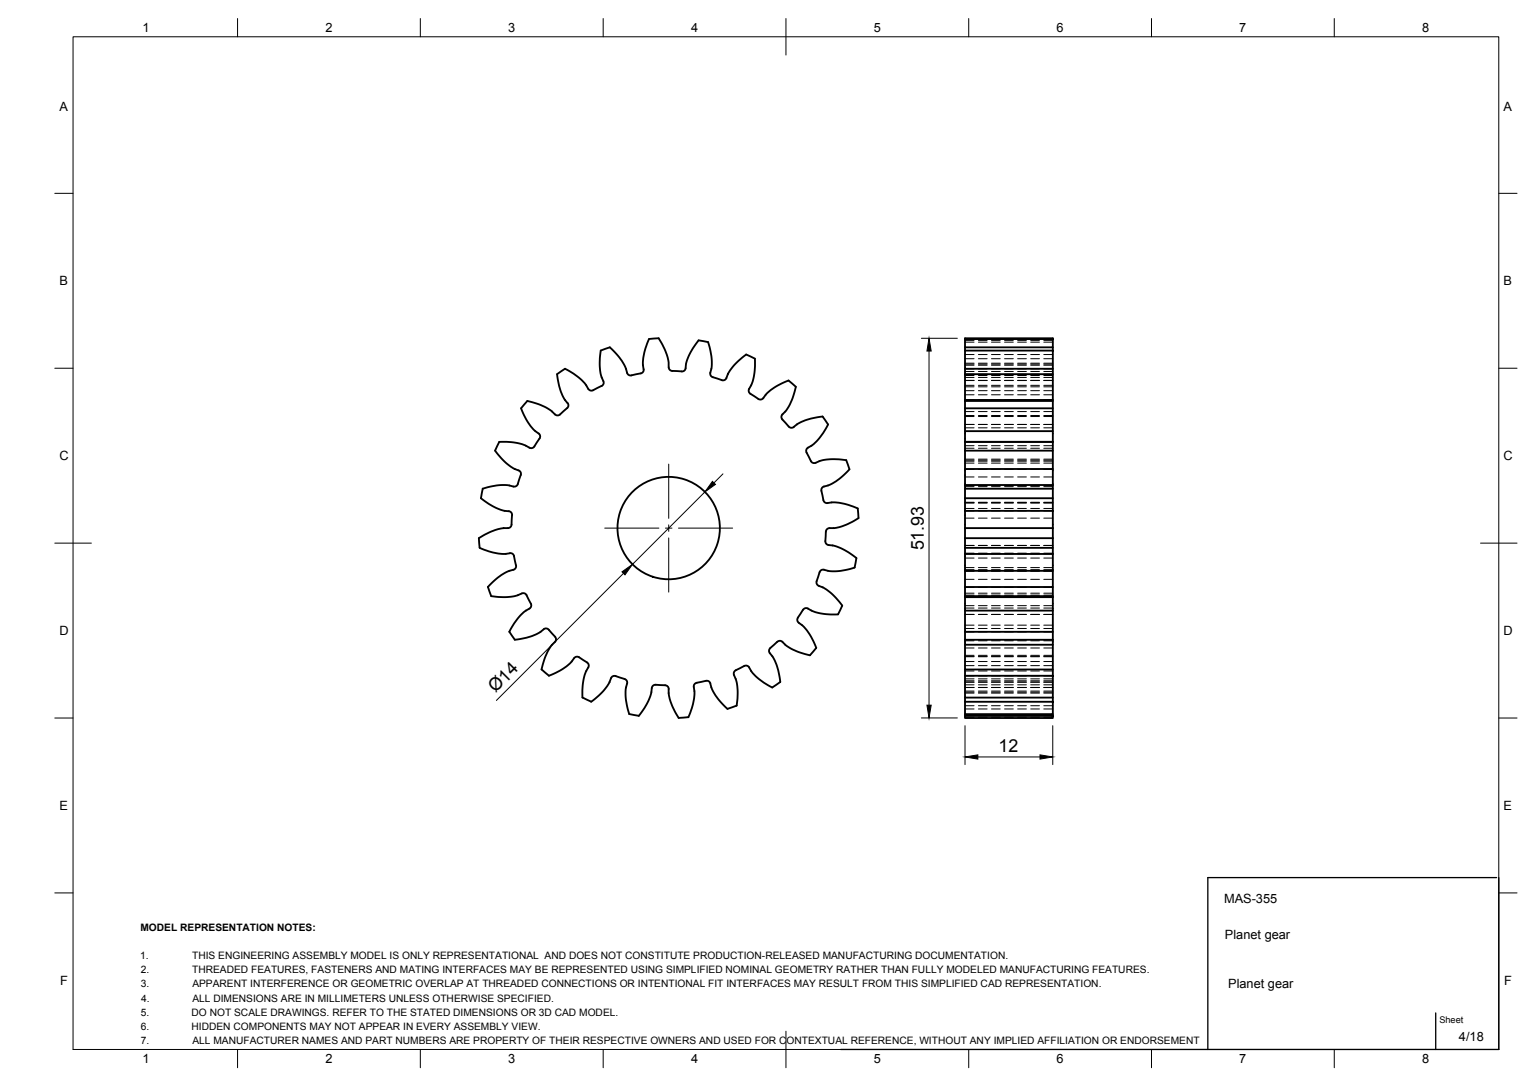
ISO-10303-21;
HEADER;
/* Generated by software containing ST-Developer
 * from STEP Tools, Inc. (www.steptools.com) 
 */

FILE_DESCRIPTION(
/* description */ ('Independent two-stage fixed-ring planetary gearbox,24/24/72 teeth,mod
ule2,20deg involutes,three planets per stage,4:1 x4:1=16:1. Native cut
-space/fillet/pattern tooth profiles derived from reusable gear blanks
; shared sun/planet/ring/carrier parts across both stages. Captured br
onze-journal input/carriers, headed retained planet pins, keyed inters
tage drive and modular keyed output interface. Native ideal gear links
; no torque, precision grade, production backlash/fits, lubrication, s
peed or life rating.'),
/* implementation_level */ '2;1');

FILE_NAME(
/* name */ 'Planet gear.step',
/* time_stamp */ '2026-11-08T19:10:00-08:00',
/* author */ (''),
/* organization */ (''),
/* preprocessor_version */ 'ST-DEVELOPER v20.2',
/* originating_system */ 'Autodesk Translation Framework v15.17.0.0',
/* authorisation */ '');

FILE_SCHEMA (('AUTOMOTIVE_DESIGN { 1 0 10303 214 3 1 1 }'));
ENDSEC;

DATA;
#10=MECHANICAL_DESIGN_GEOMETRIC_PRESENTATION_REPRESENTATION('',(#1169),#259224);
#787=(
BOUNDED_CURVE()
B_SPLINE_CURVE(5,(#216419,#216420,#216421,#216422,#216423,#216424,#216425,
#216426,#216427,#216428,#216429,#216430,#216431,#216432,#216433,#216434,
#216435,#216436,#216437,#216438,#216439,#216440,#216441,#216442,#216443,
#216444,#216445,#216446,#216447,#216448,#216449,#216450,#216451,#216452,
#216453,#216454,#216455,#216456,#216457,#216458,#216459,#216460,#216461,
#216462,#216463,#216464,#216465,#216466,#216467,#216468,#216469,#216470,
#216471,#216472,#216473,#216474,#216475,#216476,#216477,#216478,#216479,
#216480,#216481,#216482,#216483,#216484,#216485,#216486,#216487,#216488,
#216489,#216490,#216491,#216492,#216493,#216494,#216495,#216496,#216497,
#216498,#216499,#216500,#216501,#216502,#216503,#216504,#216505,#216506,
#216507,#216508,#216509,#216510,#216511,#216512,#216513,#216514,#216515,
#216516,#216517,#216518,#216519,#216520,#216521,#216522,#216523,#216524,
#216525,#216526,#216527,#216528,#216529,#216530,#216531,#216532,#216533,
#216534,#216535,#216536,#216537,#216538,#216539,#216540,#216541,#216542,
#216543,#216544,#216545,#216546,#216547,#216548,#216549,#216550,#216551,
#216552,#216553,#216554,#216555,#216556,#216557,#216558,#216559,#216560,
#216561,#216562,#216563,#216564,#216565,#216566,#216567,#216568,#216569,
#216570,#216571,#216572,#216573,#216574,#216575,#216576,#216577,#216578,
#216579,#216580,#216581,#216582,#216583,#216584,#216585,#216586,#216587,
#216588,#216589,#216590,#216591,#216592,#216593,#216594,#216595,#216596,
#216597,#216598,#216599,#216600,#216601,#216602,#216603,#216604,#216605,
#216606,#216607,#216608,#216609,#216610,#216611,#216612,#216613,#216614,
#216615,#216616,#216617,#216618,#216619,#216620,#216621,#216622,#216623),
 .UNSPECIFIED.,.F.,.F.)
B_SPLINE_CURVE_WITH_KNOTS((6,1,1,1,1,1,1,1,1,1,1,1,1,1,1,1,1,1,1,1,1,1,
1,1,1,1,1,1,1,1,1,1,1,1,1,1,1,1,1,1,1,1,1,1,1,1,1,1,1,1,1,1,1,1,1,1,1,1,
1,1,1,1,1,1,1,1,1,1,1,1,1,1,1,1,1,1,1,1,1,1,1,1,1,1,1,1,1,1,1,1,1,1,1,1,
1,1,1,1,1,1,1,1,1,1,1,1,1,1,1,1,1,1,1,1,1,1,1,1,1,1,1,1,1,1,1,1,1,1,1,1,
1,1,1,1,1,1,1,1,1,1,1,1,1,1,1,1,1,1,1,1,1,1,1,1,1,1,1,1,1,1,1,1,1,1,1,1,
1,1,1,1,1,1,1,1,1,1,1,1,1,1,1,1,1,1,1,1,1,1,1,1,1,1,1,1,1,1,1,1,1,1,6),
(-1.,-0.995000000000001,-0.990000000000001,-0.985000000000001,-0.980000000000001,
-0.975000000000001,-0.970000000000001,-0.965000000000001,-0.960000000000001,
-0.955000000000001,-0.950000000000001,-0.945000000000001,-0.940000000000001,
-0.935000000000001,-0.930000000000001,-0.925000000000001,-0.920000000000001,
-0.915000000000001,-0.910000000000001,-0.905000000000001,-0.900000000000001,
-0.895000000000001,-0.890000000000001,-0.885000000000001,-0.880000000000001,
-0.875000000000001,-0.870000000000001,-0.865000000000001,-0.860000000000001,
-0.855000000000001,-0.850000000000001,-0.845000000000001,-0.840000000000001,
-0.835000000000001,-0.830000000000001,-0.825000000000001,-0.820000000000001,
-0.815000000000001,-0.810000000000001,-0.805000000000001,-0.800000000000001,
-0.795000000000001,-0.790000000000001,-0.785000000000001,-0.780000000000001,
-0.775000000000001,-0.770000000000001,-0.765000000000001,-0.760000000000001,
-0.755000000000001,-0.750000000000001,-0.745000000000001,-0.740000000000001,
-0.735000000000001,-0.730000000000001,-0.725000000000001,-0.720000000000001,
-0.715000000000001,-0.710000000000001,-0.705000000000001,-0.700000000000001,
-0.695000000000001,-0.690000000000001,-0.685,-0.68,-0.675,-0.67,-0.665,
-0.66,-0.655,-0.65,-0.645,-0.64,-0.635,-0.63,-0.625,-0.62,-0.615,-0.61,
-0.605,-0.6,-0.595,-0.59,-0.585,-0.58,-0.575,-0.57,-0.565,-0.56,-0.555,
-0.55,-0.545,-0.54,-0.535,-0.53,-0.525,-0.52,-0.515,-0.51,-0.505,-0.5,-0.495,
-0.49,-0.485,-0.48,-0.475,-0.47,-0.465,-0.46,-0.455,-0.45,-0.445,-0.44,
-0.435,-0.43,-0.425,-0.42,-0.415,-0.41,-0.405,-0.4,-0.395,-0.39,-0.385,
-0.38,-0.375,-0.37,-0.365,-0.36,-0.355,-0.35,-0.345,-0.34,-0.335,-0.33,
-0.325,-0.32,-0.315,-0.31,-0.305,-0.3,-0.295,-0.29,-0.285,-0.28,-0.275,
-0.27,-0.265,-0.26,-0.255,-0.25,-0.245,-0.24,-0.235,-0.23,-0.225,-0.22,
-0.215,-0.21,-0.205,-0.2,-0.195,-0.19,-0.185,-0.18,-0.175,-0.17,-0.165,
-0.16,-0.155,-0.15,-0.145,-0.14,-0.135,-0.13,-0.125,-0.12,-0.115,-0.11,
-0.105,-0.1,-0.095,-0.09,-0.085,-0.08,-0.075,-0.07,-0.065,-0.06,-0.055,
-0.05,-0.045,-0.04,-0.035,-0.03,-0.025,-0.02,-0.015,-0.01,-0.005,0.),
 .UNSPECIFIED.)
CURVE()
GEOMETRIC_REPRESENTATION_ITEM()
RATIONAL_B_SPLINE_CURVE((1.,1.,1.,1.,1.,1.,1.,1.,1.,1.,1.,1.,1.,1.,1.,1.,
1.,1.,1.,1.,1.,1.,1.,1.,1.,1.,1.,1.,1.,1.,1.,1.,1.,1.,1.,1.,1.,1.,1.,1.,
1.,1.,1.,1.,1.,1.,1.,1.,1.,1.,1.,1.,1.,1.,1.,1.,1.,1.,1.,1.,1.,1.,1.,1.,
1.,1.,1.,1.,1.,1.,1.,1.,1.,1.,1.,1.,1.,1.,1.,1.,1.,1.,1.,1.,1.,1.,1.,1.,
1.,1.,1.,1.,1.,1.,1.,1.,1.,1.,1.,1.,1.,1.,1.,1.,1.,1.,1.,1.,1.,1.,1.,1.,
1.,1.,1.,1.,1.,1.,1.,1.,1.,1.,1.,1.,1.,1.,1.,1.,1.,1.,1.,1.,1.,1.,1.,1.,
1.,1.,1.,1.,1.,1.,1.,1.,1.,1.,1.,1.,1.,1.,1.,1.,1.,1.,1.,1.,1.,1.,1.,1.,
1.,1.,1.,1.,1.,1.,1.,1.,1.,1.,1.,1.,1.,1.,1.,1.,1.,1.,1.,1.,1.,1.,1.,1.,
1.,1.,1.,1.,1.,1.,1.,1.,1.,1.,1.,1.,1.,1.,1.,1.,1.,1.,1.,1.,1.))
REPRESENTATION_ITEM('')
);
#788=(
BOUNDED_CURVE()
B_SPLINE_CURVE(5,(#216626,#216627,#216628,#216629,#216630,#216631,#216632,
#216633,#216634,#216635,#216636,#216637,#216638,#216639,#216640,#216641,
#216642,#216643,#216644,#216645,#216646,#216647,#216648,#216649,#216650,
#216651,#216652,#216653,#216654,#216655,#216656,#216657,#216658,#216659,
#216660,#216661,#216662,#216663,#216664,#216665,#216666,#216667,#216668,
#216669,#216670,#216671,#216672,#216673,#216674,#216675,#216676,#216677,
#216678,#216679,#216680,#216681,#216682,#216683,#216684,#216685,#216686,
#216687,#216688,#216689,#216690,#216691,#216692,#216693,#216694,#216695,
#216696,#216697,#216698,#216699,#216700,#216701,#216702,#216703,#216704,
#216705,#216706,#216707,#216708,#216709,#216710,#216711,#216712,#216713,
#216714,#216715,#216716,#216717,#216718,#216719,#216720,#216721,#216722,
#216723,#216724,#216725,#216726,#216727,#216728,#216729,#216730,#216731,
#216732,#216733,#216734,#216735,#216736,#216737,#216738,#216739,#216740,
#216741,#216742,#216743,#216744,#216745,#216746,#216747,#216748,#216749,
#216750,#216751,#216752,#216753,#216754,#216755,#216756,#216757,#216758,
#216759,#216760,#216761,#216762,#216763,#216764,#216765,#216766,#216767,
#216768,#216769,#216770,#216771,#216772,#216773,#216774,#216775,#216776,
#216777,#216778,#216779,#216780,#216781,#216782,#216783,#216784,#216785,
#216786,#216787,#216788,#216789,#216790,#216791,#216792,#216793,#216794,
#216795,#216796,#216797,#216798,#216799,#216800,#216801,#216802,#216803,
#216804,#216805,#216806,#216807,#216808,#216809,#216810,#216811,#216812,
#216813,#216814,#216815,#216816,#216817,#216818,#216819,#216820,#216821,
#216822,#216823,#216824,#216825,#216826,#216827,#216828,#216829,#216830),
 .UNSPECIFIED.,.F.,.F.)
B_SPLINE_CURVE_WITH_KNOTS((6,1,1,1,1,1,1,1,1,1,1,1,1,1,1,1,1,1,1,1,1,1,
1,1,1,1,1,1,1,1,1,1,1,1,1,1,1,1,1,1,1,1,1,1,1,1,1,1,1,1,1,1,1,1,1,1,1,1,
1,1,1,1,1,1,1,1,1,1,1,1,1,1,1,1,1,1,1,1,1,1,1,1,1,1,1,1,1,1,1,1,1,1,1,1,
1,1,1,1,1,1,1,1,1,1,1,1,1,1,1,1,1,1,1,1,1,1,1,1,1,1,1,1,1,1,1,1,1,1,1,1,
1,1,1,1,1,1,1,1,1,1,1,1,1,1,1,1,1,1,1,1,1,1,1,1,1,1,1,1,1,1,1,1,1,1,1,1,
1,1,1,1,1,1,1,1,1,1,1,1,1,1,1,1,1,1,1,1,1,1,1,1,1,1,1,1,1,1,1,1,1,1,6),
(0.,0.005,0.01,0.015,0.02,0.025,0.03,0.035,0.04,0.045,0.05,0.055,0.06,0.065,
0.07,0.075,0.08,0.085,0.09,0.095,0.1,0.105,0.11,0.115,0.12,0.125,0.13,0.135,
0.14,0.145,0.15,0.155,0.16,0.165,0.17,0.175,0.18,0.185,0.19,0.195,0.2,0.205,
0.21,0.215,0.22,0.225,0.23,0.235,0.24,0.245,0.25,0.255,0.26,0.265,0.27,
0.275,0.28,0.285,0.29,0.295,0.3,0.305,0.31,0.315,0.32,0.325,0.33,0.335,
0.34,0.345,0.35,0.355,0.36,0.365,0.37,0.375,0.38,0.385,0.39,0.395,0.4,0.405,
0.41,0.415,0.42,0.425,0.43,0.435,0.44,0.445,0.45,0.455,0.46,0.465,0.47,
0.475,0.48,0.485,0.49,0.495,0.5,0.505,0.51,0.515,0.52,0.525,0.53,0.535,
0.54,0.545,0.55,0.555,0.56,0.565,0.57,0.575,0.58,0.585,0.59,0.595,0.6,0.605,
0.61,0.615,0.62,0.625,0.63,0.635,0.64,0.645,0.65,0.655,0.66,0.665,0.67,
0.675,0.68,0.685,0.690000000000001,0.695000000000001,0.700000000000001,
0.705000000000001,0.710000000000001,0.715000000000001,0.720000000000001,
0.725000000000001,0.730000000000001,0.735000000000001,0.740000000000001,
0.745000000000001,0.750000000000001,0.755000000000001,0.760000000000001,
0.765000000000001,0.770000000000001,0.775000000000001,0.780000000000001,
0.785000000000001,0.790000000000001,0.795000000000001,0.800000000000001,
0.805000000000001,0.810000000000001,0.815000000000001,0.820000000000001,
0.825000000000001,0.830000000000001,0.835000000000001,0.840000000000001,
0.845000000000001,0.850000000000001,0.855000000000001,0.860000000000001,
0.865000000000001,0.870000000000001,0.875000000000001,0.880000000000001,
0.885000000000001,0.890000000000001,0.895000000000001,0.900000000000001,
0.905000000000001,0.910000000000001,0.915000000000001,0.920000000000001,
0.925000000000001,0.930000000000001,0.935000000000001,0.940000000000001,
0.945000000000001,0.950000000000001,0.955000000000001,0.960000000000001,
0.965000000000001,0.970000000000001,0.975000000000001,0.980000000000001,
0.985000000000001,0.990000000000001,0.995000000000001,1.),.UNSPECIFIED.)
CURVE()
GEOMETRIC_REPRESENTATION_ITEM()
RATIONAL_B_SPLINE_CURVE((1.,1.,1.,1.,1.,1.,1.,1.,1.,1.,1.,1.,1.,1.,1.,1.,
1.,1.,1.,1.,1.,1.,1.,1.,1.,1.,1.,1.,1.,1.,1.,1.,1.,1.,1.,1.,1.,1.,1.,1.,
1.,1.,1.,1.,1.,1.,1.,1.,1.,1.,1.,1.,1.,1.,1.,1.,1.,1.,1.,1.,1.,1.,1.,1.,
1.,1.,1.,1.,1.,1.,1.,1.,1.,1.,1.,1.,1.,1.,1.,1.,1.,1.,1.,1.,1.,1.,1.,1.,
1.,1.,1.,1.,1.,1.,1.,1.,1.,1.,1.,1.,1.,1.,1.,1.,1.,1.,1.,1.,1.,1.,1.,1.,
1.,1.,1.,1.,1.,1.,1.,1.,1.,1.,1.,1.,1.,1.,1.,1.,1.,1.,1.,1.,1.,1.,1.,1.,
1.,1.,1.,1.,1.,1.,1.,1.,1.,1.,1.,1.,1.,1.,1.,1.,1.,1.,1.,1.,1.,1.,1.,1.,
1.,1.,1.,1.,1.,1.,1.,1.,1.,1.,1.,1.,1.,1.,1.,1.,1.,1.,1.,1.,1.,1.,1.,1.,
1.,1.,1.,1.,1.,1.,1.,1.,1.,1.,1.,1.,1.,1.,1.,1.,1.,1.,1.,1.,1.))
REPRESENTATION_ITEM('')
);
#789=(
BOUNDED_CURVE()
B_SPLINE_CURVE(5,(#217242,#217243,#217244,#217245,#217246,#217247,#217248,
#217249,#217250,#217251,#217252,#217253,#217254,#217255,#217256,#217257,
#217258,#217259,#217260,#217261,#217262,#217263,#217264,#217265,#217266,
#217267,#217268,#217269,#217270,#217271,#217272,#217273,#217274,#217275,
#217276,#217277,#217278,#217279,#217280,#217281,#217282,#217283,#217284,
#217285,#217286,#217287,#217288,#217289,#217290,#217291,#217292,#217293,
#217294,#217295,#217296,#217297,#217298,#217299,#217300,#217301,#217302,
#217303,#217304,#217305,#217306,#217307,#217308,#217309,#217310,#217311,
#217312,#217313,#217314,#217315,#217316,#217317,#217318,#217319,#217320,
#217321,#217322,#217323,#217324,#217325,#217326,#217327,#217328,#217329,
#217330,#217331,#217332,#217333,#217334,#217335,#217336,#217337,#217338,
#217339,#217340,#217341,#217342,#217343,#217344,#217345,#217346,#217347,
#217348,#217349,#217350,#217351,#217352,#217353,#217354,#217355,#217356,
#217357,#217358,#217359,#217360,#217361,#217362,#217363,#217364,#217365,
#217366,#217367,#217368,#217369,#217370,#217371,#217372,#217373,#217374,
#217375,#217376,#217377,#217378,#217379,#217380,#217381,#217382,#217383,
#217384,#217385,#217386,#217387,#217388,#217389,#217390,#217391,#217392,
#217393,#217394,#217395,#217396,#217397,#217398,#217399,#217400,#217401,
#217402,#217403,#217404,#217405,#217406,#217407,#217408,#217409,#217410,
#217411,#217412,#217413,#217414,#217415,#217416,#217417,#217418,#217419,
#217420,#217421,#217422,#217423,#217424,#217425,#217426,#217427,#217428,
#217429,#217430,#217431,#217432,#217433,#217434,#217435,#217436,#217437,
#217438,#217439,#217440,#217441,#217442,#217443,#217444,#217445,#217446),
 .UNSPECIFIED.,.F.,.F.)
B_SPLINE_CURVE_WITH_KNOTS((6,1,1,1,1,1,1,1,1,1,1,1,1,1,1,1,1,1,1,1,1,1,
1,1,1,1,1,1,1,1,1,1,1,1,1,1,1,1,1,1,1,1,1,1,1,1,1,1,1,1,1,1,1,1,1,1,1,1,
1,1,1,1,1,1,1,1,1,1,1,1,1,1,1,1,1,1,1,1,1,1,1,1,1,1,1,1,1,1,1,1,1,1,1,1,
1,1,1,1,1,1,1,1,1,1,1,1,1,1,1,1,1,1,1,1,1,1,1,1,1,1,1,1,1,1,1,1,1,1,1,1,
1,1,1,1,1,1,1,1,1,1,1,1,1,1,1,1,1,1,1,1,1,1,1,1,1,1,1,1,1,1,1,1,1,1,1,1,
1,1,1,1,1,1,1,1,1,1,1,1,1,1,1,1,1,1,1,1,1,1,1,1,1,1,1,1,1,1,1,1,1,1,6),
(0.,0.005,0.01,0.015,0.02,0.025,0.03,0.035,0.04,0.045,0.05,0.055,0.06,0.065,
0.07,0.075,0.08,0.085,0.09,0.095,0.1,0.105,0.11,0.115,0.12,0.125,0.13,0.135,
0.14,0.145,0.15,0.155,0.16,0.165,0.17,0.175,0.18,0.185,0.19,0.195,0.2,0.205,
0.21,0.215,0.22,0.225,0.23,0.235,0.24,0.245,0.25,0.255,0.26,0.265,0.27,
0.275,0.28,0.285,0.29,0.295,0.3,0.305,0.31,0.315,0.32,0.325,0.33,0.335,
0.34,0.345,0.35,0.355,0.36,0.365,0.37,0.375,0.38,0.385,0.39,0.395,0.4,0.405,
0.41,0.415,0.42,0.425,0.43,0.435,0.44,0.445,0.45,0.455,0.46,0.465,0.47,
0.475,0.48,0.485,0.49,0.495,0.5,0.505,0.51,0.515,0.52,0.525,0.53,0.535,
0.54,0.545,0.55,0.555,0.56,0.565,0.57,0.575,0.58,0.585,0.59,0.595,0.6,0.605,
0.61,0.615,0.62,0.625,0.63,0.635,0.64,0.645,0.65,0.655,0.66,0.665,0.67,
0.675,0.68,0.685,0.690000000000001,0.695000000000001,0.700000000000001,
0.705000000000001,0.710000000000001,0.715000000000001,0.720000000000001,
0.725000000000001,0.730000000000001,0.735000000000001,0.740000000000001,
0.745000000000001,0.750000000000001,0.755000000000001,0.760000000000001,
0.765000000000001,0.770000000000001,0.775000000000001,0.780000000000001,
0.785000000000001,0.790000000000001,0.795000000000001,0.800000000000001,
0.805000000000001,0.810000000000001,0.815000000000001,0.820000000000001,
0.825000000000001,0.830000000000001,0.835000000000001,0.840000000000001,
0.845000000000001,0.850000000000001,0.855000000000001,0.860000000000001,
0.865000000000001,0.870000000000001,0.875000000000001,0.880000000000001,
0.885000000000001,0.890000000000001,0.895000000000001,0.900000000000001,
0.905000000000001,0.910000000000001,0.915000000000001,0.920000000000001,
0.925000000000001,0.930000000000001,0.935000000000001,0.940000000000001,
0.945000000000001,0.950000000000001,0.955000000000001,0.960000000000001,
0.965000000000001,0.970000000000001,0.975000000000001,0.980000000000001,
0.985000000000001,0.990000000000001,0.995000000000001,1.),.UNSPECIFIED.)
CURVE()
GEOMETRIC_REPRESENTATION_ITEM()
RATIONAL_B_SPLINE_CURVE((1.,1.,1.,1.,1.,1.,1.,1.,1.,1.,1.,1.,1.,1.,1.,1.,
1.,1.,1.,1.,1.,1.,1.,1.,1.,1.,1.,1.,1.,1.,1.,1.,1.,1.,1.,1.,1.,1.,1.,1.,
1.,1.,1.,1.,1.,1.,1.,1.,1.,1.,1.,1.,1.,1.,1.,1.,1.,1.,1.,1.,1.,1.,1.,1.,
1.,1.,1.,1.,1.,1.,1.,1.,1.,1.,1.,1.,1.,1.,1.,1.,1.,1.,1.,1.,1.,1.,1.,1.,
1.,1.,1.,1.,1.,1.,1.,1.,1.,1.,1.,1.,1.,1.,1.,1.,1.,1.,1.,1.,1.,1.,1.,1.,
1.,1.,1.,1.,1.,1.,1.,1.,1.,1.,1.,1.,1.,1.,1.,1.,1.,1.,1.,1.,1.,1.,1.,1.,
1.,1.,1.,1.,1.,1.,1.,1.,1.,1.,1.,1.,1.,1.,1.,1.,1.,1.,1.,1.,1.,1.,1.,1.,
1.,1.,1.,1.,1.,1.,1.,1.,1.,1.,1.,1.,1.,1.,1.,1.,1.,1.,1.,1.,1.,1.,1.,1.,
1.,1.,1.,1.,1.,1.,1.,1.,1.,1.,1.,1.,1.,1.,1.,1.,1.,1.,1.,1.,1.))
REPRESENTATION_ITEM('')
);
#790=(
BOUNDED_CURVE()
B_SPLINE_CURVE(5,(#217448,#217449,#217450,#217451,#217452,#217453,#217454,
#217455,#217456,#217457,#217458,#217459,#217460,#217461,#217462,#217463,
#217464,#217465,#217466,#217467,#217468,#217469,#217470,#217471,#217472,
#217473,#217474,#217475,#217476,#217477,#217478,#217479,#217480,#217481,
#217482,#217483,#217484,#217485,#217486,#217487,#217488,#217489,#217490,
#217491,#217492,#217493,#217494,#217495,#217496,#217497,#217498,#217499,
#217500,#217501,#217502,#217503,#217504,#217505,#217506,#217507,#217508,
#217509,#217510,#217511,#217512,#217513,#217514,#217515,#217516,#217517,
#217518,#217519,#217520,#217521,#217522,#217523,#217524,#217525,#217526,
#217527,#217528,#217529,#217530,#217531,#217532,#217533,#217534,#217535,
#217536,#217537,#217538,#217539,#217540,#217541,#217542,#217543,#217544,
#217545,#217546,#217547,#217548,#217549,#217550,#217551,#217552,#217553,
#217554,#217555,#217556,#217557,#217558,#217559,#217560,#217561,#217562,
#217563,#217564,#217565,#217566,#217567,#217568,#217569,#217570,#217571,
#217572,#217573,#217574,#217575,#217576,#217577,#217578,#217579,#217580,
#217581,#217582,#217583,#217584,#217585,#217586,#217587,#217588,#217589,
#217590,#217591,#217592,#217593,#217594,#217595,#217596,#217597,#217598,
#217599,#217600,#217601,#217602,#217603,#217604,#217605,#217606,#217607,
#217608,#217609,#217610,#217611,#217612,#217613,#217614,#217615,#217616,
#217617,#217618,#217619,#217620,#217621,#217622,#217623,#217624,#217625,
#217626,#217627,#217628,#217629,#217630,#217631,#217632,#217633,#217634,
#217635,#217636,#217637,#217638,#217639,#217640,#217641,#217642,#217643,
#217644,#217645,#217646,#217647,#217648,#217649,#217650,#217651,#217652),
 .UNSPECIFIED.,.F.,.F.)
B_SPLINE_CURVE_WITH_KNOTS((6,1,1,1,1,1,1,1,1,1,1,1,1,1,1,1,1,1,1,1,1,1,
1,1,1,1,1,1,1,1,1,1,1,1,1,1,1,1,1,1,1,1,1,1,1,1,1,1,1,1,1,1,1,1,1,1,1,1,
1,1,1,1,1,1,1,1,1,1,1,1,1,1,1,1,1,1,1,1,1,1,1,1,1,1,1,1,1,1,1,1,1,1,1,1,
1,1,1,1,1,1,1,1,1,1,1,1,1,1,1,1,1,1,1,1,1,1,1,1,1,1,1,1,1,1,1,1,1,1,1,1,
1,1,1,1,1,1,1,1,1,1,1,1,1,1,1,1,1,1,1,1,1,1,1,1,1,1,1,1,1,1,1,1,1,1,1,1,
1,1,1,1,1,1,1,1,1,1,1,1,1,1,1,1,1,1,1,1,1,1,1,1,1,1,1,1,1,1,1,1,1,1,6),
(-1.,-0.995000000000001,-0.990000000000001,-0.985000000000001,-0.980000000000001,
-0.975000000000001,-0.970000000000001,-0.965000000000001,-0.960000000000001,
-0.955000000000001,-0.950000000000001,-0.945000000000001,-0.940000000000001,
-0.935000000000001,-0.930000000000001,-0.925000000000001,-0.920000000000001,
-0.915000000000001,-0.910000000000001,-0.905000000000001,-0.900000000000001,
-0.895000000000001,-0.890000000000001,-0.885000000000001,-0.880000000000001,
-0.875000000000001,-0.870000000000001,-0.865000000000001,-0.860000000000001,
-0.855000000000001,-0.850000000000001,-0.845000000000001,-0.840000000000001,
-0.835000000000001,-0.830000000000001,-0.825000000000001,-0.820000000000001,
-0.815000000000001,-0.810000000000001,-0.805000000000001,-0.800000000000001,
-0.795000000000001,-0.790000000000001,-0.785000000000001,-0.780000000000001,
-0.775000000000001,-0.770000000000001,-0.765000000000001,-0.760000000000001,
-0.755000000000001,-0.750000000000001,-0.745000000000001,-0.740000000000001,
-0.735000000000001,-0.730000000000001,-0.725000000000001,-0.720000000000001,
-0.715000000000001,-0.710000000000001,-0.705000000000001,-0.700000000000001,
-0.695000000000001,-0.690000000000001,-0.685,-0.68,-0.675,-0.67,-0.665,
-0.66,-0.655,-0.65,-0.645,-0.64,-0.635,-0.63,-0.625,-0.62,-0.615,-0.61,
-0.605,-0.6,-0.595,-0.59,-0.585,-0.58,-0.575,-0.57,-0.565,-0.56,-0.555,
-0.55,-0.545,-0.54,-0.535,-0.53,-0.525,-0.52,-0.515,-0.51,-0.505,-0.5,-0.495,
-0.49,-0.485,-0.48,-0.475,-0.47,-0.465,-0.46,-0.455,-0.45,-0.445,-0.44,
-0.435,-0.43,-0.425,-0.42,-0.415,-0.41,-0.405,-0.4,-0.395,-0.39,-0.385,
-0.38,-0.375,-0.37,-0.365,-0.36,-0.355,-0.35,-0.345,-0.34,-0.335,-0.33,
-0.325,-0.32,-0.315,-0.31,-0.305,-0.3,-0.295,-0.29,-0.285,-0.28,-0.275,
-0.27,-0.265,-0.26,-0.255,-0.25,-0.245,-0.24,-0.235,-0.23,-0.225,-0.22,
-0.215,-0.21,-0.205,-0.2,-0.195,-0.19,-0.185,-0.18,-0.175,-0.17,-0.165,
-0.16,-0.155,-0.15,-0.145,-0.14,-0.135,-0.13,-0.125,-0.12,-0.115,-0.11,
-0.105,-0.1,-0.095,-0.09,-0.085,-0.08,-0.075,-0.07,-0.065,-0.06,-0.055,
-0.05,-0.045,-0.04,-0.035,-0.03,-0.025,-0.02,-0.015,-0.01,-0.005,0.),
 .UNSPECIFIED.)
CURVE()
GEOMETRIC_REPRESENTATION_ITEM()
RATIONAL_B_SPLINE_CURVE((1.,1.,1.,1.,1.,1.,1.,1.,1.,1.,1.,1.,1.,1.,1.,1.,
1.,1.,1.,1.,1.,1.,1.,1.,1.,1.,1.,1.,1.,1.,1.,1.,1.,1.,1.,1.,1.,1.,1.,1.,
1.,1.,1.,1.,1.,1.,1.,1.,1.,1.,1.,1.,1.,1.,1.,1.,1.,1.,1.,1.,1.,1.,1.,1.,
1.,1.,1.,1.,1.,1.,1.,1.,1.,1.,1.,1.,1.,1.,1.,1.,1.,1.,1.,1.,1.,1.,1.,1.,
1.,1.,1.,1.,1.,1.,1.,1.,1.,1.,1.,1.,1.,1.,1.,1.,1.,1.,1.,1.,1.,1.,1.,1.,
1.,1.,1.,1.,1.,1.,1.,1.,1.,1.,1.,1.,1.,1.,1.,1.,1.,1.,1.,1.,1.,1.,1.,1.,
1.,1.,1.,1.,1.,1.,1.,1.,1.,1.,1.,1.,1.,1.,1.,1.,1.,1.,1.,1.,1.,1.,1.,1.,
1.,1.,1.,1.,1.,1.,1.,1.,1.,1.,1.,1.,1.,1.,1.,1.,1.,1.,1.,1.,1.,1.,1.,1.,
1.,1.,1.,1.,1.,1.,1.,1.,1.,1.,1.,1.,1.,1.,1.,1.,1.,1.,1.,1.,1.))
REPRESENTATION_ITEM('')
);
#791=(
BOUNDED_CURVE()
B_SPLINE_CURVE(5,(#218071,#218072,#218073,#218074,#218075,#218076,#218077,
#218078,#218079,#218080,#218081,#218082,#218083,#218084,#218085,#218086,
#218087,#218088,#218089,#218090,#218091,#218092,#218093,#218094,#218095,
#218096,#218097,#218098,#218099,#218100,#218101,#218102,#218103,#218104,
#218105,#218106,#218107,#218108,#218109,#218110,#218111,#218112,#218113,
#218114,#218115,#218116,#218117,#218118,#218119,#218120,#218121,#218122,
#218123,#218124,#218125,#218126,#218127,#218128,#218129,#218130,#218131,
#218132,#218133,#218134,#218135,#218136,#218137,#218138,#218139,#218140,
#218141,#218142,#218143,#218144,#218145,#218146,#218147,#218148,#218149,
#218150,#218151,#218152,#218153,#218154,#218155,#218156,#218157,#218158,
#218159,#218160,#218161,#218162,#218163,#218164,#218165,#218166,#218167,
#218168,#218169,#218170,#218171,#218172,#218173,#218174,#218175,#218176,
#218177,#218178,#218179,#218180,#218181,#218182,#218183,#218184,#218185,
#218186,#218187,#218188,#218189,#218190,#218191,#218192,#218193,#218194,
#218195,#218196,#218197,#218198,#218199,#218200,#218201,#218202,#218203,
#218204,#218205,#218206,#218207,#218208,#218209,#218210,#218211,#218212,
#218213,#218214,#218215,#218216,#218217,#218218,#218219,#218220,#218221,
#218222,#218223,#218224,#218225,#218226,#218227,#218228,#218229,#218230,
#218231,#218232,#218233,#218234,#218235,#218236,#218237,#218238,#218239,
#218240,#218241,#218242,#218243,#218244,#218245,#218246,#218247,#218248,
#218249,#218250,#218251,#218252,#218253,#218254,#218255,#218256,#218257,
#218258,#218259,#218260,#218261,#218262,#218263,#218264,#218265,#218266,
#218267,#218268,#218269,#218270,#218271,#218272,#218273,#218274,#218275),
 .UNSPECIFIED.,.F.,.F.)
B_SPLINE_CURVE_WITH_KNOTS((6,1,1,1,1,1,1,1,1,1,1,1,1,1,1,1,1,1,1,1,1,1,
1,1,1,1,1,1,1,1,1,1,1,1,1,1,1,1,1,1,1,1,1,1,1,1,1,1,1,1,1,1,1,1,1,1,1,1,
1,1,1,1,1,1,1,1,1,1,1,1,1,1,1,1,1,1,1,1,1,1,1,1,1,1,1,1,1,1,1,1,1,1,1,1,
1,1,1,1,1,1,1,1,1,1,1,1,1,1,1,1,1,1,1,1,1,1,1,1,1,1,1,1,1,1,1,1,1,1,1,1,
1,1,1,1,1,1,1,1,1,1,1,1,1,1,1,1,1,1,1,1,1,1,1,1,1,1,1,1,1,1,1,1,1,1,1,1,
1,1,1,1,1,1,1,1,1,1,1,1,1,1,1,1,1,1,1,1,1,1,1,1,1,1,1,1,1,1,1,1,1,1,6),
(-1.,-0.995000000000001,-0.990000000000001,-0.985000000000001,-0.980000000000001,
-0.975000000000001,-0.970000000000001,-0.965000000000001,-0.960000000000001,
-0.955000000000001,-0.950000000000001,-0.945000000000001,-0.940000000000001,
-0.935000000000001,-0.930000000000001,-0.925000000000001,-0.920000000000001,
-0.915000000000001,-0.910000000000001,-0.905000000000001,-0.900000000000001,
-0.895000000000001,-0.890000000000001,-0.885000000000001,-0.880000000000001,
-0.875000000000001,-0.870000000000001,-0.865000000000001,-0.860000000000001,
-0.855000000000001,-0.850000000000001,-0.845000000000001,-0.840000000000001,
-0.835000000000001,-0.830000000000001,-0.825000000000001,-0.820000000000001,
-0.815000000000001,-0.810000000000001,-0.805000000000001,-0.800000000000001,
-0.795000000000001,-0.790000000000001,-0.785000000000001,-0.780000000000001,
-0.775000000000001,-0.770000000000001,-0.765000000000001,-0.760000000000001,
-0.755000000000001,-0.750000000000001,-0.745000000000001,-0.740000000000001,
-0.735000000000001,-0.730000000000001,-0.725000000000001,-0.720000000000001,
-0.715000000000001,-0.710000000000001,-0.705000000000001,-0.700000000000001,
-0.695000000000001,-0.690000000000001,-0.685,-0.68,-0.675,-0.67,-0.665,
-0.66,-0.655,-0.65,-0.645,-0.64,-0.635,-0.63,-0.625,-0.62,-0.615,-0.61,
-0.605,-0.6,-0.595,-0.59,-0.585,-0.58,-0.575,-0.57,-0.565,-0.56,-0.555,
-0.55,-0.545,-0.54,-0.535,-0.53,-0.525,-0.52,-0.515,-0.51,-0.505,-0.5,-0.495,
-0.49,-0.485,-0.48,-0.475,-0.47,-0.465,-0.46,-0.455,-0.45,-0.445,-0.44,
-0.435,-0.43,-0.425,-0.42,-0.415,-0.41,-0.405,-0.4,-0.395,-0.39,-0.385,
-0.38,-0.375,-0.37,-0.365,-0.36,-0.355,-0.35,-0.345,-0.34,-0.335,-0.33,
-0.325,-0.32,-0.315,-0.31,-0.305,-0.3,-0.295,-0.29,-0.285,-0.28,-0.275,
-0.27,-0.265,-0.26,-0.255,-0.25,-0.245,-0.24,-0.235,-0.23,-0.225,-0.22,
-0.215,-0.21,-0.205,-0.2,-0.195,-0.19,-0.185,-0.18,-0.175,-0.17,-0.165,
-0.16,-0.155,-0.15,-0.145,-0.14,-0.135,-0.13,-0.125,-0.12,-0.115,-0.11,
-0.105,-0.1,-0.095,-0.09,-0.085,-0.08,-0.075,-0.07,-0.065,-0.06,-0.055,
-0.05,-0.045,-0.04,-0.035,-0.03,-0.025,-0.02,-0.015,-0.01,-0.005,0.),
 .UNSPECIFIED.)
CURVE()
GEOMETRIC_REPRESENTATION_ITEM()
RATIONAL_B_SPLINE_CURVE((1.,1.,1.,1.,1.,1.,1.,1.,1.,1.,1.,1.,1.,1.,1.,1.,
1.,1.,1.,1.,1.,1.,1.,1.,1.,1.,1.,1.,1.,1.,1.,1.,1.,1.,1.,1.,1.,1.,1.,1.,
1.,1.,1.,1.,1.,1.,1.,1.,1.,1.,1.,1.,1.,1.,1.,1.,1.,1.,1.,1.,1.,1.,1.,1.,
1.,1.,1.,1.,1.,1.,1.,1.,1.,1.,1.,1.,1.,1.,1.,1.,1.,1.,1.,1.,1.,1.,1.,1.,
1.,1.,1.,1.,1.,1.,1.,1.,1.,1.,1.,1.,1.,1.,1.,1.,1.,1.,1.,1.,1.,1.,1.,1.,
1.,1.,1.,1.,1.,1.,1.,1.,1.,1.,1.,1.,1.,1.,1.,1.,1.,1.,1.,1.,1.,1.,1.,1.,
1.,1.,1.,1.,1.,1.,1.,1.,1.,1.,1.,1.,1.,1.,1.,1.,1.,1.,1.,1.,1.,1.,1.,1.,
1.,1.,1.,1.,1.,1.,1.,1.,1.,1.,1.,1.,1.,1.,1.,1.,1.,1.,1.,1.,1.,1.,1.,1.,
1.,1.,1.,1.,1.,1.,1.,1.,1.,1.,1.,1.,1.,1.,1.,1.,1.,1.,1.,1.,1.))
REPRESENTATION_ITEM('')
);
#792=(
BOUNDED_CURVE()
B_SPLINE_CURVE(5,(#218278,#218279,#218280,#218281,#218282,#218283,#218284,
#218285,#218286,#218287,#218288,#218289,#218290,#218291,#218292,#218293,
#218294,#218295,#218296,#218297,#218298,#218299,#218300,#218301,#218302,
#218303,#218304,#218305,#218306,#218307,#218308,#218309,#218310,#218311,
#218312,#218313,#218314,#218315,#218316,#218317,#218318,#218319,#218320,
#218321,#218322,#218323,#218324,#218325,#218326,#218327,#218328,#218329,
#218330,#218331,#218332,#218333,#218334,#218335,#218336,#218337,#218338,
#218339,#218340,#218341,#218342,#218343,#218344,#218345,#218346,#218347,
#218348,#218349,#218350,#218351,#218352,#218353,#218354,#218355,#218356,
#218357,#218358,#218359,#218360,#218361,#218362,#218363,#218364,#218365,
#218366,#218367,#218368,#218369,#218370,#218371,#218372,#218373,#218374,
#218375,#218376,#218377,#218378,#218379,#218380,#218381,#218382,#218383,
#218384,#218385,#218386,#218387,#218388,#218389,#218390,#218391,#218392,
#218393,#218394,#218395,#218396,#218397,#218398,#218399,#218400,#218401,
#218402,#218403,#218404,#218405,#218406,#218407,#218408,#218409,#218410,
#218411,#218412,#218413,#218414,#218415,#218416,#218417,#218418,#218419,
#218420,#218421,#218422,#218423,#218424,#218425,#218426,#218427,#218428,
#218429,#218430,#218431,#218432,#218433,#218434,#218435,#218436,#218437,
#218438,#218439,#218440,#218441,#218442,#218443,#218444,#218445,#218446,
#218447,#218448,#218449,#218450,#218451,#218452,#218453,#218454,#218455,
#218456,#218457,#218458,#218459,#218460,#218461,#218462,#218463,#218464,
#218465,#218466,#218467,#218468,#218469,#218470,#218471,#218472,#218473,
#218474,#218475,#218476,#218477,#218478,#218479,#218480,#218481,#218482),
 .UNSPECIFIED.,.F.,.F.)
B_SPLINE_CURVE_WITH_KNOTS((6,1,1,1,1,1,1,1,1,1,1,1,1,1,1,1,1,1,1,1,1,1,
1,1,1,1,1,1,1,1,1,1,1,1,1,1,1,1,1,1,1,1,1,1,1,1,1,1,1,1,1,1,1,1,1,1,1,1,
1,1,1,1,1,1,1,1,1,1,1,1,1,1,1,1,1,1,1,1,1,1,1,1,1,1,1,1,1,1,1,1,1,1,1,1,
1,1,1,1,1,1,1,1,1,1,1,1,1,1,1,1,1,1,1,1,1,1,1,1,1,1,1,1,1,1,1,1,1,1,1,1,
1,1,1,1,1,1,1,1,1,1,1,1,1,1,1,1,1,1,1,1,1,1,1,1,1,1,1,1,1,1,1,1,1,1,1,1,
1,1,1,1,1,1,1,1,1,1,1,1,1,1,1,1,1,1,1,1,1,1,1,1,1,1,1,1,1,1,1,1,1,1,6),
(0.,0.005,0.01,0.015,0.02,0.025,0.03,0.035,0.04,0.045,0.05,0.055,0.06,0.065,
0.07,0.075,0.08,0.085,0.09,0.095,0.1,0.105,0.11,0.115,0.12,0.125,0.13,0.135,
0.14,0.145,0.15,0.155,0.16,0.165,0.17,0.175,0.18,0.185,0.19,0.195,0.2,0.205,
0.21,0.215,0.22,0.225,0.23,0.235,0.24,0.245,0.25,0.255,0.26,0.265,0.27,
0.275,0.28,0.285,0.29,0.295,0.3,0.305,0.31,0.315,0.32,0.325,0.33,0.335,
0.34,0.345,0.35,0.355,0.36,0.365,0.37,0.375,0.38,0.385,0.39,0.395,0.4,0.405,
0.41,0.415,0.42,0.425,0.43,0.435,0.44,0.445,0.45,0.455,0.46,0.465,0.47,
0.475,0.48,0.485,0.49,0.495,0.5,0.505,0.51,0.515,0.52,0.525,0.53,0.535,
0.54,0.545,0.55,0.555,0.56,0.565,0.57,0.575,0.58,0.585,0.59,0.595,0.6,0.605,
0.61,0.615,0.62,0.625,0.63,0.635,0.64,0.645,0.65,0.655,0.66,0.665,0.67,
0.675,0.68,0.685,0.690000000000001,0.695000000000001,0.700000000000001,
0.705000000000001,0.710000000000001,0.715000000000001,0.720000000000001,
0.725000000000001,0.730000000000001,0.735000000000001,0.740000000000001,
0.745000000000001,0.750000000000001,0.755000000000001,0.760000000000001,
0.765000000000001,0.770000000000001,0.775000000000001,0.780000000000001,
0.785000000000001,0.790000000000001,0.795000000000001,0.800000000000001,
0.805000000000001,0.810000000000001,0.815000000000001,0.820000000000001,
0.825000000000001,0.830000000000001,0.835000000000001,0.840000000000001,
0.845000000000001,0.850000000000001,0.855000000000001,0.860000000000001,
0.865000000000001,0.870000000000001,0.875000000000001,0.880000000000001,
0.885000000000001,0.890000000000001,0.895000000000001,0.900000000000001,
0.905000000000001,0.910000000000001,0.915000000000001,0.920000000000001,
0.925000000000001,0.930000000000001,0.935000000000001,0.940000000000001,
0.945000000000001,0.950000000000001,0.955000000000001,0.960000000000001,
0.965000000000001,0.970000000000001,0.975000000000001,0.980000000000001,
0.985000000000001,0.990000000000001,0.995000000000001,1.),.UNSPECIFIED.)
CURVE()
GEOMETRIC_REPRESENTATION_ITEM()
RATIONAL_B_SPLINE_CURVE((1.,1.,1.,1.,1.,1.,1.,1.,1.,1.,1.,1.,1.,1.,1.,1.,
1.,1.,1.,1.,1.,1.,1.,1.,1.,1.,1.,1.,1.,1.,1.,1.,1.,1.,1.,1.,1.,1.,1.,1.,
1.,1.,1.,1.,1.,1.,1.,1.,1.,1.,1.,1.,1.,1.,1.,1.,1.,1.,1.,1.,1.,1.,1.,1.,
1.,1.,1.,1.,1.,1.,1.,1.,1.,1.,1.,1.,1.,1.,1.,1.,1.,1.,1.,1.,1.,1.,1.,1.,
1.,1.,1.,1.,1.,1.,1.,1.,1.,1.,1.,1.,1.,1.,1.,1.,1.,1.,1.,1.,1.,1.,1.,1.,
1.,1.,1.,1.,1.,1.,1.,1.,1.,1.,1.,1.,1.,1.,1.,1.,1.,1.,1.,1.,1.,1.,1.,1.,
1.,1.,1.,1.,1.,1.,1.,1.,1.,1.,1.,1.,1.,1.,1.,1.,1.,1.,1.,1.,1.,1.,1.,1.,
1.,1.,1.,1.,1.,1.,1.,1.,1.,1.,1.,1.,1.,1.,1.,1.,1.,1.,1.,1.,1.,1.,1.,1.,
1.,1.,1.,1.,1.,1.,1.,1.,1.,1.,1.,1.,1.,1.,1.,1.,1.,1.,1.,1.,1.))
REPRESENTATION_ITEM('')
);
#793=(
BOUNDED_CURVE()
B_SPLINE_CURVE(5,(#218894,#218895,#218896,#218897,#218898,#218899,#218900,
#218901,#218902,#218903,#218904,#218905,#218906,#218907,#218908,#218909,
#218910,#218911,#218912,#218913,#218914,#218915,#218916,#218917,#218918,
#218919,#218920,#218921,#218922,#218923,#218924,#218925,#218926,#218927,
#218928,#218929,#218930,#218931,#218932,#218933,#218934,#218935,#218936,
#218937,#218938,#218939,#218940,#218941,#218942,#218943,#218944,#218945,
#218946,#218947,#218948,#218949,#218950,#218951,#218952,#218953,#218954,
#218955,#218956,#218957,#218958,#218959,#218960,#218961,#218962,#218963,
#218964,#218965,#218966,#218967,#218968,#218969,#218970,#218971,#218972,
#218973,#218974,#218975,#218976,#218977,#218978,#218979,#218980,#218981,
#218982,#218983,#218984,#218985,#218986,#218987,#218988,#218989,#218990,
#218991,#218992,#218993,#218994,#218995,#218996,#218997,#218998,#218999,
#219000,#219001,#219002,#219003,#219004,#219005,#219006,#219007,#219008,
#219009,#219010,#219011,#219012,#219013,#219014,#219015,#219016,#219017,
#219018,#219019,#219020,#219021,#219022,#219023,#219024,#219025,#219026,
#219027,#219028,#219029,#219030,#219031,#219032,#219033,#219034,#219035,
#219036,#219037,#219038,#219039,#219040,#219041,#219042,#219043,#219044,
#219045,#219046,#219047,#219048,#219049,#219050,#219051,#219052,#219053,
#219054,#219055,#219056,#219057,#219058,#219059,#219060,#219061,#219062,
#219063,#219064,#219065,#219066,#219067,#219068,#219069,#219070,#219071,
#219072,#219073,#219074,#219075,#219076,#219077,#219078,#219079,#219080,
#219081,#219082,#219083,#219084,#219085,#219086,#219087,#219088,#219089,
#219090,#219091,#219092,#219093,#219094,#219095,#219096,#219097,#219098),
 .UNSPECIFIED.,.F.,.F.)
B_SPLINE_CURVE_WITH_KNOTS((6,1,1,1,1,1,1,1,1,1,1,1,1,1,1,1,1,1,1,1,1,1,
1,1,1,1,1,1,1,1,1,1,1,1,1,1,1,1,1,1,1,1,1,1,1,1,1,1,1,1,1,1,1,1,1,1,1,1,
1,1,1,1,1,1,1,1,1,1,1,1,1,1,1,1,1,1,1,1,1,1,1,1,1,1,1,1,1,1,1,1,1,1,1,1,
1,1,1,1,1,1,1,1,1,1,1,1,1,1,1,1,1,1,1,1,1,1,1,1,1,1,1,1,1,1,1,1,1,1,1,1,
1,1,1,1,1,1,1,1,1,1,1,1,1,1,1,1,1,1,1,1,1,1,1,1,1,1,1,1,1,1,1,1,1,1,1,1,
1,1,1,1,1,1,1,1,1,1,1,1,1,1,1,1,1,1,1,1,1,1,1,1,1,1,1,1,1,1,1,1,1,1,6),
(0.,0.005,0.01,0.015,0.02,0.025,0.03,0.035,0.04,0.045,0.05,0.055,0.06,0.065,
0.07,0.075,0.08,0.085,0.09,0.095,0.1,0.105,0.11,0.115,0.12,0.125,0.13,0.135,
0.14,0.145,0.15,0.155,0.16,0.165,0.17,0.175,0.18,0.185,0.19,0.195,0.2,0.205,
0.21,0.215,0.22,0.225,0.23,0.235,0.24,0.245,0.25,0.255,0.26,0.265,0.27,
0.275,0.28,0.285,0.29,0.295,0.3,0.305,0.31,0.315,0.32,0.325,0.33,0.335,
0.34,0.345,0.35,0.355,0.36,0.365,0.37,0.375,0.38,0.385,0.39,0.395,0.4,0.405,
0.41,0.415,0.42,0.425,0.43,0.435,0.44,0.445,0.45,0.455,0.46,0.465,0.47,
0.475,0.48,0.485,0.49,0.495,0.5,0.505,0.51,0.515,0.52,0.525,0.53,0.535,
0.54,0.545,0.55,0.555,0.56,0.565,0.57,0.575,0.58,0.585,0.59,0.595,0.6,0.605,
0.61,0.615,0.62,0.625,0.63,0.635,0.64,0.645,0.65,0.655,0.66,0.665,0.67,
0.675,0.68,0.685,0.690000000000001,0.695000000000001,0.700000000000001,
0.705000000000001,0.710000000000001,0.715000000000001,0.720000000000001,
0.725000000000001,0.730000000000001,0.735000000000001,0.740000000000001,
0.745000000000001,0.750000000000001,0.755000000000001,0.760000000000001,
0.765000000000001,0.770000000000001,0.775000000000001,0.780000000000001,
0.785000000000001,0.790000000000001,0.795000000000001,0.800000000000001,
0.805000000000001,0.810000000000001,0.815000000000001,0.820000000000001,
0.825000000000001,0.830000000000001,0.835000000000001,0.840000000000001,
0.845000000000001,0.850000000000001,0.855000000000001,0.860000000000001,
0.865000000000001,0.870000000000001,0.875000000000001,0.880000000000001,
0.885000000000001,0.890000000000001,0.895000000000001,0.900000000000001,
0.905000000000001,0.910000000000001,0.915000000000001,0.920000000000001,
0.925000000000001,0.930000000000001,0.935000000000001,0.940000000000001,
0.945000000000001,0.950000000000001,0.955000000000001,0.960000000000001,
0.965000000000001,0.970000000000001,0.975000000000001,0.980000000000001,
0.985000000000001,0.990000000000001,0.995000000000001,1.),.UNSPECIFIED.)
CURVE()
GEOMETRIC_REPRESENTATION_ITEM()
RATIONAL_B_SPLINE_CURVE((1.,1.,1.,1.,1.,1.,1.,1.,1.,1.,1.,1.,1.,1.,1.,1.,
1.,1.,1.,1.,1.,1.,1.,1.,1.,1.,1.,1.,1.,1.,1.,1.,1.,1.,1.,1.,1.,1.,1.,1.,
1.,1.,1.,1.,1.,1.,1.,1.,1.,1.,1.,1.,1.,1.,1.,1.,1.,1.,1.,1.,1.,1.,1.,1.,
1.,1.,1.,1.,1.,1.,1.,1.,1.,1.,1.,1.,1.,1.,1.,1.,1.,1.,1.,1.,1.,1.,1.,1.,
1.,1.,1.,1.,1.,1.,1.,1.,1.,1.,1.,1.,1.,1.,1.,1.,1.,1.,1.,1.,1.,1.,1.,1.,
1.,1.,1.,1.,1.,1.,1.,1.,1.,1.,1.,1.,1.,1.,1.,1.,1.,1.,1.,1.,1.,1.,1.,1.,
1.,1.,1.,1.,1.,1.,1.,1.,1.,1.,1.,1.,1.,1.,1.,1.,1.,1.,1.,1.,1.,1.,1.,1.,
1.,1.,1.,1.,1.,1.,1.,1.,1.,1.,1.,1.,1.,1.,1.,1.,1.,1.,1.,1.,1.,1.,1.,1.,
1.,1.,1.,1.,1.,1.,1.,1.,1.,1.,1.,1.,1.,1.,1.,1.,1.,1.,1.,1.,1.))
REPRESENTATION_ITEM('')
);
#794=(
BOUNDED_CURVE()
B_SPLINE_CURVE(5,(#219100,#219101,#219102,#219103,#219104,#219105,#219106,
#219107,#219108,#219109,#219110,#219111,#219112,#219113,#219114,#219115,
#219116,#219117,#219118,#219119,#219120,#219121,#219122,#219123,#219124,
#219125,#219126,#219127,#219128,#219129,#219130,#219131,#219132,#219133,
#219134,#219135,#219136,#219137,#219138,#219139,#219140,#219141,#219142,
#219143,#219144,#219145,#219146,#219147,#219148,#219149,#219150,#219151,
#219152,#219153,#219154,#219155,#219156,#219157,#219158,#219159,#219160,
#219161,#219162,#219163,#219164,#219165,#219166,#219167,#219168,#219169,
#219170,#219171,#219172,#219173,#219174,#219175,#219176,#219177,#219178,
#219179,#219180,#219181,#219182,#219183,#219184,#219185,#219186,#219187,
#219188,#219189,#219190,#219191,#219192,#219193,#219194,#219195,#219196,
#219197,#219198,#219199,#219200,#219201,#219202,#219203,#219204,#219205,
#219206,#219207,#219208,#219209,#219210,#219211,#219212,#219213,#219214,
#219215,#219216,#219217,#219218,#219219,#219220,#219221,#219222,#219223,
#219224,#219225,#219226,#219227,#219228,#219229,#219230,#219231,#219232,
#219233,#219234,#219235,#219236,#219237,#219238,#219239,#219240,#219241,
#219242,#219243,#219244,#219245,#219246,#219247,#219248,#219249,#219250,
#219251,#219252,#219253,#219254,#219255,#219256,#219257,#219258,#219259,
#219260,#219261,#219262,#219263,#219264,#219265,#219266,#219267,#219268,
#219269,#219270,#219271,#219272,#219273,#219274,#219275,#219276,#219277,
#219278,#219279,#219280,#219281,#219282,#219283,#219284,#219285,#219286,
#219287,#219288,#219289,#219290,#219291,#219292,#219293,#219294,#219295,
#219296,#219297,#219298,#219299,#219300,#219301,#219302,#219303,#219304),
 .UNSPECIFIED.,.F.,.F.)
B_SPLINE_CURVE_WITH_KNOTS((6,1,1,1,1,1,1,1,1,1,1,1,1,1,1,1,1,1,1,1,1,1,
1,1,1,1,1,1,1,1,1,1,1,1,1,1,1,1,1,1,1,1,1,1,1,1,1,1,1,1,1,1,1,1,1,1,1,1,
1,1,1,1,1,1,1,1,1,1,1,1,1,1,1,1,1,1,1,1,1,1,1,1,1,1,1,1,1,1,1,1,1,1,1,1,
1,1,1,1,1,1,1,1,1,1,1,1,1,1,1,1,1,1,1,1,1,1,1,1,1,1,1,1,1,1,1,1,1,1,1,1,
1,1,1,1,1,1,1,1,1,1,1,1,1,1,1,1,1,1,1,1,1,1,1,1,1,1,1,1,1,1,1,1,1,1,1,1,
1,1,1,1,1,1,1,1,1,1,1,1,1,1,1,1,1,1,1,1,1,1,1,1,1,1,1,1,1,1,1,1,1,1,6),
(-1.,-0.995000000000001,-0.990000000000001,-0.985000000000001,-0.980000000000001,
-0.975000000000001,-0.970000000000001,-0.965000000000001,-0.960000000000001,
-0.955000000000001,-0.950000000000001,-0.945000000000001,-0.940000000000001,
-0.935000000000001,-0.930000000000001,-0.925000000000001,-0.920000000000001,
-0.915000000000001,-0.910000000000001,-0.905000000000001,-0.900000000000001,
-0.895000000000001,-0.890000000000001,-0.885000000000001,-0.880000000000001,
-0.875000000000001,-0.870000000000001,-0.865000000000001,-0.860000000000001,
-0.855000000000001,-0.850000000000001,-0.845000000000001,-0.840000000000001,
-0.835000000000001,-0.830000000000001,-0.825000000000001,-0.820000000000001,
-0.815000000000001,-0.810000000000001,-0.805000000000001,-0.800000000000001,
-0.795000000000001,-0.790000000000001,-0.785000000000001,-0.780000000000001,
-0.775000000000001,-0.770000000000001,-0.765000000000001,-0.760000000000001,
-0.755000000000001,-0.750000000000001,-0.745000000000001,-0.740000000000001,
-0.735000000000001,-0.730000000000001,-0.725000000000001,-0.720000000000001,
-0.715000000000001,-0.710000000000001,-0.705000000000001,-0.700000000000001,
-0.695000000000001,-0.690000000000001,-0.685,-0.68,-0.675,-0.67,-0.665,
-0.66,-0.655,-0.65,-0.645,-0.64,-0.635,-0.63,-0.625,-0.62,-0.615,-0.61,
-0.605,-0.6,-0.595,-0.59,-0.585,-0.58,-0.575,-0.57,-0.565,-0.56,-0.555,
-0.55,-0.545,-0.54,-0.535,-0.53,-0.525,-0.52,-0.515,-0.51,-0.505,-0.5,-0.495,
-0.49,-0.485,-0.48,-0.475,-0.47,-0.465,-0.46,-0.455,-0.45,-0.445,-0.44,
-0.435,-0.43,-0.425,-0.42,-0.415,-0.41,-0.405,-0.4,-0.395,-0.39,-0.385,
-0.38,-0.375,-0.37,-0.365,-0.36,-0.355,-0.35,-0.345,-0.34,-0.335,-0.33,
-0.325,-0.32,-0.315,-0.31,-0.305,-0.3,-0.295,-0.29,-0.285,-0.28,-0.275,
-0.27,-0.265,-0.26,-0.255,-0.25,-0.245,-0.24,-0.235,-0.23,-0.225,-0.22,
-0.215,-0.21,-0.205,-0.2,-0.195,-0.19,-0.185,-0.18,-0.175,-0.17,-0.165,
-0.16,-0.155,-0.15,-0.145,-0.14,-0.135,-0.13,-0.125,-0.12,-0.115,-0.11,
-0.105,-0.1,-0.095,-0.09,-0.085,-0.08,-0.075,-0.07,-0.065,-0.06,-0.055,
-0.05,-0.045,-0.04,-0.035,-0.03,-0.025,-0.02,-0.015,-0.01,-0.005,0.),
 .UNSPECIFIED.)
CURVE()
GEOMETRIC_REPRESENTATION_ITEM()
RATIONAL_B_SPLINE_CURVE((1.,1.,1.,1.,1.,1.,1.,1.,1.,1.,1.,1.,1.,1.,1.,1.,
1.,1.,1.,1.,1.,1.,1.,1.,1.,1.,1.,1.,1.,1.,1.,1.,1.,1.,1.,1.,1.,1.,1.,1.,
1.,1.,1.,1.,1.,1.,1.,1.,1.,1.,1.,1.,1.,1.,1.,1.,1.,1.,1.,1.,1.,1.,1.,1.,
1.,1.,1.,1.,1.,1.,1.,1.,1.,1.,1.,1.,1.,1.,1.,1.,1.,1.,1.,1.,1.,1.,1.,1.,
1.,1.,1.,1.,1.,1.,1.,1.,1.,1.,1.,1.,1.,1.,1.,1.,1.,1.,1.,1.,1.,1.,1.,1.,
1.,1.,1.,1.,1.,1.,1.,1.,1.,1.,1.,1.,1.,1.,1.,1.,1.,1.,1.,1.,1.,1.,1.,1.,
1.,1.,1.,1.,1.,1.,1.,1.,1.,1.,1.,1.,1.,1.,1.,1.,1.,1.,1.,1.,1.,1.,1.,1.,
1.,1.,1.,1.,1.,1.,1.,1.,1.,1.,1.,1.,1.,1.,1.,1.,1.,1.,1.,1.,1.,1.,1.,1.,
1.,1.,1.,1.,1.,1.,1.,1.,1.,1.,1.,1.,1.,1.,1.,1.,1.,1.,1.,1.,1.))
REPRESENTATION_ITEM('')
);
#795=(
BOUNDED_CURVE()
B_SPLINE_CURVE(5,(#219723,#219724,#219725,#219726,#219727,#219728,#219729,
#219730,#219731,#219732,#219733,#219734,#219735,#219736,#219737,#219738,
#219739,#219740,#219741,#219742,#219743,#219744,#219745,#219746,#219747,
#219748,#219749,#219750,#219751,#219752,#219753,#219754,#219755,#219756,
#219757,#219758,#219759,#219760,#219761,#219762,#219763,#219764,#219765,
#219766,#219767,#219768,#219769,#219770,#219771,#219772,#219773,#219774,
#219775,#219776,#219777,#219778,#219779,#219780,#219781,#219782,#219783,
#219784,#219785,#219786,#219787,#219788,#219789,#219790,#219791,#219792,
#219793,#219794,#219795,#219796,#219797,#219798,#219799,#219800,#219801,
#219802,#219803,#219804,#219805,#219806,#219807,#219808,#219809,#219810,
#219811,#219812,#219813,#219814,#219815,#219816,#219817,#219818,#219819,
#219820,#219821,#219822,#219823,#219824,#219825,#219826,#219827,#219828,
#219829,#219830,#219831,#219832,#219833,#219834,#219835,#219836,#219837,
#219838,#219839,#219840,#219841,#219842,#219843,#219844,#219845,#219846,
#219847,#219848,#219849,#219850,#219851,#219852,#219853,#219854,#219855,
#219856,#219857,#219858,#219859,#219860,#219861,#219862,#219863,#219864,
#219865,#219866,#219867,#219868,#219869,#219870,#219871,#219872,#219873,
#219874,#219875,#219876,#219877,#219878,#219879,#219880,#219881,#219882,
#219883,#219884,#219885,#219886,#219887,#219888,#219889,#219890,#219891,
#219892,#219893,#219894,#219895,#219896,#219897,#219898,#219899,#219900,
#219901,#219902,#219903,#219904,#219905,#219906,#219907,#219908,#219909,
#219910,#219911,#219912,#219913,#219914,#219915,#219916,#219917,#219918,
#219919,#219920,#219921,#219922,#219923,#219924,#219925,#219926,#219927),
 .UNSPECIFIED.,.F.,.F.)
B_SPLINE_CURVE_WITH_KNOTS((6,1,1,1,1,1,1,1,1,1,1,1,1,1,1,1,1,1,1,1,1,1,
1,1,1,1,1,1,1,1,1,1,1,1,1,1,1,1,1,1,1,1,1,1,1,1,1,1,1,1,1,1,1,1,1,1,1,1,
1,1,1,1,1,1,1,1,1,1,1,1,1,1,1,1,1,1,1,1,1,1,1,1,1,1,1,1,1,1,1,1,1,1,1,1,
1,1,1,1,1,1,1,1,1,1,1,1,1,1,1,1,1,1,1,1,1,1,1,1,1,1,1,1,1,1,1,1,1,1,1,1,
1,1,1,1,1,1,1,1,1,1,1,1,1,1,1,1,1,1,1,1,1,1,1,1,1,1,1,1,1,1,1,1,1,1,1,1,
1,1,1,1,1,1,1,1,1,1,1,1,1,1,1,1,1,1,1,1,1,1,1,1,1,1,1,1,1,1,1,1,1,1,6),
(-1.,-0.995000000000001,-0.990000000000001,-0.985000000000001,-0.980000000000001,
-0.975000000000001,-0.970000000000001,-0.965000000000001,-0.960000000000001,
-0.955000000000001,-0.950000000000001,-0.945000000000001,-0.940000000000001,
-0.935000000000001,-0.930000000000001,-0.925000000000001,-0.920000000000001,
-0.915000000000001,-0.910000000000001,-0.905000000000001,-0.900000000000001,
-0.895000000000001,-0.890000000000001,-0.885000000000001,-0.880000000000001,
-0.875000000000001,-0.870000000000001,-0.865000000000001,-0.860000000000001,
-0.855000000000001,-0.850000000000001,-0.845000000000001,-0.840000000000001,
-0.835000000000001,-0.830000000000001,-0.825000000000001,-0.820000000000001,
-0.815000000000001,-0.810000000000001,-0.805000000000001,-0.800000000000001,
-0.795000000000001,-0.790000000000001,-0.785000000000001,-0.780000000000001,
-0.775000000000001,-0.770000000000001,-0.765000000000001,-0.760000000000001,
-0.755000000000001,-0.750000000000001,-0.745000000000001,-0.740000000000001,
-0.735000000000001,-0.730000000000001,-0.725000000000001,-0.720000000000001,
-0.715000000000001,-0.710000000000001,-0.705000000000001,-0.700000000000001,
-0.695000000000001,-0.690000000000001,-0.685,-0.68,-0.675,-0.67,-0.665,
-0.66,-0.655,-0.65,-0.645,-0.64,-0.635,-0.63,-0.625,-0.62,-0.615,-0.61,
-0.605,-0.6,-0.595,-0.59,-0.585,-0.58,-0.575,-0.57,-0.565,-0.56,-0.555,
-0.55,-0.545,-0.54,-0.535,-0.53,-0.525,-0.52,-0.515,-0.51,-0.505,-0.5,-0.495,
-0.49,-0.485,-0.48,-0.475,-0.47,-0.465,-0.46,-0.455,-0.45,-0.445,-0.44,
-0.435,-0.43,-0.425,-0.42,-0.415,-0.41,-0.405,-0.4,-0.395,-0.39,-0.385,
-0.38,-0.375,-0.37,-0.365,-0.36,-0.355,-0.35,-0.345,-0.34,-0.335,-0.33,
-0.325,-0.32,-0.315,-0.31,-0.305,-0.3,-0.295,-0.29,-0.285,-0.28,-0.275,
-0.27,-0.265,-0.26,-0.255,-0.25,-0.245,-0.24,-0.235,-0.23,-0.225,-0.22,
-0.215,-0.21,-0.205,-0.2,-0.195,-0.19,-0.185,-0.18,-0.175,-0.17,-0.165,
-0.16,-0.155,-0.15,-0.145,-0.14,-0.135,-0.13,-0.125,-0.12,-0.115,-0.11,
-0.105,-0.1,-0.095,-0.09,-0.085,-0.08,-0.075,-0.07,-0.065,-0.06,-0.055,
-0.05,-0.045,-0.04,-0.035,-0.03,-0.025,-0.02,-0.015,-0.01,-0.005,0.),
 .UNSPECIFIED.)
CURVE()
GEOMETRIC_REPRESENTATION_ITEM()
RATIONAL_B_SPLINE_CURVE((1.,1.,1.,1.,1.,1.,1.,1.,1.,1.,1.,1.,1.,1.,1.,1.,
1.,1.,1.,1.,1.,1.,1.,1.,1.,1.,1.,1.,1.,1.,1.,1.,1.,1.,1.,1.,1.,1.,1.,1.,
1.,1.,1.,1.,1.,1.,1.,1.,1.,1.,1.,1.,1.,1.,1.,1.,1.,1.,1.,1.,1.,1.,1.,1.,
1.,1.,1.,1.,1.,1.,1.,1.,1.,1.,1.,1.,1.,1.,1.,1.,1.,1.,1.,1.,1.,1.,1.,1.,
1.,1.,1.,1.,1.,1.,1.,1.,1.,1.,1.,1.,1.,1.,1.,1.,1.,1.,1.,1.,1.,1.,1.,1.,
1.,1.,1.,1.,1.,1.,1.,1.,1.,1.,1.,1.,1.,1.,1.,1.,1.,1.,1.,1.,1.,1.,1.,1.,
1.,1.,1.,1.,1.,1.,1.,1.,1.,1.,1.,1.,1.,1.,1.,1.,1.,1.,1.,1.,1.,1.,1.,1.,
1.,1.,1.,1.,1.,1.,1.,1.,1.,1.,1.,1.,1.,1.,1.,1.,1.,1.,1.,1.,1.,1.,1.,1.,
1.,1.,1.,1.,1.,1.,1.,1.,1.,1.,1.,1.,1.,1.,1.,1.,1.,1.,1.,1.,1.))
REPRESENTATION_ITEM('')
);
#796=(
BOUNDED_CURVE()
B_SPLINE_CURVE(5,(#219930,#219931,#219932,#219933,#219934,#219935,#219936,
#219937,#219938,#219939,#219940,#219941,#219942,#219943,#219944,#219945,
#219946,#219947,#219948,#219949,#219950,#219951,#219952,#219953,#219954,
#219955,#219956,#219957,#219958,#219959,#219960,#219961,#219962,#219963,
#219964,#219965,#219966,#219967,#219968,#219969,#219970,#219971,#219972,
#219973,#219974,#219975,#219976,#219977,#219978,#219979,#219980,#219981,
#219982,#219983,#219984,#219985,#219986,#219987,#219988,#219989,#219990,
#219991,#219992,#219993,#219994,#219995,#219996,#219997,#219998,#219999,
#220000,#220001,#220002,#220003,#220004,#220005,#220006,#220007,#220008,
#220009,#220010,#220011,#220012,#220013,#220014,#220015,#220016,#220017,
#220018,#220019,#220020,#220021,#220022,#220023,#220024,#220025,#220026,
#220027,#220028,#220029,#220030,#220031,#220032,#220033,#220034,#220035,
#220036,#220037,#220038,#220039,#220040,#220041,#220042,#220043,#220044,
#220045,#220046,#220047,#220048,#220049,#220050,#220051,#220052,#220053,
#220054,#220055,#220056,#220057,#220058,#220059,#220060,#220061,#220062,
#220063,#220064,#220065,#220066,#220067,#220068,#220069,#220070,#220071,
#220072,#220073,#220074,#220075,#220076,#220077,#220078,#220079,#220080,
#220081,#220082,#220083,#220084,#220085,#220086,#220087,#220088,#220089,
#220090,#220091,#220092,#220093,#220094,#220095,#220096,#220097,#220098,
#220099,#220100,#220101,#220102,#220103,#220104,#220105,#220106,#220107,
#220108,#220109,#220110,#220111,#220112,#220113,#220114,#220115,#220116,
#220117,#220118,#220119,#220120,#220121,#220122,#220123,#220124,#220125,
#220126,#220127,#220128,#220129,#220130,#220131,#220132,#220133,#220134),
 .UNSPECIFIED.,.F.,.F.)
B_SPLINE_CURVE_WITH_KNOTS((6,1,1,1,1,1,1,1,1,1,1,1,1,1,1,1,1,1,1,1,1,1,
1,1,1,1,1,1,1,1,1,1,1,1,1,1,1,1,1,1,1,1,1,1,1,1,1,1,1,1,1,1,1,1,1,1,1,1,
1,1,1,1,1,1,1,1,1,1,1,1,1,1,1,1,1,1,1,1,1,1,1,1,1,1,1,1,1,1,1,1,1,1,1,1,
1,1,1,1,1,1,1,1,1,1,1,1,1,1,1,1,1,1,1,1,1,1,1,1,1,1,1,1,1,1,1,1,1,1,1,1,
1,1,1,1,1,1,1,1,1,1,1,1,1,1,1,1,1,1,1,1,1,1,1,1,1,1,1,1,1,1,1,1,1,1,1,1,
1,1,1,1,1,1,1,1,1,1,1,1,1,1,1,1,1,1,1,1,1,1,1,1,1,1,1,1,1,1,1,1,1,1,6),
(0.,0.005,0.01,0.015,0.02,0.025,0.03,0.035,0.04,0.045,0.05,0.055,0.06,0.065,
0.07,0.075,0.08,0.085,0.09,0.095,0.1,0.105,0.11,0.115,0.12,0.125,0.13,0.135,
0.14,0.145,0.15,0.155,0.16,0.165,0.17,0.175,0.18,0.185,0.19,0.195,0.2,0.205,
0.21,0.215,0.22,0.225,0.23,0.235,0.24,0.245,0.25,0.255,0.26,0.265,0.27,
0.275,0.28,0.285,0.29,0.295,0.3,0.305,0.31,0.315,0.32,0.325,0.33,0.335,
0.34,0.345,0.35,0.355,0.36,0.365,0.37,0.375,0.38,0.385,0.39,0.395,0.4,0.405,
0.41,0.415,0.42,0.425,0.43,0.435,0.44,0.445,0.45,0.455,0.46,0.465,0.47,
0.475,0.48,0.485,0.49,0.495,0.5,0.505,0.51,0.515,0.52,0.525,0.53,0.535,
0.54,0.545,0.55,0.555,0.56,0.565,0.57,0.575,0.58,0.585,0.59,0.595,0.6,0.605,
0.61,0.615,0.62,0.625,0.63,0.635,0.64,0.645,0.65,0.655,0.66,0.665,0.67,
0.675,0.68,0.685,0.690000000000001,0.695000000000001,0.700000000000001,
0.705000000000001,0.710000000000001,0.715000000000001,0.720000000000001,
0.725000000000001,0.730000000000001,0.735000000000001,0.740000000000001,
0.745000000000001,0.750000000000001,0.755000000000001,0.760000000000001,
0.765000000000001,0.770000000000001,0.775000000000001,0.780000000000001,
0.785000000000001,0.790000000000001,0.795000000000001,0.800000000000001,
0.805000000000001,0.810000000000001,0.815000000000001,0.820000000000001,
0.825000000000001,0.830000000000001,0.835000000000001,0.840000000000001,
0.845000000000001,0.850000000000001,0.855000000000001,0.860000000000001,
0.865000000000001,0.870000000000001,0.875000000000001,0.880000000000001,
0.885000000000001,0.890000000000001,0.895000000000001,0.900000000000001,
0.905000000000001,0.910000000000001,0.915000000000001,0.920000000000001,
0.925000000000001,0.930000000000001,0.935000000000001,0.940000000000001,
0.945000000000001,0.950000000000001,0.955000000000001,0.960000000000001,
0.965000000000001,0.970000000000001,0.975000000000001,0.980000000000001,
0.985000000000001,0.990000000000001,0.995000000000001,1.),.UNSPECIFIED.)
CURVE()
GEOMETRIC_REPRESENTATION_ITEM()
RATIONAL_B_SPLINE_CURVE((1.,1.,1.,1.,1.,1.,1.,1.,1.,1.,1.,1.,1.,1.,1.,1.,
1.,1.,1.,1.,1.,1.,1.,1.,1.,1.,1.,1.,1.,1.,1.,1.,1.,1.,1.,1.,1.,1.,1.,1.,
1.,1.,1.,1.,1.,1.,1.,1.,1.,1.,1.,1.,1.,1.,1.,1.,1.,1.,1.,1.,1.,1.,1.,1.,
1.,1.,1.,1.,1.,1.,1.,1.,1.,1.,1.,1.,1.,1.,1.,1.,1.,1.,1.,1.,1.,1.,1.,1.,
1.,1.,1.,1.,1.,1.,1.,1.,1.,1.,1.,1.,1.,1.,1.,1.,1.,1.,1.,1.,1.,1.,1.,1.,
1.,1.,1.,1.,1.,1.,1.,1.,1.,1.,1.,1.,1.,1.,1.,1.,1.,1.,1.,1.,1.,1.,1.,1.,
1.,1.,1.,1.,1.,1.,1.,1.,1.,1.,1.,1.,1.,1.,1.,1.,1.,1.,1.,1.,1.,1.,1.,1.,
1.,1.,1.,1.,1.,1.,1.,1.,1.,1.,1.,1.,1.,1.,1.,1.,1.,1.,1.,1.,1.,1.,1.,1.,
1.,1.,1.,1.,1.,1.,1.,1.,1.,1.,1.,1.,1.,1.,1.,1.,1.,1.,1.,1.,1.))
REPRESENTATION_ITEM('')
);
#797=(
BOUNDED_CURVE()
B_SPLINE_CURVE(5,(#220546,#220547,#220548,#220549,#220550,#220551,#220552,
#220553,#220554,#220555,#220556,#220557,#220558,#220559,#220560,#220561,
#220562,#220563,#220564,#220565,#220566,#220567,#220568,#220569,#220570,
#220571,#220572,#220573,#220574,#220575,#220576,#220577,#220578,#220579,
#220580,#220581,#220582,#220583,#220584,#220585,#220586,#220587,#220588,
#220589,#220590,#220591,#220592,#220593,#220594,#220595,#220596,#220597,
#220598,#220599,#220600,#220601,#220602,#220603,#220604,#220605,#220606,
#220607,#220608,#220609,#220610,#220611,#220612,#220613,#220614,#220615,
#220616,#220617,#220618,#220619,#220620,#220621,#220622,#220623,#220624,
#220625,#220626,#220627,#220628,#220629,#220630,#220631,#220632,#220633,
#220634,#220635,#220636,#220637,#220638,#220639,#220640,#220641,#220642,
#220643,#220644,#220645,#220646,#220647,#220648,#220649,#220650,#220651,
#220652,#220653,#220654,#220655,#220656,#220657,#220658,#220659,#220660,
#220661,#220662,#220663,#220664,#220665,#220666,#220667,#220668,#220669,
#220670,#220671,#220672,#220673,#220674,#220675,#220676,#220677,#220678,
#220679,#220680,#220681,#220682,#220683,#220684,#220685,#220686,#220687,
#220688,#220689,#220690,#220691,#220692,#220693,#220694,#220695,#220696,
#220697,#220698,#220699,#220700,#220701,#220702,#220703,#220704,#220705,
#220706,#220707,#220708,#220709,#220710,#220711,#220712,#220713,#220714,
#220715,#220716,#220717,#220718,#220719,#220720,#220721,#220722,#220723,
#220724,#220725,#220726,#220727,#220728,#220729,#220730,#220731,#220732,
#220733,#220734,#220735,#220736,#220737,#220738,#220739,#220740,#220741,
#220742,#220743,#220744,#220745,#220746,#220747,#220748,#220749,#220750),
 .UNSPECIFIED.,.F.,.F.)
B_SPLINE_CURVE_WITH_KNOTS((6,1,1,1,1,1,1,1,1,1,1,1,1,1,1,1,1,1,1,1,1,1,
1,1,1,1,1,1,1,1,1,1,1,1,1,1,1,1,1,1,1,1,1,1,1,1,1,1,1,1,1,1,1,1,1,1,1,1,
1,1,1,1,1,1,1,1,1,1,1,1,1,1,1,1,1,1,1,1,1,1,1,1,1,1,1,1,1,1,1,1,1,1,1,1,
1,1,1,1,1,1,1,1,1,1,1,1,1,1,1,1,1,1,1,1,1,1,1,1,1,1,1,1,1,1,1,1,1,1,1,1,
1,1,1,1,1,1,1,1,1,1,1,1,1,1,1,1,1,1,1,1,1,1,1,1,1,1,1,1,1,1,1,1,1,1,1,1,
1,1,1,1,1,1,1,1,1,1,1,1,1,1,1,1,1,1,1,1,1,1,1,1,1,1,1,1,1,1,1,1,1,1,6),
(0.,0.005,0.01,0.015,0.02,0.025,0.03,0.035,0.04,0.045,0.05,0.055,0.06,0.065,
0.07,0.075,0.08,0.085,0.09,0.095,0.1,0.105,0.11,0.115,0.12,0.125,0.13,0.135,
0.14,0.145,0.15,0.155,0.16,0.165,0.17,0.175,0.18,0.185,0.19,0.195,0.2,0.205,
0.21,0.215,0.22,0.225,0.23,0.235,0.24,0.245,0.25,0.255,0.26,0.265,0.27,
0.275,0.28,0.285,0.29,0.295,0.3,0.305,0.31,0.315,0.32,0.325,0.33,0.335,
0.34,0.345,0.35,0.355,0.36,0.365,0.37,0.375,0.38,0.385,0.39,0.395,0.4,0.405,
0.41,0.415,0.42,0.425,0.43,0.435,0.44,0.445,0.45,0.455,0.46,0.465,0.47,
0.475,0.48,0.485,0.49,0.495,0.5,0.505,0.51,0.515,0.52,0.525,0.53,0.535,
0.54,0.545,0.55,0.555,0.56,0.565,0.57,0.575,0.58,0.585,0.59,0.595,0.6,0.605,
0.61,0.615,0.62,0.625,0.63,0.635,0.64,0.645,0.65,0.655,0.66,0.665,0.67,
0.675,0.68,0.685,0.690000000000001,0.695000000000001,0.700000000000001,
0.705000000000001,0.710000000000001,0.715000000000001,0.720000000000001,
0.725000000000001,0.730000000000001,0.735000000000001,0.740000000000001,
0.745000000000001,0.750000000000001,0.755000000000001,0.760000000000001,
0.765000000000001,0.770000000000001,0.775000000000001,0.780000000000001,
0.785000000000001,0.790000000000001,0.795000000000001,0.800000000000001,
0.805000000000001,0.810000000000001,0.815000000000001,0.820000000000001,
0.825000000000001,0.830000000000001,0.835000000000001,0.840000000000001,
0.845000000000001,0.850000000000001,0.855000000000001,0.860000000000001,
0.865000000000001,0.870000000000001,0.875000000000001,0.880000000000001,
0.885000000000001,0.890000000000001,0.895000000000001,0.900000000000001,
0.905000000000001,0.910000000000001,0.915000000000001,0.920000000000001,
0.925000000000001,0.930000000000001,0.935000000000001,0.940000000000001,
0.945000000000001,0.950000000000001,0.955000000000001,0.960000000000001,
0.965000000000001,0.970000000000001,0.975000000000001,0.980000000000001,
0.985000000000001,0.990000000000001,0.995000000000001,1.),.UNSPECIFIED.)
CURVE()
GEOMETRIC_REPRESENTATION_ITEM()
RATIONAL_B_SPLINE_CURVE((1.,1.,1.,1.,1.,1.,1.,1.,1.,1.,1.,1.,1.,1.,1.,1.,
1.,1.,1.,1.,1.,1.,1.,1.,1.,1.,1.,1.,1.,1.,1.,1.,1.,1.,1.,1.,1.,1.,1.,1.,
1.,1.,1.,1.,1.,1.,1.,1.,1.,1.,1.,1.,1.,1.,1.,1.,1.,1.,1.,1.,1.,1.,1.,1.,
1.,1.,1.,1.,1.,1.,1.,1.,1.,1.,1.,1.,1.,1.,1.,1.,1.,1.,1.,1.,1.,1.,1.,1.,
1.,1.,1.,1.,1.,1.,1.,1.,1.,1.,1.,1.,1.,1.,1.,1.,1.,1.,1.,1.,1.,1.,1.,1.,
1.,1.,1.,1.,1.,1.,1.,1.,1.,1.,1.,1.,1.,1.,1.,1.,1.,1.,1.,1.,1.,1.,1.,1.,
1.,1.,1.,1.,1.,1.,1.,1.,1.,1.,1.,1.,1.,1.,1.,1.,1.,1.,1.,1.,1.,1.,1.,1.,
1.,1.,1.,1.,1.,1.,1.,1.,1.,1.,1.,1.,1.,1.,1.,1.,1.,1.,1.,1.,1.,1.,1.,1.,
1.,1.,1.,1.,1.,1.,1.,1.,1.,1.,1.,1.,1.,1.,1.,1.,1.,1.,1.,1.,1.))
REPRESENTATION_ITEM('')
);
#798=(
BOUNDED_CURVE()
B_SPLINE_CURVE(5,(#220752,#220753,#220754,#220755,#220756,#220757,#220758,
#220759,#220760,#220761,#220762,#220763,#220764,#220765,#220766,#220767,
#220768,#220769,#220770,#220771,#220772,#220773,#220774,#220775,#220776,
#220777,#220778,#220779,#220780,#220781,#220782,#220783,#220784,#220785,
#220786,#220787,#220788,#220789,#220790,#220791,#220792,#220793,#220794,
#220795,#220796,#220797,#220798,#220799,#220800,#220801,#220802,#220803,
#220804,#220805,#220806,#220807,#220808,#220809,#220810,#220811,#220812,
#220813,#220814,#220815,#220816,#220817,#220818,#220819,#220820,#220821,
#220822,#220823,#220824,#220825,#220826,#220827,#220828,#220829,#220830,
#220831,#220832,#220833,#220834,#220835,#220836,#220837,#220838,#220839,
#220840,#220841,#220842,#220843,#220844,#220845,#220846,#220847,#220848,
#220849,#220850,#220851,#220852,#220853,#220854,#220855,#220856,#220857,
#220858,#220859,#220860,#220861,#220862,#220863,#220864,#220865,#220866,
#220867,#220868,#220869,#220870,#220871,#220872,#220873,#220874,#220875,
#220876,#220877,#220878,#220879,#220880,#220881,#220882,#220883,#220884,
#220885,#220886,#220887,#220888,#220889,#220890,#220891,#220892,#220893,
#220894,#220895,#220896,#220897,#220898,#220899,#220900,#220901,#220902,
#220903,#220904,#220905,#220906,#220907,#220908,#220909,#220910,#220911,
#220912,#220913,#220914,#220915,#220916,#220917,#220918,#220919,#220920,
#220921,#220922,#220923,#220924,#220925,#220926,#220927,#220928,#220929,
#220930,#220931,#220932,#220933,#220934,#220935,#220936,#220937,#220938,
#220939,#220940,#220941,#220942,#220943,#220944,#220945,#220946,#220947,
#220948,#220949,#220950,#220951,#220952,#220953,#220954,#220955,#220956),
 .UNSPECIFIED.,.F.,.F.)
B_SPLINE_CURVE_WITH_KNOTS((6,1,1,1,1,1,1,1,1,1,1,1,1,1,1,1,1,1,1,1,1,1,
1,1,1,1,1,1,1,1,1,1,1,1,1,1,1,1,1,1,1,1,1,1,1,1,1,1,1,1,1,1,1,1,1,1,1,1,
1,1,1,1,1,1,1,1,1,1,1,1,1,1,1,1,1,1,1,1,1,1,1,1,1,1,1,1,1,1,1,1,1,1,1,1,
1,1,1,1,1,1,1,1,1,1,1,1,1,1,1,1,1,1,1,1,1,1,1,1,1,1,1,1,1,1,1,1,1,1,1,1,
1,1,1,1,1,1,1,1,1,1,1,1,1,1,1,1,1,1,1,1,1,1,1,1,1,1,1,1,1,1,1,1,1,1,1,1,
1,1,1,1,1,1,1,1,1,1,1,1,1,1,1,1,1,1,1,1,1,1,1,1,1,1,1,1,1,1,1,1,1,1,6),
(-1.,-0.995000000000001,-0.990000000000001,-0.985000000000001,-0.980000000000001,
-0.975000000000001,-0.970000000000001,-0.965000000000001,-0.960000000000001,
-0.955000000000001,-0.950000000000001,-0.945000000000001,-0.940000000000001,
-0.935000000000001,-0.930000000000001,-0.925000000000001,-0.920000000000001,
-0.915000000000001,-0.910000000000001,-0.905000000000001,-0.900000000000001,
-0.895000000000001,-0.890000000000001,-0.885000000000001,-0.880000000000001,
-0.875000000000001,-0.870000000000001,-0.865000000000001,-0.860000000000001,
-0.855000000000001,-0.850000000000001,-0.845000000000001,-0.840000000000001,
-0.835000000000001,-0.830000000000001,-0.825000000000001,-0.820000000000001,
-0.815000000000001,-0.810000000000001,-0.805000000000001,-0.800000000000001,
-0.795000000000001,-0.790000000000001,-0.785000000000001,-0.780000000000001,
-0.775000000000001,-0.770000000000001,-0.765000000000001,-0.760000000000001,
-0.755000000000001,-0.750000000000001,-0.745000000000001,-0.740000000000001,
-0.735000000000001,-0.730000000000001,-0.725000000000001,-0.720000000000001,
-0.715000000000001,-0.710000000000001,-0.705000000000001,-0.700000000000001,
-0.695000000000001,-0.690000000000001,-0.685,-0.68,-0.675,-0.67,-0.665,
-0.66,-0.655,-0.65,-0.645,-0.64,-0.635,-0.63,-0.625,-0.62,-0.615,-0.61,
-0.605,-0.6,-0.595,-0.59,-0.585,-0.58,-0.575,-0.57,-0.565,-0.56,-0.555,
-0.55,-0.545,-0.54,-0.535,-0.53,-0.525,-0.52,-0.515,-0.51,-0.505,-0.5,-0.495,
-0.49,-0.485,-0.48,-0.475,-0.47,-0.465,-0.46,-0.455,-0.45,-0.445,-0.44,
-0.435,-0.43,-0.425,-0.42,-0.415,-0.41,-0.405,-0.4,-0.395,-0.39,-0.385,
-0.38,-0.375,-0.37,-0.365,-0.36,-0.355,-0.35,-0.345,-0.34,-0.335,-0.33,
-0.325,-0.32,-0.315,-0.31,-0.305,-0.3,-0.295,-0.29,-0.285,-0.28,-0.275,
-0.27,-0.265,-0.26,-0.255,-0.25,-0.245,-0.24,-0.235,-0.23,-0.225,-0.22,
-0.215,-0.21,-0.205,-0.2,-0.195,-0.19,-0.185,-0.18,-0.175,-0.17,-0.165,
-0.16,-0.155,-0.15,-0.145,-0.14,-0.135,-0.13,-0.125,-0.12,-0.115,-0.11,
-0.105,-0.1,-0.095,-0.09,-0.085,-0.08,-0.075,-0.07,-0.065,-0.06,-0.055,
-0.05,-0.045,-0.04,-0.035,-0.03,-0.025,-0.02,-0.015,-0.01,-0.005,0.),
 .UNSPECIFIED.)
CURVE()
GEOMETRIC_REPRESENTATION_ITEM()
RATIONAL_B_SPLINE_CURVE((1.,1.,1.,1.,1.,1.,1.,1.,1.,1.,1.,1.,1.,1.,1.,1.,
1.,1.,1.,1.,1.,1.,1.,1.,1.,1.,1.,1.,1.,1.,1.,1.,1.,1.,1.,1.,1.,1.,1.,1.,
1.,1.,1.,1.,1.,1.,1.,1.,1.,1.,1.,1.,1.,1.,1.,1.,1.,1.,1.,1.,1.,1.,1.,1.,
1.,1.,1.,1.,1.,1.,1.,1.,1.,1.,1.,1.,1.,1.,1.,1.,1.,1.,1.,1.,1.,1.,1.,1.,
1.,1.,1.,1.,1.,1.,1.,1.,1.,1.,1.,1.,1.,1.,1.,1.,1.,1.,1.,1.,1.,1.,1.,1.,
1.,1.,1.,1.,1.,1.,1.,1.,1.,1.,1.,1.,1.,1.,1.,1.,1.,1.,1.,1.,1.,1.,1.,1.,
1.,1.,1.,1.,1.,1.,1.,1.,1.,1.,1.,1.,1.,1.,1.,1.,1.,1.,1.,1.,1.,1.,1.,1.,
1.,1.,1.,1.,1.,1.,1.,1.,1.,1.,1.,1.,1.,1.,1.,1.,1.,1.,1.,1.,1.,1.,1.,1.,
1.,1.,1.,1.,1.,1.,1.,1.,1.,1.,1.,1.,1.,1.,1.,1.,1.,1.,1.,1.,1.))
REPRESENTATION_ITEM('')
);
#799=(
BOUNDED_CURVE()
B_SPLINE_CURVE(5,(#221375,#221376,#221377,#221378,#221379,#221380,#221381,
#221382,#221383,#221384,#221385,#221386,#221387,#221388,#221389,#221390,
#221391,#221392,#221393,#221394,#221395,#221396,#221397,#221398,#221399,
#221400,#221401,#221402,#221403,#221404,#221405,#221406,#221407,#221408,
#221409,#221410,#221411,#221412,#221413,#221414,#221415,#221416,#221417,
#221418,#221419,#221420,#221421,#221422,#221423,#221424,#221425,#221426,
#221427,#221428,#221429,#221430,#221431,#221432,#221433,#221434,#221435,
#221436,#221437,#221438,#221439,#221440,#221441,#221442,#221443,#221444,
#221445,#221446,#221447,#221448,#221449,#221450,#221451,#221452,#221453,
#221454,#221455,#221456,#221457,#221458,#221459,#221460,#221461,#221462,
#221463,#221464,#221465,#221466,#221467,#221468,#221469,#221470,#221471,
#221472,#221473,#221474,#221475,#221476,#221477,#221478,#221479,#221480,
#221481,#221482,#221483,#221484,#221485,#221486,#221487,#221488,#221489,
#221490,#221491,#221492,#221493,#221494,#221495,#221496,#221497,#221498,
#221499,#221500,#221501,#221502,#221503,#221504,#221505,#221506,#221507,
#221508,#221509,#221510,#221511,#221512,#221513,#221514,#221515,#221516,
#221517,#221518,#221519,#221520,#221521,#221522,#221523,#221524,#221525,
#221526,#221527,#221528,#221529,#221530,#221531,#221532,#221533,#221534,
#221535,#221536,#221537,#221538,#221539,#221540,#221541,#221542,#221543,
#221544,#221545,#221546,#221547,#221548,#221549,#221550,#221551,#221552,
#221553,#221554,#221555,#221556,#221557,#221558,#221559,#221560,#221561,
#221562,#221563,#221564,#221565,#221566,#221567,#221568,#221569,#221570,
#221571,#221572,#221573,#221574,#221575,#221576,#221577,#221578,#221579),
 .UNSPECIFIED.,.F.,.F.)
B_SPLINE_CURVE_WITH_KNOTS((6,1,1,1,1,1,1,1,1,1,1,1,1,1,1,1,1,1,1,1,1,1,
1,1,1,1,1,1,1,1,1,1,1,1,1,1,1,1,1,1,1,1,1,1,1,1,1,1,1,1,1,1,1,1,1,1,1,1,
1,1,1,1,1,1,1,1,1,1,1,1,1,1,1,1,1,1,1,1,1,1,1,1,1,1,1,1,1,1,1,1,1,1,1,1,
1,1,1,1,1,1,1,1,1,1,1,1,1,1,1,1,1,1,1,1,1,1,1,1,1,1,1,1,1,1,1,1,1,1,1,1,
1,1,1,1,1,1,1,1,1,1,1,1,1,1,1,1,1,1,1,1,1,1,1,1,1,1,1,1,1,1,1,1,1,1,1,1,
1,1,1,1,1,1,1,1,1,1,1,1,1,1,1,1,1,1,1,1,1,1,1,1,1,1,1,1,1,1,1,1,1,1,6),
(-1.,-0.995000000000001,-0.990000000000001,-0.985000000000001,-0.980000000000001,
-0.975000000000001,-0.970000000000001,-0.965000000000001,-0.960000000000001,
-0.955000000000001,-0.950000000000001,-0.945000000000001,-0.940000000000001,
-0.935000000000001,-0.930000000000001,-0.925000000000001,-0.920000000000001,
-0.915000000000001,-0.910000000000001,-0.905000000000001,-0.900000000000001,
-0.895000000000001,-0.890000000000001,-0.885000000000001,-0.880000000000001,
-0.875000000000001,-0.870000000000001,-0.865000000000001,-0.860000000000001,
-0.855000000000001,-0.850000000000001,-0.845000000000001,-0.840000000000001,
-0.835000000000001,-0.830000000000001,-0.825000000000001,-0.820000000000001,
-0.815000000000001,-0.810000000000001,-0.805000000000001,-0.800000000000001,
-0.795000000000001,-0.790000000000001,-0.785000000000001,-0.780000000000001,
-0.775000000000001,-0.770000000000001,-0.765000000000001,-0.760000000000001,
-0.755000000000001,-0.750000000000001,-0.745000000000001,-0.740000000000001,
-0.735000000000001,-0.730000000000001,-0.725000000000001,-0.720000000000001,
-0.715000000000001,-0.710000000000001,-0.705000000000001,-0.700000000000001,
-0.695000000000001,-0.690000000000001,-0.685,-0.68,-0.675,-0.67,-0.665,
-0.66,-0.655,-0.65,-0.645,-0.64,-0.635,-0.63,-0.625,-0.62,-0.615,-0.61,
-0.605,-0.6,-0.595,-0.59,-0.585,-0.58,-0.575,-0.57,-0.565,-0.56,-0.555,
-0.55,-0.545,-0.54,-0.535,-0.53,-0.525,-0.52,-0.515,-0.51,-0.505,-0.5,-0.495,
-0.49,-0.485,-0.48,-0.475,-0.47,-0.465,-0.46,-0.455,-0.45,-0.445,-0.44,
-0.435,-0.43,-0.425,-0.42,-0.415,-0.41,-0.405,-0.4,-0.395,-0.39,-0.385,
-0.38,-0.375,-0.37,-0.365,-0.36,-0.355,-0.35,-0.345,-0.34,-0.335,-0.33,
-0.325,-0.32,-0.315,-0.31,-0.305,-0.3,-0.295,-0.29,-0.285,-0.28,-0.275,
-0.27,-0.265,-0.26,-0.255,-0.25,-0.245,-0.24,-0.235,-0.23,-0.225,-0.22,
-0.215,-0.21,-0.205,-0.2,-0.195,-0.19,-0.185,-0.18,-0.175,-0.17,-0.165,
-0.16,-0.155,-0.15,-0.145,-0.14,-0.135,-0.13,-0.125,-0.12,-0.115,-0.11,
-0.105,-0.1,-0.095,-0.09,-0.085,-0.08,-0.075,-0.07,-0.065,-0.06,-0.055,
-0.05,-0.045,-0.04,-0.035,-0.03,-0.025,-0.02,-0.015,-0.01,-0.005,0.),
 .UNSPECIFIED.)
CURVE()
GEOMETRIC_REPRESENTATION_ITEM()
RATIONAL_B_SPLINE_CURVE((1.,1.,1.,1.,1.,1.,1.,1.,1.,1.,1.,1.,1.,1.,1.,1.,
1.,1.,1.,1.,1.,1.,1.,1.,1.,1.,1.,1.,1.,1.,1.,1.,1.,1.,1.,1.,1.,1.,1.,1.,
1.,1.,1.,1.,1.,1.,1.,1.,1.,1.,1.,1.,1.,1.,1.,1.,1.,1.,1.,1.,1.,1.,1.,1.,
1.,1.,1.,1.,1.,1.,1.,1.,1.,1.,1.,1.,1.,1.,1.,1.,1.,1.,1.,1.,1.,1.,1.,1.,
1.,1.,1.,1.,1.,1.,1.,1.,1.,1.,1.,1.,1.,1.,1.,1.,1.,1.,1.,1.,1.,1.,1.,1.,
1.,1.,1.,1.,1.,1.,1.,1.,1.,1.,1.,1.,1.,1.,1.,1.,1.,1.,1.,1.,1.,1.,1.,1.,
1.,1.,1.,1.,1.,1.,1.,1.,1.,1.,1.,1.,1.,1.,1.,1.,1.,1.,1.,1.,1.,1.,1.,1.,
1.,1.,1.,1.,1.,1.,1.,1.,1.,1.,1.,1.,1.,1.,1.,1.,1.,1.,1.,1.,1.,1.,1.,1.,
1.,1.,1.,1.,1.,1.,1.,1.,1.,1.,1.,1.,1.,1.,1.,1.,1.,1.,1.,1.,1.))
REPRESENTATION_ITEM('')
);
#800=(
BOUNDED_CURVE()
B_SPLINE_CURVE(5,(#221582,#221583,#221584,#221585,#221586,#221587,#221588,
#221589,#221590,#221591,#221592,#221593,#221594,#221595,#221596,#221597,
#221598,#221599,#221600,#221601,#221602,#221603,#221604,#221605,#221606,
#221607,#221608,#221609,#221610,#221611,#221612,#221613,#221614,#221615,
#221616,#221617,#221618,#221619,#221620,#221621,#221622,#221623,#221624,
#221625,#221626,#221627,#221628,#221629,#221630,#221631,#221632,#221633,
#221634,#221635,#221636,#221637,#221638,#221639,#221640,#221641,#221642,
#221643,#221644,#221645,#221646,#221647,#221648,#221649,#221650,#221651,
#221652,#221653,#221654,#221655,#221656,#221657,#221658,#221659,#221660,
#221661,#221662,#221663,#221664,#221665,#221666,#221667,#221668,#221669,
#221670,#221671,#221672,#221673,#221674,#221675,#221676,#221677,#221678,
#221679,#221680,#221681,#221682,#221683,#221684,#221685,#221686,#221687,
#221688,#221689,#221690,#221691,#221692,#221693,#221694,#221695,#221696,
#221697,#221698,#221699,#221700,#221701,#221702,#221703,#221704,#221705,
#221706,#221707,#221708,#221709,#221710,#221711,#221712,#221713,#221714,
#221715,#221716,#221717,#221718,#221719,#221720,#221721,#221722,#221723,
#221724,#221725,#221726,#221727,#221728,#221729,#221730,#221731,#221732,
#221733,#221734,#221735,#221736,#221737,#221738,#221739,#221740,#221741,
#221742,#221743,#221744,#221745,#221746,#221747,#221748,#221749,#221750,
#221751,#221752,#221753,#221754,#221755,#221756,#221757,#221758,#221759,
#221760,#221761,#221762,#221763,#221764,#221765,#221766,#221767,#221768,
#221769,#221770,#221771,#221772,#221773,#221774,#221775,#221776,#221777,
#221778,#221779,#221780,#221781,#221782,#221783,#221784,#221785,#221786),
 .UNSPECIFIED.,.F.,.F.)
B_SPLINE_CURVE_WITH_KNOTS((6,1,1,1,1,1,1,1,1,1,1,1,1,1,1,1,1,1,1,1,1,1,
1,1,1,1,1,1,1,1,1,1,1,1,1,1,1,1,1,1,1,1,1,1,1,1,1,1,1,1,1,1,1,1,1,1,1,1,
1,1,1,1,1,1,1,1,1,1,1,1,1,1,1,1,1,1,1,1,1,1,1,1,1,1,1,1,1,1,1,1,1,1,1,1,
1,1,1,1,1,1,1,1,1,1,1,1,1,1,1,1,1,1,1,1,1,1,1,1,1,1,1,1,1,1,1,1,1,1,1,1,
1,1,1,1,1,1,1,1,1,1,1,1,1,1,1,1,1,1,1,1,1,1,1,1,1,1,1,1,1,1,1,1,1,1,1,1,
1,1,1,1,1,1,1,1,1,1,1,1,1,1,1,1,1,1,1,1,1,1,1,1,1,1,1,1,1,1,1,1,1,1,6),
(0.,0.005,0.01,0.015,0.02,0.025,0.03,0.035,0.04,0.045,0.05,0.055,0.06,0.065,
0.07,0.075,0.08,0.085,0.09,0.095,0.1,0.105,0.11,0.115,0.12,0.125,0.13,0.135,
0.14,0.145,0.15,0.155,0.16,0.165,0.17,0.175,0.18,0.185,0.19,0.195,0.2,0.205,
0.21,0.215,0.22,0.225,0.23,0.235,0.24,0.245,0.25,0.255,0.26,0.265,0.27,
0.275,0.28,0.285,0.29,0.295,0.3,0.305,0.31,0.315,0.32,0.325,0.33,0.335,
0.34,0.345,0.35,0.355,0.36,0.365,0.37,0.375,0.38,0.385,0.39,0.395,0.4,0.405,
0.41,0.415,0.42,0.425,0.43,0.435,0.44,0.445,0.45,0.455,0.46,0.465,0.47,
0.475,0.48,0.485,0.49,0.495,0.5,0.505,0.51,0.515,0.52,0.525,0.53,0.535,
0.54,0.545,0.55,0.555,0.56,0.565,0.57,0.575,0.58,0.585,0.59,0.595,0.6,0.605,
0.61,0.615,0.62,0.625,0.63,0.635,0.64,0.645,0.65,0.655,0.66,0.665,0.67,
0.675,0.68,0.685,0.690000000000001,0.695000000000001,0.700000000000001,
0.705000000000001,0.710000000000001,0.715000000000001,0.720000000000001,
0.725000000000001,0.730000000000001,0.735000000000001,0.740000000000001,
0.745000000000001,0.750000000000001,0.755000000000001,0.760000000000001,
0.765000000000001,0.770000000000001,0.775000000000001,0.780000000000001,
0.785000000000001,0.790000000000001,0.795000000000001,0.800000000000001,
0.805000000000001,0.810000000000001,0.815000000000001,0.820000000000001,
0.825000000000001,0.830000000000001,0.835000000000001,0.840000000000001,
0.845000000000001,0.850000000000001,0.855000000000001,0.860000000000001,
0.865000000000001,0.870000000000001,0.875000000000001,0.880000000000001,
0.885000000000001,0.890000000000001,0.895000000000001,0.900000000000001,
0.905000000000001,0.910000000000001,0.915000000000001,0.920000000000001,
0.925000000000001,0.930000000000001,0.935000000000001,0.940000000000001,
0.945000000000001,0.950000000000001,0.955000000000001,0.960000000000001,
0.965000000000001,0.970000000000001,0.975000000000001,0.980000000000001,
0.985000000000001,0.990000000000001,0.995000000000001,1.),.UNSPECIFIED.)
CURVE()
GEOMETRIC_REPRESENTATION_ITEM()
RATIONAL_B_SPLINE_CURVE((1.,1.,1.,1.,1.,1.,1.,1.,1.,1.,1.,1.,1.,1.,1.,1.,
1.,1.,1.,1.,1.,1.,1.,1.,1.,1.,1.,1.,1.,1.,1.,1.,1.,1.,1.,1.,1.,1.,1.,1.,
1.,1.,1.,1.,1.,1.,1.,1.,1.,1.,1.,1.,1.,1.,1.,1.,1.,1.,1.,1.,1.,1.,1.,1.,
1.,1.,1.,1.,1.,1.,1.,1.,1.,1.,1.,1.,1.,1.,1.,1.,1.,1.,1.,1.,1.,1.,1.,1.,
1.,1.,1.,1.,1.,1.,1.,1.,1.,1.,1.,1.,1.,1.,1.,1.,1.,1.,1.,1.,1.,1.,1.,1.,
1.,1.,1.,1.,1.,1.,1.,1.,1.,1.,1.,1.,1.,1.,1.,1.,1.,1.,1.,1.,1.,1.,1.,1.,
1.,1.,1.,1.,1.,1.,1.,1.,1.,1.,1.,1.,1.,1.,1.,1.,1.,1.,1.,1.,1.,1.,1.,1.,
1.,1.,1.,1.,1.,1.,1.,1.,1.,1.,1.,1.,1.,1.,1.,1.,1.,1.,1.,1.,1.,1.,1.,1.,
1.,1.,1.,1.,1.,1.,1.,1.,1.,1.,1.,1.,1.,1.,1.,1.,1.,1.,1.,1.,1.))
REPRESENTATION_ITEM('')
);
#801=(
BOUNDED_CURVE()
B_SPLINE_CURVE(5,(#222198,#222199,#222200,#222201,#222202,#222203,#222204,
#222205,#222206,#222207,#222208,#222209,#222210,#222211,#222212,#222213,
#222214,#222215,#222216,#222217,#222218,#222219,#222220,#222221,#222222,
#222223,#222224,#222225,#222226,#222227,#222228,#222229,#222230,#222231,
#222232,#222233,#222234,#222235,#222236,#222237,#222238,#222239,#222240,
#222241,#222242,#222243,#222244,#222245,#222246,#222247,#222248,#222249,
#222250,#222251,#222252,#222253,#222254,#222255,#222256,#222257,#222258,
#222259,#222260,#222261,#222262,#222263,#222264,#222265,#222266,#222267,
#222268,#222269,#222270,#222271,#222272,#222273,#222274,#222275,#222276,
#222277,#222278,#222279,#222280,#222281,#222282,#222283,#222284,#222285,
#222286,#222287,#222288,#222289,#222290,#222291,#222292,#222293,#222294,
#222295,#222296,#222297,#222298,#222299,#222300,#222301,#222302,#222303,
#222304,#222305,#222306,#222307,#222308,#222309,#222310,#222311,#222312,
#222313,#222314,#222315,#222316,#222317,#222318,#222319,#222320,#222321,
#222322,#222323,#222324,#222325,#222326,#222327,#222328,#222329,#222330,
#222331,#222332,#222333,#222334,#222335,#222336,#222337,#222338,#222339,
#222340,#222341,#222342,#222343,#222344,#222345,#222346,#222347,#222348,
#222349,#222350,#222351,#222352,#222353,#222354,#222355,#222356,#222357,
#222358,#222359,#222360,#222361,#222362,#222363,#222364,#222365,#222366,
#222367,#222368,#222369,#222370,#222371,#222372,#222373,#222374,#222375,
#222376,#222377,#222378,#222379,#222380,#222381,#222382,#222383,#222384,
#222385,#222386,#222387,#222388,#222389,#222390,#222391,#222392,#222393,
#222394,#222395,#222396,#222397,#222398,#222399,#222400,#222401,#222402),
 .UNSPECIFIED.,.F.,.F.)
B_SPLINE_CURVE_WITH_KNOTS((6,1,1,1,1,1,1,1,1,1,1,1,1,1,1,1,1,1,1,1,1,1,
1,1,1,1,1,1,1,1,1,1,1,1,1,1,1,1,1,1,1,1,1,1,1,1,1,1,1,1,1,1,1,1,1,1,1,1,
1,1,1,1,1,1,1,1,1,1,1,1,1,1,1,1,1,1,1,1,1,1,1,1,1,1,1,1,1,1,1,1,1,1,1,1,
1,1,1,1,1,1,1,1,1,1,1,1,1,1,1,1,1,1,1,1,1,1,1,1,1,1,1,1,1,1,1,1,1,1,1,1,
1,1,1,1,1,1,1,1,1,1,1,1,1,1,1,1,1,1,1,1,1,1,1,1,1,1,1,1,1,1,1,1,1,1,1,1,
1,1,1,1,1,1,1,1,1,1,1,1,1,1,1,1,1,1,1,1,1,1,1,1,1,1,1,1,1,1,1,1,1,1,6),
(0.,0.005,0.01,0.015,0.02,0.025,0.03,0.035,0.04,0.045,0.05,0.055,0.06,0.065,
0.07,0.075,0.08,0.085,0.09,0.095,0.1,0.105,0.11,0.115,0.12,0.125,0.13,0.135,
0.14,0.145,0.15,0.155,0.16,0.165,0.17,0.175,0.18,0.185,0.19,0.195,0.2,0.205,
0.21,0.215,0.22,0.225,0.23,0.235,0.24,0.245,0.25,0.255,0.26,0.265,0.27,
0.275,0.28,0.285,0.29,0.295,0.3,0.305,0.31,0.315,0.32,0.325,0.33,0.335,
0.34,0.345,0.35,0.355,0.36,0.365,0.37,0.375,0.38,0.385,0.39,0.395,0.4,0.405,
0.41,0.415,0.42,0.425,0.43,0.435,0.44,0.445,0.45,0.455,0.46,0.465,0.47,
0.475,0.48,0.485,0.49,0.495,0.5,0.505,0.51,0.515,0.52,0.525,0.53,0.535,
0.54,0.545,0.55,0.555,0.56,0.565,0.57,0.575,0.58,0.585,0.59,0.595,0.6,0.605,
0.61,0.615,0.62,0.625,0.63,0.635,0.64,0.645,0.65,0.655,0.66,0.665,0.67,
0.675,0.68,0.685,0.690000000000001,0.695000000000001,0.700000000000001,
0.705000000000001,0.710000000000001,0.715000000000001,0.720000000000001,
0.725000000000001,0.730000000000001,0.735000000000001,0.740000000000001,
0.745000000000001,0.750000000000001,0.755000000000001,0.760000000000001,
0.765000000000001,0.770000000000001,0.775000000000001,0.780000000000001,
0.785000000000001,0.790000000000001,0.795000000000001,0.800000000000001,
0.805000000000001,0.810000000000001,0.815000000000001,0.820000000000001,
0.825000000000001,0.830000000000001,0.835000000000001,0.840000000000001,
0.845000000000001,0.850000000000001,0.855000000000001,0.860000000000001,
0.865000000000001,0.870000000000001,0.875000000000001,0.880000000000001,
0.885000000000001,0.890000000000001,0.895000000000001,0.900000000000001,
0.905000000000001,0.910000000000001,0.915000000000001,0.920000000000001,
0.925000000000001,0.930000000000001,0.935000000000001,0.940000000000001,
0.945000000000001,0.950000000000001,0.955000000000001,0.960000000000001,
0.965000000000001,0.970000000000001,0.975000000000001,0.980000000000001,
0.985000000000001,0.990000000000001,0.995000000000001,1.),.UNSPECIFIED.)
CURVE()
GEOMETRIC_REPRESENTATION_ITEM()
RATIONAL_B_SPLINE_CURVE((1.,1.,1.,1.,1.,1.,1.,1.,1.,1.,1.,1.,1.,1.,1.,1.,
1.,1.,1.,1.,1.,1.,1.,1.,1.,1.,1.,1.,1.,1.,1.,1.,1.,1.,1.,1.,1.,1.,1.,1.,
1.,1.,1.,1.,1.,1.,1.,1.,1.,1.,1.,1.,1.,1.,1.,1.,1.,1.,1.,1.,1.,1.,1.,1.,
1.,1.,1.,1.,1.,1.,1.,1.,1.,1.,1.,1.,1.,1.,1.,1.,1.,1.,1.,1.,1.,1.,1.,1.,
1.,1.,1.,1.,1.,1.,1.,1.,1.,1.,1.,1.,1.,1.,1.,1.,1.,1.,1.,1.,1.,1.,1.,1.,
1.,1.,1.,1.,1.,1.,1.,1.,1.,1.,1.,1.,1.,1.,1.,1.,1.,1.,1.,1.,1.,1.,1.,1.,
1.,1.,1.,1.,1.,1.,1.,1.,1.,1.,1.,1.,1.,1.,1.,1.,1.,1.,1.,1.,1.,1.,1.,1.,
1.,1.,1.,1.,1.,1.,1.,1.,1.,1.,1.,1.,1.,1.,1.,1.,1.,1.,1.,1.,1.,1.,1.,1.,
1.,1.,1.,1.,1.,1.,1.,1.,1.,1.,1.,1.,1.,1.,1.,1.,1.,1.,1.,1.,1.))
REPRESENTATION_ITEM('')
);
#802=(
BOUNDED_CURVE()
B_SPLINE_CURVE(5,(#222404,#222405,#222406,#222407,#222408,#222409,#222410,
#222411,#222412,#222413,#222414,#222415,#222416,#222417,#222418,#222419,
#222420,#222421,#222422,#222423,#222424,#222425,#222426,#222427,#222428,
#222429,#222430,#222431,#222432,#222433,#222434,#222435,#222436,#222437,
#222438,#222439,#222440,#222441,#222442,#222443,#222444,#222445,#222446,
#222447,#222448,#222449,#222450,#222451,#222452,#222453,#222454,#222455,
#222456,#222457,#222458,#222459,#222460,#222461,#222462,#222463,#222464,
#222465,#222466,#222467,#222468,#222469,#222470,#222471,#222472,#222473,
#222474,#222475,#222476,#222477,#222478,#222479,#222480,#222481,#222482,
#222483,#222484,#222485,#222486,#222487,#222488,#222489,#222490,#222491,
#222492,#222493,#222494,#222495,#222496,#222497,#222498,#222499,#222500,
#222501,#222502,#222503,#222504,#222505,#222506,#222507,#222508,#222509,
#222510,#222511,#222512,#222513,#222514,#222515,#222516,#222517,#222518,
#222519,#222520,#222521,#222522,#222523,#222524,#222525,#222526,#222527,
#222528,#222529,#222530,#222531,#222532,#222533,#222534,#222535,#222536,
#222537,#222538,#222539,#222540,#222541,#222542,#222543,#222544,#222545,
#222546,#222547,#222548,#222549,#222550,#222551,#222552,#222553,#222554,
#222555,#222556,#222557,#222558,#222559,#222560,#222561,#222562,#222563,
#222564,#222565,#222566,#222567,#222568,#222569,#222570,#222571,#222572,
#222573,#222574,#222575,#222576,#222577,#222578,#222579,#222580,#222581,
#222582,#222583,#222584,#222585,#222586,#222587,#222588,#222589,#222590,
#222591,#222592,#222593,#222594,#222595,#222596,#222597,#222598,#222599,
#222600,#222601,#222602,#222603,#222604,#222605,#222606,#222607,#222608),
 .UNSPECIFIED.,.F.,.F.)
B_SPLINE_CURVE_WITH_KNOTS((6,1,1,1,1,1,1,1,1,1,1,1,1,1,1,1,1,1,1,1,1,1,
1,1,1,1,1,1,1,1,1,1,1,1,1,1,1,1,1,1,1,1,1,1,1,1,1,1,1,1,1,1,1,1,1,1,1,1,
1,1,1,1,1,1,1,1,1,1,1,1,1,1,1,1,1,1,1,1,1,1,1,1,1,1,1,1,1,1,1,1,1,1,1,1,
1,1,1,1,1,1,1,1,1,1,1,1,1,1,1,1,1,1,1,1,1,1,1,1,1,1,1,1,1,1,1,1,1,1,1,1,
1,1,1,1,1,1,1,1,1,1,1,1,1,1,1,1,1,1,1,1,1,1,1,1,1,1,1,1,1,1,1,1,1,1,1,1,
1,1,1,1,1,1,1,1,1,1,1,1,1,1,1,1,1,1,1,1,1,1,1,1,1,1,1,1,1,1,1,1,1,1,6),
(-1.,-0.995000000000001,-0.990000000000001,-0.985000000000001,-0.980000000000001,
-0.975000000000001,-0.970000000000001,-0.965000000000001,-0.960000000000001,
-0.955000000000001,-0.950000000000001,-0.945000000000001,-0.940000000000001,
-0.935000000000001,-0.930000000000001,-0.925000000000001,-0.920000000000001,
-0.915000000000001,-0.910000000000001,-0.905000000000001,-0.900000000000001,
-0.895000000000001,-0.890000000000001,-0.885000000000001,-0.880000000000001,
-0.875000000000001,-0.870000000000001,-0.865000000000001,-0.860000000000001,
-0.855000000000001,-0.850000000000001,-0.845000000000001,-0.840000000000001,
-0.835000000000001,-0.830000000000001,-0.825000000000001,-0.820000000000001,
-0.815000000000001,-0.810000000000001,-0.805000000000001,-0.800000000000001,
-0.795000000000001,-0.790000000000001,-0.785000000000001,-0.780000000000001,
-0.775000000000001,-0.770000000000001,-0.765000000000001,-0.760000000000001,
-0.755000000000001,-0.750000000000001,-0.745000000000001,-0.740000000000001,
-0.735000000000001,-0.730000000000001,-0.725000000000001,-0.720000000000001,
-0.715000000000001,-0.710000000000001,-0.705000000000001,-0.700000000000001,
-0.695000000000001,-0.690000000000001,-0.685,-0.68,-0.675,-0.67,-0.665,
-0.66,-0.655,-0.65,-0.645,-0.64,-0.635,-0.63,-0.625,-0.62,-0.615,-0.61,
-0.605,-0.6,-0.595,-0.59,-0.585,-0.58,-0.575,-0.57,-0.565,-0.56,-0.555,
-0.55,-0.545,-0.54,-0.535,-0.53,-0.525,-0.52,-0.515,-0.51,-0.505,-0.5,-0.495,
-0.49,-0.485,-0.48,-0.475,-0.47,-0.465,-0.46,-0.455,-0.45,-0.445,-0.44,
-0.435,-0.43,-0.425,-0.42,-0.415,-0.41,-0.405,-0.4,-0.395,-0.39,-0.385,
-0.38,-0.375,-0.37,-0.365,-0.36,-0.355,-0.35,-0.345,-0.34,-0.335,-0.33,
-0.325,-0.32,-0.315,-0.31,-0.305,-0.3,-0.295,-0.29,-0.285,-0.28,-0.275,
-0.27,-0.265,-0.26,-0.255,-0.25,-0.245,-0.24,-0.235,-0.23,-0.225,-0.22,
-0.215,-0.21,-0.205,-0.2,-0.195,-0.19,-0.185,-0.18,-0.175,-0.17,-0.165,
-0.16,-0.155,-0.15,-0.145,-0.14,-0.135,-0.13,-0.125,-0.12,-0.115,-0.11,
-0.105,-0.1,-0.095,-0.09,-0.085,-0.08,-0.075,-0.07,-0.065,-0.06,-0.055,
-0.05,-0.045,-0.04,-0.035,-0.03,-0.025,-0.02,-0.015,-0.01,-0.005,0.),
 .UNSPECIFIED.)
CURVE()
GEOMETRIC_REPRESENTATION_ITEM()
RATIONAL_B_SPLINE_CURVE((1.,1.,1.,1.,1.,1.,1.,1.,1.,1.,1.,1.,1.,1.,1.,1.,
1.,1.,1.,1.,1.,1.,1.,1.,1.,1.,1.,1.,1.,1.,1.,1.,1.,1.,1.,1.,1.,1.,1.,1.,
1.,1.,1.,1.,1.,1.,1.,1.,1.,1.,1.,1.,1.,1.,1.,1.,1.,1.,1.,1.,1.,1.,1.,1.,
1.,1.,1.,1.,1.,1.,1.,1.,1.,1.,1.,1.,1.,1.,1.,1.,1.,1.,1.,1.,1.,1.,1.,1.,
1.,1.,1.,1.,1.,1.,1.,1.,1.,1.,1.,1.,1.,1.,1.,1.,1.,1.,1.,1.,1.,1.,1.,1.,
1.,1.,1.,1.,1.,1.,1.,1.,1.,1.,1.,1.,1.,1.,1.,1.,1.,1.,1.,1.,1.,1.,1.,1.,
1.,1.,1.,1.,1.,1.,1.,1.,1.,1.,1.,1.,1.,1.,1.,1.,1.,1.,1.,1.,1.,1.,1.,1.,
1.,1.,1.,1.,1.,1.,1.,1.,1.,1.,1.,1.,1.,1.,1.,1.,1.,1.,1.,1.,1.,1.,1.,1.,
1.,1.,1.,1.,1.,1.,1.,1.,1.,1.,1.,1.,1.,1.,1.,1.,1.,1.,1.,1.,1.))
REPRESENTATION_ITEM('')
);
#803=(
BOUNDED_CURVE()
B_SPLINE_CURVE(5,(#223027,#223028,#223029,#223030,#223031,#223032,#223033,
#223034,#223035,#223036,#223037,#223038,#223039,#223040,#223041,#223042,
#223043,#223044,#223045,#223046,#223047,#223048,#223049,#223050,#223051,
#223052,#223053,#223054,#223055,#223056,#223057,#223058,#223059,#223060,
#223061,#223062,#223063,#223064,#223065,#223066,#223067,#223068,#223069,
#223070,#223071,#223072,#223073,#223074,#223075,#223076,#223077,#223078,
#223079,#223080,#223081,#223082,#223083,#223084,#223085,#223086,#223087,
#223088,#223089,#223090,#223091,#223092,#223093,#223094,#223095,#223096,
#223097,#223098,#223099,#223100,#223101,#223102,#223103,#223104,#223105,
#223106,#223107,#223108,#223109,#223110,#223111,#223112,#223113,#223114,
#223115,#223116,#223117,#223118,#223119,#223120,#223121,#223122,#223123,
#223124,#223125,#223126,#223127,#223128,#223129,#223130,#223131,#223132,
#223133,#223134,#223135,#223136,#223137,#223138,#223139,#223140,#223141,
#223142,#223143,#223144,#223145,#223146,#223147,#223148,#223149,#223150,
#223151,#223152,#223153,#223154,#223155,#223156,#223157,#223158,#223159,
#223160,#223161,#223162,#223163,#223164,#223165,#223166,#223167,#223168,
#223169,#223170,#223171,#223172,#223173,#223174,#223175,#223176,#223177,
#223178,#223179,#223180,#223181,#223182,#223183,#223184,#223185,#223186,
#223187,#223188,#223189,#223190,#223191,#223192,#223193,#223194,#223195,
#223196,#223197,#223198,#223199,#223200,#223201,#223202,#223203,#223204,
#223205,#223206,#223207,#223208,#223209,#223210,#223211,#223212,#223213,
#223214,#223215,#223216,#223217,#223218,#223219,#223220,#223221,#223222,
#223223,#223224,#223225,#223226,#223227,#223228,#223229,#223230,#223231),
 .UNSPECIFIED.,.F.,.F.)
B_SPLINE_CURVE_WITH_KNOTS((6,1,1,1,1,1,1,1,1,1,1,1,1,1,1,1,1,1,1,1,1,1,
1,1,1,1,1,1,1,1,1,1,1,1,1,1,1,1,1,1,1,1,1,1,1,1,1,1,1,1,1,1,1,1,1,1,1,1,
1,1,1,1,1,1,1,1,1,1,1,1,1,1,1,1,1,1,1,1,1,1,1,1,1,1,1,1,1,1,1,1,1,1,1,1,
1,1,1,1,1,1,1,1,1,1,1,1,1,1,1,1,1,1,1,1,1,1,1,1,1,1,1,1,1,1,1,1,1,1,1,1,
1,1,1,1,1,1,1,1,1,1,1,1,1,1,1,1,1,1,1,1,1,1,1,1,1,1,1,1,1,1,1,1,1,1,1,1,
1,1,1,1,1,1,1,1,1,1,1,1,1,1,1,1,1,1,1,1,1,1,1,1,1,1,1,1,1,1,1,1,1,1,6),
(-1.,-0.995000000000001,-0.990000000000001,-0.985000000000001,-0.980000000000001,
-0.975000000000001,-0.970000000000001,-0.965000000000001,-0.960000000000001,
-0.955000000000001,-0.950000000000001,-0.945000000000001,-0.940000000000001,
-0.935000000000001,-0.930000000000001,-0.925000000000001,-0.920000000000001,
-0.915000000000001,-0.910000000000001,-0.905000000000001,-0.900000000000001,
-0.895000000000001,-0.890000000000001,-0.885000000000001,-0.880000000000001,
-0.875000000000001,-0.870000000000001,-0.865000000000001,-0.860000000000001,
-0.855000000000001,-0.850000000000001,-0.845000000000001,-0.840000000000001,
-0.835000000000001,-0.830000000000001,-0.825000000000001,-0.820000000000001,
-0.815000000000001,-0.810000000000001,-0.805000000000001,-0.800000000000001,
-0.795000000000001,-0.790000000000001,-0.785000000000001,-0.780000000000001,
-0.775000000000001,-0.770000000000001,-0.765000000000001,-0.760000000000001,
-0.755000000000001,-0.750000000000001,-0.745000000000001,-0.740000000000001,
-0.735000000000001,-0.730000000000001,-0.725000000000001,-0.720000000000001,
-0.715000000000001,-0.710000000000001,-0.705000000000001,-0.700000000000001,
-0.695000000000001,-0.690000000000001,-0.685,-0.68,-0.675,-0.67,-0.665,
-0.66,-0.655,-0.65,-0.645,-0.64,-0.635,-0.63,-0.625,-0.62,-0.615,-0.61,
-0.605,-0.6,-0.595,-0.59,-0.585,-0.58,-0.575,-0.57,-0.565,-0.56,-0.555,
-0.55,-0.545,-0.54,-0.535,-0.53,-0.525,-0.52,-0.515,-0.51,-0.505,-0.5,-0.495,
-0.49,-0.485,-0.48,-0.475,-0.47,-0.465,-0.46,-0.455,-0.45,-0.445,-0.44,
-0.435,-0.43,-0.425,-0.42,-0.415,-0.41,-0.405,-0.4,-0.395,-0.39,-0.385,
-0.38,-0.375,-0.37,-0.365,-0.36,-0.355,-0.35,-0.345,-0.34,-0.335,-0.33,
-0.325,-0.32,-0.315,-0.31,-0.305,-0.3,-0.295,-0.29,-0.285,-0.28,-0.275,
-0.27,-0.265,-0.26,-0.255,-0.25,-0.245,-0.24,-0.235,-0.23,-0.225,-0.22,
-0.215,-0.21,-0.205,-0.2,-0.195,-0.19,-0.185,-0.18,-0.175,-0.17,-0.165,
-0.16,-0.155,-0.15,-0.145,-0.14,-0.135,-0.13,-0.125,-0.12,-0.115,-0.11,
-0.105,-0.1,-0.095,-0.09,-0.085,-0.08,-0.075,-0.07,-0.065,-0.06,-0.055,
-0.05,-0.045,-0.04,-0.035,-0.03,-0.025,-0.02,-0.015,-0.01,-0.005,0.),
 .UNSPECIFIED.)
CURVE()
GEOMETRIC_REPRESENTATION_ITEM()
RATIONAL_B_SPLINE_CURVE((1.,1.,1.,1.,1.,1.,1.,1.,1.,1.,1.,1.,1.,1.,1.,1.,
1.,1.,1.,1.,1.,1.,1.,1.,1.,1.,1.,1.,1.,1.,1.,1.,1.,1.,1.,1.,1.,1.,1.,1.,
1.,1.,1.,1.,1.,1.,1.,1.,1.,1.,1.,1.,1.,1.,1.,1.,1.,1.,1.,1.,1.,1.,1.,1.,
1.,1.,1.,1.,1.,1.,1.,1.,1.,1.,1.,1.,1.,1.,1.,1.,1.,1.,1.,1.,1.,1.,1.,1.,
1.,1.,1.,1.,1.,1.,1.,1.,1.,1.,1.,1.,1.,1.,1.,1.,1.,1.,1.,1.,1.,1.,1.,1.,
1.,1.,1.,1.,1.,1.,1.,1.,1.,1.,1.,1.,1.,1.,1.,1.,1.,1.,1.,1.,1.,1.,1.,1.,
1.,1.,1.,1.,1.,1.,1.,1.,1.,1.,1.,1.,1.,1.,1.,1.,1.,1.,1.,1.,1.,1.,1.,1.,
1.,1.,1.,1.,1.,1.,1.,1.,1.,1.,1.,1.,1.,1.,1.,1.,1.,1.,1.,1.,1.,1.,1.,1.,
1.,1.,1.,1.,1.,1.,1.,1.,1.,1.,1.,1.,1.,1.,1.,1.,1.,1.,1.,1.,1.))
REPRESENTATION_ITEM('')
);
#804=(
BOUNDED_CURVE()
B_SPLINE_CURVE(5,(#223234,#223235,#223236,#223237,#223238,#223239,#223240,
#223241,#223242,#223243,#223244,#223245,#223246,#223247,#223248,#223249,
#223250,#223251,#223252,#223253,#223254,#223255,#223256,#223257,#223258,
#223259,#223260,#223261,#223262,#223263,#223264,#223265,#223266,#223267,
#223268,#223269,#223270,#223271,#223272,#223273,#223274,#223275,#223276,
#223277,#223278,#223279,#223280,#223281,#223282,#223283,#223284,#223285,
#223286,#223287,#223288,#223289,#223290,#223291,#223292,#223293,#223294,
#223295,#223296,#223297,#223298,#223299,#223300,#223301,#223302,#223303,
#223304,#223305,#223306,#223307,#223308,#223309,#223310,#223311,#223312,
#223313,#223314,#223315,#223316,#223317,#223318,#223319,#223320,#223321,
#223322,#223323,#223324,#223325,#223326,#223327,#223328,#223329,#223330,
#223331,#223332,#223333,#223334,#223335,#223336,#223337,#223338,#223339,
#223340,#223341,#223342,#223343,#223344,#223345,#223346,#223347,#223348,
#223349,#223350,#223351,#223352,#223353,#223354,#223355,#223356,#223357,
#223358,#223359,#223360,#223361,#223362,#223363,#223364,#223365,#223366,
#223367,#223368,#223369,#223370,#223371,#223372,#223373,#223374,#223375,
#223376,#223377,#223378,#223379,#223380,#223381,#223382,#223383,#223384,
#223385,#223386,#223387,#223388,#223389,#223390,#223391,#223392,#223393,
#223394,#223395,#223396,#223397,#223398,#223399,#223400,#223401,#223402,
#223403,#223404,#223405,#223406,#223407,#223408,#223409,#223410,#223411,
#223412,#223413,#223414,#223415,#223416,#223417,#223418,#223419,#223420,
#223421,#223422,#223423,#223424,#223425,#223426,#223427,#223428,#223429,
#223430,#223431,#223432,#223433,#223434,#223435,#223436,#223437,#223438),
 .UNSPECIFIED.,.F.,.F.)
B_SPLINE_CURVE_WITH_KNOTS((6,1,1,1,1,1,1,1,1,1,1,1,1,1,1,1,1,1,1,1,1,1,
1,1,1,1,1,1,1,1,1,1,1,1,1,1,1,1,1,1,1,1,1,1,1,1,1,1,1,1,1,1,1,1,1,1,1,1,
1,1,1,1,1,1,1,1,1,1,1,1,1,1,1,1,1,1,1,1,1,1,1,1,1,1,1,1,1,1,1,1,1,1,1,1,
1,1,1,1,1,1,1,1,1,1,1,1,1,1,1,1,1,1,1,1,1,1,1,1,1,1,1,1,1,1,1,1,1,1,1,1,
1,1,1,1,1,1,1,1,1,1,1,1,1,1,1,1,1,1,1,1,1,1,1,1,1,1,1,1,1,1,1,1,1,1,1,1,
1,1,1,1,1,1,1,1,1,1,1,1,1,1,1,1,1,1,1,1,1,1,1,1,1,1,1,1,1,1,1,1,1,1,6),
(0.,0.005,0.01,0.015,0.02,0.025,0.03,0.035,0.04,0.045,0.05,0.055,0.06,0.065,
0.07,0.075,0.08,0.085,0.09,0.095,0.1,0.105,0.11,0.115,0.12,0.125,0.13,0.135,
0.14,0.145,0.15,0.155,0.16,0.165,0.17,0.175,0.18,0.185,0.19,0.195,0.2,0.205,
0.21,0.215,0.22,0.225,0.23,0.235,0.24,0.245,0.25,0.255,0.26,0.265,0.27,
0.275,0.28,0.285,0.29,0.295,0.3,0.305,0.31,0.315,0.32,0.325,0.33,0.335,
0.34,0.345,0.35,0.355,0.36,0.365,0.37,0.375,0.38,0.385,0.39,0.395,0.4,0.405,
0.41,0.415,0.42,0.425,0.43,0.435,0.44,0.445,0.45,0.455,0.46,0.465,0.47,
0.475,0.48,0.485,0.49,0.495,0.5,0.505,0.51,0.515,0.52,0.525,0.53,0.535,
0.54,0.545,0.55,0.555,0.56,0.565,0.57,0.575,0.58,0.585,0.59,0.595,0.6,0.605,
0.61,0.615,0.62,0.625,0.63,0.635,0.64,0.645,0.65,0.655,0.66,0.665,0.67,
0.675,0.68,0.685,0.690000000000001,0.695000000000001,0.700000000000001,
0.705000000000001,0.710000000000001,0.715000000000001,0.720000000000001,
0.725000000000001,0.730000000000001,0.735000000000001,0.740000000000001,
0.745000000000001,0.750000000000001,0.755000000000001,0.760000000000001,
0.765000000000001,0.770000000000001,0.775000000000001,0.780000000000001,
0.785000000000001,0.790000000000001,0.795000000000001,0.800000000000001,
0.805000000000001,0.810000000000001,0.815000000000001,0.820000000000001,
0.825000000000001,0.830000000000001,0.835000000000001,0.840000000000001,
0.845000000000001,0.850000000000001,0.855000000000001,0.860000000000001,
0.865000000000001,0.870000000000001,0.875000000000001,0.880000000000001,
0.885000000000001,0.890000000000001,0.895000000000001,0.900000000000001,
0.905000000000001,0.910000000000001,0.915000000000001,0.920000000000001,
0.925000000000001,0.930000000000001,0.935000000000001,0.940000000000001,
0.945000000000001,0.950000000000001,0.955000000000001,0.960000000000001,
0.965000000000001,0.970000000000001,0.975000000000001,0.980000000000001,
0.985000000000001,0.990000000000001,0.995000000000001,1.),.UNSPECIFIED.)
CURVE()
GEOMETRIC_REPRESENTATION_ITEM()
RATIONAL_B_SPLINE_CURVE((1.,1.,1.,1.,1.,1.,1.,1.,1.,1.,1.,1.,1.,1.,1.,1.,
1.,1.,1.,1.,1.,1.,1.,1.,1.,1.,1.,1.,1.,1.,1.,1.,1.,1.,1.,1.,1.,1.,1.,1.,
1.,1.,1.,1.,1.,1.,1.,1.,1.,1.,1.,1.,1.,1.,1.,1.,1.,1.,1.,1.,1.,1.,1.,1.,
1.,1.,1.,1.,1.,1.,1.,1.,1.,1.,1.,1.,1.,1.,1.,1.,1.,1.,1.,1.,1.,1.,1.,1.,
1.,1.,1.,1.,1.,1.,1.,1.,1.,1.,1.,1.,1.,1.,1.,1.,1.,1.,1.,1.,1.,1.,1.,1.,
1.,1.,1.,1.,1.,1.,1.,1.,1.,1.,1.,1.,1.,1.,1.,1.,1.,1.,1.,1.,1.,1.,1.,1.,
1.,1.,1.,1.,1.,1.,1.,1.,1.,1.,1.,1.,1.,1.,1.,1.,1.,1.,1.,1.,1.,1.,1.,1.,
1.,1.,1.,1.,1.,1.,1.,1.,1.,1.,1.,1.,1.,1.,1.,1.,1.,1.,1.,1.,1.,1.,1.,1.,
1.,1.,1.,1.,1.,1.,1.,1.,1.,1.,1.,1.,1.,1.,1.,1.,1.,1.,1.,1.,1.))
REPRESENTATION_ITEM('')
);
#805=(
BOUNDED_CURVE()
B_SPLINE_CURVE(5,(#223850,#223851,#223852,#223853,#223854,#223855,#223856,
#223857,#223858,#223859,#223860,#223861,#223862,#223863,#223864,#223865,
#223866,#223867,#223868,#223869,#223870,#223871,#223872,#223873,#223874,
#223875,#223876,#223877,#223878,#223879,#223880,#223881,#223882,#223883,
#223884,#223885,#223886,#223887,#223888,#223889,#223890,#223891,#223892,
#223893,#223894,#223895,#223896,#223897,#223898,#223899,#223900,#223901,
#223902,#223903,#223904,#223905,#223906,#223907,#223908,#223909,#223910,
#223911,#223912,#223913,#223914,#223915,#223916,#223917,#223918,#223919,
#223920,#223921,#223922,#223923,#223924,#223925,#223926,#223927,#223928,
#223929,#223930,#223931,#223932,#223933,#223934,#223935,#223936,#223937,
#223938,#223939,#223940,#223941,#223942,#223943,#223944,#223945,#223946,
#223947,#223948,#223949,#223950,#223951,#223952,#223953,#223954,#223955,
#223956,#223957,#223958,#223959,#223960,#223961,#223962,#223963,#223964,
#223965,#223966,#223967,#223968,#223969,#223970,#223971,#223972,#223973,
#223974,#223975,#223976,#223977,#223978,#223979,#223980,#223981,#223982,
#223983,#223984,#223985,#223986,#223987,#223988,#223989,#223990,#223991,
#223992,#223993,#223994,#223995,#223996,#223997,#223998,#223999,#224000,
#224001,#224002,#224003,#224004,#224005,#224006,#224007,#224008,#224009,
#224010,#224011,#224012,#224013,#224014,#224015,#224016,#224017,#224018,
#224019,#224020,#224021,#224022,#224023,#224024,#224025,#224026,#224027,
#224028,#224029,#224030,#224031,#224032,#224033,#224034,#224035,#224036,
#224037,#224038,#224039,#224040,#224041,#224042,#224043,#224044,#224045,
#224046,#224047,#224048,#224049,#224050,#224051,#224052,#224053,#224054),
 .UNSPECIFIED.,.F.,.F.)
B_SPLINE_CURVE_WITH_KNOTS((6,1,1,1,1,1,1,1,1,1,1,1,1,1,1,1,1,1,1,1,1,1,
1,1,1,1,1,1,1,1,1,1,1,1,1,1,1,1,1,1,1,1,1,1,1,1,1,1,1,1,1,1,1,1,1,1,1,1,
1,1,1,1,1,1,1,1,1,1,1,1,1,1,1,1,1,1,1,1,1,1,1,1,1,1,1,1,1,1,1,1,1,1,1,1,
1,1,1,1,1,1,1,1,1,1,1,1,1,1,1,1,1,1,1,1,1,1,1,1,1,1,1,1,1,1,1,1,1,1,1,1,
1,1,1,1,1,1,1,1,1,1,1,1,1,1,1,1,1,1,1,1,1,1,1,1,1,1,1,1,1,1,1,1,1,1,1,1,
1,1,1,1,1,1,1,1,1,1,1,1,1,1,1,1,1,1,1,1,1,1,1,1,1,1,1,1,1,1,1,1,1,1,6),
(0.,0.005,0.01,0.015,0.02,0.025,0.03,0.035,0.04,0.045,0.05,0.055,0.06,0.065,
0.07,0.075,0.08,0.085,0.09,0.095,0.1,0.105,0.11,0.115,0.12,0.125,0.13,0.135,
0.14,0.145,0.15,0.155,0.16,0.165,0.17,0.175,0.18,0.185,0.19,0.195,0.2,0.205,
0.21,0.215,0.22,0.225,0.23,0.235,0.24,0.245,0.25,0.255,0.26,0.265,0.27,
0.275,0.28,0.285,0.29,0.295,0.3,0.305,0.31,0.315,0.32,0.325,0.33,0.335,
0.34,0.345,0.35,0.355,0.36,0.365,0.37,0.375,0.38,0.385,0.39,0.395,0.4,0.405,
0.41,0.415,0.42,0.425,0.43,0.435,0.44,0.445,0.45,0.455,0.46,0.465,0.47,
0.475,0.48,0.485,0.49,0.495,0.5,0.505,0.51,0.515,0.52,0.525,0.53,0.535,
0.54,0.545,0.55,0.555,0.56,0.565,0.57,0.575,0.58,0.585,0.59,0.595,0.6,0.605,
0.61,0.615,0.62,0.625,0.63,0.635,0.64,0.645,0.65,0.655,0.66,0.665,0.67,
0.675,0.68,0.685,0.690000000000001,0.695000000000001,0.700000000000001,
0.705000000000001,0.710000000000001,0.715000000000001,0.720000000000001,
0.725000000000001,0.730000000000001,0.735000000000001,0.740000000000001,
0.745000000000001,0.750000000000001,0.755000000000001,0.760000000000001,
0.765000000000001,0.770000000000001,0.775000000000001,0.780000000000001,
0.785000000000001,0.790000000000001,0.795000000000001,0.800000000000001,
0.805000000000001,0.810000000000001,0.815000000000001,0.820000000000001,
0.825000000000001,0.830000000000001,0.835000000000001,0.840000000000001,
0.845000000000001,0.850000000000001,0.855000000000001,0.860000000000001,
0.865000000000001,0.870000000000001,0.875000000000001,0.880000000000001,
0.885000000000001,0.890000000000001,0.895000000000001,0.900000000000001,
0.905000000000001,0.910000000000001,0.915000000000001,0.920000000000001,
0.925000000000001,0.930000000000001,0.935000000000001,0.940000000000001,
0.945000000000001,0.950000000000001,0.955000000000001,0.960000000000001,
0.965000000000001,0.970000000000001,0.975000000000001,0.980000000000001,
0.985000000000001,0.990000000000001,0.995000000000001,1.),.UNSPECIFIED.)
CURVE()
GEOMETRIC_REPRESENTATION_ITEM()
RATIONAL_B_SPLINE_CURVE((1.,1.,1.,1.,1.,1.,1.,1.,1.,1.,1.,1.,1.,1.,1.,1.,
1.,1.,1.,1.,1.,1.,1.,1.,1.,1.,1.,1.,1.,1.,1.,1.,1.,1.,1.,1.,1.,1.,1.,1.,
1.,1.,1.,1.,1.,1.,1.,1.,1.,1.,1.,1.,1.,1.,1.,1.,1.,1.,1.,1.,1.,1.,1.,1.,
1.,1.,1.,1.,1.,1.,1.,1.,1.,1.,1.,1.,1.,1.,1.,1.,1.,1.,1.,1.,1.,1.,1.,1.,
1.,1.,1.,1.,1.,1.,1.,1.,1.,1.,1.,1.,1.,1.,1.,1.,1.,1.,1.,1.,1.,1.,1.,1.,
1.,1.,1.,1.,1.,1.,1.,1.,1.,1.,1.,1.,1.,1.,1.,1.,1.,1.,1.,1.,1.,1.,1.,1.,
1.,1.,1.,1.,1.,1.,1.,1.,1.,1.,1.,1.,1.,1.,1.,1.,1.,1.,1.,1.,1.,1.,1.,1.,
1.,1.,1.,1.,1.,1.,1.,1.,1.,1.,1.,1.,1.,1.,1.,1.,1.,1.,1.,1.,1.,1.,1.,1.,
1.,1.,1.,1.,1.,1.,1.,1.,1.,1.,1.,1.,1.,1.,1.,1.,1.,1.,1.,1.,1.))
REPRESENTATION_ITEM('')
);
#806=(
BOUNDED_CURVE()
B_SPLINE_CURVE(5,(#224056,#224057,#224058,#224059,#224060,#224061,#224062,
#224063,#224064,#224065,#224066,#224067,#224068,#224069,#224070,#224071,
#224072,#224073,#224074,#224075,#224076,#224077,#224078,#224079,#224080,
#224081,#224082,#224083,#224084,#224085,#224086,#224087,#224088,#224089,
#224090,#224091,#224092,#224093,#224094,#224095,#224096,#224097,#224098,
#224099,#224100,#224101,#224102,#224103,#224104,#224105,#224106,#224107,
#224108,#224109,#224110,#224111,#224112,#224113,#224114,#224115,#224116,
#224117,#224118,#224119,#224120,#224121,#224122,#224123,#224124,#224125,
#224126,#224127,#224128,#224129,#224130,#224131,#224132,#224133,#224134,
#224135,#224136,#224137,#224138,#224139,#224140,#224141,#224142,#224143,
#224144,#224145,#224146,#224147,#224148,#224149,#224150,#224151,#224152,
#224153,#224154,#224155,#224156,#224157,#224158,#224159,#224160,#224161,
#224162,#224163,#224164,#224165,#224166,#224167,#224168,#224169,#224170,
#224171,#224172,#224173,#224174,#224175,#224176,#224177,#224178,#224179,
#224180,#224181,#224182,#224183,#224184,#224185,#224186,#224187,#224188,
#224189,#224190,#224191,#224192,#224193,#224194,#224195,#224196,#224197,
#224198,#224199,#224200,#224201,#224202,#224203,#224204,#224205,#224206,
#224207,#224208,#224209,#224210,#224211,#224212,#224213,#224214,#224215,
#224216,#224217,#224218,#224219,#224220,#224221,#224222,#224223,#224224,
#224225,#224226,#224227,#224228,#224229,#224230,#224231,#224232,#224233,
#224234,#224235,#224236,#224237,#224238,#224239,#224240,#224241,#224242,
#224243,#224244,#224245,#224246,#224247,#224248,#224249,#224250,#224251,
#224252,#224253,#224254,#224255,#224256,#224257,#224258,#224259,#224260),
 .UNSPECIFIED.,.F.,.F.)
B_SPLINE_CURVE_WITH_KNOTS((6,1,1,1,1,1,1,1,1,1,1,1,1,1,1,1,1,1,1,1,1,1,
1,1,1,1,1,1,1,1,1,1,1,1,1,1,1,1,1,1,1,1,1,1,1,1,1,1,1,1,1,1,1,1,1,1,1,1,
1,1,1,1,1,1,1,1,1,1,1,1,1,1,1,1,1,1,1,1,1,1,1,1,1,1,1,1,1,1,1,1,1,1,1,1,
1,1,1,1,1,1,1,1,1,1,1,1,1,1,1,1,1,1,1,1,1,1,1,1,1,1,1,1,1,1,1,1,1,1,1,1,
1,1,1,1,1,1,1,1,1,1,1,1,1,1,1,1,1,1,1,1,1,1,1,1,1,1,1,1,1,1,1,1,1,1,1,1,
1,1,1,1,1,1,1,1,1,1,1,1,1,1,1,1,1,1,1,1,1,1,1,1,1,1,1,1,1,1,1,1,1,1,6),
(-1.,-0.995000000000001,-0.990000000000001,-0.985000000000001,-0.980000000000001,
-0.975000000000001,-0.970000000000001,-0.965000000000001,-0.960000000000001,
-0.955000000000001,-0.950000000000001,-0.945000000000001,-0.940000000000001,
-0.935000000000001,-0.930000000000001,-0.925000000000001,-0.920000000000001,
-0.915000000000001,-0.910000000000001,-0.905000000000001,-0.900000000000001,
-0.895000000000001,-0.890000000000001,-0.885000000000001,-0.880000000000001,
-0.875000000000001,-0.870000000000001,-0.865000000000001,-0.860000000000001,
-0.855000000000001,-0.850000000000001,-0.845000000000001,-0.840000000000001,
-0.835000000000001,-0.830000000000001,-0.825000000000001,-0.820000000000001,
-0.815000000000001,-0.810000000000001,-0.805000000000001,-0.800000000000001,
-0.795000000000001,-0.790000000000001,-0.785000000000001,-0.780000000000001,
-0.775000000000001,-0.770000000000001,-0.765000000000001,-0.760000000000001,
-0.755000000000001,-0.750000000000001,-0.745000000000001,-0.740000000000001,
-0.735000000000001,-0.730000000000001,-0.725000000000001,-0.720000000000001,
-0.715000000000001,-0.710000000000001,-0.705000000000001,-0.700000000000001,
-0.695000000000001,-0.690000000000001,-0.685,-0.68,-0.675,-0.67,-0.665,
-0.66,-0.655,-0.65,-0.645,-0.64,-0.635,-0.63,-0.625,-0.62,-0.615,-0.61,
-0.605,-0.6,-0.595,-0.59,-0.585,-0.58,-0.575,-0.57,-0.565,-0.56,-0.555,
-0.55,-0.545,-0.54,-0.535,-0.53,-0.525,-0.52,-0.515,-0.51,-0.505,-0.5,-0.495,
-0.49,-0.485,-0.48,-0.475,-0.47,-0.465,-0.46,-0.455,-0.45,-0.445,-0.44,
-0.435,-0.43,-0.425,-0.42,-0.415,-0.41,-0.405,-0.4,-0.395,-0.39,-0.385,
-0.38,-0.375,-0.37,-0.365,-0.36,-0.355,-0.35,-0.345,-0.34,-0.335,-0.33,
-0.325,-0.32,-0.315,-0.31,-0.305,-0.3,-0.295,-0.29,-0.285,-0.28,-0.275,
-0.27,-0.265,-0.26,-0.255,-0.25,-0.245,-0.24,-0.235,-0.23,-0.225,-0.22,
-0.215,-0.21,-0.205,-0.2,-0.195,-0.19,-0.185,-0.18,-0.175,-0.17,-0.165,
-0.16,-0.155,-0.15,-0.145,-0.14,-0.135,-0.13,-0.125,-0.12,-0.115,-0.11,
-0.105,-0.1,-0.095,-0.09,-0.085,-0.08,-0.075,-0.07,-0.065,-0.06,-0.055,
-0.05,-0.045,-0.04,-0.035,-0.03,-0.025,-0.02,-0.015,-0.01,-0.005,0.),
 .UNSPECIFIED.)
CURVE()
GEOMETRIC_REPRESENTATION_ITEM()
RATIONAL_B_SPLINE_CURVE((1.,1.,1.,1.,1.,1.,1.,1.,1.,1.,1.,1.,1.,1.,1.,1.,
1.,1.,1.,1.,1.,1.,1.,1.,1.,1.,1.,1.,1.,1.,1.,1.,1.,1.,1.,1.,1.,1.,1.,1.,
1.,1.,1.,1.,1.,1.,1.,1.,1.,1.,1.,1.,1.,1.,1.,1.,1.,1.,1.,1.,1.,1.,1.,1.,
1.,1.,1.,1.,1.,1.,1.,1.,1.,1.,1.,1.,1.,1.,1.,1.,1.,1.,1.,1.,1.,1.,1.,1.,
1.,1.,1.,1.,1.,1.,1.,1.,1.,1.,1.,1.,1.,1.,1.,1.,1.,1.,1.,1.,1.,1.,1.,1.,
1.,1.,1.,1.,1.,1.,1.,1.,1.,1.,1.,1.,1.,1.,1.,1.,1.,1.,1.,1.,1.,1.,1.,1.,
1.,1.,1.,1.,1.,1.,1.,1.,1.,1.,1.,1.,1.,1.,1.,1.,1.,1.,1.,1.,1.,1.,1.,1.,
1.,1.,1.,1.,1.,1.,1.,1.,1.,1.,1.,1.,1.,1.,1.,1.,1.,1.,1.,1.,1.,1.,1.,1.,
1.,1.,1.,1.,1.,1.,1.,1.,1.,1.,1.,1.,1.,1.,1.,1.,1.,1.,1.,1.,1.))
REPRESENTATION_ITEM('')
);
#807=(
BOUNDED_CURVE()
B_SPLINE_CURVE(5,(#224679,#224680,#224681,#224682,#224683,#224684,#224685,
#224686,#224687,#224688,#224689,#224690,#224691,#224692,#224693,#224694,
#224695,#224696,#224697,#224698,#224699,#224700,#224701,#224702,#224703,
#224704,#224705,#224706,#224707,#224708,#224709,#224710,#224711,#224712,
#224713,#224714,#224715,#224716,#224717,#224718,#224719,#224720,#224721,
#224722,#224723,#224724,#224725,#224726,#224727,#224728,#224729,#224730,
#224731,#224732,#224733,#224734,#224735,#224736,#224737,#224738,#224739,
#224740,#224741,#224742,#224743,#224744,#224745,#224746,#224747,#224748,
#224749,#224750,#224751,#224752,#224753,#224754,#224755,#224756,#224757,
#224758,#224759,#224760,#224761,#224762,#224763,#224764,#224765,#224766,
#224767,#224768,#224769,#224770,#224771,#224772,#224773,#224774,#224775,
#224776,#224777,#224778,#224779,#224780,#224781,#224782,#224783,#224784,
#224785,#224786,#224787,#224788,#224789,#224790,#224791,#224792,#224793,
#224794,#224795,#224796,#224797,#224798,#224799,#224800,#224801,#224802,
#224803,#224804,#224805,#224806,#224807,#224808,#224809,#224810,#224811,
#224812,#224813,#224814,#224815,#224816,#224817,#224818,#224819,#224820,
#224821,#224822,#224823,#224824,#224825,#224826,#224827,#224828,#224829,
#224830,#224831,#224832,#224833,#224834,#224835,#224836,#224837,#224838,
#224839,#224840,#224841,#224842,#224843,#224844,#224845,#224846,#224847,
#224848,#224849,#224850,#224851,#224852,#224853,#224854,#224855,#224856,
#224857,#224858,#224859,#224860,#224861,#224862,#224863,#224864,#224865,
#224866,#224867,#224868,#224869,#224870,#224871,#224872,#224873,#224874,
#224875,#224876,#224877,#224878,#224879,#224880,#224881,#224882,#224883),
 .UNSPECIFIED.,.F.,.F.)
B_SPLINE_CURVE_WITH_KNOTS((6,1,1,1,1,1,1,1,1,1,1,1,1,1,1,1,1,1,1,1,1,1,
1,1,1,1,1,1,1,1,1,1,1,1,1,1,1,1,1,1,1,1,1,1,1,1,1,1,1,1,1,1,1,1,1,1,1,1,
1,1,1,1,1,1,1,1,1,1,1,1,1,1,1,1,1,1,1,1,1,1,1,1,1,1,1,1,1,1,1,1,1,1,1,1,
1,1,1,1,1,1,1,1,1,1,1,1,1,1,1,1,1,1,1,1,1,1,1,1,1,1,1,1,1,1,1,1,1,1,1,1,
1,1,1,1,1,1,1,1,1,1,1,1,1,1,1,1,1,1,1,1,1,1,1,1,1,1,1,1,1,1,1,1,1,1,1,1,
1,1,1,1,1,1,1,1,1,1,1,1,1,1,1,1,1,1,1,1,1,1,1,1,1,1,1,1,1,1,1,1,1,1,6),
(-1.,-0.995000000000001,-0.990000000000001,-0.985000000000001,-0.980000000000001,
-0.975000000000001,-0.970000000000001,-0.965000000000001,-0.960000000000001,
-0.955000000000001,-0.950000000000001,-0.945000000000001,-0.940000000000001,
-0.935000000000001,-0.930000000000001,-0.925000000000001,-0.920000000000001,
-0.915000000000001,-0.910000000000001,-0.905000000000001,-0.900000000000001,
-0.895000000000001,-0.890000000000001,-0.885000000000001,-0.880000000000001,
-0.875000000000001,-0.870000000000001,-0.865000000000001,-0.860000000000001,
-0.855000000000001,-0.850000000000001,-0.845000000000001,-0.840000000000001,
-0.835000000000001,-0.830000000000001,-0.825000000000001,-0.820000000000001,
-0.815000000000001,-0.810000000000001,-0.805000000000001,-0.800000000000001,
-0.795000000000001,-0.790000000000001,-0.785000000000001,-0.780000000000001,
-0.775000000000001,-0.770000000000001,-0.765000000000001,-0.760000000000001,
-0.755000000000001,-0.750000000000001,-0.745000000000001,-0.740000000000001,
-0.735000000000001,-0.730000000000001,-0.725000000000001,-0.720000000000001,
-0.715000000000001,-0.710000000000001,-0.705000000000001,-0.700000000000001,
-0.695000000000001,-0.690000000000001,-0.685,-0.68,-0.675,-0.67,-0.665,
-0.66,-0.655,-0.65,-0.645,-0.64,-0.635,-0.63,-0.625,-0.62,-0.615,-0.61,
-0.605,-0.6,-0.595,-0.59,-0.585,-0.58,-0.575,-0.57,-0.565,-0.56,-0.555,
-0.55,-0.545,-0.54,-0.535,-0.53,-0.525,-0.52,-0.515,-0.51,-0.505,-0.5,-0.495,
-0.49,-0.485,-0.48,-0.475,-0.47,-0.465,-0.46,-0.455,-0.45,-0.445,-0.44,
-0.435,-0.43,-0.425,-0.42,-0.415,-0.41,-0.405,-0.4,-0.395,-0.39,-0.385,
-0.38,-0.375,-0.37,-0.365,-0.36,-0.355,-0.35,-0.345,-0.34,-0.335,-0.33,
-0.325,-0.32,-0.315,-0.31,-0.305,-0.3,-0.295,-0.29,-0.285,-0.28,-0.275,
-0.27,-0.265,-0.26,-0.255,-0.25,-0.245,-0.24,-0.235,-0.23,-0.225,-0.22,
-0.215,-0.21,-0.205,-0.2,-0.195,-0.19,-0.185,-0.18,-0.175,-0.17,-0.165,
-0.16,-0.155,-0.15,-0.145,-0.14,-0.135,-0.13,-0.125,-0.12,-0.115,-0.11,
-0.105,-0.1,-0.095,-0.09,-0.085,-0.08,-0.075,-0.07,-0.065,-0.06,-0.055,
-0.05,-0.045,-0.04,-0.035,-0.03,-0.025,-0.02,-0.015,-0.01,-0.005,0.),
 .UNSPECIFIED.)
CURVE()
GEOMETRIC_REPRESENTATION_ITEM()
RATIONAL_B_SPLINE_CURVE((1.,1.,1.,1.,1.,1.,1.,1.,1.,1.,1.,1.,1.,1.,1.,1.,
1.,1.,1.,1.,1.,1.,1.,1.,1.,1.,1.,1.,1.,1.,1.,1.,1.,1.,1.,1.,1.,1.,1.,1.,
1.,1.,1.,1.,1.,1.,1.,1.,1.,1.,1.,1.,1.,1.,1.,1.,1.,1.,1.,1.,1.,1.,1.,1.,
1.,1.,1.,1.,1.,1.,1.,1.,1.,1.,1.,1.,1.,1.,1.,1.,1.,1.,1.,1.,1.,1.,1.,1.,
1.,1.,1.,1.,1.,1.,1.,1.,1.,1.,1.,1.,1.,1.,1.,1.,1.,1.,1.,1.,1.,1.,1.,1.,
1.,1.,1.,1.,1.,1.,1.,1.,1.,1.,1.,1.,1.,1.,1.,1.,1.,1.,1.,1.,1.,1.,1.,1.,
1.,1.,1.,1.,1.,1.,1.,1.,1.,1.,1.,1.,1.,1.,1.,1.,1.,1.,1.,1.,1.,1.,1.,1.,
1.,1.,1.,1.,1.,1.,1.,1.,1.,1.,1.,1.,1.,1.,1.,1.,1.,1.,1.,1.,1.,1.,1.,1.,
1.,1.,1.,1.,1.,1.,1.,1.,1.,1.,1.,1.,1.,1.,1.,1.,1.,1.,1.,1.,1.))
REPRESENTATION_ITEM('')
);
#808=(
BOUNDED_CURVE()
B_SPLINE_CURVE(5,(#224886,#224887,#224888,#224889,#224890,#224891,#224892,
#224893,#224894,#224895,#224896,#224897,#224898,#224899,#224900,#224901,
#224902,#224903,#224904,#224905,#224906,#224907,#224908,#224909,#224910,
#224911,#224912,#224913,#224914,#224915,#224916,#224917,#224918,#224919,
#224920,#224921,#224922,#224923,#224924,#224925,#224926,#224927,#224928,
#224929,#224930,#224931,#224932,#224933,#224934,#224935,#224936,#224937,
#224938,#224939,#224940,#224941,#224942,#224943,#224944,#224945,#224946,
#224947,#224948,#224949,#224950,#224951,#224952,#224953,#224954,#224955,
#224956,#224957,#224958,#224959,#224960,#224961,#224962,#224963,#224964,
#224965,#224966,#224967,#224968,#224969,#224970,#224971,#224972,#224973,
#224974,#224975,#224976,#224977,#224978,#224979,#224980,#224981,#224982,
#224983,#224984,#224985,#224986,#224987,#224988,#224989,#224990,#224991,
#224992,#224993,#224994,#224995,#224996,#224997,#224998,#224999,#225000,
#225001,#225002,#225003,#225004,#225005,#225006,#225007,#225008,#225009,
#225010,#225011,#225012,#225013,#225014,#225015,#225016,#225017,#225018,
#225019,#225020,#225021,#225022,#225023,#225024,#225025,#225026,#225027,
#225028,#225029,#225030,#225031,#225032,#225033,#225034,#225035,#225036,
#225037,#225038,#225039,#225040,#225041,#225042,#225043,#225044,#225045,
#225046,#225047,#225048,#225049,#225050,#225051,#225052,#225053,#225054,
#225055,#225056,#225057,#225058,#225059,#225060,#225061,#225062,#225063,
#225064,#225065,#225066,#225067,#225068,#225069,#225070,#225071,#225072,
#225073,#225074,#225075,#225076,#225077,#225078,#225079,#225080,#225081,
#225082,#225083,#225084,#225085,#225086,#225087,#225088,#225089,#225090),
 .UNSPECIFIED.,.F.,.F.)
B_SPLINE_CURVE_WITH_KNOTS((6,1,1,1,1,1,1,1,1,1,1,1,1,1,1,1,1,1,1,1,1,1,
1,1,1,1,1,1,1,1,1,1,1,1,1,1,1,1,1,1,1,1,1,1,1,1,1,1,1,1,1,1,1,1,1,1,1,1,
1,1,1,1,1,1,1,1,1,1,1,1,1,1,1,1,1,1,1,1,1,1,1,1,1,1,1,1,1,1,1,1,1,1,1,1,
1,1,1,1,1,1,1,1,1,1,1,1,1,1,1,1,1,1,1,1,1,1,1,1,1,1,1,1,1,1,1,1,1,1,1,1,
1,1,1,1,1,1,1,1,1,1,1,1,1,1,1,1,1,1,1,1,1,1,1,1,1,1,1,1,1,1,1,1,1,1,1,1,
1,1,1,1,1,1,1,1,1,1,1,1,1,1,1,1,1,1,1,1,1,1,1,1,1,1,1,1,1,1,1,1,1,1,6),
(0.,0.005,0.01,0.015,0.02,0.025,0.03,0.035,0.04,0.045,0.05,0.055,0.06,0.065,
0.07,0.075,0.08,0.085,0.09,0.095,0.1,0.105,0.11,0.115,0.12,0.125,0.13,0.135,
0.14,0.145,0.15,0.155,0.16,0.165,0.17,0.175,0.18,0.185,0.19,0.195,0.2,0.205,
0.21,0.215,0.22,0.225,0.23,0.235,0.24,0.245,0.25,0.255,0.26,0.265,0.27,
0.275,0.28,0.285,0.29,0.295,0.3,0.305,0.31,0.315,0.32,0.325,0.33,0.335,
0.34,0.345,0.35,0.355,0.36,0.365,0.37,0.375,0.38,0.385,0.39,0.395,0.4,0.405,
0.41,0.415,0.42,0.425,0.43,0.435,0.44,0.445,0.45,0.455,0.46,0.465,0.47,
0.475,0.48,0.485,0.49,0.495,0.5,0.505,0.51,0.515,0.52,0.525,0.53,0.535,
0.54,0.545,0.55,0.555,0.56,0.565,0.57,0.575,0.58,0.585,0.59,0.595,0.6,0.605,
0.61,0.615,0.62,0.625,0.63,0.635,0.64,0.645,0.65,0.655,0.66,0.665,0.67,
0.675,0.68,0.685,0.690000000000001,0.695000000000001,0.700000000000001,
0.705000000000001,0.710000000000001,0.715000000000001,0.720000000000001,
0.725000000000001,0.730000000000001,0.735000000000001,0.740000000000001,
0.745000000000001,0.750000000000001,0.755000000000001,0.760000000000001,
0.765000000000001,0.770000000000001,0.775000000000001,0.780000000000001,
0.785000000000001,0.790000000000001,0.795000000000001,0.800000000000001,
0.805000000000001,0.810000000000001,0.815000000000001,0.820000000000001,
0.825000000000001,0.830000000000001,0.835000000000001,0.840000000000001,
0.845000000000001,0.850000000000001,0.855000000000001,0.860000000000001,
0.865000000000001,0.870000000000001,0.875000000000001,0.880000000000001,
0.885000000000001,0.890000000000001,0.895000000000001,0.900000000000001,
0.905000000000001,0.910000000000001,0.915000000000001,0.920000000000001,
0.925000000000001,0.930000000000001,0.935000000000001,0.940000000000001,
0.945000000000001,0.950000000000001,0.955000000000001,0.960000000000001,
0.965000000000001,0.970000000000001,0.975000000000001,0.980000000000001,
0.985000000000001,0.990000000000001,0.995000000000001,1.),.UNSPECIFIED.)
CURVE()
GEOMETRIC_REPRESENTATION_ITEM()
RATIONAL_B_SPLINE_CURVE((1.,1.,1.,1.,1.,1.,1.,1.,1.,1.,1.,1.,1.,1.,1.,1.,
1.,1.,1.,1.,1.,1.,1.,1.,1.,1.,1.,1.,1.,1.,1.,1.,1.,1.,1.,1.,1.,1.,1.,1.,
1.,1.,1.,1.,1.,1.,1.,1.,1.,1.,1.,1.,1.,1.,1.,1.,1.,1.,1.,1.,1.,1.,1.,1.,
1.,1.,1.,1.,1.,1.,1.,1.,1.,1.,1.,1.,1.,1.,1.,1.,1.,1.,1.,1.,1.,1.,1.,1.,
1.,1.,1.,1.,1.,1.,1.,1.,1.,1.,1.,1.,1.,1.,1.,1.,1.,1.,1.,1.,1.,1.,1.,1.,
1.,1.,1.,1.,1.,1.,1.,1.,1.,1.,1.,1.,1.,1.,1.,1.,1.,1.,1.,1.,1.,1.,1.,1.,
1.,1.,1.,1.,1.,1.,1.,1.,1.,1.,1.,1.,1.,1.,1.,1.,1.,1.,1.,1.,1.,1.,1.,1.,
1.,1.,1.,1.,1.,1.,1.,1.,1.,1.,1.,1.,1.,1.,1.,1.,1.,1.,1.,1.,1.,1.,1.,1.,
1.,1.,1.,1.,1.,1.,1.,1.,1.,1.,1.,1.,1.,1.,1.,1.,1.,1.,1.,1.,1.))
REPRESENTATION_ITEM('')
);
#809=(
BOUNDED_CURVE()
B_SPLINE_CURVE(5,(#225502,#225503,#225504,#225505,#225506,#225507,#225508,
#225509,#225510,#225511,#225512,#225513,#225514,#225515,#225516,#225517,
#225518,#225519,#225520,#225521,#225522,#225523,#225524,#225525,#225526,
#225527,#225528,#225529,#225530,#225531,#225532,#225533,#225534,#225535,
#225536,#225537,#225538,#225539,#225540,#225541,#225542,#225543,#225544,
#225545,#225546,#225547,#225548,#225549,#225550,#225551,#225552,#225553,
#225554,#225555,#225556,#225557,#225558,#225559,#225560,#225561,#225562,
#225563,#225564,#225565,#225566,#225567,#225568,#225569,#225570,#225571,
#225572,#225573,#225574,#225575,#225576,#225577,#225578,#225579,#225580,
#225581,#225582,#225583,#225584,#225585,#225586,#225587,#225588,#225589,
#225590,#225591,#225592,#225593,#225594,#225595,#225596,#225597,#225598,
#225599,#225600,#225601,#225602,#225603,#225604,#225605,#225606,#225607,
#225608,#225609,#225610,#225611,#225612,#225613,#225614,#225615,#225616,
#225617,#225618,#225619,#225620,#225621,#225622,#225623,#225624,#225625,
#225626,#225627,#225628,#225629,#225630,#225631,#225632,#225633,#225634,
#225635,#225636,#225637,#225638,#225639,#225640,#225641,#225642,#225643,
#225644,#225645,#225646,#225647,#225648,#225649,#225650,#225651,#225652,
#225653,#225654,#225655,#225656,#225657,#225658,#225659,#225660,#225661,
#225662,#225663,#225664,#225665,#225666,#225667,#225668,#225669,#225670,
#225671,#225672,#225673,#225674,#225675,#225676,#225677,#225678,#225679,
#225680,#225681,#225682,#225683,#225684,#225685,#225686,#225687,#225688,
#225689,#225690,#225691,#225692,#225693,#225694,#225695,#225696,#225697,
#225698,#225699,#225700,#225701,#225702,#225703,#225704,#225705,#225706),
 .UNSPECIFIED.,.F.,.F.)
B_SPLINE_CURVE_WITH_KNOTS((6,1,1,1,1,1,1,1,1,1,1,1,1,1,1,1,1,1,1,1,1,1,
1,1,1,1,1,1,1,1,1,1,1,1,1,1,1,1,1,1,1,1,1,1,1,1,1,1,1,1,1,1,1,1,1,1,1,1,
1,1,1,1,1,1,1,1,1,1,1,1,1,1,1,1,1,1,1,1,1,1,1,1,1,1,1,1,1,1,1,1,1,1,1,1,
1,1,1,1,1,1,1,1,1,1,1,1,1,1,1,1,1,1,1,1,1,1,1,1,1,1,1,1,1,1,1,1,1,1,1,1,
1,1,1,1,1,1,1,1,1,1,1,1,1,1,1,1,1,1,1,1,1,1,1,1,1,1,1,1,1,1,1,1,1,1,1,1,
1,1,1,1,1,1,1,1,1,1,1,1,1,1,1,1,1,1,1,1,1,1,1,1,1,1,1,1,1,1,1,1,1,1,6),
(0.,0.005,0.01,0.015,0.02,0.025,0.03,0.035,0.04,0.045,0.05,0.055,0.06,0.065,
0.07,0.075,0.08,0.085,0.09,0.095,0.1,0.105,0.11,0.115,0.12,0.125,0.13,0.135,
0.14,0.145,0.15,0.155,0.16,0.165,0.17,0.175,0.18,0.185,0.19,0.195,0.2,0.205,
0.21,0.215,0.22,0.225,0.23,0.235,0.24,0.245,0.25,0.255,0.26,0.265,0.27,
0.275,0.28,0.285,0.29,0.295,0.3,0.305,0.31,0.315,0.32,0.325,0.33,0.335,
0.34,0.345,0.35,0.355,0.36,0.365,0.37,0.375,0.38,0.385,0.39,0.395,0.4,0.405,
0.41,0.415,0.42,0.425,0.43,0.435,0.44,0.445,0.45,0.455,0.46,0.465,0.47,
0.475,0.48,0.485,0.49,0.495,0.5,0.505,0.51,0.515,0.52,0.525,0.53,0.535,
0.54,0.545,0.55,0.555,0.56,0.565,0.57,0.575,0.58,0.585,0.59,0.595,0.6,0.605,
0.61,0.615,0.62,0.625,0.63,0.635,0.64,0.645,0.65,0.655,0.66,0.665,0.67,
0.675,0.68,0.685,0.690000000000001,0.695000000000001,0.700000000000001,
0.705000000000001,0.710000000000001,0.715000000000001,0.720000000000001,
0.725000000000001,0.730000000000001,0.735000000000001,0.740000000000001,
0.745000000000001,0.750000000000001,0.755000000000001,0.760000000000001,
0.765000000000001,0.770000000000001,0.775000000000001,0.780000000000001,
0.785000000000001,0.790000000000001,0.795000000000001,0.800000000000001,
0.805000000000001,0.810000000000001,0.815000000000001,0.820000000000001,
0.825000000000001,0.830000000000001,0.835000000000001,0.840000000000001,
0.845000000000001,0.850000000000001,0.855000000000001,0.860000000000001,
0.865000000000001,0.870000000000001,0.875000000000001,0.880000000000001,
0.885000000000001,0.890000000000001,0.895000000000001,0.900000000000001,
0.905000000000001,0.910000000000001,0.915000000000001,0.920000000000001,
0.925000000000001,0.930000000000001,0.935000000000001,0.940000000000001,
0.945000000000001,0.950000000000001,0.955000000000001,0.960000000000001,
0.965000000000001,0.970000000000001,0.975000000000001,0.980000000000001,
0.985000000000001,0.990000000000001,0.995000000000001,1.),.UNSPECIFIED.)
CURVE()
GEOMETRIC_REPRESENTATION_ITEM()
RATIONAL_B_SPLINE_CURVE((1.,1.,1.,1.,1.,1.,1.,1.,1.,1.,1.,1.,1.,1.,1.,1.,
1.,1.,1.,1.,1.,1.,1.,1.,1.,1.,1.,1.,1.,1.,1.,1.,1.,1.,1.,1.,1.,1.,1.,1.,
1.,1.,1.,1.,1.,1.,1.,1.,1.,1.,1.,1.,1.,1.,1.,1.,1.,1.,1.,1.,1.,1.,1.,1.,
1.,1.,1.,1.,1.,1.,1.,1.,1.,1.,1.,1.,1.,1.,1.,1.,1.,1.,1.,1.,1.,1.,1.,1.,
1.,1.,1.,1.,1.,1.,1.,1.,1.,1.,1.,1.,1.,1.,1.,1.,1.,1.,1.,1.,1.,1.,1.,1.,
1.,1.,1.,1.,1.,1.,1.,1.,1.,1.,1.,1.,1.,1.,1.,1.,1.,1.,1.,1.,1.,1.,1.,1.,
1.,1.,1.,1.,1.,1.,1.,1.,1.,1.,1.,1.,1.,1.,1.,1.,1.,1.,1.,1.,1.,1.,1.,1.,
1.,1.,1.,1.,1.,1.,1.,1.,1.,1.,1.,1.,1.,1.,1.,1.,1.,1.,1.,1.,1.,1.,1.,1.,
1.,1.,1.,1.,1.,1.,1.,1.,1.,1.,1.,1.,1.,1.,1.,1.,1.,1.,1.,1.,1.))
REPRESENTATION_ITEM('')
);
#810=(
BOUNDED_CURVE()
B_SPLINE_CURVE(5,(#225708,#225709,#225710,#225711,#225712,#225713,#225714,
#225715,#225716,#225717,#225718,#225719,#225720,#225721,#225722,#225723,
#225724,#225725,#225726,#225727,#225728,#225729,#225730,#225731,#225732,
#225733,#225734,#225735,#225736,#225737,#225738,#225739,#225740,#225741,
#225742,#225743,#225744,#225745,#225746,#225747,#225748,#225749,#225750,
#225751,#225752,#225753,#225754,#225755,#225756,#225757,#225758,#225759,
#225760,#225761,#225762,#225763,#225764,#225765,#225766,#225767,#225768,
#225769,#225770,#225771,#225772,#225773,#225774,#225775,#225776,#225777,
#225778,#225779,#225780,#225781,#225782,#225783,#225784,#225785,#225786,
#225787,#225788,#225789,#225790,#225791,#225792,#225793,#225794,#225795,
#225796,#225797,#225798,#225799,#225800,#225801,#225802,#225803,#225804,
#225805,#225806,#225807,#225808,#225809,#225810,#225811,#225812,#225813,
#225814,#225815,#225816,#225817,#225818,#225819,#225820,#225821,#225822,
#225823,#225824,#225825,#225826,#225827,#225828,#225829,#225830,#225831,
#225832,#225833,#225834,#225835,#225836,#225837,#225838,#225839,#225840,
#225841,#225842,#225843,#225844,#225845,#225846,#225847,#225848,#225849,
#225850,#225851,#225852,#225853,#225854,#225855,#225856,#225857,#225858,
#225859,#225860,#225861,#225862,#225863,#225864,#225865,#225866,#225867,
#225868,#225869,#225870,#225871,#225872,#225873,#225874,#225875,#225876,
#225877,#225878,#225879,#225880,#225881,#225882,#225883,#225884,#225885,
#225886,#225887,#225888,#225889,#225890,#225891,#225892,#225893,#225894,
#225895,#225896,#225897,#225898,#225899,#225900,#225901,#225902,#225903,
#225904,#225905,#225906,#225907,#225908,#225909,#225910,#225911,#225912),
 .UNSPECIFIED.,.F.,.F.)
B_SPLINE_CURVE_WITH_KNOTS((6,1,1,1,1,1,1,1,1,1,1,1,1,1,1,1,1,1,1,1,1,1,
1,1,1,1,1,1,1,1,1,1,1,1,1,1,1,1,1,1,1,1,1,1,1,1,1,1,1,1,1,1,1,1,1,1,1,1,
1,1,1,1,1,1,1,1,1,1,1,1,1,1,1,1,1,1,1,1,1,1,1,1,1,1,1,1,1,1,1,1,1,1,1,1,
1,1,1,1,1,1,1,1,1,1,1,1,1,1,1,1,1,1,1,1,1,1,1,1,1,1,1,1,1,1,1,1,1,1,1,1,
1,1,1,1,1,1,1,1,1,1,1,1,1,1,1,1,1,1,1,1,1,1,1,1,1,1,1,1,1,1,1,1,1,1,1,1,
1,1,1,1,1,1,1,1,1,1,1,1,1,1,1,1,1,1,1,1,1,1,1,1,1,1,1,1,1,1,1,1,1,1,6),
(-1.,-0.995000000000001,-0.990000000000001,-0.985000000000001,-0.980000000000001,
-0.975000000000001,-0.970000000000001,-0.965000000000001,-0.960000000000001,
-0.955000000000001,-0.950000000000001,-0.945000000000001,-0.940000000000001,
-0.935000000000001,-0.930000000000001,-0.925000000000001,-0.920000000000001,
-0.915000000000001,-0.910000000000001,-0.905000000000001,-0.900000000000001,
-0.895000000000001,-0.890000000000001,-0.885000000000001,-0.880000000000001,
-0.875000000000001,-0.870000000000001,-0.865000000000001,-0.860000000000001,
-0.855000000000001,-0.850000000000001,-0.845000000000001,-0.840000000000001,
-0.835000000000001,-0.830000000000001,-0.825000000000001,-0.820000000000001,
-0.815000000000001,-0.810000000000001,-0.805000000000001,-0.800000000000001,
-0.795000000000001,-0.790000000000001,-0.785000000000001,-0.780000000000001,
-0.775000000000001,-0.770000000000001,-0.765000000000001,-0.760000000000001,
-0.755000000000001,-0.750000000000001,-0.745000000000001,-0.740000000000001,
-0.735000000000001,-0.730000000000001,-0.725000000000001,-0.720000000000001,
-0.715000000000001,-0.710000000000001,-0.705000000000001,-0.700000000000001,
-0.695000000000001,-0.690000000000001,-0.685,-0.68,-0.675,-0.67,-0.665,
-0.66,-0.655,-0.65,-0.645,-0.64,-0.635,-0.63,-0.625,-0.62,-0.615,-0.61,
-0.605,-0.6,-0.595,-0.59,-0.585,-0.58,-0.575,-0.57,-0.565,-0.56,-0.555,
-0.55,-0.545,-0.54,-0.535,-0.53,-0.525,-0.52,-0.515,-0.51,-0.505,-0.5,-0.495,
-0.49,-0.485,-0.48,-0.475,-0.47,-0.465,-0.46,-0.455,-0.45,-0.445,-0.44,
-0.435,-0.43,-0.425,-0.42,-0.415,-0.41,-0.405,-0.4,-0.395,-0.39,-0.385,
-0.38,-0.375,-0.37,-0.365,-0.36,-0.355,-0.35,-0.345,-0.34,-0.335,-0.33,
-0.325,-0.32,-0.315,-0.31,-0.305,-0.3,-0.295,-0.29,-0.285,-0.28,-0.275,
-0.27,-0.265,-0.26,-0.255,-0.25,-0.245,-0.24,-0.235,-0.23,-0.225,-0.22,
-0.215,-0.21,-0.205,-0.2,-0.195,-0.19,-0.185,-0.18,-0.175,-0.17,-0.165,
-0.16,-0.155,-0.15,-0.145,-0.14,-0.135,-0.13,-0.125,-0.12,-0.115,-0.11,
-0.105,-0.1,-0.095,-0.09,-0.085,-0.08,-0.075,-0.07,-0.065,-0.06,-0.055,
-0.05,-0.045,-0.04,-0.035,-0.03,-0.025,-0.02,-0.015,-0.01,-0.005,0.),
 .UNSPECIFIED.)
CURVE()
GEOMETRIC_REPRESENTATION_ITEM()
RATIONAL_B_SPLINE_CURVE((1.,1.,1.,1.,1.,1.,1.,1.,1.,1.,1.,1.,1.,1.,1.,1.,
1.,1.,1.,1.,1.,1.,1.,1.,1.,1.,1.,1.,1.,1.,1.,1.,1.,1.,1.,1.,1.,1.,1.,1.,
1.,1.,1.,1.,1.,1.,1.,1.,1.,1.,1.,1.,1.,1.,1.,1.,1.,1.,1.,1.,1.,1.,1.,1.,
1.,1.,1.,1.,1.,1.,1.,1.,1.,1.,1.,1.,1.,1.,1.,1.,1.,1.,1.,1.,1.,1.,1.,1.,
1.,1.,1.,1.,1.,1.,1.,1.,1.,1.,1.,1.,1.,1.,1.,1.,1.,1.,1.,1.,1.,1.,1.,1.,
1.,1.,1.,1.,1.,1.,1.,1.,1.,1.,1.,1.,1.,1.,1.,1.,1.,1.,1.,1.,1.,1.,1.,1.,
1.,1.,1.,1.,1.,1.,1.,1.,1.,1.,1.,1.,1.,1.,1.,1.,1.,1.,1.,1.,1.,1.,1.,1.,
1.,1.,1.,1.,1.,1.,1.,1.,1.,1.,1.,1.,1.,1.,1.,1.,1.,1.,1.,1.,1.,1.,1.,1.,
1.,1.,1.,1.,1.,1.,1.,1.,1.,1.,1.,1.,1.,1.,1.,1.,1.,1.,1.,1.,1.))
REPRESENTATION_ITEM('')
);
#811=(
BOUNDED_CURVE()
B_SPLINE_CURVE(5,(#226331,#226332,#226333,#226334,#226335,#226336,#226337,
#226338,#226339,#226340,#226341,#226342,#226343,#226344,#226345,#226346,
#226347,#226348,#226349,#226350,#226351,#226352,#226353,#226354,#226355,
#226356,#226357,#226358,#226359,#226360,#226361,#226362,#226363,#226364,
#226365,#226366,#226367,#226368,#226369,#226370,#226371,#226372,#226373,
#226374,#226375,#226376,#226377,#226378,#226379,#226380,#226381,#226382,
#226383,#226384,#226385,#226386,#226387,#226388,#226389,#226390,#226391,
#226392,#226393,#226394,#226395,#226396,#226397,#226398,#226399,#226400,
#226401,#226402,#226403,#226404,#226405,#226406,#226407,#226408,#226409,
#226410,#226411,#226412,#226413,#226414,#226415,#226416,#226417,#226418,
#226419,#226420,#226421,#226422,#226423,#226424,#226425,#226426,#226427,
#226428,#226429,#226430,#226431,#226432,#226433,#226434,#226435,#226436,
#226437,#226438,#226439,#226440,#226441,#226442,#226443,#226444,#226445,
#226446,#226447,#226448,#226449,#226450,#226451,#226452,#226453,#226454,
#226455,#226456,#226457,#226458,#226459,#226460,#226461,#226462,#226463,
#226464,#226465,#226466,#226467,#226468,#226469,#226470,#226471,#226472,
#226473,#226474,#226475,#226476,#226477,#226478,#226479,#226480,#226481,
#226482,#226483,#226484,#226485,#226486,#226487,#226488,#226489,#226490,
#226491,#226492,#226493,#226494,#226495,#226496,#226497,#226498,#226499,
#226500,#226501,#226502,#226503,#226504,#226505,#226506,#226507,#226508,
#226509,#226510,#226511,#226512,#226513,#226514,#226515,#226516,#226517,
#226518,#226519,#226520,#226521,#226522,#226523,#226524,#226525,#226526,
#226527,#226528,#226529,#226530,#226531,#226532,#226533,#226534,#226535),
 .UNSPECIFIED.,.F.,.F.)
B_SPLINE_CURVE_WITH_KNOTS((6,1,1,1,1,1,1,1,1,1,1,1,1,1,1,1,1,1,1,1,1,1,
1,1,1,1,1,1,1,1,1,1,1,1,1,1,1,1,1,1,1,1,1,1,1,1,1,1,1,1,1,1,1,1,1,1,1,1,
1,1,1,1,1,1,1,1,1,1,1,1,1,1,1,1,1,1,1,1,1,1,1,1,1,1,1,1,1,1,1,1,1,1,1,1,
1,1,1,1,1,1,1,1,1,1,1,1,1,1,1,1,1,1,1,1,1,1,1,1,1,1,1,1,1,1,1,1,1,1,1,1,
1,1,1,1,1,1,1,1,1,1,1,1,1,1,1,1,1,1,1,1,1,1,1,1,1,1,1,1,1,1,1,1,1,1,1,1,
1,1,1,1,1,1,1,1,1,1,1,1,1,1,1,1,1,1,1,1,1,1,1,1,1,1,1,1,1,1,1,1,1,1,6),
(-1.,-0.995000000000001,-0.990000000000001,-0.985000000000001,-0.980000000000001,
-0.975000000000001,-0.970000000000001,-0.965000000000001,-0.960000000000001,
-0.955000000000001,-0.950000000000001,-0.945000000000001,-0.940000000000001,
-0.935000000000001,-0.930000000000001,-0.925000000000001,-0.920000000000001,
-0.915000000000001,-0.910000000000001,-0.905000000000001,-0.900000000000001,
-0.895000000000001,-0.890000000000001,-0.885000000000001,-0.880000000000001,
-0.875000000000001,-0.870000000000001,-0.865000000000001,-0.860000000000001,
-0.855000000000001,-0.850000000000001,-0.845000000000001,-0.840000000000001,
-0.835000000000001,-0.830000000000001,-0.825000000000001,-0.820000000000001,
-0.815000000000001,-0.810000000000001,-0.805000000000001,-0.800000000000001,
-0.795000000000001,-0.790000000000001,-0.785000000000001,-0.780000000000001,
-0.775000000000001,-0.770000000000001,-0.765000000000001,-0.760000000000001,
-0.755000000000001,-0.750000000000001,-0.745000000000001,-0.740000000000001,
-0.735000000000001,-0.730000000000001,-0.725000000000001,-0.720000000000001,
-0.715000000000001,-0.710000000000001,-0.705000000000001,-0.700000000000001,
-0.695000000000001,-0.690000000000001,-0.685,-0.68,-0.675,-0.67,-0.665,
-0.66,-0.655,-0.65,-0.645,-0.64,-0.635,-0.63,-0.625,-0.62,-0.615,-0.61,
-0.605,-0.6,-0.595,-0.59,-0.585,-0.58,-0.575,-0.57,-0.565,-0.56,-0.555,
-0.55,-0.545,-0.54,-0.535,-0.53,-0.525,-0.52,-0.515,-0.51,-0.505,-0.5,-0.495,
-0.49,-0.485,-0.48,-0.475,-0.47,-0.465,-0.46,-0.455,-0.45,-0.445,-0.44,
-0.435,-0.43,-0.425,-0.42,-0.415,-0.41,-0.405,-0.4,-0.395,-0.39,-0.385,
-0.38,-0.375,-0.37,-0.365,-0.36,-0.355,-0.35,-0.345,-0.34,-0.335,-0.33,
-0.325,-0.32,-0.315,-0.31,-0.305,-0.3,-0.295,-0.29,-0.285,-0.28,-0.275,
-0.27,-0.265,-0.26,-0.255,-0.25,-0.245,-0.24,-0.235,-0.23,-0.225,-0.22,
-0.215,-0.21,-0.205,-0.2,-0.195,-0.19,-0.185,-0.18,-0.175,-0.17,-0.165,
-0.16,-0.155,-0.15,-0.145,-0.14,-0.135,-0.13,-0.125,-0.12,-0.115,-0.11,
-0.105,-0.1,-0.095,-0.09,-0.085,-0.08,-0.075,-0.07,-0.065,-0.06,-0.055,
-0.05,-0.045,-0.04,-0.035,-0.03,-0.025,-0.02,-0.015,-0.01,-0.005,0.),
 .UNSPECIFIED.)
CURVE()
GEOMETRIC_REPRESENTATION_ITEM()
RATIONAL_B_SPLINE_CURVE((1.,1.,1.,1.,1.,1.,1.,1.,1.,1.,1.,1.,1.,1.,1.,1.,
1.,1.,1.,1.,1.,1.,1.,1.,1.,1.,1.,1.,1.,1.,1.,1.,1.,1.,1.,1.,1.,1.,1.,1.,
1.,1.,1.,1.,1.,1.,1.,1.,1.,1.,1.,1.,1.,1.,1.,1.,1.,1.,1.,1.,1.,1.,1.,1.,
1.,1.,1.,1.,1.,1.,1.,1.,1.,1.,1.,1.,1.,1.,1.,1.,1.,1.,1.,1.,1.,1.,1.,1.,
1.,1.,1.,1.,1.,1.,1.,1.,1.,1.,1.,1.,1.,1.,1.,1.,1.,1.,1.,1.,1.,1.,1.,1.,
1.,1.,1.,1.,1.,1.,1.,1.,1.,1.,1.,1.,1.,1.,1.,1.,1.,1.,1.,1.,1.,1.,1.,1.,
1.,1.,1.,1.,1.,1.,1.,1.,1.,1.,1.,1.,1.,1.,1.,1.,1.,1.,1.,1.,1.,1.,1.,1.,
1.,1.,1.,1.,1.,1.,1.,1.,1.,1.,1.,1.,1.,1.,1.,1.,1.,1.,1.,1.,1.,1.,1.,1.,
1.,1.,1.,1.,1.,1.,1.,1.,1.,1.,1.,1.,1.,1.,1.,1.,1.,1.,1.,1.,1.))
REPRESENTATION_ITEM('')
);
#812=(
BOUNDED_CURVE()
B_SPLINE_CURVE(5,(#226538,#226539,#226540,#226541,#226542,#226543,#226544,
#226545,#226546,#226547,#226548,#226549,#226550,#226551,#226552,#226553,
#226554,#226555,#226556,#226557,#226558,#226559,#226560,#226561,#226562,
#226563,#226564,#226565,#226566,#226567,#226568,#226569,#226570,#226571,
#226572,#226573,#226574,#226575,#226576,#226577,#226578,#226579,#226580,
#226581,#226582,#226583,#226584,#226585,#226586,#226587,#226588,#226589,
#226590,#226591,#226592,#226593,#226594,#226595,#226596,#226597,#226598,
#226599,#226600,#226601,#226602,#226603,#226604,#226605,#226606,#226607,
#226608,#226609,#226610,#226611,#226612,#226613,#226614,#226615,#226616,
#226617,#226618,#226619,#226620,#226621,#226622,#226623,#226624,#226625,
#226626,#226627,#226628,#226629,#226630,#226631,#226632,#226633,#226634,
#226635,#226636,#226637,#226638,#226639,#226640,#226641,#226642,#226643,
#226644,#226645,#226646,#226647,#226648,#226649,#226650,#226651,#226652,
#226653,#226654,#226655,#226656,#226657,#226658,#226659,#226660,#226661,
#226662,#226663,#226664,#226665,#226666,#226667,#226668,#226669,#226670,
#226671,#226672,#226673,#226674,#226675,#226676,#226677,#226678,#226679,
#226680,#226681,#226682,#226683,#226684,#226685,#226686,#226687,#226688,
#226689,#226690,#226691,#226692,#226693,#226694,#226695,#226696,#226697,
#226698,#226699,#226700,#226701,#226702,#226703,#226704,#226705,#226706,
#226707,#226708,#226709,#226710,#226711,#226712,#226713,#226714,#226715,
#226716,#226717,#226718,#226719,#226720,#226721,#226722,#226723,#226724,
#226725,#226726,#226727,#226728,#226729,#226730,#226731,#226732,#226733,
#226734,#226735,#226736,#226737,#226738,#226739,#226740,#226741,#226742),
 .UNSPECIFIED.,.F.,.F.)
B_SPLINE_CURVE_WITH_KNOTS((6,1,1,1,1,1,1,1,1,1,1,1,1,1,1,1,1,1,1,1,1,1,
1,1,1,1,1,1,1,1,1,1,1,1,1,1,1,1,1,1,1,1,1,1,1,1,1,1,1,1,1,1,1,1,1,1,1,1,
1,1,1,1,1,1,1,1,1,1,1,1,1,1,1,1,1,1,1,1,1,1,1,1,1,1,1,1,1,1,1,1,1,1,1,1,
1,1,1,1,1,1,1,1,1,1,1,1,1,1,1,1,1,1,1,1,1,1,1,1,1,1,1,1,1,1,1,1,1,1,1,1,
1,1,1,1,1,1,1,1,1,1,1,1,1,1,1,1,1,1,1,1,1,1,1,1,1,1,1,1,1,1,1,1,1,1,1,1,
1,1,1,1,1,1,1,1,1,1,1,1,1,1,1,1,1,1,1,1,1,1,1,1,1,1,1,1,1,1,1,1,1,1,6),
(0.,0.005,0.01,0.015,0.02,0.025,0.03,0.035,0.04,0.045,0.05,0.055,0.06,0.065,
0.07,0.075,0.08,0.085,0.09,0.095,0.1,0.105,0.11,0.115,0.12,0.125,0.13,0.135,
0.14,0.145,0.15,0.155,0.16,0.165,0.17,0.175,0.18,0.185,0.19,0.195,0.2,0.205,
0.21,0.215,0.22,0.225,0.23,0.235,0.24,0.245,0.25,0.255,0.26,0.265,0.27,
0.275,0.28,0.285,0.29,0.295,0.3,0.305,0.31,0.315,0.32,0.325,0.33,0.335,
0.34,0.345,0.35,0.355,0.36,0.365,0.37,0.375,0.38,0.385,0.39,0.395,0.4,0.405,
0.41,0.415,0.42,0.425,0.43,0.435,0.44,0.445,0.45,0.455,0.46,0.465,0.47,
0.475,0.48,0.485,0.49,0.495,0.5,0.505,0.51,0.515,0.52,0.525,0.53,0.535,
0.54,0.545,0.55,0.555,0.56,0.565,0.57,0.575,0.58,0.585,0.59,0.595,0.6,0.605,
0.61,0.615,0.62,0.625,0.63,0.635,0.64,0.645,0.65,0.655,0.66,0.665,0.67,
0.675,0.68,0.685,0.690000000000001,0.695000000000001,0.700000000000001,
0.705000000000001,0.710000000000001,0.715000000000001,0.720000000000001,
0.725000000000001,0.730000000000001,0.735000000000001,0.740000000000001,
0.745000000000001,0.750000000000001,0.755000000000001,0.760000000000001,
0.765000000000001,0.770000000000001,0.775000000000001,0.780000000000001,
0.785000000000001,0.790000000000001,0.795000000000001,0.800000000000001,
0.805000000000001,0.810000000000001,0.815000000000001,0.820000000000001,
0.825000000000001,0.830000000000001,0.835000000000001,0.840000000000001,
0.845000000000001,0.850000000000001,0.855000000000001,0.860000000000001,
0.865000000000001,0.870000000000001,0.875000000000001,0.880000000000001,
0.885000000000001,0.890000000000001,0.895000000000001,0.900000000000001,
0.905000000000001,0.910000000000001,0.915000000000001,0.920000000000001,
0.925000000000001,0.930000000000001,0.935000000000001,0.940000000000001,
0.945000000000001,0.950000000000001,0.955000000000001,0.960000000000001,
0.965000000000001,0.970000000000001,0.975000000000001,0.980000000000001,
0.985000000000001,0.990000000000001,0.995000000000001,1.),.UNSPECIFIED.)
CURVE()
GEOMETRIC_REPRESENTATION_ITEM()
RATIONAL_B_SPLINE_CURVE((1.,1.,1.,1.,1.,1.,1.,1.,1.,1.,1.,1.,1.,1.,1.,1.,
1.,1.,1.,1.,1.,1.,1.,1.,1.,1.,1.,1.,1.,1.,1.,1.,1.,1.,1.,1.,1.,1.,1.,1.,
1.,1.,1.,1.,1.,1.,1.,1.,1.,1.,1.,1.,1.,1.,1.,1.,1.,1.,1.,1.,1.,1.,1.,1.,
1.,1.,1.,1.,1.,1.,1.,1.,1.,1.,1.,1.,1.,1.,1.,1.,1.,1.,1.,1.,1.,1.,1.,1.,
1.,1.,1.,1.,1.,1.,1.,1.,1.,1.,1.,1.,1.,1.,1.,1.,1.,1.,1.,1.,1.,1.,1.,1.,
1.,1.,1.,1.,1.,1.,1.,1.,1.,1.,1.,1.,1.,1.,1.,1.,1.,1.,1.,1.,1.,1.,1.,1.,
1.,1.,1.,1.,1.,1.,1.,1.,1.,1.,1.,1.,1.,1.,1.,1.,1.,1.,1.,1.,1.,1.,1.,1.,
1.,1.,1.,1.,1.,1.,1.,1.,1.,1.,1.,1.,1.,1.,1.,1.,1.,1.,1.,1.,1.,1.,1.,1.,
1.,1.,1.,1.,1.,1.,1.,1.,1.,1.,1.,1.,1.,1.,1.,1.,1.,1.,1.,1.,1.))
REPRESENTATION_ITEM('')
);
#813=(
BOUNDED_CURVE()
B_SPLINE_CURVE(5,(#227154,#227155,#227156,#227157,#227158,#227159,#227160,
#227161,#227162,#227163,#227164,#227165,#227166,#227167,#227168,#227169,
#227170,#227171,#227172,#227173,#227174,#227175,#227176,#227177,#227178,
#227179,#227180,#227181,#227182,#227183,#227184,#227185,#227186,#227187,
#227188,#227189,#227190,#227191,#227192,#227193,#227194,#227195,#227196,
#227197,#227198,#227199,#227200,#227201,#227202,#227203,#227204,#227205,
#227206,#227207,#227208,#227209,#227210,#227211,#227212,#227213,#227214,
#227215,#227216,#227217,#227218,#227219,#227220,#227221,#227222,#227223,
#227224,#227225,#227226,#227227,#227228,#227229,#227230,#227231,#227232,
#227233,#227234,#227235,#227236,#227237,#227238,#227239,#227240,#227241,
#227242,#227243,#227244,#227245,#227246,#227247,#227248,#227249,#227250,
#227251,#227252,#227253,#227254,#227255,#227256,#227257,#227258,#227259,
#227260,#227261,#227262,#227263,#227264,#227265,#227266,#227267,#227268,
#227269,#227270,#227271,#227272,#227273,#227274,#227275,#227276,#227277,
#227278,#227279,#227280,#227281,#227282,#227283,#227284,#227285,#227286,
#227287,#227288,#227289,#227290,#227291,#227292,#227293,#227294,#227295,
#227296,#227297,#227298,#227299,#227300,#227301,#227302,#227303,#227304,
#227305,#227306,#227307,#227308,#227309,#227310,#227311,#227312,#227313,
#227314,#227315,#227316,#227317,#227318,#227319,#227320,#227321,#227322,
#227323,#227324,#227325,#227326,#227327,#227328,#227329,#227330,#227331,
#227332,#227333,#227334,#227335,#227336,#227337,#227338,#227339,#227340,
#227341,#227342,#227343,#227344,#227345,#227346,#227347,#227348,#227349,
#227350,#227351,#227352,#227353,#227354,#227355,#227356,#227357,#227358),
 .UNSPECIFIED.,.F.,.F.)
B_SPLINE_CURVE_WITH_KNOTS((6,1,1,1,1,1,1,1,1,1,1,1,1,1,1,1,1,1,1,1,1,1,
1,1,1,1,1,1,1,1,1,1,1,1,1,1,1,1,1,1,1,1,1,1,1,1,1,1,1,1,1,1,1,1,1,1,1,1,
1,1,1,1,1,1,1,1,1,1,1,1,1,1,1,1,1,1,1,1,1,1,1,1,1,1,1,1,1,1,1,1,1,1,1,1,
1,1,1,1,1,1,1,1,1,1,1,1,1,1,1,1,1,1,1,1,1,1,1,1,1,1,1,1,1,1,1,1,1,1,1,1,
1,1,1,1,1,1,1,1,1,1,1,1,1,1,1,1,1,1,1,1,1,1,1,1,1,1,1,1,1,1,1,1,1,1,1,1,
1,1,1,1,1,1,1,1,1,1,1,1,1,1,1,1,1,1,1,1,1,1,1,1,1,1,1,1,1,1,1,1,1,1,6),
(0.,0.005,0.01,0.015,0.02,0.025,0.03,0.035,0.04,0.045,0.05,0.055,0.06,0.065,
0.07,0.075,0.08,0.085,0.09,0.095,0.1,0.105,0.11,0.115,0.12,0.125,0.13,0.135,
0.14,0.145,0.15,0.155,0.16,0.165,0.17,0.175,0.18,0.185,0.19,0.195,0.2,0.205,
0.21,0.215,0.22,0.225,0.23,0.235,0.24,0.245,0.25,0.255,0.26,0.265,0.27,
0.275,0.28,0.285,0.29,0.295,0.3,0.305,0.31,0.315,0.32,0.325,0.33,0.335,
0.34,0.345,0.35,0.355,0.36,0.365,0.37,0.375,0.38,0.385,0.39,0.395,0.4,0.405,
0.41,0.415,0.42,0.425,0.43,0.435,0.44,0.445,0.45,0.455,0.46,0.465,0.47,
0.475,0.48,0.485,0.49,0.495,0.5,0.505,0.51,0.515,0.52,0.525,0.53,0.535,
0.54,0.545,0.55,0.555,0.56,0.565,0.57,0.575,0.58,0.585,0.59,0.595,0.6,0.605,
0.61,0.615,0.62,0.625,0.63,0.635,0.64,0.645,0.65,0.655,0.66,0.665,0.67,
0.675,0.68,0.685,0.690000000000001,0.695000000000001,0.700000000000001,
0.705000000000001,0.710000000000001,0.715000000000001,0.720000000000001,
0.725000000000001,0.730000000000001,0.735000000000001,0.740000000000001,
0.745000000000001,0.750000000000001,0.755000000000001,0.760000000000001,
0.765000000000001,0.770000000000001,0.775000000000001,0.780000000000001,
0.785000000000001,0.790000000000001,0.795000000000001,0.800000000000001,
0.805000000000001,0.810000000000001,0.815000000000001,0.820000000000001,
0.825000000000001,0.830000000000001,0.835000000000001,0.840000000000001,
0.845000000000001,0.850000000000001,0.855000000000001,0.860000000000001,
0.865000000000001,0.870000000000001,0.875000000000001,0.880000000000001,
0.885000000000001,0.890000000000001,0.895000000000001,0.900000000000001,
0.905000000000001,0.910000000000001,0.915000000000001,0.920000000000001,
0.925000000000001,0.930000000000001,0.935000000000001,0.940000000000001,
0.945000000000001,0.950000000000001,0.955000000000001,0.960000000000001,
0.965000000000001,0.970000000000001,0.975000000000001,0.980000000000001,
0.985000000000001,0.990000000000001,0.995000000000001,1.),.UNSPECIFIED.)
CURVE()
GEOMETRIC_REPRESENTATION_ITEM()
RATIONAL_B_SPLINE_CURVE((1.,1.,1.,1.,1.,1.,1.,1.,1.,1.,1.,1.,1.,1.,1.,1.,
1.,1.,1.,1.,1.,1.,1.,1.,1.,1.,1.,1.,1.,1.,1.,1.,1.,1.,1.,1.,1.,1.,1.,1.,
1.,1.,1.,1.,1.,1.,1.,1.,1.,1.,1.,1.,1.,1.,1.,1.,1.,1.,1.,1.,1.,1.,1.,1.,
1.,1.,1.,1.,1.,1.,1.,1.,1.,1.,1.,1.,1.,1.,1.,1.,1.,1.,1.,1.,1.,1.,1.,1.,
1.,1.,1.,1.,1.,1.,1.,1.,1.,1.,1.,1.,1.,1.,1.,1.,1.,1.,1.,1.,1.,1.,1.,1.,
1.,1.,1.,1.,1.,1.,1.,1.,1.,1.,1.,1.,1.,1.,1.,1.,1.,1.,1.,1.,1.,1.,1.,1.,
1.,1.,1.,1.,1.,1.,1.,1.,1.,1.,1.,1.,1.,1.,1.,1.,1.,1.,1.,1.,1.,1.,1.,1.,
1.,1.,1.,1.,1.,1.,1.,1.,1.,1.,1.,1.,1.,1.,1.,1.,1.,1.,1.,1.,1.,1.,1.,1.,
1.,1.,1.,1.,1.,1.,1.,1.,1.,1.,1.,1.,1.,1.,1.,1.,1.,1.,1.,1.,1.))
REPRESENTATION_ITEM('')
);
#814=(
BOUNDED_CURVE()
B_SPLINE_CURVE(5,(#227360,#227361,#227362,#227363,#227364,#227365,#227366,
#227367,#227368,#227369,#227370,#227371,#227372,#227373,#227374,#227375,
#227376,#227377,#227378,#227379,#227380,#227381,#227382,#227383,#227384,
#227385,#227386,#227387,#227388,#227389,#227390,#227391,#227392,#227393,
#227394,#227395,#227396,#227397,#227398,#227399,#227400,#227401,#227402,
#227403,#227404,#227405,#227406,#227407,#227408,#227409,#227410,#227411,
#227412,#227413,#227414,#227415,#227416,#227417,#227418,#227419,#227420,
#227421,#227422,#227423,#227424,#227425,#227426,#227427,#227428,#227429,
#227430,#227431,#227432,#227433,#227434,#227435,#227436,#227437,#227438,
#227439,#227440,#227441,#227442,#227443,#227444,#227445,#227446,#227447,
#227448,#227449,#227450,#227451,#227452,#227453,#227454,#227455,#227456,
#227457,#227458,#227459,#227460,#227461,#227462,#227463,#227464,#227465,
#227466,#227467,#227468,#227469,#227470,#227471,#227472,#227473,#227474,
#227475,#227476,#227477,#227478,#227479,#227480,#227481,#227482,#227483,
#227484,#227485,#227486,#227487,#227488,#227489,#227490,#227491,#227492,
#227493,#227494,#227495,#227496,#227497,#227498,#227499,#227500,#227501,
#227502,#227503,#227504,#227505,#227506,#227507,#227508,#227509,#227510,
#227511,#227512,#227513,#227514,#227515,#227516,#227517,#227518,#227519,
#227520,#227521,#227522,#227523,#227524,#227525,#227526,#227527,#227528,
#227529,#227530,#227531,#227532,#227533,#227534,#227535,#227536,#227537,
#227538,#227539,#227540,#227541,#227542,#227543,#227544,#227545,#227546,
#227547,#227548,#227549,#227550,#227551,#227552,#227553,#227554,#227555,
#227556,#227557,#227558,#227559,#227560,#227561,#227562,#227563,#227564),
 .UNSPECIFIED.,.F.,.F.)
B_SPLINE_CURVE_WITH_KNOTS((6,1,1,1,1,1,1,1,1,1,1,1,1,1,1,1,1,1,1,1,1,1,
1,1,1,1,1,1,1,1,1,1,1,1,1,1,1,1,1,1,1,1,1,1,1,1,1,1,1,1,1,1,1,1,1,1,1,1,
1,1,1,1,1,1,1,1,1,1,1,1,1,1,1,1,1,1,1,1,1,1,1,1,1,1,1,1,1,1,1,1,1,1,1,1,
1,1,1,1,1,1,1,1,1,1,1,1,1,1,1,1,1,1,1,1,1,1,1,1,1,1,1,1,1,1,1,1,1,1,1,1,
1,1,1,1,1,1,1,1,1,1,1,1,1,1,1,1,1,1,1,1,1,1,1,1,1,1,1,1,1,1,1,1,1,1,1,1,
1,1,1,1,1,1,1,1,1,1,1,1,1,1,1,1,1,1,1,1,1,1,1,1,1,1,1,1,1,1,1,1,1,1,6),
(-1.,-0.995000000000001,-0.990000000000001,-0.985000000000001,-0.980000000000001,
-0.975000000000001,-0.970000000000001,-0.965000000000001,-0.960000000000001,
-0.955000000000001,-0.950000000000001,-0.945000000000001,-0.940000000000001,
-0.935000000000001,-0.930000000000001,-0.925000000000001,-0.920000000000001,
-0.915000000000001,-0.910000000000001,-0.905000000000001,-0.900000000000001,
-0.895000000000001,-0.890000000000001,-0.885000000000001,-0.880000000000001,
-0.875000000000001,-0.870000000000001,-0.865000000000001,-0.860000000000001,
-0.855000000000001,-0.850000000000001,-0.845000000000001,-0.840000000000001,
-0.835000000000001,-0.830000000000001,-0.825000000000001,-0.820000000000001,
-0.815000000000001,-0.810000000000001,-0.805000000000001,-0.800000000000001,
-0.795000000000001,-0.790000000000001,-0.785000000000001,-0.780000000000001,
-0.775000000000001,-0.770000000000001,-0.765000000000001,-0.760000000000001,
-0.755000000000001,-0.750000000000001,-0.745000000000001,-0.740000000000001,
-0.735000000000001,-0.730000000000001,-0.725000000000001,-0.720000000000001,
-0.715000000000001,-0.710000000000001,-0.705000000000001,-0.700000000000001,
-0.695000000000001,-0.690000000000001,-0.685,-0.68,-0.675,-0.67,-0.665,
-0.66,-0.655,-0.65,-0.645,-0.64,-0.635,-0.63,-0.625,-0.62,-0.615,-0.61,
-0.605,-0.6,-0.595,-0.59,-0.585,-0.58,-0.575,-0.57,-0.565,-0.56,-0.555,
-0.55,-0.545,-0.54,-0.535,-0.53,-0.525,-0.52,-0.515,-0.51,-0.505,-0.5,-0.495,
-0.49,-0.485,-0.48,-0.475,-0.47,-0.465,-0.46,-0.455,-0.45,-0.445,-0.44,
-0.435,-0.43,-0.425,-0.42,-0.415,-0.41,-0.405,-0.4,-0.395,-0.39,-0.385,
-0.38,-0.375,-0.37,-0.365,-0.36,-0.355,-0.35,-0.345,-0.34,-0.335,-0.33,
-0.325,-0.32,-0.315,-0.31,-0.305,-0.3,-0.295,-0.29,-0.285,-0.28,-0.275,
-0.27,-0.265,-0.26,-0.255,-0.25,-0.245,-0.24,-0.235,-0.23,-0.225,-0.22,
-0.215,-0.21,-0.205,-0.2,-0.195,-0.19,-0.185,-0.18,-0.175,-0.17,-0.165,
-0.16,-0.155,-0.15,-0.145,-0.14,-0.135,-0.13,-0.125,-0.12,-0.115,-0.11,
-0.105,-0.1,-0.095,-0.09,-0.085,-0.08,-0.075,-0.07,-0.065,-0.06,-0.055,
-0.05,-0.045,-0.04,-0.035,-0.03,-0.025,-0.02,-0.015,-0.01,-0.005,0.),
 .UNSPECIFIED.)
CURVE()
GEOMETRIC_REPRESENTATION_ITEM()
RATIONAL_B_SPLINE_CURVE((1.,1.,1.,1.,1.,1.,1.,1.,1.,1.,1.,1.,1.,1.,1.,1.,
1.,1.,1.,1.,1.,1.,1.,1.,1.,1.,1.,1.,1.,1.,1.,1.,1.,1.,1.,1.,1.,1.,1.,1.,
1.,1.,1.,1.,1.,1.,1.,1.,1.,1.,1.,1.,1.,1.,1.,1.,1.,1.,1.,1.,1.,1.,1.,1.,
1.,1.,1.,1.,1.,1.,1.,1.,1.,1.,1.,1.,1.,1.,1.,1.,1.,1.,1.,1.,1.,1.,1.,1.,
1.,1.,1.,1.,1.,1.,1.,1.,1.,1.,1.,1.,1.,1.,1.,1.,1.,1.,1.,1.,1.,1.,1.,1.,
1.,1.,1.,1.,1.,1.,1.,1.,1.,1.,1.,1.,1.,1.,1.,1.,1.,1.,1.,1.,1.,1.,1.,1.,
1.,1.,1.,1.,1.,1.,1.,1.,1.,1.,1.,1.,1.,1.,1.,1.,1.,1.,1.,1.,1.,1.,1.,1.,
1.,1.,1.,1.,1.,1.,1.,1.,1.,1.,1.,1.,1.,1.,1.,1.,1.,1.,1.,1.,1.,1.,1.,1.,
1.,1.,1.,1.,1.,1.,1.,1.,1.,1.,1.,1.,1.,1.,1.,1.,1.,1.,1.,1.,1.))
REPRESENTATION_ITEM('')
);
#815=(
BOUNDED_CURVE()
B_SPLINE_CURVE(5,(#227983,#227984,#227985,#227986,#227987,#227988,#227989,
#227990,#227991,#227992,#227993,#227994,#227995,#227996,#227997,#227998,
#227999,#228000,#228001,#228002,#228003,#228004,#228005,#228006,#228007,
#228008,#228009,#228010,#228011,#228012,#228013,#228014,#228015,#228016,
#228017,#228018,#228019,#228020,#228021,#228022,#228023,#228024,#228025,
#228026,#228027,#228028,#228029,#228030,#228031,#228032,#228033,#228034,
#228035,#228036,#228037,#228038,#228039,#228040,#228041,#228042,#228043,
#228044,#228045,#228046,#228047,#228048,#228049,#228050,#228051,#228052,
#228053,#228054,#228055,#228056,#228057,#228058,#228059,#228060,#228061,
#228062,#228063,#228064,#228065,#228066,#228067,#228068,#228069,#228070,
#228071,#228072,#228073,#228074,#228075,#228076,#228077,#228078,#228079,
#228080,#228081,#228082,#228083,#228084,#228085,#228086,#228087,#228088,
#228089,#228090,#228091,#228092,#228093,#228094,#228095,#228096,#228097,
#228098,#228099,#228100,#228101,#228102,#228103,#228104,#228105,#228106,
#228107,#228108,#228109,#228110,#228111,#228112,#228113,#228114,#228115,
#228116,#228117,#228118,#228119,#228120,#228121,#228122,#228123,#228124,
#228125,#228126,#228127,#228128,#228129,#228130,#228131,#228132,#228133,
#228134,#228135,#228136,#228137,#228138,#228139,#228140,#228141,#228142,
#228143,#228144,#228145,#228146,#228147,#228148,#228149,#228150,#228151,
#228152,#228153,#228154,#228155,#228156,#228157,#228158,#228159,#228160,
#228161,#228162,#228163,#228164,#228165,#228166,#228167,#228168,#228169,
#228170,#228171,#228172,#228173,#228174,#228175,#228176,#228177,#228178,
#228179,#228180,#228181,#228182,#228183,#228184,#228185,#228186,#228187),
 .UNSPECIFIED.,.F.,.F.)
B_SPLINE_CURVE_WITH_KNOTS((6,1,1,1,1,1,1,1,1,1,1,1,1,1,1,1,1,1,1,1,1,1,
1,1,1,1,1,1,1,1,1,1,1,1,1,1,1,1,1,1,1,1,1,1,1,1,1,1,1,1,1,1,1,1,1,1,1,1,
1,1,1,1,1,1,1,1,1,1,1,1,1,1,1,1,1,1,1,1,1,1,1,1,1,1,1,1,1,1,1,1,1,1,1,1,
1,1,1,1,1,1,1,1,1,1,1,1,1,1,1,1,1,1,1,1,1,1,1,1,1,1,1,1,1,1,1,1,1,1,1,1,
1,1,1,1,1,1,1,1,1,1,1,1,1,1,1,1,1,1,1,1,1,1,1,1,1,1,1,1,1,1,1,1,1,1,1,1,
1,1,1,1,1,1,1,1,1,1,1,1,1,1,1,1,1,1,1,1,1,1,1,1,1,1,1,1,1,1,1,1,1,1,6),
(-1.,-0.995000000000001,-0.990000000000001,-0.985000000000001,-0.980000000000001,
-0.975000000000001,-0.970000000000001,-0.965000000000001,-0.960000000000001,
-0.955000000000001,-0.950000000000001,-0.945000000000001,-0.940000000000001,
-0.935000000000001,-0.930000000000001,-0.925000000000001,-0.920000000000001,
-0.915000000000001,-0.910000000000001,-0.905000000000001,-0.900000000000001,
-0.895000000000001,-0.890000000000001,-0.885000000000001,-0.880000000000001,
-0.875000000000001,-0.870000000000001,-0.865000000000001,-0.860000000000001,
-0.855000000000001,-0.850000000000001,-0.845000000000001,-0.840000000000001,
-0.835000000000001,-0.830000000000001,-0.825000000000001,-0.820000000000001,
-0.815000000000001,-0.810000000000001,-0.805000000000001,-0.800000000000001,
-0.795000000000001,-0.790000000000001,-0.785000000000001,-0.780000000000001,
-0.775000000000001,-0.770000000000001,-0.765000000000001,-0.760000000000001,
-0.755000000000001,-0.750000000000001,-0.745000000000001,-0.740000000000001,
-0.735000000000001,-0.730000000000001,-0.725000000000001,-0.720000000000001,
-0.715000000000001,-0.710000000000001,-0.705000000000001,-0.700000000000001,
-0.695000000000001,-0.690000000000001,-0.685,-0.68,-0.675,-0.67,-0.665,
-0.66,-0.655,-0.65,-0.645,-0.64,-0.635,-0.63,-0.625,-0.62,-0.615,-0.61,
-0.605,-0.6,-0.595,-0.59,-0.585,-0.58,-0.575,-0.57,-0.565,-0.56,-0.555,
-0.55,-0.545,-0.54,-0.535,-0.53,-0.525,-0.52,-0.515,-0.51,-0.505,-0.5,-0.495,
-0.49,-0.485,-0.48,-0.475,-0.47,-0.465,-0.46,-0.455,-0.45,-0.445,-0.44,
-0.435,-0.43,-0.425,-0.42,-0.415,-0.41,-0.405,-0.4,-0.395,-0.39,-0.385,
-0.38,-0.375,-0.37,-0.365,-0.36,-0.355,-0.35,-0.345,-0.34,-0.335,-0.33,
-0.325,-0.32,-0.315,-0.31,-0.305,-0.3,-0.295,-0.29,-0.285,-0.28,-0.275,
-0.27,-0.265,-0.26,-0.255,-0.25,-0.245,-0.24,-0.235,-0.23,-0.225,-0.22,
-0.215,-0.21,-0.205,-0.2,-0.195,-0.19,-0.185,-0.18,-0.175,-0.17,-0.165,
-0.16,-0.155,-0.15,-0.145,-0.14,-0.135,-0.13,-0.125,-0.12,-0.115,-0.11,
-0.105,-0.1,-0.095,-0.09,-0.085,-0.08,-0.075,-0.07,-0.065,-0.06,-0.055,
-0.05,-0.045,-0.04,-0.035,-0.03,-0.025,-0.02,-0.015,-0.01,-0.005,0.),
 .UNSPECIFIED.)
CURVE()
GEOMETRIC_REPRESENTATION_ITEM()
RATIONAL_B_SPLINE_CURVE((1.,1.,1.,1.,1.,1.,1.,1.,1.,1.,1.,1.,1.,1.,1.,1.,
1.,1.,1.,1.,1.,1.,1.,1.,1.,1.,1.,1.,1.,1.,1.,1.,1.,1.,1.,1.,1.,1.,1.,1.,
1.,1.,1.,1.,1.,1.,1.,1.,1.,1.,1.,1.,1.,1.,1.,1.,1.,1.,1.,1.,1.,1.,1.,1.,
1.,1.,1.,1.,1.,1.,1.,1.,1.,1.,1.,1.,1.,1.,1.,1.,1.,1.,1.,1.,1.,1.,1.,1.,
1.,1.,1.,1.,1.,1.,1.,1.,1.,1.,1.,1.,1.,1.,1.,1.,1.,1.,1.,1.,1.,1.,1.,1.,
1.,1.,1.,1.,1.,1.,1.,1.,1.,1.,1.,1.,1.,1.,1.,1.,1.,1.,1.,1.,1.,1.,1.,1.,
1.,1.,1.,1.,1.,1.,1.,1.,1.,1.,1.,1.,1.,1.,1.,1.,1.,1.,1.,1.,1.,1.,1.,1.,
1.,1.,1.,1.,1.,1.,1.,1.,1.,1.,1.,1.,1.,1.,1.,1.,1.,1.,1.,1.,1.,1.,1.,1.,
1.,1.,1.,1.,1.,1.,1.,1.,1.,1.,1.,1.,1.,1.,1.,1.,1.,1.,1.,1.,1.))
REPRESENTATION_ITEM('')
);
#816=(
BOUNDED_CURVE()
B_SPLINE_CURVE(5,(#228190,#228191,#228192,#228193,#228194,#228195,#228196,
#228197,#228198,#228199,#228200,#228201,#228202,#228203,#228204,#228205,
#228206,#228207,#228208,#228209,#228210,#228211,#228212,#228213,#228214,
#228215,#228216,#228217,#228218,#228219,#228220,#228221,#228222,#228223,
#228224,#228225,#228226,#228227,#228228,#228229,#228230,#228231,#228232,
#228233,#228234,#228235,#228236,#228237,#228238,#228239,#228240,#228241,
#228242,#228243,#228244,#228245,#228246,#228247,#228248,#228249,#228250,
#228251,#228252,#228253,#228254,#228255,#228256,#228257,#228258,#228259,
#228260,#228261,#228262,#228263,#228264,#228265,#228266,#228267,#228268,
#228269,#228270,#228271,#228272,#228273,#228274,#228275,#228276,#228277,
#228278,#228279,#228280,#228281,#228282,#228283,#228284,#228285,#228286,
#228287,#228288,#228289,#228290,#228291,#228292,#228293,#228294,#228295,
#228296,#228297,#228298,#228299,#228300,#228301,#228302,#228303,#228304,
#228305,#228306,#228307,#228308,#228309,#228310,#228311,#228312,#228313,
#228314,#228315,#228316,#228317,#228318,#228319,#228320,#228321,#228322,
#228323,#228324,#228325,#228326,#228327,#228328,#228329,#228330,#228331,
#228332,#228333,#228334,#228335,#228336,#228337,#228338,#228339,#228340,
#228341,#228342,#228343,#228344,#228345,#228346,#228347,#228348,#228349,
#228350,#228351,#228352,#228353,#228354,#228355,#228356,#228357,#228358,
#228359,#228360,#228361,#228362,#228363,#228364,#228365,#228366,#228367,
#228368,#228369,#228370,#228371,#228372,#228373,#228374,#228375,#228376,
#228377,#228378,#228379,#228380,#228381,#228382,#228383,#228384,#228385,
#228386,#228387,#228388,#228389,#228390,#228391,#228392,#228393,#228394),
 .UNSPECIFIED.,.F.,.F.)
B_SPLINE_CURVE_WITH_KNOTS((6,1,1,1,1,1,1,1,1,1,1,1,1,1,1,1,1,1,1,1,1,1,
1,1,1,1,1,1,1,1,1,1,1,1,1,1,1,1,1,1,1,1,1,1,1,1,1,1,1,1,1,1,1,1,1,1,1,1,
1,1,1,1,1,1,1,1,1,1,1,1,1,1,1,1,1,1,1,1,1,1,1,1,1,1,1,1,1,1,1,1,1,1,1,1,
1,1,1,1,1,1,1,1,1,1,1,1,1,1,1,1,1,1,1,1,1,1,1,1,1,1,1,1,1,1,1,1,1,1,1,1,
1,1,1,1,1,1,1,1,1,1,1,1,1,1,1,1,1,1,1,1,1,1,1,1,1,1,1,1,1,1,1,1,1,1,1,1,
1,1,1,1,1,1,1,1,1,1,1,1,1,1,1,1,1,1,1,1,1,1,1,1,1,1,1,1,1,1,1,1,1,1,6),
(0.,0.005,0.01,0.015,0.02,0.025,0.03,0.035,0.04,0.045,0.05,0.055,0.06,0.065,
0.07,0.075,0.08,0.085,0.09,0.095,0.1,0.105,0.11,0.115,0.12,0.125,0.13,0.135,
0.14,0.145,0.15,0.155,0.16,0.165,0.17,0.175,0.18,0.185,0.19,0.195,0.2,0.205,
0.21,0.215,0.22,0.225,0.23,0.235,0.24,0.245,0.25,0.255,0.26,0.265,0.27,
0.275,0.28,0.285,0.29,0.295,0.3,0.305,0.31,0.315,0.32,0.325,0.33,0.335,
0.34,0.345,0.35,0.355,0.36,0.365,0.37,0.375,0.38,0.385,0.39,0.395,0.4,0.405,
0.41,0.415,0.42,0.425,0.43,0.435,0.44,0.445,0.45,0.455,0.46,0.465,0.47,
0.475,0.48,0.485,0.49,0.495,0.5,0.505,0.51,0.515,0.52,0.525,0.53,0.535,
0.54,0.545,0.55,0.555,0.56,0.565,0.57,0.575,0.58,0.585,0.59,0.595,0.6,0.605,
0.61,0.615,0.62,0.625,0.63,0.635,0.64,0.645,0.65,0.655,0.66,0.665,0.67,
0.675,0.68,0.685,0.690000000000001,0.695000000000001,0.700000000000001,
0.705000000000001,0.710000000000001,0.715000000000001,0.720000000000001,
0.725000000000001,0.730000000000001,0.735000000000001,0.740000000000001,
0.745000000000001,0.750000000000001,0.755000000000001,0.760000000000001,
0.765000000000001,0.770000000000001,0.775000000000001,0.780000000000001,
0.785000000000001,0.790000000000001,0.795000000000001,0.800000000000001,
0.805000000000001,0.810000000000001,0.815000000000001,0.820000000000001,
0.825000000000001,0.830000000000001,0.835000000000001,0.840000000000001,
0.845000000000001,0.850000000000001,0.855000000000001,0.860000000000001,
0.865000000000001,0.870000000000001,0.875000000000001,0.880000000000001,
0.885000000000001,0.890000000000001,0.895000000000001,0.900000000000001,
0.905000000000001,0.910000000000001,0.915000000000001,0.920000000000001,
0.925000000000001,0.930000000000001,0.935000000000001,0.940000000000001,
0.945000000000001,0.950000000000001,0.955000000000001,0.960000000000001,
0.965000000000001,0.970000000000001,0.975000000000001,0.980000000000001,
0.985000000000001,0.990000000000001,0.995000000000001,1.),.UNSPECIFIED.)
CURVE()
GEOMETRIC_REPRESENTATION_ITEM()
RATIONAL_B_SPLINE_CURVE((1.,1.,1.,1.,1.,1.,1.,1.,1.,1.,1.,1.,1.,1.,1.,1.,
1.,1.,1.,1.,1.,1.,1.,1.,1.,1.,1.,1.,1.,1.,1.,1.,1.,1.,1.,1.,1.,1.,1.,1.,
1.,1.,1.,1.,1.,1.,1.,1.,1.,1.,1.,1.,1.,1.,1.,1.,1.,1.,1.,1.,1.,1.,1.,1.,
1.,1.,1.,1.,1.,1.,1.,1.,1.,1.,1.,1.,1.,1.,1.,1.,1.,1.,1.,1.,1.,1.,1.,1.,
1.,1.,1.,1.,1.,1.,1.,1.,1.,1.,1.,1.,1.,1.,1.,1.,1.,1.,1.,1.,1.,1.,1.,1.,
1.,1.,1.,1.,1.,1.,1.,1.,1.,1.,1.,1.,1.,1.,1.,1.,1.,1.,1.,1.,1.,1.,1.,1.,
1.,1.,1.,1.,1.,1.,1.,1.,1.,1.,1.,1.,1.,1.,1.,1.,1.,1.,1.,1.,1.,1.,1.,1.,
1.,1.,1.,1.,1.,1.,1.,1.,1.,1.,1.,1.,1.,1.,1.,1.,1.,1.,1.,1.,1.,1.,1.,1.,
1.,1.,1.,1.,1.,1.,1.,1.,1.,1.,1.,1.,1.,1.,1.,1.,1.,1.,1.,1.,1.))
REPRESENTATION_ITEM('')
);
#817=(
BOUNDED_CURVE()
B_SPLINE_CURVE(5,(#228806,#228807,#228808,#228809,#228810,#228811,#228812,
#228813,#228814,#228815,#228816,#228817,#228818,#228819,#228820,#228821,
#228822,#228823,#228824,#228825,#228826,#228827,#228828,#228829,#228830,
#228831,#228832,#228833,#228834,#228835,#228836,#228837,#228838,#228839,
#228840,#228841,#228842,#228843,#228844,#228845,#228846,#228847,#228848,
#228849,#228850,#228851,#228852,#228853,#228854,#228855,#228856,#228857,
#228858,#228859,#228860,#228861,#228862,#228863,#228864,#228865,#228866,
#228867,#228868,#228869,#228870,#228871,#228872,#228873,#228874,#228875,
#228876,#228877,#228878,#228879,#228880,#228881,#228882,#228883,#228884,
#228885,#228886,#228887,#228888,#228889,#228890,#228891,#228892,#228893,
#228894,#228895,#228896,#228897,#228898,#228899,#228900,#228901,#228902,
#228903,#228904,#228905,#228906,#228907,#228908,#228909,#228910,#228911,
#228912,#228913,#228914,#228915,#228916,#228917,#228918,#228919,#228920,
#228921,#228922,#228923,#228924,#228925,#228926,#228927,#228928,#228929,
#228930,#228931,#228932,#228933,#228934,#228935,#228936,#228937,#228938,
#228939,#228940,#228941,#228942,#228943,#228944,#228945,#228946,#228947,
#228948,#228949,#228950,#228951,#228952,#228953,#228954,#228955,#228956,
#228957,#228958,#228959,#228960,#228961,#228962,#228963,#228964,#228965,
#228966,#228967,#228968,#228969,#228970,#228971,#228972,#228973,#228974,
#228975,#228976,#228977,#228978,#228979,#228980,#228981,#228982,#228983,
#228984,#228985,#228986,#228987,#228988,#228989,#228990,#228991,#228992,
#228993,#228994,#228995,#228996,#228997,#228998,#228999,#229000,#229001,
#229002,#229003,#229004,#229005,#229006,#229007,#229008,#229009,#229010),
 .UNSPECIFIED.,.F.,.F.)
B_SPLINE_CURVE_WITH_KNOTS((6,1,1,1,1,1,1,1,1,1,1,1,1,1,1,1,1,1,1,1,1,1,
1,1,1,1,1,1,1,1,1,1,1,1,1,1,1,1,1,1,1,1,1,1,1,1,1,1,1,1,1,1,1,1,1,1,1,1,
1,1,1,1,1,1,1,1,1,1,1,1,1,1,1,1,1,1,1,1,1,1,1,1,1,1,1,1,1,1,1,1,1,1,1,1,
1,1,1,1,1,1,1,1,1,1,1,1,1,1,1,1,1,1,1,1,1,1,1,1,1,1,1,1,1,1,1,1,1,1,1,1,
1,1,1,1,1,1,1,1,1,1,1,1,1,1,1,1,1,1,1,1,1,1,1,1,1,1,1,1,1,1,1,1,1,1,1,1,
1,1,1,1,1,1,1,1,1,1,1,1,1,1,1,1,1,1,1,1,1,1,1,1,1,1,1,1,1,1,1,1,1,1,6),
(0.,0.005,0.01,0.015,0.02,0.025,0.03,0.035,0.04,0.045,0.05,0.055,0.06,0.065,
0.07,0.075,0.08,0.085,0.09,0.095,0.1,0.105,0.11,0.115,0.12,0.125,0.13,0.135,
0.14,0.145,0.15,0.155,0.16,0.165,0.17,0.175,0.18,0.185,0.19,0.195,0.2,0.205,
0.21,0.215,0.22,0.225,0.23,0.235,0.24,0.245,0.25,0.255,0.26,0.265,0.27,
0.275,0.28,0.285,0.29,0.295,0.3,0.305,0.31,0.315,0.32,0.325,0.33,0.335,
0.34,0.345,0.35,0.355,0.36,0.365,0.37,0.375,0.38,0.385,0.39,0.395,0.4,0.405,
0.41,0.415,0.42,0.425,0.43,0.435,0.44,0.445,0.45,0.455,0.46,0.465,0.47,
0.475,0.48,0.485,0.49,0.495,0.5,0.505,0.51,0.515,0.52,0.525,0.53,0.535,
0.54,0.545,0.55,0.555,0.56,0.565,0.57,0.575,0.58,0.585,0.59,0.595,0.6,0.605,
0.61,0.615,0.62,0.625,0.63,0.635,0.64,0.645,0.65,0.655,0.66,0.665,0.67,
0.675,0.68,0.685,0.690000000000001,0.695000000000001,0.700000000000001,
0.705000000000001,0.710000000000001,0.715000000000001,0.720000000000001,
0.725000000000001,0.730000000000001,0.735000000000001,0.740000000000001,
0.745000000000001,0.750000000000001,0.755000000000001,0.760000000000001,
0.765000000000001,0.770000000000001,0.775000000000001,0.780000000000001,
0.785000000000001,0.790000000000001,0.795000000000001,0.800000000000001,
0.805000000000001,0.810000000000001,0.815000000000001,0.820000000000001,
0.825000000000001,0.830000000000001,0.835000000000001,0.840000000000001,
0.845000000000001,0.850000000000001,0.855000000000001,0.860000000000001,
0.865000000000001,0.870000000000001,0.875000000000001,0.880000000000001,
0.885000000000001,0.890000000000001,0.895000000000001,0.900000000000001,
0.905000000000001,0.910000000000001,0.915000000000001,0.920000000000001,
0.925000000000001,0.930000000000001,0.935000000000001,0.940000000000001,
0.945000000000001,0.950000000000001,0.955000000000001,0.960000000000001,
0.965000000000001,0.970000000000001,0.975000000000001,0.980000000000001,
0.985000000000001,0.990000000000001,0.995000000000001,1.),.UNSPECIFIED.)
CURVE()
GEOMETRIC_REPRESENTATION_ITEM()
RATIONAL_B_SPLINE_CURVE((1.,1.,1.,1.,1.,1.,1.,1.,1.,1.,1.,1.,1.,1.,1.,1.,
1.,1.,1.,1.,1.,1.,1.,1.,1.,1.,1.,1.,1.,1.,1.,1.,1.,1.,1.,1.,1.,1.,1.,1.,
1.,1.,1.,1.,1.,1.,1.,1.,1.,1.,1.,1.,1.,1.,1.,1.,1.,1.,1.,1.,1.,1.,1.,1.,
1.,1.,1.,1.,1.,1.,1.,1.,1.,1.,1.,1.,1.,1.,1.,1.,1.,1.,1.,1.,1.,1.,1.,1.,
1.,1.,1.,1.,1.,1.,1.,1.,1.,1.,1.,1.,1.,1.,1.,1.,1.,1.,1.,1.,1.,1.,1.,1.,
1.,1.,1.,1.,1.,1.,1.,1.,1.,1.,1.,1.,1.,1.,1.,1.,1.,1.,1.,1.,1.,1.,1.,1.,
1.,1.,1.,1.,1.,1.,1.,1.,1.,1.,1.,1.,1.,1.,1.,1.,1.,1.,1.,1.,1.,1.,1.,1.,
1.,1.,1.,1.,1.,1.,1.,1.,1.,1.,1.,1.,1.,1.,1.,1.,1.,1.,1.,1.,1.,1.,1.,1.,
1.,1.,1.,1.,1.,1.,1.,1.,1.,1.,1.,1.,1.,1.,1.,1.,1.,1.,1.,1.,1.))
REPRESENTATION_ITEM('')
);
#818=(
BOUNDED_CURVE()
B_SPLINE_CURVE(5,(#229012,#229013,#229014,#229015,#229016,#229017,#229018,
#229019,#229020,#229021,#229022,#229023,#229024,#229025,#229026,#229027,
#229028,#229029,#229030,#229031,#229032,#229033,#229034,#229035,#229036,
#229037,#229038,#229039,#229040,#229041,#229042,#229043,#229044,#229045,
#229046,#229047,#229048,#229049,#229050,#229051,#229052,#229053,#229054,
#229055,#229056,#229057,#229058,#229059,#229060,#229061,#229062,#229063,
#229064,#229065,#229066,#229067,#229068,#229069,#229070,#229071,#229072,
#229073,#229074,#229075,#229076,#229077,#229078,#229079,#229080,#229081,
#229082,#229083,#229084,#229085,#229086,#229087,#229088,#229089,#229090,
#229091,#229092,#229093,#229094,#229095,#229096,#229097,#229098,#229099,
#229100,#229101,#229102,#229103,#229104,#229105,#229106,#229107,#229108,
#229109,#229110,#229111,#229112,#229113,#229114,#229115,#229116,#229117,
#229118,#229119,#229120,#229121,#229122,#229123,#229124,#229125,#229126,
#229127,#229128,#229129,#229130,#229131,#229132,#229133,#229134,#229135,
#229136,#229137,#229138,#229139,#229140,#229141,#229142,#229143,#229144,
#229145,#229146,#229147,#229148,#229149,#229150,#229151,#229152,#229153,
#229154,#229155,#229156,#229157,#229158,#229159,#229160,#229161,#229162,
#229163,#229164,#229165,#229166,#229167,#229168,#229169,#229170,#229171,
#229172,#229173,#229174,#229175,#229176,#229177,#229178,#229179,#229180,
#229181,#229182,#229183,#229184,#229185,#229186,#229187,#229188,#229189,
#229190,#229191,#229192,#229193,#229194,#229195,#229196,#229197,#229198,
#229199,#229200,#229201,#229202,#229203,#229204,#229205,#229206,#229207,
#229208,#229209,#229210,#229211,#229212,#229213,#229214,#229215,#229216),
 .UNSPECIFIED.,.F.,.F.)
B_SPLINE_CURVE_WITH_KNOTS((6,1,1,1,1,1,1,1,1,1,1,1,1,1,1,1,1,1,1,1,1,1,
1,1,1,1,1,1,1,1,1,1,1,1,1,1,1,1,1,1,1,1,1,1,1,1,1,1,1,1,1,1,1,1,1,1,1,1,
1,1,1,1,1,1,1,1,1,1,1,1,1,1,1,1,1,1,1,1,1,1,1,1,1,1,1,1,1,1,1,1,1,1,1,1,
1,1,1,1,1,1,1,1,1,1,1,1,1,1,1,1,1,1,1,1,1,1,1,1,1,1,1,1,1,1,1,1,1,1,1,1,
1,1,1,1,1,1,1,1,1,1,1,1,1,1,1,1,1,1,1,1,1,1,1,1,1,1,1,1,1,1,1,1,1,1,1,1,
1,1,1,1,1,1,1,1,1,1,1,1,1,1,1,1,1,1,1,1,1,1,1,1,1,1,1,1,1,1,1,1,1,1,6),
(-1.,-0.995000000000001,-0.990000000000001,-0.985000000000001,-0.980000000000001,
-0.975000000000001,-0.970000000000001,-0.965000000000001,-0.960000000000001,
-0.955000000000001,-0.950000000000001,-0.945000000000001,-0.940000000000001,
-0.935000000000001,-0.930000000000001,-0.925000000000001,-0.920000000000001,
-0.915000000000001,-0.910000000000001,-0.905000000000001,-0.900000000000001,
-0.895000000000001,-0.890000000000001,-0.885000000000001,-0.880000000000001,
-0.875000000000001,-0.870000000000001,-0.865000000000001,-0.860000000000001,
-0.855000000000001,-0.850000000000001,-0.845000000000001,-0.840000000000001,
-0.835000000000001,-0.830000000000001,-0.825000000000001,-0.820000000000001,
-0.815000000000001,-0.810000000000001,-0.805000000000001,-0.800000000000001,
-0.795000000000001,-0.790000000000001,-0.785000000000001,-0.780000000000001,
-0.775000000000001,-0.770000000000001,-0.765000000000001,-0.760000000000001,
-0.755000000000001,-0.750000000000001,-0.745000000000001,-0.740000000000001,
-0.735000000000001,-0.730000000000001,-0.725000000000001,-0.720000000000001,
-0.715000000000001,-0.710000000000001,-0.705000000000001,-0.700000000000001,
-0.695000000000001,-0.690000000000001,-0.685,-0.68,-0.675,-0.67,-0.665,
-0.66,-0.655,-0.65,-0.645,-0.64,-0.635,-0.63,-0.625,-0.62,-0.615,-0.61,
-0.605,-0.6,-0.595,-0.59,-0.585,-0.58,-0.575,-0.57,-0.565,-0.56,-0.555,
-0.55,-0.545,-0.54,-0.535,-0.53,-0.525,-0.52,-0.515,-0.51,-0.505,-0.5,-0.495,
-0.49,-0.485,-0.48,-0.475,-0.47,-0.465,-0.46,-0.455,-0.45,-0.445,-0.44,
-0.435,-0.43,-0.425,-0.42,-0.415,-0.41,-0.405,-0.4,-0.395,-0.39,-0.385,
-0.38,-0.375,-0.37,-0.365,-0.36,-0.355,-0.35,-0.345,-0.34,-0.335,-0.33,
-0.325,-0.32,-0.315,-0.31,-0.305,-0.3,-0.295,-0.29,-0.285,-0.28,-0.275,
-0.27,-0.265,-0.26,-0.255,-0.25,-0.245,-0.24,-0.235,-0.23,-0.225,-0.22,
-0.215,-0.21,-0.205,-0.2,-0.195,-0.19,-0.185,-0.18,-0.175,-0.17,-0.165,
-0.16,-0.155,-0.15,-0.145,-0.14,-0.135,-0.13,-0.125,-0.12,-0.115,-0.11,
-0.105,-0.1,-0.095,-0.09,-0.085,-0.08,-0.075,-0.07,-0.065,-0.06,-0.055,
-0.05,-0.045,-0.04,-0.035,-0.03,-0.025,-0.02,-0.015,-0.01,-0.005,0.),
 .UNSPECIFIED.)
CURVE()
GEOMETRIC_REPRESENTATION_ITEM()
RATIONAL_B_SPLINE_CURVE((1.,1.,1.,1.,1.,1.,1.,1.,1.,1.,1.,1.,1.,1.,1.,1.,
1.,1.,1.,1.,1.,1.,1.,1.,1.,1.,1.,1.,1.,1.,1.,1.,1.,1.,1.,1.,1.,1.,1.,1.,
1.,1.,1.,1.,1.,1.,1.,1.,1.,1.,1.,1.,1.,1.,1.,1.,1.,1.,1.,1.,1.,1.,1.,1.,
1.,1.,1.,1.,1.,1.,1.,1.,1.,1.,1.,1.,1.,1.,1.,1.,1.,1.,1.,1.,1.,1.,1.,1.,
1.,1.,1.,1.,1.,1.,1.,1.,1.,1.,1.,1.,1.,1.,1.,1.,1.,1.,1.,1.,1.,1.,1.,1.,
1.,1.,1.,1.,1.,1.,1.,1.,1.,1.,1.,1.,1.,1.,1.,1.,1.,1.,1.,1.,1.,1.,1.,1.,
1.,1.,1.,1.,1.,1.,1.,1.,1.,1.,1.,1.,1.,1.,1.,1.,1.,1.,1.,1.,1.,1.,1.,1.,
1.,1.,1.,1.,1.,1.,1.,1.,1.,1.,1.,1.,1.,1.,1.,1.,1.,1.,1.,1.,1.,1.,1.,1.,
1.,1.,1.,1.,1.,1.,1.,1.,1.,1.,1.,1.,1.,1.,1.,1.,1.,1.,1.,1.,1.))
REPRESENTATION_ITEM('')
);
#819=(
BOUNDED_CURVE()
B_SPLINE_CURVE(5,(#229635,#229636,#229637,#229638,#229639,#229640,#229641,
#229642,#229643,#229644,#229645,#229646,#229647,#229648,#229649,#229650,
#229651,#229652,#229653,#229654,#229655,#229656,#229657,#229658,#229659,
#229660,#229661,#229662,#229663,#229664,#229665,#229666,#229667,#229668,
#229669,#229670,#229671,#229672,#229673,#229674,#229675,#229676,#229677,
#229678,#229679,#229680,#229681,#229682,#229683,#229684,#229685,#229686,
#229687,#229688,#229689,#229690,#229691,#229692,#229693,#229694,#229695,
#229696,#229697,#229698,#229699,#229700,#229701,#229702,#229703,#229704,
#229705,#229706,#229707,#229708,#229709,#229710,#229711,#229712,#229713,
#229714,#229715,#229716,#229717,#229718,#229719,#229720,#229721,#229722,
#229723,#229724,#229725,#229726,#229727,#229728,#229729,#229730,#229731,
#229732,#229733,#229734,#229735,#229736,#229737,#229738,#229739,#229740,
#229741,#229742,#229743,#229744,#229745,#229746,#229747,#229748,#229749,
#229750,#229751,#229752,#229753,#229754,#229755,#229756,#229757,#229758,
#229759,#229760,#229761,#229762,#229763,#229764,#229765,#229766,#229767,
#229768,#229769,#229770,#229771,#229772,#229773,#229774,#229775,#229776,
#229777,#229778,#229779,#229780,#229781,#229782,#229783,#229784,#229785,
#229786,#229787,#229788,#229789,#229790,#229791,#229792,#229793,#229794,
#229795,#229796,#229797,#229798,#229799,#229800,#229801,#229802,#229803,
#229804,#229805,#229806,#229807,#229808,#229809,#229810,#229811,#229812,
#229813,#229814,#229815,#229816,#229817,#229818,#229819,#229820,#229821,
#229822,#229823,#229824,#229825,#229826,#229827,#229828,#229829,#229830,
#229831,#229832,#229833,#229834,#229835,#229836,#229837,#229838,#229839),
 .UNSPECIFIED.,.F.,.F.)
B_SPLINE_CURVE_WITH_KNOTS((6,1,1,1,1,1,1,1,1,1,1,1,1,1,1,1,1,1,1,1,1,1,
1,1,1,1,1,1,1,1,1,1,1,1,1,1,1,1,1,1,1,1,1,1,1,1,1,1,1,1,1,1,1,1,1,1,1,1,
1,1,1,1,1,1,1,1,1,1,1,1,1,1,1,1,1,1,1,1,1,1,1,1,1,1,1,1,1,1,1,1,1,1,1,1,
1,1,1,1,1,1,1,1,1,1,1,1,1,1,1,1,1,1,1,1,1,1,1,1,1,1,1,1,1,1,1,1,1,1,1,1,
1,1,1,1,1,1,1,1,1,1,1,1,1,1,1,1,1,1,1,1,1,1,1,1,1,1,1,1,1,1,1,1,1,1,1,1,
1,1,1,1,1,1,1,1,1,1,1,1,1,1,1,1,1,1,1,1,1,1,1,1,1,1,1,1,1,1,1,1,1,1,6),
(-1.,-0.995000000000001,-0.990000000000001,-0.985000000000001,-0.980000000000001,
-0.975000000000001,-0.970000000000001,-0.965000000000001,-0.960000000000001,
-0.955000000000001,-0.950000000000001,-0.945000000000001,-0.940000000000001,
-0.935000000000001,-0.930000000000001,-0.925000000000001,-0.920000000000001,
-0.915000000000001,-0.910000000000001,-0.905000000000001,-0.900000000000001,
-0.895000000000001,-0.890000000000001,-0.885000000000001,-0.880000000000001,
-0.875000000000001,-0.870000000000001,-0.865000000000001,-0.860000000000001,
-0.855000000000001,-0.850000000000001,-0.845000000000001,-0.840000000000001,
-0.835000000000001,-0.830000000000001,-0.825000000000001,-0.820000000000001,
-0.815000000000001,-0.810000000000001,-0.805000000000001,-0.800000000000001,
-0.795000000000001,-0.790000000000001,-0.785000000000001,-0.780000000000001,
-0.775000000000001,-0.770000000000001,-0.765000000000001,-0.760000000000001,
-0.755000000000001,-0.750000000000001,-0.745000000000001,-0.740000000000001,
-0.735000000000001,-0.730000000000001,-0.725000000000001,-0.720000000000001,
-0.715000000000001,-0.710000000000001,-0.705000000000001,-0.700000000000001,
-0.695000000000001,-0.690000000000001,-0.685,-0.68,-0.675,-0.67,-0.665,
-0.66,-0.655,-0.65,-0.645,-0.64,-0.635,-0.63,-0.625,-0.62,-0.615,-0.61,
-0.605,-0.6,-0.595,-0.59,-0.585,-0.58,-0.575,-0.57,-0.565,-0.56,-0.555,
-0.55,-0.545,-0.54,-0.535,-0.53,-0.525,-0.52,-0.515,-0.51,-0.505,-0.5,-0.495,
-0.49,-0.485,-0.48,-0.475,-0.47,-0.465,-0.46,-0.455,-0.45,-0.445,-0.44,
-0.435,-0.43,-0.425,-0.42,-0.415,-0.41,-0.405,-0.4,-0.395,-0.39,-0.385,
-0.38,-0.375,-0.37,-0.365,-0.36,-0.355,-0.35,-0.345,-0.34,-0.335,-0.33,
-0.325,-0.32,-0.315,-0.31,-0.305,-0.3,-0.295,-0.29,-0.285,-0.28,-0.275,
-0.27,-0.265,-0.26,-0.255,-0.25,-0.245,-0.24,-0.235,-0.23,-0.225,-0.22,
-0.215,-0.21,-0.205,-0.2,-0.195,-0.19,-0.185,-0.18,-0.175,-0.17,-0.165,
-0.16,-0.155,-0.15,-0.145,-0.14,-0.135,-0.13,-0.125,-0.12,-0.115,-0.11,
-0.105,-0.1,-0.095,-0.09,-0.085,-0.08,-0.075,-0.07,-0.065,-0.06,-0.055,
-0.05,-0.045,-0.04,-0.035,-0.03,-0.025,-0.02,-0.015,-0.01,-0.005,0.),
 .UNSPECIFIED.)
CURVE()
GEOMETRIC_REPRESENTATION_ITEM()
RATIONAL_B_SPLINE_CURVE((1.,1.,1.,1.,1.,1.,1.,1.,1.,1.,1.,1.,1.,1.,1.,1.,
1.,1.,1.,1.,1.,1.,1.,1.,1.,1.,1.,1.,1.,1.,1.,1.,1.,1.,1.,1.,1.,1.,1.,1.,
1.,1.,1.,1.,1.,1.,1.,1.,1.,1.,1.,1.,1.,1.,1.,1.,1.,1.,1.,1.,1.,1.,1.,1.,
1.,1.,1.,1.,1.,1.,1.,1.,1.,1.,1.,1.,1.,1.,1.,1.,1.,1.,1.,1.,1.,1.,1.,1.,
1.,1.,1.,1.,1.,1.,1.,1.,1.,1.,1.,1.,1.,1.,1.,1.,1.,1.,1.,1.,1.,1.,1.,1.,
1.,1.,1.,1.,1.,1.,1.,1.,1.,1.,1.,1.,1.,1.,1.,1.,1.,1.,1.,1.,1.,1.,1.,1.,
1.,1.,1.,1.,1.,1.,1.,1.,1.,1.,1.,1.,1.,1.,1.,1.,1.,1.,1.,1.,1.,1.,1.,1.,
1.,1.,1.,1.,1.,1.,1.,1.,1.,1.,1.,1.,1.,1.,1.,1.,1.,1.,1.,1.,1.,1.,1.,1.,
1.,1.,1.,1.,1.,1.,1.,1.,1.,1.,1.,1.,1.,1.,1.,1.,1.,1.,1.,1.,1.))
REPRESENTATION_ITEM('')
);
#820=(
BOUNDED_CURVE()
B_SPLINE_CURVE(5,(#229842,#229843,#229844,#229845,#229846,#229847,#229848,
#229849,#229850,#229851,#229852,#229853,#229854,#229855,#229856,#229857,
#229858,#229859,#229860,#229861,#229862,#229863,#229864,#229865,#229866,
#229867,#229868,#229869,#229870,#229871,#229872,#229873,#229874,#229875,
#229876,#229877,#229878,#229879,#229880,#229881,#229882,#229883,#229884,
#229885,#229886,#229887,#229888,#229889,#229890,#229891,#229892,#229893,
#229894,#229895,#229896,#229897,#229898,#229899,#229900,#229901,#229902,
#229903,#229904,#229905,#229906,#229907,#229908,#229909,#229910,#229911,
#229912,#229913,#229914,#229915,#229916,#229917,#229918,#229919,#229920,
#229921,#229922,#229923,#229924,#229925,#229926,#229927,#229928,#229929,
#229930,#229931,#229932,#229933,#229934,#229935,#229936,#229937,#229938,
#229939,#229940,#229941,#229942,#229943,#229944,#229945,#229946,#229947,
#229948,#229949,#229950,#229951,#229952,#229953,#229954,#229955,#229956,
#229957,#229958,#229959,#229960,#229961,#229962,#229963,#229964,#229965,
#229966,#229967,#229968,#229969,#229970,#229971,#229972,#229973,#229974,
#229975,#229976,#229977,#229978,#229979,#229980,#229981,#229982,#229983,
#229984,#229985,#229986,#229987,#229988,#229989,#229990,#229991,#229992,
#229993,#229994,#229995,#229996,#229997,#229998,#229999,#230000,#230001,
#230002,#230003,#230004,#230005,#230006,#230007,#230008,#230009,#230010,
#230011,#230012,#230013,#230014,#230015,#230016,#230017,#230018,#230019,
#230020,#230021,#230022,#230023,#230024,#230025,#230026,#230027,#230028,
#230029,#230030,#230031,#230032,#230033,#230034,#230035,#230036,#230037,
#230038,#230039,#230040,#230041,#230042,#230043,#230044,#230045,#230046),
 .UNSPECIFIED.,.F.,.F.)
B_SPLINE_CURVE_WITH_KNOTS((6,1,1,1,1,1,1,1,1,1,1,1,1,1,1,1,1,1,1,1,1,1,
1,1,1,1,1,1,1,1,1,1,1,1,1,1,1,1,1,1,1,1,1,1,1,1,1,1,1,1,1,1,1,1,1,1,1,1,
1,1,1,1,1,1,1,1,1,1,1,1,1,1,1,1,1,1,1,1,1,1,1,1,1,1,1,1,1,1,1,1,1,1,1,1,
1,1,1,1,1,1,1,1,1,1,1,1,1,1,1,1,1,1,1,1,1,1,1,1,1,1,1,1,1,1,1,1,1,1,1,1,
1,1,1,1,1,1,1,1,1,1,1,1,1,1,1,1,1,1,1,1,1,1,1,1,1,1,1,1,1,1,1,1,1,1,1,1,
1,1,1,1,1,1,1,1,1,1,1,1,1,1,1,1,1,1,1,1,1,1,1,1,1,1,1,1,1,1,1,1,1,1,6),
(0.,0.005,0.01,0.015,0.02,0.025,0.03,0.035,0.04,0.045,0.05,0.055,0.06,0.065,
0.07,0.075,0.08,0.085,0.09,0.095,0.1,0.105,0.11,0.115,0.12,0.125,0.13,0.135,
0.14,0.145,0.15,0.155,0.16,0.165,0.17,0.175,0.18,0.185,0.19,0.195,0.2,0.205,
0.21,0.215,0.22,0.225,0.23,0.235,0.24,0.245,0.25,0.255,0.26,0.265,0.27,
0.275,0.28,0.285,0.29,0.295,0.3,0.305,0.31,0.315,0.32,0.325,0.33,0.335,
0.34,0.345,0.35,0.355,0.36,0.365,0.37,0.375,0.38,0.385,0.39,0.395,0.4,0.405,
0.41,0.415,0.42,0.425,0.43,0.435,0.44,0.445,0.45,0.455,0.46,0.465,0.47,
0.475,0.48,0.485,0.49,0.495,0.5,0.505,0.51,0.515,0.52,0.525,0.53,0.535,
0.54,0.545,0.55,0.555,0.56,0.565,0.57,0.575,0.58,0.585,0.59,0.595,0.6,0.605,
0.61,0.615,0.62,0.625,0.63,0.635,0.64,0.645,0.65,0.655,0.66,0.665,0.67,
0.675,0.68,0.685,0.690000000000001,0.695000000000001,0.700000000000001,
0.705000000000001,0.710000000000001,0.715000000000001,0.720000000000001,
0.725000000000001,0.730000000000001,0.735000000000001,0.740000000000001,
0.745000000000001,0.750000000000001,0.755000000000001,0.760000000000001,
0.765000000000001,0.770000000000001,0.775000000000001,0.780000000000001,
0.785000000000001,0.790000000000001,0.795000000000001,0.800000000000001,
0.805000000000001,0.810000000000001,0.815000000000001,0.820000000000001,
0.825000000000001,0.830000000000001,0.835000000000001,0.840000000000001,
0.845000000000001,0.850000000000001,0.855000000000001,0.860000000000001,
0.865000000000001,0.870000000000001,0.875000000000001,0.880000000000001,
0.885000000000001,0.890000000000001,0.895000000000001,0.900000000000001,
0.905000000000001,0.910000000000001,0.915000000000001,0.920000000000001,
0.925000000000001,0.930000000000001,0.935000000000001,0.940000000000001,
0.945000000000001,0.950000000000001,0.955000000000001,0.960000000000001,
0.965000000000001,0.970000000000001,0.975000000000001,0.980000000000001,
0.985000000000001,0.990000000000001,0.995000000000001,1.),.UNSPECIFIED.)
CURVE()
GEOMETRIC_REPRESENTATION_ITEM()
RATIONAL_B_SPLINE_CURVE((1.,1.,1.,1.,1.,1.,1.,1.,1.,1.,1.,1.,1.,1.,1.,1.,
1.,1.,1.,1.,1.,1.,1.,1.,1.,1.,1.,1.,1.,1.,1.,1.,1.,1.,1.,1.,1.,1.,1.,1.,
1.,1.,1.,1.,1.,1.,1.,1.,1.,1.,1.,1.,1.,1.,1.,1.,1.,1.,1.,1.,1.,1.,1.,1.,
1.,1.,1.,1.,1.,1.,1.,1.,1.,1.,1.,1.,1.,1.,1.,1.,1.,1.,1.,1.,1.,1.,1.,1.,
1.,1.,1.,1.,1.,1.,1.,1.,1.,1.,1.,1.,1.,1.,1.,1.,1.,1.,1.,1.,1.,1.,1.,1.,
1.,1.,1.,1.,1.,1.,1.,1.,1.,1.,1.,1.,1.,1.,1.,1.,1.,1.,1.,1.,1.,1.,1.,1.,
1.,1.,1.,1.,1.,1.,1.,1.,1.,1.,1.,1.,1.,1.,1.,1.,1.,1.,1.,1.,1.,1.,1.,1.,
1.,1.,1.,1.,1.,1.,1.,1.,1.,1.,1.,1.,1.,1.,1.,1.,1.,1.,1.,1.,1.,1.,1.,1.,
1.,1.,1.,1.,1.,1.,1.,1.,1.,1.,1.,1.,1.,1.,1.,1.,1.,1.,1.,1.,1.))
REPRESENTATION_ITEM('')
);
#821=(
BOUNDED_CURVE()
B_SPLINE_CURVE(5,(#230458,#230459,#230460,#230461,#230462,#230463,#230464,
#230465,#230466,#230467,#230468,#230469,#230470,#230471,#230472,#230473,
#230474,#230475,#230476,#230477,#230478,#230479,#230480,#230481,#230482,
#230483,#230484,#230485,#230486,#230487,#230488,#230489,#230490,#230491,
#230492,#230493,#230494,#230495,#230496,#230497,#230498,#230499,#230500,
#230501,#230502,#230503,#230504,#230505,#230506,#230507,#230508,#230509,
#230510,#230511,#230512,#230513,#230514,#230515,#230516,#230517,#230518,
#230519,#230520,#230521,#230522,#230523,#230524,#230525,#230526,#230527,
#230528,#230529,#230530,#230531,#230532,#230533,#230534,#230535,#230536,
#230537,#230538,#230539,#230540,#230541,#230542,#230543,#230544,#230545,
#230546,#230547,#230548,#230549,#230550,#230551,#230552,#230553,#230554,
#230555,#230556,#230557,#230558,#230559,#230560,#230561,#230562,#230563,
#230564,#230565,#230566,#230567,#230568,#230569,#230570,#230571,#230572,
#230573,#230574,#230575,#230576,#230577,#230578,#230579,#230580,#230581,
#230582,#230583,#230584,#230585,#230586,#230587,#230588,#230589,#230590,
#230591,#230592,#230593,#230594,#230595,#230596,#230597,#230598,#230599,
#230600,#230601,#230602,#230603,#230604,#230605,#230606,#230607,#230608,
#230609,#230610,#230611,#230612,#230613,#230614,#230615,#230616,#230617,
#230618,#230619,#230620,#230621,#230622,#230623,#230624,#230625,#230626,
#230627,#230628,#230629,#230630,#230631,#230632,#230633,#230634,#230635,
#230636,#230637,#230638,#230639,#230640,#230641,#230642,#230643,#230644,
#230645,#230646,#230647,#230648,#230649,#230650,#230651,#230652,#230653,
#230654,#230655,#230656,#230657,#230658,#230659,#230660,#230661,#230662),
 .UNSPECIFIED.,.F.,.F.)
B_SPLINE_CURVE_WITH_KNOTS((6,1,1,1,1,1,1,1,1,1,1,1,1,1,1,1,1,1,1,1,1,1,
1,1,1,1,1,1,1,1,1,1,1,1,1,1,1,1,1,1,1,1,1,1,1,1,1,1,1,1,1,1,1,1,1,1,1,1,
1,1,1,1,1,1,1,1,1,1,1,1,1,1,1,1,1,1,1,1,1,1,1,1,1,1,1,1,1,1,1,1,1,1,1,1,
1,1,1,1,1,1,1,1,1,1,1,1,1,1,1,1,1,1,1,1,1,1,1,1,1,1,1,1,1,1,1,1,1,1,1,1,
1,1,1,1,1,1,1,1,1,1,1,1,1,1,1,1,1,1,1,1,1,1,1,1,1,1,1,1,1,1,1,1,1,1,1,1,
1,1,1,1,1,1,1,1,1,1,1,1,1,1,1,1,1,1,1,1,1,1,1,1,1,1,1,1,1,1,1,1,1,1,6),
(0.,0.005,0.01,0.015,0.02,0.025,0.03,0.035,0.04,0.045,0.05,0.055,0.06,0.065,
0.07,0.075,0.08,0.085,0.09,0.095,0.1,0.105,0.11,0.115,0.12,0.125,0.13,0.135,
0.14,0.145,0.15,0.155,0.16,0.165,0.17,0.175,0.18,0.185,0.19,0.195,0.2,0.205,
0.21,0.215,0.22,0.225,0.23,0.235,0.24,0.245,0.25,0.255,0.26,0.265,0.27,
0.275,0.28,0.285,0.29,0.295,0.3,0.305,0.31,0.315,0.32,0.325,0.33,0.335,
0.34,0.345,0.35,0.355,0.36,0.365,0.37,0.375,0.38,0.385,0.39,0.395,0.4,0.405,
0.41,0.415,0.42,0.425,0.43,0.435,0.44,0.445,0.45,0.455,0.46,0.465,0.47,
0.475,0.48,0.485,0.49,0.495,0.5,0.505,0.51,0.515,0.52,0.525,0.53,0.535,
0.54,0.545,0.55,0.555,0.56,0.565,0.57,0.575,0.58,0.585,0.59,0.595,0.6,0.605,
0.61,0.615,0.62,0.625,0.63,0.635,0.64,0.645,0.65,0.655,0.66,0.665,0.67,
0.675,0.68,0.685,0.690000000000001,0.695000000000001,0.700000000000001,
0.705000000000001,0.710000000000001,0.715000000000001,0.720000000000001,
0.725000000000001,0.730000000000001,0.735000000000001,0.740000000000001,
0.745000000000001,0.750000000000001,0.755000000000001,0.760000000000001,
0.765000000000001,0.770000000000001,0.775000000000001,0.780000000000001,
0.785000000000001,0.790000000000001,0.795000000000001,0.800000000000001,
0.805000000000001,0.810000000000001,0.815000000000001,0.820000000000001,
0.825000000000001,0.830000000000001,0.835000000000001,0.840000000000001,
0.845000000000001,0.850000000000001,0.855000000000001,0.860000000000001,
0.865000000000001,0.870000000000001,0.875000000000001,0.880000000000001,
0.885000000000001,0.890000000000001,0.895000000000001,0.900000000000001,
0.905000000000001,0.910000000000001,0.915000000000001,0.920000000000001,
0.925000000000001,0.930000000000001,0.935000000000001,0.940000000000001,
0.945000000000001,0.950000000000001,0.955000000000001,0.960000000000001,
0.965000000000001,0.970000000000001,0.975000000000001,0.980000000000001,
0.985000000000001,0.990000000000001,0.995000000000001,1.),.UNSPECIFIED.)
CURVE()
GEOMETRIC_REPRESENTATION_ITEM()
RATIONAL_B_SPLINE_CURVE((1.,1.,1.,1.,1.,1.,1.,1.,1.,1.,1.,1.,1.,1.,1.,1.,
1.,1.,1.,1.,1.,1.,1.,1.,1.,1.,1.,1.,1.,1.,1.,1.,1.,1.,1.,1.,1.,1.,1.,1.,
1.,1.,1.,1.,1.,1.,1.,1.,1.,1.,1.,1.,1.,1.,1.,1.,1.,1.,1.,1.,1.,1.,1.,1.,
1.,1.,1.,1.,1.,1.,1.,1.,1.,1.,1.,1.,1.,1.,1.,1.,1.,1.,1.,1.,1.,1.,1.,1.,
1.,1.,1.,1.,1.,1.,1.,1.,1.,1.,1.,1.,1.,1.,1.,1.,1.,1.,1.,1.,1.,1.,1.,1.,
1.,1.,1.,1.,1.,1.,1.,1.,1.,1.,1.,1.,1.,1.,1.,1.,1.,1.,1.,1.,1.,1.,1.,1.,
1.,1.,1.,1.,1.,1.,1.,1.,1.,1.,1.,1.,1.,1.,1.,1.,1.,1.,1.,1.,1.,1.,1.,1.,
1.,1.,1.,1.,1.,1.,1.,1.,1.,1.,1.,1.,1.,1.,1.,1.,1.,1.,1.,1.,1.,1.,1.,1.,
1.,1.,1.,1.,1.,1.,1.,1.,1.,1.,1.,1.,1.,1.,1.,1.,1.,1.,1.,1.,1.))
REPRESENTATION_ITEM('')
);
#822=(
BOUNDED_CURVE()
B_SPLINE_CURVE(5,(#230664,#230665,#230666,#230667,#230668,#230669,#230670,
#230671,#230672,#230673,#230674,#230675,#230676,#230677,#230678,#230679,
#230680,#230681,#230682,#230683,#230684,#230685,#230686,#230687,#230688,
#230689,#230690,#230691,#230692,#230693,#230694,#230695,#230696,#230697,
#230698,#230699,#230700,#230701,#230702,#230703,#230704,#230705,#230706,
#230707,#230708,#230709,#230710,#230711,#230712,#230713,#230714,#230715,
#230716,#230717,#230718,#230719,#230720,#230721,#230722,#230723,#230724,
#230725,#230726,#230727,#230728,#230729,#230730,#230731,#230732,#230733,
#230734,#230735,#230736,#230737,#230738,#230739,#230740,#230741,#230742,
#230743,#230744,#230745,#230746,#230747,#230748,#230749,#230750,#230751,
#230752,#230753,#230754,#230755,#230756,#230757,#230758,#230759,#230760,
#230761,#230762,#230763,#230764,#230765,#230766,#230767,#230768,#230769,
#230770,#230771,#230772,#230773,#230774,#230775,#230776,#230777,#230778,
#230779,#230780,#230781,#230782,#230783,#230784,#230785,#230786,#230787,
#230788,#230789,#230790,#230791,#230792,#230793,#230794,#230795,#230796,
#230797,#230798,#230799,#230800,#230801,#230802,#230803,#230804,#230805,
#230806,#230807,#230808,#230809,#230810,#230811,#230812,#230813,#230814,
#230815,#230816,#230817,#230818,#230819,#230820,#230821,#230822,#230823,
#230824,#230825,#230826,#230827,#230828,#230829,#230830,#230831,#230832,
#230833,#230834,#230835,#230836,#230837,#230838,#230839,#230840,#230841,
#230842,#230843,#230844,#230845,#230846,#230847,#230848,#230849,#230850,
#230851,#230852,#230853,#230854,#230855,#230856,#230857,#230858,#230859,
#230860,#230861,#230862,#230863,#230864,#230865,#230866,#230867,#230868),
 .UNSPECIFIED.,.F.,.F.)
B_SPLINE_CURVE_WITH_KNOTS((6,1,1,1,1,1,1,1,1,1,1,1,1,1,1,1,1,1,1,1,1,1,
1,1,1,1,1,1,1,1,1,1,1,1,1,1,1,1,1,1,1,1,1,1,1,1,1,1,1,1,1,1,1,1,1,1,1,1,
1,1,1,1,1,1,1,1,1,1,1,1,1,1,1,1,1,1,1,1,1,1,1,1,1,1,1,1,1,1,1,1,1,1,1,1,
1,1,1,1,1,1,1,1,1,1,1,1,1,1,1,1,1,1,1,1,1,1,1,1,1,1,1,1,1,1,1,1,1,1,1,1,
1,1,1,1,1,1,1,1,1,1,1,1,1,1,1,1,1,1,1,1,1,1,1,1,1,1,1,1,1,1,1,1,1,1,1,1,
1,1,1,1,1,1,1,1,1,1,1,1,1,1,1,1,1,1,1,1,1,1,1,1,1,1,1,1,1,1,1,1,1,1,6),
(-1.,-0.995000000000001,-0.990000000000001,-0.985000000000001,-0.980000000000001,
-0.975000000000001,-0.970000000000001,-0.965000000000001,-0.960000000000001,
-0.955000000000001,-0.950000000000001,-0.945000000000001,-0.940000000000001,
-0.935000000000001,-0.930000000000001,-0.925000000000001,-0.920000000000001,
-0.915000000000001,-0.910000000000001,-0.905000000000001,-0.900000000000001,
-0.895000000000001,-0.890000000000001,-0.885000000000001,-0.880000000000001,
-0.875000000000001,-0.870000000000001,-0.865000000000001,-0.860000000000001,
-0.855000000000001,-0.850000000000001,-0.845000000000001,-0.840000000000001,
-0.835000000000001,-0.830000000000001,-0.825000000000001,-0.820000000000001,
-0.815000000000001,-0.810000000000001,-0.805000000000001,-0.800000000000001,
-0.795000000000001,-0.790000000000001,-0.785000000000001,-0.780000000000001,
-0.775000000000001,-0.770000000000001,-0.765000000000001,-0.760000000000001,
-0.755000000000001,-0.750000000000001,-0.745000000000001,-0.740000000000001,
-0.735000000000001,-0.730000000000001,-0.725000000000001,-0.720000000000001,
-0.715000000000001,-0.710000000000001,-0.705000000000001,-0.700000000000001,
-0.695000000000001,-0.690000000000001,-0.685,-0.68,-0.675,-0.67,-0.665,
-0.66,-0.655,-0.65,-0.645,-0.64,-0.635,-0.63,-0.625,-0.62,-0.615,-0.61,
-0.605,-0.6,-0.595,-0.59,-0.585,-0.58,-0.575,-0.57,-0.565,-0.56,-0.555,
-0.55,-0.545,-0.54,-0.535,-0.53,-0.525,-0.52,-0.515,-0.51,-0.505,-0.5,-0.495,
-0.49,-0.485,-0.48,-0.475,-0.47,-0.465,-0.46,-0.455,-0.45,-0.445,-0.44,
-0.435,-0.43,-0.425,-0.42,-0.415,-0.41,-0.405,-0.4,-0.395,-0.39,-0.385,
-0.38,-0.375,-0.37,-0.365,-0.36,-0.355,-0.35,-0.345,-0.34,-0.335,-0.33,
-0.325,-0.32,-0.315,-0.31,-0.305,-0.3,-0.295,-0.29,-0.285,-0.28,-0.275,
-0.27,-0.265,-0.26,-0.255,-0.25,-0.245,-0.24,-0.235,-0.23,-0.225,-0.22,
-0.215,-0.21,-0.205,-0.2,-0.195,-0.19,-0.185,-0.18,-0.175,-0.17,-0.165,
-0.16,-0.155,-0.15,-0.145,-0.14,-0.135,-0.13,-0.125,-0.12,-0.115,-0.11,
-0.105,-0.1,-0.095,-0.09,-0.085,-0.08,-0.075,-0.07,-0.065,-0.06,-0.055,
-0.05,-0.045,-0.04,-0.035,-0.03,-0.025,-0.02,-0.015,-0.01,-0.005,0.),
 .UNSPECIFIED.)
CURVE()
GEOMETRIC_REPRESENTATION_ITEM()
RATIONAL_B_SPLINE_CURVE((1.,1.,1.,1.,1.,1.,1.,1.,1.,1.,1.,1.,1.,1.,1.,1.,
1.,1.,1.,1.,1.,1.,1.,1.,1.,1.,1.,1.,1.,1.,1.,1.,1.,1.,1.,1.,1.,1.,1.,1.,
1.,1.,1.,1.,1.,1.,1.,1.,1.,1.,1.,1.,1.,1.,1.,1.,1.,1.,1.,1.,1.,1.,1.,1.,
1.,1.,1.,1.,1.,1.,1.,1.,1.,1.,1.,1.,1.,1.,1.,1.,1.,1.,1.,1.,1.,1.,1.,1.,
1.,1.,1.,1.,1.,1.,1.,1.,1.,1.,1.,1.,1.,1.,1.,1.,1.,1.,1.,1.,1.,1.,1.,1.,
1.,1.,1.,1.,1.,1.,1.,1.,1.,1.,1.,1.,1.,1.,1.,1.,1.,1.,1.,1.,1.,1.,1.,1.,
1.,1.,1.,1.,1.,1.,1.,1.,1.,1.,1.,1.,1.,1.,1.,1.,1.,1.,1.,1.,1.,1.,1.,1.,
1.,1.,1.,1.,1.,1.,1.,1.,1.,1.,1.,1.,1.,1.,1.,1.,1.,1.,1.,1.,1.,1.,1.,1.,
1.,1.,1.,1.,1.,1.,1.,1.,1.,1.,1.,1.,1.,1.,1.,1.,1.,1.,1.,1.,1.))
REPRESENTATION_ITEM('')
);
#823=(
BOUNDED_CURVE()
B_SPLINE_CURVE(5,(#231287,#231288,#231289,#231290,#231291,#231292,#231293,
#231294,#231295,#231296,#231297,#231298,#231299,#231300,#231301,#231302,
#231303,#231304,#231305,#231306,#231307,#231308,#231309,#231310,#231311,
#231312,#231313,#231314,#231315,#231316,#231317,#231318,#231319,#231320,
#231321,#231322,#231323,#231324,#231325,#231326,#231327,#231328,#231329,
#231330,#231331,#231332,#231333,#231334,#231335,#231336,#231337,#231338,
#231339,#231340,#231341,#231342,#231343,#231344,#231345,#231346,#231347,
#231348,#231349,#231350,#231351,#231352,#231353,#231354,#231355,#231356,
#231357,#231358,#231359,#231360,#231361,#231362,#231363,#231364,#231365,
#231366,#231367,#231368,#231369,#231370,#231371,#231372,#231373,#231374,
#231375,#231376,#231377,#231378,#231379,#231380,#231381,#231382,#231383,
#231384,#231385,#231386,#231387,#231388,#231389,#231390,#231391,#231392,
#231393,#231394,#231395,#231396,#231397,#231398,#231399,#231400,#231401,
#231402,#231403,#231404,#231405,#231406,#231407,#231408,#231409,#231410,
#231411,#231412,#231413,#231414,#231415,#231416,#231417,#231418,#231419,
#231420,#231421,#231422,#231423,#231424,#231425,#231426,#231427,#231428,
#231429,#231430,#231431,#231432,#231433,#231434,#231435,#231436,#231437,
#231438,#231439,#231440,#231441,#231442,#231443,#231444,#231445,#231446,
#231447,#231448,#231449,#231450,#231451,#231452,#231453,#231454,#231455,
#231456,#231457,#231458,#231459,#231460,#231461,#231462,#231463,#231464,
#231465,#231466,#231467,#231468,#231469,#231470,#231471,#231472,#231473,
#231474,#231475,#231476,#231477,#231478,#231479,#231480,#231481,#231482,
#231483,#231484,#231485,#231486,#231487,#231488,#231489,#231490,#231491),
 .UNSPECIFIED.,.F.,.F.)
B_SPLINE_CURVE_WITH_KNOTS((6,1,1,1,1,1,1,1,1,1,1,1,1,1,1,1,1,1,1,1,1,1,
1,1,1,1,1,1,1,1,1,1,1,1,1,1,1,1,1,1,1,1,1,1,1,1,1,1,1,1,1,1,1,1,1,1,1,1,
1,1,1,1,1,1,1,1,1,1,1,1,1,1,1,1,1,1,1,1,1,1,1,1,1,1,1,1,1,1,1,1,1,1,1,1,
1,1,1,1,1,1,1,1,1,1,1,1,1,1,1,1,1,1,1,1,1,1,1,1,1,1,1,1,1,1,1,1,1,1,1,1,
1,1,1,1,1,1,1,1,1,1,1,1,1,1,1,1,1,1,1,1,1,1,1,1,1,1,1,1,1,1,1,1,1,1,1,1,
1,1,1,1,1,1,1,1,1,1,1,1,1,1,1,1,1,1,1,1,1,1,1,1,1,1,1,1,1,1,1,1,1,1,6),
(-1.,-0.995000000000001,-0.990000000000001,-0.985000000000001,-0.980000000000001,
-0.975000000000001,-0.970000000000001,-0.965000000000001,-0.960000000000001,
-0.955000000000001,-0.950000000000001,-0.945000000000001,-0.940000000000001,
-0.935000000000001,-0.930000000000001,-0.925000000000001,-0.920000000000001,
-0.915000000000001,-0.910000000000001,-0.905000000000001,-0.900000000000001,
-0.895000000000001,-0.890000000000001,-0.885000000000001,-0.880000000000001,
-0.875000000000001,-0.870000000000001,-0.865000000000001,-0.860000000000001,
-0.855000000000001,-0.850000000000001,-0.845000000000001,-0.840000000000001,
-0.835000000000001,-0.830000000000001,-0.825000000000001,-0.820000000000001,
-0.815000000000001,-0.810000000000001,-0.805000000000001,-0.800000000000001,
-0.795000000000001,-0.790000000000001,-0.785000000000001,-0.780000000000001,
-0.775000000000001,-0.770000000000001,-0.765000000000001,-0.760000000000001,
-0.755000000000001,-0.750000000000001,-0.745000000000001,-0.740000000000001,
-0.735000000000001,-0.730000000000001,-0.725000000000001,-0.720000000000001,
-0.715000000000001,-0.710000000000001,-0.705000000000001,-0.700000000000001,
-0.695000000000001,-0.690000000000001,-0.685,-0.68,-0.675,-0.67,-0.665,
-0.66,-0.655,-0.65,-0.645,-0.64,-0.635,-0.63,-0.625,-0.62,-0.615,-0.61,
-0.605,-0.6,-0.595,-0.59,-0.585,-0.58,-0.575,-0.57,-0.565,-0.56,-0.555,
-0.55,-0.545,-0.54,-0.535,-0.53,-0.525,-0.52,-0.515,-0.51,-0.505,-0.5,-0.495,
-0.49,-0.485,-0.48,-0.475,-0.47,-0.465,-0.46,-0.455,-0.45,-0.445,-0.44,
-0.435,-0.43,-0.425,-0.42,-0.415,-0.41,-0.405,-0.4,-0.395,-0.39,-0.385,
-0.38,-0.375,-0.37,-0.365,-0.36,-0.355,-0.35,-0.345,-0.34,-0.335,-0.33,
-0.325,-0.32,-0.315,-0.31,-0.305,-0.3,-0.295,-0.29,-0.285,-0.28,-0.275,
-0.27,-0.265,-0.26,-0.255,-0.25,-0.245,-0.24,-0.235,-0.23,-0.225,-0.22,
-0.215,-0.21,-0.205,-0.2,-0.195,-0.19,-0.185,-0.18,-0.175,-0.17,-0.165,
-0.16,-0.155,-0.15,-0.145,-0.14,-0.135,-0.13,-0.125,-0.12,-0.115,-0.11,
-0.105,-0.1,-0.095,-0.09,-0.085,-0.08,-0.075,-0.07,-0.065,-0.06,-0.055,
-0.05,-0.045,-0.04,-0.035,-0.03,-0.025,-0.02,-0.015,-0.01,-0.005,0.),
 .UNSPECIFIED.)
CURVE()
GEOMETRIC_REPRESENTATION_ITEM()
RATIONAL_B_SPLINE_CURVE((1.,1.,1.,1.,1.,1.,1.,1.,1.,1.,1.,1.,1.,1.,1.,1.,
1.,1.,1.,1.,1.,1.,1.,1.,1.,1.,1.,1.,1.,1.,1.,1.,1.,1.,1.,1.,1.,1.,1.,1.,
1.,1.,1.,1.,1.,1.,1.,1.,1.,1.,1.,1.,1.,1.,1.,1.,1.,1.,1.,1.,1.,1.,1.,1.,
1.,1.,1.,1.,1.,1.,1.,1.,1.,1.,1.,1.,1.,1.,1.,1.,1.,1.,1.,1.,1.,1.,1.,1.,
1.,1.,1.,1.,1.,1.,1.,1.,1.,1.,1.,1.,1.,1.,1.,1.,1.,1.,1.,1.,1.,1.,1.,1.,
1.,1.,1.,1.,1.,1.,1.,1.,1.,1.,1.,1.,1.,1.,1.,1.,1.,1.,1.,1.,1.,1.,1.,1.,
1.,1.,1.,1.,1.,1.,1.,1.,1.,1.,1.,1.,1.,1.,1.,1.,1.,1.,1.,1.,1.,1.,1.,1.,
1.,1.,1.,1.,1.,1.,1.,1.,1.,1.,1.,1.,1.,1.,1.,1.,1.,1.,1.,1.,1.,1.,1.,1.,
1.,1.,1.,1.,1.,1.,1.,1.,1.,1.,1.,1.,1.,1.,1.,1.,1.,1.,1.,1.,1.))
REPRESENTATION_ITEM('')
);
#824=(
BOUNDED_CURVE()
B_SPLINE_CURVE(5,(#231494,#231495,#231496,#231497,#231498,#231499,#231500,
#231501,#231502,#231503,#231504,#231505,#231506,#231507,#231508,#231509,
#231510,#231511,#231512,#231513,#231514,#231515,#231516,#231517,#231518,
#231519,#231520,#231521,#231522,#231523,#231524,#231525,#231526,#231527,
#231528,#231529,#231530,#231531,#231532,#231533,#231534,#231535,#231536,
#231537,#231538,#231539,#231540,#231541,#231542,#231543,#231544,#231545,
#231546,#231547,#231548,#231549,#231550,#231551,#231552,#231553,#231554,
#231555,#231556,#231557,#231558,#231559,#231560,#231561,#231562,#231563,
#231564,#231565,#231566,#231567,#231568,#231569,#231570,#231571,#231572,
#231573,#231574,#231575,#231576,#231577,#231578,#231579,#231580,#231581,
#231582,#231583,#231584,#231585,#231586,#231587,#231588,#231589,#231590,
#231591,#231592,#231593,#231594,#231595,#231596,#231597,#231598,#231599,
#231600,#231601,#231602,#231603,#231604,#231605,#231606,#231607,#231608,
#231609,#231610,#231611,#231612,#231613,#231614,#231615,#231616,#231617,
#231618,#231619,#231620,#231621,#231622,#231623,#231624,#231625,#231626,
#231627,#231628,#231629,#231630,#231631,#231632,#231633,#231634,#231635,
#231636,#231637,#231638,#231639,#231640,#231641,#231642,#231643,#231644,
#231645,#231646,#231647,#231648,#231649,#231650,#231651,#231652,#231653,
#231654,#231655,#231656,#231657,#231658,#231659,#231660,#231661,#231662,
#231663,#231664,#231665,#231666,#231667,#231668,#231669,#231670,#231671,
#231672,#231673,#231674,#231675,#231676,#231677,#231678,#231679,#231680,
#231681,#231682,#231683,#231684,#231685,#231686,#231687,#231688,#231689,
#231690,#231691,#231692,#231693,#231694,#231695,#231696,#231697,#231698),
 .UNSPECIFIED.,.F.,.F.)
B_SPLINE_CURVE_WITH_KNOTS((6,1,1,1,1,1,1,1,1,1,1,1,1,1,1,1,1,1,1,1,1,1,
1,1,1,1,1,1,1,1,1,1,1,1,1,1,1,1,1,1,1,1,1,1,1,1,1,1,1,1,1,1,1,1,1,1,1,1,
1,1,1,1,1,1,1,1,1,1,1,1,1,1,1,1,1,1,1,1,1,1,1,1,1,1,1,1,1,1,1,1,1,1,1,1,
1,1,1,1,1,1,1,1,1,1,1,1,1,1,1,1,1,1,1,1,1,1,1,1,1,1,1,1,1,1,1,1,1,1,1,1,
1,1,1,1,1,1,1,1,1,1,1,1,1,1,1,1,1,1,1,1,1,1,1,1,1,1,1,1,1,1,1,1,1,1,1,1,
1,1,1,1,1,1,1,1,1,1,1,1,1,1,1,1,1,1,1,1,1,1,1,1,1,1,1,1,1,1,1,1,1,1,6),
(0.,0.005,0.01,0.015,0.02,0.025,0.03,0.035,0.04,0.045,0.05,0.055,0.06,0.065,
0.07,0.075,0.08,0.085,0.09,0.095,0.1,0.105,0.11,0.115,0.12,0.125,0.13,0.135,
0.14,0.145,0.15,0.155,0.16,0.165,0.17,0.175,0.18,0.185,0.19,0.195,0.2,0.205,
0.21,0.215,0.22,0.225,0.23,0.235,0.24,0.245,0.25,0.255,0.26,0.265,0.27,
0.275,0.28,0.285,0.29,0.295,0.3,0.305,0.31,0.315,0.32,0.325,0.33,0.335,
0.34,0.345,0.35,0.355,0.36,0.365,0.37,0.375,0.38,0.385,0.39,0.395,0.4,0.405,
0.41,0.415,0.42,0.425,0.43,0.435,0.44,0.445,0.45,0.455,0.46,0.465,0.47,
0.475,0.48,0.485,0.49,0.495,0.5,0.505,0.51,0.515,0.52,0.525,0.53,0.535,
0.54,0.545,0.55,0.555,0.56,0.565,0.57,0.575,0.58,0.585,0.59,0.595,0.6,0.605,
0.61,0.615,0.62,0.625,0.63,0.635,0.64,0.645,0.65,0.655,0.66,0.665,0.67,
0.675,0.68,0.685,0.690000000000001,0.695000000000001,0.700000000000001,
0.705000000000001,0.710000000000001,0.715000000000001,0.720000000000001,
0.725000000000001,0.730000000000001,0.735000000000001,0.740000000000001,
0.745000000000001,0.750000000000001,0.755000000000001,0.760000000000001,
0.765000000000001,0.770000000000001,0.775000000000001,0.780000000000001,
0.785000000000001,0.790000000000001,0.795000000000001,0.800000000000001,
0.805000000000001,0.810000000000001,0.815000000000001,0.820000000000001,
0.825000000000001,0.830000000000001,0.835000000000001,0.840000000000001,
0.845000000000001,0.850000000000001,0.855000000000001,0.860000000000001,
0.865000000000001,0.870000000000001,0.875000000000001,0.880000000000001,
0.885000000000001,0.890000000000001,0.895000000000001,0.900000000000001,
0.905000000000001,0.910000000000001,0.915000000000001,0.920000000000001,
0.925000000000001,0.930000000000001,0.935000000000001,0.940000000000001,
0.945000000000001,0.950000000000001,0.955000000000001,0.960000000000001,
0.965000000000001,0.970000000000001,0.975000000000001,0.980000000000001,
0.985000000000001,0.990000000000001,0.995000000000001,1.),.UNSPECIFIED.)
CURVE()
GEOMETRIC_REPRESENTATION_ITEM()
RATIONAL_B_SPLINE_CURVE((1.,1.,1.,1.,1.,1.,1.,1.,1.,1.,1.,1.,1.,1.,1.,1.,
1.,1.,1.,1.,1.,1.,1.,1.,1.,1.,1.,1.,1.,1.,1.,1.,1.,1.,1.,1.,1.,1.,1.,1.,
1.,1.,1.,1.,1.,1.,1.,1.,1.,1.,1.,1.,1.,1.,1.,1.,1.,1.,1.,1.,1.,1.,1.,1.,
1.,1.,1.,1.,1.,1.,1.,1.,1.,1.,1.,1.,1.,1.,1.,1.,1.,1.,1.,1.,1.,1.,1.,1.,
1.,1.,1.,1.,1.,1.,1.,1.,1.,1.,1.,1.,1.,1.,1.,1.,1.,1.,1.,1.,1.,1.,1.,1.,
1.,1.,1.,1.,1.,1.,1.,1.,1.,1.,1.,1.,1.,1.,1.,1.,1.,1.,1.,1.,1.,1.,1.,1.,
1.,1.,1.,1.,1.,1.,1.,1.,1.,1.,1.,1.,1.,1.,1.,1.,1.,1.,1.,1.,1.,1.,1.,1.,
1.,1.,1.,1.,1.,1.,1.,1.,1.,1.,1.,1.,1.,1.,1.,1.,1.,1.,1.,1.,1.,1.,1.,1.,
1.,1.,1.,1.,1.,1.,1.,1.,1.,1.,1.,1.,1.,1.,1.,1.,1.,1.,1.,1.,1.))
REPRESENTATION_ITEM('')
);
#825=(
BOUNDED_CURVE()
B_SPLINE_CURVE(5,(#232110,#232111,#232112,#232113,#232114,#232115,#232116,
#232117,#232118,#232119,#232120,#232121,#232122,#232123,#232124,#232125,
#232126,#232127,#232128,#232129,#232130,#232131,#232132,#232133,#232134,
#232135,#232136,#232137,#232138,#232139,#232140,#232141,#232142,#232143,
#232144,#232145,#232146,#232147,#232148,#232149,#232150,#232151,#232152,
#232153,#232154,#232155,#232156,#232157,#232158,#232159,#232160,#232161,
#232162,#232163,#232164,#232165,#232166,#232167,#232168,#232169,#232170,
#232171,#232172,#232173,#232174,#232175,#232176,#232177,#232178,#232179,
#232180,#232181,#232182,#232183,#232184,#232185,#232186,#232187,#232188,
#232189,#232190,#232191,#232192,#232193,#232194,#232195,#232196,#232197,
#232198,#232199,#232200,#232201,#232202,#232203,#232204,#232205,#232206,
#232207,#232208,#232209,#232210,#232211,#232212,#232213,#232214,#232215,
#232216,#232217,#232218,#232219,#232220,#232221,#232222,#232223,#232224,
#232225,#232226,#232227,#232228,#232229,#232230,#232231,#232232,#232233,
#232234,#232235,#232236,#232237,#232238,#232239,#232240,#232241,#232242,
#232243,#232244,#232245,#232246,#232247,#232248,#232249,#232250,#232251,
#232252,#232253,#232254,#232255,#232256,#232257,#232258,#232259,#232260,
#232261,#232262,#232263,#232264,#232265,#232266,#232267,#232268,#232269,
#232270,#232271,#232272,#232273,#232274,#232275,#232276,#232277,#232278,
#232279,#232280,#232281,#232282,#232283,#232284,#232285,#232286,#232287,
#232288,#232289,#232290,#232291,#232292,#232293,#232294,#232295,#232296,
#232297,#232298,#232299,#232300,#232301,#232302,#232303,#232304,#232305,
#232306,#232307,#232308,#232309,#232310,#232311,#232312,#232313,#232314),
 .UNSPECIFIED.,.F.,.F.)
B_SPLINE_CURVE_WITH_KNOTS((6,1,1,1,1,1,1,1,1,1,1,1,1,1,1,1,1,1,1,1,1,1,
1,1,1,1,1,1,1,1,1,1,1,1,1,1,1,1,1,1,1,1,1,1,1,1,1,1,1,1,1,1,1,1,1,1,1,1,
1,1,1,1,1,1,1,1,1,1,1,1,1,1,1,1,1,1,1,1,1,1,1,1,1,1,1,1,1,1,1,1,1,1,1,1,
1,1,1,1,1,1,1,1,1,1,1,1,1,1,1,1,1,1,1,1,1,1,1,1,1,1,1,1,1,1,1,1,1,1,1,1,
1,1,1,1,1,1,1,1,1,1,1,1,1,1,1,1,1,1,1,1,1,1,1,1,1,1,1,1,1,1,1,1,1,1,1,1,
1,1,1,1,1,1,1,1,1,1,1,1,1,1,1,1,1,1,1,1,1,1,1,1,1,1,1,1,1,1,1,1,1,1,6),
(0.,0.005,0.01,0.015,0.02,0.025,0.03,0.035,0.04,0.045,0.05,0.055,0.06,0.065,
0.07,0.075,0.08,0.085,0.09,0.095,0.1,0.105,0.11,0.115,0.12,0.125,0.13,0.135,
0.14,0.145,0.15,0.155,0.16,0.165,0.17,0.175,0.18,0.185,0.19,0.195,0.2,0.205,
0.21,0.215,0.22,0.225,0.23,0.235,0.24,0.245,0.25,0.255,0.26,0.265,0.27,
0.275,0.28,0.285,0.29,0.295,0.3,0.305,0.31,0.315,0.32,0.325,0.33,0.335,
0.34,0.345,0.35,0.355,0.36,0.365,0.37,0.375,0.38,0.385,0.39,0.395,0.4,0.405,
0.41,0.415,0.42,0.425,0.43,0.435,0.44,0.445,0.45,0.455,0.46,0.465,0.47,
0.475,0.48,0.485,0.49,0.495,0.5,0.505,0.51,0.515,0.52,0.525,0.53,0.535,
0.54,0.545,0.55,0.555,0.56,0.565,0.57,0.575,0.58,0.585,0.59,0.595,0.6,0.605,
0.61,0.615,0.62,0.625,0.63,0.635,0.64,0.645,0.65,0.655,0.66,0.665,0.67,
0.675,0.68,0.685,0.690000000000001,0.695000000000001,0.700000000000001,
0.705000000000001,0.710000000000001,0.715000000000001,0.720000000000001,
0.725000000000001,0.730000000000001,0.735000000000001,0.740000000000001,
0.745000000000001,0.750000000000001,0.755000000000001,0.760000000000001,
0.765000000000001,0.770000000000001,0.775000000000001,0.780000000000001,
0.785000000000001,0.790000000000001,0.795000000000001,0.800000000000001,
0.805000000000001,0.810000000000001,0.815000000000001,0.820000000000001,
0.825000000000001,0.830000000000001,0.835000000000001,0.840000000000001,
0.845000000000001,0.850000000000001,0.855000000000001,0.860000000000001,
0.865000000000001,0.870000000000001,0.875000000000001,0.880000000000001,
0.885000000000001,0.890000000000001,0.895000000000001,0.900000000000001,
0.905000000000001,0.910000000000001,0.915000000000001,0.920000000000001,
0.925000000000001,0.930000000000001,0.935000000000001,0.940000000000001,
0.945000000000001,0.950000000000001,0.955000000000001,0.960000000000001,
0.965000000000001,0.970000000000001,0.975000000000001,0.980000000000001,
0.985000000000001,0.990000000000001,0.995000000000001,1.),.UNSPECIFIED.)
CURVE()
GEOMETRIC_REPRESENTATION_ITEM()
RATIONAL_B_SPLINE_CURVE((1.,1.,1.,1.,1.,1.,1.,1.,1.,1.,1.,1.,1.,1.,1.,1.,
1.,1.,1.,1.,1.,1.,1.,1.,1.,1.,1.,1.,1.,1.,1.,1.,1.,1.,1.,1.,1.,1.,1.,1.,
1.,1.,1.,1.,1.,1.,1.,1.,1.,1.,1.,1.,1.,1.,1.,1.,1.,1.,1.,1.,1.,1.,1.,1.,
1.,1.,1.,1.,1.,1.,1.,1.,1.,1.,1.,1.,1.,1.,1.,1.,1.,1.,1.,1.,1.,1.,1.,1.,
1.,1.,1.,1.,1.,1.,1.,1.,1.,1.,1.,1.,1.,1.,1.,1.,1.,1.,1.,1.,1.,1.,1.,1.,
1.,1.,1.,1.,1.,1.,1.,1.,1.,1.,1.,1.,1.,1.,1.,1.,1.,1.,1.,1.,1.,1.,1.,1.,
1.,1.,1.,1.,1.,1.,1.,1.,1.,1.,1.,1.,1.,1.,1.,1.,1.,1.,1.,1.,1.,1.,1.,1.,
1.,1.,1.,1.,1.,1.,1.,1.,1.,1.,1.,1.,1.,1.,1.,1.,1.,1.,1.,1.,1.,1.,1.,1.,
1.,1.,1.,1.,1.,1.,1.,1.,1.,1.,1.,1.,1.,1.,1.,1.,1.,1.,1.,1.,1.))
REPRESENTATION_ITEM('')
);
#826=(
BOUNDED_CURVE()
B_SPLINE_CURVE(5,(#232316,#232317,#232318,#232319,#232320,#232321,#232322,
#232323,#232324,#232325,#232326,#232327,#232328,#232329,#232330,#232331,
#232332,#232333,#232334,#232335,#232336,#232337,#232338,#232339,#232340,
#232341,#232342,#232343,#232344,#232345,#232346,#232347,#232348,#232349,
#232350,#232351,#232352,#232353,#232354,#232355,#232356,#232357,#232358,
#232359,#232360,#232361,#232362,#232363,#232364,#232365,#232366,#232367,
#232368,#232369,#232370,#232371,#232372,#232373,#232374,#232375,#232376,
#232377,#232378,#232379,#232380,#232381,#232382,#232383,#232384,#232385,
#232386,#232387,#232388,#232389,#232390,#232391,#232392,#232393,#232394,
#232395,#232396,#232397,#232398,#232399,#232400,#232401,#232402,#232403,
#232404,#232405,#232406,#232407,#232408,#232409,#232410,#232411,#232412,
#232413,#232414,#232415,#232416,#232417,#232418,#232419,#232420,#232421,
#232422,#232423,#232424,#232425,#232426,#232427,#232428,#232429,#232430,
#232431,#232432,#232433,#232434,#232435,#232436,#232437,#232438,#232439,
#232440,#232441,#232442,#232443,#232444,#232445,#232446,#232447,#232448,
#232449,#232450,#232451,#232452,#232453,#232454,#232455,#232456,#232457,
#232458,#232459,#232460,#232461,#232462,#232463,#232464,#232465,#232466,
#232467,#232468,#232469,#232470,#232471,#232472,#232473,#232474,#232475,
#232476,#232477,#232478,#232479,#232480,#232481,#232482,#232483,#232484,
#232485,#232486,#232487,#232488,#232489,#232490,#232491,#232492,#232493,
#232494,#232495,#232496,#232497,#232498,#232499,#232500,#232501,#232502,
#232503,#232504,#232505,#232506,#232507,#232508,#232509,#232510,#232511,
#232512,#232513,#232514,#232515,#232516,#232517,#232518,#232519,#232520),
 .UNSPECIFIED.,.F.,.F.)
B_SPLINE_CURVE_WITH_KNOTS((6,1,1,1,1,1,1,1,1,1,1,1,1,1,1,1,1,1,1,1,1,1,
1,1,1,1,1,1,1,1,1,1,1,1,1,1,1,1,1,1,1,1,1,1,1,1,1,1,1,1,1,1,1,1,1,1,1,1,
1,1,1,1,1,1,1,1,1,1,1,1,1,1,1,1,1,1,1,1,1,1,1,1,1,1,1,1,1,1,1,1,1,1,1,1,
1,1,1,1,1,1,1,1,1,1,1,1,1,1,1,1,1,1,1,1,1,1,1,1,1,1,1,1,1,1,1,1,1,1,1,1,
1,1,1,1,1,1,1,1,1,1,1,1,1,1,1,1,1,1,1,1,1,1,1,1,1,1,1,1,1,1,1,1,1,1,1,1,
1,1,1,1,1,1,1,1,1,1,1,1,1,1,1,1,1,1,1,1,1,1,1,1,1,1,1,1,1,1,1,1,1,1,6),
(-1.,-0.995000000000001,-0.990000000000001,-0.985000000000001,-0.980000000000001,
-0.975000000000001,-0.970000000000001,-0.965000000000001,-0.960000000000001,
-0.955000000000001,-0.950000000000001,-0.945000000000001,-0.940000000000001,
-0.935000000000001,-0.930000000000001,-0.925000000000001,-0.920000000000001,
-0.915000000000001,-0.910000000000001,-0.905000000000001,-0.900000000000001,
-0.895000000000001,-0.890000000000001,-0.885000000000001,-0.880000000000001,
-0.875000000000001,-0.870000000000001,-0.865000000000001,-0.860000000000001,
-0.855000000000001,-0.850000000000001,-0.845000000000001,-0.840000000000001,
-0.835000000000001,-0.830000000000001,-0.825000000000001,-0.820000000000001,
-0.815000000000001,-0.810000000000001,-0.805000000000001,-0.800000000000001,
-0.795000000000001,-0.790000000000001,-0.785000000000001,-0.780000000000001,
-0.775000000000001,-0.770000000000001,-0.765000000000001,-0.760000000000001,
-0.755000000000001,-0.750000000000001,-0.745000000000001,-0.740000000000001,
-0.735000000000001,-0.730000000000001,-0.725000000000001,-0.720000000000001,
-0.715000000000001,-0.710000000000001,-0.705000000000001,-0.700000000000001,
-0.695000000000001,-0.690000000000001,-0.685,-0.68,-0.675,-0.67,-0.665,
-0.66,-0.655,-0.65,-0.645,-0.64,-0.635,-0.63,-0.625,-0.62,-0.615,-0.61,
-0.605,-0.6,-0.595,-0.59,-0.585,-0.58,-0.575,-0.57,-0.565,-0.56,-0.555,
-0.55,-0.545,-0.54,-0.535,-0.53,-0.525,-0.52,-0.515,-0.51,-0.505,-0.5,-0.495,
-0.49,-0.485,-0.48,-0.475,-0.47,-0.465,-0.46,-0.455,-0.45,-0.445,-0.44,
-0.435,-0.43,-0.425,-0.42,-0.415,-0.41,-0.405,-0.4,-0.395,-0.39,-0.385,
-0.38,-0.375,-0.37,-0.365,-0.36,-0.355,-0.35,-0.345,-0.34,-0.335,-0.33,
-0.325,-0.32,-0.315,-0.31,-0.305,-0.3,-0.295,-0.29,-0.285,-0.28,-0.275,
-0.27,-0.265,-0.26,-0.255,-0.25,-0.245,-0.24,-0.235,-0.23,-0.225,-0.22,
-0.215,-0.21,-0.205,-0.2,-0.195,-0.19,-0.185,-0.18,-0.175,-0.17,-0.165,
-0.16,-0.155,-0.15,-0.145,-0.14,-0.135,-0.13,-0.125,-0.12,-0.115,-0.11,
-0.105,-0.1,-0.095,-0.09,-0.085,-0.08,-0.075,-0.07,-0.065,-0.06,-0.055,
-0.05,-0.045,-0.04,-0.035,-0.03,-0.025,-0.02,-0.015,-0.01,-0.005,0.),
 .UNSPECIFIED.)
CURVE()
GEOMETRIC_REPRESENTATION_ITEM()
RATIONAL_B_SPLINE_CURVE((1.,1.,1.,1.,1.,1.,1.,1.,1.,1.,1.,1.,1.,1.,1.,1.,
1.,1.,1.,1.,1.,1.,1.,1.,1.,1.,1.,1.,1.,1.,1.,1.,1.,1.,1.,1.,1.,1.,1.,1.,
1.,1.,1.,1.,1.,1.,1.,1.,1.,1.,1.,1.,1.,1.,1.,1.,1.,1.,1.,1.,1.,1.,1.,1.,
1.,1.,1.,1.,1.,1.,1.,1.,1.,1.,1.,1.,1.,1.,1.,1.,1.,1.,1.,1.,1.,1.,1.,1.,
1.,1.,1.,1.,1.,1.,1.,1.,1.,1.,1.,1.,1.,1.,1.,1.,1.,1.,1.,1.,1.,1.,1.,1.,
1.,1.,1.,1.,1.,1.,1.,1.,1.,1.,1.,1.,1.,1.,1.,1.,1.,1.,1.,1.,1.,1.,1.,1.,
1.,1.,1.,1.,1.,1.,1.,1.,1.,1.,1.,1.,1.,1.,1.,1.,1.,1.,1.,1.,1.,1.,1.,1.,
1.,1.,1.,1.,1.,1.,1.,1.,1.,1.,1.,1.,1.,1.,1.,1.,1.,1.,1.,1.,1.,1.,1.,1.,
1.,1.,1.,1.,1.,1.,1.,1.,1.,1.,1.,1.,1.,1.,1.,1.,1.,1.,1.,1.,1.))
REPRESENTATION_ITEM('')
);
#827=(
BOUNDED_CURVE()
B_SPLINE_CURVE(5,(#232939,#232940,#232941,#232942,#232943,#232944,#232945,
#232946,#232947,#232948,#232949,#232950,#232951,#232952,#232953,#232954,
#232955,#232956,#232957,#232958,#232959,#232960,#232961,#232962,#232963,
#232964,#232965,#232966,#232967,#232968,#232969,#232970,#232971,#232972,
#232973,#232974,#232975,#232976,#232977,#232978,#232979,#232980,#232981,
#232982,#232983,#232984,#232985,#232986,#232987,#232988,#232989,#232990,
#232991,#232992,#232993,#232994,#232995,#232996,#232997,#232998,#232999,
#233000,#233001,#233002,#233003,#233004,#233005,#233006,#233007,#233008,
#233009,#233010,#233011,#233012,#233013,#233014,#233015,#233016,#233017,
#233018,#233019,#233020,#233021,#233022,#233023,#233024,#233025,#233026,
#233027,#233028,#233029,#233030,#233031,#233032,#233033,#233034,#233035,
#233036,#233037,#233038,#233039,#233040,#233041,#233042,#233043,#233044,
#233045,#233046,#233047,#233048,#233049,#233050,#233051,#233052,#233053,
#233054,#233055,#233056,#233057,#233058,#233059,#233060,#233061,#233062,
#233063,#233064,#233065,#233066,#233067,#233068,#233069,#233070,#233071,
#233072,#233073,#233074,#233075,#233076,#233077,#233078,#233079,#233080,
#233081,#233082,#233083,#233084,#233085,#233086,#233087,#233088,#233089,
#233090,#233091,#233092,#233093,#233094,#233095,#233096,#233097,#233098,
#233099,#233100,#233101,#233102,#233103,#233104,#233105,#233106,#233107,
#233108,#233109,#233110,#233111,#233112,#233113,#233114,#233115,#233116,
#233117,#233118,#233119,#233120,#233121,#233122,#233123,#233124,#233125,
#233126,#233127,#233128,#233129,#233130,#233131,#233132,#233133,#233134,
#233135,#233136,#233137,#233138,#233139,#233140,#233141,#233142,#233143),
 .UNSPECIFIED.,.F.,.F.)
B_SPLINE_CURVE_WITH_KNOTS((6,1,1,1,1,1,1,1,1,1,1,1,1,1,1,1,1,1,1,1,1,1,
1,1,1,1,1,1,1,1,1,1,1,1,1,1,1,1,1,1,1,1,1,1,1,1,1,1,1,1,1,1,1,1,1,1,1,1,
1,1,1,1,1,1,1,1,1,1,1,1,1,1,1,1,1,1,1,1,1,1,1,1,1,1,1,1,1,1,1,1,1,1,1,1,
1,1,1,1,1,1,1,1,1,1,1,1,1,1,1,1,1,1,1,1,1,1,1,1,1,1,1,1,1,1,1,1,1,1,1,1,
1,1,1,1,1,1,1,1,1,1,1,1,1,1,1,1,1,1,1,1,1,1,1,1,1,1,1,1,1,1,1,1,1,1,1,1,
1,1,1,1,1,1,1,1,1,1,1,1,1,1,1,1,1,1,1,1,1,1,1,1,1,1,1,1,1,1,1,1,1,1,6),
(-1.,-0.995000000000001,-0.990000000000001,-0.985000000000001,-0.980000000000001,
-0.975000000000001,-0.970000000000001,-0.965000000000001,-0.960000000000001,
-0.955000000000001,-0.950000000000001,-0.945000000000001,-0.940000000000001,
-0.935000000000001,-0.930000000000001,-0.925000000000001,-0.920000000000001,
-0.915000000000001,-0.910000000000001,-0.905000000000001,-0.900000000000001,
-0.895000000000001,-0.890000000000001,-0.885000000000001,-0.880000000000001,
-0.875000000000001,-0.870000000000001,-0.865000000000001,-0.860000000000001,
-0.855000000000001,-0.850000000000001,-0.845000000000001,-0.840000000000001,
-0.835000000000001,-0.830000000000001,-0.825000000000001,-0.820000000000001,
-0.815000000000001,-0.810000000000001,-0.805000000000001,-0.800000000000001,
-0.795000000000001,-0.790000000000001,-0.785000000000001,-0.780000000000001,
-0.775000000000001,-0.770000000000001,-0.765000000000001,-0.760000000000001,
-0.755000000000001,-0.750000000000001,-0.745000000000001,-0.740000000000001,
-0.735000000000001,-0.730000000000001,-0.725000000000001,-0.720000000000001,
-0.715000000000001,-0.710000000000001,-0.705000000000001,-0.700000000000001,
-0.695000000000001,-0.690000000000001,-0.685,-0.68,-0.675,-0.67,-0.665,
-0.66,-0.655,-0.65,-0.645,-0.64,-0.635,-0.63,-0.625,-0.62,-0.615,-0.61,
-0.605,-0.6,-0.595,-0.59,-0.585,-0.58,-0.575,-0.57,-0.565,-0.56,-0.555,
-0.55,-0.545,-0.54,-0.535,-0.53,-0.525,-0.52,-0.515,-0.51,-0.505,-0.5,-0.495,
-0.49,-0.485,-0.48,-0.475,-0.47,-0.465,-0.46,-0.455,-0.45,-0.445,-0.44,
-0.435,-0.43,-0.425,-0.42,-0.415,-0.41,-0.405,-0.4,-0.395,-0.39,-0.385,
-0.38,-0.375,-0.37,-0.365,-0.36,-0.355,-0.35,-0.345,-0.34,-0.335,-0.33,
-0.325,-0.32,-0.315,-0.31,-0.305,-0.3,-0.295,-0.29,-0.285,-0.28,-0.275,
-0.27,-0.265,-0.26,-0.255,-0.25,-0.245,-0.24,-0.235,-0.23,-0.225,-0.22,
-0.215,-0.21,-0.205,-0.2,-0.195,-0.19,-0.185,-0.18,-0.175,-0.17,-0.165,
-0.16,-0.155,-0.15,-0.145,-0.14,-0.135,-0.13,-0.125,-0.12,-0.115,-0.11,
-0.105,-0.1,-0.095,-0.09,-0.085,-0.08,-0.075,-0.07,-0.065,-0.06,-0.055,
-0.05,-0.045,-0.04,-0.035,-0.03,-0.025,-0.02,-0.015,-0.01,-0.005,0.),
 .UNSPECIFIED.)
CURVE()
GEOMETRIC_REPRESENTATION_ITEM()
RATIONAL_B_SPLINE_CURVE((1.,1.,1.,1.,1.,1.,1.,1.,1.,1.,1.,1.,1.,1.,1.,1.,
1.,1.,1.,1.,1.,1.,1.,1.,1.,1.,1.,1.,1.,1.,1.,1.,1.,1.,1.,1.,1.,1.,1.,1.,
1.,1.,1.,1.,1.,1.,1.,1.,1.,1.,1.,1.,1.,1.,1.,1.,1.,1.,1.,1.,1.,1.,1.,1.,
1.,1.,1.,1.,1.,1.,1.,1.,1.,1.,1.,1.,1.,1.,1.,1.,1.,1.,1.,1.,1.,1.,1.,1.,
1.,1.,1.,1.,1.,1.,1.,1.,1.,1.,1.,1.,1.,1.,1.,1.,1.,1.,1.,1.,1.,1.,1.,1.,
1.,1.,1.,1.,1.,1.,1.,1.,1.,1.,1.,1.,1.,1.,1.,1.,1.,1.,1.,1.,1.,1.,1.,1.,
1.,1.,1.,1.,1.,1.,1.,1.,1.,1.,1.,1.,1.,1.,1.,1.,1.,1.,1.,1.,1.,1.,1.,1.,
1.,1.,1.,1.,1.,1.,1.,1.,1.,1.,1.,1.,1.,1.,1.,1.,1.,1.,1.,1.,1.,1.,1.,1.,
1.,1.,1.,1.,1.,1.,1.,1.,1.,1.,1.,1.,1.,1.,1.,1.,1.,1.,1.,1.,1.))
REPRESENTATION_ITEM('')
);
#828=(
BOUNDED_CURVE()
B_SPLINE_CURVE(5,(#233146,#233147,#233148,#233149,#233150,#233151,#233152,
#233153,#233154,#233155,#233156,#233157,#233158,#233159,#233160,#233161,
#233162,#233163,#233164,#233165,#233166,#233167,#233168,#233169,#233170,
#233171,#233172,#233173,#233174,#233175,#233176,#233177,#233178,#233179,
#233180,#233181,#233182,#233183,#233184,#233185,#233186,#233187,#233188,
#233189,#233190,#233191,#233192,#233193,#233194,#233195,#233196,#233197,
#233198,#233199,#233200,#233201,#233202,#233203,#233204,#233205,#233206,
#233207,#233208,#233209,#233210,#233211,#233212,#233213,#233214,#233215,
#233216,#233217,#233218,#233219,#233220,#233221,#233222,#233223,#233224,
#233225,#233226,#233227,#233228,#233229,#233230,#233231,#233232,#233233,
#233234,#233235,#233236,#233237,#233238,#233239,#233240,#233241,#233242,
#233243,#233244,#233245,#233246,#233247,#233248,#233249,#233250,#233251,
#233252,#233253,#233254,#233255,#233256,#233257,#233258,#233259,#233260,
#233261,#233262,#233263,#233264,#233265,#233266,#233267,#233268,#233269,
#233270,#233271,#233272,#233273,#233274,#233275,#233276,#233277,#233278,
#233279,#233280,#233281,#233282,#233283,#233284,#233285,#233286,#233287,
#233288,#233289,#233290,#233291,#233292,#233293,#233294,#233295,#233296,
#233297,#233298,#233299,#233300,#233301,#233302,#233303,#233304,#233305,
#233306,#233307,#233308,#233309,#233310,#233311,#233312,#233313,#233314,
#233315,#233316,#233317,#233318,#233319,#233320,#233321,#233322,#233323,
#233324,#233325,#233326,#233327,#233328,#233329,#233330,#233331,#233332,
#233333,#233334,#233335,#233336,#233337,#233338,#233339,#233340,#233341,
#233342,#233343,#233344,#233345,#233346,#233347,#233348,#233349,#233350),
 .UNSPECIFIED.,.F.,.F.)
B_SPLINE_CURVE_WITH_KNOTS((6,1,1,1,1,1,1,1,1,1,1,1,1,1,1,1,1,1,1,1,1,1,
1,1,1,1,1,1,1,1,1,1,1,1,1,1,1,1,1,1,1,1,1,1,1,1,1,1,1,1,1,1,1,1,1,1,1,1,
1,1,1,1,1,1,1,1,1,1,1,1,1,1,1,1,1,1,1,1,1,1,1,1,1,1,1,1,1,1,1,1,1,1,1,1,
1,1,1,1,1,1,1,1,1,1,1,1,1,1,1,1,1,1,1,1,1,1,1,1,1,1,1,1,1,1,1,1,1,1,1,1,
1,1,1,1,1,1,1,1,1,1,1,1,1,1,1,1,1,1,1,1,1,1,1,1,1,1,1,1,1,1,1,1,1,1,1,1,
1,1,1,1,1,1,1,1,1,1,1,1,1,1,1,1,1,1,1,1,1,1,1,1,1,1,1,1,1,1,1,1,1,1,6),
(0.,0.005,0.01,0.015,0.02,0.025,0.03,0.035,0.04,0.045,0.05,0.055,0.06,0.065,
0.07,0.075,0.08,0.085,0.09,0.095,0.1,0.105,0.11,0.115,0.12,0.125,0.13,0.135,
0.14,0.145,0.15,0.155,0.16,0.165,0.17,0.175,0.18,0.185,0.19,0.195,0.2,0.205,
0.21,0.215,0.22,0.225,0.23,0.235,0.24,0.245,0.25,0.255,0.26,0.265,0.27,
0.275,0.28,0.285,0.29,0.295,0.3,0.305,0.31,0.315,0.32,0.325,0.33,0.335,
0.34,0.345,0.35,0.355,0.36,0.365,0.37,0.375,0.38,0.385,0.39,0.395,0.4,0.405,
0.41,0.415,0.42,0.425,0.43,0.435,0.44,0.445,0.45,0.455,0.46,0.465,0.47,
0.475,0.48,0.485,0.49,0.495,0.5,0.505,0.51,0.515,0.52,0.525,0.53,0.535,
0.54,0.545,0.55,0.555,0.56,0.565,0.57,0.575,0.58,0.585,0.59,0.595,0.6,0.605,
0.61,0.615,0.62,0.625,0.63,0.635,0.64,0.645,0.65,0.655,0.66,0.665,0.67,
0.675,0.68,0.685,0.690000000000001,0.695000000000001,0.700000000000001,
0.705000000000001,0.710000000000001,0.715000000000001,0.720000000000001,
0.725000000000001,0.730000000000001,0.735000000000001,0.740000000000001,
0.745000000000001,0.750000000000001,0.755000000000001,0.760000000000001,
0.765000000000001,0.770000000000001,0.775000000000001,0.780000000000001,
0.785000000000001,0.790000000000001,0.795000000000001,0.800000000000001,
0.805000000000001,0.810000000000001,0.815000000000001,0.820000000000001,
0.825000000000001,0.830000000000001,0.835000000000001,0.840000000000001,
0.845000000000001,0.850000000000001,0.855000000000001,0.860000000000001,
0.865000000000001,0.870000000000001,0.875000000000001,0.880000000000001,
0.885000000000001,0.890000000000001,0.895000000000001,0.900000000000001,
0.905000000000001,0.910000000000001,0.915000000000001,0.920000000000001,
0.925000000000001,0.930000000000001,0.935000000000001,0.940000000000001,
0.945000000000001,0.950000000000001,0.955000000000001,0.960000000000001,
0.965000000000001,0.970000000000001,0.975000000000001,0.980000000000001,
0.985000000000001,0.990000000000001,0.995000000000001,1.),.UNSPECIFIED.)
CURVE()
GEOMETRIC_REPRESENTATION_ITEM()
RATIONAL_B_SPLINE_CURVE((1.,1.,1.,1.,1.,1.,1.,1.,1.,1.,1.,1.,1.,1.,1.,1.,
1.,1.,1.,1.,1.,1.,1.,1.,1.,1.,1.,1.,1.,1.,1.,1.,1.,1.,1.,1.,1.,1.,1.,1.,
1.,1.,1.,1.,1.,1.,1.,1.,1.,1.,1.,1.,1.,1.,1.,1.,1.,1.,1.,1.,1.,1.,1.,1.,
1.,1.,1.,1.,1.,1.,1.,1.,1.,1.,1.,1.,1.,1.,1.,1.,1.,1.,1.,1.,1.,1.,1.,1.,
1.,1.,1.,1.,1.,1.,1.,1.,1.,1.,1.,1.,1.,1.,1.,1.,1.,1.,1.,1.,1.,1.,1.,1.,
1.,1.,1.,1.,1.,1.,1.,1.,1.,1.,1.,1.,1.,1.,1.,1.,1.,1.,1.,1.,1.,1.,1.,1.,
1.,1.,1.,1.,1.,1.,1.,1.,1.,1.,1.,1.,1.,1.,1.,1.,1.,1.,1.,1.,1.,1.,1.,1.,
1.,1.,1.,1.,1.,1.,1.,1.,1.,1.,1.,1.,1.,1.,1.,1.,1.,1.,1.,1.,1.,1.,1.,1.,
1.,1.,1.,1.,1.,1.,1.,1.,1.,1.,1.,1.,1.,1.,1.,1.,1.,1.,1.,1.,1.))
REPRESENTATION_ITEM('')
);
#829=(
BOUNDED_CURVE()
B_SPLINE_CURVE(5,(#233762,#233763,#233764,#233765,#233766,#233767,#233768,
#233769,#233770,#233771,#233772,#233773,#233774,#233775,#233776,#233777,
#233778,#233779,#233780,#233781,#233782,#233783,#233784,#233785,#233786,
#233787,#233788,#233789,#233790,#233791,#233792,#233793,#233794,#233795,
#233796,#233797,#233798,#233799,#233800,#233801,#233802,#233803,#233804,
#233805,#233806,#233807,#233808,#233809,#233810,#233811,#233812,#233813,
#233814,#233815,#233816,#233817,#233818,#233819,#233820,#233821,#233822,
#233823,#233824,#233825,#233826,#233827,#233828,#233829,#233830,#233831,
#233832,#233833,#233834,#233835,#233836,#233837,#233838,#233839,#233840,
#233841,#233842,#233843,#233844,#233845,#233846,#233847,#233848,#233849,
#233850,#233851,#233852,#233853,#233854,#233855,#233856,#233857,#233858,
#233859,#233860,#233861,#233862,#233863,#233864,#233865,#233866,#233867,
#233868,#233869,#233870,#233871,#233872,#233873,#233874,#233875,#233876,
#233877,#233878,#233879,#233880,#233881,#233882,#233883,#233884,#233885,
#233886,#233887,#233888,#233889,#233890,#233891,#233892,#233893,#233894,
#233895,#233896,#233897,#233898,#233899,#233900,#233901,#233902,#233903,
#233904,#233905,#233906,#233907,#233908,#233909,#233910,#233911,#233912,
#233913,#233914,#233915,#233916,#233917,#233918,#233919,#233920,#233921,
#233922,#233923,#233924,#233925,#233926,#233927,#233928,#233929,#233930,
#233931,#233932,#233933,#233934,#233935,#233936,#233937,#233938,#233939,
#233940,#233941,#233942,#233943,#233944,#233945,#233946,#233947,#233948,
#233949,#233950,#233951,#233952,#233953,#233954,#233955,#233956,#233957,
#233958,#233959,#233960,#233961,#233962,#233963,#233964,#233965,#233966),
 .UNSPECIFIED.,.F.,.F.)
B_SPLINE_CURVE_WITH_KNOTS((6,1,1,1,1,1,1,1,1,1,1,1,1,1,1,1,1,1,1,1,1,1,
1,1,1,1,1,1,1,1,1,1,1,1,1,1,1,1,1,1,1,1,1,1,1,1,1,1,1,1,1,1,1,1,1,1,1,1,
1,1,1,1,1,1,1,1,1,1,1,1,1,1,1,1,1,1,1,1,1,1,1,1,1,1,1,1,1,1,1,1,1,1,1,1,
1,1,1,1,1,1,1,1,1,1,1,1,1,1,1,1,1,1,1,1,1,1,1,1,1,1,1,1,1,1,1,1,1,1,1,1,
1,1,1,1,1,1,1,1,1,1,1,1,1,1,1,1,1,1,1,1,1,1,1,1,1,1,1,1,1,1,1,1,1,1,1,1,
1,1,1,1,1,1,1,1,1,1,1,1,1,1,1,1,1,1,1,1,1,1,1,1,1,1,1,1,1,1,1,1,1,1,6),
(0.,0.005,0.01,0.015,0.02,0.025,0.03,0.035,0.04,0.045,0.05,0.055,0.06,0.065,
0.07,0.075,0.08,0.085,0.09,0.095,0.1,0.105,0.11,0.115,0.12,0.125,0.13,0.135,
0.14,0.145,0.15,0.155,0.16,0.165,0.17,0.175,0.18,0.185,0.19,0.195,0.2,0.205,
0.21,0.215,0.22,0.225,0.23,0.235,0.24,0.245,0.25,0.255,0.26,0.265,0.27,
0.275,0.28,0.285,0.29,0.295,0.3,0.305,0.31,0.315,0.32,0.325,0.33,0.335,
0.34,0.345,0.35,0.355,0.36,0.365,0.37,0.375,0.38,0.385,0.39,0.395,0.4,0.405,
0.41,0.415,0.42,0.425,0.43,0.435,0.44,0.445,0.45,0.455,0.46,0.465,0.47,
0.475,0.48,0.485,0.49,0.495,0.5,0.505,0.51,0.515,0.52,0.525,0.53,0.535,
0.54,0.545,0.55,0.555,0.56,0.565,0.57,0.575,0.58,0.585,0.59,0.595,0.6,0.605,
0.61,0.615,0.62,0.625,0.63,0.635,0.64,0.645,0.65,0.655,0.66,0.665,0.67,
0.675,0.68,0.685,0.690000000000001,0.695000000000001,0.700000000000001,
0.705000000000001,0.710000000000001,0.715000000000001,0.720000000000001,
0.725000000000001,0.730000000000001,0.735000000000001,0.740000000000001,
0.745000000000001,0.750000000000001,0.755000000000001,0.760000000000001,
0.765000000000001,0.770000000000001,0.775000000000001,0.780000000000001,
0.785000000000001,0.790000000000001,0.795000000000001,0.800000000000001,
0.805000000000001,0.810000000000001,0.815000000000001,0.820000000000001,
0.825000000000001,0.830000000000001,0.835000000000001,0.840000000000001,
0.845000000000001,0.850000000000001,0.855000000000001,0.860000000000001,
0.865000000000001,0.870000000000001,0.875000000000001,0.880000000000001,
0.885000000000001,0.890000000000001,0.895000000000001,0.900000000000001,
0.905000000000001,0.910000000000001,0.915000000000001,0.920000000000001,
0.925000000000001,0.930000000000001,0.935000000000001,0.940000000000001,
0.945000000000001,0.950000000000001,0.955000000000001,0.960000000000001,
0.965000000000001,0.970000000000001,0.975000000000001,0.980000000000001,
0.985000000000001,0.990000000000001,0.995000000000001,1.),.UNSPECIFIED.)
CURVE()
GEOMETRIC_REPRESENTATION_ITEM()
RATIONAL_B_SPLINE_CURVE((1.,1.,1.,1.,1.,1.,1.,1.,1.,1.,1.,1.,1.,1.,1.,1.,
1.,1.,1.,1.,1.,1.,1.,1.,1.,1.,1.,1.,1.,1.,1.,1.,1.,1.,1.,1.,1.,1.,1.,1.,
1.,1.,1.,1.,1.,1.,1.,1.,1.,1.,1.,1.,1.,1.,1.,1.,1.,1.,1.,1.,1.,1.,1.,1.,
1.,1.,1.,1.,1.,1.,1.,1.,1.,1.,1.,1.,1.,1.,1.,1.,1.,1.,1.,1.,1.,1.,1.,1.,
1.,1.,1.,1.,1.,1.,1.,1.,1.,1.,1.,1.,1.,1.,1.,1.,1.,1.,1.,1.,1.,1.,1.,1.,
1.,1.,1.,1.,1.,1.,1.,1.,1.,1.,1.,1.,1.,1.,1.,1.,1.,1.,1.,1.,1.,1.,1.,1.,
1.,1.,1.,1.,1.,1.,1.,1.,1.,1.,1.,1.,1.,1.,1.,1.,1.,1.,1.,1.,1.,1.,1.,1.,
1.,1.,1.,1.,1.,1.,1.,1.,1.,1.,1.,1.,1.,1.,1.,1.,1.,1.,1.,1.,1.,1.,1.,1.,
1.,1.,1.,1.,1.,1.,1.,1.,1.,1.,1.,1.,1.,1.,1.,1.,1.,1.,1.,1.,1.))
REPRESENTATION_ITEM('')
);
#830=(
BOUNDED_CURVE()
B_SPLINE_CURVE(5,(#233968,#233969,#233970,#233971,#233972,#233973,#233974,
#233975,#233976,#233977,#233978,#233979,#233980,#233981,#233982,#233983,
#233984,#233985,#233986,#233987,#233988,#233989,#233990,#233991,#233992,
#233993,#233994,#233995,#233996,#233997,#233998,#233999,#234000,#234001,
#234002,#234003,#234004,#234005,#234006,#234007,#234008,#234009,#234010,
#234011,#234012,#234013,#234014,#234015,#234016,#234017,#234018,#234019,
#234020,#234021,#234022,#234023,#234024,#234025,#234026,#234027,#234028,
#234029,#234030,#234031,#234032,#234033,#234034,#234035,#234036,#234037,
#234038,#234039,#234040,#234041,#234042,#234043,#234044,#234045,#234046,
#234047,#234048,#234049,#234050,#234051,#234052,#234053,#234054,#234055,
#234056,#234057,#234058,#234059,#234060,#234061,#234062,#234063,#234064,
#234065,#234066,#234067,#234068,#234069,#234070,#234071,#234072,#234073,
#234074,#234075,#234076,#234077,#234078,#234079,#234080,#234081,#234082,
#234083,#234084,#234085,#234086,#234087,#234088,#234089,#234090,#234091,
#234092,#234093,#234094,#234095,#234096,#234097,#234098,#234099,#234100,
#234101,#234102,#234103,#234104,#234105,#234106,#234107,#234108,#234109,
#234110,#234111,#234112,#234113,#234114,#234115,#234116,#234117,#234118,
#234119,#234120,#234121,#234122,#234123,#234124,#234125,#234126,#234127,
#234128,#234129,#234130,#234131,#234132,#234133,#234134,#234135,#234136,
#234137,#234138,#234139,#234140,#234141,#234142,#234143,#234144,#234145,
#234146,#234147,#234148,#234149,#234150,#234151,#234152,#234153,#234154,
#234155,#234156,#234157,#234158,#234159,#234160,#234161,#234162,#234163,
#234164,#234165,#234166,#234167,#234168,#234169,#234170,#234171,#234172),
 .UNSPECIFIED.,.F.,.F.)
B_SPLINE_CURVE_WITH_KNOTS((6,1,1,1,1,1,1,1,1,1,1,1,1,1,1,1,1,1,1,1,1,1,
1,1,1,1,1,1,1,1,1,1,1,1,1,1,1,1,1,1,1,1,1,1,1,1,1,1,1,1,1,1,1,1,1,1,1,1,
1,1,1,1,1,1,1,1,1,1,1,1,1,1,1,1,1,1,1,1,1,1,1,1,1,1,1,1,1,1,1,1,1,1,1,1,
1,1,1,1,1,1,1,1,1,1,1,1,1,1,1,1,1,1,1,1,1,1,1,1,1,1,1,1,1,1,1,1,1,1,1,1,
1,1,1,1,1,1,1,1,1,1,1,1,1,1,1,1,1,1,1,1,1,1,1,1,1,1,1,1,1,1,1,1,1,1,1,1,
1,1,1,1,1,1,1,1,1,1,1,1,1,1,1,1,1,1,1,1,1,1,1,1,1,1,1,1,1,1,1,1,1,1,6),
(-1.,-0.995000000000001,-0.990000000000001,-0.985000000000001,-0.980000000000001,
-0.975000000000001,-0.970000000000001,-0.965000000000001,-0.960000000000001,
-0.955000000000001,-0.950000000000001,-0.945000000000001,-0.940000000000001,
-0.935000000000001,-0.930000000000001,-0.925000000000001,-0.920000000000001,
-0.915000000000001,-0.910000000000001,-0.905000000000001,-0.900000000000001,
-0.895000000000001,-0.890000000000001,-0.885000000000001,-0.880000000000001,
-0.875000000000001,-0.870000000000001,-0.865000000000001,-0.860000000000001,
-0.855000000000001,-0.850000000000001,-0.845000000000001,-0.840000000000001,
-0.835000000000001,-0.830000000000001,-0.825000000000001,-0.820000000000001,
-0.815000000000001,-0.810000000000001,-0.805000000000001,-0.800000000000001,
-0.795000000000001,-0.790000000000001,-0.785000000000001,-0.780000000000001,
-0.775000000000001,-0.770000000000001,-0.765000000000001,-0.760000000000001,
-0.755000000000001,-0.750000000000001,-0.745000000000001,-0.740000000000001,
-0.735000000000001,-0.730000000000001,-0.725000000000001,-0.720000000000001,
-0.715000000000001,-0.710000000000001,-0.705000000000001,-0.700000000000001,
-0.695000000000001,-0.690000000000001,-0.685,-0.68,-0.675,-0.67,-0.665,
-0.66,-0.655,-0.65,-0.645,-0.64,-0.635,-0.63,-0.625,-0.62,-0.615,-0.61,
-0.605,-0.6,-0.595,-0.59,-0.585,-0.58,-0.575,-0.57,-0.565,-0.56,-0.555,
-0.55,-0.545,-0.54,-0.535,-0.53,-0.525,-0.52,-0.515,-0.51,-0.505,-0.5,-0.495,
-0.49,-0.485,-0.48,-0.475,-0.47,-0.465,-0.46,-0.455,-0.45,-0.445,-0.44,
-0.435,-0.43,-0.425,-0.42,-0.415,-0.41,-0.405,-0.4,-0.395,-0.39,-0.385,
-0.38,-0.375,-0.37,-0.365,-0.36,-0.355,-0.35,-0.345,-0.34,-0.335,-0.33,
-0.325,-0.32,-0.315,-0.31,-0.305,-0.3,-0.295,-0.29,-0.285,-0.28,-0.275,
-0.27,-0.265,-0.26,-0.255,-0.25,-0.245,-0.24,-0.235,-0.23,-0.225,-0.22,
-0.215,-0.21,-0.205,-0.2,-0.195,-0.19,-0.185,-0.18,-0.175,-0.17,-0.165,
-0.16,-0.155,-0.15,-0.145,-0.14,-0.135,-0.13,-0.125,-0.12,-0.115,-0.11,
-0.105,-0.1,-0.095,-0.09,-0.085,-0.08,-0.075,-0.07,-0.065,-0.06,-0.055,
-0.05,-0.045,-0.04,-0.035,-0.03,-0.025,-0.02,-0.015,-0.01,-0.005,0.),
 .UNSPECIFIED.)
CURVE()
GEOMETRIC_REPRESENTATION_ITEM()
RATIONAL_B_SPLINE_CURVE((1.,1.,1.,1.,1.,1.,1.,1.,1.,1.,1.,1.,1.,1.,1.,1.,
1.,1.,1.,1.,1.,1.,1.,1.,1.,1.,1.,1.,1.,1.,1.,1.,1.,1.,1.,1.,1.,1.,1.,1.,
1.,1.,1.,1.,1.,1.,1.,1.,1.,1.,1.,1.,1.,1.,1.,1.,1.,1.,1.,1.,1.,1.,1.,1.,
1.,1.,1.,1.,1.,1.,1.,1.,1.,1.,1.,1.,1.,1.,1.,1.,1.,1.,1.,1.,1.,1.,1.,1.,
1.,1.,1.,1.,1.,1.,1.,1.,1.,1.,1.,1.,1.,1.,1.,1.,1.,1.,1.,1.,1.,1.,1.,1.,
1.,1.,1.,1.,1.,1.,1.,1.,1.,1.,1.,1.,1.,1.,1.,1.,1.,1.,1.,1.,1.,1.,1.,1.,
1.,1.,1.,1.,1.,1.,1.,1.,1.,1.,1.,1.,1.,1.,1.,1.,1.,1.,1.,1.,1.,1.,1.,1.,
1.,1.,1.,1.,1.,1.,1.,1.,1.,1.,1.,1.,1.,1.,1.,1.,1.,1.,1.,1.,1.,1.,1.,1.,
1.,1.,1.,1.,1.,1.,1.,1.,1.,1.,1.,1.,1.,1.,1.,1.,1.,1.,1.,1.,1.))
REPRESENTATION_ITEM('')
);
#831=(
BOUNDED_CURVE()
B_SPLINE_CURVE(5,(#234591,#234592,#234593,#234594,#234595,#234596,#234597,
#234598,#234599,#234600,#234601,#234602,#234603,#234604,#234605,#234606,
#234607,#234608,#234609,#234610,#234611,#234612,#234613,#234614,#234615,
#234616,#234617,#234618,#234619,#234620,#234621,#234622,#234623,#234624,
#234625,#234626,#234627,#234628,#234629,#234630,#234631,#234632,#234633,
#234634,#234635,#234636,#234637,#234638,#234639,#234640,#234641,#234642,
#234643,#234644,#234645,#234646,#234647,#234648,#234649,#234650,#234651,
#234652,#234653,#234654,#234655,#234656,#234657,#234658,#234659,#234660,
#234661,#234662,#234663,#234664,#234665,#234666,#234667,#234668,#234669,
#234670,#234671,#234672,#234673,#234674,#234675,#234676,#234677,#234678,
#234679,#234680,#234681,#234682,#234683,#234684,#234685,#234686,#234687,
#234688,#234689,#234690,#234691,#234692,#234693,#234694,#234695,#234696,
#234697,#234698,#234699,#234700,#234701,#234702,#234703,#234704,#234705,
#234706,#234707,#234708,#234709,#234710,#234711,#234712,#234713,#234714,
#234715,#234716,#234717,#234718,#234719,#234720,#234721,#234722,#234723,
#234724,#234725,#234726,#234727,#234728,#234729,#234730,#234731,#234732,
#234733,#234734,#234735,#234736,#234737,#234738,#234739,#234740,#234741,
#234742,#234743,#234744,#234745,#234746,#234747,#234748,#234749,#234750,
#234751,#234752,#234753,#234754,#234755,#234756,#234757,#234758,#234759,
#234760,#234761,#234762,#234763,#234764,#234765,#234766,#234767,#234768,
#234769,#234770,#234771,#234772,#234773,#234774,#234775,#234776,#234777,
#234778,#234779,#234780,#234781,#234782,#234783,#234784,#234785,#234786,
#234787,#234788,#234789,#234790,#234791,#234792,#234793,#234794,#234795),
 .UNSPECIFIED.,.F.,.F.)
B_SPLINE_CURVE_WITH_KNOTS((6,1,1,1,1,1,1,1,1,1,1,1,1,1,1,1,1,1,1,1,1,1,
1,1,1,1,1,1,1,1,1,1,1,1,1,1,1,1,1,1,1,1,1,1,1,1,1,1,1,1,1,1,1,1,1,1,1,1,
1,1,1,1,1,1,1,1,1,1,1,1,1,1,1,1,1,1,1,1,1,1,1,1,1,1,1,1,1,1,1,1,1,1,1,1,
1,1,1,1,1,1,1,1,1,1,1,1,1,1,1,1,1,1,1,1,1,1,1,1,1,1,1,1,1,1,1,1,1,1,1,1,
1,1,1,1,1,1,1,1,1,1,1,1,1,1,1,1,1,1,1,1,1,1,1,1,1,1,1,1,1,1,1,1,1,1,1,1,
1,1,1,1,1,1,1,1,1,1,1,1,1,1,1,1,1,1,1,1,1,1,1,1,1,1,1,1,1,1,1,1,1,1,6),
(-1.,-0.995000000000001,-0.990000000000001,-0.985000000000001,-0.980000000000001,
-0.975000000000001,-0.970000000000001,-0.965000000000001,-0.960000000000001,
-0.955000000000001,-0.950000000000001,-0.945000000000001,-0.940000000000001,
-0.935000000000001,-0.930000000000001,-0.925000000000001,-0.920000000000001,
-0.915000000000001,-0.910000000000001,-0.905000000000001,-0.900000000000001,
-0.895000000000001,-0.890000000000001,-0.885000000000001,-0.880000000000001,
-0.875000000000001,-0.870000000000001,-0.865000000000001,-0.860000000000001,
-0.855000000000001,-0.850000000000001,-0.845000000000001,-0.840000000000001,
-0.835000000000001,-0.830000000000001,-0.825000000000001,-0.820000000000001,
-0.815000000000001,-0.810000000000001,-0.805000000000001,-0.800000000000001,
-0.795000000000001,-0.790000000000001,-0.785000000000001,-0.780000000000001,
-0.775000000000001,-0.770000000000001,-0.765000000000001,-0.760000000000001,
-0.755000000000001,-0.750000000000001,-0.745000000000001,-0.740000000000001,
-0.735000000000001,-0.730000000000001,-0.725000000000001,-0.720000000000001,
-0.715000000000001,-0.710000000000001,-0.705000000000001,-0.700000000000001,
-0.695000000000001,-0.690000000000001,-0.685,-0.68,-0.675,-0.67,-0.665,
-0.66,-0.655,-0.65,-0.645,-0.64,-0.635,-0.63,-0.625,-0.62,-0.615,-0.61,
-0.605,-0.6,-0.595,-0.59,-0.585,-0.58,-0.575,-0.57,-0.565,-0.56,-0.555,
-0.55,-0.545,-0.54,-0.535,-0.53,-0.525,-0.52,-0.515,-0.51,-0.505,-0.5,-0.495,
-0.49,-0.485,-0.48,-0.475,-0.47,-0.465,-0.46,-0.455,-0.45,-0.445,-0.44,
-0.435,-0.43,-0.425,-0.42,-0.415,-0.41,-0.405,-0.4,-0.395,-0.39,-0.385,
-0.38,-0.375,-0.37,-0.365,-0.36,-0.355,-0.35,-0.345,-0.34,-0.335,-0.33,
-0.325,-0.32,-0.315,-0.31,-0.305,-0.3,-0.295,-0.29,-0.285,-0.28,-0.275,
-0.27,-0.265,-0.26,-0.255,-0.25,-0.245,-0.24,-0.235,-0.23,-0.225,-0.22,
-0.215,-0.21,-0.205,-0.2,-0.195,-0.19,-0.185,-0.18,-0.175,-0.17,-0.165,
-0.16,-0.155,-0.15,-0.145,-0.14,-0.135,-0.13,-0.125,-0.12,-0.115,-0.11,
-0.105,-0.1,-0.095,-0.09,-0.085,-0.08,-0.075,-0.07,-0.065,-0.06,-0.055,
-0.05,-0.045,-0.04,-0.035,-0.03,-0.025,-0.02,-0.015,-0.01,-0.005,0.),
 .UNSPECIFIED.)
CURVE()
GEOMETRIC_REPRESENTATION_ITEM()
RATIONAL_B_SPLINE_CURVE((1.,1.,1.,1.,1.,1.,1.,1.,1.,1.,1.,1.,1.,1.,1.,1.,
1.,1.,1.,1.,1.,1.,1.,1.,1.,1.,1.,1.,1.,1.,1.,1.,1.,1.,1.,1.,1.,1.,1.,1.,
1.,1.,1.,1.,1.,1.,1.,1.,1.,1.,1.,1.,1.,1.,1.,1.,1.,1.,1.,1.,1.,1.,1.,1.,
1.,1.,1.,1.,1.,1.,1.,1.,1.,1.,1.,1.,1.,1.,1.,1.,1.,1.,1.,1.,1.,1.,1.,1.,
1.,1.,1.,1.,1.,1.,1.,1.,1.,1.,1.,1.,1.,1.,1.,1.,1.,1.,1.,1.,1.,1.,1.,1.,
1.,1.,1.,1.,1.,1.,1.,1.,1.,1.,1.,1.,1.,1.,1.,1.,1.,1.,1.,1.,1.,1.,1.,1.,
1.,1.,1.,1.,1.,1.,1.,1.,1.,1.,1.,1.,1.,1.,1.,1.,1.,1.,1.,1.,1.,1.,1.,1.,
1.,1.,1.,1.,1.,1.,1.,1.,1.,1.,1.,1.,1.,1.,1.,1.,1.,1.,1.,1.,1.,1.,1.,1.,
1.,1.,1.,1.,1.,1.,1.,1.,1.,1.,1.,1.,1.,1.,1.,1.,1.,1.,1.,1.,1.))
REPRESENTATION_ITEM('')
);
#832=(
BOUNDED_CURVE()
B_SPLINE_CURVE(5,(#234798,#234799,#234800,#234801,#234802,#234803,#234804,
#234805,#234806,#234807,#234808,#234809,#234810,#234811,#234812,#234813,
#234814,#234815,#234816,#234817,#234818,#234819,#234820,#234821,#234822,
#234823,#234824,#234825,#234826,#234827,#234828,#234829,#234830,#234831,
#234832,#234833,#234834,#234835,#234836,#234837,#234838,#234839,#234840,
#234841,#234842,#234843,#234844,#234845,#234846,#234847,#234848,#234849,
#234850,#234851,#234852,#234853,#234854,#234855,#234856,#234857,#234858,
#234859,#234860,#234861,#234862,#234863,#234864,#234865,#234866,#234867,
#234868,#234869,#234870,#234871,#234872,#234873,#234874,#234875,#234876,
#234877,#234878,#234879,#234880,#234881,#234882,#234883,#234884,#234885,
#234886,#234887,#234888,#234889,#234890,#234891,#234892,#234893,#234894,
#234895,#234896,#234897,#234898,#234899,#234900,#234901,#234902,#234903,
#234904,#234905,#234906,#234907,#234908,#234909,#234910,#234911,#234912,
#234913,#234914,#234915,#234916,#234917,#234918,#234919,#234920,#234921,
#234922,#234923,#234924,#234925,#234926,#234927,#234928,#234929,#234930,
#234931,#234932,#234933,#234934,#234935,#234936,#234937,#234938,#234939,
#234940,#234941,#234942,#234943,#234944,#234945,#234946,#234947,#234948,
#234949,#234950,#234951,#234952,#234953,#234954,#234955,#234956,#234957,
#234958,#234959,#234960,#234961,#234962,#234963,#234964,#234965,#234966,
#234967,#234968,#234969,#234970,#234971,#234972,#234973,#234974,#234975,
#234976,#234977,#234978,#234979,#234980,#234981,#234982,#234983,#234984,
#234985,#234986,#234987,#234988,#234989,#234990,#234991,#234992,#234993,
#234994,#234995,#234996,#234997,#234998,#234999,#235000,#235001,#235002),
 .UNSPECIFIED.,.F.,.F.)
B_SPLINE_CURVE_WITH_KNOTS((6,1,1,1,1,1,1,1,1,1,1,1,1,1,1,1,1,1,1,1,1,1,
1,1,1,1,1,1,1,1,1,1,1,1,1,1,1,1,1,1,1,1,1,1,1,1,1,1,1,1,1,1,1,1,1,1,1,1,
1,1,1,1,1,1,1,1,1,1,1,1,1,1,1,1,1,1,1,1,1,1,1,1,1,1,1,1,1,1,1,1,1,1,1,1,
1,1,1,1,1,1,1,1,1,1,1,1,1,1,1,1,1,1,1,1,1,1,1,1,1,1,1,1,1,1,1,1,1,1,1,1,
1,1,1,1,1,1,1,1,1,1,1,1,1,1,1,1,1,1,1,1,1,1,1,1,1,1,1,1,1,1,1,1,1,1,1,1,
1,1,1,1,1,1,1,1,1,1,1,1,1,1,1,1,1,1,1,1,1,1,1,1,1,1,1,1,1,1,1,1,1,1,6),
(0.,0.005,0.01,0.015,0.02,0.025,0.03,0.035,0.04,0.045,0.05,0.055,0.06,0.065,
0.07,0.075,0.08,0.085,0.09,0.095,0.1,0.105,0.11,0.115,0.12,0.125,0.13,0.135,
0.14,0.145,0.15,0.155,0.16,0.165,0.17,0.175,0.18,0.185,0.19,0.195,0.2,0.205,
0.21,0.215,0.22,0.225,0.23,0.235,0.24,0.245,0.25,0.255,0.26,0.265,0.27,
0.275,0.28,0.285,0.29,0.295,0.3,0.305,0.31,0.315,0.32,0.325,0.33,0.335,
0.34,0.345,0.35,0.355,0.36,0.365,0.37,0.375,0.38,0.385,0.39,0.395,0.4,0.405,
0.41,0.415,0.42,0.425,0.43,0.435,0.44,0.445,0.45,0.455,0.46,0.465,0.47,
0.475,0.48,0.485,0.49,0.495,0.5,0.505,0.51,0.515,0.52,0.525,0.53,0.535,
0.54,0.545,0.55,0.555,0.56,0.565,0.57,0.575,0.58,0.585,0.59,0.595,0.6,0.605,
0.61,0.615,0.62,0.625,0.63,0.635,0.64,0.645,0.65,0.655,0.66,0.665,0.67,
0.675,0.68,0.685,0.690000000000001,0.695000000000001,0.700000000000001,
0.705000000000001,0.710000000000001,0.715000000000001,0.720000000000001,
0.725000000000001,0.730000000000001,0.735000000000001,0.740000000000001,
0.745000000000001,0.750000000000001,0.755000000000001,0.760000000000001,
0.765000000000001,0.770000000000001,0.775000000000001,0.780000000000001,
0.785000000000001,0.790000000000001,0.795000000000001,0.800000000000001,
0.805000000000001,0.810000000000001,0.815000000000001,0.820000000000001,
0.825000000000001,0.830000000000001,0.835000000000001,0.840000000000001,
0.845000000000001,0.850000000000001,0.855000000000001,0.860000000000001,
0.865000000000001,0.870000000000001,0.875000000000001,0.880000000000001,
0.885000000000001,0.890000000000001,0.895000000000001,0.900000000000001,
0.905000000000001,0.910000000000001,0.915000000000001,0.920000000000001,
0.925000000000001,0.930000000000001,0.935000000000001,0.940000000000001,
0.945000000000001,0.950000000000001,0.955000000000001,0.960000000000001,
0.965000000000001,0.970000000000001,0.975000000000001,0.980000000000001,
0.985000000000001,0.990000000000001,0.995000000000001,1.),.UNSPECIFIED.)
CURVE()
GEOMETRIC_REPRESENTATION_ITEM()
RATIONAL_B_SPLINE_CURVE((1.,1.,1.,1.,1.,1.,1.,1.,1.,1.,1.,1.,1.,1.,1.,1.,
1.,1.,1.,1.,1.,1.,1.,1.,1.,1.,1.,1.,1.,1.,1.,1.,1.,1.,1.,1.,1.,1.,1.,1.,
1.,1.,1.,1.,1.,1.,1.,1.,1.,1.,1.,1.,1.,1.,1.,1.,1.,1.,1.,1.,1.,1.,1.,1.,
1.,1.,1.,1.,1.,1.,1.,1.,1.,1.,1.,1.,1.,1.,1.,1.,1.,1.,1.,1.,1.,1.,1.,1.,
1.,1.,1.,1.,1.,1.,1.,1.,1.,1.,1.,1.,1.,1.,1.,1.,1.,1.,1.,1.,1.,1.,1.,1.,
1.,1.,1.,1.,1.,1.,1.,1.,1.,1.,1.,1.,1.,1.,1.,1.,1.,1.,1.,1.,1.,1.,1.,1.,
1.,1.,1.,1.,1.,1.,1.,1.,1.,1.,1.,1.,1.,1.,1.,1.,1.,1.,1.,1.,1.,1.,1.,1.,
1.,1.,1.,1.,1.,1.,1.,1.,1.,1.,1.,1.,1.,1.,1.,1.,1.,1.,1.,1.,1.,1.,1.,1.,
1.,1.,1.,1.,1.,1.,1.,1.,1.,1.,1.,1.,1.,1.,1.,1.,1.,1.,1.,1.,1.))
REPRESENTATION_ITEM('')
);
#833=(
BOUNDED_CURVE()
B_SPLINE_CURVE(5,(#235414,#235415,#235416,#235417,#235418,#235419,#235420,
#235421,#235422,#235423,#235424,#235425,#235426,#235427,#235428,#235429,
#235430,#235431,#235432,#235433,#235434,#235435,#235436,#235437,#235438,
#235439,#235440,#235441,#235442,#235443,#235444,#235445,#235446,#235447,
#235448,#235449,#235450,#235451,#235452,#235453,#235454,#235455,#235456,
#235457,#235458,#235459,#235460,#235461,#235462,#235463,#235464,#235465,
#235466,#235467,#235468,#235469,#235470,#235471,#235472,#235473,#235474,
#235475,#235476,#235477,#235478,#235479,#235480,#235481,#235482,#235483,
#235484,#235485,#235486,#235487,#235488,#235489,#235490,#235491,#235492,
#235493,#235494,#235495,#235496,#235497,#235498,#235499,#235500,#235501,
#235502,#235503,#235504,#235505,#235506,#235507,#235508,#235509,#235510,
#235511,#235512,#235513,#235514,#235515,#235516,#235517,#235518,#235519,
#235520,#235521,#235522,#235523,#235524,#235525,#235526,#235527,#235528,
#235529,#235530,#235531,#235532,#235533,#235534,#235535,#235536,#235537,
#235538,#235539,#235540,#235541,#235542,#235543,#235544,#235545,#235546,
#235547,#235548,#235549,#235550,#235551,#235552,#235553,#235554,#235555,
#235556,#235557,#235558,#235559,#235560,#235561,#235562,#235563,#235564,
#235565,#235566,#235567,#235568,#235569,#235570,#235571,#235572,#235573,
#235574,#235575,#235576,#235577,#235578,#235579,#235580,#235581,#235582,
#235583,#235584,#235585,#235586,#235587,#235588,#235589,#235590,#235591,
#235592,#235593,#235594,#235595,#235596,#235597,#235598,#235599,#235600,
#235601,#235602,#235603,#235604,#235605,#235606,#235607,#235608,#235609,
#235610,#235611,#235612,#235613,#235614,#235615,#235616,#235617,#235618),
 .UNSPECIFIED.,.F.,.F.)
B_SPLINE_CURVE_WITH_KNOTS((6,1,1,1,1,1,1,1,1,1,1,1,1,1,1,1,1,1,1,1,1,1,
1,1,1,1,1,1,1,1,1,1,1,1,1,1,1,1,1,1,1,1,1,1,1,1,1,1,1,1,1,1,1,1,1,1,1,1,
1,1,1,1,1,1,1,1,1,1,1,1,1,1,1,1,1,1,1,1,1,1,1,1,1,1,1,1,1,1,1,1,1,1,1,1,
1,1,1,1,1,1,1,1,1,1,1,1,1,1,1,1,1,1,1,1,1,1,1,1,1,1,1,1,1,1,1,1,1,1,1,1,
1,1,1,1,1,1,1,1,1,1,1,1,1,1,1,1,1,1,1,1,1,1,1,1,1,1,1,1,1,1,1,1,1,1,1,1,
1,1,1,1,1,1,1,1,1,1,1,1,1,1,1,1,1,1,1,1,1,1,1,1,1,1,1,1,1,1,1,1,1,1,6),
(0.,0.005,0.01,0.015,0.02,0.025,0.03,0.035,0.04,0.045,0.05,0.055,0.06,0.065,
0.07,0.075,0.08,0.085,0.09,0.095,0.1,0.105,0.11,0.115,0.12,0.125,0.13,0.135,
0.14,0.145,0.15,0.155,0.16,0.165,0.17,0.175,0.18,0.185,0.19,0.195,0.2,0.205,
0.21,0.215,0.22,0.225,0.23,0.235,0.24,0.245,0.25,0.255,0.26,0.265,0.27,
0.275,0.28,0.285,0.29,0.295,0.3,0.305,0.31,0.315,0.32,0.325,0.33,0.335,
0.34,0.345,0.35,0.355,0.36,0.365,0.37,0.375,0.38,0.385,0.39,0.395,0.4,0.405,
0.41,0.415,0.42,0.425,0.43,0.435,0.44,0.445,0.45,0.455,0.46,0.465,0.47,
0.475,0.48,0.485,0.49,0.495,0.5,0.505,0.51,0.515,0.52,0.525,0.53,0.535,
0.54,0.545,0.55,0.555,0.56,0.565,0.57,0.575,0.58,0.585,0.59,0.595,0.6,0.605,
0.61,0.615,0.62,0.625,0.63,0.635,0.64,0.645,0.65,0.655,0.66,0.665,0.67,
0.675,0.68,0.685,0.690000000000001,0.695000000000001,0.700000000000001,
0.705000000000001,0.710000000000001,0.715000000000001,0.720000000000001,
0.725000000000001,0.730000000000001,0.735000000000001,0.740000000000001,
0.745000000000001,0.750000000000001,0.755000000000001,0.760000000000001,
0.765000000000001,0.770000000000001,0.775000000000001,0.780000000000001,
0.785000000000001,0.790000000000001,0.795000000000001,0.800000000000001,
0.805000000000001,0.810000000000001,0.815000000000001,0.820000000000001,
0.825000000000001,0.830000000000001,0.835000000000001,0.840000000000001,
0.845000000000001,0.850000000000001,0.855000000000001,0.860000000000001,
0.865000000000001,0.870000000000001,0.875000000000001,0.880000000000001,
0.885000000000001,0.890000000000001,0.895000000000001,0.900000000000001,
0.905000000000001,0.910000000000001,0.915000000000001,0.920000000000001,
0.925000000000001,0.930000000000001,0.935000000000001,0.940000000000001,
0.945000000000001,0.950000000000001,0.955000000000001,0.960000000000001,
0.965000000000001,0.970000000000001,0.975000000000001,0.980000000000001,
0.985000000000001,0.990000000000001,0.995000000000001,1.),.UNSPECIFIED.)
CURVE()
GEOMETRIC_REPRESENTATION_ITEM()
RATIONAL_B_SPLINE_CURVE((1.,1.,1.,1.,1.,1.,1.,1.,1.,1.,1.,1.,1.,1.,1.,1.,
1.,1.,1.,1.,1.,1.,1.,1.,1.,1.,1.,1.,1.,1.,1.,1.,1.,1.,1.,1.,1.,1.,1.,1.,
1.,1.,1.,1.,1.,1.,1.,1.,1.,1.,1.,1.,1.,1.,1.,1.,1.,1.,1.,1.,1.,1.,1.,1.,
1.,1.,1.,1.,1.,1.,1.,1.,1.,1.,1.,1.,1.,1.,1.,1.,1.,1.,1.,1.,1.,1.,1.,1.,
1.,1.,1.,1.,1.,1.,1.,1.,1.,1.,1.,1.,1.,1.,1.,1.,1.,1.,1.,1.,1.,1.,1.,1.,
1.,1.,1.,1.,1.,1.,1.,1.,1.,1.,1.,1.,1.,1.,1.,1.,1.,1.,1.,1.,1.,1.,1.,1.,
1.,1.,1.,1.,1.,1.,1.,1.,1.,1.,1.,1.,1.,1.,1.,1.,1.,1.,1.,1.,1.,1.,1.,1.,
1.,1.,1.,1.,1.,1.,1.,1.,1.,1.,1.,1.,1.,1.,1.,1.,1.,1.,1.,1.,1.,1.,1.,1.,
1.,1.,1.,1.,1.,1.,1.,1.,1.,1.,1.,1.,1.,1.,1.,1.,1.,1.,1.,1.,1.))
REPRESENTATION_ITEM('')
);
#834=(
BOUNDED_CURVE()
B_SPLINE_CURVE(5,(#235620,#235621,#235622,#235623,#235624,#235625,#235626,
#235627,#235628,#235629,#235630,#235631,#235632,#235633,#235634,#235635,
#235636,#235637,#235638,#235639,#235640,#235641,#235642,#235643,#235644,
#235645,#235646,#235647,#235648,#235649,#235650,#235651,#235652,#235653,
#235654,#235655,#235656,#235657,#235658,#235659,#235660,#235661,#235662,
#235663,#235664,#235665,#235666,#235667,#235668,#235669,#235670,#235671,
#235672,#235673,#235674,#235675,#235676,#235677,#235678,#235679,#235680,
#235681,#235682,#235683,#235684,#235685,#235686,#235687,#235688,#235689,
#235690,#235691,#235692,#235693,#235694,#235695,#235696,#235697,#235698,
#235699,#235700,#235701,#235702,#235703,#235704,#235705,#235706,#235707,
#235708,#235709,#235710,#235711,#235712,#235713,#235714,#235715,#235716,
#235717,#235718,#235719,#235720,#235721,#235722,#235723,#235724,#235725,
#235726,#235727,#235728,#235729,#235730,#235731,#235732,#235733,#235734,
#235735,#235736,#235737,#235738,#235739,#235740,#235741,#235742,#235743,
#235744,#235745,#235746,#235747,#235748,#235749,#235750,#235751,#235752,
#235753,#235754,#235755,#235756,#235757,#235758,#235759,#235760,#235761,
#235762,#235763,#235764,#235765,#235766,#235767,#235768,#235769,#235770,
#235771,#235772,#235773,#235774,#235775,#235776,#235777,#235778,#235779,
#235780,#235781,#235782,#235783,#235784,#235785,#235786,#235787,#235788,
#235789,#235790,#235791,#235792,#235793,#235794,#235795,#235796,#235797,
#235798,#235799,#235800,#235801,#235802,#235803,#235804,#235805,#235806,
#235807,#235808,#235809,#235810,#235811,#235812,#235813,#235814,#235815,
#235816,#235817,#235818,#235819,#235820,#235821,#235822,#235823,#235824),
 .UNSPECIFIED.,.F.,.F.)
B_SPLINE_CURVE_WITH_KNOTS((6,1,1,1,1,1,1,1,1,1,1,1,1,1,1,1,1,1,1,1,1,1,
1,1,1,1,1,1,1,1,1,1,1,1,1,1,1,1,1,1,1,1,1,1,1,1,1,1,1,1,1,1,1,1,1,1,1,1,
1,1,1,1,1,1,1,1,1,1,1,1,1,1,1,1,1,1,1,1,1,1,1,1,1,1,1,1,1,1,1,1,1,1,1,1,
1,1,1,1,1,1,1,1,1,1,1,1,1,1,1,1,1,1,1,1,1,1,1,1,1,1,1,1,1,1,1,1,1,1,1,1,
1,1,1,1,1,1,1,1,1,1,1,1,1,1,1,1,1,1,1,1,1,1,1,1,1,1,1,1,1,1,1,1,1,1,1,1,
1,1,1,1,1,1,1,1,1,1,1,1,1,1,1,1,1,1,1,1,1,1,1,1,1,1,1,1,1,1,1,1,1,1,6),
(-1.,-0.995000000000001,-0.990000000000001,-0.985000000000001,-0.980000000000001,
-0.975000000000001,-0.970000000000001,-0.965000000000001,-0.960000000000001,
-0.955000000000001,-0.950000000000001,-0.945000000000001,-0.940000000000001,
-0.935000000000001,-0.930000000000001,-0.925000000000001,-0.920000000000001,
-0.915000000000001,-0.910000000000001,-0.905000000000001,-0.900000000000001,
-0.895000000000001,-0.890000000000001,-0.885000000000001,-0.880000000000001,
-0.875000000000001,-0.870000000000001,-0.865000000000001,-0.860000000000001,
-0.855000000000001,-0.850000000000001,-0.845000000000001,-0.840000000000001,
-0.835000000000001,-0.830000000000001,-0.825000000000001,-0.820000000000001,
-0.815000000000001,-0.810000000000001,-0.805000000000001,-0.800000000000001,
-0.795000000000001,-0.790000000000001,-0.785000000000001,-0.780000000000001,
-0.775000000000001,-0.770000000000001,-0.765000000000001,-0.760000000000001,
-0.755000000000001,-0.750000000000001,-0.745000000000001,-0.740000000000001,
-0.735000000000001,-0.730000000000001,-0.725000000000001,-0.720000000000001,
-0.715000000000001,-0.710000000000001,-0.705000000000001,-0.700000000000001,
-0.695000000000001,-0.690000000000001,-0.685,-0.68,-0.675,-0.67,-0.665,
-0.66,-0.655,-0.65,-0.645,-0.64,-0.635,-0.63,-0.625,-0.62,-0.615,-0.61,
-0.605,-0.6,-0.595,-0.59,-0.585,-0.58,-0.575,-0.57,-0.565,-0.56,-0.555,
-0.55,-0.545,-0.54,-0.535,-0.53,-0.525,-0.52,-0.515,-0.51,-0.505,-0.5,-0.495,
-0.49,-0.485,-0.48,-0.475,-0.47,-0.465,-0.46,-0.455,-0.45,-0.445,-0.44,
-0.435,-0.43,-0.425,-0.42,-0.415,-0.41,-0.405,-0.4,-0.395,-0.39,-0.385,
-0.38,-0.375,-0.37,-0.365,-0.36,-0.355,-0.35,-0.345,-0.34,-0.335,-0.33,
-0.325,-0.32,-0.315,-0.31,-0.305,-0.3,-0.295,-0.29,-0.285,-0.28,-0.275,
-0.27,-0.265,-0.26,-0.255,-0.25,-0.245,-0.24,-0.235,-0.23,-0.225,-0.22,
-0.215,-0.21,-0.205,-0.2,-0.195,-0.19,-0.185,-0.18,-0.175,-0.17,-0.165,
-0.16,-0.155,-0.15,-0.145,-0.14,-0.135,-0.13,-0.125,-0.12,-0.115,-0.11,
-0.105,-0.1,-0.095,-0.09,-0.085,-0.08,-0.075,-0.07,-0.065,-0.06,-0.055,
-0.05,-0.045,-0.04,-0.035,-0.03,-0.025,-0.02,-0.015,-0.01,-0.005,0.),
 .UNSPECIFIED.)
CURVE()
GEOMETRIC_REPRESENTATION_ITEM()
RATIONAL_B_SPLINE_CURVE((1.,1.,1.,1.,1.,1.,1.,1.,1.,1.,1.,1.,1.,1.,1.,1.,
1.,1.,1.,1.,1.,1.,1.,1.,1.,1.,1.,1.,1.,1.,1.,1.,1.,1.,1.,1.,1.,1.,1.,1.,
1.,1.,1.,1.,1.,1.,1.,1.,1.,1.,1.,1.,1.,1.,1.,1.,1.,1.,1.,1.,1.,1.,1.,1.,
1.,1.,1.,1.,1.,1.,1.,1.,1.,1.,1.,1.,1.,1.,1.,1.,1.,1.,1.,1.,1.,1.,1.,1.,
1.,1.,1.,1.,1.,1.,1.,1.,1.,1.,1.,1.,1.,1.,1.,1.,1.,1.,1.,1.,1.,1.,1.,1.,
1.,1.,1.,1.,1.,1.,1.,1.,1.,1.,1.,1.,1.,1.,1.,1.,1.,1.,1.,1.,1.,1.,1.,1.,
1.,1.,1.,1.,1.,1.,1.,1.,1.,1.,1.,1.,1.,1.,1.,1.,1.,1.,1.,1.,1.,1.,1.,1.,
1.,1.,1.,1.,1.,1.,1.,1.,1.,1.,1.,1.,1.,1.,1.,1.,1.,1.,1.,1.,1.,1.,1.,1.,
1.,1.,1.,1.,1.,1.,1.,1.,1.,1.,1.,1.,1.,1.,1.,1.,1.,1.,1.,1.,1.))
REPRESENTATION_ITEM('')
);
#835=(
BOUNDED_CURVE()
B_SPLINE_CURVE(5,(#236243,#236244,#236245,#236246,#236247,#236248,#236249,
#236250,#236251,#236252,#236253,#236254,#236255,#236256,#236257,#236258,
#236259,#236260,#236261,#236262,#236263,#236264,#236265,#236266,#236267,
#236268,#236269,#236270,#236271,#236272,#236273,#236274,#236275,#236276,
#236277,#236278,#236279,#236280,#236281,#236282,#236283,#236284,#236285,
#236286,#236287,#236288,#236289,#236290,#236291,#236292,#236293,#236294,
#236295,#236296,#236297,#236298,#236299,#236300,#236301,#236302,#236303,
#236304,#236305,#236306,#236307,#236308,#236309,#236310,#236311,#236312,
#236313,#236314,#236315,#236316,#236317,#236318,#236319,#236320,#236321,
#236322,#236323,#236324,#236325,#236326,#236327,#236328,#236329,#236330,
#236331,#236332,#236333,#236334,#236335,#236336,#236337,#236338,#236339,
#236340,#236341,#236342,#236343,#236344,#236345,#236346,#236347,#236348,
#236349,#236350,#236351,#236352,#236353,#236354,#236355,#236356,#236357,
#236358,#236359,#236360,#236361,#236362,#236363,#236364,#236365,#236366,
#236367,#236368,#236369,#236370,#236371,#236372,#236373,#236374,#236375,
#236376,#236377,#236378,#236379,#236380,#236381,#236382,#236383,#236384,
#236385,#236386,#236387,#236388,#236389,#236390,#236391,#236392,#236393,
#236394,#236395,#236396,#236397,#236398,#236399,#236400,#236401,#236402,
#236403,#236404,#236405,#236406,#236407,#236408,#236409,#236410,#236411,
#236412,#236413,#236414,#236415,#236416,#236417,#236418,#236419,#236420,
#236421,#236422,#236423,#236424,#236425,#236426,#236427,#236428,#236429,
#236430,#236431,#236432,#236433,#236434,#236435,#236436,#236437,#236438,
#236439,#236440,#236441,#236442,#236443,#236444,#236445,#236446,#236447),
 .UNSPECIFIED.,.F.,.F.)
B_SPLINE_CURVE_WITH_KNOTS((6,1,1,1,1,1,1,1,1,1,1,1,1,1,1,1,1,1,1,1,1,1,
1,1,1,1,1,1,1,1,1,1,1,1,1,1,1,1,1,1,1,1,1,1,1,1,1,1,1,1,1,1,1,1,1,1,1,1,
1,1,1,1,1,1,1,1,1,1,1,1,1,1,1,1,1,1,1,1,1,1,1,1,1,1,1,1,1,1,1,1,1,1,1,1,
1,1,1,1,1,1,1,1,1,1,1,1,1,1,1,1,1,1,1,1,1,1,1,1,1,1,1,1,1,1,1,1,1,1,1,1,
1,1,1,1,1,1,1,1,1,1,1,1,1,1,1,1,1,1,1,1,1,1,1,1,1,1,1,1,1,1,1,1,1,1,1,1,
1,1,1,1,1,1,1,1,1,1,1,1,1,1,1,1,1,1,1,1,1,1,1,1,1,1,1,1,1,1,1,1,1,1,6),
(-1.,-0.995000000000001,-0.990000000000001,-0.985000000000001,-0.980000000000001,
-0.975000000000001,-0.970000000000001,-0.965000000000001,-0.960000000000001,
-0.955000000000001,-0.950000000000001,-0.945000000000001,-0.940000000000001,
-0.935000000000001,-0.930000000000001,-0.925000000000001,-0.920000000000001,
-0.915000000000001,-0.910000000000001,-0.905000000000001,-0.900000000000001,
-0.895000000000001,-0.890000000000001,-0.885000000000001,-0.880000000000001,
-0.875000000000001,-0.870000000000001,-0.865000000000001,-0.860000000000001,
-0.855000000000001,-0.850000000000001,-0.845000000000001,-0.840000000000001,
-0.835000000000001,-0.830000000000001,-0.825000000000001,-0.820000000000001,
-0.815000000000001,-0.810000000000001,-0.805000000000001,-0.800000000000001,
-0.795000000000001,-0.790000000000001,-0.785000000000001,-0.780000000000001,
-0.775000000000001,-0.770000000000001,-0.765000000000001,-0.760000000000001,
-0.755000000000001,-0.750000000000001,-0.745000000000001,-0.740000000000001,
-0.735000000000001,-0.730000000000001,-0.725000000000001,-0.720000000000001,
-0.715000000000001,-0.710000000000001,-0.705000000000001,-0.700000000000001,
-0.695000000000001,-0.690000000000001,-0.685,-0.68,-0.675,-0.67,-0.665,
-0.66,-0.655,-0.65,-0.645,-0.64,-0.635,-0.63,-0.625,-0.62,-0.615,-0.61,
-0.605,-0.6,-0.595,-0.59,-0.585,-0.58,-0.575,-0.57,-0.565,-0.56,-0.555,
-0.55,-0.545,-0.54,-0.535,-0.53,-0.525,-0.52,-0.515,-0.51,-0.505,-0.5,-0.495,
-0.49,-0.485,-0.48,-0.475,-0.47,-0.465,-0.46,-0.455,-0.45,-0.445,-0.44,
-0.435,-0.43,-0.425,-0.42,-0.415,-0.41,-0.405,-0.4,-0.395,-0.39,-0.385,
-0.38,-0.375,-0.37,-0.365,-0.36,-0.355,-0.35,-0.345,-0.34,-0.335,-0.33,
-0.325,-0.32,-0.315,-0.31,-0.305,-0.3,-0.295,-0.29,-0.285,-0.28,-0.275,
-0.27,-0.265,-0.26,-0.255,-0.25,-0.245,-0.24,-0.235,-0.23,-0.225,-0.22,
-0.215,-0.21,-0.205,-0.2,-0.195,-0.19,-0.185,-0.18,-0.175,-0.17,-0.165,
-0.16,-0.155,-0.15,-0.145,-0.14,-0.135,-0.13,-0.125,-0.12,-0.115,-0.11,
-0.105,-0.1,-0.095,-0.09,-0.085,-0.08,-0.075,-0.07,-0.065,-0.06,-0.055,
-0.05,-0.045,-0.04,-0.035,-0.03,-0.025,-0.02,-0.015,-0.01,-0.005,0.),
 .UNSPECIFIED.)
CURVE()
GEOMETRIC_REPRESENTATION_ITEM()
RATIONAL_B_SPLINE_CURVE((1.,1.,1.,1.,1.,1.,1.,1.,1.,1.,1.,1.,1.,1.,1.,1.,
1.,1.,1.,1.,1.,1.,1.,1.,1.,1.,1.,1.,1.,1.,1.,1.,1.,1.,1.,1.,1.,1.,1.,1.,
1.,1.,1.,1.,1.,1.,1.,1.,1.,1.,1.,1.,1.,1.,1.,1.,1.,1.,1.,1.,1.,1.,1.,1.,
1.,1.,1.,1.,1.,1.,1.,1.,1.,1.,1.,1.,1.,1.,1.,1.,1.,1.,1.,1.,1.,1.,1.,1.,
1.,1.,1.,1.,1.,1.,1.,1.,1.,1.,1.,1.,1.,1.,1.,1.,1.,1.,1.,1.,1.,1.,1.,1.,
1.,1.,1.,1.,1.,1.,1.,1.,1.,1.,1.,1.,1.,1.,1.,1.,1.,1.,1.,1.,1.,1.,1.,1.,
1.,1.,1.,1.,1.,1.,1.,1.,1.,1.,1.,1.,1.,1.,1.,1.,1.,1.,1.,1.,1.,1.,1.,1.,
1.,1.,1.,1.,1.,1.,1.,1.,1.,1.,1.,1.,1.,1.,1.,1.,1.,1.,1.,1.,1.,1.,1.,1.,
1.,1.,1.,1.,1.,1.,1.,1.,1.,1.,1.,1.,1.,1.,1.,1.,1.,1.,1.,1.,1.))
REPRESENTATION_ITEM('')
);
#836=(
BOUNDED_CURVE()
B_SPLINE_CURVE(5,(#236450,#236451,#236452,#236453,#236454,#236455,#236456,
#236457,#236458,#236459,#236460,#236461,#236462,#236463,#236464,#236465,
#236466,#236467,#236468,#236469,#236470,#236471,#236472,#236473,#236474,
#236475,#236476,#236477,#236478,#236479,#236480,#236481,#236482,#236483,
#236484,#236485,#236486,#236487,#236488,#236489,#236490,#236491,#236492,
#236493,#236494,#236495,#236496,#236497,#236498,#236499,#236500,#236501,
#236502,#236503,#236504,#236505,#236506,#236507,#236508,#236509,#236510,
#236511,#236512,#236513,#236514,#236515,#236516,#236517,#236518,#236519,
#236520,#236521,#236522,#236523,#236524,#236525,#236526,#236527,#236528,
#236529,#236530,#236531,#236532,#236533,#236534,#236535,#236536,#236537,
#236538,#236539,#236540,#236541,#236542,#236543,#236544,#236545,#236546,
#236547,#236548,#236549,#236550,#236551,#236552,#236553,#236554,#236555,
#236556,#236557,#236558,#236559,#236560,#236561,#236562,#236563,#236564,
#236565,#236566,#236567,#236568,#236569,#236570,#236571,#236572,#236573,
#236574,#236575,#236576,#236577,#236578,#236579,#236580,#236581,#236582,
#236583,#236584,#236585,#236586,#236587,#236588,#236589,#236590,#236591,
#236592,#236593,#236594,#236595,#236596,#236597,#236598,#236599,#236600,
#236601,#236602,#236603,#236604,#236605,#236606,#236607,#236608,#236609,
#236610,#236611,#236612,#236613,#236614,#236615,#236616,#236617,#236618,
#236619,#236620,#236621,#236622,#236623,#236624,#236625,#236626,#236627,
#236628,#236629,#236630,#236631,#236632,#236633,#236634,#236635,#236636,
#236637,#236638,#236639,#236640,#236641,#236642,#236643,#236644,#236645,
#236646,#236647,#236648,#236649,#236650,#236651,#236652,#236653,#236654),
 .UNSPECIFIED.,.F.,.F.)
B_SPLINE_CURVE_WITH_KNOTS((6,1,1,1,1,1,1,1,1,1,1,1,1,1,1,1,1,1,1,1,1,1,
1,1,1,1,1,1,1,1,1,1,1,1,1,1,1,1,1,1,1,1,1,1,1,1,1,1,1,1,1,1,1,1,1,1,1,1,
1,1,1,1,1,1,1,1,1,1,1,1,1,1,1,1,1,1,1,1,1,1,1,1,1,1,1,1,1,1,1,1,1,1,1,1,
1,1,1,1,1,1,1,1,1,1,1,1,1,1,1,1,1,1,1,1,1,1,1,1,1,1,1,1,1,1,1,1,1,1,1,1,
1,1,1,1,1,1,1,1,1,1,1,1,1,1,1,1,1,1,1,1,1,1,1,1,1,1,1,1,1,1,1,1,1,1,1,1,
1,1,1,1,1,1,1,1,1,1,1,1,1,1,1,1,1,1,1,1,1,1,1,1,1,1,1,1,1,1,1,1,1,1,6),
(0.,0.005,0.01,0.015,0.02,0.025,0.03,0.035,0.04,0.045,0.05,0.055,0.06,0.065,
0.07,0.075,0.08,0.085,0.09,0.095,0.1,0.105,0.11,0.115,0.12,0.125,0.13,0.135,
0.14,0.145,0.15,0.155,0.16,0.165,0.17,0.175,0.18,0.185,0.19,0.195,0.2,0.205,
0.21,0.215,0.22,0.225,0.23,0.235,0.24,0.245,0.25,0.255,0.26,0.265,0.27,
0.275,0.28,0.285,0.29,0.295,0.3,0.305,0.31,0.315,0.32,0.325,0.33,0.335,
0.34,0.345,0.35,0.355,0.36,0.365,0.37,0.375,0.38,0.385,0.39,0.395,0.4,0.405,
0.41,0.415,0.42,0.425,0.43,0.435,0.44,0.445,0.45,0.455,0.46,0.465,0.47,
0.475,0.48,0.485,0.49,0.495,0.5,0.505,0.51,0.515,0.52,0.525,0.53,0.535,
0.54,0.545,0.55,0.555,0.56,0.565,0.57,0.575,0.58,0.585,0.59,0.595,0.6,0.605,
0.61,0.615,0.62,0.625,0.63,0.635,0.64,0.645,0.65,0.655,0.66,0.665,0.67,
0.675,0.68,0.685,0.690000000000001,0.695000000000001,0.700000000000001,
0.705000000000001,0.710000000000001,0.715000000000001,0.720000000000001,
0.725000000000001,0.730000000000001,0.735000000000001,0.740000000000001,
0.745000000000001,0.750000000000001,0.755000000000001,0.760000000000001,
0.765000000000001,0.770000000000001,0.775000000000001,0.780000000000001,
0.785000000000001,0.790000000000001,0.795000000000001,0.800000000000001,
0.805000000000001,0.810000000000001,0.815000000000001,0.820000000000001,
0.825000000000001,0.830000000000001,0.835000000000001,0.840000000000001,
0.845000000000001,0.850000000000001,0.855000000000001,0.860000000000001,
0.865000000000001,0.870000000000001,0.875000000000001,0.880000000000001,
0.885000000000001,0.890000000000001,0.895000000000001,0.900000000000001,
0.905000000000001,0.910000000000001,0.915000000000001,0.920000000000001,
0.925000000000001,0.930000000000001,0.935000000000001,0.940000000000001,
0.945000000000001,0.950000000000001,0.955000000000001,0.960000000000001,
0.965000000000001,0.970000000000001,0.975000000000001,0.980000000000001,
0.985000000000001,0.990000000000001,0.995000000000001,1.),.UNSPECIFIED.)
CURVE()
GEOMETRIC_REPRESENTATION_ITEM()
RATIONAL_B_SPLINE_CURVE((1.,1.,1.,1.,1.,1.,1.,1.,1.,1.,1.,1.,1.,1.,1.,1.,
1.,1.,1.,1.,1.,1.,1.,1.,1.,1.,1.,1.,1.,1.,1.,1.,1.,1.,1.,1.,1.,1.,1.,1.,
1.,1.,1.,1.,1.,1.,1.,1.,1.,1.,1.,1.,1.,1.,1.,1.,1.,1.,1.,1.,1.,1.,1.,1.,
1.,1.,1.,1.,1.,1.,1.,1.,1.,1.,1.,1.,1.,1.,1.,1.,1.,1.,1.,1.,1.,1.,1.,1.,
1.,1.,1.,1.,1.,1.,1.,1.,1.,1.,1.,1.,1.,1.,1.,1.,1.,1.,1.,1.,1.,1.,1.,1.,
1.,1.,1.,1.,1.,1.,1.,1.,1.,1.,1.,1.,1.,1.,1.,1.,1.,1.,1.,1.,1.,1.,1.,1.,
1.,1.,1.,1.,1.,1.,1.,1.,1.,1.,1.,1.,1.,1.,1.,1.,1.,1.,1.,1.,1.,1.,1.,1.,
1.,1.,1.,1.,1.,1.,1.,1.,1.,1.,1.,1.,1.,1.,1.,1.,1.,1.,1.,1.,1.,1.,1.,1.,
1.,1.,1.,1.,1.,1.,1.,1.,1.,1.,1.,1.,1.,1.,1.,1.,1.,1.,1.,1.,1.))
REPRESENTATION_ITEM('')
);
#837=(
BOUNDED_CURVE()
B_SPLINE_CURVE(5,(#237066,#237067,#237068,#237069,#237070,#237071,#237072,
#237073,#237074,#237075,#237076,#237077,#237078,#237079,#237080,#237081,
#237082,#237083,#237084,#237085,#237086,#237087,#237088,#237089,#237090,
#237091,#237092,#237093,#237094,#237095,#237096,#237097,#237098,#237099,
#237100,#237101,#237102,#237103,#237104,#237105,#237106,#237107,#237108,
#237109,#237110,#237111,#237112,#237113,#237114,#237115,#237116,#237117,
#237118,#237119,#237120,#237121,#237122,#237123,#237124,#237125,#237126,
#237127,#237128,#237129,#237130,#237131,#237132,#237133,#237134,#237135,
#237136,#237137,#237138,#237139,#237140,#237141,#237142,#237143,#237144,
#237145,#237146,#237147,#237148,#237149,#237150,#237151,#237152,#237153,
#237154,#237155,#237156,#237157,#237158,#237159,#237160,#237161,#237162,
#237163,#237164,#237165,#237166,#237167,#237168,#237169,#237170,#237171,
#237172,#237173,#237174,#237175,#237176,#237177,#237178,#237179,#237180,
#237181,#237182,#237183,#237184,#237185,#237186,#237187,#237188,#237189,
#237190,#237191,#237192,#237193,#237194,#237195,#237196,#237197,#237198,
#237199,#237200,#237201,#237202,#237203,#237204,#237205,#237206,#237207,
#237208,#237209,#237210,#237211,#237212,#237213,#237214,#237215,#237216,
#237217,#237218,#237219,#237220,#237221,#237222,#237223,#237224,#237225,
#237226,#237227,#237228,#237229,#237230,#237231,#237232,#237233,#237234,
#237235,#237236,#237237,#237238,#237239,#237240,#237241,#237242,#237243,
#237244,#237245,#237246,#237247,#237248,#237249,#237250,#237251,#237252,
#237253,#237254,#237255,#237256,#237257,#237258,#237259,#237260,#237261,
#237262,#237263,#237264,#237265,#237266,#237267,#237268,#237269,#237270),
 .UNSPECIFIED.,.F.,.F.)
B_SPLINE_CURVE_WITH_KNOTS((6,1,1,1,1,1,1,1,1,1,1,1,1,1,1,1,1,1,1,1,1,1,
1,1,1,1,1,1,1,1,1,1,1,1,1,1,1,1,1,1,1,1,1,1,1,1,1,1,1,1,1,1,1,1,1,1,1,1,
1,1,1,1,1,1,1,1,1,1,1,1,1,1,1,1,1,1,1,1,1,1,1,1,1,1,1,1,1,1,1,1,1,1,1,1,
1,1,1,1,1,1,1,1,1,1,1,1,1,1,1,1,1,1,1,1,1,1,1,1,1,1,1,1,1,1,1,1,1,1,1,1,
1,1,1,1,1,1,1,1,1,1,1,1,1,1,1,1,1,1,1,1,1,1,1,1,1,1,1,1,1,1,1,1,1,1,1,1,
1,1,1,1,1,1,1,1,1,1,1,1,1,1,1,1,1,1,1,1,1,1,1,1,1,1,1,1,1,1,1,1,1,1,6),
(0.,0.005,0.01,0.015,0.02,0.025,0.03,0.035,0.04,0.045,0.05,0.055,0.06,0.065,
0.07,0.075,0.08,0.085,0.09,0.095,0.1,0.105,0.11,0.115,0.12,0.125,0.13,0.135,
0.14,0.145,0.15,0.155,0.16,0.165,0.17,0.175,0.18,0.185,0.19,0.195,0.2,0.205,
0.21,0.215,0.22,0.225,0.23,0.235,0.24,0.245,0.25,0.255,0.26,0.265,0.27,
0.275,0.28,0.285,0.29,0.295,0.3,0.305,0.31,0.315,0.32,0.325,0.33,0.335,
0.34,0.345,0.35,0.355,0.36,0.365,0.37,0.375,0.38,0.385,0.39,0.395,0.4,0.405,
0.41,0.415,0.42,0.425,0.43,0.435,0.44,0.445,0.45,0.455,0.46,0.465,0.47,
0.475,0.48,0.485,0.49,0.495,0.5,0.505,0.51,0.515,0.52,0.525,0.53,0.535,
0.54,0.545,0.55,0.555,0.56,0.565,0.57,0.575,0.58,0.585,0.59,0.595,0.6,0.605,
0.61,0.615,0.62,0.625,0.63,0.635,0.64,0.645,0.65,0.655,0.66,0.665,0.67,
0.675,0.68,0.685,0.690000000000001,0.695000000000001,0.700000000000001,
0.705000000000001,0.710000000000001,0.715000000000001,0.720000000000001,
0.725000000000001,0.730000000000001,0.735000000000001,0.740000000000001,
0.745000000000001,0.750000000000001,0.755000000000001,0.760000000000001,
0.765000000000001,0.770000000000001,0.775000000000001,0.780000000000001,
0.785000000000001,0.790000000000001,0.795000000000001,0.800000000000001,
0.805000000000001,0.810000000000001,0.815000000000001,0.820000000000001,
0.825000000000001,0.830000000000001,0.835000000000001,0.840000000000001,
0.845000000000001,0.850000000000001,0.855000000000001,0.860000000000001,
0.865000000000001,0.870000000000001,0.875000000000001,0.880000000000001,
0.885000000000001,0.890000000000001,0.895000000000001,0.900000000000001,
0.905000000000001,0.910000000000001,0.915000000000001,0.920000000000001,
0.925000000000001,0.930000000000001,0.935000000000001,0.940000000000001,
0.945000000000001,0.950000000000001,0.955000000000001,0.960000000000001,
0.965000000000001,0.970000000000001,0.975000000000001,0.980000000000001,
0.985000000000001,0.990000000000001,0.995000000000001,1.),.UNSPECIFIED.)
CURVE()
GEOMETRIC_REPRESENTATION_ITEM()
RATIONAL_B_SPLINE_CURVE((1.,1.,1.,1.,1.,1.,1.,1.,1.,1.,1.,1.,1.,1.,1.,1.,
1.,1.,1.,1.,1.,1.,1.,1.,1.,1.,1.,1.,1.,1.,1.,1.,1.,1.,1.,1.,1.,1.,1.,1.,
1.,1.,1.,1.,1.,1.,1.,1.,1.,1.,1.,1.,1.,1.,1.,1.,1.,1.,1.,1.,1.,1.,1.,1.,
1.,1.,1.,1.,1.,1.,1.,1.,1.,1.,1.,1.,1.,1.,1.,1.,1.,1.,1.,1.,1.,1.,1.,1.,
1.,1.,1.,1.,1.,1.,1.,1.,1.,1.,1.,1.,1.,1.,1.,1.,1.,1.,1.,1.,1.,1.,1.,1.,
1.,1.,1.,1.,1.,1.,1.,1.,1.,1.,1.,1.,1.,1.,1.,1.,1.,1.,1.,1.,1.,1.,1.,1.,
1.,1.,1.,1.,1.,1.,1.,1.,1.,1.,1.,1.,1.,1.,1.,1.,1.,1.,1.,1.,1.,1.,1.,1.,
1.,1.,1.,1.,1.,1.,1.,1.,1.,1.,1.,1.,1.,1.,1.,1.,1.,1.,1.,1.,1.,1.,1.,1.,
1.,1.,1.,1.,1.,1.,1.,1.,1.,1.,1.,1.,1.,1.,1.,1.,1.,1.,1.,1.,1.))
REPRESENTATION_ITEM('')
);
#838=(
BOUNDED_CURVE()
B_SPLINE_CURVE(5,(#237272,#237273,#237274,#237275,#237276,#237277,#237278,
#237279,#237280,#237281,#237282,#237283,#237284,#237285,#237286,#237287,
#237288,#237289,#237290,#237291,#237292,#237293,#237294,#237295,#237296,
#237297,#237298,#237299,#237300,#237301,#237302,#237303,#237304,#237305,
#237306,#237307,#237308,#237309,#237310,#237311,#237312,#237313,#237314,
#237315,#237316,#237317,#237318,#237319,#237320,#237321,#237322,#237323,
#237324,#237325,#237326,#237327,#237328,#237329,#237330,#237331,#237332,
#237333,#237334,#237335,#237336,#237337,#237338,#237339,#237340,#237341,
#237342,#237343,#237344,#237345,#237346,#237347,#237348,#237349,#237350,
#237351,#237352,#237353,#237354,#237355,#237356,#237357,#237358,#237359,
#237360,#237361,#237362,#237363,#237364,#237365,#237366,#237367,#237368,
#237369,#237370,#237371,#237372,#237373,#237374,#237375,#237376,#237377,
#237378,#237379,#237380,#237381,#237382,#237383,#237384,#237385,#237386,
#237387,#237388,#237389,#237390,#237391,#237392,#237393,#237394,#237395,
#237396,#237397,#237398,#237399,#237400,#237401,#237402,#237403,#237404,
#237405,#237406,#237407,#237408,#237409,#237410,#237411,#237412,#237413,
#237414,#237415,#237416,#237417,#237418,#237419,#237420,#237421,#237422,
#237423,#237424,#237425,#237426,#237427,#237428,#237429,#237430,#237431,
#237432,#237433,#237434,#237435,#237436,#237437,#237438,#237439,#237440,
#237441,#237442,#237443,#237444,#237445,#237446,#237447,#237448,#237449,
#237450,#237451,#237452,#237453,#237454,#237455,#237456,#237457,#237458,
#237459,#237460,#237461,#237462,#237463,#237464,#237465,#237466,#237467,
#237468,#237469,#237470,#237471,#237472,#237473,#237474,#237475,#237476),
 .UNSPECIFIED.,.F.,.F.)
B_SPLINE_CURVE_WITH_KNOTS((6,1,1,1,1,1,1,1,1,1,1,1,1,1,1,1,1,1,1,1,1,1,
1,1,1,1,1,1,1,1,1,1,1,1,1,1,1,1,1,1,1,1,1,1,1,1,1,1,1,1,1,1,1,1,1,1,1,1,
1,1,1,1,1,1,1,1,1,1,1,1,1,1,1,1,1,1,1,1,1,1,1,1,1,1,1,1,1,1,1,1,1,1,1,1,
1,1,1,1,1,1,1,1,1,1,1,1,1,1,1,1,1,1,1,1,1,1,1,1,1,1,1,1,1,1,1,1,1,1,1,1,
1,1,1,1,1,1,1,1,1,1,1,1,1,1,1,1,1,1,1,1,1,1,1,1,1,1,1,1,1,1,1,1,1,1,1,1,
1,1,1,1,1,1,1,1,1,1,1,1,1,1,1,1,1,1,1,1,1,1,1,1,1,1,1,1,1,1,1,1,1,1,6),
(-1.,-0.995000000000001,-0.990000000000001,-0.985000000000001,-0.980000000000001,
-0.975000000000001,-0.970000000000001,-0.965000000000001,-0.960000000000001,
-0.955000000000001,-0.950000000000001,-0.945000000000001,-0.940000000000001,
-0.935000000000001,-0.930000000000001,-0.925000000000001,-0.920000000000001,
-0.915000000000001,-0.910000000000001,-0.905000000000001,-0.900000000000001,
-0.895000000000001,-0.890000000000001,-0.885000000000001,-0.880000000000001,
-0.875000000000001,-0.870000000000001,-0.865000000000001,-0.860000000000001,
-0.855000000000001,-0.850000000000001,-0.845000000000001,-0.840000000000001,
-0.835000000000001,-0.830000000000001,-0.825000000000001,-0.820000000000001,
-0.815000000000001,-0.810000000000001,-0.805000000000001,-0.800000000000001,
-0.795000000000001,-0.790000000000001,-0.785000000000001,-0.780000000000001,
-0.775000000000001,-0.770000000000001,-0.765000000000001,-0.760000000000001,
-0.755000000000001,-0.750000000000001,-0.745000000000001,-0.740000000000001,
-0.735000000000001,-0.730000000000001,-0.725000000000001,-0.720000000000001,
-0.715000000000001,-0.710000000000001,-0.705000000000001,-0.700000000000001,
-0.695000000000001,-0.690000000000001,-0.685,-0.68,-0.675,-0.67,-0.665,
-0.66,-0.655,-0.65,-0.645,-0.64,-0.635,-0.63,-0.625,-0.62,-0.615,-0.61,
-0.605,-0.6,-0.595,-0.59,-0.585,-0.58,-0.575,-0.57,-0.565,-0.56,-0.555,
-0.55,-0.545,-0.54,-0.535,-0.53,-0.525,-0.52,-0.515,-0.51,-0.505,-0.5,-0.495,
-0.49,-0.485,-0.48,-0.475,-0.47,-0.465,-0.46,-0.455,-0.45,-0.445,-0.44,
-0.435,-0.43,-0.425,-0.42,-0.415,-0.41,-0.405,-0.4,-0.395,-0.39,-0.385,
-0.38,-0.375,-0.37,-0.365,-0.36,-0.355,-0.35,-0.345,-0.34,-0.335,-0.33,
-0.325,-0.32,-0.315,-0.31,-0.305,-0.3,-0.295,-0.29,-0.285,-0.28,-0.275,
-0.27,-0.265,-0.26,-0.255,-0.25,-0.245,-0.24,-0.235,-0.23,-0.225,-0.22,
-0.215,-0.21,-0.205,-0.2,-0.195,-0.19,-0.185,-0.18,-0.175,-0.17,-0.165,
-0.16,-0.155,-0.15,-0.145,-0.14,-0.135,-0.13,-0.125,-0.12,-0.115,-0.11,
-0.105,-0.1,-0.095,-0.09,-0.085,-0.08,-0.075,-0.07,-0.065,-0.06,-0.055,
-0.05,-0.045,-0.04,-0.035,-0.03,-0.025,-0.02,-0.015,-0.01,-0.005,0.),
 .UNSPECIFIED.)
CURVE()
GEOMETRIC_REPRESENTATION_ITEM()
RATIONAL_B_SPLINE_CURVE((1.,1.,1.,1.,1.,1.,1.,1.,1.,1.,1.,1.,1.,1.,1.,1.,
1.,1.,1.,1.,1.,1.,1.,1.,1.,1.,1.,1.,1.,1.,1.,1.,1.,1.,1.,1.,1.,1.,1.,1.,
1.,1.,1.,1.,1.,1.,1.,1.,1.,1.,1.,1.,1.,1.,1.,1.,1.,1.,1.,1.,1.,1.,1.,1.,
1.,1.,1.,1.,1.,1.,1.,1.,1.,1.,1.,1.,1.,1.,1.,1.,1.,1.,1.,1.,1.,1.,1.,1.,
1.,1.,1.,1.,1.,1.,1.,1.,1.,1.,1.,1.,1.,1.,1.,1.,1.,1.,1.,1.,1.,1.,1.,1.,
1.,1.,1.,1.,1.,1.,1.,1.,1.,1.,1.,1.,1.,1.,1.,1.,1.,1.,1.,1.,1.,1.,1.,1.,
1.,1.,1.,1.,1.,1.,1.,1.,1.,1.,1.,1.,1.,1.,1.,1.,1.,1.,1.,1.,1.,1.,1.,1.,
1.,1.,1.,1.,1.,1.,1.,1.,1.,1.,1.,1.,1.,1.,1.,1.,1.,1.,1.,1.,1.,1.,1.,1.,
1.,1.,1.,1.,1.,1.,1.,1.,1.,1.,1.,1.,1.,1.,1.,1.,1.,1.,1.,1.,1.))
REPRESENTATION_ITEM('')
);
#839=(
BOUNDED_CURVE()
B_SPLINE_CURVE(5,(#237895,#237896,#237897,#237898,#237899,#237900,#237901,
#237902,#237903,#237904,#237905,#237906,#237907,#237908,#237909,#237910,
#237911,#237912,#237913,#237914,#237915,#237916,#237917,#237918,#237919,
#237920,#237921,#237922,#237923,#237924,#237925,#237926,#237927,#237928,
#237929,#237930,#237931,#237932,#237933,#237934,#237935,#237936,#237937,
#237938,#237939,#237940,#237941,#237942,#237943,#237944,#237945,#237946,
#237947,#237948,#237949,#237950,#237951,#237952,#237953,#237954,#237955,
#237956,#237957,#237958,#237959,#237960,#237961,#237962,#237963,#237964,
#237965,#237966,#237967,#237968,#237969,#237970,#237971,#237972,#237973,
#237974,#237975,#237976,#237977,#237978,#237979,#237980,#237981,#237982,
#237983,#237984,#237985,#237986,#237987,#237988,#237989,#237990,#237991,
#237992,#237993,#237994,#237995,#237996,#237997,#237998,#237999,#238000,
#238001,#238002,#238003,#238004,#238005,#238006,#238007,#238008,#238009,
#238010,#238011,#238012,#238013,#238014,#238015,#238016,#238017,#238018,
#238019,#238020,#238021,#238022,#238023,#238024,#238025,#238026,#238027,
#238028,#238029,#238030,#238031,#238032,#238033,#238034,#238035,#238036,
#238037,#238038,#238039,#238040,#238041,#238042,#238043,#238044,#238045,
#238046,#238047,#238048,#238049,#238050,#238051,#238052,#238053,#238054,
#238055,#238056,#238057,#238058,#238059,#238060,#238061,#238062,#238063,
#238064,#238065,#238066,#238067,#238068,#238069,#238070,#238071,#238072,
#238073,#238074,#238075,#238076,#238077,#238078,#238079,#238080,#238081,
#238082,#238083,#238084,#238085,#238086,#238087,#238088,#238089,#238090,
#238091,#238092,#238093,#238094,#238095,#238096,#238097,#238098,#238099),
 .UNSPECIFIED.,.F.,.F.)
B_SPLINE_CURVE_WITH_KNOTS((6,1,1,1,1,1,1,1,1,1,1,1,1,1,1,1,1,1,1,1,1,1,
1,1,1,1,1,1,1,1,1,1,1,1,1,1,1,1,1,1,1,1,1,1,1,1,1,1,1,1,1,1,1,1,1,1,1,1,
1,1,1,1,1,1,1,1,1,1,1,1,1,1,1,1,1,1,1,1,1,1,1,1,1,1,1,1,1,1,1,1,1,1,1,1,
1,1,1,1,1,1,1,1,1,1,1,1,1,1,1,1,1,1,1,1,1,1,1,1,1,1,1,1,1,1,1,1,1,1,1,1,
1,1,1,1,1,1,1,1,1,1,1,1,1,1,1,1,1,1,1,1,1,1,1,1,1,1,1,1,1,1,1,1,1,1,1,1,
1,1,1,1,1,1,1,1,1,1,1,1,1,1,1,1,1,1,1,1,1,1,1,1,1,1,1,1,1,1,1,1,1,1,6),
(-1.,-0.995000000000001,-0.990000000000001,-0.985000000000001,-0.980000000000001,
-0.975000000000001,-0.970000000000001,-0.965000000000001,-0.960000000000001,
-0.955000000000001,-0.950000000000001,-0.945000000000001,-0.940000000000001,
-0.935000000000001,-0.930000000000001,-0.925000000000001,-0.920000000000001,
-0.915000000000001,-0.910000000000001,-0.905000000000001,-0.900000000000001,
-0.895000000000001,-0.890000000000001,-0.885000000000001,-0.880000000000001,
-0.875000000000001,-0.870000000000001,-0.865000000000001,-0.860000000000001,
-0.855000000000001,-0.850000000000001,-0.845000000000001,-0.840000000000001,
-0.835000000000001,-0.830000000000001,-0.825000000000001,-0.820000000000001,
-0.815000000000001,-0.810000000000001,-0.805000000000001,-0.800000000000001,
-0.795000000000001,-0.790000000000001,-0.785000000000001,-0.780000000000001,
-0.775000000000001,-0.770000000000001,-0.765000000000001,-0.760000000000001,
-0.755000000000001,-0.750000000000001,-0.745000000000001,-0.740000000000001,
-0.735000000000001,-0.730000000000001,-0.725000000000001,-0.720000000000001,
-0.715000000000001,-0.710000000000001,-0.705000000000001,-0.700000000000001,
-0.695000000000001,-0.690000000000001,-0.685,-0.68,-0.675,-0.67,-0.665,
-0.66,-0.655,-0.65,-0.645,-0.64,-0.635,-0.63,-0.625,-0.62,-0.615,-0.61,
-0.605,-0.6,-0.595,-0.59,-0.585,-0.58,-0.575,-0.57,-0.565,-0.56,-0.555,
-0.55,-0.545,-0.54,-0.535,-0.53,-0.525,-0.52,-0.515,-0.51,-0.505,-0.5,-0.495,
-0.49,-0.485,-0.48,-0.475,-0.47,-0.465,-0.46,-0.455,-0.45,-0.445,-0.44,
-0.435,-0.43,-0.425,-0.42,-0.415,-0.41,-0.405,-0.4,-0.395,-0.39,-0.385,
-0.38,-0.375,-0.37,-0.365,-0.36,-0.355,-0.35,-0.345,-0.34,-0.335,-0.33,
-0.325,-0.32,-0.315,-0.31,-0.305,-0.3,-0.295,-0.29,-0.285,-0.28,-0.275,
-0.27,-0.265,-0.26,-0.255,-0.25,-0.245,-0.24,-0.235,-0.23,-0.225,-0.22,
-0.215,-0.21,-0.205,-0.2,-0.195,-0.19,-0.185,-0.18,-0.175,-0.17,-0.165,
-0.16,-0.155,-0.15,-0.145,-0.14,-0.135,-0.13,-0.125,-0.12,-0.115,-0.11,
-0.105,-0.1,-0.095,-0.09,-0.085,-0.08,-0.075,-0.07,-0.065,-0.06,-0.055,
-0.05,-0.045,-0.04,-0.035,-0.03,-0.025,-0.02,-0.015,-0.01,-0.005,0.),
 .UNSPECIFIED.)
CURVE()
GEOMETRIC_REPRESENTATION_ITEM()
RATIONAL_B_SPLINE_CURVE((1.,1.,1.,1.,1.,1.,1.,1.,1.,1.,1.,1.,1.,1.,1.,1.,
1.,1.,1.,1.,1.,1.,1.,1.,1.,1.,1.,1.,1.,1.,1.,1.,1.,1.,1.,1.,1.,1.,1.,1.,
1.,1.,1.,1.,1.,1.,1.,1.,1.,1.,1.,1.,1.,1.,1.,1.,1.,1.,1.,1.,1.,1.,1.,1.,
1.,1.,1.,1.,1.,1.,1.,1.,1.,1.,1.,1.,1.,1.,1.,1.,1.,1.,1.,1.,1.,1.,1.,1.,
1.,1.,1.,1.,1.,1.,1.,1.,1.,1.,1.,1.,1.,1.,1.,1.,1.,1.,1.,1.,1.,1.,1.,1.,
1.,1.,1.,1.,1.,1.,1.,1.,1.,1.,1.,1.,1.,1.,1.,1.,1.,1.,1.,1.,1.,1.,1.,1.,
1.,1.,1.,1.,1.,1.,1.,1.,1.,1.,1.,1.,1.,1.,1.,1.,1.,1.,1.,1.,1.,1.,1.,1.,
1.,1.,1.,1.,1.,1.,1.,1.,1.,1.,1.,1.,1.,1.,1.,1.,1.,1.,1.,1.,1.,1.,1.,1.,
1.,1.,1.,1.,1.,1.,1.,1.,1.,1.,1.,1.,1.,1.,1.,1.,1.,1.,1.,1.,1.))
REPRESENTATION_ITEM('')
);
#840=(
BOUNDED_CURVE()
B_SPLINE_CURVE(5,(#238102,#238103,#238104,#238105,#238106,#238107,#238108,
#238109,#238110,#238111,#238112,#238113,#238114,#238115,#238116,#238117,
#238118,#238119,#238120,#238121,#238122,#238123,#238124,#238125,#238126,
#238127,#238128,#238129,#238130,#238131,#238132,#238133,#238134,#238135,
#238136,#238137,#238138,#238139,#238140,#238141,#238142,#238143,#238144,
#238145,#238146,#238147,#238148,#238149,#238150,#238151,#238152,#238153,
#238154,#238155,#238156,#238157,#238158,#238159,#238160,#238161,#238162,
#238163,#238164,#238165,#238166,#238167,#238168,#238169,#238170,#238171,
#238172,#238173,#238174,#238175,#238176,#238177,#238178,#238179,#238180,
#238181,#238182,#238183,#238184,#238185,#238186,#238187,#238188,#238189,
#238190,#238191,#238192,#238193,#238194,#238195,#238196,#238197,#238198,
#238199,#238200,#238201,#238202,#238203,#238204,#238205,#238206,#238207,
#238208,#238209,#238210,#238211,#238212,#238213,#238214,#238215,#238216,
#238217,#238218,#238219,#238220,#238221,#238222,#238223,#238224,#238225,
#238226,#238227,#238228,#238229,#238230,#238231,#238232,#238233,#238234,
#238235,#238236,#238237,#238238,#238239,#238240,#238241,#238242,#238243,
#238244,#238245,#238246,#238247,#238248,#238249,#238250,#238251,#238252,
#238253,#238254,#238255,#238256,#238257,#238258,#238259,#238260,#238261,
#238262,#238263,#238264,#238265,#238266,#238267,#238268,#238269,#238270,
#238271,#238272,#238273,#238274,#238275,#238276,#238277,#238278,#238279,
#238280,#238281,#238282,#238283,#238284,#238285,#238286,#238287,#238288,
#238289,#238290,#238291,#238292,#238293,#238294,#238295,#238296,#238297,
#238298,#238299,#238300,#238301,#238302,#238303,#238304,#238305,#238306),
 .UNSPECIFIED.,.F.,.F.)
B_SPLINE_CURVE_WITH_KNOTS((6,1,1,1,1,1,1,1,1,1,1,1,1,1,1,1,1,1,1,1,1,1,
1,1,1,1,1,1,1,1,1,1,1,1,1,1,1,1,1,1,1,1,1,1,1,1,1,1,1,1,1,1,1,1,1,1,1,1,
1,1,1,1,1,1,1,1,1,1,1,1,1,1,1,1,1,1,1,1,1,1,1,1,1,1,1,1,1,1,1,1,1,1,1,1,
1,1,1,1,1,1,1,1,1,1,1,1,1,1,1,1,1,1,1,1,1,1,1,1,1,1,1,1,1,1,1,1,1,1,1,1,
1,1,1,1,1,1,1,1,1,1,1,1,1,1,1,1,1,1,1,1,1,1,1,1,1,1,1,1,1,1,1,1,1,1,1,1,
1,1,1,1,1,1,1,1,1,1,1,1,1,1,1,1,1,1,1,1,1,1,1,1,1,1,1,1,1,1,1,1,1,1,6),
(0.,0.005,0.01,0.015,0.02,0.025,0.03,0.035,0.04,0.045,0.05,0.055,0.06,0.065,
0.07,0.075,0.08,0.085,0.09,0.095,0.1,0.105,0.11,0.115,0.12,0.125,0.13,0.135,
0.14,0.145,0.15,0.155,0.16,0.165,0.17,0.175,0.18,0.185,0.19,0.195,0.2,0.205,
0.21,0.215,0.22,0.225,0.23,0.235,0.24,0.245,0.25,0.255,0.26,0.265,0.27,
0.275,0.28,0.285,0.29,0.295,0.3,0.305,0.31,0.315,0.32,0.325,0.33,0.335,
0.34,0.345,0.35,0.355,0.36,0.365,0.37,0.375,0.38,0.385,0.39,0.395,0.4,0.405,
0.41,0.415,0.42,0.425,0.43,0.435,0.44,0.445,0.45,0.455,0.46,0.465,0.47,
0.475,0.48,0.485,0.49,0.495,0.5,0.505,0.51,0.515,0.52,0.525,0.53,0.535,
0.54,0.545,0.55,0.555,0.56,0.565,0.57,0.575,0.58,0.585,0.59,0.595,0.6,0.605,
0.61,0.615,0.62,0.625,0.63,0.635,0.64,0.645,0.65,0.655,0.66,0.665,0.67,
0.675,0.68,0.685,0.690000000000001,0.695000000000001,0.700000000000001,
0.705000000000001,0.710000000000001,0.715000000000001,0.720000000000001,
0.725000000000001,0.730000000000001,0.735000000000001,0.740000000000001,
0.745000000000001,0.750000000000001,0.755000000000001,0.760000000000001,
0.765000000000001,0.770000000000001,0.775000000000001,0.780000000000001,
0.785000000000001,0.790000000000001,0.795000000000001,0.800000000000001,
0.805000000000001,0.810000000000001,0.815000000000001,0.820000000000001,
0.825000000000001,0.830000000000001,0.835000000000001,0.840000000000001,
0.845000000000001,0.850000000000001,0.855000000000001,0.860000000000001,
0.865000000000001,0.870000000000001,0.875000000000001,0.880000000000001,
0.885000000000001,0.890000000000001,0.895000000000001,0.900000000000001,
0.905000000000001,0.910000000000001,0.915000000000001,0.920000000000001,
0.925000000000001,0.930000000000001,0.935000000000001,0.940000000000001,
0.945000000000001,0.950000000000001,0.955000000000001,0.960000000000001,
0.965000000000001,0.970000000000001,0.975000000000001,0.980000000000001,
0.985000000000001,0.990000000000001,0.995000000000001,1.),.UNSPECIFIED.)
CURVE()
GEOMETRIC_REPRESENTATION_ITEM()
RATIONAL_B_SPLINE_CURVE((1.,1.,1.,1.,1.,1.,1.,1.,1.,1.,1.,1.,1.,1.,1.,1.,
1.,1.,1.,1.,1.,1.,1.,1.,1.,1.,1.,1.,1.,1.,1.,1.,1.,1.,1.,1.,1.,1.,1.,1.,
1.,1.,1.,1.,1.,1.,1.,1.,1.,1.,1.,1.,1.,1.,1.,1.,1.,1.,1.,1.,1.,1.,1.,1.,
1.,1.,1.,1.,1.,1.,1.,1.,1.,1.,1.,1.,1.,1.,1.,1.,1.,1.,1.,1.,1.,1.,1.,1.,
1.,1.,1.,1.,1.,1.,1.,1.,1.,1.,1.,1.,1.,1.,1.,1.,1.,1.,1.,1.,1.,1.,1.,1.,
1.,1.,1.,1.,1.,1.,1.,1.,1.,1.,1.,1.,1.,1.,1.,1.,1.,1.,1.,1.,1.,1.,1.,1.,
1.,1.,1.,1.,1.,1.,1.,1.,1.,1.,1.,1.,1.,1.,1.,1.,1.,1.,1.,1.,1.,1.,1.,1.,
1.,1.,1.,1.,1.,1.,1.,1.,1.,1.,1.,1.,1.,1.,1.,1.,1.,1.,1.,1.,1.,1.,1.,1.,
1.,1.,1.,1.,1.,1.,1.,1.,1.,1.,1.,1.,1.,1.,1.,1.,1.,1.,1.,1.,1.))
REPRESENTATION_ITEM('')
);
#841=(
BOUNDED_CURVE()
B_SPLINE_CURVE(5,(#238718,#238719,#238720,#238721,#238722,#238723,#238724,
#238725,#238726,#238727,#238728,#238729,#238730,#238731,#238732,#238733,
#238734,#238735,#238736,#238737,#238738,#238739,#238740,#238741,#238742,
#238743,#238744,#238745,#238746,#238747,#238748,#238749,#238750,#238751,
#238752,#238753,#238754,#238755,#238756,#238757,#238758,#238759,#238760,
#238761,#238762,#238763,#238764,#238765,#238766,#238767,#238768,#238769,
#238770,#238771,#238772,#238773,#238774,#238775,#238776,#238777,#238778,
#238779,#238780,#238781,#238782,#238783,#238784,#238785,#238786,#238787,
#238788,#238789,#238790,#238791,#238792,#238793,#238794,#238795,#238796,
#238797,#238798,#238799,#238800,#238801,#238802,#238803,#238804,#238805,
#238806,#238807,#238808,#238809,#238810,#238811,#238812,#238813,#238814,
#238815,#238816,#238817,#238818,#238819,#238820,#238821,#238822,#238823,
#238824,#238825,#238826,#238827,#238828,#238829,#238830,#238831,#238832,
#238833,#238834,#238835,#238836,#238837,#238838,#238839,#238840,#238841,
#238842,#238843,#238844,#238845,#238846,#238847,#238848,#238849,#238850,
#238851,#238852,#238853,#238854,#238855,#238856,#238857,#238858,#238859,
#238860,#238861,#238862,#238863,#238864,#238865,#238866,#238867,#238868,
#238869,#238870,#238871,#238872,#238873,#238874,#238875,#238876,#238877,
#238878,#238879,#238880,#238881,#238882,#238883,#238884,#238885,#238886,
#238887,#238888,#238889,#238890,#238891,#238892,#238893,#238894,#238895,
#238896,#238897,#238898,#238899,#238900,#238901,#238902,#238903,#238904,
#238905,#238906,#238907,#238908,#238909,#238910,#238911,#238912,#238913,
#238914,#238915,#238916,#238917,#238918,#238919,#238920,#238921,#238922),
 .UNSPECIFIED.,.F.,.F.)
B_SPLINE_CURVE_WITH_KNOTS((6,1,1,1,1,1,1,1,1,1,1,1,1,1,1,1,1,1,1,1,1,1,
1,1,1,1,1,1,1,1,1,1,1,1,1,1,1,1,1,1,1,1,1,1,1,1,1,1,1,1,1,1,1,1,1,1,1,1,
1,1,1,1,1,1,1,1,1,1,1,1,1,1,1,1,1,1,1,1,1,1,1,1,1,1,1,1,1,1,1,1,1,1,1,1,
1,1,1,1,1,1,1,1,1,1,1,1,1,1,1,1,1,1,1,1,1,1,1,1,1,1,1,1,1,1,1,1,1,1,1,1,
1,1,1,1,1,1,1,1,1,1,1,1,1,1,1,1,1,1,1,1,1,1,1,1,1,1,1,1,1,1,1,1,1,1,1,1,
1,1,1,1,1,1,1,1,1,1,1,1,1,1,1,1,1,1,1,1,1,1,1,1,1,1,1,1,1,1,1,1,1,1,6),
(0.,0.005,0.01,0.015,0.02,0.025,0.03,0.035,0.04,0.045,0.05,0.055,0.06,0.065,
0.07,0.075,0.08,0.085,0.09,0.095,0.1,0.105,0.11,0.115,0.12,0.125,0.13,0.135,
0.14,0.145,0.15,0.155,0.16,0.165,0.17,0.175,0.18,0.185,0.19,0.195,0.2,0.205,
0.21,0.215,0.22,0.225,0.23,0.235,0.24,0.245,0.25,0.255,0.26,0.265,0.27,
0.275,0.28,0.285,0.29,0.295,0.3,0.305,0.31,0.315,0.32,0.325,0.33,0.335,
0.34,0.345,0.35,0.355,0.36,0.365,0.37,0.375,0.38,0.385,0.39,0.395,0.4,0.405,
0.41,0.415,0.42,0.425,0.43,0.435,0.44,0.445,0.45,0.455,0.46,0.465,0.47,
0.475,0.48,0.485,0.49,0.495,0.5,0.505,0.51,0.515,0.52,0.525,0.53,0.535,
0.54,0.545,0.55,0.555,0.56,0.565,0.57,0.575,0.58,0.585,0.59,0.595,0.6,0.605,
0.61,0.615,0.62,0.625,0.63,0.635,0.64,0.645,0.65,0.655,0.66,0.665,0.67,
0.675,0.68,0.685,0.690000000000001,0.695000000000001,0.700000000000001,
0.705000000000001,0.710000000000001,0.715000000000001,0.720000000000001,
0.725000000000001,0.730000000000001,0.735000000000001,0.740000000000001,
0.745000000000001,0.750000000000001,0.755000000000001,0.760000000000001,
0.765000000000001,0.770000000000001,0.775000000000001,0.780000000000001,
0.785000000000001,0.790000000000001,0.795000000000001,0.800000000000001,
0.805000000000001,0.810000000000001,0.815000000000001,0.820000000000001,
0.825000000000001,0.830000000000001,0.835000000000001,0.840000000000001,
0.845000000000001,0.850000000000001,0.855000000000001,0.860000000000001,
0.865000000000001,0.870000000000001,0.875000000000001,0.880000000000001,
0.885000000000001,0.890000000000001,0.895000000000001,0.900000000000001,
0.905000000000001,0.910000000000001,0.915000000000001,0.920000000000001,
0.925000000000001,0.930000000000001,0.935000000000001,0.940000000000001,
0.945000000000001,0.950000000000001,0.955000000000001,0.960000000000001,
0.965000000000001,0.970000000000001,0.975000000000001,0.980000000000001,
0.985000000000001,0.990000000000001,0.995000000000001,1.),.UNSPECIFIED.)
CURVE()
GEOMETRIC_REPRESENTATION_ITEM()
RATIONAL_B_SPLINE_CURVE((1.,1.,1.,1.,1.,1.,1.,1.,1.,1.,1.,1.,1.,1.,1.,1.,
1.,1.,1.,1.,1.,1.,1.,1.,1.,1.,1.,1.,1.,1.,1.,1.,1.,1.,1.,1.,1.,1.,1.,1.,
1.,1.,1.,1.,1.,1.,1.,1.,1.,1.,1.,1.,1.,1.,1.,1.,1.,1.,1.,1.,1.,1.,1.,1.,
1.,1.,1.,1.,1.,1.,1.,1.,1.,1.,1.,1.,1.,1.,1.,1.,1.,1.,1.,1.,1.,1.,1.,1.,
1.,1.,1.,1.,1.,1.,1.,1.,1.,1.,1.,1.,1.,1.,1.,1.,1.,1.,1.,1.,1.,1.,1.,1.,
1.,1.,1.,1.,1.,1.,1.,1.,1.,1.,1.,1.,1.,1.,1.,1.,1.,1.,1.,1.,1.,1.,1.,1.,
1.,1.,1.,1.,1.,1.,1.,1.,1.,1.,1.,1.,1.,1.,1.,1.,1.,1.,1.,1.,1.,1.,1.,1.,
1.,1.,1.,1.,1.,1.,1.,1.,1.,1.,1.,1.,1.,1.,1.,1.,1.,1.,1.,1.,1.,1.,1.,1.,
1.,1.,1.,1.,1.,1.,1.,1.,1.,1.,1.,1.,1.,1.,1.,1.,1.,1.,1.,1.,1.))
REPRESENTATION_ITEM('')
);
#842=(
BOUNDED_CURVE()
B_SPLINE_CURVE(5,(#238924,#238925,#238926,#238927,#238928,#238929,#238930,
#238931,#238932,#238933,#238934,#238935,#238936,#238937,#238938,#238939,
#238940,#238941,#238942,#238943,#238944,#238945,#238946,#238947,#238948,
#238949,#238950,#238951,#238952,#238953,#238954,#238955,#238956,#238957,
#238958,#238959,#238960,#238961,#238962,#238963,#238964,#238965,#238966,
#238967,#238968,#238969,#238970,#238971,#238972,#238973,#238974,#238975,
#238976,#238977,#238978,#238979,#238980,#238981,#238982,#238983,#238984,
#238985,#238986,#238987,#238988,#238989,#238990,#238991,#238992,#238993,
#238994,#238995,#238996,#238997,#238998,#238999,#239000,#239001,#239002,
#239003,#239004,#239005,#239006,#239007,#239008,#239009,#239010,#239011,
#239012,#239013,#239014,#239015,#239016,#239017,#239018,#239019,#239020,
#239021,#239022,#239023,#239024,#239025,#239026,#239027,#239028,#239029,
#239030,#239031,#239032,#239033,#239034,#239035,#239036,#239037,#239038,
#239039,#239040,#239041,#239042,#239043,#239044,#239045,#239046,#239047,
#239048,#239049,#239050,#239051,#239052,#239053,#239054,#239055,#239056,
#239057,#239058,#239059,#239060,#239061,#239062,#239063,#239064,#239065,
#239066,#239067,#239068,#239069,#239070,#239071,#239072,#239073,#239074,
#239075,#239076,#239077,#239078,#239079,#239080,#239081,#239082,#239083,
#239084,#239085,#239086,#239087,#239088,#239089,#239090,#239091,#239092,
#239093,#239094,#239095,#239096,#239097,#239098,#239099,#239100,#239101,
#239102,#239103,#239104,#239105,#239106,#239107,#239108,#239109,#239110,
#239111,#239112,#239113,#239114,#239115,#239116,#239117,#239118,#239119,
#239120,#239121,#239122,#239123,#239124,#239125,#239126,#239127,#239128),
 .UNSPECIFIED.,.F.,.F.)
B_SPLINE_CURVE_WITH_KNOTS((6,1,1,1,1,1,1,1,1,1,1,1,1,1,1,1,1,1,1,1,1,1,
1,1,1,1,1,1,1,1,1,1,1,1,1,1,1,1,1,1,1,1,1,1,1,1,1,1,1,1,1,1,1,1,1,1,1,1,
1,1,1,1,1,1,1,1,1,1,1,1,1,1,1,1,1,1,1,1,1,1,1,1,1,1,1,1,1,1,1,1,1,1,1,1,
1,1,1,1,1,1,1,1,1,1,1,1,1,1,1,1,1,1,1,1,1,1,1,1,1,1,1,1,1,1,1,1,1,1,1,1,
1,1,1,1,1,1,1,1,1,1,1,1,1,1,1,1,1,1,1,1,1,1,1,1,1,1,1,1,1,1,1,1,1,1,1,1,
1,1,1,1,1,1,1,1,1,1,1,1,1,1,1,1,1,1,1,1,1,1,1,1,1,1,1,1,1,1,1,1,1,1,6),
(-1.,-0.995000000000001,-0.990000000000001,-0.985000000000001,-0.980000000000001,
-0.975000000000001,-0.970000000000001,-0.965000000000001,-0.960000000000001,
-0.955000000000001,-0.950000000000001,-0.945000000000001,-0.940000000000001,
-0.935000000000001,-0.930000000000001,-0.925000000000001,-0.920000000000001,
-0.915000000000001,-0.910000000000001,-0.905000000000001,-0.900000000000001,
-0.895000000000001,-0.890000000000001,-0.885000000000001,-0.880000000000001,
-0.875000000000001,-0.870000000000001,-0.865000000000001,-0.860000000000001,
-0.855000000000001,-0.850000000000001,-0.845000000000001,-0.840000000000001,
-0.835000000000001,-0.830000000000001,-0.825000000000001,-0.820000000000001,
-0.815000000000001,-0.810000000000001,-0.805000000000001,-0.800000000000001,
-0.795000000000001,-0.790000000000001,-0.785000000000001,-0.780000000000001,
-0.775000000000001,-0.770000000000001,-0.765000000000001,-0.760000000000001,
-0.755000000000001,-0.750000000000001,-0.745000000000001,-0.740000000000001,
-0.735000000000001,-0.730000000000001,-0.725000000000001,-0.720000000000001,
-0.715000000000001,-0.710000000000001,-0.705000000000001,-0.700000000000001,
-0.695000000000001,-0.690000000000001,-0.685,-0.68,-0.675,-0.67,-0.665,
-0.66,-0.655,-0.65,-0.645,-0.64,-0.635,-0.63,-0.625,-0.62,-0.615,-0.61,
-0.605,-0.6,-0.595,-0.59,-0.585,-0.58,-0.575,-0.57,-0.565,-0.56,-0.555,
-0.55,-0.545,-0.54,-0.535,-0.53,-0.525,-0.52,-0.515,-0.51,-0.505,-0.5,-0.495,
-0.49,-0.485,-0.48,-0.475,-0.47,-0.465,-0.46,-0.455,-0.45,-0.445,-0.44,
-0.435,-0.43,-0.425,-0.42,-0.415,-0.41,-0.405,-0.4,-0.395,-0.39,-0.385,
-0.38,-0.375,-0.37,-0.365,-0.36,-0.355,-0.35,-0.345,-0.34,-0.335,-0.33,
-0.325,-0.32,-0.315,-0.31,-0.305,-0.3,-0.295,-0.29,-0.285,-0.28,-0.275,
-0.27,-0.265,-0.26,-0.255,-0.25,-0.245,-0.24,-0.235,-0.23,-0.225,-0.22,
-0.215,-0.21,-0.205,-0.2,-0.195,-0.19,-0.185,-0.18,-0.175,-0.17,-0.165,
-0.16,-0.155,-0.15,-0.145,-0.14,-0.135,-0.13,-0.125,-0.12,-0.115,-0.11,
-0.105,-0.1,-0.095,-0.09,-0.085,-0.08,-0.075,-0.07,-0.065,-0.06,-0.055,
-0.05,-0.045,-0.04,-0.035,-0.03,-0.025,-0.02,-0.015,-0.01,-0.005,0.),
 .UNSPECIFIED.)
CURVE()
GEOMETRIC_REPRESENTATION_ITEM()
RATIONAL_B_SPLINE_CURVE((1.,1.,1.,1.,1.,1.,1.,1.,1.,1.,1.,1.,1.,1.,1.,1.,
1.,1.,1.,1.,1.,1.,1.,1.,1.,1.,1.,1.,1.,1.,1.,1.,1.,1.,1.,1.,1.,1.,1.,1.,
1.,1.,1.,1.,1.,1.,1.,1.,1.,1.,1.,1.,1.,1.,1.,1.,1.,1.,1.,1.,1.,1.,1.,1.,
1.,1.,1.,1.,1.,1.,1.,1.,1.,1.,1.,1.,1.,1.,1.,1.,1.,1.,1.,1.,1.,1.,1.,1.,
1.,1.,1.,1.,1.,1.,1.,1.,1.,1.,1.,1.,1.,1.,1.,1.,1.,1.,1.,1.,1.,1.,1.,1.,
1.,1.,1.,1.,1.,1.,1.,1.,1.,1.,1.,1.,1.,1.,1.,1.,1.,1.,1.,1.,1.,1.,1.,1.,
1.,1.,1.,1.,1.,1.,1.,1.,1.,1.,1.,1.,1.,1.,1.,1.,1.,1.,1.,1.,1.,1.,1.,1.,
1.,1.,1.,1.,1.,1.,1.,1.,1.,1.,1.,1.,1.,1.,1.,1.,1.,1.,1.,1.,1.,1.,1.,1.,
1.,1.,1.,1.,1.,1.,1.,1.,1.,1.,1.,1.,1.,1.,1.,1.,1.,1.,1.,1.,1.))
REPRESENTATION_ITEM('')
);
#843=(
BOUNDED_CURVE()
B_SPLINE_CURVE(5,(#239547,#239548,#239549,#239550,#239551,#239552,#239553,
#239554,#239555,#239556,#239557,#239558,#239559,#239560,#239561,#239562,
#239563,#239564,#239565,#239566,#239567,#239568,#239569,#239570,#239571,
#239572,#239573,#239574,#239575,#239576,#239577,#239578,#239579,#239580,
#239581,#239582,#239583,#239584,#239585,#239586,#239587,#239588,#239589,
#239590,#239591,#239592,#239593,#239594,#239595,#239596,#239597,#239598,
#239599,#239600,#239601,#239602,#239603,#239604,#239605,#239606,#239607,
#239608,#239609,#239610,#239611,#239612,#239613,#239614,#239615,#239616,
#239617,#239618,#239619,#239620,#239621,#239622,#239623,#239624,#239625,
#239626,#239627,#239628,#239629,#239630,#239631,#239632,#239633,#239634,
#239635,#239636,#239637,#239638,#239639,#239640,#239641,#239642,#239643,
#239644,#239645,#239646,#239647,#239648,#239649,#239650,#239651,#239652,
#239653,#239654,#239655,#239656,#239657,#239658,#239659,#239660,#239661,
#239662,#239663,#239664,#239665,#239666,#239667,#239668,#239669,#239670,
#239671,#239672,#239673,#239674,#239675,#239676,#239677,#239678,#239679,
#239680,#239681,#239682,#239683,#239684,#239685,#239686,#239687,#239688,
#239689,#239690,#239691,#239692,#239693,#239694,#239695,#239696,#239697,
#239698,#239699,#239700,#239701,#239702,#239703,#239704,#239705,#239706,
#239707,#239708,#239709,#239710,#239711,#239712,#239713,#239714,#239715,
#239716,#239717,#239718,#239719,#239720,#239721,#239722,#239723,#239724,
#239725,#239726,#239727,#239728,#239729,#239730,#239731,#239732,#239733,
#239734,#239735,#239736,#239737,#239738,#239739,#239740,#239741,#239742,
#239743,#239744,#239745,#239746,#239747,#239748,#239749,#239750,#239751),
 .UNSPECIFIED.,.F.,.F.)
B_SPLINE_CURVE_WITH_KNOTS((6,1,1,1,1,1,1,1,1,1,1,1,1,1,1,1,1,1,1,1,1,1,
1,1,1,1,1,1,1,1,1,1,1,1,1,1,1,1,1,1,1,1,1,1,1,1,1,1,1,1,1,1,1,1,1,1,1,1,
1,1,1,1,1,1,1,1,1,1,1,1,1,1,1,1,1,1,1,1,1,1,1,1,1,1,1,1,1,1,1,1,1,1,1,1,
1,1,1,1,1,1,1,1,1,1,1,1,1,1,1,1,1,1,1,1,1,1,1,1,1,1,1,1,1,1,1,1,1,1,1,1,
1,1,1,1,1,1,1,1,1,1,1,1,1,1,1,1,1,1,1,1,1,1,1,1,1,1,1,1,1,1,1,1,1,1,1,1,
1,1,1,1,1,1,1,1,1,1,1,1,1,1,1,1,1,1,1,1,1,1,1,1,1,1,1,1,1,1,1,1,1,1,6),
(-1.,-0.995000000000001,-0.990000000000001,-0.985000000000001,-0.980000000000001,
-0.975000000000001,-0.970000000000001,-0.965000000000001,-0.960000000000001,
-0.955000000000001,-0.950000000000001,-0.945000000000001,-0.940000000000001,
-0.935000000000001,-0.930000000000001,-0.925000000000001,-0.920000000000001,
-0.915000000000001,-0.910000000000001,-0.905000000000001,-0.900000000000001,
-0.895000000000001,-0.890000000000001,-0.885000000000001,-0.880000000000001,
-0.875000000000001,-0.870000000000001,-0.865000000000001,-0.860000000000001,
-0.855000000000001,-0.850000000000001,-0.845000000000001,-0.840000000000001,
-0.835000000000001,-0.830000000000001,-0.825000000000001,-0.820000000000001,
-0.815000000000001,-0.810000000000001,-0.805000000000001,-0.800000000000001,
-0.795000000000001,-0.790000000000001,-0.785000000000001,-0.780000000000001,
-0.775000000000001,-0.770000000000001,-0.765000000000001,-0.760000000000001,
-0.755000000000001,-0.750000000000001,-0.745000000000001,-0.740000000000001,
-0.735000000000001,-0.730000000000001,-0.725000000000001,-0.720000000000001,
-0.715000000000001,-0.710000000000001,-0.705000000000001,-0.700000000000001,
-0.695000000000001,-0.690000000000001,-0.685,-0.68,-0.675,-0.67,-0.665,
-0.66,-0.655,-0.65,-0.645,-0.64,-0.635,-0.63,-0.625,-0.62,-0.615,-0.61,
-0.605,-0.6,-0.595,-0.59,-0.585,-0.58,-0.575,-0.57,-0.565,-0.56,-0.555,
-0.55,-0.545,-0.54,-0.535,-0.53,-0.525,-0.52,-0.515,-0.51,-0.505,-0.5,-0.495,
-0.49,-0.485,-0.48,-0.475,-0.47,-0.465,-0.46,-0.455,-0.45,-0.445,-0.44,
-0.435,-0.43,-0.425,-0.42,-0.415,-0.41,-0.405,-0.4,-0.395,-0.39,-0.385,
-0.38,-0.375,-0.37,-0.365,-0.36,-0.355,-0.35,-0.345,-0.34,-0.335,-0.33,
-0.325,-0.32,-0.315,-0.31,-0.305,-0.3,-0.295,-0.29,-0.285,-0.28,-0.275,
-0.27,-0.265,-0.26,-0.255,-0.25,-0.245,-0.24,-0.235,-0.23,-0.225,-0.22,
-0.215,-0.21,-0.205,-0.2,-0.195,-0.19,-0.185,-0.18,-0.175,-0.17,-0.165,
-0.16,-0.155,-0.15,-0.145,-0.14,-0.135,-0.13,-0.125,-0.12,-0.115,-0.11,
-0.105,-0.1,-0.095,-0.09,-0.085,-0.08,-0.075,-0.07,-0.065,-0.06,-0.055,
-0.05,-0.045,-0.04,-0.035,-0.03,-0.025,-0.02,-0.015,-0.01,-0.005,0.),
 .UNSPECIFIED.)
CURVE()
GEOMETRIC_REPRESENTATION_ITEM()
RATIONAL_B_SPLINE_CURVE((1.,1.,1.,1.,1.,1.,1.,1.,1.,1.,1.,1.,1.,1.,1.,1.,
1.,1.,1.,1.,1.,1.,1.,1.,1.,1.,1.,1.,1.,1.,1.,1.,1.,1.,1.,1.,1.,1.,1.,1.,
1.,1.,1.,1.,1.,1.,1.,1.,1.,1.,1.,1.,1.,1.,1.,1.,1.,1.,1.,1.,1.,1.,1.,1.,
1.,1.,1.,1.,1.,1.,1.,1.,1.,1.,1.,1.,1.,1.,1.,1.,1.,1.,1.,1.,1.,1.,1.,1.,
1.,1.,1.,1.,1.,1.,1.,1.,1.,1.,1.,1.,1.,1.,1.,1.,1.,1.,1.,1.,1.,1.,1.,1.,
1.,1.,1.,1.,1.,1.,1.,1.,1.,1.,1.,1.,1.,1.,1.,1.,1.,1.,1.,1.,1.,1.,1.,1.,
1.,1.,1.,1.,1.,1.,1.,1.,1.,1.,1.,1.,1.,1.,1.,1.,1.,1.,1.,1.,1.,1.,1.,1.,
1.,1.,1.,1.,1.,1.,1.,1.,1.,1.,1.,1.,1.,1.,1.,1.,1.,1.,1.,1.,1.,1.,1.,1.,
1.,1.,1.,1.,1.,1.,1.,1.,1.,1.,1.,1.,1.,1.,1.,1.,1.,1.,1.,1.,1.))
REPRESENTATION_ITEM('')
);
#844=(
BOUNDED_CURVE()
B_SPLINE_CURVE(5,(#239754,#239755,#239756,#239757,#239758,#239759,#239760,
#239761,#239762,#239763,#239764,#239765,#239766,#239767,#239768,#239769,
#239770,#239771,#239772,#239773,#239774,#239775,#239776,#239777,#239778,
#239779,#239780,#239781,#239782,#239783,#239784,#239785,#239786,#239787,
#239788,#239789,#239790,#239791,#239792,#239793,#239794,#239795,#239796,
#239797,#239798,#239799,#239800,#239801,#239802,#239803,#239804,#239805,
#239806,#239807,#239808,#239809,#239810,#239811,#239812,#239813,#239814,
#239815,#239816,#239817,#239818,#239819,#239820,#239821,#239822,#239823,
#239824,#239825,#239826,#239827,#239828,#239829,#239830,#239831,#239832,
#239833,#239834,#239835,#239836,#239837,#239838,#239839,#239840,#239841,
#239842,#239843,#239844,#239845,#239846,#239847,#239848,#239849,#239850,
#239851,#239852,#239853,#239854,#239855,#239856,#239857,#239858,#239859,
#239860,#239861,#239862,#239863,#239864,#239865,#239866,#239867,#239868,
#239869,#239870,#239871,#239872,#239873,#239874,#239875,#239876,#239877,
#239878,#239879,#239880,#239881,#239882,#239883,#239884,#239885,#239886,
#239887,#239888,#239889,#239890,#239891,#239892,#239893,#239894,#239895,
#239896,#239897,#239898,#239899,#239900,#239901,#239902,#239903,#239904,
#239905,#239906,#239907,#239908,#239909,#239910,#239911,#239912,#239913,
#239914,#239915,#239916,#239917,#239918,#239919,#239920,#239921,#239922,
#239923,#239924,#239925,#239926,#239927,#239928,#239929,#239930,#239931,
#239932,#239933,#239934,#239935,#239936,#239937,#239938,#239939,#239940,
#239941,#239942,#239943,#239944,#239945,#239946,#239947,#239948,#239949,
#239950,#239951,#239952,#239953,#239954,#239955,#239956,#239957,#239958),
 .UNSPECIFIED.,.F.,.F.)
B_SPLINE_CURVE_WITH_KNOTS((6,1,1,1,1,1,1,1,1,1,1,1,1,1,1,1,1,1,1,1,1,1,
1,1,1,1,1,1,1,1,1,1,1,1,1,1,1,1,1,1,1,1,1,1,1,1,1,1,1,1,1,1,1,1,1,1,1,1,
1,1,1,1,1,1,1,1,1,1,1,1,1,1,1,1,1,1,1,1,1,1,1,1,1,1,1,1,1,1,1,1,1,1,1,1,
1,1,1,1,1,1,1,1,1,1,1,1,1,1,1,1,1,1,1,1,1,1,1,1,1,1,1,1,1,1,1,1,1,1,1,1,
1,1,1,1,1,1,1,1,1,1,1,1,1,1,1,1,1,1,1,1,1,1,1,1,1,1,1,1,1,1,1,1,1,1,1,1,
1,1,1,1,1,1,1,1,1,1,1,1,1,1,1,1,1,1,1,1,1,1,1,1,1,1,1,1,1,1,1,1,1,1,6),
(0.,0.005,0.01,0.015,0.02,0.025,0.03,0.035,0.04,0.045,0.05,0.055,0.06,0.065,
0.07,0.075,0.08,0.085,0.09,0.095,0.1,0.105,0.11,0.115,0.12,0.125,0.13,0.135,
0.14,0.145,0.15,0.155,0.16,0.165,0.17,0.175,0.18,0.185,0.19,0.195,0.2,0.205,
0.21,0.215,0.22,0.225,0.23,0.235,0.24,0.245,0.25,0.255,0.26,0.265,0.27,
0.275,0.28,0.285,0.29,0.295,0.3,0.305,0.31,0.315,0.32,0.325,0.33,0.335,
0.34,0.345,0.35,0.355,0.36,0.365,0.37,0.375,0.38,0.385,0.39,0.395,0.4,0.405,
0.41,0.415,0.42,0.425,0.43,0.435,0.44,0.445,0.45,0.455,0.46,0.465,0.47,
0.475,0.48,0.485,0.49,0.495,0.5,0.505,0.51,0.515,0.52,0.525,0.53,0.535,
0.54,0.545,0.55,0.555,0.56,0.565,0.57,0.575,0.58,0.585,0.59,0.595,0.6,0.605,
0.61,0.615,0.62,0.625,0.63,0.635,0.64,0.645,0.65,0.655,0.66,0.665,0.67,
0.675,0.68,0.685,0.690000000000001,0.695000000000001,0.700000000000001,
0.705000000000001,0.710000000000001,0.715000000000001,0.720000000000001,
0.725000000000001,0.730000000000001,0.735000000000001,0.740000000000001,
0.745000000000001,0.750000000000001,0.755000000000001,0.760000000000001,
0.765000000000001,0.770000000000001,0.775000000000001,0.780000000000001,
0.785000000000001,0.790000000000001,0.795000000000001,0.800000000000001,
0.805000000000001,0.810000000000001,0.815000000000001,0.820000000000001,
0.825000000000001,0.830000000000001,0.835000000000001,0.840000000000001,
0.845000000000001,0.850000000000001,0.855000000000001,0.860000000000001,
0.865000000000001,0.870000000000001,0.875000000000001,0.880000000000001,
0.885000000000001,0.890000000000001,0.895000000000001,0.900000000000001,
0.905000000000001,0.910000000000001,0.915000000000001,0.920000000000001,
0.925000000000001,0.930000000000001,0.935000000000001,0.940000000000001,
0.945000000000001,0.950000000000001,0.955000000000001,0.960000000000001,
0.965000000000001,0.970000000000001,0.975000000000001,0.980000000000001,
0.985000000000001,0.990000000000001,0.995000000000001,1.),.UNSPECIFIED.)
CURVE()
GEOMETRIC_REPRESENTATION_ITEM()
RATIONAL_B_SPLINE_CURVE((1.,1.,1.,1.,1.,1.,1.,1.,1.,1.,1.,1.,1.,1.,1.,1.,
1.,1.,1.,1.,1.,1.,1.,1.,1.,1.,1.,1.,1.,1.,1.,1.,1.,1.,1.,1.,1.,1.,1.,1.,
1.,1.,1.,1.,1.,1.,1.,1.,1.,1.,1.,1.,1.,1.,1.,1.,1.,1.,1.,1.,1.,1.,1.,1.,
1.,1.,1.,1.,1.,1.,1.,1.,1.,1.,1.,1.,1.,1.,1.,1.,1.,1.,1.,1.,1.,1.,1.,1.,
1.,1.,1.,1.,1.,1.,1.,1.,1.,1.,1.,1.,1.,1.,1.,1.,1.,1.,1.,1.,1.,1.,1.,1.,
1.,1.,1.,1.,1.,1.,1.,1.,1.,1.,1.,1.,1.,1.,1.,1.,1.,1.,1.,1.,1.,1.,1.,1.,
1.,1.,1.,1.,1.,1.,1.,1.,1.,1.,1.,1.,1.,1.,1.,1.,1.,1.,1.,1.,1.,1.,1.,1.,
1.,1.,1.,1.,1.,1.,1.,1.,1.,1.,1.,1.,1.,1.,1.,1.,1.,1.,1.,1.,1.,1.,1.,1.,
1.,1.,1.,1.,1.,1.,1.,1.,1.,1.,1.,1.,1.,1.,1.,1.,1.,1.,1.,1.,1.))
REPRESENTATION_ITEM('')
);
#845=(
BOUNDED_CURVE()
B_SPLINE_CURVE(5,(#240370,#240371,#240372,#240373,#240374,#240375,#240376,
#240377,#240378,#240379,#240380,#240381,#240382,#240383,#240384,#240385,
#240386,#240387,#240388,#240389,#240390,#240391,#240392,#240393,#240394,
#240395,#240396,#240397,#240398,#240399,#240400,#240401,#240402,#240403,
#240404,#240405,#240406,#240407,#240408,#240409,#240410,#240411,#240412,
#240413,#240414,#240415,#240416,#240417,#240418,#240419,#240420,#240421,
#240422,#240423,#240424,#240425,#240426,#240427,#240428,#240429,#240430,
#240431,#240432,#240433,#240434,#240435,#240436,#240437,#240438,#240439,
#240440,#240441,#240442,#240443,#240444,#240445,#240446,#240447,#240448,
#240449,#240450,#240451,#240452,#240453,#240454,#240455,#240456,#240457,
#240458,#240459,#240460,#240461,#240462,#240463,#240464,#240465,#240466,
#240467,#240468,#240469,#240470,#240471,#240472,#240473,#240474,#240475,
#240476,#240477,#240478,#240479,#240480,#240481,#240482,#240483,#240484,
#240485,#240486,#240487,#240488,#240489,#240490,#240491,#240492,#240493,
#240494,#240495,#240496,#240497,#240498,#240499,#240500,#240501,#240502,
#240503,#240504,#240505,#240506,#240507,#240508,#240509,#240510,#240511,
#240512,#240513,#240514,#240515,#240516,#240517,#240518,#240519,#240520,
#240521,#240522,#240523,#240524,#240525,#240526,#240527,#240528,#240529,
#240530,#240531,#240532,#240533,#240534,#240535,#240536,#240537,#240538,
#240539,#240540,#240541,#240542,#240543,#240544,#240545,#240546,#240547,
#240548,#240549,#240550,#240551,#240552,#240553,#240554,#240555,#240556,
#240557,#240558,#240559,#240560,#240561,#240562,#240563,#240564,#240565,
#240566,#240567,#240568,#240569,#240570,#240571,#240572,#240573,#240574),
 .UNSPECIFIED.,.F.,.F.)
B_SPLINE_CURVE_WITH_KNOTS((6,1,1,1,1,1,1,1,1,1,1,1,1,1,1,1,1,1,1,1,1,1,
1,1,1,1,1,1,1,1,1,1,1,1,1,1,1,1,1,1,1,1,1,1,1,1,1,1,1,1,1,1,1,1,1,1,1,1,
1,1,1,1,1,1,1,1,1,1,1,1,1,1,1,1,1,1,1,1,1,1,1,1,1,1,1,1,1,1,1,1,1,1,1,1,
1,1,1,1,1,1,1,1,1,1,1,1,1,1,1,1,1,1,1,1,1,1,1,1,1,1,1,1,1,1,1,1,1,1,1,1,
1,1,1,1,1,1,1,1,1,1,1,1,1,1,1,1,1,1,1,1,1,1,1,1,1,1,1,1,1,1,1,1,1,1,1,1,
1,1,1,1,1,1,1,1,1,1,1,1,1,1,1,1,1,1,1,1,1,1,1,1,1,1,1,1,1,1,1,1,1,1,6),
(0.,0.005,0.01,0.015,0.02,0.025,0.03,0.035,0.04,0.045,0.05,0.055,0.06,0.065,
0.07,0.075,0.08,0.085,0.09,0.095,0.1,0.105,0.11,0.115,0.12,0.125,0.13,0.135,
0.14,0.145,0.15,0.155,0.16,0.165,0.17,0.175,0.18,0.185,0.19,0.195,0.2,0.205,
0.21,0.215,0.22,0.225,0.23,0.235,0.24,0.245,0.25,0.255,0.26,0.265,0.27,
0.275,0.28,0.285,0.29,0.295,0.3,0.305,0.31,0.315,0.32,0.325,0.33,0.335,
0.34,0.345,0.35,0.355,0.36,0.365,0.37,0.375,0.38,0.385,0.39,0.395,0.4,0.405,
0.41,0.415,0.42,0.425,0.43,0.435,0.44,0.445,0.45,0.455,0.46,0.465,0.47,
0.475,0.48,0.485,0.49,0.495,0.5,0.505,0.51,0.515,0.52,0.525,0.53,0.535,
0.54,0.545,0.55,0.555,0.56,0.565,0.57,0.575,0.58,0.585,0.59,0.595,0.6,0.605,
0.61,0.615,0.62,0.625,0.63,0.635,0.64,0.645,0.65,0.655,0.66,0.665,0.67,
0.675,0.68,0.685,0.690000000000001,0.695000000000001,0.700000000000001,
0.705000000000001,0.710000000000001,0.715000000000001,0.720000000000001,
0.725000000000001,0.730000000000001,0.735000000000001,0.740000000000001,
0.745000000000001,0.750000000000001,0.755000000000001,0.760000000000001,
0.765000000000001,0.770000000000001,0.775000000000001,0.780000000000001,
0.785000000000001,0.790000000000001,0.795000000000001,0.800000000000001,
0.805000000000001,0.810000000000001,0.815000000000001,0.820000000000001,
0.825000000000001,0.830000000000001,0.835000000000001,0.840000000000001,
0.845000000000001,0.850000000000001,0.855000000000001,0.860000000000001,
0.865000000000001,0.870000000000001,0.875000000000001,0.880000000000001,
0.885000000000001,0.890000000000001,0.895000000000001,0.900000000000001,
0.905000000000001,0.910000000000001,0.915000000000001,0.920000000000001,
0.925000000000001,0.930000000000001,0.935000000000001,0.940000000000001,
0.945000000000001,0.950000000000001,0.955000000000001,0.960000000000001,
0.965000000000001,0.970000000000001,0.975000000000001,0.980000000000001,
0.985000000000001,0.990000000000001,0.995000000000001,1.),.UNSPECIFIED.)
CURVE()
GEOMETRIC_REPRESENTATION_ITEM()
RATIONAL_B_SPLINE_CURVE((1.,1.,1.,1.,1.,1.,1.,1.,1.,1.,1.,1.,1.,1.,1.,1.,
1.,1.,1.,1.,1.,1.,1.,1.,1.,1.,1.,1.,1.,1.,1.,1.,1.,1.,1.,1.,1.,1.,1.,1.,
1.,1.,1.,1.,1.,1.,1.,1.,1.,1.,1.,1.,1.,1.,1.,1.,1.,1.,1.,1.,1.,1.,1.,1.,
1.,1.,1.,1.,1.,1.,1.,1.,1.,1.,1.,1.,1.,1.,1.,1.,1.,1.,1.,1.,1.,1.,1.,1.,
1.,1.,1.,1.,1.,1.,1.,1.,1.,1.,1.,1.,1.,1.,1.,1.,1.,1.,1.,1.,1.,1.,1.,1.,
1.,1.,1.,1.,1.,1.,1.,1.,1.,1.,1.,1.,1.,1.,1.,1.,1.,1.,1.,1.,1.,1.,1.,1.,
1.,1.,1.,1.,1.,1.,1.,1.,1.,1.,1.,1.,1.,1.,1.,1.,1.,1.,1.,1.,1.,1.,1.,1.,
1.,1.,1.,1.,1.,1.,1.,1.,1.,1.,1.,1.,1.,1.,1.,1.,1.,1.,1.,1.,1.,1.,1.,1.,
1.,1.,1.,1.,1.,1.,1.,1.,1.,1.,1.,1.,1.,1.,1.,1.,1.,1.,1.,1.,1.))
REPRESENTATION_ITEM('')
);
#846=(
BOUNDED_CURVE()
B_SPLINE_CURVE(5,(#240576,#240577,#240578,#240579,#240580,#240581,#240582,
#240583,#240584,#240585,#240586,#240587,#240588,#240589,#240590,#240591,
#240592,#240593,#240594,#240595,#240596,#240597,#240598,#240599,#240600,
#240601,#240602,#240603,#240604,#240605,#240606,#240607,#240608,#240609,
#240610,#240611,#240612,#240613,#240614,#240615,#240616,#240617,#240618,
#240619,#240620,#240621,#240622,#240623,#240624,#240625,#240626,#240627,
#240628,#240629,#240630,#240631,#240632,#240633,#240634,#240635,#240636,
#240637,#240638,#240639,#240640,#240641,#240642,#240643,#240644,#240645,
#240646,#240647,#240648,#240649,#240650,#240651,#240652,#240653,#240654,
#240655,#240656,#240657,#240658,#240659,#240660,#240661,#240662,#240663,
#240664,#240665,#240666,#240667,#240668,#240669,#240670,#240671,#240672,
#240673,#240674,#240675,#240676,#240677,#240678,#240679,#240680,#240681,
#240682,#240683,#240684,#240685,#240686,#240687,#240688,#240689,#240690,
#240691,#240692,#240693,#240694,#240695,#240696,#240697,#240698,#240699,
#240700,#240701,#240702,#240703,#240704,#240705,#240706,#240707,#240708,
#240709,#240710,#240711,#240712,#240713,#240714,#240715,#240716,#240717,
#240718,#240719,#240720,#240721,#240722,#240723,#240724,#240725,#240726,
#240727,#240728,#240729,#240730,#240731,#240732,#240733,#240734,#240735,
#240736,#240737,#240738,#240739,#240740,#240741,#240742,#240743,#240744,
#240745,#240746,#240747,#240748,#240749,#240750,#240751,#240752,#240753,
#240754,#240755,#240756,#240757,#240758,#240759,#240760,#240761,#240762,
#240763,#240764,#240765,#240766,#240767,#240768,#240769,#240770,#240771,
#240772,#240773,#240774,#240775,#240776,#240777,#240778,#240779,#240780),
 .UNSPECIFIED.,.F.,.F.)
B_SPLINE_CURVE_WITH_KNOTS((6,1,1,1,1,1,1,1,1,1,1,1,1,1,1,1,1,1,1,1,1,1,
1,1,1,1,1,1,1,1,1,1,1,1,1,1,1,1,1,1,1,1,1,1,1,1,1,1,1,1,1,1,1,1,1,1,1,1,
1,1,1,1,1,1,1,1,1,1,1,1,1,1,1,1,1,1,1,1,1,1,1,1,1,1,1,1,1,1,1,1,1,1,1,1,
1,1,1,1,1,1,1,1,1,1,1,1,1,1,1,1,1,1,1,1,1,1,1,1,1,1,1,1,1,1,1,1,1,1,1,1,
1,1,1,1,1,1,1,1,1,1,1,1,1,1,1,1,1,1,1,1,1,1,1,1,1,1,1,1,1,1,1,1,1,1,1,1,
1,1,1,1,1,1,1,1,1,1,1,1,1,1,1,1,1,1,1,1,1,1,1,1,1,1,1,1,1,1,1,1,1,1,6),
(-1.,-0.995000000000001,-0.990000000000001,-0.985000000000001,-0.980000000000001,
-0.975000000000001,-0.970000000000001,-0.965000000000001,-0.960000000000001,
-0.955000000000001,-0.950000000000001,-0.945000000000001,-0.940000000000001,
-0.935000000000001,-0.930000000000001,-0.925000000000001,-0.920000000000001,
-0.915000000000001,-0.910000000000001,-0.905000000000001,-0.900000000000001,
-0.895000000000001,-0.890000000000001,-0.885000000000001,-0.880000000000001,
-0.875000000000001,-0.870000000000001,-0.865000000000001,-0.860000000000001,
-0.855000000000001,-0.850000000000001,-0.845000000000001,-0.840000000000001,
-0.835000000000001,-0.830000000000001,-0.825000000000001,-0.820000000000001,
-0.815000000000001,-0.810000000000001,-0.805000000000001,-0.800000000000001,
-0.795000000000001,-0.790000000000001,-0.785000000000001,-0.780000000000001,
-0.775000000000001,-0.770000000000001,-0.765000000000001,-0.760000000000001,
-0.755000000000001,-0.750000000000001,-0.745000000000001,-0.740000000000001,
-0.735000000000001,-0.730000000000001,-0.725000000000001,-0.720000000000001,
-0.715000000000001,-0.710000000000001,-0.705000000000001,-0.700000000000001,
-0.695000000000001,-0.690000000000001,-0.685,-0.68,-0.675,-0.67,-0.665,
-0.66,-0.655,-0.65,-0.645,-0.64,-0.635,-0.63,-0.625,-0.62,-0.615,-0.61,
-0.605,-0.6,-0.595,-0.59,-0.585,-0.58,-0.575,-0.57,-0.565,-0.56,-0.555,
-0.55,-0.545,-0.54,-0.535,-0.53,-0.525,-0.52,-0.515,-0.51,-0.505,-0.5,-0.495,
-0.49,-0.485,-0.48,-0.475,-0.47,-0.465,-0.46,-0.455,-0.45,-0.445,-0.44,
-0.435,-0.43,-0.425,-0.42,-0.415,-0.41,-0.405,-0.4,-0.395,-0.39,-0.385,
-0.38,-0.375,-0.37,-0.365,-0.36,-0.355,-0.35,-0.345,-0.34,-0.335,-0.33,
-0.325,-0.32,-0.315,-0.31,-0.305,-0.3,-0.295,-0.29,-0.285,-0.28,-0.275,
-0.27,-0.265,-0.26,-0.255,-0.25,-0.245,-0.24,-0.235,-0.23,-0.225,-0.22,
-0.215,-0.21,-0.205,-0.2,-0.195,-0.19,-0.185,-0.18,-0.175,-0.17,-0.165,
-0.16,-0.155,-0.15,-0.145,-0.14,-0.135,-0.13,-0.125,-0.12,-0.115,-0.11,
-0.105,-0.1,-0.095,-0.09,-0.085,-0.08,-0.075,-0.07,-0.065,-0.06,-0.055,
-0.05,-0.045,-0.04,-0.035,-0.03,-0.025,-0.02,-0.015,-0.01,-0.005,0.),
 .UNSPECIFIED.)
CURVE()
GEOMETRIC_REPRESENTATION_ITEM()
RATIONAL_B_SPLINE_CURVE((1.,1.,1.,1.,1.,1.,1.,1.,1.,1.,1.,1.,1.,1.,1.,1.,
1.,1.,1.,1.,1.,1.,1.,1.,1.,1.,1.,1.,1.,1.,1.,1.,1.,1.,1.,1.,1.,1.,1.,1.,
1.,1.,1.,1.,1.,1.,1.,1.,1.,1.,1.,1.,1.,1.,1.,1.,1.,1.,1.,1.,1.,1.,1.,1.,
1.,1.,1.,1.,1.,1.,1.,1.,1.,1.,1.,1.,1.,1.,1.,1.,1.,1.,1.,1.,1.,1.,1.,1.,
1.,1.,1.,1.,1.,1.,1.,1.,1.,1.,1.,1.,1.,1.,1.,1.,1.,1.,1.,1.,1.,1.,1.,1.,
1.,1.,1.,1.,1.,1.,1.,1.,1.,1.,1.,1.,1.,1.,1.,1.,1.,1.,1.,1.,1.,1.,1.,1.,
1.,1.,1.,1.,1.,1.,1.,1.,1.,1.,1.,1.,1.,1.,1.,1.,1.,1.,1.,1.,1.,1.,1.,1.,
1.,1.,1.,1.,1.,1.,1.,1.,1.,1.,1.,1.,1.,1.,1.,1.,1.,1.,1.,1.,1.,1.,1.,1.,
1.,1.,1.,1.,1.,1.,1.,1.,1.,1.,1.,1.,1.,1.,1.,1.,1.,1.,1.,1.,1.))
REPRESENTATION_ITEM('')
);
#847=(
BOUNDED_CURVE()
B_SPLINE_CURVE(5,(#241199,#241200,#241201,#241202,#241203,#241204,#241205,
#241206,#241207,#241208,#241209,#241210,#241211,#241212,#241213,#241214,
#241215,#241216,#241217,#241218,#241219,#241220,#241221,#241222,#241223,
#241224,#241225,#241226,#241227,#241228,#241229,#241230,#241231,#241232,
#241233,#241234,#241235,#241236,#241237,#241238,#241239,#241240,#241241,
#241242,#241243,#241244,#241245,#241246,#241247,#241248,#241249,#241250,
#241251,#241252,#241253,#241254,#241255,#241256,#241257,#241258,#241259,
#241260,#241261,#241262,#241263,#241264,#241265,#241266,#241267,#241268,
#241269,#241270,#241271,#241272,#241273,#241274,#241275,#241276,#241277,
#241278,#241279,#241280,#241281,#241282,#241283,#241284,#241285,#241286,
#241287,#241288,#241289,#241290,#241291,#241292,#241293,#241294,#241295,
#241296,#241297,#241298,#241299,#241300,#241301,#241302,#241303,#241304,
#241305,#241306,#241307,#241308,#241309,#241310,#241311,#241312,#241313,
#241314,#241315,#241316,#241317,#241318,#241319,#241320,#241321,#241322,
#241323,#241324,#241325,#241326,#241327,#241328,#241329,#241330,#241331,
#241332,#241333,#241334,#241335,#241336,#241337,#241338,#241339,#241340,
#241341,#241342,#241343,#241344,#241345,#241346,#241347,#241348,#241349,
#241350,#241351,#241352,#241353,#241354,#241355,#241356,#241357,#241358,
#241359,#241360,#241361,#241362,#241363,#241364,#241365,#241366,#241367,
#241368,#241369,#241370,#241371,#241372,#241373,#241374,#241375,#241376,
#241377,#241378,#241379,#241380,#241381,#241382,#241383,#241384,#241385,
#241386,#241387,#241388,#241389,#241390,#241391,#241392,#241393,#241394,
#241395,#241396,#241397,#241398,#241399,#241400,#241401,#241402,#241403),
 .UNSPECIFIED.,.F.,.F.)
B_SPLINE_CURVE_WITH_KNOTS((6,1,1,1,1,1,1,1,1,1,1,1,1,1,1,1,1,1,1,1,1,1,
1,1,1,1,1,1,1,1,1,1,1,1,1,1,1,1,1,1,1,1,1,1,1,1,1,1,1,1,1,1,1,1,1,1,1,1,
1,1,1,1,1,1,1,1,1,1,1,1,1,1,1,1,1,1,1,1,1,1,1,1,1,1,1,1,1,1,1,1,1,1,1,1,
1,1,1,1,1,1,1,1,1,1,1,1,1,1,1,1,1,1,1,1,1,1,1,1,1,1,1,1,1,1,1,1,1,1,1,1,
1,1,1,1,1,1,1,1,1,1,1,1,1,1,1,1,1,1,1,1,1,1,1,1,1,1,1,1,1,1,1,1,1,1,1,1,
1,1,1,1,1,1,1,1,1,1,1,1,1,1,1,1,1,1,1,1,1,1,1,1,1,1,1,1,1,1,1,1,1,1,6),
(-1.,-0.995000000000001,-0.990000000000001,-0.985000000000001,-0.980000000000001,
-0.975000000000001,-0.970000000000001,-0.965000000000001,-0.960000000000001,
-0.955000000000001,-0.950000000000001,-0.945000000000001,-0.940000000000001,
-0.935000000000001,-0.930000000000001,-0.925000000000001,-0.920000000000001,
-0.915000000000001,-0.910000000000001,-0.905000000000001,-0.900000000000001,
-0.895000000000001,-0.890000000000001,-0.885000000000001,-0.880000000000001,
-0.875000000000001,-0.870000000000001,-0.865000000000001,-0.860000000000001,
-0.855000000000001,-0.850000000000001,-0.845000000000001,-0.840000000000001,
-0.835000000000001,-0.830000000000001,-0.825000000000001,-0.820000000000001,
-0.815000000000001,-0.810000000000001,-0.805000000000001,-0.800000000000001,
-0.795000000000001,-0.790000000000001,-0.785000000000001,-0.780000000000001,
-0.775000000000001,-0.770000000000001,-0.765000000000001,-0.760000000000001,
-0.755000000000001,-0.750000000000001,-0.745000000000001,-0.740000000000001,
-0.735000000000001,-0.730000000000001,-0.725000000000001,-0.720000000000001,
-0.715000000000001,-0.710000000000001,-0.705000000000001,-0.700000000000001,
-0.695000000000001,-0.690000000000001,-0.685,-0.68,-0.675,-0.67,-0.665,
-0.66,-0.655,-0.65,-0.645,-0.64,-0.635,-0.63,-0.625,-0.62,-0.615,-0.61,
-0.605,-0.6,-0.595,-0.59,-0.585,-0.58,-0.575,-0.57,-0.565,-0.56,-0.555,
-0.55,-0.545,-0.54,-0.535,-0.53,-0.525,-0.52,-0.515,-0.51,-0.505,-0.5,-0.495,
-0.49,-0.485,-0.48,-0.475,-0.47,-0.465,-0.46,-0.455,-0.45,-0.445,-0.44,
-0.435,-0.43,-0.425,-0.42,-0.415,-0.41,-0.405,-0.4,-0.395,-0.39,-0.385,
-0.38,-0.375,-0.37,-0.365,-0.36,-0.355,-0.35,-0.345,-0.34,-0.335,-0.33,
-0.325,-0.32,-0.315,-0.31,-0.305,-0.3,-0.295,-0.29,-0.285,-0.28,-0.275,
-0.27,-0.265,-0.26,-0.255,-0.25,-0.245,-0.24,-0.235,-0.23,-0.225,-0.22,
-0.215,-0.21,-0.205,-0.2,-0.195,-0.19,-0.185,-0.18,-0.175,-0.17,-0.165,
-0.16,-0.155,-0.15,-0.145,-0.14,-0.135,-0.13,-0.125,-0.12,-0.115,-0.11,
-0.105,-0.1,-0.095,-0.09,-0.085,-0.08,-0.075,-0.07,-0.065,-0.06,-0.055,
-0.05,-0.045,-0.04,-0.035,-0.03,-0.025,-0.02,-0.015,-0.01,-0.005,0.),
 .UNSPECIFIED.)
CURVE()
GEOMETRIC_REPRESENTATION_ITEM()
RATIONAL_B_SPLINE_CURVE((1.,1.,1.,1.,1.,1.,1.,1.,1.,1.,1.,1.,1.,1.,1.,1.,
1.,1.,1.,1.,1.,1.,1.,1.,1.,1.,1.,1.,1.,1.,1.,1.,1.,1.,1.,1.,1.,1.,1.,1.,
1.,1.,1.,1.,1.,1.,1.,1.,1.,1.,1.,1.,1.,1.,1.,1.,1.,1.,1.,1.,1.,1.,1.,1.,
1.,1.,1.,1.,1.,1.,1.,1.,1.,1.,1.,1.,1.,1.,1.,1.,1.,1.,1.,1.,1.,1.,1.,1.,
1.,1.,1.,1.,1.,1.,1.,1.,1.,1.,1.,1.,1.,1.,1.,1.,1.,1.,1.,1.,1.,1.,1.,1.,
1.,1.,1.,1.,1.,1.,1.,1.,1.,1.,1.,1.,1.,1.,1.,1.,1.,1.,1.,1.,1.,1.,1.,1.,
1.,1.,1.,1.,1.,1.,1.,1.,1.,1.,1.,1.,1.,1.,1.,1.,1.,1.,1.,1.,1.,1.,1.,1.,
1.,1.,1.,1.,1.,1.,1.,1.,1.,1.,1.,1.,1.,1.,1.,1.,1.,1.,1.,1.,1.,1.,1.,1.,
1.,1.,1.,1.,1.,1.,1.,1.,1.,1.,1.,1.,1.,1.,1.,1.,1.,1.,1.,1.,1.))
REPRESENTATION_ITEM('')
);
#848=(
BOUNDED_CURVE()
B_SPLINE_CURVE(5,(#241406,#241407,#241408,#241409,#241410,#241411,#241412,
#241413,#241414,#241415,#241416,#241417,#241418,#241419,#241420,#241421,
#241422,#241423,#241424,#241425,#241426,#241427,#241428,#241429,#241430,
#241431,#241432,#241433,#241434,#241435,#241436,#241437,#241438,#241439,
#241440,#241441,#241442,#241443,#241444,#241445,#241446,#241447,#241448,
#241449,#241450,#241451,#241452,#241453,#241454,#241455,#241456,#241457,
#241458,#241459,#241460,#241461,#241462,#241463,#241464,#241465,#241466,
#241467,#241468,#241469,#241470,#241471,#241472,#241473,#241474,#241475,
#241476,#241477,#241478,#241479,#241480,#241481,#241482,#241483,#241484,
#241485,#241486,#241487,#241488,#241489,#241490,#241491,#241492,#241493,
#241494,#241495,#241496,#241497,#241498,#241499,#241500,#241501,#241502,
#241503,#241504,#241505,#241506,#241507,#241508,#241509,#241510,#241511,
#241512,#241513,#241514,#241515,#241516,#241517,#241518,#241519,#241520,
#241521,#241522,#241523,#241524,#241525,#241526,#241527,#241528,#241529,
#241530,#241531,#241532,#241533,#241534,#241535,#241536,#241537,#241538,
#241539,#241540,#241541,#241542,#241543,#241544,#241545,#241546,#241547,
#241548,#241549,#241550,#241551,#241552,#241553,#241554,#241555,#241556,
#241557,#241558,#241559,#241560,#241561,#241562,#241563,#241564,#241565,
#241566,#241567,#241568,#241569,#241570,#241571,#241572,#241573,#241574,
#241575,#241576,#241577,#241578,#241579,#241580,#241581,#241582,#241583,
#241584,#241585,#241586,#241587,#241588,#241589,#241590,#241591,#241592,
#241593,#241594,#241595,#241596,#241597,#241598,#241599,#241600,#241601,
#241602,#241603,#241604,#241605,#241606,#241607,#241608,#241609,#241610),
 .UNSPECIFIED.,.F.,.F.)
B_SPLINE_CURVE_WITH_KNOTS((6,1,1,1,1,1,1,1,1,1,1,1,1,1,1,1,1,1,1,1,1,1,
1,1,1,1,1,1,1,1,1,1,1,1,1,1,1,1,1,1,1,1,1,1,1,1,1,1,1,1,1,1,1,1,1,1,1,1,
1,1,1,1,1,1,1,1,1,1,1,1,1,1,1,1,1,1,1,1,1,1,1,1,1,1,1,1,1,1,1,1,1,1,1,1,
1,1,1,1,1,1,1,1,1,1,1,1,1,1,1,1,1,1,1,1,1,1,1,1,1,1,1,1,1,1,1,1,1,1,1,1,
1,1,1,1,1,1,1,1,1,1,1,1,1,1,1,1,1,1,1,1,1,1,1,1,1,1,1,1,1,1,1,1,1,1,1,1,
1,1,1,1,1,1,1,1,1,1,1,1,1,1,1,1,1,1,1,1,1,1,1,1,1,1,1,1,1,1,1,1,1,1,6),
(0.,0.005,0.01,0.015,0.02,0.025,0.03,0.035,0.04,0.045,0.05,0.055,0.06,0.065,
0.07,0.075,0.08,0.085,0.09,0.095,0.1,0.105,0.11,0.115,0.12,0.125,0.13,0.135,
0.14,0.145,0.15,0.155,0.16,0.165,0.17,0.175,0.18,0.185,0.19,0.195,0.2,0.205,
0.21,0.215,0.22,0.225,0.23,0.235,0.24,0.245,0.25,0.255,0.26,0.265,0.27,
0.275,0.28,0.285,0.29,0.295,0.3,0.305,0.31,0.315,0.32,0.325,0.33,0.335,
0.34,0.345,0.35,0.355,0.36,0.365,0.37,0.375,0.38,0.385,0.39,0.395,0.4,0.405,
0.41,0.415,0.42,0.425,0.43,0.435,0.44,0.445,0.45,0.455,0.46,0.465,0.47,
0.475,0.48,0.485,0.49,0.495,0.5,0.505,0.51,0.515,0.52,0.525,0.53,0.535,
0.54,0.545,0.55,0.555,0.56,0.565,0.57,0.575,0.58,0.585,0.59,0.595,0.6,0.605,
0.61,0.615,0.62,0.625,0.63,0.635,0.64,0.645,0.65,0.655,0.66,0.665,0.67,
0.675,0.68,0.685,0.690000000000001,0.695000000000001,0.700000000000001,
0.705000000000001,0.710000000000001,0.715000000000001,0.720000000000001,
0.725000000000001,0.730000000000001,0.735000000000001,0.740000000000001,
0.745000000000001,0.750000000000001,0.755000000000001,0.760000000000001,
0.765000000000001,0.770000000000001,0.775000000000001,0.780000000000001,
0.785000000000001,0.790000000000001,0.795000000000001,0.800000000000001,
0.805000000000001,0.810000000000001,0.815000000000001,0.820000000000001,
0.825000000000001,0.830000000000001,0.835000000000001,0.840000000000001,
0.845000000000001,0.850000000000001,0.855000000000001,0.860000000000001,
0.865000000000001,0.870000000000001,0.875000000000001,0.880000000000001,
0.885000000000001,0.890000000000001,0.895000000000001,0.900000000000001,
0.905000000000001,0.910000000000001,0.915000000000001,0.920000000000001,
0.925000000000001,0.930000000000001,0.935000000000001,0.940000000000001,
0.945000000000001,0.950000000000001,0.955000000000001,0.960000000000001,
0.965000000000001,0.970000000000001,0.975000000000001,0.980000000000001,
0.985000000000001,0.990000000000001,0.995000000000001,1.),.UNSPECIFIED.)
CURVE()
GEOMETRIC_REPRESENTATION_ITEM()
RATIONAL_B_SPLINE_CURVE((1.,1.,1.,1.,1.,1.,1.,1.,1.,1.,1.,1.,1.,1.,1.,1.,
1.,1.,1.,1.,1.,1.,1.,1.,1.,1.,1.,1.,1.,1.,1.,1.,1.,1.,1.,1.,1.,1.,1.,1.,
1.,1.,1.,1.,1.,1.,1.,1.,1.,1.,1.,1.,1.,1.,1.,1.,1.,1.,1.,1.,1.,1.,1.,1.,
1.,1.,1.,1.,1.,1.,1.,1.,1.,1.,1.,1.,1.,1.,1.,1.,1.,1.,1.,1.,1.,1.,1.,1.,
1.,1.,1.,1.,1.,1.,1.,1.,1.,1.,1.,1.,1.,1.,1.,1.,1.,1.,1.,1.,1.,1.,1.,1.,
1.,1.,1.,1.,1.,1.,1.,1.,1.,1.,1.,1.,1.,1.,1.,1.,1.,1.,1.,1.,1.,1.,1.,1.,
1.,1.,1.,1.,1.,1.,1.,1.,1.,1.,1.,1.,1.,1.,1.,1.,1.,1.,1.,1.,1.,1.,1.,1.,
1.,1.,1.,1.,1.,1.,1.,1.,1.,1.,1.,1.,1.,1.,1.,1.,1.,1.,1.,1.,1.,1.,1.,1.,
1.,1.,1.,1.,1.,1.,1.,1.,1.,1.,1.,1.,1.,1.,1.,1.,1.,1.,1.,1.,1.))
REPRESENTATION_ITEM('')
);
#849=(
BOUNDED_CURVE()
B_SPLINE_CURVE(5,(#242022,#242023,#242024,#242025,#242026,#242027,#242028,
#242029,#242030,#242031,#242032,#242033,#242034,#242035,#242036,#242037,
#242038,#242039,#242040,#242041,#242042,#242043,#242044,#242045,#242046,
#242047,#242048,#242049,#242050,#242051,#242052,#242053,#242054,#242055,
#242056,#242057,#242058,#242059,#242060,#242061,#242062,#242063,#242064,
#242065,#242066,#242067,#242068,#242069,#242070,#242071,#242072,#242073,
#242074,#242075,#242076,#242077,#242078,#242079,#242080,#242081,#242082,
#242083,#242084,#242085,#242086,#242087,#242088,#242089,#242090,#242091,
#242092,#242093,#242094,#242095,#242096,#242097,#242098,#242099,#242100,
#242101,#242102,#242103,#242104,#242105,#242106,#242107,#242108,#242109,
#242110,#242111,#242112,#242113,#242114,#242115,#242116,#242117,#242118,
#242119,#242120,#242121,#242122,#242123,#242124,#242125,#242126,#242127,
#242128,#242129,#242130,#242131,#242132,#242133,#242134,#242135,#242136,
#242137,#242138,#242139,#242140,#242141,#242142,#242143,#242144,#242145,
#242146,#242147,#242148,#242149,#242150,#242151,#242152,#242153,#242154,
#242155,#242156,#242157,#242158,#242159,#242160,#242161,#242162,#242163,
#242164,#242165,#242166,#242167,#242168,#242169,#242170,#242171,#242172,
#242173,#242174,#242175,#242176,#242177,#242178,#242179,#242180,#242181,
#242182,#242183,#242184,#242185,#242186,#242187,#242188,#242189,#242190,
#242191,#242192,#242193,#242194,#242195,#242196,#242197,#242198,#242199,
#242200,#242201,#242202,#242203,#242204,#242205,#242206,#242207,#242208,
#242209,#242210,#242211,#242212,#242213,#242214,#242215,#242216,#242217,
#242218,#242219,#242220,#242221,#242222,#242223,#242224,#242225,#242226),
 .UNSPECIFIED.,.F.,.F.)
B_SPLINE_CURVE_WITH_KNOTS((6,1,1,1,1,1,1,1,1,1,1,1,1,1,1,1,1,1,1,1,1,1,
1,1,1,1,1,1,1,1,1,1,1,1,1,1,1,1,1,1,1,1,1,1,1,1,1,1,1,1,1,1,1,1,1,1,1,1,
1,1,1,1,1,1,1,1,1,1,1,1,1,1,1,1,1,1,1,1,1,1,1,1,1,1,1,1,1,1,1,1,1,1,1,1,
1,1,1,1,1,1,1,1,1,1,1,1,1,1,1,1,1,1,1,1,1,1,1,1,1,1,1,1,1,1,1,1,1,1,1,1,
1,1,1,1,1,1,1,1,1,1,1,1,1,1,1,1,1,1,1,1,1,1,1,1,1,1,1,1,1,1,1,1,1,1,1,1,
1,1,1,1,1,1,1,1,1,1,1,1,1,1,1,1,1,1,1,1,1,1,1,1,1,1,1,1,1,1,1,1,1,1,6),
(0.,0.005,0.01,0.015,0.02,0.025,0.03,0.035,0.04,0.045,0.05,0.055,0.06,0.065,
0.07,0.075,0.08,0.085,0.09,0.095,0.1,0.105,0.11,0.115,0.12,0.125,0.13,0.135,
0.14,0.145,0.15,0.155,0.16,0.165,0.17,0.175,0.18,0.185,0.19,0.195,0.2,0.205,
0.21,0.215,0.22,0.225,0.23,0.235,0.24,0.245,0.25,0.255,0.26,0.265,0.27,
0.275,0.28,0.285,0.29,0.295,0.3,0.305,0.31,0.315,0.32,0.325,0.33,0.335,
0.34,0.345,0.35,0.355,0.36,0.365,0.37,0.375,0.38,0.385,0.39,0.395,0.4,0.405,
0.41,0.415,0.42,0.425,0.43,0.435,0.44,0.445,0.45,0.455,0.46,0.465,0.47,
0.475,0.48,0.485,0.49,0.495,0.5,0.505,0.51,0.515,0.52,0.525,0.53,0.535,
0.54,0.545,0.55,0.555,0.56,0.565,0.57,0.575,0.58,0.585,0.59,0.595,0.6,0.605,
0.61,0.615,0.62,0.625,0.63,0.635,0.64,0.645,0.65,0.655,0.66,0.665,0.67,
0.675,0.68,0.685,0.690000000000001,0.695000000000001,0.700000000000001,
0.705000000000001,0.710000000000001,0.715000000000001,0.720000000000001,
0.725000000000001,0.730000000000001,0.735000000000001,0.740000000000001,
0.745000000000001,0.750000000000001,0.755000000000001,0.760000000000001,
0.765000000000001,0.770000000000001,0.775000000000001,0.780000000000001,
0.785000000000001,0.790000000000001,0.795000000000001,0.800000000000001,
0.805000000000001,0.810000000000001,0.815000000000001,0.820000000000001,
0.825000000000001,0.830000000000001,0.835000000000001,0.840000000000001,
0.845000000000001,0.850000000000001,0.855000000000001,0.860000000000001,
0.865000000000001,0.870000000000001,0.875000000000001,0.880000000000001,
0.885000000000001,0.890000000000001,0.895000000000001,0.900000000000001,
0.905000000000001,0.910000000000001,0.915000000000001,0.920000000000001,
0.925000000000001,0.930000000000001,0.935000000000001,0.940000000000001,
0.945000000000001,0.950000000000001,0.955000000000001,0.960000000000001,
0.965000000000001,0.970000000000001,0.975000000000001,0.980000000000001,
0.985000000000001,0.990000000000001,0.995000000000001,1.),.UNSPECIFIED.)
CURVE()
GEOMETRIC_REPRESENTATION_ITEM()
RATIONAL_B_SPLINE_CURVE((1.,1.,1.,1.,1.,1.,1.,1.,1.,1.,1.,1.,1.,1.,1.,1.,
1.,1.,1.,1.,1.,1.,1.,1.,1.,1.,1.,1.,1.,1.,1.,1.,1.,1.,1.,1.,1.,1.,1.,1.,
1.,1.,1.,1.,1.,1.,1.,1.,1.,1.,1.,1.,1.,1.,1.,1.,1.,1.,1.,1.,1.,1.,1.,1.,
1.,1.,1.,1.,1.,1.,1.,1.,1.,1.,1.,1.,1.,1.,1.,1.,1.,1.,1.,1.,1.,1.,1.,1.,
1.,1.,1.,1.,1.,1.,1.,1.,1.,1.,1.,1.,1.,1.,1.,1.,1.,1.,1.,1.,1.,1.,1.,1.,
1.,1.,1.,1.,1.,1.,1.,1.,1.,1.,1.,1.,1.,1.,1.,1.,1.,1.,1.,1.,1.,1.,1.,1.,
1.,1.,1.,1.,1.,1.,1.,1.,1.,1.,1.,1.,1.,1.,1.,1.,1.,1.,1.,1.,1.,1.,1.,1.,
1.,1.,1.,1.,1.,1.,1.,1.,1.,1.,1.,1.,1.,1.,1.,1.,1.,1.,1.,1.,1.,1.,1.,1.,
1.,1.,1.,1.,1.,1.,1.,1.,1.,1.,1.,1.,1.,1.,1.,1.,1.,1.,1.,1.,1.))
REPRESENTATION_ITEM('')
);
#850=(
BOUNDED_CURVE()
B_SPLINE_CURVE(5,(#242228,#242229,#242230,#242231,#242232,#242233,#242234,
#242235,#242236,#242237,#242238,#242239,#242240,#242241,#242242,#242243,
#242244,#242245,#242246,#242247,#242248,#242249,#242250,#242251,#242252,
#242253,#242254,#242255,#242256,#242257,#242258,#242259,#242260,#242261,
#242262,#242263,#242264,#242265,#242266,#242267,#242268,#242269,#242270,
#242271,#242272,#242273,#242274,#242275,#242276,#242277,#242278,#242279,
#242280,#242281,#242282,#242283,#242284,#242285,#242286,#242287,#242288,
#242289,#242290,#242291,#242292,#242293,#242294,#242295,#242296,#242297,
#242298,#242299,#242300,#242301,#242302,#242303,#242304,#242305,#242306,
#242307,#242308,#242309,#242310,#242311,#242312,#242313,#242314,#242315,
#242316,#242317,#242318,#242319,#242320,#242321,#242322,#242323,#242324,
#242325,#242326,#242327,#242328,#242329,#242330,#242331,#242332,#242333,
#242334,#242335,#242336,#242337,#242338,#242339,#242340,#242341,#242342,
#242343,#242344,#242345,#242346,#242347,#242348,#242349,#242350,#242351,
#242352,#242353,#242354,#242355,#242356,#242357,#242358,#242359,#242360,
#242361,#242362,#242363,#242364,#242365,#242366,#242367,#242368,#242369,
#242370,#242371,#242372,#242373,#242374,#242375,#242376,#242377,#242378,
#242379,#242380,#242381,#242382,#242383,#242384,#242385,#242386,#242387,
#242388,#242389,#242390,#242391,#242392,#242393,#242394,#242395,#242396,
#242397,#242398,#242399,#242400,#242401,#242402,#242403,#242404,#242405,
#242406,#242407,#242408,#242409,#242410,#242411,#242412,#242413,#242414,
#242415,#242416,#242417,#242418,#242419,#242420,#242421,#242422,#242423,
#242424,#242425,#242426,#242427,#242428,#242429,#242430,#242431,#242432),
 .UNSPECIFIED.,.F.,.F.)
B_SPLINE_CURVE_WITH_KNOTS((6,1,1,1,1,1,1,1,1,1,1,1,1,1,1,1,1,1,1,1,1,1,
1,1,1,1,1,1,1,1,1,1,1,1,1,1,1,1,1,1,1,1,1,1,1,1,1,1,1,1,1,1,1,1,1,1,1,1,
1,1,1,1,1,1,1,1,1,1,1,1,1,1,1,1,1,1,1,1,1,1,1,1,1,1,1,1,1,1,1,1,1,1,1,1,
1,1,1,1,1,1,1,1,1,1,1,1,1,1,1,1,1,1,1,1,1,1,1,1,1,1,1,1,1,1,1,1,1,1,1,1,
1,1,1,1,1,1,1,1,1,1,1,1,1,1,1,1,1,1,1,1,1,1,1,1,1,1,1,1,1,1,1,1,1,1,1,1,
1,1,1,1,1,1,1,1,1,1,1,1,1,1,1,1,1,1,1,1,1,1,1,1,1,1,1,1,1,1,1,1,1,1,6),
(-1.,-0.995000000000001,-0.990000000000001,-0.985000000000001,-0.980000000000001,
-0.975000000000001,-0.970000000000001,-0.965000000000001,-0.960000000000001,
-0.955000000000001,-0.950000000000001,-0.945000000000001,-0.940000000000001,
-0.935000000000001,-0.930000000000001,-0.925000000000001,-0.920000000000001,
-0.915000000000001,-0.910000000000001,-0.905000000000001,-0.900000000000001,
-0.895000000000001,-0.890000000000001,-0.885000000000001,-0.880000000000001,
-0.875000000000001,-0.870000000000001,-0.865000000000001,-0.860000000000001,
-0.855000000000001,-0.850000000000001,-0.845000000000001,-0.840000000000001,
-0.835000000000001,-0.830000000000001,-0.825000000000001,-0.820000000000001,
-0.815000000000001,-0.810000000000001,-0.805000000000001,-0.800000000000001,
-0.795000000000001,-0.790000000000001,-0.785000000000001,-0.780000000000001,
-0.775000000000001,-0.770000000000001,-0.765000000000001,-0.760000000000001,
-0.755000000000001,-0.750000000000001,-0.745000000000001,-0.740000000000001,
-0.735000000000001,-0.730000000000001,-0.725000000000001,-0.720000000000001,
-0.715000000000001,-0.710000000000001,-0.705000000000001,-0.700000000000001,
-0.695000000000001,-0.690000000000001,-0.685,-0.68,-0.675,-0.67,-0.665,
-0.66,-0.655,-0.65,-0.645,-0.64,-0.635,-0.63,-0.625,-0.62,-0.615,-0.61,
-0.605,-0.6,-0.595,-0.59,-0.585,-0.58,-0.575,-0.57,-0.565,-0.56,-0.555,
-0.55,-0.545,-0.54,-0.535,-0.53,-0.525,-0.52,-0.515,-0.51,-0.505,-0.5,-0.495,
-0.49,-0.485,-0.48,-0.475,-0.47,-0.465,-0.46,-0.455,-0.45,-0.445,-0.44,
-0.435,-0.43,-0.425,-0.42,-0.415,-0.41,-0.405,-0.4,-0.395,-0.39,-0.385,
-0.38,-0.375,-0.37,-0.365,-0.36,-0.355,-0.35,-0.345,-0.34,-0.335,-0.33,
-0.325,-0.32,-0.315,-0.31,-0.305,-0.3,-0.295,-0.29,-0.285,-0.28,-0.275,
-0.27,-0.265,-0.26,-0.255,-0.25,-0.245,-0.24,-0.235,-0.23,-0.225,-0.22,
-0.215,-0.21,-0.205,-0.2,-0.195,-0.19,-0.185,-0.18,-0.175,-0.17,-0.165,
-0.16,-0.155,-0.15,-0.145,-0.14,-0.135,-0.13,-0.125,-0.12,-0.115,-0.11,
-0.105,-0.1,-0.095,-0.09,-0.085,-0.08,-0.075,-0.07,-0.065,-0.06,-0.055,
-0.05,-0.045,-0.04,-0.035,-0.03,-0.025,-0.02,-0.015,-0.01,-0.005,0.),
 .UNSPECIFIED.)
CURVE()
GEOMETRIC_REPRESENTATION_ITEM()
RATIONAL_B_SPLINE_CURVE((1.,1.,1.,1.,1.,1.,1.,1.,1.,1.,1.,1.,1.,1.,1.,1.,
1.,1.,1.,1.,1.,1.,1.,1.,1.,1.,1.,1.,1.,1.,1.,1.,1.,1.,1.,1.,1.,1.,1.,1.,
1.,1.,1.,1.,1.,1.,1.,1.,1.,1.,1.,1.,1.,1.,1.,1.,1.,1.,1.,1.,1.,1.,1.,1.,
1.,1.,1.,1.,1.,1.,1.,1.,1.,1.,1.,1.,1.,1.,1.,1.,1.,1.,1.,1.,1.,1.,1.,1.,
1.,1.,1.,1.,1.,1.,1.,1.,1.,1.,1.,1.,1.,1.,1.,1.,1.,1.,1.,1.,1.,1.,1.,1.,
1.,1.,1.,1.,1.,1.,1.,1.,1.,1.,1.,1.,1.,1.,1.,1.,1.,1.,1.,1.,1.,1.,1.,1.,
1.,1.,1.,1.,1.,1.,1.,1.,1.,1.,1.,1.,1.,1.,1.,1.,1.,1.,1.,1.,1.,1.,1.,1.,
1.,1.,1.,1.,1.,1.,1.,1.,1.,1.,1.,1.,1.,1.,1.,1.,1.,1.,1.,1.,1.,1.,1.,1.,
1.,1.,1.,1.,1.,1.,1.,1.,1.,1.,1.,1.,1.,1.,1.,1.,1.,1.,1.,1.,1.))
REPRESENTATION_ITEM('')
);
#851=(
BOUNDED_CURVE()
B_SPLINE_CURVE(5,(#242851,#242852,#242853,#242854,#242855,#242856,#242857,
#242858,#242859,#242860,#242861,#242862,#242863,#242864,#242865,#242866,
#242867,#242868,#242869,#242870,#242871,#242872,#242873,#242874,#242875,
#242876,#242877,#242878,#242879,#242880,#242881,#242882,#242883,#242884,
#242885,#242886,#242887,#242888,#242889,#242890,#242891,#242892,#242893,
#242894,#242895,#242896,#242897,#242898,#242899,#242900,#242901,#242902,
#242903,#242904,#242905,#242906,#242907,#242908,#242909,#242910,#242911,
#242912,#242913,#242914,#242915,#242916,#242917,#242918,#242919,#242920,
#242921,#242922,#242923,#242924,#242925,#242926,#242927,#242928,#242929,
#242930,#242931,#242932,#242933,#242934,#242935,#242936,#242937,#242938,
#242939,#242940,#242941,#242942,#242943,#242944,#242945,#242946,#242947,
#242948,#242949,#242950,#242951,#242952,#242953,#242954,#242955,#242956,
#242957,#242958,#242959,#242960,#242961,#242962,#242963,#242964,#242965,
#242966,#242967,#242968,#242969,#242970,#242971,#242972,#242973,#242974,
#242975,#242976,#242977,#242978,#242979,#242980,#242981,#242982,#242983,
#242984,#242985,#242986,#242987,#242988,#242989,#242990,#242991,#242992,
#242993,#242994,#242995,#242996,#242997,#242998,#242999,#243000,#243001,
#243002,#243003,#243004,#243005,#243006,#243007,#243008,#243009,#243010,
#243011,#243012,#243013,#243014,#243015,#243016,#243017,#243018,#243019,
#243020,#243021,#243022,#243023,#243024,#243025,#243026,#243027,#243028,
#243029,#243030,#243031,#243032,#243033,#243034,#243035,#243036,#243037,
#243038,#243039,#243040,#243041,#243042,#243043,#243044,#243045,#243046,
#243047,#243048,#243049,#243050,#243051,#243052,#243053,#243054,#243055),
 .UNSPECIFIED.,.F.,.F.)
B_SPLINE_CURVE_WITH_KNOTS((6,1,1,1,1,1,1,1,1,1,1,1,1,1,1,1,1,1,1,1,1,1,
1,1,1,1,1,1,1,1,1,1,1,1,1,1,1,1,1,1,1,1,1,1,1,1,1,1,1,1,1,1,1,1,1,1,1,1,
1,1,1,1,1,1,1,1,1,1,1,1,1,1,1,1,1,1,1,1,1,1,1,1,1,1,1,1,1,1,1,1,1,1,1,1,
1,1,1,1,1,1,1,1,1,1,1,1,1,1,1,1,1,1,1,1,1,1,1,1,1,1,1,1,1,1,1,1,1,1,1,1,
1,1,1,1,1,1,1,1,1,1,1,1,1,1,1,1,1,1,1,1,1,1,1,1,1,1,1,1,1,1,1,1,1,1,1,1,
1,1,1,1,1,1,1,1,1,1,1,1,1,1,1,1,1,1,1,1,1,1,1,1,1,1,1,1,1,1,1,1,1,1,6),
(-1.,-0.995000000000001,-0.990000000000001,-0.985000000000001,-0.980000000000001,
-0.975000000000001,-0.970000000000001,-0.965000000000001,-0.960000000000001,
-0.955000000000001,-0.950000000000001,-0.945000000000001,-0.940000000000001,
-0.935000000000001,-0.930000000000001,-0.925000000000001,-0.920000000000001,
-0.915000000000001,-0.910000000000001,-0.905000000000001,-0.900000000000001,
-0.895000000000001,-0.890000000000001,-0.885000000000001,-0.880000000000001,
-0.875000000000001,-0.870000000000001,-0.865000000000001,-0.860000000000001,
-0.855000000000001,-0.850000000000001,-0.845000000000001,-0.840000000000001,
-0.835000000000001,-0.830000000000001,-0.825000000000001,-0.820000000000001,
-0.815000000000001,-0.810000000000001,-0.805000000000001,-0.800000000000001,
-0.795000000000001,-0.790000000000001,-0.785000000000001,-0.780000000000001,
-0.775000000000001,-0.770000000000001,-0.765000000000001,-0.760000000000001,
-0.755000000000001,-0.750000000000001,-0.745000000000001,-0.740000000000001,
-0.735000000000001,-0.730000000000001,-0.725000000000001,-0.720000000000001,
-0.715000000000001,-0.710000000000001,-0.705000000000001,-0.700000000000001,
-0.695000000000001,-0.690000000000001,-0.685,-0.68,-0.675,-0.67,-0.665,
-0.66,-0.655,-0.65,-0.645,-0.64,-0.635,-0.63,-0.625,-0.62,-0.615,-0.61,
-0.605,-0.6,-0.595,-0.59,-0.585,-0.58,-0.575,-0.57,-0.565,-0.56,-0.555,
-0.55,-0.545,-0.54,-0.535,-0.53,-0.525,-0.52,-0.515,-0.51,-0.505,-0.5,-0.495,
-0.49,-0.485,-0.48,-0.475,-0.47,-0.465,-0.46,-0.455,-0.45,-0.445,-0.44,
-0.435,-0.43,-0.425,-0.42,-0.415,-0.41,-0.405,-0.4,-0.395,-0.39,-0.385,
-0.38,-0.375,-0.37,-0.365,-0.36,-0.355,-0.35,-0.345,-0.34,-0.335,-0.33,
-0.325,-0.32,-0.315,-0.31,-0.305,-0.3,-0.295,-0.29,-0.285,-0.28,-0.275,
-0.27,-0.265,-0.26,-0.255,-0.25,-0.245,-0.24,-0.235,-0.23,-0.225,-0.22,
-0.215,-0.21,-0.205,-0.2,-0.195,-0.19,-0.185,-0.18,-0.175,-0.17,-0.165,
-0.16,-0.155,-0.15,-0.145,-0.14,-0.135,-0.13,-0.125,-0.12,-0.115,-0.11,
-0.105,-0.1,-0.095,-0.09,-0.085,-0.08,-0.075,-0.07,-0.065,-0.06,-0.055,
-0.05,-0.045,-0.04,-0.035,-0.03,-0.025,-0.02,-0.015,-0.01,-0.005,0.),
 .UNSPECIFIED.)
CURVE()
GEOMETRIC_REPRESENTATION_ITEM()
RATIONAL_B_SPLINE_CURVE((1.,1.,1.,1.,1.,1.,1.,1.,1.,1.,1.,1.,1.,1.,1.,1.,
1.,1.,1.,1.,1.,1.,1.,1.,1.,1.,1.,1.,1.,1.,1.,1.,1.,1.,1.,1.,1.,1.,1.,1.,
1.,1.,1.,1.,1.,1.,1.,1.,1.,1.,1.,1.,1.,1.,1.,1.,1.,1.,1.,1.,1.,1.,1.,1.,
1.,1.,1.,1.,1.,1.,1.,1.,1.,1.,1.,1.,1.,1.,1.,1.,1.,1.,1.,1.,1.,1.,1.,1.,
1.,1.,1.,1.,1.,1.,1.,1.,1.,1.,1.,1.,1.,1.,1.,1.,1.,1.,1.,1.,1.,1.,1.,1.,
1.,1.,1.,1.,1.,1.,1.,1.,1.,1.,1.,1.,1.,1.,1.,1.,1.,1.,1.,1.,1.,1.,1.,1.,
1.,1.,1.,1.,1.,1.,1.,1.,1.,1.,1.,1.,1.,1.,1.,1.,1.,1.,1.,1.,1.,1.,1.,1.,
1.,1.,1.,1.,1.,1.,1.,1.,1.,1.,1.,1.,1.,1.,1.,1.,1.,1.,1.,1.,1.,1.,1.,1.,
1.,1.,1.,1.,1.,1.,1.,1.,1.,1.,1.,1.,1.,1.,1.,1.,1.,1.,1.,1.,1.))
REPRESENTATION_ITEM('')
);
#852=(
BOUNDED_CURVE()
B_SPLINE_CURVE(5,(#243058,#243059,#243060,#243061,#243062,#243063,#243064,
#243065,#243066,#243067,#243068,#243069,#243070,#243071,#243072,#243073,
#243074,#243075,#243076,#243077,#243078,#243079,#243080,#243081,#243082,
#243083,#243084,#243085,#243086,#243087,#243088,#243089,#243090,#243091,
#243092,#243093,#243094,#243095,#243096,#243097,#243098,#243099,#243100,
#243101,#243102,#243103,#243104,#243105,#243106,#243107,#243108,#243109,
#243110,#243111,#243112,#243113,#243114,#243115,#243116,#243117,#243118,
#243119,#243120,#243121,#243122,#243123,#243124,#243125,#243126,#243127,
#243128,#243129,#243130,#243131,#243132,#243133,#243134,#243135,#243136,
#243137,#243138,#243139,#243140,#243141,#243142,#243143,#243144,#243145,
#243146,#243147,#243148,#243149,#243150,#243151,#243152,#243153,#243154,
#243155,#243156,#243157,#243158,#243159,#243160,#243161,#243162,#243163,
#243164,#243165,#243166,#243167,#243168,#243169,#243170,#243171,#243172,
#243173,#243174,#243175,#243176,#243177,#243178,#243179,#243180,#243181,
#243182,#243183,#243184,#243185,#243186,#243187,#243188,#243189,#243190,
#243191,#243192,#243193,#243194,#243195,#243196,#243197,#243198,#243199,
#243200,#243201,#243202,#243203,#243204,#243205,#243206,#243207,#243208,
#243209,#243210,#243211,#243212,#243213,#243214,#243215,#243216,#243217,
#243218,#243219,#243220,#243221,#243222,#243223,#243224,#243225,#243226,
#243227,#243228,#243229,#243230,#243231,#243232,#243233,#243234,#243235,
#243236,#243237,#243238,#243239,#243240,#243241,#243242,#243243,#243244,
#243245,#243246,#243247,#243248,#243249,#243250,#243251,#243252,#243253,
#243254,#243255,#243256,#243257,#243258,#243259,#243260,#243261,#243262),
 .UNSPECIFIED.,.F.,.F.)
B_SPLINE_CURVE_WITH_KNOTS((6,1,1,1,1,1,1,1,1,1,1,1,1,1,1,1,1,1,1,1,1,1,
1,1,1,1,1,1,1,1,1,1,1,1,1,1,1,1,1,1,1,1,1,1,1,1,1,1,1,1,1,1,1,1,1,1,1,1,
1,1,1,1,1,1,1,1,1,1,1,1,1,1,1,1,1,1,1,1,1,1,1,1,1,1,1,1,1,1,1,1,1,1,1,1,
1,1,1,1,1,1,1,1,1,1,1,1,1,1,1,1,1,1,1,1,1,1,1,1,1,1,1,1,1,1,1,1,1,1,1,1,
1,1,1,1,1,1,1,1,1,1,1,1,1,1,1,1,1,1,1,1,1,1,1,1,1,1,1,1,1,1,1,1,1,1,1,1,
1,1,1,1,1,1,1,1,1,1,1,1,1,1,1,1,1,1,1,1,1,1,1,1,1,1,1,1,1,1,1,1,1,1,6),
(0.,0.005,0.01,0.015,0.02,0.025,0.03,0.035,0.04,0.045,0.05,0.055,0.06,0.065,
0.07,0.075,0.08,0.085,0.09,0.095,0.1,0.105,0.11,0.115,0.12,0.125,0.13,0.135,
0.14,0.145,0.15,0.155,0.16,0.165,0.17,0.175,0.18,0.185,0.19,0.195,0.2,0.205,
0.21,0.215,0.22,0.225,0.23,0.235,0.24,0.245,0.25,0.255,0.26,0.265,0.27,
0.275,0.28,0.285,0.29,0.295,0.3,0.305,0.31,0.315,0.32,0.325,0.33,0.335,
0.34,0.345,0.35,0.355,0.36,0.365,0.37,0.375,0.38,0.385,0.39,0.395,0.4,0.405,
0.41,0.415,0.42,0.425,0.43,0.435,0.44,0.445,0.45,0.455,0.46,0.465,0.47,
0.475,0.48,0.485,0.49,0.495,0.5,0.505,0.51,0.515,0.52,0.525,0.53,0.535,
0.54,0.545,0.55,0.555,0.56,0.565,0.57,0.575,0.58,0.585,0.59,0.595,0.6,0.605,
0.61,0.615,0.62,0.625,0.63,0.635,0.64,0.645,0.65,0.655,0.66,0.665,0.67,
0.675,0.68,0.685,0.690000000000001,0.695000000000001,0.700000000000001,
0.705000000000001,0.710000000000001,0.715000000000001,0.720000000000001,
0.725000000000001,0.730000000000001,0.735000000000001,0.740000000000001,
0.745000000000001,0.750000000000001,0.755000000000001,0.760000000000001,
0.765000000000001,0.770000000000001,0.775000000000001,0.780000000000001,
0.785000000000001,0.790000000000001,0.795000000000001,0.800000000000001,
0.805000000000001,0.810000000000001,0.815000000000001,0.820000000000001,
0.825000000000001,0.830000000000001,0.835000000000001,0.840000000000001,
0.845000000000001,0.850000000000001,0.855000000000001,0.860000000000001,
0.865000000000001,0.870000000000001,0.875000000000001,0.880000000000001,
0.885000000000001,0.890000000000001,0.895000000000001,0.900000000000001,
0.905000000000001,0.910000000000001,0.915000000000001,0.920000000000001,
0.925000000000001,0.930000000000001,0.935000000000001,0.940000000000001,
0.945000000000001,0.950000000000001,0.955000000000001,0.960000000000001,
0.965000000000001,0.970000000000001,0.975000000000001,0.980000000000001,
0.985000000000001,0.990000000000001,0.995000000000001,1.),.UNSPECIFIED.)
CURVE()
GEOMETRIC_REPRESENTATION_ITEM()
RATIONAL_B_SPLINE_CURVE((1.,1.,1.,1.,1.,1.,1.,1.,1.,1.,1.,1.,1.,1.,1.,1.,
1.,1.,1.,1.,1.,1.,1.,1.,1.,1.,1.,1.,1.,1.,1.,1.,1.,1.,1.,1.,1.,1.,1.,1.,
1.,1.,1.,1.,1.,1.,1.,1.,1.,1.,1.,1.,1.,1.,1.,1.,1.,1.,1.,1.,1.,1.,1.,1.,
1.,1.,1.,1.,1.,1.,1.,1.,1.,1.,1.,1.,1.,1.,1.,1.,1.,1.,1.,1.,1.,1.,1.,1.,
1.,1.,1.,1.,1.,1.,1.,1.,1.,1.,1.,1.,1.,1.,1.,1.,1.,1.,1.,1.,1.,1.,1.,1.,
1.,1.,1.,1.,1.,1.,1.,1.,1.,1.,1.,1.,1.,1.,1.,1.,1.,1.,1.,1.,1.,1.,1.,1.,
1.,1.,1.,1.,1.,1.,1.,1.,1.,1.,1.,1.,1.,1.,1.,1.,1.,1.,1.,1.,1.,1.,1.,1.,
1.,1.,1.,1.,1.,1.,1.,1.,1.,1.,1.,1.,1.,1.,1.,1.,1.,1.,1.,1.,1.,1.,1.,1.,
1.,1.,1.,1.,1.,1.,1.,1.,1.,1.,1.,1.,1.,1.,1.,1.,1.,1.,1.,1.,1.))
REPRESENTATION_ITEM('')
);
#853=(
BOUNDED_CURVE()
B_SPLINE_CURVE(5,(#243674,#243675,#243676,#243677,#243678,#243679,#243680,
#243681,#243682,#243683,#243684,#243685,#243686,#243687,#243688,#243689,
#243690,#243691,#243692,#243693,#243694,#243695,#243696,#243697,#243698,
#243699,#243700,#243701,#243702,#243703,#243704,#243705,#243706,#243707,
#243708,#243709,#243710,#243711,#243712,#243713,#243714,#243715,#243716,
#243717,#243718,#243719,#243720,#243721,#243722,#243723,#243724,#243725,
#243726,#243727,#243728,#243729,#243730,#243731,#243732,#243733,#243734,
#243735,#243736,#243737,#243738,#243739,#243740,#243741,#243742,#243743,
#243744,#243745,#243746,#243747,#243748,#243749,#243750,#243751,#243752,
#243753,#243754,#243755,#243756,#243757,#243758,#243759,#243760,#243761,
#243762,#243763,#243764,#243765,#243766,#243767,#243768,#243769,#243770,
#243771,#243772,#243773,#243774,#243775,#243776,#243777,#243778,#243779,
#243780,#243781,#243782,#243783,#243784,#243785,#243786,#243787,#243788,
#243789,#243790,#243791,#243792,#243793,#243794,#243795,#243796,#243797,
#243798,#243799,#243800,#243801,#243802,#243803,#243804,#243805,#243806,
#243807,#243808,#243809,#243810,#243811,#243812,#243813,#243814,#243815,
#243816,#243817,#243818,#243819,#243820,#243821,#243822,#243823,#243824,
#243825,#243826,#243827,#243828,#243829,#243830,#243831,#243832,#243833,
#243834,#243835,#243836,#243837,#243838,#243839,#243840,#243841,#243842,
#243843,#243844,#243845,#243846,#243847,#243848,#243849,#243850,#243851,
#243852,#243853,#243854,#243855,#243856,#243857,#243858,#243859,#243860,
#243861,#243862,#243863,#243864,#243865,#243866,#243867,#243868,#243869,
#243870,#243871,#243872,#243873,#243874,#243875,#243876,#243877,#243878),
 .UNSPECIFIED.,.F.,.F.)
B_SPLINE_CURVE_WITH_KNOTS((6,1,1,1,1,1,1,1,1,1,1,1,1,1,1,1,1,1,1,1,1,1,
1,1,1,1,1,1,1,1,1,1,1,1,1,1,1,1,1,1,1,1,1,1,1,1,1,1,1,1,1,1,1,1,1,1,1,1,
1,1,1,1,1,1,1,1,1,1,1,1,1,1,1,1,1,1,1,1,1,1,1,1,1,1,1,1,1,1,1,1,1,1,1,1,
1,1,1,1,1,1,1,1,1,1,1,1,1,1,1,1,1,1,1,1,1,1,1,1,1,1,1,1,1,1,1,1,1,1,1,1,
1,1,1,1,1,1,1,1,1,1,1,1,1,1,1,1,1,1,1,1,1,1,1,1,1,1,1,1,1,1,1,1,1,1,1,1,
1,1,1,1,1,1,1,1,1,1,1,1,1,1,1,1,1,1,1,1,1,1,1,1,1,1,1,1,1,1,1,1,1,1,6),
(0.,0.005,0.01,0.015,0.02,0.025,0.03,0.035,0.04,0.045,0.05,0.055,0.06,0.065,
0.07,0.075,0.08,0.085,0.09,0.095,0.1,0.105,0.11,0.115,0.12,0.125,0.13,0.135,
0.14,0.145,0.15,0.155,0.16,0.165,0.17,0.175,0.18,0.185,0.19,0.195,0.2,0.205,
0.21,0.215,0.22,0.225,0.23,0.235,0.24,0.245,0.25,0.255,0.26,0.265,0.27,
0.275,0.28,0.285,0.29,0.295,0.3,0.305,0.31,0.315,0.32,0.325,0.33,0.335,
0.34,0.345,0.35,0.355,0.36,0.365,0.37,0.375,0.38,0.385,0.39,0.395,0.4,0.405,
0.41,0.415,0.42,0.425,0.43,0.435,0.44,0.445,0.45,0.455,0.46,0.465,0.47,
0.475,0.48,0.485,0.49,0.495,0.5,0.505,0.51,0.515,0.52,0.525,0.53,0.535,
0.54,0.545,0.55,0.555,0.56,0.565,0.57,0.575,0.58,0.585,0.59,0.595,0.6,0.605,
0.61,0.615,0.62,0.625,0.63,0.635,0.64,0.645,0.65,0.655,0.66,0.665,0.67,
0.675,0.68,0.685,0.690000000000001,0.695000000000001,0.700000000000001,
0.705000000000001,0.710000000000001,0.715000000000001,0.720000000000001,
0.725000000000001,0.730000000000001,0.735000000000001,0.740000000000001,
0.745000000000001,0.750000000000001,0.755000000000001,0.760000000000001,
0.765000000000001,0.770000000000001,0.775000000000001,0.780000000000001,
0.785000000000001,0.790000000000001,0.795000000000001,0.800000000000001,
0.805000000000001,0.810000000000001,0.815000000000001,0.820000000000001,
0.825000000000001,0.830000000000001,0.835000000000001,0.840000000000001,
0.845000000000001,0.850000000000001,0.855000000000001,0.860000000000001,
0.865000000000001,0.870000000000001,0.875000000000001,0.880000000000001,
0.885000000000001,0.890000000000001,0.895000000000001,0.900000000000001,
0.905000000000001,0.910000000000001,0.915000000000001,0.920000000000001,
0.925000000000001,0.930000000000001,0.935000000000001,0.940000000000001,
0.945000000000001,0.950000000000001,0.955000000000001,0.960000000000001,
0.965000000000001,0.970000000000001,0.975000000000001,0.980000000000001,
0.985000000000001,0.990000000000001,0.995000000000001,1.),.UNSPECIFIED.)
CURVE()
GEOMETRIC_REPRESENTATION_ITEM()
RATIONAL_B_SPLINE_CURVE((1.,1.,1.,1.,1.,1.,1.,1.,1.,1.,1.,1.,1.,1.,1.,1.,
1.,1.,1.,1.,1.,1.,1.,1.,1.,1.,1.,1.,1.,1.,1.,1.,1.,1.,1.,1.,1.,1.,1.,1.,
1.,1.,1.,1.,1.,1.,1.,1.,1.,1.,1.,1.,1.,1.,1.,1.,1.,1.,1.,1.,1.,1.,1.,1.,
1.,1.,1.,1.,1.,1.,1.,1.,1.,1.,1.,1.,1.,1.,1.,1.,1.,1.,1.,1.,1.,1.,1.,1.,
1.,1.,1.,1.,1.,1.,1.,1.,1.,1.,1.,1.,1.,1.,1.,1.,1.,1.,1.,1.,1.,1.,1.,1.,
1.,1.,1.,1.,1.,1.,1.,1.,1.,1.,1.,1.,1.,1.,1.,1.,1.,1.,1.,1.,1.,1.,1.,1.,
1.,1.,1.,1.,1.,1.,1.,1.,1.,1.,1.,1.,1.,1.,1.,1.,1.,1.,1.,1.,1.,1.,1.,1.,
1.,1.,1.,1.,1.,1.,1.,1.,1.,1.,1.,1.,1.,1.,1.,1.,1.,1.,1.,1.,1.,1.,1.,1.,
1.,1.,1.,1.,1.,1.,1.,1.,1.,1.,1.,1.,1.,1.,1.,1.,1.,1.,1.,1.,1.))
REPRESENTATION_ITEM('')
);
#854=(
BOUNDED_CURVE()
B_SPLINE_CURVE(5,(#243880,#243881,#243882,#243883,#243884,#243885,#243886,
#243887,#243888,#243889,#243890,#243891,#243892,#243893,#243894,#243895,
#243896,#243897,#243898,#243899,#243900,#243901,#243902,#243903,#243904,
#243905,#243906,#243907,#243908,#243909,#243910,#243911,#243912,#243913,
#243914,#243915,#243916,#243917,#243918,#243919,#243920,#243921,#243922,
#243923,#243924,#243925,#243926,#243927,#243928,#243929,#243930,#243931,
#243932,#243933,#243934,#243935,#243936,#243937,#243938,#243939,#243940,
#243941,#243942,#243943,#243944,#243945,#243946,#243947,#243948,#243949,
#243950,#243951,#243952,#243953,#243954,#243955,#243956,#243957,#243958,
#243959,#243960,#243961,#243962,#243963,#243964,#243965,#243966,#243967,
#243968,#243969,#243970,#243971,#243972,#243973,#243974,#243975,#243976,
#243977,#243978,#243979,#243980,#243981,#243982,#243983,#243984,#243985,
#243986,#243987,#243988,#243989,#243990,#243991,#243992,#243993,#243994,
#243995,#243996,#243997,#243998,#243999,#244000,#244001,#244002,#244003,
#244004,#244005,#244006,#244007,#244008,#244009,#244010,#244011,#244012,
#244013,#244014,#244015,#244016,#244017,#244018,#244019,#244020,#244021,
#244022,#244023,#244024,#244025,#244026,#244027,#244028,#244029,#244030,
#244031,#244032,#244033,#244034,#244035,#244036,#244037,#244038,#244039,
#244040,#244041,#244042,#244043,#244044,#244045,#244046,#244047,#244048,
#244049,#244050,#244051,#244052,#244053,#244054,#244055,#244056,#244057,
#244058,#244059,#244060,#244061,#244062,#244063,#244064,#244065,#244066,
#244067,#244068,#244069,#244070,#244071,#244072,#244073,#244074,#244075,
#244076,#244077,#244078,#244079,#244080,#244081,#244082,#244083,#244084),
 .UNSPECIFIED.,.F.,.F.)
B_SPLINE_CURVE_WITH_KNOTS((6,1,1,1,1,1,1,1,1,1,1,1,1,1,1,1,1,1,1,1,1,1,
1,1,1,1,1,1,1,1,1,1,1,1,1,1,1,1,1,1,1,1,1,1,1,1,1,1,1,1,1,1,1,1,1,1,1,1,
1,1,1,1,1,1,1,1,1,1,1,1,1,1,1,1,1,1,1,1,1,1,1,1,1,1,1,1,1,1,1,1,1,1,1,1,
1,1,1,1,1,1,1,1,1,1,1,1,1,1,1,1,1,1,1,1,1,1,1,1,1,1,1,1,1,1,1,1,1,1,1,1,
1,1,1,1,1,1,1,1,1,1,1,1,1,1,1,1,1,1,1,1,1,1,1,1,1,1,1,1,1,1,1,1,1,1,1,1,
1,1,1,1,1,1,1,1,1,1,1,1,1,1,1,1,1,1,1,1,1,1,1,1,1,1,1,1,1,1,1,1,1,1,6),
(-1.,-0.995000000000001,-0.990000000000001,-0.985000000000001,-0.980000000000001,
-0.975000000000001,-0.970000000000001,-0.965000000000001,-0.960000000000001,
-0.955000000000001,-0.950000000000001,-0.945000000000001,-0.940000000000001,
-0.935000000000001,-0.930000000000001,-0.925000000000001,-0.920000000000001,
-0.915000000000001,-0.910000000000001,-0.905000000000001,-0.900000000000001,
-0.895000000000001,-0.890000000000001,-0.885000000000001,-0.880000000000001,
-0.875000000000001,-0.870000000000001,-0.865000000000001,-0.860000000000001,
-0.855000000000001,-0.850000000000001,-0.845000000000001,-0.840000000000001,
-0.835000000000001,-0.830000000000001,-0.825000000000001,-0.820000000000001,
-0.815000000000001,-0.810000000000001,-0.805000000000001,-0.800000000000001,
-0.795000000000001,-0.790000000000001,-0.785000000000001,-0.780000000000001,
-0.775000000000001,-0.770000000000001,-0.765000000000001,-0.760000000000001,
-0.755000000000001,-0.750000000000001,-0.745000000000001,-0.740000000000001,
-0.735000000000001,-0.730000000000001,-0.725000000000001,-0.720000000000001,
-0.715000000000001,-0.710000000000001,-0.705000000000001,-0.700000000000001,
-0.695000000000001,-0.690000000000001,-0.685,-0.68,-0.675,-0.67,-0.665,
-0.66,-0.655,-0.65,-0.645,-0.64,-0.635,-0.63,-0.625,-0.62,-0.615,-0.61,
-0.605,-0.6,-0.595,-0.59,-0.585,-0.58,-0.575,-0.57,-0.565,-0.56,-0.555,
-0.55,-0.545,-0.54,-0.535,-0.53,-0.525,-0.52,-0.515,-0.51,-0.505,-0.5,-0.495,
-0.49,-0.485,-0.48,-0.475,-0.47,-0.465,-0.46,-0.455,-0.45,-0.445,-0.44,
-0.435,-0.43,-0.425,-0.42,-0.415,-0.41,-0.405,-0.4,-0.395,-0.39,-0.385,
-0.38,-0.375,-0.37,-0.365,-0.36,-0.355,-0.35,-0.345,-0.34,-0.335,-0.33,
-0.325,-0.32,-0.315,-0.31,-0.305,-0.3,-0.295,-0.29,-0.285,-0.28,-0.275,
-0.27,-0.265,-0.26,-0.255,-0.25,-0.245,-0.24,-0.235,-0.23,-0.225,-0.22,
-0.215,-0.21,-0.205,-0.2,-0.195,-0.19,-0.185,-0.18,-0.175,-0.17,-0.165,
-0.16,-0.155,-0.15,-0.145,-0.14,-0.135,-0.13,-0.125,-0.12,-0.115,-0.11,
-0.105,-0.1,-0.095,-0.09,-0.085,-0.08,-0.075,-0.07,-0.065,-0.06,-0.055,
-0.05,-0.045,-0.04,-0.035,-0.03,-0.025,-0.02,-0.015,-0.01,-0.005,0.),
 .UNSPECIFIED.)
CURVE()
GEOMETRIC_REPRESENTATION_ITEM()
RATIONAL_B_SPLINE_CURVE((1.,1.,1.,1.,1.,1.,1.,1.,1.,1.,1.,1.,1.,1.,1.,1.,
1.,1.,1.,1.,1.,1.,1.,1.,1.,1.,1.,1.,1.,1.,1.,1.,1.,1.,1.,1.,1.,1.,1.,1.,
1.,1.,1.,1.,1.,1.,1.,1.,1.,1.,1.,1.,1.,1.,1.,1.,1.,1.,1.,1.,1.,1.,1.,1.,
1.,1.,1.,1.,1.,1.,1.,1.,1.,1.,1.,1.,1.,1.,1.,1.,1.,1.,1.,1.,1.,1.,1.,1.,
1.,1.,1.,1.,1.,1.,1.,1.,1.,1.,1.,1.,1.,1.,1.,1.,1.,1.,1.,1.,1.,1.,1.,1.,
1.,1.,1.,1.,1.,1.,1.,1.,1.,1.,1.,1.,1.,1.,1.,1.,1.,1.,1.,1.,1.,1.,1.,1.,
1.,1.,1.,1.,1.,1.,1.,1.,1.,1.,1.,1.,1.,1.,1.,1.,1.,1.,1.,1.,1.,1.,1.,1.,
1.,1.,1.,1.,1.,1.,1.,1.,1.,1.,1.,1.,1.,1.,1.,1.,1.,1.,1.,1.,1.,1.,1.,1.,
1.,1.,1.,1.,1.,1.,1.,1.,1.,1.,1.,1.,1.,1.,1.,1.,1.,1.,1.,1.,1.))
REPRESENTATION_ITEM('')
);
#855=(
BOUNDED_CURVE()
B_SPLINE_CURVE(5,(#244503,#244504,#244505,#244506,#244507,#244508,#244509,
#244510,#244511,#244512,#244513,#244514,#244515,#244516,#244517,#244518,
#244519,#244520,#244521,#244522,#244523,#244524,#244525,#244526,#244527,
#244528,#244529,#244530,#244531,#244532,#244533,#244534,#244535,#244536,
#244537,#244538,#244539,#244540,#244541,#244542,#244543,#244544,#244545,
#244546,#244547,#244548,#244549,#244550,#244551,#244552,#244553,#244554,
#244555,#244556,#244557,#244558,#244559,#244560,#244561,#244562,#244563,
#244564,#244565,#244566,#244567,#244568,#244569,#244570,#244571,#244572,
#244573,#244574,#244575,#244576,#244577,#244578,#244579,#244580,#244581,
#244582,#244583,#244584,#244585,#244586,#244587,#244588,#244589,#244590,
#244591,#244592,#244593,#244594,#244595,#244596,#244597,#244598,#244599,
#244600,#244601,#244602,#244603,#244604,#244605,#244606,#244607,#244608,
#244609,#244610,#244611,#244612,#244613,#244614,#244615,#244616,#244617,
#244618,#244619,#244620,#244621,#244622,#244623,#244624,#244625,#244626,
#244627,#244628,#244629,#244630,#244631,#244632,#244633,#244634,#244635,
#244636,#244637,#244638,#244639,#244640,#244641,#244642,#244643,#244644,
#244645,#244646,#244647,#244648,#244649,#244650,#244651,#244652,#244653,
#244654,#244655,#244656,#244657,#244658,#244659,#244660,#244661,#244662,
#244663,#244664,#244665,#244666,#244667,#244668,#244669,#244670,#244671,
#244672,#244673,#244674,#244675,#244676,#244677,#244678,#244679,#244680,
#244681,#244682,#244683,#244684,#244685,#244686,#244687,#244688,#244689,
#244690,#244691,#244692,#244693,#244694,#244695,#244696,#244697,#244698,
#244699,#244700,#244701,#244702,#244703,#244704,#244705,#244706,#244707),
 .UNSPECIFIED.,.F.,.F.)
B_SPLINE_CURVE_WITH_KNOTS((6,1,1,1,1,1,1,1,1,1,1,1,1,1,1,1,1,1,1,1,1,1,
1,1,1,1,1,1,1,1,1,1,1,1,1,1,1,1,1,1,1,1,1,1,1,1,1,1,1,1,1,1,1,1,1,1,1,1,
1,1,1,1,1,1,1,1,1,1,1,1,1,1,1,1,1,1,1,1,1,1,1,1,1,1,1,1,1,1,1,1,1,1,1,1,
1,1,1,1,1,1,1,1,1,1,1,1,1,1,1,1,1,1,1,1,1,1,1,1,1,1,1,1,1,1,1,1,1,1,1,1,
1,1,1,1,1,1,1,1,1,1,1,1,1,1,1,1,1,1,1,1,1,1,1,1,1,1,1,1,1,1,1,1,1,1,1,1,
1,1,1,1,1,1,1,1,1,1,1,1,1,1,1,1,1,1,1,1,1,1,1,1,1,1,1,1,1,1,1,1,1,1,6),
(-1.,-0.995000000000001,-0.990000000000001,-0.985000000000001,-0.980000000000001,
-0.975000000000001,-0.970000000000001,-0.965000000000001,-0.960000000000001,
-0.955000000000001,-0.950000000000001,-0.945000000000001,-0.940000000000001,
-0.935000000000001,-0.930000000000001,-0.925000000000001,-0.920000000000001,
-0.915000000000001,-0.910000000000001,-0.905000000000001,-0.900000000000001,
-0.895000000000001,-0.890000000000001,-0.885000000000001,-0.880000000000001,
-0.875000000000001,-0.870000000000001,-0.865000000000001,-0.860000000000001,
-0.855000000000001,-0.850000000000001,-0.845000000000001,-0.840000000000001,
-0.835000000000001,-0.830000000000001,-0.825000000000001,-0.820000000000001,
-0.815000000000001,-0.810000000000001,-0.805000000000001,-0.800000000000001,
-0.795000000000001,-0.790000000000001,-0.785000000000001,-0.780000000000001,
-0.775000000000001,-0.770000000000001,-0.765000000000001,-0.760000000000001,
-0.755000000000001,-0.750000000000001,-0.745000000000001,-0.740000000000001,
-0.735000000000001,-0.730000000000001,-0.725000000000001,-0.720000000000001,
-0.715000000000001,-0.710000000000001,-0.705000000000001,-0.700000000000001,
-0.695000000000001,-0.690000000000001,-0.685,-0.68,-0.675,-0.67,-0.665,
-0.66,-0.655,-0.65,-0.645,-0.64,-0.635,-0.63,-0.625,-0.62,-0.615,-0.61,
-0.605,-0.6,-0.595,-0.59,-0.585,-0.58,-0.575,-0.57,-0.565,-0.56,-0.555,
-0.55,-0.545,-0.54,-0.535,-0.53,-0.525,-0.52,-0.515,-0.51,-0.505,-0.5,-0.495,
-0.49,-0.485,-0.48,-0.475,-0.47,-0.465,-0.46,-0.455,-0.45,-0.445,-0.44,
-0.435,-0.43,-0.425,-0.42,-0.415,-0.41,-0.405,-0.4,-0.395,-0.39,-0.385,
-0.38,-0.375,-0.37,-0.365,-0.36,-0.355,-0.35,-0.345,-0.34,-0.335,-0.33,
-0.325,-0.32,-0.315,-0.31,-0.305,-0.3,-0.295,-0.29,-0.285,-0.28,-0.275,
-0.27,-0.265,-0.26,-0.255,-0.25,-0.245,-0.24,-0.235,-0.23,-0.225,-0.22,
-0.215,-0.21,-0.205,-0.2,-0.195,-0.19,-0.185,-0.18,-0.175,-0.17,-0.165,
-0.16,-0.155,-0.15,-0.145,-0.14,-0.135,-0.13,-0.125,-0.12,-0.115,-0.11,
-0.105,-0.1,-0.095,-0.09,-0.085,-0.08,-0.075,-0.07,-0.065,-0.06,-0.055,
-0.05,-0.045,-0.04,-0.035,-0.03,-0.025,-0.02,-0.015,-0.01,-0.005,0.),
 .UNSPECIFIED.)
CURVE()
GEOMETRIC_REPRESENTATION_ITEM()
RATIONAL_B_SPLINE_CURVE((1.,1.,1.,1.,1.,1.,1.,1.,1.,1.,1.,1.,1.,1.,1.,1.,
1.,1.,1.,1.,1.,1.,1.,1.,1.,1.,1.,1.,1.,1.,1.,1.,1.,1.,1.,1.,1.,1.,1.,1.,
1.,1.,1.,1.,1.,1.,1.,1.,1.,1.,1.,1.,1.,1.,1.,1.,1.,1.,1.,1.,1.,1.,1.,1.,
1.,1.,1.,1.,1.,1.,1.,1.,1.,1.,1.,1.,1.,1.,1.,1.,1.,1.,1.,1.,1.,1.,1.,1.,
1.,1.,1.,1.,1.,1.,1.,1.,1.,1.,1.,1.,1.,1.,1.,1.,1.,1.,1.,1.,1.,1.,1.,1.,
1.,1.,1.,1.,1.,1.,1.,1.,1.,1.,1.,1.,1.,1.,1.,1.,1.,1.,1.,1.,1.,1.,1.,1.,
1.,1.,1.,1.,1.,1.,1.,1.,1.,1.,1.,1.,1.,1.,1.,1.,1.,1.,1.,1.,1.,1.,1.,1.,
1.,1.,1.,1.,1.,1.,1.,1.,1.,1.,1.,1.,1.,1.,1.,1.,1.,1.,1.,1.,1.,1.,1.,1.,
1.,1.,1.,1.,1.,1.,1.,1.,1.,1.,1.,1.,1.,1.,1.,1.,1.,1.,1.,1.,1.))
REPRESENTATION_ITEM('')
);
#856=(
BOUNDED_CURVE()
B_SPLINE_CURVE(5,(#244710,#244711,#244712,#244713,#244714,#244715,#244716,
#244717,#244718,#244719,#244720,#244721,#244722,#244723,#244724,#244725,
#244726,#244727,#244728,#244729,#244730,#244731,#244732,#244733,#244734,
#244735,#244736,#244737,#244738,#244739,#244740,#244741,#244742,#244743,
#244744,#244745,#244746,#244747,#244748,#244749,#244750,#244751,#244752,
#244753,#244754,#244755,#244756,#244757,#244758,#244759,#244760,#244761,
#244762,#244763,#244764,#244765,#244766,#244767,#244768,#244769,#244770,
#244771,#244772,#244773,#244774,#244775,#244776,#244777,#244778,#244779,
#244780,#244781,#244782,#244783,#244784,#244785,#244786,#244787,#244788,
#244789,#244790,#244791,#244792,#244793,#244794,#244795,#244796,#244797,
#244798,#244799,#244800,#244801,#244802,#244803,#244804,#244805,#244806,
#244807,#244808,#244809,#244810,#244811,#244812,#244813,#244814,#244815,
#244816,#244817,#244818,#244819,#244820,#244821,#244822,#244823,#244824,
#244825,#244826,#244827,#244828,#244829,#244830,#244831,#244832,#244833,
#244834,#244835,#244836,#244837,#244838,#244839,#244840,#244841,#244842,
#244843,#244844,#244845,#244846,#244847,#244848,#244849,#244850,#244851,
#244852,#244853,#244854,#244855,#244856,#244857,#244858,#244859,#244860,
#244861,#244862,#244863,#244864,#244865,#244866,#244867,#244868,#244869,
#244870,#244871,#244872,#244873,#244874,#244875,#244876,#244877,#244878,
#244879,#244880,#244881,#244882,#244883,#244884,#244885,#244886,#244887,
#244888,#244889,#244890,#244891,#244892,#244893,#244894,#244895,#244896,
#244897,#244898,#244899,#244900,#244901,#244902,#244903,#244904,#244905,
#244906,#244907,#244908,#244909,#244910,#244911,#244912,#244913,#244914),
 .UNSPECIFIED.,.F.,.F.)
B_SPLINE_CURVE_WITH_KNOTS((6,1,1,1,1,1,1,1,1,1,1,1,1,1,1,1,1,1,1,1,1,1,
1,1,1,1,1,1,1,1,1,1,1,1,1,1,1,1,1,1,1,1,1,1,1,1,1,1,1,1,1,1,1,1,1,1,1,1,
1,1,1,1,1,1,1,1,1,1,1,1,1,1,1,1,1,1,1,1,1,1,1,1,1,1,1,1,1,1,1,1,1,1,1,1,
1,1,1,1,1,1,1,1,1,1,1,1,1,1,1,1,1,1,1,1,1,1,1,1,1,1,1,1,1,1,1,1,1,1,1,1,
1,1,1,1,1,1,1,1,1,1,1,1,1,1,1,1,1,1,1,1,1,1,1,1,1,1,1,1,1,1,1,1,1,1,1,1,
1,1,1,1,1,1,1,1,1,1,1,1,1,1,1,1,1,1,1,1,1,1,1,1,1,1,1,1,1,1,1,1,1,1,6),
(0.,0.005,0.01,0.015,0.02,0.025,0.03,0.035,0.04,0.045,0.05,0.055,0.06,0.065,
0.07,0.075,0.08,0.085,0.09,0.095,0.1,0.105,0.11,0.115,0.12,0.125,0.13,0.135,
0.14,0.145,0.15,0.155,0.16,0.165,0.17,0.175,0.18,0.185,0.19,0.195,0.2,0.205,
0.21,0.215,0.22,0.225,0.23,0.235,0.24,0.245,0.25,0.255,0.26,0.265,0.27,
0.275,0.28,0.285,0.29,0.295,0.3,0.305,0.31,0.315,0.32,0.325,0.33,0.335,
0.34,0.345,0.35,0.355,0.36,0.365,0.37,0.375,0.38,0.385,0.39,0.395,0.4,0.405,
0.41,0.415,0.42,0.425,0.43,0.435,0.44,0.445,0.45,0.455,0.46,0.465,0.47,
0.475,0.48,0.485,0.49,0.495,0.5,0.505,0.51,0.515,0.52,0.525,0.53,0.535,
0.54,0.545,0.55,0.555,0.56,0.565,0.57,0.575,0.58,0.585,0.59,0.595,0.6,0.605,
0.61,0.615,0.62,0.625,0.63,0.635,0.64,0.645,0.65,0.655,0.66,0.665,0.67,
0.675,0.68,0.685,0.690000000000001,0.695000000000001,0.700000000000001,
0.705000000000001,0.710000000000001,0.715000000000001,0.720000000000001,
0.725000000000001,0.730000000000001,0.735000000000001,0.740000000000001,
0.745000000000001,0.750000000000001,0.755000000000001,0.760000000000001,
0.765000000000001,0.770000000000001,0.775000000000001,0.780000000000001,
0.785000000000001,0.790000000000001,0.795000000000001,0.800000000000001,
0.805000000000001,0.810000000000001,0.815000000000001,0.820000000000001,
0.825000000000001,0.830000000000001,0.835000000000001,0.840000000000001,
0.845000000000001,0.850000000000001,0.855000000000001,0.860000000000001,
0.865000000000001,0.870000000000001,0.875000000000001,0.880000000000001,
0.885000000000001,0.890000000000001,0.895000000000001,0.900000000000001,
0.905000000000001,0.910000000000001,0.915000000000001,0.920000000000001,
0.925000000000001,0.930000000000001,0.935000000000001,0.940000000000001,
0.945000000000001,0.950000000000001,0.955000000000001,0.960000000000001,
0.965000000000001,0.970000000000001,0.975000000000001,0.980000000000001,
0.985000000000001,0.990000000000001,0.995000000000001,1.),.UNSPECIFIED.)
CURVE()
GEOMETRIC_REPRESENTATION_ITEM()
RATIONAL_B_SPLINE_CURVE((1.,1.,1.,1.,1.,1.,1.,1.,1.,1.,1.,1.,1.,1.,1.,1.,
1.,1.,1.,1.,1.,1.,1.,1.,1.,1.,1.,1.,1.,1.,1.,1.,1.,1.,1.,1.,1.,1.,1.,1.,
1.,1.,1.,1.,1.,1.,1.,1.,1.,1.,1.,1.,1.,1.,1.,1.,1.,1.,1.,1.,1.,1.,1.,1.,
1.,1.,1.,1.,1.,1.,1.,1.,1.,1.,1.,1.,1.,1.,1.,1.,1.,1.,1.,1.,1.,1.,1.,1.,
1.,1.,1.,1.,1.,1.,1.,1.,1.,1.,1.,1.,1.,1.,1.,1.,1.,1.,1.,1.,1.,1.,1.,1.,
1.,1.,1.,1.,1.,1.,1.,1.,1.,1.,1.,1.,1.,1.,1.,1.,1.,1.,1.,1.,1.,1.,1.,1.,
1.,1.,1.,1.,1.,1.,1.,1.,1.,1.,1.,1.,1.,1.,1.,1.,1.,1.,1.,1.,1.,1.,1.,1.,
1.,1.,1.,1.,1.,1.,1.,1.,1.,1.,1.,1.,1.,1.,1.,1.,1.,1.,1.,1.,1.,1.,1.,1.,
1.,1.,1.,1.,1.,1.,1.,1.,1.,1.,1.,1.,1.,1.,1.,1.,1.,1.,1.,1.,1.))
REPRESENTATION_ITEM('')
);
#857=(
BOUNDED_CURVE()
B_SPLINE_CURVE(5,(#245326,#245327,#245328,#245329,#245330,#245331,#245332,
#245333,#245334,#245335,#245336,#245337,#245338,#245339,#245340,#245341,
#245342,#245343,#245344,#245345,#245346,#245347,#245348,#245349,#245350,
#245351,#245352,#245353,#245354,#245355,#245356,#245357,#245358,#245359,
#245360,#245361,#245362,#245363,#245364,#245365,#245366,#245367,#245368,
#245369,#245370,#245371,#245372,#245373,#245374,#245375,#245376,#245377,
#245378,#245379,#245380,#245381,#245382,#245383,#245384,#245385,#245386,
#245387,#245388,#245389,#245390,#245391,#245392,#245393,#245394,#245395,
#245396,#245397,#245398,#245399,#245400,#245401,#245402,#245403,#245404,
#245405,#245406,#245407,#245408,#245409,#245410,#245411,#245412,#245413,
#245414,#245415,#245416,#245417,#245418,#245419,#245420,#245421,#245422,
#245423,#245424,#245425,#245426,#245427,#245428,#245429,#245430,#245431,
#245432,#245433,#245434,#245435,#245436,#245437,#245438,#245439,#245440,
#245441,#245442,#245443,#245444,#245445,#245446,#245447,#245448,#245449,
#245450,#245451,#245452,#245453,#245454,#245455,#245456,#245457,#245458,
#245459,#245460,#245461,#245462,#245463,#245464,#245465,#245466,#245467,
#245468,#245469,#245470,#245471,#245472,#245473,#245474,#245475,#245476,
#245477,#245478,#245479,#245480,#245481,#245482,#245483,#245484,#245485,
#245486,#245487,#245488,#245489,#245490,#245491,#245492,#245493,#245494,
#245495,#245496,#245497,#245498,#245499,#245500,#245501,#245502,#245503,
#245504,#245505,#245506,#245507,#245508,#245509,#245510,#245511,#245512,
#245513,#245514,#245515,#245516,#245517,#245518,#245519,#245520,#245521,
#245522,#245523,#245524,#245525,#245526,#245527,#245528,#245529,#245530),
 .UNSPECIFIED.,.F.,.F.)
B_SPLINE_CURVE_WITH_KNOTS((6,1,1,1,1,1,1,1,1,1,1,1,1,1,1,1,1,1,1,1,1,1,
1,1,1,1,1,1,1,1,1,1,1,1,1,1,1,1,1,1,1,1,1,1,1,1,1,1,1,1,1,1,1,1,1,1,1,1,
1,1,1,1,1,1,1,1,1,1,1,1,1,1,1,1,1,1,1,1,1,1,1,1,1,1,1,1,1,1,1,1,1,1,1,1,
1,1,1,1,1,1,1,1,1,1,1,1,1,1,1,1,1,1,1,1,1,1,1,1,1,1,1,1,1,1,1,1,1,1,1,1,
1,1,1,1,1,1,1,1,1,1,1,1,1,1,1,1,1,1,1,1,1,1,1,1,1,1,1,1,1,1,1,1,1,1,1,1,
1,1,1,1,1,1,1,1,1,1,1,1,1,1,1,1,1,1,1,1,1,1,1,1,1,1,1,1,1,1,1,1,1,1,6),
(0.,0.005,0.01,0.015,0.02,0.025,0.03,0.035,0.04,0.045,0.05,0.055,0.06,0.065,
0.07,0.075,0.08,0.085,0.09,0.095,0.1,0.105,0.11,0.115,0.12,0.125,0.13,0.135,
0.14,0.145,0.15,0.155,0.16,0.165,0.17,0.175,0.18,0.185,0.19,0.195,0.2,0.205,
0.21,0.215,0.22,0.225,0.23,0.235,0.24,0.245,0.25,0.255,0.26,0.265,0.27,
0.275,0.28,0.285,0.29,0.295,0.3,0.305,0.31,0.315,0.32,0.325,0.33,0.335,
0.34,0.345,0.35,0.355,0.36,0.365,0.37,0.375,0.38,0.385,0.39,0.395,0.4,0.405,
0.41,0.415,0.42,0.425,0.43,0.435,0.44,0.445,0.45,0.455,0.46,0.465,0.47,
0.475,0.48,0.485,0.49,0.495,0.5,0.505,0.51,0.515,0.52,0.525,0.53,0.535,
0.54,0.545,0.55,0.555,0.56,0.565,0.57,0.575,0.58,0.585,0.59,0.595,0.6,0.605,
0.61,0.615,0.62,0.625,0.63,0.635,0.64,0.645,0.65,0.655,0.66,0.665,0.67,
0.675,0.68,0.685,0.690000000000001,0.695000000000001,0.700000000000001,
0.705000000000001,0.710000000000001,0.715000000000001,0.720000000000001,
0.725000000000001,0.730000000000001,0.735000000000001,0.740000000000001,
0.745000000000001,0.750000000000001,0.755000000000001,0.760000000000001,
0.765000000000001,0.770000000000001,0.775000000000001,0.780000000000001,
0.785000000000001,0.790000000000001,0.795000000000001,0.800000000000001,
0.805000000000001,0.810000000000001,0.815000000000001,0.820000000000001,
0.825000000000001,0.830000000000001,0.835000000000001,0.840000000000001,
0.845000000000001,0.850000000000001,0.855000000000001,0.860000000000001,
0.865000000000001,0.870000000000001,0.875000000000001,0.880000000000001,
0.885000000000001,0.890000000000001,0.895000000000001,0.900000000000001,
0.905000000000001,0.910000000000001,0.915000000000001,0.920000000000001,
0.925000000000001,0.930000000000001,0.935000000000001,0.940000000000001,
0.945000000000001,0.950000000000001,0.955000000000001,0.960000000000001,
0.965000000000001,0.970000000000001,0.975000000000001,0.980000000000001,
0.985000000000001,0.990000000000001,0.995000000000001,1.),.UNSPECIFIED.)
CURVE()
GEOMETRIC_REPRESENTATION_ITEM()
RATIONAL_B_SPLINE_CURVE((1.,1.,1.,1.,1.,1.,1.,1.,1.,1.,1.,1.,1.,1.,1.,1.,
1.,1.,1.,1.,1.,1.,1.,1.,1.,1.,1.,1.,1.,1.,1.,1.,1.,1.,1.,1.,1.,1.,1.,1.,
1.,1.,1.,1.,1.,1.,1.,1.,1.,1.,1.,1.,1.,1.,1.,1.,1.,1.,1.,1.,1.,1.,1.,1.,
1.,1.,1.,1.,1.,1.,1.,1.,1.,1.,1.,1.,1.,1.,1.,1.,1.,1.,1.,1.,1.,1.,1.,1.,
1.,1.,1.,1.,1.,1.,1.,1.,1.,1.,1.,1.,1.,1.,1.,1.,1.,1.,1.,1.,1.,1.,1.,1.,
1.,1.,1.,1.,1.,1.,1.,1.,1.,1.,1.,1.,1.,1.,1.,1.,1.,1.,1.,1.,1.,1.,1.,1.,
1.,1.,1.,1.,1.,1.,1.,1.,1.,1.,1.,1.,1.,1.,1.,1.,1.,1.,1.,1.,1.,1.,1.,1.,
1.,1.,1.,1.,1.,1.,1.,1.,1.,1.,1.,1.,1.,1.,1.,1.,1.,1.,1.,1.,1.,1.,1.,1.,
1.,1.,1.,1.,1.,1.,1.,1.,1.,1.,1.,1.,1.,1.,1.,1.,1.,1.,1.,1.,1.))
REPRESENTATION_ITEM('')
);
#858=(
BOUNDED_CURVE()
B_SPLINE_CURVE(5,(#245532,#245533,#245534,#245535,#245536,#245537,#245538,
#245539,#245540,#245541,#245542,#245543,#245544,#245545,#245546,#245547,
#245548,#245549,#245550,#245551,#245552,#245553,#245554,#245555,#245556,
#245557,#245558,#245559,#245560,#245561,#245562,#245563,#245564,#245565,
#245566,#245567,#245568,#245569,#245570,#245571,#245572,#245573,#245574,
#245575,#245576,#245577,#245578,#245579,#245580,#245581,#245582,#245583,
#245584,#245585,#245586,#245587,#245588,#245589,#245590,#245591,#245592,
#245593,#245594,#245595,#245596,#245597,#245598,#245599,#245600,#245601,
#245602,#245603,#245604,#245605,#245606,#245607,#245608,#245609,#245610,
#245611,#245612,#245613,#245614,#245615,#245616,#245617,#245618,#245619,
#245620,#245621,#245622,#245623,#245624,#245625,#245626,#245627,#245628,
#245629,#245630,#245631,#245632,#245633,#245634,#245635,#245636,#245637,
#245638,#245639,#245640,#245641,#245642,#245643,#245644,#245645,#245646,
#245647,#245648,#245649,#245650,#245651,#245652,#245653,#245654,#245655,
#245656,#245657,#245658,#245659,#245660,#245661,#245662,#245663,#245664,
#245665,#245666,#245667,#245668,#245669,#245670,#245671,#245672,#245673,
#245674,#245675,#245676,#245677,#245678,#245679,#245680,#245681,#245682,
#245683,#245684,#245685,#245686,#245687,#245688,#245689,#245690,#245691,
#245692,#245693,#245694,#245695,#245696,#245697,#245698,#245699,#245700,
#245701,#245702,#245703,#245704,#245705,#245706,#245707,#245708,#245709,
#245710,#245711,#245712,#245713,#245714,#245715,#245716,#245717,#245718,
#245719,#245720,#245721,#245722,#245723,#245724,#245725,#245726,#245727,
#245728,#245729,#245730,#245731,#245732,#245733,#245734,#245735,#245736),
 .UNSPECIFIED.,.F.,.F.)
B_SPLINE_CURVE_WITH_KNOTS((6,1,1,1,1,1,1,1,1,1,1,1,1,1,1,1,1,1,1,1,1,1,
1,1,1,1,1,1,1,1,1,1,1,1,1,1,1,1,1,1,1,1,1,1,1,1,1,1,1,1,1,1,1,1,1,1,1,1,
1,1,1,1,1,1,1,1,1,1,1,1,1,1,1,1,1,1,1,1,1,1,1,1,1,1,1,1,1,1,1,1,1,1,1,1,
1,1,1,1,1,1,1,1,1,1,1,1,1,1,1,1,1,1,1,1,1,1,1,1,1,1,1,1,1,1,1,1,1,1,1,1,
1,1,1,1,1,1,1,1,1,1,1,1,1,1,1,1,1,1,1,1,1,1,1,1,1,1,1,1,1,1,1,1,1,1,1,1,
1,1,1,1,1,1,1,1,1,1,1,1,1,1,1,1,1,1,1,1,1,1,1,1,1,1,1,1,1,1,1,1,1,1,6),
(-1.,-0.995000000000001,-0.990000000000001,-0.985000000000001,-0.980000000000001,
-0.975000000000001,-0.970000000000001,-0.965000000000001,-0.960000000000001,
-0.955000000000001,-0.950000000000001,-0.945000000000001,-0.940000000000001,
-0.935000000000001,-0.930000000000001,-0.925000000000001,-0.920000000000001,
-0.915000000000001,-0.910000000000001,-0.905000000000001,-0.900000000000001,
-0.895000000000001,-0.890000000000001,-0.885000000000001,-0.880000000000001,
-0.875000000000001,-0.870000000000001,-0.865000000000001,-0.860000000000001,
-0.855000000000001,-0.850000000000001,-0.845000000000001,-0.840000000000001,
-0.835000000000001,-0.830000000000001,-0.825000000000001,-0.820000000000001,
-0.815000000000001,-0.810000000000001,-0.805000000000001,-0.800000000000001,
-0.795000000000001,-0.790000000000001,-0.785000000000001,-0.780000000000001,
-0.775000000000001,-0.770000000000001,-0.765000000000001,-0.760000000000001,
-0.755000000000001,-0.750000000000001,-0.745000000000001,-0.740000000000001,
-0.735000000000001,-0.730000000000001,-0.725000000000001,-0.720000000000001,
-0.715000000000001,-0.710000000000001,-0.705000000000001,-0.700000000000001,
-0.695000000000001,-0.690000000000001,-0.685,-0.68,-0.675,-0.67,-0.665,
-0.66,-0.655,-0.65,-0.645,-0.64,-0.635,-0.63,-0.625,-0.62,-0.615,-0.61,
-0.605,-0.6,-0.595,-0.59,-0.585,-0.58,-0.575,-0.57,-0.565,-0.56,-0.555,
-0.55,-0.545,-0.54,-0.535,-0.53,-0.525,-0.52,-0.515,-0.51,-0.505,-0.5,-0.495,
-0.49,-0.485,-0.48,-0.475,-0.47,-0.465,-0.46,-0.455,-0.45,-0.445,-0.44,
-0.435,-0.43,-0.425,-0.42,-0.415,-0.41,-0.405,-0.4,-0.395,-0.39,-0.385,
-0.38,-0.375,-0.37,-0.365,-0.36,-0.355,-0.35,-0.345,-0.34,-0.335,-0.33,
-0.325,-0.32,-0.315,-0.31,-0.305,-0.3,-0.295,-0.29,-0.285,-0.28,-0.275,
-0.27,-0.265,-0.26,-0.255,-0.25,-0.245,-0.24,-0.235,-0.23,-0.225,-0.22,
-0.215,-0.21,-0.205,-0.2,-0.195,-0.19,-0.185,-0.18,-0.175,-0.17,-0.165,
-0.16,-0.155,-0.15,-0.145,-0.14,-0.135,-0.13,-0.125,-0.12,-0.115,-0.11,
-0.105,-0.1,-0.095,-0.09,-0.085,-0.08,-0.075,-0.07,-0.065,-0.06,-0.055,
-0.05,-0.045,-0.04,-0.035,-0.03,-0.025,-0.02,-0.015,-0.01,-0.005,0.),
 .UNSPECIFIED.)
CURVE()
GEOMETRIC_REPRESENTATION_ITEM()
RATIONAL_B_SPLINE_CURVE((1.,1.,1.,1.,1.,1.,1.,1.,1.,1.,1.,1.,1.,1.,1.,1.,
1.,1.,1.,1.,1.,1.,1.,1.,1.,1.,1.,1.,1.,1.,1.,1.,1.,1.,1.,1.,1.,1.,1.,1.,
1.,1.,1.,1.,1.,1.,1.,1.,1.,1.,1.,1.,1.,1.,1.,1.,1.,1.,1.,1.,1.,1.,1.,1.,
1.,1.,1.,1.,1.,1.,1.,1.,1.,1.,1.,1.,1.,1.,1.,1.,1.,1.,1.,1.,1.,1.,1.,1.,
1.,1.,1.,1.,1.,1.,1.,1.,1.,1.,1.,1.,1.,1.,1.,1.,1.,1.,1.,1.,1.,1.,1.,1.,
1.,1.,1.,1.,1.,1.,1.,1.,1.,1.,1.,1.,1.,1.,1.,1.,1.,1.,1.,1.,1.,1.,1.,1.,
1.,1.,1.,1.,1.,1.,1.,1.,1.,1.,1.,1.,1.,1.,1.,1.,1.,1.,1.,1.,1.,1.,1.,1.,
1.,1.,1.,1.,1.,1.,1.,1.,1.,1.,1.,1.,1.,1.,1.,1.,1.,1.,1.,1.,1.,1.,1.,1.,
1.,1.,1.,1.,1.,1.,1.,1.,1.,1.,1.,1.,1.,1.,1.,1.,1.,1.,1.,1.,1.))
REPRESENTATION_ITEM('')
);
#859=(
BOUNDED_CURVE()
B_SPLINE_CURVE(5,(#246155,#246156,#246157,#246158,#246159,#246160,#246161,
#246162,#246163,#246164,#246165,#246166,#246167,#246168,#246169,#246170,
#246171,#246172,#246173,#246174,#246175,#246176,#246177,#246178,#246179,
#246180,#246181,#246182,#246183,#246184,#246185,#246186,#246187,#246188,
#246189,#246190,#246191,#246192,#246193,#246194,#246195,#246196,#246197,
#246198,#246199,#246200,#246201,#246202,#246203,#246204,#246205,#246206,
#246207,#246208,#246209,#246210,#246211,#246212,#246213,#246214,#246215,
#246216,#246217,#246218,#246219,#246220,#246221,#246222,#246223,#246224,
#246225,#246226,#246227,#246228,#246229,#246230,#246231,#246232,#246233,
#246234,#246235,#246236,#246237,#246238,#246239,#246240,#246241,#246242,
#246243,#246244,#246245,#246246,#246247,#246248,#246249,#246250,#246251,
#246252,#246253,#246254,#246255,#246256,#246257,#246258,#246259,#246260,
#246261,#246262,#246263,#246264,#246265,#246266,#246267,#246268,#246269,
#246270,#246271,#246272,#246273,#246274,#246275,#246276,#246277,#246278,
#246279,#246280,#246281,#246282,#246283,#246284,#246285,#246286,#246287,
#246288,#246289,#246290,#246291,#246292,#246293,#246294,#246295,#246296,
#246297,#246298,#246299,#246300,#246301,#246302,#246303,#246304,#246305,
#246306,#246307,#246308,#246309,#246310,#246311,#246312,#246313,#246314,
#246315,#246316,#246317,#246318,#246319,#246320,#246321,#246322,#246323,
#246324,#246325,#246326,#246327,#246328,#246329,#246330,#246331,#246332,
#246333,#246334,#246335,#246336,#246337,#246338,#246339,#246340,#246341,
#246342,#246343,#246344,#246345,#246346,#246347,#246348,#246349,#246350,
#246351,#246352,#246353,#246354,#246355,#246356,#246357,#246358,#246359),
 .UNSPECIFIED.,.F.,.F.)
B_SPLINE_CURVE_WITH_KNOTS((6,1,1,1,1,1,1,1,1,1,1,1,1,1,1,1,1,1,1,1,1,1,
1,1,1,1,1,1,1,1,1,1,1,1,1,1,1,1,1,1,1,1,1,1,1,1,1,1,1,1,1,1,1,1,1,1,1,1,
1,1,1,1,1,1,1,1,1,1,1,1,1,1,1,1,1,1,1,1,1,1,1,1,1,1,1,1,1,1,1,1,1,1,1,1,
1,1,1,1,1,1,1,1,1,1,1,1,1,1,1,1,1,1,1,1,1,1,1,1,1,1,1,1,1,1,1,1,1,1,1,1,
1,1,1,1,1,1,1,1,1,1,1,1,1,1,1,1,1,1,1,1,1,1,1,1,1,1,1,1,1,1,1,1,1,1,1,1,
1,1,1,1,1,1,1,1,1,1,1,1,1,1,1,1,1,1,1,1,1,1,1,1,1,1,1,1,1,1,1,1,1,1,6),
(-1.,-0.995000000000001,-0.990000000000001,-0.985000000000001,-0.980000000000001,
-0.975000000000001,-0.970000000000001,-0.965000000000001,-0.960000000000001,
-0.955000000000001,-0.950000000000001,-0.945000000000001,-0.940000000000001,
-0.935000000000001,-0.930000000000001,-0.925000000000001,-0.920000000000001,
-0.915000000000001,-0.910000000000001,-0.905000000000001,-0.900000000000001,
-0.895000000000001,-0.890000000000001,-0.885000000000001,-0.880000000000001,
-0.875000000000001,-0.870000000000001,-0.865000000000001,-0.860000000000001,
-0.855000000000001,-0.850000000000001,-0.845000000000001,-0.840000000000001,
-0.835000000000001,-0.830000000000001,-0.825000000000001,-0.820000000000001,
-0.815000000000001,-0.810000000000001,-0.805000000000001,-0.800000000000001,
-0.795000000000001,-0.790000000000001,-0.785000000000001,-0.780000000000001,
-0.775000000000001,-0.770000000000001,-0.765000000000001,-0.760000000000001,
-0.755000000000001,-0.750000000000001,-0.745000000000001,-0.740000000000001,
-0.735000000000001,-0.730000000000001,-0.725000000000001,-0.720000000000001,
-0.715000000000001,-0.710000000000001,-0.705000000000001,-0.700000000000001,
-0.695000000000001,-0.690000000000001,-0.685,-0.68,-0.675,-0.67,-0.665,
-0.66,-0.655,-0.65,-0.645,-0.64,-0.635,-0.63,-0.625,-0.62,-0.615,-0.61,
-0.605,-0.6,-0.595,-0.59,-0.585,-0.58,-0.575,-0.57,-0.565,-0.56,-0.555,
-0.55,-0.545,-0.54,-0.535,-0.53,-0.525,-0.52,-0.515,-0.51,-0.505,-0.5,-0.495,
-0.49,-0.485,-0.48,-0.475,-0.47,-0.465,-0.46,-0.455,-0.45,-0.445,-0.44,
-0.435,-0.43,-0.425,-0.42,-0.415,-0.41,-0.405,-0.4,-0.395,-0.39,-0.385,
-0.38,-0.375,-0.37,-0.365,-0.36,-0.355,-0.35,-0.345,-0.34,-0.335,-0.33,
-0.325,-0.32,-0.315,-0.31,-0.305,-0.3,-0.295,-0.29,-0.285,-0.28,-0.275,
-0.27,-0.265,-0.26,-0.255,-0.25,-0.245,-0.24,-0.235,-0.23,-0.225,-0.22,
-0.215,-0.21,-0.205,-0.2,-0.195,-0.19,-0.185,-0.18,-0.175,-0.17,-0.165,
-0.16,-0.155,-0.15,-0.145,-0.14,-0.135,-0.13,-0.125,-0.12,-0.115,-0.11,
-0.105,-0.1,-0.095,-0.09,-0.085,-0.08,-0.075,-0.07,-0.065,-0.06,-0.055,
-0.05,-0.045,-0.04,-0.035,-0.03,-0.025,-0.02,-0.015,-0.01,-0.005,0.),
 .UNSPECIFIED.)
CURVE()
GEOMETRIC_REPRESENTATION_ITEM()
RATIONAL_B_SPLINE_CURVE((1.,1.,1.,1.,1.,1.,1.,1.,1.,1.,1.,1.,1.,1.,1.,1.,
1.,1.,1.,1.,1.,1.,1.,1.,1.,1.,1.,1.,1.,1.,1.,1.,1.,1.,1.,1.,1.,1.,1.,1.,
1.,1.,1.,1.,1.,1.,1.,1.,1.,1.,1.,1.,1.,1.,1.,1.,1.,1.,1.,1.,1.,1.,1.,1.,
1.,1.,1.,1.,1.,1.,1.,1.,1.,1.,1.,1.,1.,1.,1.,1.,1.,1.,1.,1.,1.,1.,1.,1.,
1.,1.,1.,1.,1.,1.,1.,1.,1.,1.,1.,1.,1.,1.,1.,1.,1.,1.,1.,1.,1.,1.,1.,1.,
1.,1.,1.,1.,1.,1.,1.,1.,1.,1.,1.,1.,1.,1.,1.,1.,1.,1.,1.,1.,1.,1.,1.,1.,
1.,1.,1.,1.,1.,1.,1.,1.,1.,1.,1.,1.,1.,1.,1.,1.,1.,1.,1.,1.,1.,1.,1.,1.,
1.,1.,1.,1.,1.,1.,1.,1.,1.,1.,1.,1.,1.,1.,1.,1.,1.,1.,1.,1.,1.,1.,1.,1.,
1.,1.,1.,1.,1.,1.,1.,1.,1.,1.,1.,1.,1.,1.,1.,1.,1.,1.,1.,1.,1.))
REPRESENTATION_ITEM('')
);
#860=(
BOUNDED_CURVE()
B_SPLINE_CURVE(5,(#246362,#246363,#246364,#246365,#246366,#246367,#246368,
#246369,#246370,#246371,#246372,#246373,#246374,#246375,#246376,#246377,
#246378,#246379,#246380,#246381,#246382,#246383,#246384,#246385,#246386,
#246387,#246388,#246389,#246390,#246391,#246392,#246393,#246394,#246395,
#246396,#246397,#246398,#246399,#246400,#246401,#246402,#246403,#246404,
#246405,#246406,#246407,#246408,#246409,#246410,#246411,#246412,#246413,
#246414,#246415,#246416,#246417,#246418,#246419,#246420,#246421,#246422,
#246423,#246424,#246425,#246426,#246427,#246428,#246429,#246430,#246431,
#246432,#246433,#246434,#246435,#246436,#246437,#246438,#246439,#246440,
#246441,#246442,#246443,#246444,#246445,#246446,#246447,#246448,#246449,
#246450,#246451,#246452,#246453,#246454,#246455,#246456,#246457,#246458,
#246459,#246460,#246461,#246462,#246463,#246464,#246465,#246466,#246467,
#246468,#246469,#246470,#246471,#246472,#246473,#246474,#246475,#246476,
#246477,#246478,#246479,#246480,#246481,#246482,#246483,#246484,#246485,
#246486,#246487,#246488,#246489,#246490,#246491,#246492,#246493,#246494,
#246495,#246496,#246497,#246498,#246499,#246500,#246501,#246502,#246503,
#246504,#246505,#246506,#246507,#246508,#246509,#246510,#246511,#246512,
#246513,#246514,#246515,#246516,#246517,#246518,#246519,#246520,#246521,
#246522,#246523,#246524,#246525,#246526,#246527,#246528,#246529,#246530,
#246531,#246532,#246533,#246534,#246535,#246536,#246537,#246538,#246539,
#246540,#246541,#246542,#246543,#246544,#246545,#246546,#246547,#246548,
#246549,#246550,#246551,#246552,#246553,#246554,#246555,#246556,#246557,
#246558,#246559,#246560,#246561,#246562,#246563,#246564,#246565,#246566),
 .UNSPECIFIED.,.F.,.F.)
B_SPLINE_CURVE_WITH_KNOTS((6,1,1,1,1,1,1,1,1,1,1,1,1,1,1,1,1,1,1,1,1,1,
1,1,1,1,1,1,1,1,1,1,1,1,1,1,1,1,1,1,1,1,1,1,1,1,1,1,1,1,1,1,1,1,1,1,1,1,
1,1,1,1,1,1,1,1,1,1,1,1,1,1,1,1,1,1,1,1,1,1,1,1,1,1,1,1,1,1,1,1,1,1,1,1,
1,1,1,1,1,1,1,1,1,1,1,1,1,1,1,1,1,1,1,1,1,1,1,1,1,1,1,1,1,1,1,1,1,1,1,1,
1,1,1,1,1,1,1,1,1,1,1,1,1,1,1,1,1,1,1,1,1,1,1,1,1,1,1,1,1,1,1,1,1,1,1,1,
1,1,1,1,1,1,1,1,1,1,1,1,1,1,1,1,1,1,1,1,1,1,1,1,1,1,1,1,1,1,1,1,1,1,6),
(0.,0.005,0.01,0.015,0.02,0.025,0.03,0.035,0.04,0.045,0.05,0.055,0.06,0.065,
0.07,0.075,0.08,0.085,0.09,0.095,0.1,0.105,0.11,0.115,0.12,0.125,0.13,0.135,
0.14,0.145,0.15,0.155,0.16,0.165,0.17,0.175,0.18,0.185,0.19,0.195,0.2,0.205,
0.21,0.215,0.22,0.225,0.23,0.235,0.24,0.245,0.25,0.255,0.26,0.265,0.27,
0.275,0.28,0.285,0.29,0.295,0.3,0.305,0.31,0.315,0.32,0.325,0.33,0.335,
0.34,0.345,0.35,0.355,0.36,0.365,0.37,0.375,0.38,0.385,0.39,0.395,0.4,0.405,
0.41,0.415,0.42,0.425,0.43,0.435,0.44,0.445,0.45,0.455,0.46,0.465,0.47,
0.475,0.48,0.485,0.49,0.495,0.5,0.505,0.51,0.515,0.52,0.525,0.53,0.535,
0.54,0.545,0.55,0.555,0.56,0.565,0.57,0.575,0.58,0.585,0.59,0.595,0.6,0.605,
0.61,0.615,0.62,0.625,0.63,0.635,0.64,0.645,0.65,0.655,0.66,0.665,0.67,
0.675,0.68,0.685,0.690000000000001,0.695000000000001,0.700000000000001,
0.705000000000001,0.710000000000001,0.715000000000001,0.720000000000001,
0.725000000000001,0.730000000000001,0.735000000000001,0.740000000000001,
0.745000000000001,0.750000000000001,0.755000000000001,0.760000000000001,
0.765000000000001,0.770000000000001,0.775000000000001,0.780000000000001,
0.785000000000001,0.790000000000001,0.795000000000001,0.800000000000001,
0.805000000000001,0.810000000000001,0.815000000000001,0.820000000000001,
0.825000000000001,0.830000000000001,0.835000000000001,0.840000000000001,
0.845000000000001,0.850000000000001,0.855000000000001,0.860000000000001,
0.865000000000001,0.870000000000001,0.875000000000001,0.880000000000001,
0.885000000000001,0.890000000000001,0.895000000000001,0.900000000000001,
0.905000000000001,0.910000000000001,0.915000000000001,0.920000000000001,
0.925000000000001,0.930000000000001,0.935000000000001,0.940000000000001,
0.945000000000001,0.950000000000001,0.955000000000001,0.960000000000001,
0.965000000000001,0.970000000000001,0.975000000000001,0.980000000000001,
0.985000000000001,0.990000000000001,0.995000000000001,1.),.UNSPECIFIED.)
CURVE()
GEOMETRIC_REPRESENTATION_ITEM()
RATIONAL_B_SPLINE_CURVE((1.,1.,1.,1.,1.,1.,1.,1.,1.,1.,1.,1.,1.,1.,1.,1.,
1.,1.,1.,1.,1.,1.,1.,1.,1.,1.,1.,1.,1.,1.,1.,1.,1.,1.,1.,1.,1.,1.,1.,1.,
1.,1.,1.,1.,1.,1.,1.,1.,1.,1.,1.,1.,1.,1.,1.,1.,1.,1.,1.,1.,1.,1.,1.,1.,
1.,1.,1.,1.,1.,1.,1.,1.,1.,1.,1.,1.,1.,1.,1.,1.,1.,1.,1.,1.,1.,1.,1.,1.,
1.,1.,1.,1.,1.,1.,1.,1.,1.,1.,1.,1.,1.,1.,1.,1.,1.,1.,1.,1.,1.,1.,1.,1.,
1.,1.,1.,1.,1.,1.,1.,1.,1.,1.,1.,1.,1.,1.,1.,1.,1.,1.,1.,1.,1.,1.,1.,1.,
1.,1.,1.,1.,1.,1.,1.,1.,1.,1.,1.,1.,1.,1.,1.,1.,1.,1.,1.,1.,1.,1.,1.,1.,
1.,1.,1.,1.,1.,1.,1.,1.,1.,1.,1.,1.,1.,1.,1.,1.,1.,1.,1.,1.,1.,1.,1.,1.,
1.,1.,1.,1.,1.,1.,1.,1.,1.,1.,1.,1.,1.,1.,1.,1.,1.,1.,1.,1.,1.))
REPRESENTATION_ITEM('')
);
#861=(
BOUNDED_CURVE()
B_SPLINE_CURVE(5,(#246978,#246979,#246980,#246981,#246982,#246983,#246984,
#246985,#246986,#246987,#246988,#246989,#246990,#246991,#246992,#246993,
#246994,#246995,#246996,#246997,#246998,#246999,#247000,#247001,#247002,
#247003,#247004,#247005,#247006,#247007,#247008,#247009,#247010,#247011,
#247012,#247013,#247014,#247015,#247016,#247017,#247018,#247019,#247020,
#247021,#247022,#247023,#247024,#247025,#247026,#247027,#247028,#247029,
#247030,#247031,#247032,#247033,#247034,#247035,#247036,#247037,#247038,
#247039,#247040,#247041,#247042,#247043,#247044,#247045,#247046,#247047,
#247048,#247049,#247050,#247051,#247052,#247053,#247054,#247055,#247056,
#247057,#247058,#247059,#247060,#247061,#247062,#247063,#247064,#247065,
#247066,#247067,#247068,#247069,#247070,#247071,#247072,#247073,#247074,
#247075,#247076,#247077,#247078,#247079,#247080,#247081,#247082,#247083,
#247084,#247085,#247086,#247087,#247088,#247089,#247090,#247091,#247092,
#247093,#247094,#247095,#247096,#247097,#247098,#247099,#247100,#247101,
#247102,#247103,#247104,#247105,#247106,#247107,#247108,#247109,#247110,
#247111,#247112,#247113,#247114,#247115,#247116,#247117,#247118,#247119,
#247120,#247121,#247122,#247123,#247124,#247125,#247126,#247127,#247128,
#247129,#247130,#247131,#247132,#247133,#247134,#247135,#247136,#247137,
#247138,#247139,#247140,#247141,#247142,#247143,#247144,#247145,#247146,
#247147,#247148,#247149,#247150,#247151,#247152,#247153,#247154,#247155,
#247156,#247157,#247158,#247159,#247160,#247161,#247162,#247163,#247164,
#247165,#247166,#247167,#247168,#247169,#247170,#247171,#247172,#247173,
#247174,#247175,#247176,#247177,#247178,#247179,#247180,#247181,#247182),
 .UNSPECIFIED.,.F.,.F.)
B_SPLINE_CURVE_WITH_KNOTS((6,1,1,1,1,1,1,1,1,1,1,1,1,1,1,1,1,1,1,1,1,1,
1,1,1,1,1,1,1,1,1,1,1,1,1,1,1,1,1,1,1,1,1,1,1,1,1,1,1,1,1,1,1,1,1,1,1,1,
1,1,1,1,1,1,1,1,1,1,1,1,1,1,1,1,1,1,1,1,1,1,1,1,1,1,1,1,1,1,1,1,1,1,1,1,
1,1,1,1,1,1,1,1,1,1,1,1,1,1,1,1,1,1,1,1,1,1,1,1,1,1,1,1,1,1,1,1,1,1,1,1,
1,1,1,1,1,1,1,1,1,1,1,1,1,1,1,1,1,1,1,1,1,1,1,1,1,1,1,1,1,1,1,1,1,1,1,1,
1,1,1,1,1,1,1,1,1,1,1,1,1,1,1,1,1,1,1,1,1,1,1,1,1,1,1,1,1,1,1,1,1,1,6),
(0.,0.005,0.01,0.015,0.02,0.025,0.03,0.035,0.04,0.045,0.05,0.055,0.06,0.065,
0.07,0.075,0.08,0.085,0.09,0.095,0.1,0.105,0.11,0.115,0.12,0.125,0.13,0.135,
0.14,0.145,0.15,0.155,0.16,0.165,0.17,0.175,0.18,0.185,0.19,0.195,0.2,0.205,
0.21,0.215,0.22,0.225,0.23,0.235,0.24,0.245,0.25,0.255,0.26,0.265,0.27,
0.275,0.28,0.285,0.29,0.295,0.3,0.305,0.31,0.315,0.32,0.325,0.33,0.335,
0.34,0.345,0.35,0.355,0.36,0.365,0.37,0.375,0.38,0.385,0.39,0.395,0.4,0.405,
0.41,0.415,0.42,0.425,0.43,0.435,0.44,0.445,0.45,0.455,0.46,0.465,0.47,
0.475,0.48,0.485,0.49,0.495,0.5,0.505,0.51,0.515,0.52,0.525,0.53,0.535,
0.54,0.545,0.55,0.555,0.56,0.565,0.57,0.575,0.58,0.585,0.59,0.595,0.6,0.605,
0.61,0.615,0.62,0.625,0.63,0.635,0.64,0.645,0.65,0.655,0.66,0.665,0.67,
0.675,0.68,0.685,0.690000000000001,0.695000000000001,0.700000000000001,
0.705000000000001,0.710000000000001,0.715000000000001,0.720000000000001,
0.725000000000001,0.730000000000001,0.735000000000001,0.740000000000001,
0.745000000000001,0.750000000000001,0.755000000000001,0.760000000000001,
0.765000000000001,0.770000000000001,0.775000000000001,0.780000000000001,
0.785000000000001,0.790000000000001,0.795000000000001,0.800000000000001,
0.805000000000001,0.810000000000001,0.815000000000001,0.820000000000001,
0.825000000000001,0.830000000000001,0.835000000000001,0.840000000000001,
0.845000000000001,0.850000000000001,0.855000000000001,0.860000000000001,
0.865000000000001,0.870000000000001,0.875000000000001,0.880000000000001,
0.885000000000001,0.890000000000001,0.895000000000001,0.900000000000001,
0.905000000000001,0.910000000000001,0.915000000000001,0.920000000000001,
0.925000000000001,0.930000000000001,0.935000000000001,0.940000000000001,
0.945000000000001,0.950000000000001,0.955000000000001,0.960000000000001,
0.965000000000001,0.970000000000001,0.975000000000001,0.980000000000001,
0.985000000000001,0.990000000000001,0.995000000000001,1.),.UNSPECIFIED.)
CURVE()
GEOMETRIC_REPRESENTATION_ITEM()
RATIONAL_B_SPLINE_CURVE((1.,1.,1.,1.,1.,1.,1.,1.,1.,1.,1.,1.,1.,1.,1.,1.,
1.,1.,1.,1.,1.,1.,1.,1.,1.,1.,1.,1.,1.,1.,1.,1.,1.,1.,1.,1.,1.,1.,1.,1.,
1.,1.,1.,1.,1.,1.,1.,1.,1.,1.,1.,1.,1.,1.,1.,1.,1.,1.,1.,1.,1.,1.,1.,1.,
1.,1.,1.,1.,1.,1.,1.,1.,1.,1.,1.,1.,1.,1.,1.,1.,1.,1.,1.,1.,1.,1.,1.,1.,
1.,1.,1.,1.,1.,1.,1.,1.,1.,1.,1.,1.,1.,1.,1.,1.,1.,1.,1.,1.,1.,1.,1.,1.,
1.,1.,1.,1.,1.,1.,1.,1.,1.,1.,1.,1.,1.,1.,1.,1.,1.,1.,1.,1.,1.,1.,1.,1.,
1.,1.,1.,1.,1.,1.,1.,1.,1.,1.,1.,1.,1.,1.,1.,1.,1.,1.,1.,1.,1.,1.,1.,1.,
1.,1.,1.,1.,1.,1.,1.,1.,1.,1.,1.,1.,1.,1.,1.,1.,1.,1.,1.,1.,1.,1.,1.,1.,
1.,1.,1.,1.,1.,1.,1.,1.,1.,1.,1.,1.,1.,1.,1.,1.,1.,1.,1.,1.,1.))
REPRESENTATION_ITEM('')
);
#862=(
BOUNDED_CURVE()
B_SPLINE_CURVE(5,(#247184,#247185,#247186,#247187,#247188,#247189,#247190,
#247191,#247192,#247193,#247194,#247195,#247196,#247197,#247198,#247199,
#247200,#247201,#247202,#247203,#247204,#247205,#247206,#247207,#247208,
#247209,#247210,#247211,#247212,#247213,#247214,#247215,#247216,#247217,
#247218,#247219,#247220,#247221,#247222,#247223,#247224,#247225,#247226,
#247227,#247228,#247229,#247230,#247231,#247232,#247233,#247234,#247235,
#247236,#247237,#247238,#247239,#247240,#247241,#247242,#247243,#247244,
#247245,#247246,#247247,#247248,#247249,#247250,#247251,#247252,#247253,
#247254,#247255,#247256,#247257,#247258,#247259,#247260,#247261,#247262,
#247263,#247264,#247265,#247266,#247267,#247268,#247269,#247270,#247271,
#247272,#247273,#247274,#247275,#247276,#247277,#247278,#247279,#247280,
#247281,#247282,#247283,#247284,#247285,#247286,#247287,#247288,#247289,
#247290,#247291,#247292,#247293,#247294,#247295,#247296,#247297,#247298,
#247299,#247300,#247301,#247302,#247303,#247304,#247305,#247306,#247307,
#247308,#247309,#247310,#247311,#247312,#247313,#247314,#247315,#247316,
#247317,#247318,#247319,#247320,#247321,#247322,#247323,#247324,#247325,
#247326,#247327,#247328,#247329,#247330,#247331,#247332,#247333,#247334,
#247335,#247336,#247337,#247338,#247339,#247340,#247341,#247342,#247343,
#247344,#247345,#247346,#247347,#247348,#247349,#247350,#247351,#247352,
#247353,#247354,#247355,#247356,#247357,#247358,#247359,#247360,#247361,
#247362,#247363,#247364,#247365,#247366,#247367,#247368,#247369,#247370,
#247371,#247372,#247373,#247374,#247375,#247376,#247377,#247378,#247379,
#247380,#247381,#247382,#247383,#247384,#247385,#247386,#247387,#247388),
 .UNSPECIFIED.,.F.,.F.)
B_SPLINE_CURVE_WITH_KNOTS((6,1,1,1,1,1,1,1,1,1,1,1,1,1,1,1,1,1,1,1,1,1,
1,1,1,1,1,1,1,1,1,1,1,1,1,1,1,1,1,1,1,1,1,1,1,1,1,1,1,1,1,1,1,1,1,1,1,1,
1,1,1,1,1,1,1,1,1,1,1,1,1,1,1,1,1,1,1,1,1,1,1,1,1,1,1,1,1,1,1,1,1,1,1,1,
1,1,1,1,1,1,1,1,1,1,1,1,1,1,1,1,1,1,1,1,1,1,1,1,1,1,1,1,1,1,1,1,1,1,1,1,
1,1,1,1,1,1,1,1,1,1,1,1,1,1,1,1,1,1,1,1,1,1,1,1,1,1,1,1,1,1,1,1,1,1,1,1,
1,1,1,1,1,1,1,1,1,1,1,1,1,1,1,1,1,1,1,1,1,1,1,1,1,1,1,1,1,1,1,1,1,1,6),
(-1.,-0.995000000000001,-0.990000000000001,-0.985000000000001,-0.980000000000001,
-0.975000000000001,-0.970000000000001,-0.965000000000001,-0.960000000000001,
-0.955000000000001,-0.950000000000001,-0.945000000000001,-0.940000000000001,
-0.935000000000001,-0.930000000000001,-0.925000000000001,-0.920000000000001,
-0.915000000000001,-0.910000000000001,-0.905000000000001,-0.900000000000001,
-0.895000000000001,-0.890000000000001,-0.885000000000001,-0.880000000000001,
-0.875000000000001,-0.870000000000001,-0.865000000000001,-0.860000000000001,
-0.855000000000001,-0.850000000000001,-0.845000000000001,-0.840000000000001,
-0.835000000000001,-0.830000000000001,-0.825000000000001,-0.820000000000001,
-0.815000000000001,-0.810000000000001,-0.805000000000001,-0.800000000000001,
-0.795000000000001,-0.790000000000001,-0.785000000000001,-0.780000000000001,
-0.775000000000001,-0.770000000000001,-0.765000000000001,-0.760000000000001,
-0.755000000000001,-0.750000000000001,-0.745000000000001,-0.740000000000001,
-0.735000000000001,-0.730000000000001,-0.725000000000001,-0.720000000000001,
-0.715000000000001,-0.710000000000001,-0.705000000000001,-0.700000000000001,
-0.695000000000001,-0.690000000000001,-0.685,-0.68,-0.675,-0.67,-0.665,
-0.66,-0.655,-0.65,-0.645,-0.64,-0.635,-0.63,-0.625,-0.62,-0.615,-0.61,
-0.605,-0.6,-0.595,-0.59,-0.585,-0.58,-0.575,-0.57,-0.565,-0.56,-0.555,
-0.55,-0.545,-0.54,-0.535,-0.53,-0.525,-0.52,-0.515,-0.51,-0.505,-0.5,-0.495,
-0.49,-0.485,-0.48,-0.475,-0.47,-0.465,-0.46,-0.455,-0.45,-0.445,-0.44,
-0.435,-0.43,-0.425,-0.42,-0.415,-0.41,-0.405,-0.4,-0.395,-0.39,-0.385,
-0.38,-0.375,-0.37,-0.365,-0.36,-0.355,-0.35,-0.345,-0.34,-0.335,-0.33,
-0.325,-0.32,-0.315,-0.31,-0.305,-0.3,-0.295,-0.29,-0.285,-0.28,-0.275,
-0.27,-0.265,-0.26,-0.255,-0.25,-0.245,-0.24,-0.235,-0.23,-0.225,-0.22,
-0.215,-0.21,-0.205,-0.2,-0.195,-0.19,-0.185,-0.18,-0.175,-0.17,-0.165,
-0.16,-0.155,-0.15,-0.145,-0.14,-0.135,-0.13,-0.125,-0.12,-0.115,-0.11,
-0.105,-0.1,-0.095,-0.09,-0.085,-0.08,-0.075,-0.07,-0.065,-0.06,-0.055,
-0.05,-0.045,-0.04,-0.035,-0.03,-0.025,-0.02,-0.015,-0.01,-0.005,0.),
 .UNSPECIFIED.)
CURVE()
GEOMETRIC_REPRESENTATION_ITEM()
RATIONAL_B_SPLINE_CURVE((1.,1.,1.,1.,1.,1.,1.,1.,1.,1.,1.,1.,1.,1.,1.,1.,
1.,1.,1.,1.,1.,1.,1.,1.,1.,1.,1.,1.,1.,1.,1.,1.,1.,1.,1.,1.,1.,1.,1.,1.,
1.,1.,1.,1.,1.,1.,1.,1.,1.,1.,1.,1.,1.,1.,1.,1.,1.,1.,1.,1.,1.,1.,1.,1.,
1.,1.,1.,1.,1.,1.,1.,1.,1.,1.,1.,1.,1.,1.,1.,1.,1.,1.,1.,1.,1.,1.,1.,1.,
1.,1.,1.,1.,1.,1.,1.,1.,1.,1.,1.,1.,1.,1.,1.,1.,1.,1.,1.,1.,1.,1.,1.,1.,
1.,1.,1.,1.,1.,1.,1.,1.,1.,1.,1.,1.,1.,1.,1.,1.,1.,1.,1.,1.,1.,1.,1.,1.,
1.,1.,1.,1.,1.,1.,1.,1.,1.,1.,1.,1.,1.,1.,1.,1.,1.,1.,1.,1.,1.,1.,1.,1.,
1.,1.,1.,1.,1.,1.,1.,1.,1.,1.,1.,1.,1.,1.,1.,1.,1.,1.,1.,1.,1.,1.,1.,1.,
1.,1.,1.,1.,1.,1.,1.,1.,1.,1.,1.,1.,1.,1.,1.,1.,1.,1.,1.,1.,1.))
REPRESENTATION_ITEM('')
);
#863=(
BOUNDED_CURVE()
B_SPLINE_CURVE(5,(#247807,#247808,#247809,#247810,#247811,#247812,#247813,
#247814,#247815,#247816,#247817,#247818,#247819,#247820,#247821,#247822,
#247823,#247824,#247825,#247826,#247827,#247828,#247829,#247830,#247831,
#247832,#247833,#247834,#247835,#247836,#247837,#247838,#247839,#247840,
#247841,#247842,#247843,#247844,#247845,#247846,#247847,#247848,#247849,
#247850,#247851,#247852,#247853,#247854,#247855,#247856,#247857,#247858,
#247859,#247860,#247861,#247862,#247863,#247864,#247865,#247866,#247867,
#247868,#247869,#247870,#247871,#247872,#247873,#247874,#247875,#247876,
#247877,#247878,#247879,#247880,#247881,#247882,#247883,#247884,#247885,
#247886,#247887,#247888,#247889,#247890,#247891,#247892,#247893,#247894,
#247895,#247896,#247897,#247898,#247899,#247900,#247901,#247902,#247903,
#247904,#247905,#247906,#247907,#247908,#247909,#247910,#247911,#247912,
#247913,#247914,#247915,#247916,#247917,#247918,#247919,#247920,#247921,
#247922,#247923,#247924,#247925,#247926,#247927,#247928,#247929,#247930,
#247931,#247932,#247933,#247934,#247935,#247936,#247937,#247938,#247939,
#247940,#247941,#247942,#247943,#247944,#247945,#247946,#247947,#247948,
#247949,#247950,#247951,#247952,#247953,#247954,#247955,#247956,#247957,
#247958,#247959,#247960,#247961,#247962,#247963,#247964,#247965,#247966,
#247967,#247968,#247969,#247970,#247971,#247972,#247973,#247974,#247975,
#247976,#247977,#247978,#247979,#247980,#247981,#247982,#247983,#247984,
#247985,#247986,#247987,#247988,#247989,#247990,#247991,#247992,#247993,
#247994,#247995,#247996,#247997,#247998,#247999,#248000,#248001,#248002,
#248003,#248004,#248005,#248006,#248007,#248008,#248009,#248010,#248011),
 .UNSPECIFIED.,.F.,.F.)
B_SPLINE_CURVE_WITH_KNOTS((6,1,1,1,1,1,1,1,1,1,1,1,1,1,1,1,1,1,1,1,1,1,
1,1,1,1,1,1,1,1,1,1,1,1,1,1,1,1,1,1,1,1,1,1,1,1,1,1,1,1,1,1,1,1,1,1,1,1,
1,1,1,1,1,1,1,1,1,1,1,1,1,1,1,1,1,1,1,1,1,1,1,1,1,1,1,1,1,1,1,1,1,1,1,1,
1,1,1,1,1,1,1,1,1,1,1,1,1,1,1,1,1,1,1,1,1,1,1,1,1,1,1,1,1,1,1,1,1,1,1,1,
1,1,1,1,1,1,1,1,1,1,1,1,1,1,1,1,1,1,1,1,1,1,1,1,1,1,1,1,1,1,1,1,1,1,1,1,
1,1,1,1,1,1,1,1,1,1,1,1,1,1,1,1,1,1,1,1,1,1,1,1,1,1,1,1,1,1,1,1,1,1,6),
(-1.,-0.995000000000001,-0.990000000000001,-0.985000000000001,-0.980000000000001,
-0.975000000000001,-0.970000000000001,-0.965000000000001,-0.960000000000001,
-0.955000000000001,-0.950000000000001,-0.945000000000001,-0.940000000000001,
-0.935000000000001,-0.930000000000001,-0.925000000000001,-0.920000000000001,
-0.915000000000001,-0.910000000000001,-0.905000000000001,-0.900000000000001,
-0.895000000000001,-0.890000000000001,-0.885000000000001,-0.880000000000001,
-0.875000000000001,-0.870000000000001,-0.865000000000001,-0.860000000000001,
-0.855000000000001,-0.850000000000001,-0.845000000000001,-0.840000000000001,
-0.835000000000001,-0.830000000000001,-0.825000000000001,-0.820000000000001,
-0.815000000000001,-0.810000000000001,-0.805000000000001,-0.800000000000001,
-0.795000000000001,-0.790000000000001,-0.785000000000001,-0.780000000000001,
-0.775000000000001,-0.770000000000001,-0.765000000000001,-0.760000000000001,
-0.755000000000001,-0.750000000000001,-0.745000000000001,-0.740000000000001,
-0.735000000000001,-0.730000000000001,-0.725000000000001,-0.720000000000001,
-0.715000000000001,-0.710000000000001,-0.705000000000001,-0.700000000000001,
-0.695000000000001,-0.690000000000001,-0.685,-0.68,-0.675,-0.67,-0.665,
-0.66,-0.655,-0.65,-0.645,-0.64,-0.635,-0.63,-0.625,-0.62,-0.615,-0.61,
-0.605,-0.6,-0.595,-0.59,-0.585,-0.58,-0.575,-0.57,-0.565,-0.56,-0.555,
-0.55,-0.545,-0.54,-0.535,-0.53,-0.525,-0.52,-0.515,-0.51,-0.505,-0.5,-0.495,
-0.49,-0.485,-0.48,-0.475,-0.47,-0.465,-0.46,-0.455,-0.45,-0.445,-0.44,
-0.435,-0.43,-0.425,-0.42,-0.415,-0.41,-0.405,-0.4,-0.395,-0.39,-0.385,
-0.38,-0.375,-0.37,-0.365,-0.36,-0.355,-0.35,-0.345,-0.34,-0.335,-0.33,
-0.325,-0.32,-0.315,-0.31,-0.305,-0.3,-0.295,-0.29,-0.285,-0.28,-0.275,
-0.27,-0.265,-0.26,-0.255,-0.25,-0.245,-0.24,-0.235,-0.23,-0.225,-0.22,
-0.215,-0.21,-0.205,-0.2,-0.195,-0.19,-0.185,-0.18,-0.175,-0.17,-0.165,
-0.16,-0.155,-0.15,-0.145,-0.14,-0.135,-0.13,-0.125,-0.12,-0.115,-0.11,
-0.105,-0.1,-0.095,-0.09,-0.085,-0.08,-0.075,-0.07,-0.065,-0.06,-0.055,
-0.05,-0.045,-0.04,-0.035,-0.03,-0.025,-0.02,-0.015,-0.01,-0.005,0.),
 .UNSPECIFIED.)
CURVE()
GEOMETRIC_REPRESENTATION_ITEM()
RATIONAL_B_SPLINE_CURVE((1.,1.,1.,1.,1.,1.,1.,1.,1.,1.,1.,1.,1.,1.,1.,1.,
1.,1.,1.,1.,1.,1.,1.,1.,1.,1.,1.,1.,1.,1.,1.,1.,1.,1.,1.,1.,1.,1.,1.,1.,
1.,1.,1.,1.,1.,1.,1.,1.,1.,1.,1.,1.,1.,1.,1.,1.,1.,1.,1.,1.,1.,1.,1.,1.,
1.,1.,1.,1.,1.,1.,1.,1.,1.,1.,1.,1.,1.,1.,1.,1.,1.,1.,1.,1.,1.,1.,1.,1.,
1.,1.,1.,1.,1.,1.,1.,1.,1.,1.,1.,1.,1.,1.,1.,1.,1.,1.,1.,1.,1.,1.,1.,1.,
1.,1.,1.,1.,1.,1.,1.,1.,1.,1.,1.,1.,1.,1.,1.,1.,1.,1.,1.,1.,1.,1.,1.,1.,
1.,1.,1.,1.,1.,1.,1.,1.,1.,1.,1.,1.,1.,1.,1.,1.,1.,1.,1.,1.,1.,1.,1.,1.,
1.,1.,1.,1.,1.,1.,1.,1.,1.,1.,1.,1.,1.,1.,1.,1.,1.,1.,1.,1.,1.,1.,1.,1.,
1.,1.,1.,1.,1.,1.,1.,1.,1.,1.,1.,1.,1.,1.,1.,1.,1.,1.,1.,1.,1.))
REPRESENTATION_ITEM('')
);
#864=(
BOUNDED_CURVE()
B_SPLINE_CURVE(5,(#248014,#248015,#248016,#248017,#248018,#248019,#248020,
#248021,#248022,#248023,#248024,#248025,#248026,#248027,#248028,#248029,
#248030,#248031,#248032,#248033,#248034,#248035,#248036,#248037,#248038,
#248039,#248040,#248041,#248042,#248043,#248044,#248045,#248046,#248047,
#248048,#248049,#248050,#248051,#248052,#248053,#248054,#248055,#248056,
#248057,#248058,#248059,#248060,#248061,#248062,#248063,#248064,#248065,
#248066,#248067,#248068,#248069,#248070,#248071,#248072,#248073,#248074,
#248075,#248076,#248077,#248078,#248079,#248080,#248081,#248082,#248083,
#248084,#248085,#248086,#248087,#248088,#248089,#248090,#248091,#248092,
#248093,#248094,#248095,#248096,#248097,#248098,#248099,#248100,#248101,
#248102,#248103,#248104,#248105,#248106,#248107,#248108,#248109,#248110,
#248111,#248112,#248113,#248114,#248115,#248116,#248117,#248118,#248119,
#248120,#248121,#248122,#248123,#248124,#248125,#248126,#248127,#248128,
#248129,#248130,#248131,#248132,#248133,#248134,#248135,#248136,#248137,
#248138,#248139,#248140,#248141,#248142,#248143,#248144,#248145,#248146,
#248147,#248148,#248149,#248150,#248151,#248152,#248153,#248154,#248155,
#248156,#248157,#248158,#248159,#248160,#248161,#248162,#248163,#248164,
#248165,#248166,#248167,#248168,#248169,#248170,#248171,#248172,#248173,
#248174,#248175,#248176,#248177,#248178,#248179,#248180,#248181,#248182,
#248183,#248184,#248185,#248186,#248187,#248188,#248189,#248190,#248191,
#248192,#248193,#248194,#248195,#248196,#248197,#248198,#248199,#248200,
#248201,#248202,#248203,#248204,#248205,#248206,#248207,#248208,#248209,
#248210,#248211,#248212,#248213,#248214,#248215,#248216,#248217,#248218),
 .UNSPECIFIED.,.F.,.F.)
B_SPLINE_CURVE_WITH_KNOTS((6,1,1,1,1,1,1,1,1,1,1,1,1,1,1,1,1,1,1,1,1,1,
1,1,1,1,1,1,1,1,1,1,1,1,1,1,1,1,1,1,1,1,1,1,1,1,1,1,1,1,1,1,1,1,1,1,1,1,
1,1,1,1,1,1,1,1,1,1,1,1,1,1,1,1,1,1,1,1,1,1,1,1,1,1,1,1,1,1,1,1,1,1,1,1,
1,1,1,1,1,1,1,1,1,1,1,1,1,1,1,1,1,1,1,1,1,1,1,1,1,1,1,1,1,1,1,1,1,1,1,1,
1,1,1,1,1,1,1,1,1,1,1,1,1,1,1,1,1,1,1,1,1,1,1,1,1,1,1,1,1,1,1,1,1,1,1,1,
1,1,1,1,1,1,1,1,1,1,1,1,1,1,1,1,1,1,1,1,1,1,1,1,1,1,1,1,1,1,1,1,1,1,6),
(0.,0.005,0.01,0.015,0.02,0.025,0.03,0.035,0.04,0.045,0.05,0.055,0.06,0.065,
0.07,0.075,0.08,0.085,0.09,0.095,0.1,0.105,0.11,0.115,0.12,0.125,0.13,0.135,
0.14,0.145,0.15,0.155,0.16,0.165,0.17,0.175,0.18,0.185,0.19,0.195,0.2,0.205,
0.21,0.215,0.22,0.225,0.23,0.235,0.24,0.245,0.25,0.255,0.26,0.265,0.27,
0.275,0.28,0.285,0.29,0.295,0.3,0.305,0.31,0.315,0.32,0.325,0.33,0.335,
0.34,0.345,0.35,0.355,0.36,0.365,0.37,0.375,0.38,0.385,0.39,0.395,0.4,0.405,
0.41,0.415,0.42,0.425,0.43,0.435,0.44,0.445,0.45,0.455,0.46,0.465,0.47,
0.475,0.48,0.485,0.49,0.495,0.5,0.505,0.51,0.515,0.52,0.525,0.53,0.535,
0.54,0.545,0.55,0.555,0.56,0.565,0.57,0.575,0.58,0.585,0.59,0.595,0.6,0.605,
0.61,0.615,0.62,0.625,0.63,0.635,0.64,0.645,0.65,0.655,0.66,0.665,0.67,
0.675,0.68,0.685,0.690000000000001,0.695000000000001,0.700000000000001,
0.705000000000001,0.710000000000001,0.715000000000001,0.720000000000001,
0.725000000000001,0.730000000000001,0.735000000000001,0.740000000000001,
0.745000000000001,0.750000000000001,0.755000000000001,0.760000000000001,
0.765000000000001,0.770000000000001,0.775000000000001,0.780000000000001,
0.785000000000001,0.790000000000001,0.795000000000001,0.800000000000001,
0.805000000000001,0.810000000000001,0.815000000000001,0.820000000000001,
0.825000000000001,0.830000000000001,0.835000000000001,0.840000000000001,
0.845000000000001,0.850000000000001,0.855000000000001,0.860000000000001,
0.865000000000001,0.870000000000001,0.875000000000001,0.880000000000001,
0.885000000000001,0.890000000000001,0.895000000000001,0.900000000000001,
0.905000000000001,0.910000000000001,0.915000000000001,0.920000000000001,
0.925000000000001,0.930000000000001,0.935000000000001,0.940000000000001,
0.945000000000001,0.950000000000001,0.955000000000001,0.960000000000001,
0.965000000000001,0.970000000000001,0.975000000000001,0.980000000000001,
0.985000000000001,0.990000000000001,0.995000000000001,1.),.UNSPECIFIED.)
CURVE()
GEOMETRIC_REPRESENTATION_ITEM()
RATIONAL_B_SPLINE_CURVE((1.,1.,1.,1.,1.,1.,1.,1.,1.,1.,1.,1.,1.,1.,1.,1.,
1.,1.,1.,1.,1.,1.,1.,1.,1.,1.,1.,1.,1.,1.,1.,1.,1.,1.,1.,1.,1.,1.,1.,1.,
1.,1.,1.,1.,1.,1.,1.,1.,1.,1.,1.,1.,1.,1.,1.,1.,1.,1.,1.,1.,1.,1.,1.,1.,
1.,1.,1.,1.,1.,1.,1.,1.,1.,1.,1.,1.,1.,1.,1.,1.,1.,1.,1.,1.,1.,1.,1.,1.,
1.,1.,1.,1.,1.,1.,1.,1.,1.,1.,1.,1.,1.,1.,1.,1.,1.,1.,1.,1.,1.,1.,1.,1.,
1.,1.,1.,1.,1.,1.,1.,1.,1.,1.,1.,1.,1.,1.,1.,1.,1.,1.,1.,1.,1.,1.,1.,1.,
1.,1.,1.,1.,1.,1.,1.,1.,1.,1.,1.,1.,1.,1.,1.,1.,1.,1.,1.,1.,1.,1.,1.,1.,
1.,1.,1.,1.,1.,1.,1.,1.,1.,1.,1.,1.,1.,1.,1.,1.,1.,1.,1.,1.,1.,1.,1.,1.,
1.,1.,1.,1.,1.,1.,1.,1.,1.,1.,1.,1.,1.,1.,1.,1.,1.,1.,1.,1.,1.))
REPRESENTATION_ITEM('')
);
#865=(
BOUNDED_CURVE()
B_SPLINE_CURVE(5,(#248630,#248631,#248632,#248633,#248634,#248635,#248636,
#248637,#248638,#248639,#248640,#248641,#248642,#248643,#248644,#248645,
#248646,#248647,#248648,#248649,#248650,#248651,#248652,#248653,#248654,
#248655,#248656,#248657,#248658,#248659,#248660,#248661,#248662,#248663,
#248664,#248665,#248666,#248667,#248668,#248669,#248670,#248671,#248672,
#248673,#248674,#248675,#248676,#248677,#248678,#248679,#248680,#248681,
#248682,#248683,#248684,#248685,#248686,#248687,#248688,#248689,#248690,
#248691,#248692,#248693,#248694,#248695,#248696,#248697,#248698,#248699,
#248700,#248701,#248702,#248703,#248704,#248705,#248706,#248707,#248708,
#248709,#248710,#248711,#248712,#248713,#248714,#248715,#248716,#248717,
#248718,#248719,#248720,#248721,#248722,#248723,#248724,#248725,#248726,
#248727,#248728,#248729,#248730,#248731,#248732,#248733,#248734,#248735,
#248736,#248737,#248738,#248739,#248740,#248741,#248742,#248743,#248744,
#248745,#248746,#248747,#248748,#248749,#248750,#248751,#248752,#248753,
#248754,#248755,#248756,#248757,#248758,#248759,#248760,#248761,#248762,
#248763,#248764,#248765,#248766,#248767,#248768,#248769,#248770,#248771,
#248772,#248773,#248774,#248775,#248776,#248777,#248778,#248779,#248780,
#248781,#248782,#248783,#248784,#248785,#248786,#248787,#248788,#248789,
#248790,#248791,#248792,#248793,#248794,#248795,#248796,#248797,#248798,
#248799,#248800,#248801,#248802,#248803,#248804,#248805,#248806,#248807,
#248808,#248809,#248810,#248811,#248812,#248813,#248814,#248815,#248816,
#248817,#248818,#248819,#248820,#248821,#248822,#248823,#248824,#248825,
#248826,#248827,#248828,#248829,#248830,#248831,#248832,#248833,#248834),
 .UNSPECIFIED.,.F.,.F.)
B_SPLINE_CURVE_WITH_KNOTS((6,1,1,1,1,1,1,1,1,1,1,1,1,1,1,1,1,1,1,1,1,1,
1,1,1,1,1,1,1,1,1,1,1,1,1,1,1,1,1,1,1,1,1,1,1,1,1,1,1,1,1,1,1,1,1,1,1,1,
1,1,1,1,1,1,1,1,1,1,1,1,1,1,1,1,1,1,1,1,1,1,1,1,1,1,1,1,1,1,1,1,1,1,1,1,
1,1,1,1,1,1,1,1,1,1,1,1,1,1,1,1,1,1,1,1,1,1,1,1,1,1,1,1,1,1,1,1,1,1,1,1,
1,1,1,1,1,1,1,1,1,1,1,1,1,1,1,1,1,1,1,1,1,1,1,1,1,1,1,1,1,1,1,1,1,1,1,1,
1,1,1,1,1,1,1,1,1,1,1,1,1,1,1,1,1,1,1,1,1,1,1,1,1,1,1,1,1,1,1,1,1,1,6),
(0.,0.005,0.01,0.015,0.02,0.025,0.03,0.035,0.04,0.045,0.05,0.055,0.06,0.065,
0.07,0.075,0.08,0.085,0.09,0.095,0.1,0.105,0.11,0.115,0.12,0.125,0.13,0.135,
0.14,0.145,0.15,0.155,0.16,0.165,0.17,0.175,0.18,0.185,0.19,0.195,0.2,0.205,
0.21,0.215,0.22,0.225,0.23,0.235,0.24,0.245,0.25,0.255,0.26,0.265,0.27,
0.275,0.28,0.285,0.29,0.295,0.3,0.305,0.31,0.315,0.32,0.325,0.33,0.335,
0.34,0.345,0.35,0.355,0.36,0.365,0.37,0.375,0.38,0.385,0.39,0.395,0.4,0.405,
0.41,0.415,0.42,0.425,0.43,0.435,0.44,0.445,0.45,0.455,0.46,0.465,0.47,
0.475,0.48,0.485,0.49,0.495,0.5,0.505,0.51,0.515,0.52,0.525,0.53,0.535,
0.54,0.545,0.55,0.555,0.56,0.565,0.57,0.575,0.58,0.585,0.59,0.595,0.6,0.605,
0.61,0.615,0.62,0.625,0.63,0.635,0.64,0.645,0.65,0.655,0.66,0.665,0.67,
0.675,0.68,0.685,0.690000000000001,0.695000000000001,0.700000000000001,
0.705000000000001,0.710000000000001,0.715000000000001,0.720000000000001,
0.725000000000001,0.730000000000001,0.735000000000001,0.740000000000001,
0.745000000000001,0.750000000000001,0.755000000000001,0.760000000000001,
0.765000000000001,0.770000000000001,0.775000000000001,0.780000000000001,
0.785000000000001,0.790000000000001,0.795000000000001,0.800000000000001,
0.805000000000001,0.810000000000001,0.815000000000001,0.820000000000001,
0.825000000000001,0.830000000000001,0.835000000000001,0.840000000000001,
0.845000000000001,0.850000000000001,0.855000000000001,0.860000000000001,
0.865000000000001,0.870000000000001,0.875000000000001,0.880000000000001,
0.885000000000001,0.890000000000001,0.895000000000001,0.900000000000001,
0.905000000000001,0.910000000000001,0.915000000000001,0.920000000000001,
0.925000000000001,0.930000000000001,0.935000000000001,0.940000000000001,
0.945000000000001,0.950000000000001,0.955000000000001,0.960000000000001,
0.965000000000001,0.970000000000001,0.975000000000001,0.980000000000001,
0.985000000000001,0.990000000000001,0.995000000000001,1.),.UNSPECIFIED.)
CURVE()
GEOMETRIC_REPRESENTATION_ITEM()
RATIONAL_B_SPLINE_CURVE((1.,1.,1.,1.,1.,1.,1.,1.,1.,1.,1.,1.,1.,1.,1.,1.,
1.,1.,1.,1.,1.,1.,1.,1.,1.,1.,1.,1.,1.,1.,1.,1.,1.,1.,1.,1.,1.,1.,1.,1.,
1.,1.,1.,1.,1.,1.,1.,1.,1.,1.,1.,1.,1.,1.,1.,1.,1.,1.,1.,1.,1.,1.,1.,1.,
1.,1.,1.,1.,1.,1.,1.,1.,1.,1.,1.,1.,1.,1.,1.,1.,1.,1.,1.,1.,1.,1.,1.,1.,
1.,1.,1.,1.,1.,1.,1.,1.,1.,1.,1.,1.,1.,1.,1.,1.,1.,1.,1.,1.,1.,1.,1.,1.,
1.,1.,1.,1.,1.,1.,1.,1.,1.,1.,1.,1.,1.,1.,1.,1.,1.,1.,1.,1.,1.,1.,1.,1.,
1.,1.,1.,1.,1.,1.,1.,1.,1.,1.,1.,1.,1.,1.,1.,1.,1.,1.,1.,1.,1.,1.,1.,1.,
1.,1.,1.,1.,1.,1.,1.,1.,1.,1.,1.,1.,1.,1.,1.,1.,1.,1.,1.,1.,1.,1.,1.,1.,
1.,1.,1.,1.,1.,1.,1.,1.,1.,1.,1.,1.,1.,1.,1.,1.,1.,1.,1.,1.,1.))
REPRESENTATION_ITEM('')
);
#866=(
BOUNDED_CURVE()
B_SPLINE_CURVE(5,(#248836,#248837,#248838,#248839,#248840,#248841,#248842,
#248843,#248844,#248845,#248846,#248847,#248848,#248849,#248850,#248851,
#248852,#248853,#248854,#248855,#248856,#248857,#248858,#248859,#248860,
#248861,#248862,#248863,#248864,#248865,#248866,#248867,#248868,#248869,
#248870,#248871,#248872,#248873,#248874,#248875,#248876,#248877,#248878,
#248879,#248880,#248881,#248882,#248883,#248884,#248885,#248886,#248887,
#248888,#248889,#248890,#248891,#248892,#248893,#248894,#248895,#248896,
#248897,#248898,#248899,#248900,#248901,#248902,#248903,#248904,#248905,
#248906,#248907,#248908,#248909,#248910,#248911,#248912,#248913,#248914,
#248915,#248916,#248917,#248918,#248919,#248920,#248921,#248922,#248923,
#248924,#248925,#248926,#248927,#248928,#248929,#248930,#248931,#248932,
#248933,#248934,#248935,#248936,#248937,#248938,#248939,#248940,#248941,
#248942,#248943,#248944,#248945,#248946,#248947,#248948,#248949,#248950,
#248951,#248952,#248953,#248954,#248955,#248956,#248957,#248958,#248959,
#248960,#248961,#248962,#248963,#248964,#248965,#248966,#248967,#248968,
#248969,#248970,#248971,#248972,#248973,#248974,#248975,#248976,#248977,
#248978,#248979,#248980,#248981,#248982,#248983,#248984,#248985,#248986,
#248987,#248988,#248989,#248990,#248991,#248992,#248993,#248994,#248995,
#248996,#248997,#248998,#248999,#249000,#249001,#249002,#249003,#249004,
#249005,#249006,#249007,#249008,#249009,#249010,#249011,#249012,#249013,
#249014,#249015,#249016,#249017,#249018,#249019,#249020,#249021,#249022,
#249023,#249024,#249025,#249026,#249027,#249028,#249029,#249030,#249031,
#249032,#249033,#249034,#249035,#249036,#249037,#249038,#249039,#249040),
 .UNSPECIFIED.,.F.,.F.)
B_SPLINE_CURVE_WITH_KNOTS((6,1,1,1,1,1,1,1,1,1,1,1,1,1,1,1,1,1,1,1,1,1,
1,1,1,1,1,1,1,1,1,1,1,1,1,1,1,1,1,1,1,1,1,1,1,1,1,1,1,1,1,1,1,1,1,1,1,1,
1,1,1,1,1,1,1,1,1,1,1,1,1,1,1,1,1,1,1,1,1,1,1,1,1,1,1,1,1,1,1,1,1,1,1,1,
1,1,1,1,1,1,1,1,1,1,1,1,1,1,1,1,1,1,1,1,1,1,1,1,1,1,1,1,1,1,1,1,1,1,1,1,
1,1,1,1,1,1,1,1,1,1,1,1,1,1,1,1,1,1,1,1,1,1,1,1,1,1,1,1,1,1,1,1,1,1,1,1,
1,1,1,1,1,1,1,1,1,1,1,1,1,1,1,1,1,1,1,1,1,1,1,1,1,1,1,1,1,1,1,1,1,1,6),
(-1.,-0.995000000000001,-0.990000000000001,-0.985000000000001,-0.980000000000001,
-0.975000000000001,-0.970000000000001,-0.965000000000001,-0.960000000000001,
-0.955000000000001,-0.950000000000001,-0.945000000000001,-0.940000000000001,
-0.935000000000001,-0.930000000000001,-0.925000000000001,-0.920000000000001,
-0.915000000000001,-0.910000000000001,-0.905000000000001,-0.900000000000001,
-0.895000000000001,-0.890000000000001,-0.885000000000001,-0.880000000000001,
-0.875000000000001,-0.870000000000001,-0.865000000000001,-0.860000000000001,
-0.855000000000001,-0.850000000000001,-0.845000000000001,-0.840000000000001,
-0.835000000000001,-0.830000000000001,-0.825000000000001,-0.820000000000001,
-0.815000000000001,-0.810000000000001,-0.805000000000001,-0.800000000000001,
-0.795000000000001,-0.790000000000001,-0.785000000000001,-0.780000000000001,
-0.775000000000001,-0.770000000000001,-0.765000000000001,-0.760000000000001,
-0.755000000000001,-0.750000000000001,-0.745000000000001,-0.740000000000001,
-0.735000000000001,-0.730000000000001,-0.725000000000001,-0.720000000000001,
-0.715000000000001,-0.710000000000001,-0.705000000000001,-0.700000000000001,
-0.695000000000001,-0.690000000000001,-0.685,-0.68,-0.675,-0.67,-0.665,
-0.66,-0.655,-0.65,-0.645,-0.64,-0.635,-0.63,-0.625,-0.62,-0.615,-0.61,
-0.605,-0.6,-0.595,-0.59,-0.585,-0.58,-0.575,-0.57,-0.565,-0.56,-0.555,
-0.55,-0.545,-0.54,-0.535,-0.53,-0.525,-0.52,-0.515,-0.51,-0.505,-0.5,-0.495,
-0.49,-0.485,-0.48,-0.475,-0.47,-0.465,-0.46,-0.455,-0.45,-0.445,-0.44,
-0.435,-0.43,-0.425,-0.42,-0.415,-0.41,-0.405,-0.4,-0.395,-0.39,-0.385,
-0.38,-0.375,-0.37,-0.365,-0.36,-0.355,-0.35,-0.345,-0.34,-0.335,-0.33,
-0.325,-0.32,-0.315,-0.31,-0.305,-0.3,-0.295,-0.29,-0.285,-0.28,-0.275,
-0.27,-0.265,-0.26,-0.255,-0.25,-0.245,-0.24,-0.235,-0.23,-0.225,-0.22,
-0.215,-0.21,-0.205,-0.2,-0.195,-0.19,-0.185,-0.18,-0.175,-0.17,-0.165,
-0.16,-0.155,-0.15,-0.145,-0.14,-0.135,-0.13,-0.125,-0.12,-0.115,-0.11,
-0.105,-0.1,-0.095,-0.09,-0.085,-0.08,-0.075,-0.07,-0.065,-0.06,-0.055,
-0.05,-0.045,-0.04,-0.035,-0.03,-0.025,-0.02,-0.015,-0.01,-0.005,0.),
 .UNSPECIFIED.)
CURVE()
GEOMETRIC_REPRESENTATION_ITEM()
RATIONAL_B_SPLINE_CURVE((1.,1.,1.,1.,1.,1.,1.,1.,1.,1.,1.,1.,1.,1.,1.,1.,
1.,1.,1.,1.,1.,1.,1.,1.,1.,1.,1.,1.,1.,1.,1.,1.,1.,1.,1.,1.,1.,1.,1.,1.,
1.,1.,1.,1.,1.,1.,1.,1.,1.,1.,1.,1.,1.,1.,1.,1.,1.,1.,1.,1.,1.,1.,1.,1.,
1.,1.,1.,1.,1.,1.,1.,1.,1.,1.,1.,1.,1.,1.,1.,1.,1.,1.,1.,1.,1.,1.,1.,1.,
1.,1.,1.,1.,1.,1.,1.,1.,1.,1.,1.,1.,1.,1.,1.,1.,1.,1.,1.,1.,1.,1.,1.,1.,
1.,1.,1.,1.,1.,1.,1.,1.,1.,1.,1.,1.,1.,1.,1.,1.,1.,1.,1.,1.,1.,1.,1.,1.,
1.,1.,1.,1.,1.,1.,1.,1.,1.,1.,1.,1.,1.,1.,1.,1.,1.,1.,1.,1.,1.,1.,1.,1.,
1.,1.,1.,1.,1.,1.,1.,1.,1.,1.,1.,1.,1.,1.,1.,1.,1.,1.,1.,1.,1.,1.,1.,1.,
1.,1.,1.,1.,1.,1.,1.,1.,1.,1.,1.,1.,1.,1.,1.,1.,1.,1.,1.,1.,1.))
REPRESENTATION_ITEM('')
);
#867=(
BOUNDED_CURVE()
B_SPLINE_CURVE(5,(#249459,#249460,#249461,#249462,#249463,#249464,#249465,
#249466,#249467,#249468,#249469,#249470,#249471,#249472,#249473,#249474,
#249475,#249476,#249477,#249478,#249479,#249480,#249481,#249482,#249483,
#249484,#249485,#249486,#249487,#249488,#249489,#249490,#249491,#249492,
#249493,#249494,#249495,#249496,#249497,#249498,#249499,#249500,#249501,
#249502,#249503,#249504,#249505,#249506,#249507,#249508,#249509,#249510,
#249511,#249512,#249513,#249514,#249515,#249516,#249517,#249518,#249519,
#249520,#249521,#249522,#249523,#249524,#249525,#249526,#249527,#249528,
#249529,#249530,#249531,#249532,#249533,#249534,#249535,#249536,#249537,
#249538,#249539,#249540,#249541,#249542,#249543,#249544,#249545,#249546,
#249547,#249548,#249549,#249550,#249551,#249552,#249553,#249554,#249555,
#249556,#249557,#249558,#249559,#249560,#249561,#249562,#249563,#249564,
#249565,#249566,#249567,#249568,#249569,#249570,#249571,#249572,#249573,
#249574,#249575,#249576,#249577,#249578,#249579,#249580,#249581,#249582,
#249583,#249584,#249585,#249586,#249587,#249588,#249589,#249590,#249591,
#249592,#249593,#249594,#249595,#249596,#249597,#249598,#249599,#249600,
#249601,#249602,#249603,#249604,#249605,#249606,#249607,#249608,#249609,
#249610,#249611,#249612,#249613,#249614,#249615,#249616,#249617,#249618,
#249619,#249620,#249621,#249622,#249623,#249624,#249625,#249626,#249627,
#249628,#249629,#249630,#249631,#249632,#249633,#249634,#249635,#249636,
#249637,#249638,#249639,#249640,#249641,#249642,#249643,#249644,#249645,
#249646,#249647,#249648,#249649,#249650,#249651,#249652,#249653,#249654,
#249655,#249656,#249657,#249658,#249659,#249660,#249661,#249662,#249663),
 .UNSPECIFIED.,.F.,.F.)
B_SPLINE_CURVE_WITH_KNOTS((6,1,1,1,1,1,1,1,1,1,1,1,1,1,1,1,1,1,1,1,1,1,
1,1,1,1,1,1,1,1,1,1,1,1,1,1,1,1,1,1,1,1,1,1,1,1,1,1,1,1,1,1,1,1,1,1,1,1,
1,1,1,1,1,1,1,1,1,1,1,1,1,1,1,1,1,1,1,1,1,1,1,1,1,1,1,1,1,1,1,1,1,1,1,1,
1,1,1,1,1,1,1,1,1,1,1,1,1,1,1,1,1,1,1,1,1,1,1,1,1,1,1,1,1,1,1,1,1,1,1,1,
1,1,1,1,1,1,1,1,1,1,1,1,1,1,1,1,1,1,1,1,1,1,1,1,1,1,1,1,1,1,1,1,1,1,1,1,
1,1,1,1,1,1,1,1,1,1,1,1,1,1,1,1,1,1,1,1,1,1,1,1,1,1,1,1,1,1,1,1,1,1,6),
(-1.,-0.995000000000001,-0.990000000000001,-0.985000000000001,-0.980000000000001,
-0.975000000000001,-0.970000000000001,-0.965000000000001,-0.960000000000001,
-0.955000000000001,-0.950000000000001,-0.945000000000001,-0.940000000000001,
-0.935000000000001,-0.930000000000001,-0.925000000000001,-0.920000000000001,
-0.915000000000001,-0.910000000000001,-0.905000000000001,-0.900000000000001,
-0.895000000000001,-0.890000000000001,-0.885000000000001,-0.880000000000001,
-0.875000000000001,-0.870000000000001,-0.865000000000001,-0.860000000000001,
-0.855000000000001,-0.850000000000001,-0.845000000000001,-0.840000000000001,
-0.835000000000001,-0.830000000000001,-0.825000000000001,-0.820000000000001,
-0.815000000000001,-0.810000000000001,-0.805000000000001,-0.800000000000001,
-0.795000000000001,-0.790000000000001,-0.785000000000001,-0.780000000000001,
-0.775000000000001,-0.770000000000001,-0.765000000000001,-0.760000000000001,
-0.755000000000001,-0.750000000000001,-0.745000000000001,-0.740000000000001,
-0.735000000000001,-0.730000000000001,-0.725000000000001,-0.720000000000001,
-0.715000000000001,-0.710000000000001,-0.705000000000001,-0.700000000000001,
-0.695000000000001,-0.690000000000001,-0.685,-0.68,-0.675,-0.67,-0.665,
-0.66,-0.655,-0.65,-0.645,-0.64,-0.635,-0.63,-0.625,-0.62,-0.615,-0.61,
-0.605,-0.6,-0.595,-0.59,-0.585,-0.58,-0.575,-0.57,-0.565,-0.56,-0.555,
-0.55,-0.545,-0.54,-0.535,-0.53,-0.525,-0.52,-0.515,-0.51,-0.505,-0.5,-0.495,
-0.49,-0.485,-0.48,-0.475,-0.47,-0.465,-0.46,-0.455,-0.45,-0.445,-0.44,
-0.435,-0.43,-0.425,-0.42,-0.415,-0.41,-0.405,-0.4,-0.395,-0.39,-0.385,
-0.38,-0.375,-0.37,-0.365,-0.36,-0.355,-0.35,-0.345,-0.34,-0.335,-0.33,
-0.325,-0.32,-0.315,-0.31,-0.305,-0.3,-0.295,-0.29,-0.285,-0.28,-0.275,
-0.27,-0.265,-0.26,-0.255,-0.25,-0.245,-0.24,-0.235,-0.23,-0.225,-0.22,
-0.215,-0.21,-0.205,-0.2,-0.195,-0.19,-0.185,-0.18,-0.175,-0.17,-0.165,
-0.16,-0.155,-0.15,-0.145,-0.14,-0.135,-0.13,-0.125,-0.12,-0.115,-0.11,
-0.105,-0.1,-0.095,-0.09,-0.085,-0.08,-0.075,-0.07,-0.065,-0.06,-0.055,
-0.05,-0.045,-0.04,-0.035,-0.03,-0.025,-0.02,-0.015,-0.01,-0.005,0.),
 .UNSPECIFIED.)
CURVE()
GEOMETRIC_REPRESENTATION_ITEM()
RATIONAL_B_SPLINE_CURVE((1.,1.,1.,1.,1.,1.,1.,1.,1.,1.,1.,1.,1.,1.,1.,1.,
1.,1.,1.,1.,1.,1.,1.,1.,1.,1.,1.,1.,1.,1.,1.,1.,1.,1.,1.,1.,1.,1.,1.,1.,
1.,1.,1.,1.,1.,1.,1.,1.,1.,1.,1.,1.,1.,1.,1.,1.,1.,1.,1.,1.,1.,1.,1.,1.,
1.,1.,1.,1.,1.,1.,1.,1.,1.,1.,1.,1.,1.,1.,1.,1.,1.,1.,1.,1.,1.,1.,1.,1.,
1.,1.,1.,1.,1.,1.,1.,1.,1.,1.,1.,1.,1.,1.,1.,1.,1.,1.,1.,1.,1.,1.,1.,1.,
1.,1.,1.,1.,1.,1.,1.,1.,1.,1.,1.,1.,1.,1.,1.,1.,1.,1.,1.,1.,1.,1.,1.,1.,
1.,1.,1.,1.,1.,1.,1.,1.,1.,1.,1.,1.,1.,1.,1.,1.,1.,1.,1.,1.,1.,1.,1.,1.,
1.,1.,1.,1.,1.,1.,1.,1.,1.,1.,1.,1.,1.,1.,1.,1.,1.,1.,1.,1.,1.,1.,1.,1.,
1.,1.,1.,1.,1.,1.,1.,1.,1.,1.,1.,1.,1.,1.,1.,1.,1.,1.,1.,1.,1.))
REPRESENTATION_ITEM('')
);
#868=(
BOUNDED_CURVE()
B_SPLINE_CURVE(5,(#249666,#249667,#249668,#249669,#249670,#249671,#249672,
#249673,#249674,#249675,#249676,#249677,#249678,#249679,#249680,#249681,
#249682,#249683,#249684,#249685,#249686,#249687,#249688,#249689,#249690,
#249691,#249692,#249693,#249694,#249695,#249696,#249697,#249698,#249699,
#249700,#249701,#249702,#249703,#249704,#249705,#249706,#249707,#249708,
#249709,#249710,#249711,#249712,#249713,#249714,#249715,#249716,#249717,
#249718,#249719,#249720,#249721,#249722,#249723,#249724,#249725,#249726,
#249727,#249728,#249729,#249730,#249731,#249732,#249733,#249734,#249735,
#249736,#249737,#249738,#249739,#249740,#249741,#249742,#249743,#249744,
#249745,#249746,#249747,#249748,#249749,#249750,#249751,#249752,#249753,
#249754,#249755,#249756,#249757,#249758,#249759,#249760,#249761,#249762,
#249763,#249764,#249765,#249766,#249767,#249768,#249769,#249770,#249771,
#249772,#249773,#249774,#249775,#249776,#249777,#249778,#249779,#249780,
#249781,#249782,#249783,#249784,#249785,#249786,#249787,#249788,#249789,
#249790,#249791,#249792,#249793,#249794,#249795,#249796,#249797,#249798,
#249799,#249800,#249801,#249802,#249803,#249804,#249805,#249806,#249807,
#249808,#249809,#249810,#249811,#249812,#249813,#249814,#249815,#249816,
#249817,#249818,#249819,#249820,#249821,#249822,#249823,#249824,#249825,
#249826,#249827,#249828,#249829,#249830,#249831,#249832,#249833,#249834,
#249835,#249836,#249837,#249838,#249839,#249840,#249841,#249842,#249843,
#249844,#249845,#249846,#249847,#249848,#249849,#249850,#249851,#249852,
#249853,#249854,#249855,#249856,#249857,#249858,#249859,#249860,#249861,
#249862,#249863,#249864,#249865,#249866,#249867,#249868,#249869,#249870),
 .UNSPECIFIED.,.F.,.F.)
B_SPLINE_CURVE_WITH_KNOTS((6,1,1,1,1,1,1,1,1,1,1,1,1,1,1,1,1,1,1,1,1,1,
1,1,1,1,1,1,1,1,1,1,1,1,1,1,1,1,1,1,1,1,1,1,1,1,1,1,1,1,1,1,1,1,1,1,1,1,
1,1,1,1,1,1,1,1,1,1,1,1,1,1,1,1,1,1,1,1,1,1,1,1,1,1,1,1,1,1,1,1,1,1,1,1,
1,1,1,1,1,1,1,1,1,1,1,1,1,1,1,1,1,1,1,1,1,1,1,1,1,1,1,1,1,1,1,1,1,1,1,1,
1,1,1,1,1,1,1,1,1,1,1,1,1,1,1,1,1,1,1,1,1,1,1,1,1,1,1,1,1,1,1,1,1,1,1,1,
1,1,1,1,1,1,1,1,1,1,1,1,1,1,1,1,1,1,1,1,1,1,1,1,1,1,1,1,1,1,1,1,1,1,6),
(0.,0.005,0.01,0.015,0.02,0.025,0.03,0.035,0.04,0.045,0.05,0.055,0.06,0.065,
0.07,0.075,0.08,0.085,0.09,0.095,0.1,0.105,0.11,0.115,0.12,0.125,0.13,0.135,
0.14,0.145,0.15,0.155,0.16,0.165,0.17,0.175,0.18,0.185,0.19,0.195,0.2,0.205,
0.21,0.215,0.22,0.225,0.23,0.235,0.24,0.245,0.25,0.255,0.26,0.265,0.27,
0.275,0.28,0.285,0.29,0.295,0.3,0.305,0.31,0.315,0.32,0.325,0.33,0.335,
0.34,0.345,0.35,0.355,0.36,0.365,0.37,0.375,0.38,0.385,0.39,0.395,0.4,0.405,
0.41,0.415,0.42,0.425,0.43,0.435,0.44,0.445,0.45,0.455,0.46,0.465,0.47,
0.475,0.48,0.485,0.49,0.495,0.5,0.505,0.51,0.515,0.52,0.525,0.53,0.535,
0.54,0.545,0.55,0.555,0.56,0.565,0.57,0.575,0.58,0.585,0.59,0.595,0.6,0.605,
0.61,0.615,0.62,0.625,0.63,0.635,0.64,0.645,0.65,0.655,0.66,0.665,0.67,
0.675,0.68,0.685,0.690000000000001,0.695000000000001,0.700000000000001,
0.705000000000001,0.710000000000001,0.715000000000001,0.720000000000001,
0.725000000000001,0.730000000000001,0.735000000000001,0.740000000000001,
0.745000000000001,0.750000000000001,0.755000000000001,0.760000000000001,
0.765000000000001,0.770000000000001,0.775000000000001,0.780000000000001,
0.785000000000001,0.790000000000001,0.795000000000001,0.800000000000001,
0.805000000000001,0.810000000000001,0.815000000000001,0.820000000000001,
0.825000000000001,0.830000000000001,0.835000000000001,0.840000000000001,
0.845000000000001,0.850000000000001,0.855000000000001,0.860000000000001,
0.865000000000001,0.870000000000001,0.875000000000001,0.880000000000001,
0.885000000000001,0.890000000000001,0.895000000000001,0.900000000000001,
0.905000000000001,0.910000000000001,0.915000000000001,0.920000000000001,
0.925000000000001,0.930000000000001,0.935000000000001,0.940000000000001,
0.945000000000001,0.950000000000001,0.955000000000001,0.960000000000001,
0.965000000000001,0.970000000000001,0.975000000000001,0.980000000000001,
0.985000000000001,0.990000000000001,0.995000000000001,1.),.UNSPECIFIED.)
CURVE()
GEOMETRIC_REPRESENTATION_ITEM()
RATIONAL_B_SPLINE_CURVE((1.,1.,1.,1.,1.,1.,1.,1.,1.,1.,1.,1.,1.,1.,1.,1.,
1.,1.,1.,1.,1.,1.,1.,1.,1.,1.,1.,1.,1.,1.,1.,1.,1.,1.,1.,1.,1.,1.,1.,1.,
1.,1.,1.,1.,1.,1.,1.,1.,1.,1.,1.,1.,1.,1.,1.,1.,1.,1.,1.,1.,1.,1.,1.,1.,
1.,1.,1.,1.,1.,1.,1.,1.,1.,1.,1.,1.,1.,1.,1.,1.,1.,1.,1.,1.,1.,1.,1.,1.,
1.,1.,1.,1.,1.,1.,1.,1.,1.,1.,1.,1.,1.,1.,1.,1.,1.,1.,1.,1.,1.,1.,1.,1.,
1.,1.,1.,1.,1.,1.,1.,1.,1.,1.,1.,1.,1.,1.,1.,1.,1.,1.,1.,1.,1.,1.,1.,1.,
1.,1.,1.,1.,1.,1.,1.,1.,1.,1.,1.,1.,1.,1.,1.,1.,1.,1.,1.,1.,1.,1.,1.,1.,
1.,1.,1.,1.,1.,1.,1.,1.,1.,1.,1.,1.,1.,1.,1.,1.,1.,1.,1.,1.,1.,1.,1.,1.,
1.,1.,1.,1.,1.,1.,1.,1.,1.,1.,1.,1.,1.,1.,1.,1.,1.,1.,1.,1.,1.))
REPRESENTATION_ITEM('')
);
#869=(
BOUNDED_CURVE()
B_SPLINE_CURVE(5,(#250282,#250283,#250284,#250285,#250286,#250287,#250288,
#250289,#250290,#250291,#250292,#250293,#250294,#250295,#250296,#250297,
#250298,#250299,#250300,#250301,#250302,#250303,#250304,#250305,#250306,
#250307,#250308,#250309,#250310,#250311,#250312,#250313,#250314,#250315,
#250316,#250317,#250318,#250319,#250320,#250321,#250322,#250323,#250324,
#250325,#250326,#250327,#250328,#250329,#250330,#250331,#250332,#250333,
#250334,#250335,#250336,#250337,#250338,#250339,#250340,#250341,#250342,
#250343,#250344,#250345,#250346,#250347,#250348,#250349,#250350,#250351,
#250352,#250353,#250354,#250355,#250356,#250357,#250358,#250359,#250360,
#250361,#250362,#250363,#250364,#250365,#250366,#250367,#250368,#250369,
#250370,#250371,#250372,#250373,#250374,#250375,#250376,#250377,#250378,
#250379,#250380,#250381,#250382,#250383,#250384,#250385,#250386,#250387,
#250388,#250389,#250390,#250391,#250392,#250393,#250394,#250395,#250396,
#250397,#250398,#250399,#250400,#250401,#250402,#250403,#250404,#250405,
#250406,#250407,#250408,#250409,#250410,#250411,#250412,#250413,#250414,
#250415,#250416,#250417,#250418,#250419,#250420,#250421,#250422,#250423,
#250424,#250425,#250426,#250427,#250428,#250429,#250430,#250431,#250432,
#250433,#250434,#250435,#250436,#250437,#250438,#250439,#250440,#250441,
#250442,#250443,#250444,#250445,#250446,#250447,#250448,#250449,#250450,
#250451,#250452,#250453,#250454,#250455,#250456,#250457,#250458,#250459,
#250460,#250461,#250462,#250463,#250464,#250465,#250466,#250467,#250468,
#250469,#250470,#250471,#250472,#250473,#250474,#250475,#250476,#250477,
#250478,#250479,#250480,#250481,#250482,#250483,#250484,#250485,#250486),
 .UNSPECIFIED.,.F.,.F.)
B_SPLINE_CURVE_WITH_KNOTS((6,1,1,1,1,1,1,1,1,1,1,1,1,1,1,1,1,1,1,1,1,1,
1,1,1,1,1,1,1,1,1,1,1,1,1,1,1,1,1,1,1,1,1,1,1,1,1,1,1,1,1,1,1,1,1,1,1,1,
1,1,1,1,1,1,1,1,1,1,1,1,1,1,1,1,1,1,1,1,1,1,1,1,1,1,1,1,1,1,1,1,1,1,1,1,
1,1,1,1,1,1,1,1,1,1,1,1,1,1,1,1,1,1,1,1,1,1,1,1,1,1,1,1,1,1,1,1,1,1,1,1,
1,1,1,1,1,1,1,1,1,1,1,1,1,1,1,1,1,1,1,1,1,1,1,1,1,1,1,1,1,1,1,1,1,1,1,1,
1,1,1,1,1,1,1,1,1,1,1,1,1,1,1,1,1,1,1,1,1,1,1,1,1,1,1,1,1,1,1,1,1,1,6),
(0.,0.005,0.01,0.015,0.02,0.025,0.03,0.035,0.04,0.045,0.05,0.055,0.06,0.065,
0.07,0.075,0.08,0.085,0.09,0.095,0.1,0.105,0.11,0.115,0.12,0.125,0.13,0.135,
0.14,0.145,0.15,0.155,0.16,0.165,0.17,0.175,0.18,0.185,0.19,0.195,0.2,0.205,
0.21,0.215,0.22,0.225,0.23,0.235,0.24,0.245,0.25,0.255,0.26,0.265,0.27,
0.275,0.28,0.285,0.29,0.295,0.3,0.305,0.31,0.315,0.32,0.325,0.33,0.335,
0.34,0.345,0.35,0.355,0.36,0.365,0.37,0.375,0.38,0.385,0.39,0.395,0.4,0.405,
0.41,0.415,0.42,0.425,0.43,0.435,0.44,0.445,0.45,0.455,0.46,0.465,0.47,
0.475,0.48,0.485,0.49,0.495,0.5,0.505,0.51,0.515,0.52,0.525,0.53,0.535,
0.54,0.545,0.55,0.555,0.56,0.565,0.57,0.575,0.58,0.585,0.59,0.595,0.6,0.605,
0.61,0.615,0.62,0.625,0.63,0.635,0.64,0.645,0.65,0.655,0.66,0.665,0.67,
0.675,0.68,0.685,0.690000000000001,0.695000000000001,0.700000000000001,
0.705000000000001,0.710000000000001,0.715000000000001,0.720000000000001,
0.725000000000001,0.730000000000001,0.735000000000001,0.740000000000001,
0.745000000000001,0.750000000000001,0.755000000000001,0.760000000000001,
0.765000000000001,0.770000000000001,0.775000000000001,0.780000000000001,
0.785000000000001,0.790000000000001,0.795000000000001,0.800000000000001,
0.805000000000001,0.810000000000001,0.815000000000001,0.820000000000001,
0.825000000000001,0.830000000000001,0.835000000000001,0.840000000000001,
0.845000000000001,0.850000000000001,0.855000000000001,0.860000000000001,
0.865000000000001,0.870000000000001,0.875000000000001,0.880000000000001,
0.885000000000001,0.890000000000001,0.895000000000001,0.900000000000001,
0.905000000000001,0.910000000000001,0.915000000000001,0.920000000000001,
0.925000000000001,0.930000000000001,0.935000000000001,0.940000000000001,
0.945000000000001,0.950000000000001,0.955000000000001,0.960000000000001,
0.965000000000001,0.970000000000001,0.975000000000001,0.980000000000001,
0.985000000000001,0.990000000000001,0.995000000000001,1.),.UNSPECIFIED.)
CURVE()
GEOMETRIC_REPRESENTATION_ITEM()
RATIONAL_B_SPLINE_CURVE((1.,1.,1.,1.,1.,1.,1.,1.,1.,1.,1.,1.,1.,1.,1.,1.,
1.,1.,1.,1.,1.,1.,1.,1.,1.,1.,1.,1.,1.,1.,1.,1.,1.,1.,1.,1.,1.,1.,1.,1.,
1.,1.,1.,1.,1.,1.,1.,1.,1.,1.,1.,1.,1.,1.,1.,1.,1.,1.,1.,1.,1.,1.,1.,1.,
1.,1.,1.,1.,1.,1.,1.,1.,1.,1.,1.,1.,1.,1.,1.,1.,1.,1.,1.,1.,1.,1.,1.,1.,
1.,1.,1.,1.,1.,1.,1.,1.,1.,1.,1.,1.,1.,1.,1.,1.,1.,1.,1.,1.,1.,1.,1.,1.,
1.,1.,1.,1.,1.,1.,1.,1.,1.,1.,1.,1.,1.,1.,1.,1.,1.,1.,1.,1.,1.,1.,1.,1.,
1.,1.,1.,1.,1.,1.,1.,1.,1.,1.,1.,1.,1.,1.,1.,1.,1.,1.,1.,1.,1.,1.,1.,1.,
1.,1.,1.,1.,1.,1.,1.,1.,1.,1.,1.,1.,1.,1.,1.,1.,1.,1.,1.,1.,1.,1.,1.,1.,
1.,1.,1.,1.,1.,1.,1.,1.,1.,1.,1.,1.,1.,1.,1.,1.,1.,1.,1.,1.,1.))
REPRESENTATION_ITEM('')
);
#870=(
BOUNDED_CURVE()
B_SPLINE_CURVE(5,(#250488,#250489,#250490,#250491,#250492,#250493,#250494,
#250495,#250496,#250497,#250498,#250499,#250500,#250501,#250502,#250503,
#250504,#250505,#250506,#250507,#250508,#250509,#250510,#250511,#250512,
#250513,#250514,#250515,#250516,#250517,#250518,#250519,#250520,#250521,
#250522,#250523,#250524,#250525,#250526,#250527,#250528,#250529,#250530,
#250531,#250532,#250533,#250534,#250535,#250536,#250537,#250538,#250539,
#250540,#250541,#250542,#250543,#250544,#250545,#250546,#250547,#250548,
#250549,#250550,#250551,#250552,#250553,#250554,#250555,#250556,#250557,
#250558,#250559,#250560,#250561,#250562,#250563,#250564,#250565,#250566,
#250567,#250568,#250569,#250570,#250571,#250572,#250573,#250574,#250575,
#250576,#250577,#250578,#250579,#250580,#250581,#250582,#250583,#250584,
#250585,#250586,#250587,#250588,#250589,#250590,#250591,#250592,#250593,
#250594,#250595,#250596,#250597,#250598,#250599,#250600,#250601,#250602,
#250603,#250604,#250605,#250606,#250607,#250608,#250609,#250610,#250611,
#250612,#250613,#250614,#250615,#250616,#250617,#250618,#250619,#250620,
#250621,#250622,#250623,#250624,#250625,#250626,#250627,#250628,#250629,
#250630,#250631,#250632,#250633,#250634,#250635,#250636,#250637,#250638,
#250639,#250640,#250641,#250642,#250643,#250644,#250645,#250646,#250647,
#250648,#250649,#250650,#250651,#250652,#250653,#250654,#250655,#250656,
#250657,#250658,#250659,#250660,#250661,#250662,#250663,#250664,#250665,
#250666,#250667,#250668,#250669,#250670,#250671,#250672,#250673,#250674,
#250675,#250676,#250677,#250678,#250679,#250680,#250681,#250682,#250683,
#250684,#250685,#250686,#250687,#250688,#250689,#250690,#250691,#250692),
 .UNSPECIFIED.,.F.,.F.)
B_SPLINE_CURVE_WITH_KNOTS((6,1,1,1,1,1,1,1,1,1,1,1,1,1,1,1,1,1,1,1,1,1,
1,1,1,1,1,1,1,1,1,1,1,1,1,1,1,1,1,1,1,1,1,1,1,1,1,1,1,1,1,1,1,1,1,1,1,1,
1,1,1,1,1,1,1,1,1,1,1,1,1,1,1,1,1,1,1,1,1,1,1,1,1,1,1,1,1,1,1,1,1,1,1,1,
1,1,1,1,1,1,1,1,1,1,1,1,1,1,1,1,1,1,1,1,1,1,1,1,1,1,1,1,1,1,1,1,1,1,1,1,
1,1,1,1,1,1,1,1,1,1,1,1,1,1,1,1,1,1,1,1,1,1,1,1,1,1,1,1,1,1,1,1,1,1,1,1,
1,1,1,1,1,1,1,1,1,1,1,1,1,1,1,1,1,1,1,1,1,1,1,1,1,1,1,1,1,1,1,1,1,1,6),
(-1.,-0.995000000000001,-0.990000000000001,-0.985000000000001,-0.980000000000001,
-0.975000000000001,-0.970000000000001,-0.965000000000001,-0.960000000000001,
-0.955000000000001,-0.950000000000001,-0.945000000000001,-0.940000000000001,
-0.935000000000001,-0.930000000000001,-0.925000000000001,-0.920000000000001,
-0.915000000000001,-0.910000000000001,-0.905000000000001,-0.900000000000001,
-0.895000000000001,-0.890000000000001,-0.885000000000001,-0.880000000000001,
-0.875000000000001,-0.870000000000001,-0.865000000000001,-0.860000000000001,
-0.855000000000001,-0.850000000000001,-0.845000000000001,-0.840000000000001,
-0.835000000000001,-0.830000000000001,-0.825000000000001,-0.820000000000001,
-0.815000000000001,-0.810000000000001,-0.805000000000001,-0.800000000000001,
-0.795000000000001,-0.790000000000001,-0.785000000000001,-0.780000000000001,
-0.775000000000001,-0.770000000000001,-0.765000000000001,-0.760000000000001,
-0.755000000000001,-0.750000000000001,-0.745000000000001,-0.740000000000001,
-0.735000000000001,-0.730000000000001,-0.725000000000001,-0.720000000000001,
-0.715000000000001,-0.710000000000001,-0.705000000000001,-0.700000000000001,
-0.695000000000001,-0.690000000000001,-0.685,-0.68,-0.675,-0.67,-0.665,
-0.66,-0.655,-0.65,-0.645,-0.64,-0.635,-0.63,-0.625,-0.62,-0.615,-0.61,
-0.605,-0.6,-0.595,-0.59,-0.585,-0.58,-0.575,-0.57,-0.565,-0.56,-0.555,
-0.55,-0.545,-0.54,-0.535,-0.53,-0.525,-0.52,-0.515,-0.51,-0.505,-0.5,-0.495,
-0.49,-0.485,-0.48,-0.475,-0.47,-0.465,-0.46,-0.455,-0.45,-0.445,-0.44,
-0.435,-0.43,-0.425,-0.42,-0.415,-0.41,-0.405,-0.4,-0.395,-0.39,-0.385,
-0.38,-0.375,-0.37,-0.365,-0.36,-0.355,-0.35,-0.345,-0.34,-0.335,-0.33,
-0.325,-0.32,-0.315,-0.31,-0.305,-0.3,-0.295,-0.29,-0.285,-0.28,-0.275,
-0.27,-0.265,-0.26,-0.255,-0.25,-0.245,-0.24,-0.235,-0.23,-0.225,-0.22,
-0.215,-0.21,-0.205,-0.2,-0.195,-0.19,-0.185,-0.18,-0.175,-0.17,-0.165,
-0.16,-0.155,-0.15,-0.145,-0.14,-0.135,-0.13,-0.125,-0.12,-0.115,-0.11,
-0.105,-0.1,-0.095,-0.09,-0.085,-0.08,-0.075,-0.07,-0.065,-0.06,-0.055,
-0.05,-0.045,-0.04,-0.035,-0.03,-0.025,-0.02,-0.015,-0.01,-0.005,0.),
 .UNSPECIFIED.)
CURVE()
GEOMETRIC_REPRESENTATION_ITEM()
RATIONAL_B_SPLINE_CURVE((1.,1.,1.,1.,1.,1.,1.,1.,1.,1.,1.,1.,1.,1.,1.,1.,
1.,1.,1.,1.,1.,1.,1.,1.,1.,1.,1.,1.,1.,1.,1.,1.,1.,1.,1.,1.,1.,1.,1.,1.,
1.,1.,1.,1.,1.,1.,1.,1.,1.,1.,1.,1.,1.,1.,1.,1.,1.,1.,1.,1.,1.,1.,1.,1.,
1.,1.,1.,1.,1.,1.,1.,1.,1.,1.,1.,1.,1.,1.,1.,1.,1.,1.,1.,1.,1.,1.,1.,1.,
1.,1.,1.,1.,1.,1.,1.,1.,1.,1.,1.,1.,1.,1.,1.,1.,1.,1.,1.,1.,1.,1.,1.,1.,
1.,1.,1.,1.,1.,1.,1.,1.,1.,1.,1.,1.,1.,1.,1.,1.,1.,1.,1.,1.,1.,1.,1.,1.,
1.,1.,1.,1.,1.,1.,1.,1.,1.,1.,1.,1.,1.,1.,1.,1.,1.,1.,1.,1.,1.,1.,1.,1.,
1.,1.,1.,1.,1.,1.,1.,1.,1.,1.,1.,1.,1.,1.,1.,1.,1.,1.,1.,1.,1.,1.,1.,1.,
1.,1.,1.,1.,1.,1.,1.,1.,1.,1.,1.,1.,1.,1.,1.,1.,1.,1.,1.,1.,1.))
REPRESENTATION_ITEM('')
);
#871=(
BOUNDED_CURVE()
B_SPLINE_CURVE(5,(#251111,#251112,#251113,#251114,#251115,#251116,#251117,
#251118,#251119,#251120,#251121,#251122,#251123,#251124,#251125,#251126,
#251127,#251128,#251129,#251130,#251131,#251132,#251133,#251134,#251135,
#251136,#251137,#251138,#251139,#251140,#251141,#251142,#251143,#251144,
#251145,#251146,#251147,#251148,#251149,#251150,#251151,#251152,#251153,
#251154,#251155,#251156,#251157,#251158,#251159,#251160,#251161,#251162,
#251163,#251164,#251165,#251166,#251167,#251168,#251169,#251170,#251171,
#251172,#251173,#251174,#251175,#251176,#251177,#251178,#251179,#251180,
#251181,#251182,#251183,#251184,#251185,#251186,#251187,#251188,#251189,
#251190,#251191,#251192,#251193,#251194,#251195,#251196,#251197,#251198,
#251199,#251200,#251201,#251202,#251203,#251204,#251205,#251206,#251207,
#251208,#251209,#251210,#251211,#251212,#251213,#251214,#251215,#251216,
#251217,#251218,#251219,#251220,#251221,#251222,#251223,#251224,#251225,
#251226,#251227,#251228,#251229,#251230,#251231,#251232,#251233,#251234,
#251235,#251236,#251237,#251238,#251239,#251240,#251241,#251242,#251243,
#251244,#251245,#251246,#251247,#251248,#251249,#251250,#251251,#251252,
#251253,#251254,#251255,#251256,#251257,#251258,#251259,#251260,#251261,
#251262,#251263,#251264,#251265,#251266,#251267,#251268,#251269,#251270,
#251271,#251272,#251273,#251274,#251275,#251276,#251277,#251278,#251279,
#251280,#251281,#251282,#251283,#251284,#251285,#251286,#251287,#251288,
#251289,#251290,#251291,#251292,#251293,#251294,#251295,#251296,#251297,
#251298,#251299,#251300,#251301,#251302,#251303,#251304,#251305,#251306,
#251307,#251308,#251309,#251310,#251311,#251312,#251313,#251314,#251315),
 .UNSPECIFIED.,.F.,.F.)
B_SPLINE_CURVE_WITH_KNOTS((6,1,1,1,1,1,1,1,1,1,1,1,1,1,1,1,1,1,1,1,1,1,
1,1,1,1,1,1,1,1,1,1,1,1,1,1,1,1,1,1,1,1,1,1,1,1,1,1,1,1,1,1,1,1,1,1,1,1,
1,1,1,1,1,1,1,1,1,1,1,1,1,1,1,1,1,1,1,1,1,1,1,1,1,1,1,1,1,1,1,1,1,1,1,1,
1,1,1,1,1,1,1,1,1,1,1,1,1,1,1,1,1,1,1,1,1,1,1,1,1,1,1,1,1,1,1,1,1,1,1,1,
1,1,1,1,1,1,1,1,1,1,1,1,1,1,1,1,1,1,1,1,1,1,1,1,1,1,1,1,1,1,1,1,1,1,1,1,
1,1,1,1,1,1,1,1,1,1,1,1,1,1,1,1,1,1,1,1,1,1,1,1,1,1,1,1,1,1,1,1,1,1,6),
(-1.,-0.995000000000001,-0.990000000000001,-0.985000000000001,-0.980000000000001,
-0.975000000000001,-0.970000000000001,-0.965000000000001,-0.960000000000001,
-0.955000000000001,-0.950000000000001,-0.945000000000001,-0.940000000000001,
-0.935000000000001,-0.930000000000001,-0.925000000000001,-0.920000000000001,
-0.915000000000001,-0.910000000000001,-0.905000000000001,-0.900000000000001,
-0.895000000000001,-0.890000000000001,-0.885000000000001,-0.880000000000001,
-0.875000000000001,-0.870000000000001,-0.865000000000001,-0.860000000000001,
-0.855000000000001,-0.850000000000001,-0.845000000000001,-0.840000000000001,
-0.835000000000001,-0.830000000000001,-0.825000000000001,-0.820000000000001,
-0.815000000000001,-0.810000000000001,-0.805000000000001,-0.800000000000001,
-0.795000000000001,-0.790000000000001,-0.785000000000001,-0.780000000000001,
-0.775000000000001,-0.770000000000001,-0.765000000000001,-0.760000000000001,
-0.755000000000001,-0.750000000000001,-0.745000000000001,-0.740000000000001,
-0.735000000000001,-0.730000000000001,-0.725000000000001,-0.720000000000001,
-0.715000000000001,-0.710000000000001,-0.705000000000001,-0.700000000000001,
-0.695000000000001,-0.690000000000001,-0.685,-0.68,-0.675,-0.67,-0.665,
-0.66,-0.655,-0.65,-0.645,-0.64,-0.635,-0.63,-0.625,-0.62,-0.615,-0.61,
-0.605,-0.6,-0.595,-0.59,-0.585,-0.58,-0.575,-0.57,-0.565,-0.56,-0.555,
-0.55,-0.545,-0.54,-0.535,-0.53,-0.525,-0.52,-0.515,-0.51,-0.505,-0.5,-0.495,
-0.49,-0.485,-0.48,-0.475,-0.47,-0.465,-0.46,-0.455,-0.45,-0.445,-0.44,
-0.435,-0.43,-0.425,-0.42,-0.415,-0.41,-0.405,-0.4,-0.395,-0.39,-0.385,
-0.38,-0.375,-0.37,-0.365,-0.36,-0.355,-0.35,-0.345,-0.34,-0.335,-0.33,
-0.325,-0.32,-0.315,-0.31,-0.305,-0.3,-0.295,-0.29,-0.285,-0.28,-0.275,
-0.27,-0.265,-0.26,-0.255,-0.25,-0.245,-0.24,-0.235,-0.23,-0.225,-0.22,
-0.215,-0.21,-0.205,-0.2,-0.195,-0.19,-0.185,-0.18,-0.175,-0.17,-0.165,
-0.16,-0.155,-0.15,-0.145,-0.14,-0.135,-0.13,-0.125,-0.12,-0.115,-0.11,
-0.105,-0.1,-0.095,-0.09,-0.085,-0.08,-0.075,-0.07,-0.065,-0.06,-0.055,
-0.05,-0.045,-0.04,-0.035,-0.03,-0.025,-0.02,-0.015,-0.01,-0.005,0.),
 .UNSPECIFIED.)
CURVE()
GEOMETRIC_REPRESENTATION_ITEM()
RATIONAL_B_SPLINE_CURVE((1.,1.,1.,1.,1.,1.,1.,1.,1.,1.,1.,1.,1.,1.,1.,1.,
1.,1.,1.,1.,1.,1.,1.,1.,1.,1.,1.,1.,1.,1.,1.,1.,1.,1.,1.,1.,1.,1.,1.,1.,
1.,1.,1.,1.,1.,1.,1.,1.,1.,1.,1.,1.,1.,1.,1.,1.,1.,1.,1.,1.,1.,1.,1.,1.,
1.,1.,1.,1.,1.,1.,1.,1.,1.,1.,1.,1.,1.,1.,1.,1.,1.,1.,1.,1.,1.,1.,1.,1.,
1.,1.,1.,1.,1.,1.,1.,1.,1.,1.,1.,1.,1.,1.,1.,1.,1.,1.,1.,1.,1.,1.,1.,1.,
1.,1.,1.,1.,1.,1.,1.,1.,1.,1.,1.,1.,1.,1.,1.,1.,1.,1.,1.,1.,1.,1.,1.,1.,
1.,1.,1.,1.,1.,1.,1.,1.,1.,1.,1.,1.,1.,1.,1.,1.,1.,1.,1.,1.,1.,1.,1.,1.,
1.,1.,1.,1.,1.,1.,1.,1.,1.,1.,1.,1.,1.,1.,1.,1.,1.,1.,1.,1.,1.,1.,1.,1.,
1.,1.,1.,1.,1.,1.,1.,1.,1.,1.,1.,1.,1.,1.,1.,1.,1.,1.,1.,1.,1.))
REPRESENTATION_ITEM('')
);
#872=(
BOUNDED_CURVE()
B_SPLINE_CURVE(5,(#251318,#251319,#251320,#251321,#251322,#251323,#251324,
#251325,#251326,#251327,#251328,#251329,#251330,#251331,#251332,#251333,
#251334,#251335,#251336,#251337,#251338,#251339,#251340,#251341,#251342,
#251343,#251344,#251345,#251346,#251347,#251348,#251349,#251350,#251351,
#251352,#251353,#251354,#251355,#251356,#251357,#251358,#251359,#251360,
#251361,#251362,#251363,#251364,#251365,#251366,#251367,#251368,#251369,
#251370,#251371,#251372,#251373,#251374,#251375,#251376,#251377,#251378,
#251379,#251380,#251381,#251382,#251383,#251384,#251385,#251386,#251387,
#251388,#251389,#251390,#251391,#251392,#251393,#251394,#251395,#251396,
#251397,#251398,#251399,#251400,#251401,#251402,#251403,#251404,#251405,
#251406,#251407,#251408,#251409,#251410,#251411,#251412,#251413,#251414,
#251415,#251416,#251417,#251418,#251419,#251420,#251421,#251422,#251423,
#251424,#251425,#251426,#251427,#251428,#251429,#251430,#251431,#251432,
#251433,#251434,#251435,#251436,#251437,#251438,#251439,#251440,#251441,
#251442,#251443,#251444,#251445,#251446,#251447,#251448,#251449,#251450,
#251451,#251452,#251453,#251454,#251455,#251456,#251457,#251458,#251459,
#251460,#251461,#251462,#251463,#251464,#251465,#251466,#251467,#251468,
#251469,#251470,#251471,#251472,#251473,#251474,#251475,#251476,#251477,
#251478,#251479,#251480,#251481,#251482,#251483,#251484,#251485,#251486,
#251487,#251488,#251489,#251490,#251491,#251492,#251493,#251494,#251495,
#251496,#251497,#251498,#251499,#251500,#251501,#251502,#251503,#251504,
#251505,#251506,#251507,#251508,#251509,#251510,#251511,#251512,#251513,
#251514,#251515,#251516,#251517,#251518,#251519,#251520,#251521,#251522),
 .UNSPECIFIED.,.F.,.F.)
B_SPLINE_CURVE_WITH_KNOTS((6,1,1,1,1,1,1,1,1,1,1,1,1,1,1,1,1,1,1,1,1,1,
1,1,1,1,1,1,1,1,1,1,1,1,1,1,1,1,1,1,1,1,1,1,1,1,1,1,1,1,1,1,1,1,1,1,1,1,
1,1,1,1,1,1,1,1,1,1,1,1,1,1,1,1,1,1,1,1,1,1,1,1,1,1,1,1,1,1,1,1,1,1,1,1,
1,1,1,1,1,1,1,1,1,1,1,1,1,1,1,1,1,1,1,1,1,1,1,1,1,1,1,1,1,1,1,1,1,1,1,1,
1,1,1,1,1,1,1,1,1,1,1,1,1,1,1,1,1,1,1,1,1,1,1,1,1,1,1,1,1,1,1,1,1,1,1,1,
1,1,1,1,1,1,1,1,1,1,1,1,1,1,1,1,1,1,1,1,1,1,1,1,1,1,1,1,1,1,1,1,1,1,6),
(0.,0.005,0.01,0.015,0.02,0.025,0.03,0.035,0.04,0.045,0.05,0.055,0.06,0.065,
0.07,0.075,0.08,0.085,0.09,0.095,0.1,0.105,0.11,0.115,0.12,0.125,0.13,0.135,
0.14,0.145,0.15,0.155,0.16,0.165,0.17,0.175,0.18,0.185,0.19,0.195,0.2,0.205,
0.21,0.215,0.22,0.225,0.23,0.235,0.24,0.245,0.25,0.255,0.26,0.265,0.27,
0.275,0.28,0.285,0.29,0.295,0.3,0.305,0.31,0.315,0.32,0.325,0.33,0.335,
0.34,0.345,0.35,0.355,0.36,0.365,0.37,0.375,0.38,0.385,0.39,0.395,0.4,0.405,
0.41,0.415,0.42,0.425,0.43,0.435,0.44,0.445,0.45,0.455,0.46,0.465,0.47,
0.475,0.48,0.485,0.49,0.495,0.5,0.505,0.51,0.515,0.52,0.525,0.53,0.535,
0.54,0.545,0.55,0.555,0.56,0.565,0.57,0.575,0.58,0.585,0.59,0.595,0.6,0.605,
0.61,0.615,0.62,0.625,0.63,0.635,0.64,0.645,0.65,0.655,0.66,0.665,0.67,
0.675,0.68,0.685,0.690000000000001,0.695000000000001,0.700000000000001,
0.705000000000001,0.710000000000001,0.715000000000001,0.720000000000001,
0.725000000000001,0.730000000000001,0.735000000000001,0.740000000000001,
0.745000000000001,0.750000000000001,0.755000000000001,0.760000000000001,
0.765000000000001,0.770000000000001,0.775000000000001,0.780000000000001,
0.785000000000001,0.790000000000001,0.795000000000001,0.800000000000001,
0.805000000000001,0.810000000000001,0.815000000000001,0.820000000000001,
0.825000000000001,0.830000000000001,0.835000000000001,0.840000000000001,
0.845000000000001,0.850000000000001,0.855000000000001,0.860000000000001,
0.865000000000001,0.870000000000001,0.875000000000001,0.880000000000001,
0.885000000000001,0.890000000000001,0.895000000000001,0.900000000000001,
0.905000000000001,0.910000000000001,0.915000000000001,0.920000000000001,
0.925000000000001,0.930000000000001,0.935000000000001,0.940000000000001,
0.945000000000001,0.950000000000001,0.955000000000001,0.960000000000001,
0.965000000000001,0.970000000000001,0.975000000000001,0.980000000000001,
0.985000000000001,0.990000000000001,0.995000000000001,1.),.UNSPECIFIED.)
CURVE()
GEOMETRIC_REPRESENTATION_ITEM()
RATIONAL_B_SPLINE_CURVE((1.,1.,1.,1.,1.,1.,1.,1.,1.,1.,1.,1.,1.,1.,1.,1.,
1.,1.,1.,1.,1.,1.,1.,1.,1.,1.,1.,1.,1.,1.,1.,1.,1.,1.,1.,1.,1.,1.,1.,1.,
1.,1.,1.,1.,1.,1.,1.,1.,1.,1.,1.,1.,1.,1.,1.,1.,1.,1.,1.,1.,1.,1.,1.,1.,
1.,1.,1.,1.,1.,1.,1.,1.,1.,1.,1.,1.,1.,1.,1.,1.,1.,1.,1.,1.,1.,1.,1.,1.,
1.,1.,1.,1.,1.,1.,1.,1.,1.,1.,1.,1.,1.,1.,1.,1.,1.,1.,1.,1.,1.,1.,1.,1.,
1.,1.,1.,1.,1.,1.,1.,1.,1.,1.,1.,1.,1.,1.,1.,1.,1.,1.,1.,1.,1.,1.,1.,1.,
1.,1.,1.,1.,1.,1.,1.,1.,1.,1.,1.,1.,1.,1.,1.,1.,1.,1.,1.,1.,1.,1.,1.,1.,
1.,1.,1.,1.,1.,1.,1.,1.,1.,1.,1.,1.,1.,1.,1.,1.,1.,1.,1.,1.,1.,1.,1.,1.,
1.,1.,1.,1.,1.,1.,1.,1.,1.,1.,1.,1.,1.,1.,1.,1.,1.,1.,1.,1.,1.))
REPRESENTATION_ITEM('')
);
#873=(
BOUNDED_CURVE()
B_SPLINE_CURVE(5,(#251934,#251935,#251936,#251937,#251938,#251939,#251940,
#251941,#251942,#251943,#251944,#251945,#251946,#251947,#251948,#251949,
#251950,#251951,#251952,#251953,#251954,#251955,#251956,#251957,#251958,
#251959,#251960,#251961,#251962,#251963,#251964,#251965,#251966,#251967,
#251968,#251969,#251970,#251971,#251972,#251973,#251974,#251975,#251976,
#251977,#251978,#251979,#251980,#251981,#251982,#251983,#251984,#251985,
#251986,#251987,#251988,#251989,#251990,#251991,#251992,#251993,#251994,
#251995,#251996,#251997,#251998,#251999,#252000,#252001,#252002,#252003,
#252004,#252005,#252006,#252007,#252008,#252009,#252010,#252011,#252012,
#252013,#252014,#252015,#252016,#252017,#252018,#252019,#252020,#252021,
#252022,#252023,#252024,#252025,#252026,#252027,#252028,#252029,#252030,
#252031,#252032,#252033,#252034,#252035,#252036,#252037,#252038,#252039,
#252040,#252041,#252042,#252043,#252044,#252045,#252046,#252047,#252048,
#252049,#252050,#252051,#252052,#252053,#252054,#252055,#252056,#252057,
#252058,#252059,#252060,#252061,#252062,#252063,#252064,#252065,#252066,
#252067,#252068,#252069,#252070,#252071,#252072,#252073,#252074,#252075,
#252076,#252077,#252078,#252079,#252080,#252081,#252082,#252083,#252084,
#252085,#252086,#252087,#252088,#252089,#252090,#252091,#252092,#252093,
#252094,#252095,#252096,#252097,#252098,#252099,#252100,#252101,#252102,
#252103,#252104,#252105,#252106,#252107,#252108,#252109,#252110,#252111,
#252112,#252113,#252114,#252115,#252116,#252117,#252118,#252119,#252120,
#252121,#252122,#252123,#252124,#252125,#252126,#252127,#252128,#252129,
#252130,#252131,#252132,#252133,#252134,#252135,#252136,#252137,#252138),
 .UNSPECIFIED.,.F.,.F.)
B_SPLINE_CURVE_WITH_KNOTS((6,1,1,1,1,1,1,1,1,1,1,1,1,1,1,1,1,1,1,1,1,1,
1,1,1,1,1,1,1,1,1,1,1,1,1,1,1,1,1,1,1,1,1,1,1,1,1,1,1,1,1,1,1,1,1,1,1,1,
1,1,1,1,1,1,1,1,1,1,1,1,1,1,1,1,1,1,1,1,1,1,1,1,1,1,1,1,1,1,1,1,1,1,1,1,
1,1,1,1,1,1,1,1,1,1,1,1,1,1,1,1,1,1,1,1,1,1,1,1,1,1,1,1,1,1,1,1,1,1,1,1,
1,1,1,1,1,1,1,1,1,1,1,1,1,1,1,1,1,1,1,1,1,1,1,1,1,1,1,1,1,1,1,1,1,1,1,1,
1,1,1,1,1,1,1,1,1,1,1,1,1,1,1,1,1,1,1,1,1,1,1,1,1,1,1,1,1,1,1,1,1,1,6),
(0.,0.005,0.01,0.015,0.02,0.025,0.03,0.035,0.04,0.045,0.05,0.055,0.06,0.065,
0.07,0.075,0.08,0.085,0.09,0.095,0.1,0.105,0.11,0.115,0.12,0.125,0.13,0.135,
0.14,0.145,0.15,0.155,0.16,0.165,0.17,0.175,0.18,0.185,0.19,0.195,0.2,0.205,
0.21,0.215,0.22,0.225,0.23,0.235,0.24,0.245,0.25,0.255,0.26,0.265,0.27,
0.275,0.28,0.285,0.29,0.295,0.3,0.305,0.31,0.315,0.32,0.325,0.33,0.335,
0.34,0.345,0.35,0.355,0.36,0.365,0.37,0.375,0.38,0.385,0.39,0.395,0.4,0.405,
0.41,0.415,0.42,0.425,0.43,0.435,0.44,0.445,0.45,0.455,0.46,0.465,0.47,
0.475,0.48,0.485,0.49,0.495,0.5,0.505,0.51,0.515,0.52,0.525,0.53,0.535,
0.54,0.545,0.55,0.555,0.56,0.565,0.57,0.575,0.58,0.585,0.59,0.595,0.6,0.605,
0.61,0.615,0.62,0.625,0.63,0.635,0.64,0.645,0.65,0.655,0.66,0.665,0.67,
0.675,0.68,0.685,0.690000000000001,0.695000000000001,0.700000000000001,
0.705000000000001,0.710000000000001,0.715000000000001,0.720000000000001,
0.725000000000001,0.730000000000001,0.735000000000001,0.740000000000001,
0.745000000000001,0.750000000000001,0.755000000000001,0.760000000000001,
0.765000000000001,0.770000000000001,0.775000000000001,0.780000000000001,
0.785000000000001,0.790000000000001,0.795000000000001,0.800000000000001,
0.805000000000001,0.810000000000001,0.815000000000001,0.820000000000001,
0.825000000000001,0.830000000000001,0.835000000000001,0.840000000000001,
0.845000000000001,0.850000000000001,0.855000000000001,0.860000000000001,
0.865000000000001,0.870000000000001,0.875000000000001,0.880000000000001,
0.885000000000001,0.890000000000001,0.895000000000001,0.900000000000001,
0.905000000000001,0.910000000000001,0.915000000000001,0.920000000000001,
0.925000000000001,0.930000000000001,0.935000000000001,0.940000000000001,
0.945000000000001,0.950000000000001,0.955000000000001,0.960000000000001,
0.965000000000001,0.970000000000001,0.975000000000001,0.980000000000001,
0.985000000000001,0.990000000000001,0.995000000000001,1.),.UNSPECIFIED.)
CURVE()
GEOMETRIC_REPRESENTATION_ITEM()
RATIONAL_B_SPLINE_CURVE((1.,1.,1.,1.,1.,1.,1.,1.,1.,1.,1.,1.,1.,1.,1.,1.,
1.,1.,1.,1.,1.,1.,1.,1.,1.,1.,1.,1.,1.,1.,1.,1.,1.,1.,1.,1.,1.,1.,1.,1.,
1.,1.,1.,1.,1.,1.,1.,1.,1.,1.,1.,1.,1.,1.,1.,1.,1.,1.,1.,1.,1.,1.,1.,1.,
1.,1.,1.,1.,1.,1.,1.,1.,1.,1.,1.,1.,1.,1.,1.,1.,1.,1.,1.,1.,1.,1.,1.,1.,
1.,1.,1.,1.,1.,1.,1.,1.,1.,1.,1.,1.,1.,1.,1.,1.,1.,1.,1.,1.,1.,1.,1.,1.,
1.,1.,1.,1.,1.,1.,1.,1.,1.,1.,1.,1.,1.,1.,1.,1.,1.,1.,1.,1.,1.,1.,1.,1.,
1.,1.,1.,1.,1.,1.,1.,1.,1.,1.,1.,1.,1.,1.,1.,1.,1.,1.,1.,1.,1.,1.,1.,1.,
1.,1.,1.,1.,1.,1.,1.,1.,1.,1.,1.,1.,1.,1.,1.,1.,1.,1.,1.,1.,1.,1.,1.,1.,
1.,1.,1.,1.,1.,1.,1.,1.,1.,1.,1.,1.,1.,1.,1.,1.,1.,1.,1.,1.,1.))
REPRESENTATION_ITEM('')
);
#874=(
BOUNDED_CURVE()
B_SPLINE_CURVE(5,(#252140,#252141,#252142,#252143,#252144,#252145,#252146,
#252147,#252148,#252149,#252150,#252151,#252152,#252153,#252154,#252155,
#252156,#252157,#252158,#252159,#252160,#252161,#252162,#252163,#252164,
#252165,#252166,#252167,#252168,#252169,#252170,#252171,#252172,#252173,
#252174,#252175,#252176,#252177,#252178,#252179,#252180,#252181,#252182,
#252183,#252184,#252185,#252186,#252187,#252188,#252189,#252190,#252191,
#252192,#252193,#252194,#252195,#252196,#252197,#252198,#252199,#252200,
#252201,#252202,#252203,#252204,#252205,#252206,#252207,#252208,#252209,
#252210,#252211,#252212,#252213,#252214,#252215,#252216,#252217,#252218,
#252219,#252220,#252221,#252222,#252223,#252224,#252225,#252226,#252227,
#252228,#252229,#252230,#252231,#252232,#252233,#252234,#252235,#252236,
#252237,#252238,#252239,#252240,#252241,#252242,#252243,#252244,#252245,
#252246,#252247,#252248,#252249,#252250,#252251,#252252,#252253,#252254,
#252255,#252256,#252257,#252258,#252259,#252260,#252261,#252262,#252263,
#252264,#252265,#252266,#252267,#252268,#252269,#252270,#252271,#252272,
#252273,#252274,#252275,#252276,#252277,#252278,#252279,#252280,#252281,
#252282,#252283,#252284,#252285,#252286,#252287,#252288,#252289,#252290,
#252291,#252292,#252293,#252294,#252295,#252296,#252297,#252298,#252299,
#252300,#252301,#252302,#252303,#252304,#252305,#252306,#252307,#252308,
#252309,#252310,#252311,#252312,#252313,#252314,#252315,#252316,#252317,
#252318,#252319,#252320,#252321,#252322,#252323,#252324,#252325,#252326,
#252327,#252328,#252329,#252330,#252331,#252332,#252333,#252334,#252335,
#252336,#252337,#252338,#252339,#252340,#252341,#252342,#252343,#252344),
 .UNSPECIFIED.,.F.,.F.)
B_SPLINE_CURVE_WITH_KNOTS((6,1,1,1,1,1,1,1,1,1,1,1,1,1,1,1,1,1,1,1,1,1,
1,1,1,1,1,1,1,1,1,1,1,1,1,1,1,1,1,1,1,1,1,1,1,1,1,1,1,1,1,1,1,1,1,1,1,1,
1,1,1,1,1,1,1,1,1,1,1,1,1,1,1,1,1,1,1,1,1,1,1,1,1,1,1,1,1,1,1,1,1,1,1,1,
1,1,1,1,1,1,1,1,1,1,1,1,1,1,1,1,1,1,1,1,1,1,1,1,1,1,1,1,1,1,1,1,1,1,1,1,
1,1,1,1,1,1,1,1,1,1,1,1,1,1,1,1,1,1,1,1,1,1,1,1,1,1,1,1,1,1,1,1,1,1,1,1,
1,1,1,1,1,1,1,1,1,1,1,1,1,1,1,1,1,1,1,1,1,1,1,1,1,1,1,1,1,1,1,1,1,1,6),
(-1.,-0.995000000000001,-0.990000000000001,-0.985000000000001,-0.980000000000001,
-0.975000000000001,-0.970000000000001,-0.965000000000001,-0.960000000000001,
-0.955000000000001,-0.950000000000001,-0.945000000000001,-0.940000000000001,
-0.935000000000001,-0.930000000000001,-0.925000000000001,-0.920000000000001,
-0.915000000000001,-0.910000000000001,-0.905000000000001,-0.900000000000001,
-0.895000000000001,-0.890000000000001,-0.885000000000001,-0.880000000000001,
-0.875000000000001,-0.870000000000001,-0.865000000000001,-0.860000000000001,
-0.855000000000001,-0.850000000000001,-0.845000000000001,-0.840000000000001,
-0.835000000000001,-0.830000000000001,-0.825000000000001,-0.820000000000001,
-0.815000000000001,-0.810000000000001,-0.805000000000001,-0.800000000000001,
-0.795000000000001,-0.790000000000001,-0.785000000000001,-0.780000000000001,
-0.775000000000001,-0.770000000000001,-0.765000000000001,-0.760000000000001,
-0.755000000000001,-0.750000000000001,-0.745000000000001,-0.740000000000001,
-0.735000000000001,-0.730000000000001,-0.725000000000001,-0.720000000000001,
-0.715000000000001,-0.710000000000001,-0.705000000000001,-0.700000000000001,
-0.695000000000001,-0.690000000000001,-0.685,-0.68,-0.675,-0.67,-0.665,
-0.66,-0.655,-0.65,-0.645,-0.64,-0.635,-0.63,-0.625,-0.62,-0.615,-0.61,
-0.605,-0.6,-0.595,-0.59,-0.585,-0.58,-0.575,-0.57,-0.565,-0.56,-0.555,
-0.55,-0.545,-0.54,-0.535,-0.53,-0.525,-0.52,-0.515,-0.51,-0.505,-0.5,-0.495,
-0.49,-0.485,-0.48,-0.475,-0.47,-0.465,-0.46,-0.455,-0.45,-0.445,-0.44,
-0.435,-0.43,-0.425,-0.42,-0.415,-0.41,-0.405,-0.4,-0.395,-0.39,-0.385,
-0.38,-0.375,-0.37,-0.365,-0.36,-0.355,-0.35,-0.345,-0.34,-0.335,-0.33,
-0.325,-0.32,-0.315,-0.31,-0.305,-0.3,-0.295,-0.29,-0.285,-0.28,-0.275,
-0.27,-0.265,-0.26,-0.255,-0.25,-0.245,-0.24,-0.235,-0.23,-0.225,-0.22,
-0.215,-0.21,-0.205,-0.2,-0.195,-0.19,-0.185,-0.18,-0.175,-0.17,-0.165,
-0.16,-0.155,-0.15,-0.145,-0.14,-0.135,-0.13,-0.125,-0.12,-0.115,-0.11,
-0.105,-0.1,-0.095,-0.09,-0.085,-0.08,-0.075,-0.07,-0.065,-0.06,-0.055,
-0.05,-0.045,-0.04,-0.035,-0.03,-0.025,-0.02,-0.015,-0.01,-0.005,0.),
 .UNSPECIFIED.)
CURVE()
GEOMETRIC_REPRESENTATION_ITEM()
RATIONAL_B_SPLINE_CURVE((1.,1.,1.,1.,1.,1.,1.,1.,1.,1.,1.,1.,1.,1.,1.,1.,
1.,1.,1.,1.,1.,1.,1.,1.,1.,1.,1.,1.,1.,1.,1.,1.,1.,1.,1.,1.,1.,1.,1.,1.,
1.,1.,1.,1.,1.,1.,1.,1.,1.,1.,1.,1.,1.,1.,1.,1.,1.,1.,1.,1.,1.,1.,1.,1.,
1.,1.,1.,1.,1.,1.,1.,1.,1.,1.,1.,1.,1.,1.,1.,1.,1.,1.,1.,1.,1.,1.,1.,1.,
1.,1.,1.,1.,1.,1.,1.,1.,1.,1.,1.,1.,1.,1.,1.,1.,1.,1.,1.,1.,1.,1.,1.,1.,
1.,1.,1.,1.,1.,1.,1.,1.,1.,1.,1.,1.,1.,1.,1.,1.,1.,1.,1.,1.,1.,1.,1.,1.,
1.,1.,1.,1.,1.,1.,1.,1.,1.,1.,1.,1.,1.,1.,1.,1.,1.,1.,1.,1.,1.,1.,1.,1.,
1.,1.,1.,1.,1.,1.,1.,1.,1.,1.,1.,1.,1.,1.,1.,1.,1.,1.,1.,1.,1.,1.,1.,1.,
1.,1.,1.,1.,1.,1.,1.,1.,1.,1.,1.,1.,1.,1.,1.,1.,1.,1.,1.,1.,1.))
REPRESENTATION_ITEM('')
);
#875=(
BOUNDED_CURVE()
B_SPLINE_CURVE(5,(#252763,#252764,#252765,#252766,#252767,#252768,#252769,
#252770,#252771,#252772,#252773,#252774,#252775,#252776,#252777,#252778,
#252779,#252780,#252781,#252782,#252783,#252784,#252785,#252786,#252787,
#252788,#252789,#252790,#252791,#252792,#252793,#252794,#252795,#252796,
#252797,#252798,#252799,#252800,#252801,#252802,#252803,#252804,#252805,
#252806,#252807,#252808,#252809,#252810,#252811,#252812,#252813,#252814,
#252815,#252816,#252817,#252818,#252819,#252820,#252821,#252822,#252823,
#252824,#252825,#252826,#252827,#252828,#252829,#252830,#252831,#252832,
#252833,#252834,#252835,#252836,#252837,#252838,#252839,#252840,#252841,
#252842,#252843,#252844,#252845,#252846,#252847,#252848,#252849,#252850,
#252851,#252852,#252853,#252854,#252855,#252856,#252857,#252858,#252859,
#252860,#252861,#252862,#252863,#252864,#252865,#252866,#252867,#252868,
#252869,#252870,#252871,#252872,#252873,#252874,#252875,#252876,#252877,
#252878,#252879,#252880,#252881,#252882,#252883,#252884,#252885,#252886,
#252887,#252888,#252889,#252890,#252891,#252892,#252893,#252894,#252895,
#252896,#252897,#252898,#252899,#252900,#252901,#252902,#252903,#252904,
#252905,#252906,#252907,#252908,#252909,#252910,#252911,#252912,#252913,
#252914,#252915,#252916,#252917,#252918,#252919,#252920,#252921,#252922,
#252923,#252924,#252925,#252926,#252927,#252928,#252929,#252930,#252931,
#252932,#252933,#252934,#252935,#252936,#252937,#252938,#252939,#252940,
#252941,#252942,#252943,#252944,#252945,#252946,#252947,#252948,#252949,
#252950,#252951,#252952,#252953,#252954,#252955,#252956,#252957,#252958,
#252959,#252960,#252961,#252962,#252963,#252964,#252965,#252966,#252967),
 .UNSPECIFIED.,.F.,.F.)
B_SPLINE_CURVE_WITH_KNOTS((6,1,1,1,1,1,1,1,1,1,1,1,1,1,1,1,1,1,1,1,1,1,
1,1,1,1,1,1,1,1,1,1,1,1,1,1,1,1,1,1,1,1,1,1,1,1,1,1,1,1,1,1,1,1,1,1,1,1,
1,1,1,1,1,1,1,1,1,1,1,1,1,1,1,1,1,1,1,1,1,1,1,1,1,1,1,1,1,1,1,1,1,1,1,1,
1,1,1,1,1,1,1,1,1,1,1,1,1,1,1,1,1,1,1,1,1,1,1,1,1,1,1,1,1,1,1,1,1,1,1,1,
1,1,1,1,1,1,1,1,1,1,1,1,1,1,1,1,1,1,1,1,1,1,1,1,1,1,1,1,1,1,1,1,1,1,1,1,
1,1,1,1,1,1,1,1,1,1,1,1,1,1,1,1,1,1,1,1,1,1,1,1,1,1,1,1,1,1,1,1,1,1,6),
(-1.,-0.995000000000001,-0.990000000000001,-0.985000000000001,-0.980000000000001,
-0.975000000000001,-0.970000000000001,-0.965000000000001,-0.960000000000001,
-0.955000000000001,-0.950000000000001,-0.945000000000001,-0.940000000000001,
-0.935000000000001,-0.930000000000001,-0.925000000000001,-0.920000000000001,
-0.915000000000001,-0.910000000000001,-0.905000000000001,-0.900000000000001,
-0.895000000000001,-0.890000000000001,-0.885000000000001,-0.880000000000001,
-0.875000000000001,-0.870000000000001,-0.865000000000001,-0.860000000000001,
-0.855000000000001,-0.850000000000001,-0.845000000000001,-0.840000000000001,
-0.835000000000001,-0.830000000000001,-0.825000000000001,-0.820000000000001,
-0.815000000000001,-0.810000000000001,-0.805000000000001,-0.800000000000001,
-0.795000000000001,-0.790000000000001,-0.785000000000001,-0.780000000000001,
-0.775000000000001,-0.770000000000001,-0.765000000000001,-0.760000000000001,
-0.755000000000001,-0.750000000000001,-0.745000000000001,-0.740000000000001,
-0.735000000000001,-0.730000000000001,-0.725000000000001,-0.720000000000001,
-0.715000000000001,-0.710000000000001,-0.705000000000001,-0.700000000000001,
-0.695000000000001,-0.690000000000001,-0.685,-0.68,-0.675,-0.67,-0.665,
-0.66,-0.655,-0.65,-0.645,-0.64,-0.635,-0.63,-0.625,-0.62,-0.615,-0.61,
-0.605,-0.6,-0.595,-0.59,-0.585,-0.58,-0.575,-0.57,-0.565,-0.56,-0.555,
-0.55,-0.545,-0.54,-0.535,-0.53,-0.525,-0.52,-0.515,-0.51,-0.505,-0.5,-0.495,
-0.49,-0.485,-0.48,-0.475,-0.47,-0.465,-0.46,-0.455,-0.45,-0.445,-0.44,
-0.435,-0.43,-0.425,-0.42,-0.415,-0.41,-0.405,-0.4,-0.395,-0.39,-0.385,
-0.38,-0.375,-0.37,-0.365,-0.36,-0.355,-0.35,-0.345,-0.34,-0.335,-0.33,
-0.325,-0.32,-0.315,-0.31,-0.305,-0.3,-0.295,-0.29,-0.285,-0.28,-0.275,
-0.27,-0.265,-0.26,-0.255,-0.25,-0.245,-0.24,-0.235,-0.23,-0.225,-0.22,
-0.215,-0.21,-0.205,-0.2,-0.195,-0.19,-0.185,-0.18,-0.175,-0.17,-0.165,
-0.16,-0.155,-0.15,-0.145,-0.14,-0.135,-0.13,-0.125,-0.12,-0.115,-0.11,
-0.105,-0.1,-0.095,-0.09,-0.085,-0.08,-0.075,-0.07,-0.065,-0.06,-0.055,
-0.05,-0.045,-0.04,-0.035,-0.03,-0.025,-0.02,-0.015,-0.01,-0.005,0.),
 .UNSPECIFIED.)
CURVE()
GEOMETRIC_REPRESENTATION_ITEM()
RATIONAL_B_SPLINE_CURVE((1.,1.,1.,1.,1.,1.,1.,1.,1.,1.,1.,1.,1.,1.,1.,1.,
1.,1.,1.,1.,1.,1.,1.,1.,1.,1.,1.,1.,1.,1.,1.,1.,1.,1.,1.,1.,1.,1.,1.,1.,
1.,1.,1.,1.,1.,1.,1.,1.,1.,1.,1.,1.,1.,1.,1.,1.,1.,1.,1.,1.,1.,1.,1.,1.,
1.,1.,1.,1.,1.,1.,1.,1.,1.,1.,1.,1.,1.,1.,1.,1.,1.,1.,1.,1.,1.,1.,1.,1.,
1.,1.,1.,1.,1.,1.,1.,1.,1.,1.,1.,1.,1.,1.,1.,1.,1.,1.,1.,1.,1.,1.,1.,1.,
1.,1.,1.,1.,1.,1.,1.,1.,1.,1.,1.,1.,1.,1.,1.,1.,1.,1.,1.,1.,1.,1.,1.,1.,
1.,1.,1.,1.,1.,1.,1.,1.,1.,1.,1.,1.,1.,1.,1.,1.,1.,1.,1.,1.,1.,1.,1.,1.,
1.,1.,1.,1.,1.,1.,1.,1.,1.,1.,1.,1.,1.,1.,1.,1.,1.,1.,1.,1.,1.,1.,1.,1.,
1.,1.,1.,1.,1.,1.,1.,1.,1.,1.,1.,1.,1.,1.,1.,1.,1.,1.,1.,1.,1.))
REPRESENTATION_ITEM('')
);
#876=(
BOUNDED_CURVE()
B_SPLINE_CURVE(5,(#252970,#252971,#252972,#252973,#252974,#252975,#252976,
#252977,#252978,#252979,#252980,#252981,#252982,#252983,#252984,#252985,
#252986,#252987,#252988,#252989,#252990,#252991,#252992,#252993,#252994,
#252995,#252996,#252997,#252998,#252999,#253000,#253001,#253002,#253003,
#253004,#253005,#253006,#253007,#253008,#253009,#253010,#253011,#253012,
#253013,#253014,#253015,#253016,#253017,#253018,#253019,#253020,#253021,
#253022,#253023,#253024,#253025,#253026,#253027,#253028,#253029,#253030,
#253031,#253032,#253033,#253034,#253035,#253036,#253037,#253038,#253039,
#253040,#253041,#253042,#253043,#253044,#253045,#253046,#253047,#253048,
#253049,#253050,#253051,#253052,#253053,#253054,#253055,#253056,#253057,
#253058,#253059,#253060,#253061,#253062,#253063,#253064,#253065,#253066,
#253067,#253068,#253069,#253070,#253071,#253072,#253073,#253074,#253075,
#253076,#253077,#253078,#253079,#253080,#253081,#253082,#253083,#253084,
#253085,#253086,#253087,#253088,#253089,#253090,#253091,#253092,#253093,
#253094,#253095,#253096,#253097,#253098,#253099,#253100,#253101,#253102,
#253103,#253104,#253105,#253106,#253107,#253108,#253109,#253110,#253111,
#253112,#253113,#253114,#253115,#253116,#253117,#253118,#253119,#253120,
#253121,#253122,#253123,#253124,#253125,#253126,#253127,#253128,#253129,
#253130,#253131,#253132,#253133,#253134,#253135,#253136,#253137,#253138,
#253139,#253140,#253141,#253142,#253143,#253144,#253145,#253146,#253147,
#253148,#253149,#253150,#253151,#253152,#253153,#253154,#253155,#253156,
#253157,#253158,#253159,#253160,#253161,#253162,#253163,#253164,#253165,
#253166,#253167,#253168,#253169,#253170,#253171,#253172,#253173,#253174),
 .UNSPECIFIED.,.F.,.F.)
B_SPLINE_CURVE_WITH_KNOTS((6,1,1,1,1,1,1,1,1,1,1,1,1,1,1,1,1,1,1,1,1,1,
1,1,1,1,1,1,1,1,1,1,1,1,1,1,1,1,1,1,1,1,1,1,1,1,1,1,1,1,1,1,1,1,1,1,1,1,
1,1,1,1,1,1,1,1,1,1,1,1,1,1,1,1,1,1,1,1,1,1,1,1,1,1,1,1,1,1,1,1,1,1,1,1,
1,1,1,1,1,1,1,1,1,1,1,1,1,1,1,1,1,1,1,1,1,1,1,1,1,1,1,1,1,1,1,1,1,1,1,1,
1,1,1,1,1,1,1,1,1,1,1,1,1,1,1,1,1,1,1,1,1,1,1,1,1,1,1,1,1,1,1,1,1,1,1,1,
1,1,1,1,1,1,1,1,1,1,1,1,1,1,1,1,1,1,1,1,1,1,1,1,1,1,1,1,1,1,1,1,1,1,6),
(0.,0.005,0.01,0.015,0.02,0.025,0.03,0.035,0.04,0.045,0.05,0.055,0.06,0.065,
0.07,0.075,0.08,0.085,0.09,0.095,0.1,0.105,0.11,0.115,0.12,0.125,0.13,0.135,
0.14,0.145,0.15,0.155,0.16,0.165,0.17,0.175,0.18,0.185,0.19,0.195,0.2,0.205,
0.21,0.215,0.22,0.225,0.23,0.235,0.24,0.245,0.25,0.255,0.26,0.265,0.27,
0.275,0.28,0.285,0.29,0.295,0.3,0.305,0.31,0.315,0.32,0.325,0.33,0.335,
0.34,0.345,0.35,0.355,0.36,0.365,0.37,0.375,0.38,0.385,0.39,0.395,0.4,0.405,
0.41,0.415,0.42,0.425,0.43,0.435,0.44,0.445,0.45,0.455,0.46,0.465,0.47,
0.475,0.48,0.485,0.49,0.495,0.5,0.505,0.51,0.515,0.52,0.525,0.53,0.535,
0.54,0.545,0.55,0.555,0.56,0.565,0.57,0.575,0.58,0.585,0.59,0.595,0.6,0.605,
0.61,0.615,0.62,0.625,0.63,0.635,0.64,0.645,0.65,0.655,0.66,0.665,0.67,
0.675,0.68,0.685,0.690000000000001,0.695000000000001,0.700000000000001,
0.705000000000001,0.710000000000001,0.715000000000001,0.720000000000001,
0.725000000000001,0.730000000000001,0.735000000000001,0.740000000000001,
0.745000000000001,0.750000000000001,0.755000000000001,0.760000000000001,
0.765000000000001,0.770000000000001,0.775000000000001,0.780000000000001,
0.785000000000001,0.790000000000001,0.795000000000001,0.800000000000001,
0.805000000000001,0.810000000000001,0.815000000000001,0.820000000000001,
0.825000000000001,0.830000000000001,0.835000000000001,0.840000000000001,
0.845000000000001,0.850000000000001,0.855000000000001,0.860000000000001,
0.865000000000001,0.870000000000001,0.875000000000001,0.880000000000001,
0.885000000000001,0.890000000000001,0.895000000000001,0.900000000000001,
0.905000000000001,0.910000000000001,0.915000000000001,0.920000000000001,
0.925000000000001,0.930000000000001,0.935000000000001,0.940000000000001,
0.945000000000001,0.950000000000001,0.955000000000001,0.960000000000001,
0.965000000000001,0.970000000000001,0.975000000000001,0.980000000000001,
0.985000000000001,0.990000000000001,0.995000000000001,1.),.UNSPECIFIED.)
CURVE()
GEOMETRIC_REPRESENTATION_ITEM()
RATIONAL_B_SPLINE_CURVE((1.,1.,1.,1.,1.,1.,1.,1.,1.,1.,1.,1.,1.,1.,1.,1.,
1.,1.,1.,1.,1.,1.,1.,1.,1.,1.,1.,1.,1.,1.,1.,1.,1.,1.,1.,1.,1.,1.,1.,1.,
1.,1.,1.,1.,1.,1.,1.,1.,1.,1.,1.,1.,1.,1.,1.,1.,1.,1.,1.,1.,1.,1.,1.,1.,
1.,1.,1.,1.,1.,1.,1.,1.,1.,1.,1.,1.,1.,1.,1.,1.,1.,1.,1.,1.,1.,1.,1.,1.,
1.,1.,1.,1.,1.,1.,1.,1.,1.,1.,1.,1.,1.,1.,1.,1.,1.,1.,1.,1.,1.,1.,1.,1.,
1.,1.,1.,1.,1.,1.,1.,1.,1.,1.,1.,1.,1.,1.,1.,1.,1.,1.,1.,1.,1.,1.,1.,1.,
1.,1.,1.,1.,1.,1.,1.,1.,1.,1.,1.,1.,1.,1.,1.,1.,1.,1.,1.,1.,1.,1.,1.,1.,
1.,1.,1.,1.,1.,1.,1.,1.,1.,1.,1.,1.,1.,1.,1.,1.,1.,1.,1.,1.,1.,1.,1.,1.,
1.,1.,1.,1.,1.,1.,1.,1.,1.,1.,1.,1.,1.,1.,1.,1.,1.,1.,1.,1.,1.))
REPRESENTATION_ITEM('')
);
#877=(
BOUNDED_CURVE()
B_SPLINE_CURVE(5,(#253586,#253587,#253588,#253589,#253590,#253591,#253592,
#253593,#253594,#253595,#253596,#253597,#253598,#253599,#253600,#253601,
#253602,#253603,#253604,#253605,#253606,#253607,#253608,#253609,#253610,
#253611,#253612,#253613,#253614,#253615,#253616,#253617,#253618,#253619,
#253620,#253621,#253622,#253623,#253624,#253625,#253626,#253627,#253628,
#253629,#253630,#253631,#253632,#253633,#253634,#253635,#253636,#253637,
#253638,#253639,#253640,#253641,#253642,#253643,#253644,#253645,#253646,
#253647,#253648,#253649,#253650,#253651,#253652,#253653,#253654,#253655,
#253656,#253657,#253658,#253659,#253660,#253661,#253662,#253663,#253664,
#253665,#253666,#253667,#253668,#253669,#253670,#253671,#253672,#253673,
#253674,#253675,#253676,#253677,#253678,#253679,#253680,#253681,#253682,
#253683,#253684,#253685,#253686,#253687,#253688,#253689,#253690,#253691,
#253692,#253693,#253694,#253695,#253696,#253697,#253698,#253699,#253700,
#253701,#253702,#253703,#253704,#253705,#253706,#253707,#253708,#253709,
#253710,#253711,#253712,#253713,#253714,#253715,#253716,#253717,#253718,
#253719,#253720,#253721,#253722,#253723,#253724,#253725,#253726,#253727,
#253728,#253729,#253730,#253731,#253732,#253733,#253734,#253735,#253736,
#253737,#253738,#253739,#253740,#253741,#253742,#253743,#253744,#253745,
#253746,#253747,#253748,#253749,#253750,#253751,#253752,#253753,#253754,
#253755,#253756,#253757,#253758,#253759,#253760,#253761,#253762,#253763,
#253764,#253765,#253766,#253767,#253768,#253769,#253770,#253771,#253772,
#253773,#253774,#253775,#253776,#253777,#253778,#253779,#253780,#253781,
#253782,#253783,#253784,#253785,#253786,#253787,#253788,#253789,#253790),
 .UNSPECIFIED.,.F.,.F.)
B_SPLINE_CURVE_WITH_KNOTS((6,1,1,1,1,1,1,1,1,1,1,1,1,1,1,1,1,1,1,1,1,1,
1,1,1,1,1,1,1,1,1,1,1,1,1,1,1,1,1,1,1,1,1,1,1,1,1,1,1,1,1,1,1,1,1,1,1,1,
1,1,1,1,1,1,1,1,1,1,1,1,1,1,1,1,1,1,1,1,1,1,1,1,1,1,1,1,1,1,1,1,1,1,1,1,
1,1,1,1,1,1,1,1,1,1,1,1,1,1,1,1,1,1,1,1,1,1,1,1,1,1,1,1,1,1,1,1,1,1,1,1,
1,1,1,1,1,1,1,1,1,1,1,1,1,1,1,1,1,1,1,1,1,1,1,1,1,1,1,1,1,1,1,1,1,1,1,1,
1,1,1,1,1,1,1,1,1,1,1,1,1,1,1,1,1,1,1,1,1,1,1,1,1,1,1,1,1,1,1,1,1,1,6),
(0.,0.005,0.01,0.015,0.02,0.025,0.03,0.035,0.04,0.045,0.05,0.055,0.06,0.065,
0.07,0.075,0.08,0.085,0.09,0.095,0.1,0.105,0.11,0.115,0.12,0.125,0.13,0.135,
0.14,0.145,0.15,0.155,0.16,0.165,0.17,0.175,0.18,0.185,0.19,0.195,0.2,0.205,
0.21,0.215,0.22,0.225,0.23,0.235,0.24,0.245,0.25,0.255,0.26,0.265,0.27,
0.275,0.28,0.285,0.29,0.295,0.3,0.305,0.31,0.315,0.32,0.325,0.33,0.335,
0.34,0.345,0.35,0.355,0.36,0.365,0.37,0.375,0.38,0.385,0.39,0.395,0.4,0.405,
0.41,0.415,0.42,0.425,0.43,0.435,0.44,0.445,0.45,0.455,0.46,0.465,0.47,
0.475,0.48,0.485,0.49,0.495,0.5,0.505,0.51,0.515,0.52,0.525,0.53,0.535,
0.54,0.545,0.55,0.555,0.56,0.565,0.57,0.575,0.58,0.585,0.59,0.595,0.6,0.605,
0.61,0.615,0.62,0.625,0.63,0.635,0.64,0.645,0.65,0.655,0.66,0.665,0.67,
0.675,0.68,0.685,0.690000000000001,0.695000000000001,0.700000000000001,
0.705000000000001,0.710000000000001,0.715000000000001,0.720000000000001,
0.725000000000001,0.730000000000001,0.735000000000001,0.740000000000001,
0.745000000000001,0.750000000000001,0.755000000000001,0.760000000000001,
0.765000000000001,0.770000000000001,0.775000000000001,0.780000000000001,
0.785000000000001,0.790000000000001,0.795000000000001,0.800000000000001,
0.805000000000001,0.810000000000001,0.815000000000001,0.820000000000001,
0.825000000000001,0.830000000000001,0.835000000000001,0.840000000000001,
0.845000000000001,0.850000000000001,0.855000000000001,0.860000000000001,
0.865000000000001,0.870000000000001,0.875000000000001,0.880000000000001,
0.885000000000001,0.890000000000001,0.895000000000001,0.900000000000001,
0.905000000000001,0.910000000000001,0.915000000000001,0.920000000000001,
0.925000000000001,0.930000000000001,0.935000000000001,0.940000000000001,
0.945000000000001,0.950000000000001,0.955000000000001,0.960000000000001,
0.965000000000001,0.970000000000001,0.975000000000001,0.980000000000001,
0.985000000000001,0.990000000000001,0.995000000000001,1.),.UNSPECIFIED.)
CURVE()
GEOMETRIC_REPRESENTATION_ITEM()
RATIONAL_B_SPLINE_CURVE((1.,1.,1.,1.,1.,1.,1.,1.,1.,1.,1.,1.,1.,1.,1.,1.,
1.,1.,1.,1.,1.,1.,1.,1.,1.,1.,1.,1.,1.,1.,1.,1.,1.,1.,1.,1.,1.,1.,1.,1.,
1.,1.,1.,1.,1.,1.,1.,1.,1.,1.,1.,1.,1.,1.,1.,1.,1.,1.,1.,1.,1.,1.,1.,1.,
1.,1.,1.,1.,1.,1.,1.,1.,1.,1.,1.,1.,1.,1.,1.,1.,1.,1.,1.,1.,1.,1.,1.,1.,
1.,1.,1.,1.,1.,1.,1.,1.,1.,1.,1.,1.,1.,1.,1.,1.,1.,1.,1.,1.,1.,1.,1.,1.,
1.,1.,1.,1.,1.,1.,1.,1.,1.,1.,1.,1.,1.,1.,1.,1.,1.,1.,1.,1.,1.,1.,1.,1.,
1.,1.,1.,1.,1.,1.,1.,1.,1.,1.,1.,1.,1.,1.,1.,1.,1.,1.,1.,1.,1.,1.,1.,1.,
1.,1.,1.,1.,1.,1.,1.,1.,1.,1.,1.,1.,1.,1.,1.,1.,1.,1.,1.,1.,1.,1.,1.,1.,
1.,1.,1.,1.,1.,1.,1.,1.,1.,1.,1.,1.,1.,1.,1.,1.,1.,1.,1.,1.,1.))
REPRESENTATION_ITEM('')
);
#878=(
BOUNDED_CURVE()
B_SPLINE_CURVE(5,(#253792,#253793,#253794,#253795,#253796,#253797,#253798,
#253799,#253800,#253801,#253802,#253803,#253804,#253805,#253806,#253807,
#253808,#253809,#253810,#253811,#253812,#253813,#253814,#253815,#253816,
#253817,#253818,#253819,#253820,#253821,#253822,#253823,#253824,#253825,
#253826,#253827,#253828,#253829,#253830,#253831,#253832,#253833,#253834,
#253835,#253836,#253837,#253838,#253839,#253840,#253841,#253842,#253843,
#253844,#253845,#253846,#253847,#253848,#253849,#253850,#253851,#253852,
#253853,#253854,#253855,#253856,#253857,#253858,#253859,#253860,#253861,
#253862,#253863,#253864,#253865,#253866,#253867,#253868,#253869,#253870,
#253871,#253872,#253873,#253874,#253875,#253876,#253877,#253878,#253879,
#253880,#253881,#253882,#253883,#253884,#253885,#253886,#253887,#253888,
#253889,#253890,#253891,#253892,#253893,#253894,#253895,#253896,#253897,
#253898,#253899,#253900,#253901,#253902,#253903,#253904,#253905,#253906,
#253907,#253908,#253909,#253910,#253911,#253912,#253913,#253914,#253915,
#253916,#253917,#253918,#253919,#253920,#253921,#253922,#253923,#253924,
#253925,#253926,#253927,#253928,#253929,#253930,#253931,#253932,#253933,
#253934,#253935,#253936,#253937,#253938,#253939,#253940,#253941,#253942,
#253943,#253944,#253945,#253946,#253947,#253948,#253949,#253950,#253951,
#253952,#253953,#253954,#253955,#253956,#253957,#253958,#253959,#253960,
#253961,#253962,#253963,#253964,#253965,#253966,#253967,#253968,#253969,
#253970,#253971,#253972,#253973,#253974,#253975,#253976,#253977,#253978,
#253979,#253980,#253981,#253982,#253983,#253984,#253985,#253986,#253987,
#253988,#253989,#253990,#253991,#253992,#253993,#253994,#253995,#253996),
 .UNSPECIFIED.,.F.,.F.)
B_SPLINE_CURVE_WITH_KNOTS((6,1,1,1,1,1,1,1,1,1,1,1,1,1,1,1,1,1,1,1,1,1,
1,1,1,1,1,1,1,1,1,1,1,1,1,1,1,1,1,1,1,1,1,1,1,1,1,1,1,1,1,1,1,1,1,1,1,1,
1,1,1,1,1,1,1,1,1,1,1,1,1,1,1,1,1,1,1,1,1,1,1,1,1,1,1,1,1,1,1,1,1,1,1,1,
1,1,1,1,1,1,1,1,1,1,1,1,1,1,1,1,1,1,1,1,1,1,1,1,1,1,1,1,1,1,1,1,1,1,1,1,
1,1,1,1,1,1,1,1,1,1,1,1,1,1,1,1,1,1,1,1,1,1,1,1,1,1,1,1,1,1,1,1,1,1,1,1,
1,1,1,1,1,1,1,1,1,1,1,1,1,1,1,1,1,1,1,1,1,1,1,1,1,1,1,1,1,1,1,1,1,1,6),
(-1.,-0.995000000000001,-0.990000000000001,-0.985000000000001,-0.980000000000001,
-0.975000000000001,-0.970000000000001,-0.965000000000001,-0.960000000000001,
-0.955000000000001,-0.950000000000001,-0.945000000000001,-0.940000000000001,
-0.935000000000001,-0.930000000000001,-0.925000000000001,-0.920000000000001,
-0.915000000000001,-0.910000000000001,-0.905000000000001,-0.900000000000001,
-0.895000000000001,-0.890000000000001,-0.885000000000001,-0.880000000000001,
-0.875000000000001,-0.870000000000001,-0.865000000000001,-0.860000000000001,
-0.855000000000001,-0.850000000000001,-0.845000000000001,-0.840000000000001,
-0.835000000000001,-0.830000000000001,-0.825000000000001,-0.820000000000001,
-0.815000000000001,-0.810000000000001,-0.805000000000001,-0.800000000000001,
-0.795000000000001,-0.790000000000001,-0.785000000000001,-0.780000000000001,
-0.775000000000001,-0.770000000000001,-0.765000000000001,-0.760000000000001,
-0.755000000000001,-0.750000000000001,-0.745000000000001,-0.740000000000001,
-0.735000000000001,-0.730000000000001,-0.725000000000001,-0.720000000000001,
-0.715000000000001,-0.710000000000001,-0.705000000000001,-0.700000000000001,
-0.695000000000001,-0.690000000000001,-0.685,-0.68,-0.675,-0.67,-0.665,
-0.66,-0.655,-0.65,-0.645,-0.64,-0.635,-0.63,-0.625,-0.62,-0.615,-0.61,
-0.605,-0.6,-0.595,-0.59,-0.585,-0.58,-0.575,-0.57,-0.565,-0.56,-0.555,
-0.55,-0.545,-0.54,-0.535,-0.53,-0.525,-0.52,-0.515,-0.51,-0.505,-0.5,-0.495,
-0.49,-0.485,-0.48,-0.475,-0.47,-0.465,-0.46,-0.455,-0.45,-0.445,-0.44,
-0.435,-0.43,-0.425,-0.42,-0.415,-0.41,-0.405,-0.4,-0.395,-0.39,-0.385,
-0.38,-0.375,-0.37,-0.365,-0.36,-0.355,-0.35,-0.345,-0.34,-0.335,-0.33,
-0.325,-0.32,-0.315,-0.31,-0.305,-0.3,-0.295,-0.29,-0.285,-0.28,-0.275,
-0.27,-0.265,-0.26,-0.255,-0.25,-0.245,-0.24,-0.235,-0.23,-0.225,-0.22,
-0.215,-0.21,-0.205,-0.2,-0.195,-0.19,-0.185,-0.18,-0.175,-0.17,-0.165,
-0.16,-0.155,-0.15,-0.145,-0.14,-0.135,-0.13,-0.125,-0.12,-0.115,-0.11,
-0.105,-0.1,-0.095,-0.09,-0.085,-0.08,-0.075,-0.07,-0.065,-0.06,-0.055,
-0.05,-0.045,-0.04,-0.035,-0.03,-0.025,-0.02,-0.015,-0.01,-0.005,0.),
 .UNSPECIFIED.)
CURVE()
GEOMETRIC_REPRESENTATION_ITEM()
RATIONAL_B_SPLINE_CURVE((1.,1.,1.,1.,1.,1.,1.,1.,1.,1.,1.,1.,1.,1.,1.,1.,
1.,1.,1.,1.,1.,1.,1.,1.,1.,1.,1.,1.,1.,1.,1.,1.,1.,1.,1.,1.,1.,1.,1.,1.,
1.,1.,1.,1.,1.,1.,1.,1.,1.,1.,1.,1.,1.,1.,1.,1.,1.,1.,1.,1.,1.,1.,1.,1.,
1.,1.,1.,1.,1.,1.,1.,1.,1.,1.,1.,1.,1.,1.,1.,1.,1.,1.,1.,1.,1.,1.,1.,1.,
1.,1.,1.,1.,1.,1.,1.,1.,1.,1.,1.,1.,1.,1.,1.,1.,1.,1.,1.,1.,1.,1.,1.,1.,
1.,1.,1.,1.,1.,1.,1.,1.,1.,1.,1.,1.,1.,1.,1.,1.,1.,1.,1.,1.,1.,1.,1.,1.,
1.,1.,1.,1.,1.,1.,1.,1.,1.,1.,1.,1.,1.,1.,1.,1.,1.,1.,1.,1.,1.,1.,1.,1.,
1.,1.,1.,1.,1.,1.,1.,1.,1.,1.,1.,1.,1.,1.,1.,1.,1.,1.,1.,1.,1.,1.,1.,1.,
1.,1.,1.,1.,1.,1.,1.,1.,1.,1.,1.,1.,1.,1.,1.,1.,1.,1.,1.,1.,1.))
REPRESENTATION_ITEM('')
);
#879=(
BOUNDED_CURVE()
B_SPLINE_CURVE(5,(#254024,#254025,#254026,#254027,#254028,#254029,#254030,
#254031,#254032,#254033,#254034,#254035,#254036,#254037,#254038,#254039,
#254040,#254041,#254042,#254043,#254044,#254045,#254046,#254047,#254048,
#254049,#254050,#254051,#254052,#254053,#254054,#254055,#254056,#254057,
#254058,#254059,#254060,#254061,#254062,#254063,#254064,#254065,#254066,
#254067,#254068,#254069,#254070,#254071,#254072,#254073,#254074,#254075,
#254076,#254077,#254078,#254079,#254080,#254081,#254082,#254083,#254084,
#254085,#254086,#254087,#254088,#254089,#254090,#254091,#254092,#254093,
#254094,#254095,#254096,#254097,#254098,#254099,#254100,#254101,#254102,
#254103,#254104,#254105,#254106,#254107,#254108,#254109,#254110,#254111,
#254112,#254113,#254114,#254115,#254116,#254117,#254118,#254119,#254120,
#254121,#254122,#254123,#254124,#254125,#254126,#254127,#254128,#254129,
#254130,#254131,#254132,#254133,#254134,#254135,#254136,#254137,#254138,
#254139,#254140,#254141,#254142,#254143,#254144,#254145,#254146,#254147,
#254148,#254149,#254150,#254151,#254152,#254153,#254154,#254155,#254156,
#254157,#254158,#254159,#254160,#254161,#254162,#254163,#254164,#254165,
#254166,#254167,#254168,#254169,#254170,#254171,#254172,#254173,#254174,
#254175,#254176,#254177,#254178,#254179,#254180,#254181,#254182,#254183,
#254184,#254185,#254186,#254187,#254188,#254189,#254190,#254191,#254192,
#254193,#254194,#254195,#254196,#254197,#254198,#254199,#254200,#254201,
#254202,#254203,#254204,#254205,#254206,#254207,#254208,#254209,#254210,
#254211,#254212,#254213,#254214,#254215,#254216,#254217,#254218,#254219,
#254220,#254221,#254222,#254223,#254224,#254225,#254226,#254227,#254228),
 .UNSPECIFIED.,.F.,.F.)
B_SPLINE_CURVE_WITH_KNOTS((6,1,1,1,1,1,1,1,1,1,1,1,1,1,1,1,1,1,1,1,1,1,
1,1,1,1,1,1,1,1,1,1,1,1,1,1,1,1,1,1,1,1,1,1,1,1,1,1,1,1,1,1,1,1,1,1,1,1,
1,1,1,1,1,1,1,1,1,1,1,1,1,1,1,1,1,1,1,1,1,1,1,1,1,1,1,1,1,1,1,1,1,1,1,1,
1,1,1,1,1,1,1,1,1,1,1,1,1,1,1,1,1,1,1,1,1,1,1,1,1,1,1,1,1,1,1,1,1,1,1,1,
1,1,1,1,1,1,1,1,1,1,1,1,1,1,1,1,1,1,1,1,1,1,1,1,1,1,1,1,1,1,1,1,1,1,1,1,
1,1,1,1,1,1,1,1,1,1,1,1,1,1,1,1,1,1,1,1,1,1,1,1,1,1,1,1,1,1,1,1,1,1,6),
(-1.,-0.995000000000001,-0.990000000000001,-0.985000000000001,-0.980000000000001,
-0.975000000000001,-0.970000000000001,-0.965000000000001,-0.960000000000001,
-0.955000000000001,-0.950000000000001,-0.945000000000001,-0.940000000000001,
-0.935000000000001,-0.930000000000001,-0.925000000000001,-0.920000000000001,
-0.915000000000001,-0.910000000000001,-0.905000000000001,-0.900000000000001,
-0.895000000000001,-0.890000000000001,-0.885000000000001,-0.880000000000001,
-0.875000000000001,-0.870000000000001,-0.865000000000001,-0.860000000000001,
-0.855000000000001,-0.850000000000001,-0.845000000000001,-0.840000000000001,
-0.835000000000001,-0.830000000000001,-0.825000000000001,-0.820000000000001,
-0.815000000000001,-0.810000000000001,-0.805000000000001,-0.800000000000001,
-0.795000000000001,-0.790000000000001,-0.785000000000001,-0.780000000000001,
-0.775000000000001,-0.770000000000001,-0.765000000000001,-0.760000000000001,
-0.755000000000001,-0.750000000000001,-0.745000000000001,-0.740000000000001,
-0.735000000000001,-0.730000000000001,-0.725000000000001,-0.720000000000001,
-0.715000000000001,-0.710000000000001,-0.705000000000001,-0.700000000000001,
-0.695000000000001,-0.690000000000001,-0.685,-0.68,-0.675,-0.67,-0.665,
-0.66,-0.655,-0.65,-0.645,-0.64,-0.635,-0.63,-0.625,-0.62,-0.615,-0.61,
-0.605,-0.6,-0.595,-0.59,-0.585,-0.58,-0.575,-0.57,-0.565,-0.56,-0.555,
-0.55,-0.545,-0.54,-0.535,-0.53,-0.525,-0.52,-0.515,-0.51,-0.505,-0.5,-0.495,
-0.49,-0.485,-0.48,-0.475,-0.47,-0.465,-0.46,-0.455,-0.45,-0.445,-0.44,
-0.435,-0.43,-0.425,-0.42,-0.415,-0.41,-0.405,-0.4,-0.395,-0.39,-0.385,
-0.38,-0.375,-0.37,-0.365,-0.36,-0.355,-0.35,-0.345,-0.34,-0.335,-0.33,
-0.325,-0.32,-0.315,-0.31,-0.305,-0.3,-0.295,-0.29,-0.285,-0.28,-0.275,
-0.27,-0.265,-0.26,-0.255,-0.25,-0.245,-0.24,-0.235,-0.23,-0.225,-0.22,
-0.215,-0.21,-0.205,-0.2,-0.195,-0.19,-0.185,-0.18,-0.175,-0.17,-0.165,
-0.16,-0.155,-0.15,-0.145,-0.14,-0.135,-0.13,-0.125,-0.12,-0.115,-0.11,
-0.105,-0.1,-0.095,-0.09,-0.085,-0.08,-0.075,-0.07,-0.065,-0.06,-0.055,
-0.05,-0.045,-0.04,-0.035,-0.03,-0.025,-0.02,-0.015,-0.01,-0.005,0.),
 .UNSPECIFIED.)
CURVE()
GEOMETRIC_REPRESENTATION_ITEM()
RATIONAL_B_SPLINE_CURVE((1.,1.,1.,1.,1.,1.,1.,1.,1.,1.,1.,1.,1.,1.,1.,1.,
1.,1.,1.,1.,1.,1.,1.,1.,1.,1.,1.,1.,1.,1.,1.,1.,1.,1.,1.,1.,1.,1.,1.,1.,
1.,1.,1.,1.,1.,1.,1.,1.,1.,1.,1.,1.,1.,1.,1.,1.,1.,1.,1.,1.,1.,1.,1.,1.,
1.,1.,1.,1.,1.,1.,1.,1.,1.,1.,1.,1.,1.,1.,1.,1.,1.,1.,1.,1.,1.,1.,1.,1.,
1.,1.,1.,1.,1.,1.,1.,1.,1.,1.,1.,1.,1.,1.,1.,1.,1.,1.,1.,1.,1.,1.,1.,1.,
1.,1.,1.,1.,1.,1.,1.,1.,1.,1.,1.,1.,1.,1.,1.,1.,1.,1.,1.,1.,1.,1.,1.,1.,
1.,1.,1.,1.,1.,1.,1.,1.,1.,1.,1.,1.,1.,1.,1.,1.,1.,1.,1.,1.,1.,1.,1.,1.,
1.,1.,1.,1.,1.,1.,1.,1.,1.,1.,1.,1.,1.,1.,1.,1.,1.,1.,1.,1.,1.,1.,1.,1.,
1.,1.,1.,1.,1.,1.,1.,1.,1.,1.,1.,1.,1.,1.,1.,1.,1.,1.,1.,1.,1.))
REPRESENTATION_ITEM('')
);
#880=(
BOUNDED_CURVE()
B_SPLINE_CURVE(5,(#254240,#254241,#254242,#254243,#254244,#254245,#254246,
#254247,#254248,#254249,#254250,#254251,#254252,#254253,#254254,#254255,
#254256,#254257,#254258,#254259,#254260,#254261,#254262,#254263,#254264,
#254265,#254266,#254267,#254268,#254269,#254270,#254271,#254272,#254273,
#254274,#254275,#254276,#254277,#254278,#254279,#254280,#254281,#254282,
#254283,#254284,#254285,#254286,#254287,#254288,#254289,#254290,#254291,
#254292,#254293,#254294,#254295,#254296,#254297,#254298,#254299,#254300,
#254301,#254302,#254303,#254304,#254305,#254306,#254307,#254308,#254309,
#254310,#254311,#254312,#254313,#254314,#254315,#254316,#254317,#254318,
#254319,#254320,#254321,#254322,#254323,#254324,#254325,#254326,#254327,
#254328,#254329,#254330,#254331,#254332,#254333,#254334,#254335,#254336,
#254337,#254338,#254339,#254340,#254341,#254342,#254343,#254344,#254345,
#254346,#254347,#254348,#254349,#254350,#254351,#254352,#254353,#254354,
#254355,#254356,#254357,#254358,#254359,#254360,#254361,#254362,#254363,
#254364,#254365,#254366,#254367,#254368,#254369,#254370,#254371,#254372,
#254373,#254374,#254375,#254376,#254377,#254378,#254379,#254380,#254381,
#254382,#254383,#254384,#254385,#254386,#254387,#254388,#254389,#254390,
#254391,#254392,#254393,#254394,#254395,#254396,#254397,#254398,#254399,
#254400,#254401,#254402,#254403,#254404,#254405,#254406,#254407,#254408,
#254409,#254410,#254411,#254412,#254413,#254414,#254415,#254416,#254417,
#254418,#254419,#254420,#254421,#254422,#254423,#254424,#254425,#254426,
#254427,#254428,#254429,#254430,#254431,#254432,#254433,#254434,#254435,
#254436,#254437,#254438,#254439,#254440,#254441,#254442,#254443,#254444),
 .UNSPECIFIED.,.F.,.F.)
B_SPLINE_CURVE_WITH_KNOTS((6,1,1,1,1,1,1,1,1,1,1,1,1,1,1,1,1,1,1,1,1,1,
1,1,1,1,1,1,1,1,1,1,1,1,1,1,1,1,1,1,1,1,1,1,1,1,1,1,1,1,1,1,1,1,1,1,1,1,
1,1,1,1,1,1,1,1,1,1,1,1,1,1,1,1,1,1,1,1,1,1,1,1,1,1,1,1,1,1,1,1,1,1,1,1,
1,1,1,1,1,1,1,1,1,1,1,1,1,1,1,1,1,1,1,1,1,1,1,1,1,1,1,1,1,1,1,1,1,1,1,1,
1,1,1,1,1,1,1,1,1,1,1,1,1,1,1,1,1,1,1,1,1,1,1,1,1,1,1,1,1,1,1,1,1,1,1,1,
1,1,1,1,1,1,1,1,1,1,1,1,1,1,1,1,1,1,1,1,1,1,1,1,1,1,1,1,1,1,1,1,1,1,6),
(0.,0.005,0.01,0.015,0.02,0.025,0.03,0.035,0.04,0.045,0.05,0.055,0.06,0.065,
0.07,0.075,0.08,0.085,0.09,0.095,0.1,0.105,0.11,0.115,0.12,0.125,0.13,0.135,
0.14,0.145,0.15,0.155,0.16,0.165,0.17,0.175,0.18,0.185,0.19,0.195,0.2,0.205,
0.21,0.215,0.22,0.225,0.23,0.235,0.24,0.245,0.25,0.255,0.26,0.265,0.27,
0.275,0.28,0.285,0.29,0.295,0.3,0.305,0.31,0.315,0.32,0.325,0.33,0.335,
0.34,0.345,0.35,0.355,0.36,0.365,0.37,0.375,0.38,0.385,0.39,0.395,0.4,0.405,
0.41,0.415,0.42,0.425,0.43,0.435,0.44,0.445,0.45,0.455,0.46,0.465,0.47,
0.475,0.48,0.485,0.49,0.495,0.5,0.505,0.51,0.515,0.52,0.525,0.53,0.535,
0.54,0.545,0.55,0.555,0.56,0.565,0.57,0.575,0.58,0.585,0.59,0.595,0.6,0.605,
0.61,0.615,0.62,0.625,0.63,0.635,0.64,0.645,0.65,0.655,0.66,0.665,0.67,
0.675,0.68,0.685,0.690000000000001,0.695000000000001,0.700000000000001,
0.705000000000001,0.710000000000001,0.715000000000001,0.720000000000001,
0.725000000000001,0.730000000000001,0.735000000000001,0.740000000000001,
0.745000000000001,0.750000000000001,0.755000000000001,0.760000000000001,
0.765000000000001,0.770000000000001,0.775000000000001,0.780000000000001,
0.785000000000001,0.790000000000001,0.795000000000001,0.800000000000001,
0.805000000000001,0.810000000000001,0.815000000000001,0.820000000000001,
0.825000000000001,0.830000000000001,0.835000000000001,0.840000000000001,
0.845000000000001,0.850000000000001,0.855000000000001,0.860000000000001,
0.865000000000001,0.870000000000001,0.875000000000001,0.880000000000001,
0.885000000000001,0.890000000000001,0.895000000000001,0.900000000000001,
0.905000000000001,0.910000000000001,0.915000000000001,0.920000000000001,
0.925000000000001,0.930000000000001,0.935000000000001,0.940000000000001,
0.945000000000001,0.950000000000001,0.955000000000001,0.960000000000001,
0.965000000000001,0.970000000000001,0.975000000000001,0.980000000000001,
0.985000000000001,0.990000000000001,0.995000000000001,1.),.UNSPECIFIED.)
CURVE()
GEOMETRIC_REPRESENTATION_ITEM()
RATIONAL_B_SPLINE_CURVE((1.,1.,1.,1.,1.,1.,1.,1.,1.,1.,1.,1.,1.,1.,1.,1.,
1.,1.,1.,1.,1.,1.,1.,1.,1.,1.,1.,1.,1.,1.,1.,1.,1.,1.,1.,1.,1.,1.,1.,1.,
1.,1.,1.,1.,1.,1.,1.,1.,1.,1.,1.,1.,1.,1.,1.,1.,1.,1.,1.,1.,1.,1.,1.,1.,
1.,1.,1.,1.,1.,1.,1.,1.,1.,1.,1.,1.,1.,1.,1.,1.,1.,1.,1.,1.,1.,1.,1.,1.,
1.,1.,1.,1.,1.,1.,1.,1.,1.,1.,1.,1.,1.,1.,1.,1.,1.,1.,1.,1.,1.,1.,1.,1.,
1.,1.,1.,1.,1.,1.,1.,1.,1.,1.,1.,1.,1.,1.,1.,1.,1.,1.,1.,1.,1.,1.,1.,1.,
1.,1.,1.,1.,1.,1.,1.,1.,1.,1.,1.,1.,1.,1.,1.,1.,1.,1.,1.,1.,1.,1.,1.,1.,
1.,1.,1.,1.,1.,1.,1.,1.,1.,1.,1.,1.,1.,1.,1.,1.,1.,1.,1.,1.,1.,1.,1.,1.,
1.,1.,1.,1.,1.,1.,1.,1.,1.,1.,1.,1.,1.,1.,1.,1.,1.,1.,1.,1.,1.))
REPRESENTATION_ITEM('')
);
#881=(
BOUNDED_CURVE()
B_SPLINE_CURVE(5,(#254452,#254453,#254454,#254455,#254456,#254457,#254458,
#254459,#254460,#254461,#254462,#254463,#254464,#254465,#254466,#254467,
#254468,#254469,#254470,#254471,#254472,#254473,#254474,#254475,#254476,
#254477,#254478,#254479,#254480,#254481,#254482,#254483,#254484,#254485,
#254486,#254487,#254488,#254489,#254490,#254491,#254492,#254493,#254494,
#254495,#254496,#254497,#254498,#254499,#254500,#254501,#254502,#254503,
#254504,#254505,#254506,#254507,#254508,#254509,#254510,#254511,#254512,
#254513,#254514,#254515,#254516,#254517,#254518,#254519,#254520,#254521,
#254522,#254523,#254524,#254525,#254526,#254527,#254528,#254529,#254530,
#254531,#254532,#254533,#254534,#254535,#254536,#254537,#254538,#254539,
#254540,#254541,#254542,#254543,#254544,#254545,#254546,#254547,#254548,
#254549,#254550,#254551,#254552,#254553,#254554,#254555,#254556,#254557,
#254558,#254559,#254560,#254561,#254562,#254563,#254564,#254565,#254566,
#254567,#254568,#254569,#254570,#254571,#254572,#254573,#254574,#254575,
#254576,#254577,#254578,#254579,#254580,#254581,#254582,#254583,#254584,
#254585,#254586,#254587,#254588,#254589,#254590,#254591,#254592,#254593,
#254594,#254595,#254596,#254597,#254598,#254599,#254600,#254601,#254602,
#254603,#254604,#254605,#254606,#254607,#254608,#254609,#254610,#254611,
#254612,#254613,#254614,#254615,#254616,#254617,#254618,#254619,#254620,
#254621,#254622,#254623,#254624,#254625,#254626,#254627,#254628,#254629,
#254630,#254631,#254632,#254633,#254634,#254635,#254636,#254637,#254638,
#254639,#254640,#254641,#254642,#254643,#254644,#254645,#254646,#254647,
#254648,#254649,#254650,#254651,#254652,#254653,#254654,#254655,#254656),
 .UNSPECIFIED.,.F.,.F.)
B_SPLINE_CURVE_WITH_KNOTS((6,1,1,1,1,1,1,1,1,1,1,1,1,1,1,1,1,1,1,1,1,1,
1,1,1,1,1,1,1,1,1,1,1,1,1,1,1,1,1,1,1,1,1,1,1,1,1,1,1,1,1,1,1,1,1,1,1,1,
1,1,1,1,1,1,1,1,1,1,1,1,1,1,1,1,1,1,1,1,1,1,1,1,1,1,1,1,1,1,1,1,1,1,1,1,
1,1,1,1,1,1,1,1,1,1,1,1,1,1,1,1,1,1,1,1,1,1,1,1,1,1,1,1,1,1,1,1,1,1,1,1,
1,1,1,1,1,1,1,1,1,1,1,1,1,1,1,1,1,1,1,1,1,1,1,1,1,1,1,1,1,1,1,1,1,1,1,1,
1,1,1,1,1,1,1,1,1,1,1,1,1,1,1,1,1,1,1,1,1,1,1,1,1,1,1,1,1,1,1,1,1,1,6),
(-1.,-0.995000000000001,-0.990000000000001,-0.985000000000001,-0.980000000000001,
-0.975000000000001,-0.970000000000001,-0.965000000000001,-0.960000000000001,
-0.955000000000001,-0.950000000000001,-0.945000000000001,-0.940000000000001,
-0.935000000000001,-0.930000000000001,-0.925000000000001,-0.920000000000001,
-0.915000000000001,-0.910000000000001,-0.905000000000001,-0.900000000000001,
-0.895000000000001,-0.890000000000001,-0.885000000000001,-0.880000000000001,
-0.875000000000001,-0.870000000000001,-0.865000000000001,-0.860000000000001,
-0.855000000000001,-0.850000000000001,-0.845000000000001,-0.840000000000001,
-0.835000000000001,-0.830000000000001,-0.825000000000001,-0.820000000000001,
-0.815000000000001,-0.810000000000001,-0.805000000000001,-0.800000000000001,
-0.795000000000001,-0.790000000000001,-0.785000000000001,-0.780000000000001,
-0.775000000000001,-0.770000000000001,-0.765000000000001,-0.760000000000001,
-0.755000000000001,-0.750000000000001,-0.745000000000001,-0.740000000000001,
-0.735000000000001,-0.730000000000001,-0.725000000000001,-0.720000000000001,
-0.715000000000001,-0.710000000000001,-0.705000000000001,-0.700000000000001,
-0.695000000000001,-0.690000000000001,-0.685,-0.68,-0.675,-0.67,-0.665,
-0.66,-0.655,-0.65,-0.645,-0.64,-0.635,-0.63,-0.625,-0.62,-0.615,-0.61,
-0.605,-0.6,-0.595,-0.59,-0.585,-0.58,-0.575,-0.57,-0.565,-0.56,-0.555,
-0.55,-0.545,-0.54,-0.535,-0.53,-0.525,-0.52,-0.515,-0.51,-0.505,-0.5,-0.495,
-0.49,-0.485,-0.48,-0.475,-0.47,-0.465,-0.46,-0.455,-0.45,-0.445,-0.44,
-0.435,-0.43,-0.425,-0.42,-0.415,-0.41,-0.405,-0.4,-0.395,-0.39,-0.385,
-0.38,-0.375,-0.37,-0.365,-0.36,-0.355,-0.35,-0.345,-0.34,-0.335,-0.33,
-0.325,-0.32,-0.315,-0.31,-0.305,-0.3,-0.295,-0.29,-0.285,-0.28,-0.275,
-0.27,-0.265,-0.26,-0.255,-0.25,-0.245,-0.24,-0.235,-0.23,-0.225,-0.22,
-0.215,-0.21,-0.205,-0.2,-0.195,-0.19,-0.185,-0.18,-0.175,-0.17,-0.165,
-0.16,-0.155,-0.15,-0.145,-0.14,-0.135,-0.13,-0.125,-0.12,-0.115,-0.11,
-0.105,-0.1,-0.095,-0.09,-0.085,-0.08,-0.075,-0.07,-0.065,-0.06,-0.055,
-0.05,-0.045,-0.04,-0.035,-0.03,-0.025,-0.02,-0.015,-0.01,-0.005,0.),
 .UNSPECIFIED.)
CURVE()
GEOMETRIC_REPRESENTATION_ITEM()
RATIONAL_B_SPLINE_CURVE((1.,1.,1.,1.,1.,1.,1.,1.,1.,1.,1.,1.,1.,1.,1.,1.,
1.,1.,1.,1.,1.,1.,1.,1.,1.,1.,1.,1.,1.,1.,1.,1.,1.,1.,1.,1.,1.,1.,1.,1.,
1.,1.,1.,1.,1.,1.,1.,1.,1.,1.,1.,1.,1.,1.,1.,1.,1.,1.,1.,1.,1.,1.,1.,1.,
1.,1.,1.,1.,1.,1.,1.,1.,1.,1.,1.,1.,1.,1.,1.,1.,1.,1.,1.,1.,1.,1.,1.,1.,
1.,1.,1.,1.,1.,1.,1.,1.,1.,1.,1.,1.,1.,1.,1.,1.,1.,1.,1.,1.,1.,1.,1.,1.,
1.,1.,1.,1.,1.,1.,1.,1.,1.,1.,1.,1.,1.,1.,1.,1.,1.,1.,1.,1.,1.,1.,1.,1.,
1.,1.,1.,1.,1.,1.,1.,1.,1.,1.,1.,1.,1.,1.,1.,1.,1.,1.,1.,1.,1.,1.,1.,1.,
1.,1.,1.,1.,1.,1.,1.,1.,1.,1.,1.,1.,1.,1.,1.,1.,1.,1.,1.,1.,1.,1.,1.,1.,
1.,1.,1.,1.,1.,1.,1.,1.,1.,1.,1.,1.,1.,1.,1.,1.,1.,1.,1.,1.,1.))
REPRESENTATION_ITEM('')
);
#882=(
BOUNDED_CURVE()
B_SPLINE_CURVE(5,(#254668,#254669,#254670,#254671,#254672,#254673,#254674,
#254675,#254676,#254677,#254678,#254679,#254680,#254681,#254682,#254683,
#254684,#254685,#254686,#254687,#254688,#254689,#254690,#254691,#254692,
#254693,#254694,#254695,#254696,#254697,#254698,#254699,#254700,#254701,
#254702,#254703,#254704,#254705,#254706,#254707,#254708,#254709,#254710,
#254711,#254712,#254713,#254714,#254715,#254716,#254717,#254718,#254719,
#254720,#254721,#254722,#254723,#254724,#254725,#254726,#254727,#254728,
#254729,#254730,#254731,#254732,#254733,#254734,#254735,#254736,#254737,
#254738,#254739,#254740,#254741,#254742,#254743,#254744,#254745,#254746,
#254747,#254748,#254749,#254750,#254751,#254752,#254753,#254754,#254755,
#254756,#254757,#254758,#254759,#254760,#254761,#254762,#254763,#254764,
#254765,#254766,#254767,#254768,#254769,#254770,#254771,#254772,#254773,
#254774,#254775,#254776,#254777,#254778,#254779,#254780,#254781,#254782,
#254783,#254784,#254785,#254786,#254787,#254788,#254789,#254790,#254791,
#254792,#254793,#254794,#254795,#254796,#254797,#254798,#254799,#254800,
#254801,#254802,#254803,#254804,#254805,#254806,#254807,#254808,#254809,
#254810,#254811,#254812,#254813,#254814,#254815,#254816,#254817,#254818,
#254819,#254820,#254821,#254822,#254823,#254824,#254825,#254826,#254827,
#254828,#254829,#254830,#254831,#254832,#254833,#254834,#254835,#254836,
#254837,#254838,#254839,#254840,#254841,#254842,#254843,#254844,#254845,
#254846,#254847,#254848,#254849,#254850,#254851,#254852,#254853,#254854,
#254855,#254856,#254857,#254858,#254859,#254860,#254861,#254862,#254863,
#254864,#254865,#254866,#254867,#254868,#254869,#254870,#254871,#254872),
 .UNSPECIFIED.,.F.,.F.)
B_SPLINE_CURVE_WITH_KNOTS((6,1,1,1,1,1,1,1,1,1,1,1,1,1,1,1,1,1,1,1,1,1,
1,1,1,1,1,1,1,1,1,1,1,1,1,1,1,1,1,1,1,1,1,1,1,1,1,1,1,1,1,1,1,1,1,1,1,1,
1,1,1,1,1,1,1,1,1,1,1,1,1,1,1,1,1,1,1,1,1,1,1,1,1,1,1,1,1,1,1,1,1,1,1,1,
1,1,1,1,1,1,1,1,1,1,1,1,1,1,1,1,1,1,1,1,1,1,1,1,1,1,1,1,1,1,1,1,1,1,1,1,
1,1,1,1,1,1,1,1,1,1,1,1,1,1,1,1,1,1,1,1,1,1,1,1,1,1,1,1,1,1,1,1,1,1,1,1,
1,1,1,1,1,1,1,1,1,1,1,1,1,1,1,1,1,1,1,1,1,1,1,1,1,1,1,1,1,1,1,1,1,1,6),
(0.,0.005,0.01,0.015,0.02,0.025,0.03,0.035,0.04,0.045,0.05,0.055,0.06,0.065,
0.07,0.075,0.08,0.085,0.09,0.095,0.1,0.105,0.11,0.115,0.12,0.125,0.13,0.135,
0.14,0.145,0.15,0.155,0.16,0.165,0.17,0.175,0.18,0.185,0.19,0.195,0.2,0.205,
0.21,0.215,0.22,0.225,0.23,0.235,0.24,0.245,0.25,0.255,0.26,0.265,0.27,
0.275,0.28,0.285,0.29,0.295,0.3,0.305,0.31,0.315,0.32,0.325,0.33,0.335,
0.34,0.345,0.35,0.355,0.36,0.365,0.37,0.375,0.38,0.385,0.39,0.395,0.4,0.405,
0.41,0.415,0.42,0.425,0.43,0.435,0.44,0.445,0.45,0.455,0.46,0.465,0.47,
0.475,0.48,0.485,0.49,0.495,0.5,0.505,0.51,0.515,0.52,0.525,0.53,0.535,
0.54,0.545,0.55,0.555,0.56,0.565,0.57,0.575,0.58,0.585,0.59,0.595,0.6,0.605,
0.61,0.615,0.62,0.625,0.63,0.635,0.64,0.645,0.65,0.655,0.66,0.665,0.67,
0.675,0.68,0.685,0.690000000000001,0.695000000000001,0.700000000000001,
0.705000000000001,0.710000000000001,0.715000000000001,0.720000000000001,
0.725000000000001,0.730000000000001,0.735000000000001,0.740000000000001,
0.745000000000001,0.750000000000001,0.755000000000001,0.760000000000001,
0.765000000000001,0.770000000000001,0.775000000000001,0.780000000000001,
0.785000000000001,0.790000000000001,0.795000000000001,0.800000000000001,
0.805000000000001,0.810000000000001,0.815000000000001,0.820000000000001,
0.825000000000001,0.830000000000001,0.835000000000001,0.840000000000001,
0.845000000000001,0.850000000000001,0.855000000000001,0.860000000000001,
0.865000000000001,0.870000000000001,0.875000000000001,0.880000000000001,
0.885000000000001,0.890000000000001,0.895000000000001,0.900000000000001,
0.905000000000001,0.910000000000001,0.915000000000001,0.920000000000001,
0.925000000000001,0.930000000000001,0.935000000000001,0.940000000000001,
0.945000000000001,0.950000000000001,0.955000000000001,0.960000000000001,
0.965000000000001,0.970000000000001,0.975000000000001,0.980000000000001,
0.985000000000001,0.990000000000001,0.995000000000001,1.),.UNSPECIFIED.)
CURVE()
GEOMETRIC_REPRESENTATION_ITEM()
RATIONAL_B_SPLINE_CURVE((1.,1.,1.,1.,1.,1.,1.,1.,1.,1.,1.,1.,1.,1.,1.,1.,
1.,1.,1.,1.,1.,1.,1.,1.,1.,1.,1.,1.,1.,1.,1.,1.,1.,1.,1.,1.,1.,1.,1.,1.,
1.,1.,1.,1.,1.,1.,1.,1.,1.,1.,1.,1.,1.,1.,1.,1.,1.,1.,1.,1.,1.,1.,1.,1.,
1.,1.,1.,1.,1.,1.,1.,1.,1.,1.,1.,1.,1.,1.,1.,1.,1.,1.,1.,1.,1.,1.,1.,1.,
1.,1.,1.,1.,1.,1.,1.,1.,1.,1.,1.,1.,1.,1.,1.,1.,1.,1.,1.,1.,1.,1.,1.,1.,
1.,1.,1.,1.,1.,1.,1.,1.,1.,1.,1.,1.,1.,1.,1.,1.,1.,1.,1.,1.,1.,1.,1.,1.,
1.,1.,1.,1.,1.,1.,1.,1.,1.,1.,1.,1.,1.,1.,1.,1.,1.,1.,1.,1.,1.,1.,1.,1.,
1.,1.,1.,1.,1.,1.,1.,1.,1.,1.,1.,1.,1.,1.,1.,1.,1.,1.,1.,1.,1.,1.,1.,1.,
1.,1.,1.,1.,1.,1.,1.,1.,1.,1.,1.,1.,1.,1.,1.,1.,1.,1.,1.,1.,1.))
REPRESENTATION_ITEM('')
);
#1075=(
BOUNDED_SURFACE()
B_SPLINE_SURFACE(5,1,((#216008,#216009),(#216010,#216011),(#216012,#216013),
(#216014,#216015),(#216016,#216017),(#216018,#216019),(#216020,#216021),
(#216022,#216023),(#216024,#216025),(#216026,#216027),(#216028,#216029),
(#216030,#216031),(#216032,#216033),(#216034,#216035),(#216036,#216037),
(#216038,#216039),(#216040,#216041),(#216042,#216043),(#216044,#216045),
(#216046,#216047),(#216048,#216049),(#216050,#216051),(#216052,#216053),
(#216054,#216055),(#216056,#216057),(#216058,#216059),(#216060,#216061),
(#216062,#216063),(#216064,#216065),(#216066,#216067),(#216068,#216069),
(#216070,#216071),(#216072,#216073),(#216074,#216075),(#216076,#216077),
(#216078,#216079),(#216080,#216081),(#216082,#216083),(#216084,#216085),
(#216086,#216087),(#216088,#216089),(#216090,#216091),(#216092,#216093),
(#216094,#216095),(#216096,#216097),(#216098,#216099),(#216100,#216101),
(#216102,#216103),(#216104,#216105),(#216106,#216107),(#216108,#216109),
(#216110,#216111),(#216112,#216113),(#216114,#216115),(#216116,#216117),
(#216118,#216119),(#216120,#216121),(#216122,#216123),(#216124,#216125),
(#216126,#216127),(#216128,#216129),(#216130,#216131),(#216132,#216133),
(#216134,#216135),(#216136,#216137),(#216138,#216139),(#216140,#216141),
(#216142,#216143),(#216144,#216145),(#216146,#216147),(#216148,#216149),
(#216150,#216151),(#216152,#216153),(#216154,#216155),(#216156,#216157),
(#216158,#216159),(#216160,#216161),(#216162,#216163),(#216164,#216165),
(#216166,#216167),(#216168,#216169),(#216170,#216171),(#216172,#216173),
(#216174,#216175),(#216176,#216177),(#216178,#216179),(#216180,#216181),
(#216182,#216183),(#216184,#216185),(#216186,#216187),(#216188,#216189),
(#216190,#216191),(#216192,#216193),(#216194,#216195),(#216196,#216197),
(#216198,#216199),(#216200,#216201),(#216202,#216203),(#216204,#216205),
(#216206,#216207),(#216208,#216209),(#216210,#216211),(#216212,#216213),
(#216214,#216215),(#216216,#216217),(#216218,#216219),(#216220,#216221),
(#216222,#216223),(#216224,#216225),(#216226,#216227),(#216228,#216229),
(#216230,#216231),(#216232,#216233),(#216234,#216235),(#216236,#216237),
(#216238,#216239),(#216240,#216241),(#216242,#216243),(#216244,#216245),
(#216246,#216247),(#216248,#216249),(#216250,#216251),(#216252,#216253),
(#216254,#216255),(#216256,#216257),(#216258,#216259),(#216260,#216261),
(#216262,#216263),(#216264,#216265),(#216266,#216267),(#216268,#216269),
(#216270,#216271),(#216272,#216273),(#216274,#216275),(#216276,#216277),
(#216278,#216279),(#216280,#216281),(#216282,#216283),(#216284,#216285),
(#216286,#216287),(#216288,#216289),(#216290,#216291),(#216292,#216293),
(#216294,#216295),(#216296,#216297),(#216298,#216299),(#216300,#216301),
(#216302,#216303),(#216304,#216305),(#216306,#216307),(#216308,#216309),
(#216310,#216311),(#216312,#216313),(#216314,#216315),(#216316,#216317),
(#216318,#216319),(#216320,#216321),(#216322,#216323),(#216324,#216325),
(#216326,#216327),(#216328,#216329),(#216330,#216331),(#216332,#216333),
(#216334,#216335),(#216336,#216337),(#216338,#216339),(#216340,#216341),
(#216342,#216343),(#216344,#216345),(#216346,#216347),(#216348,#216349),
(#216350,#216351),(#216352,#216353),(#216354,#216355),(#216356,#216357),
(#216358,#216359),(#216360,#216361),(#216362,#216363),(#216364,#216365),
(#216366,#216367),(#216368,#216369),(#216370,#216371),(#216372,#216373),
(#216374,#216375),(#216376,#216377),(#216378,#216379),(#216380,#216381),
(#216382,#216383),(#216384,#216385),(#216386,#216387),(#216388,#216389),
(#216390,#216391),(#216392,#216393),(#216394,#216395),(#216396,#216397),
(#216398,#216399),(#216400,#216401),(#216402,#216403),(#216404,#216405),
(#216406,#216407),(#216408,#216409),(#216410,#216411),(#216412,#216413),
(#216414,#216415),(#216416,#216417)),.UNSPECIFIED.,.F.,.F.,.F.)
B_SPLINE_SURFACE_WITH_KNOTS((6,1,1,1,1,1,1,1,1,1,1,1,1,1,1,1,1,1,1,1,1,
1,1,1,1,1,1,1,1,1,1,1,1,1,1,1,1,1,1,1,1,1,1,1,1,1,1,1,1,1,1,1,1,1,1,1,1,
1,1,1,1,1,1,1,1,1,1,1,1,1,1,1,1,1,1,1,1,1,1,1,1,1,1,1,1,1,1,1,1,1,1,1,1,
1,1,1,1,1,1,1,1,1,1,1,1,1,1,1,1,1,1,1,1,1,1,1,1,1,1,1,1,1,1,1,1,1,1,1,1,
1,1,1,1,1,1,1,1,1,1,1,1,1,1,1,1,1,1,1,1,1,1,1,1,1,1,1,1,1,1,1,1,1,1,1,1,
1,1,1,1,1,1,1,1,1,1,1,1,1,1,1,1,1,1,1,1,1,1,1,1,1,1,1,1,1,1,1,1,1,1,1,6),
(2,2),(-1.,-0.995000000000001,-0.990000000000001,-0.985000000000001,-0.980000000000001,
-0.975000000000001,-0.970000000000001,-0.965000000000001,-0.960000000000001,
-0.955000000000001,-0.950000000000001,-0.945000000000001,-0.940000000000001,
-0.935000000000001,-0.930000000000001,-0.925000000000001,-0.920000000000001,
-0.915000000000001,-0.910000000000001,-0.905000000000001,-0.900000000000001,
-0.895000000000001,-0.890000000000001,-0.885000000000001,-0.880000000000001,
-0.875000000000001,-0.870000000000001,-0.865000000000001,-0.860000000000001,
-0.855000000000001,-0.850000000000001,-0.845000000000001,-0.840000000000001,
-0.835000000000001,-0.830000000000001,-0.825000000000001,-0.820000000000001,
-0.815000000000001,-0.810000000000001,-0.805000000000001,-0.800000000000001,
-0.795000000000001,-0.790000000000001,-0.785000000000001,-0.780000000000001,
-0.775000000000001,-0.770000000000001,-0.765000000000001,-0.760000000000001,
-0.755000000000001,-0.750000000000001,-0.745000000000001,-0.740000000000001,
-0.735000000000001,-0.730000000000001,-0.725000000000001,-0.720000000000001,
-0.715000000000001,-0.710000000000001,-0.705000000000001,-0.700000000000001,
-0.695000000000001,-0.690000000000001,-0.685,-0.68,-0.675,-0.67,-0.665,
-0.66,-0.655,-0.65,-0.645,-0.64,-0.635,-0.63,-0.625,-0.62,-0.615,-0.61,
-0.605,-0.6,-0.595,-0.59,-0.585,-0.58,-0.575,-0.57,-0.565,-0.56,-0.555,
-0.55,-0.545,-0.54,-0.535,-0.53,-0.525,-0.52,-0.515,-0.51,-0.505,-0.5,-0.495,
-0.49,-0.485,-0.48,-0.475,-0.47,-0.465,-0.46,-0.455,-0.45,-0.445,-0.44,
-0.435,-0.43,-0.425,-0.42,-0.415,-0.41,-0.405,-0.4,-0.395,-0.39,-0.385,
-0.38,-0.375,-0.37,-0.365,-0.36,-0.355,-0.35,-0.345,-0.34,-0.335,-0.33,
-0.325,-0.32,-0.315,-0.31,-0.305,-0.3,-0.295,-0.29,-0.285,-0.28,-0.275,
-0.27,-0.265,-0.26,-0.255,-0.25,-0.245,-0.24,-0.235,-0.23,-0.225,-0.22,
-0.215,-0.21,-0.205,-0.2,-0.195,-0.19,-0.185,-0.18,-0.175,-0.17,-0.165,
-0.16,-0.155,-0.15,-0.145,-0.14,-0.135,-0.13,-0.125,-0.12,-0.115,-0.11,
-0.105,-0.1,-0.095,-0.09,-0.085,-0.08,-0.075,-0.07,-0.065,-0.06,-0.055,
-0.05,-0.045,-0.04,-0.035,-0.03,-0.025,-0.02,-0.015,-0.01,-0.005,0.),(0.,
1.2),.UNSPECIFIED.)
GEOMETRIC_REPRESENTATION_ITEM()
RATIONAL_B_SPLINE_SURFACE(((1.,1.),(1.,1.),(1.,1.),(1.,1.),(1.,1.),(1.,
1.),(1.,1.),(1.,1.),(1.,1.),(1.,1.),(1.,1.),(1.,1.),(1.,1.),(1.,1.),(1.,
1.),(1.,1.),(1.,1.),(1.,1.),(1.,1.),(1.,1.),(1.,1.),(1.,1.),(1.,1.),(1.,
1.),(1.,1.),(1.,1.),(1.,1.),(1.,1.),(1.,1.),(1.,1.),(1.,1.),(1.,1.),(1.,
1.),(1.,1.),(1.,1.),(1.,1.),(1.,1.),(1.,1.),(1.,1.),(1.,1.),(1.,1.),(1.,
1.),(1.,1.),(1.,1.),(1.,1.),(1.,1.),(1.,1.),(1.,1.),(1.,1.),(1.,1.),(1.,
1.),(1.,1.),(1.,1.),(1.,1.),(1.,1.),(1.,1.),(1.,1.),(1.,1.),(1.,1.),(1.,
1.),(1.,1.),(1.,1.),(1.,1.),(1.,1.),(1.,1.),(1.,1.),(1.,1.),(1.,1.),(1.,
1.),(1.,1.),(1.,1.),(1.,1.),(1.,1.),(1.,1.),(1.,1.),(1.,1.),(1.,1.),(1.,
1.),(1.,1.),(1.,1.),(1.,1.),(1.,1.),(1.,1.),(1.,1.),(1.,1.),(1.,1.),(1.,
1.),(1.,1.),(1.,1.),(1.,1.),(1.,1.),(1.,1.),(1.,1.),(1.,1.),(1.,1.),(1.,
1.),(1.,1.),(1.,1.),(1.,1.),(1.,1.),(1.,1.),(1.,1.),(1.,1.),(1.,1.),(1.,
1.),(1.,1.),(1.,1.),(1.,1.),(1.,1.),(1.,1.),(1.,1.),(1.,1.),(1.,1.),(1.,
1.),(1.,1.),(1.,1.),(1.,1.),(1.,1.),(1.,1.),(1.,1.),(1.,1.),(1.,1.),(1.,
1.),(1.,1.),(1.,1.),(1.,1.),(1.,1.),(1.,1.),(1.,1.),(1.,1.),(1.,1.),(1.,
1.),(1.,1.),(1.,1.),(1.,1.),(1.,1.),(1.,1.),(1.,1.),(1.,1.),(1.,1.),(1.,
1.),(1.,1.),(1.,1.),(1.,1.),(1.,1.),(1.,1.),(1.,1.),(1.,1.),(1.,1.),(1.,
1.),(1.,1.),(1.,1.),(1.,1.),(1.,1.),(1.,1.),(1.,1.),(1.,1.),(1.,1.),(1.,
1.),(1.,1.),(1.,1.),(1.,1.),(1.,1.),(1.,1.),(1.,1.),(1.,1.),(1.,1.),(1.,
1.),(1.,1.),(1.,1.),(1.,1.),(1.,1.),(1.,1.),(1.,1.),(1.,1.),(1.,1.),(1.,
1.),(1.,1.),(1.,1.),(1.,1.),(1.,1.),(1.,1.),(1.,1.),(1.,1.),(1.,1.),(1.,
1.),(1.,1.),(1.,1.),(1.,1.),(1.,1.),(1.,1.),(1.,1.),(1.,1.),(1.,1.),(1.,
1.),(1.,1.),(1.,1.),(1.,1.),(1.,1.),(1.,1.),(1.,1.),(1.,1.),(1.,1.),(1.,
1.),(1.,1.)))
REPRESENTATION_ITEM('')
SURFACE()
);
#1076=(
BOUNDED_SURFACE()
B_SPLINE_SURFACE(5,1,((#216831,#216832),(#216833,#216834),(#216835,#216836),
(#216837,#216838),(#216839,#216840),(#216841,#216842),(#216843,#216844),
(#216845,#216846),(#216847,#216848),(#216849,#216850),(#216851,#216852),
(#216853,#216854),(#216855,#216856),(#216857,#216858),(#216859,#216860),
(#216861,#216862),(#216863,#216864),(#216865,#216866),(#216867,#216868),
(#216869,#216870),(#216871,#216872),(#216873,#216874),(#216875,#216876),
(#216877,#216878),(#216879,#216880),(#216881,#216882),(#216883,#216884),
(#216885,#216886),(#216887,#216888),(#216889,#216890),(#216891,#216892),
(#216893,#216894),(#216895,#216896),(#216897,#216898),(#216899,#216900),
(#216901,#216902),(#216903,#216904),(#216905,#216906),(#216907,#216908),
(#216909,#216910),(#216911,#216912),(#216913,#216914),(#216915,#216916),
(#216917,#216918),(#216919,#216920),(#216921,#216922),(#216923,#216924),
(#216925,#216926),(#216927,#216928),(#216929,#216930),(#216931,#216932),
(#216933,#216934),(#216935,#216936),(#216937,#216938),(#216939,#216940),
(#216941,#216942),(#216943,#216944),(#216945,#216946),(#216947,#216948),
(#216949,#216950),(#216951,#216952),(#216953,#216954),(#216955,#216956),
(#216957,#216958),(#216959,#216960),(#216961,#216962),(#216963,#216964),
(#216965,#216966),(#216967,#216968),(#216969,#216970),(#216971,#216972),
(#216973,#216974),(#216975,#216976),(#216977,#216978),(#216979,#216980),
(#216981,#216982),(#216983,#216984),(#216985,#216986),(#216987,#216988),
(#216989,#216990),(#216991,#216992),(#216993,#216994),(#216995,#216996),
(#216997,#216998),(#216999,#217000),(#217001,#217002),(#217003,#217004),
(#217005,#217006),(#217007,#217008),(#217009,#217010),(#217011,#217012),
(#217013,#217014),(#217015,#217016),(#217017,#217018),(#217019,#217020),
(#217021,#217022),(#217023,#217024),(#217025,#217026),(#217027,#217028),
(#217029,#217030),(#217031,#217032),(#217033,#217034),(#217035,#217036),
(#217037,#217038),(#217039,#217040),(#217041,#217042),(#217043,#217044),
(#217045,#217046),(#217047,#217048),(#217049,#217050),(#217051,#217052),
(#217053,#217054),(#217055,#217056),(#217057,#217058),(#217059,#217060),
(#217061,#217062),(#217063,#217064),(#217065,#217066),(#217067,#217068),
(#217069,#217070),(#217071,#217072),(#217073,#217074),(#217075,#217076),
(#217077,#217078),(#217079,#217080),(#217081,#217082),(#217083,#217084),
(#217085,#217086),(#217087,#217088),(#217089,#217090),(#217091,#217092),
(#217093,#217094),(#217095,#217096),(#217097,#217098),(#217099,#217100),
(#217101,#217102),(#217103,#217104),(#217105,#217106),(#217107,#217108),
(#217109,#217110),(#217111,#217112),(#217113,#217114),(#217115,#217116),
(#217117,#217118),(#217119,#217120),(#217121,#217122),(#217123,#217124),
(#217125,#217126),(#217127,#217128),(#217129,#217130),(#217131,#217132),
(#217133,#217134),(#217135,#217136),(#217137,#217138),(#217139,#217140),
(#217141,#217142),(#217143,#217144),(#217145,#217146),(#217147,#217148),
(#217149,#217150),(#217151,#217152),(#217153,#217154),(#217155,#217156),
(#217157,#217158),(#217159,#217160),(#217161,#217162),(#217163,#217164),
(#217165,#217166),(#217167,#217168),(#217169,#217170),(#217171,#217172),
(#217173,#217174),(#217175,#217176),(#217177,#217178),(#217179,#217180),
(#217181,#217182),(#217183,#217184),(#217185,#217186),(#217187,#217188),
(#217189,#217190),(#217191,#217192),(#217193,#217194),(#217195,#217196),
(#217197,#217198),(#217199,#217200),(#217201,#217202),(#217203,#217204),
(#217205,#217206),(#217207,#217208),(#217209,#217210),(#217211,#217212),
(#217213,#217214),(#217215,#217216),(#217217,#217218),(#217219,#217220),
(#217221,#217222),(#217223,#217224),(#217225,#217226),(#217227,#217228),
(#217229,#217230),(#217231,#217232),(#217233,#217234),(#217235,#217236),
(#217237,#217238),(#217239,#217240)),.UNSPECIFIED.,.F.,.F.,.F.)
B_SPLINE_SURFACE_WITH_KNOTS((6,1,1,1,1,1,1,1,1,1,1,1,1,1,1,1,1,1,1,1,1,
1,1,1,1,1,1,1,1,1,1,1,1,1,1,1,1,1,1,1,1,1,1,1,1,1,1,1,1,1,1,1,1,1,1,1,1,
1,1,1,1,1,1,1,1,1,1,1,1,1,1,1,1,1,1,1,1,1,1,1,1,1,1,1,1,1,1,1,1,1,1,1,1,
1,1,1,1,1,1,1,1,1,1,1,1,1,1,1,1,1,1,1,1,1,1,1,1,1,1,1,1,1,1,1,1,1,1,1,1,
1,1,1,1,1,1,1,1,1,1,1,1,1,1,1,1,1,1,1,1,1,1,1,1,1,1,1,1,1,1,1,1,1,1,1,1,
1,1,1,1,1,1,1,1,1,1,1,1,1,1,1,1,1,1,1,1,1,1,1,1,1,1,1,1,1,1,1,1,1,1,1,6),
(2,2),(0.,0.005,0.01,0.015,0.02,0.025,0.03,0.035,0.04,0.045,0.05,0.055,
0.06,0.065,0.07,0.075,0.08,0.085,0.09,0.095,0.1,0.105,0.11,0.115,0.12,0.125,
0.13,0.135,0.14,0.145,0.15,0.155,0.16,0.165,0.17,0.175,0.18,0.185,0.19,
0.195,0.2,0.205,0.21,0.215,0.22,0.225,0.23,0.235,0.24,0.245,0.25,0.255,
0.26,0.265,0.27,0.275,0.28,0.285,0.29,0.295,0.3,0.305,0.31,0.315,0.32,0.325,
0.33,0.335,0.34,0.345,0.35,0.355,0.36,0.365,0.37,0.375,0.38,0.385,0.39,
0.395,0.4,0.405,0.41,0.415,0.42,0.425,0.43,0.435,0.44,0.445,0.45,0.455,
0.46,0.465,0.47,0.475,0.48,0.485,0.49,0.495,0.5,0.505,0.51,0.515,0.52,0.525,
0.53,0.535,0.54,0.545,0.55,0.555,0.56,0.565,0.57,0.575,0.58,0.585,0.59,
0.595,0.6,0.605,0.61,0.615,0.62,0.625,0.63,0.635,0.64,0.645,0.65,0.655,
0.66,0.665,0.67,0.675,0.68,0.685,0.690000000000001,0.695000000000001,0.700000000000001,
0.705000000000001,0.710000000000001,0.715000000000001,0.720000000000001,
0.725000000000001,0.730000000000001,0.735000000000001,0.740000000000001,
0.745000000000001,0.750000000000001,0.755000000000001,0.760000000000001,
0.765000000000001,0.770000000000001,0.775000000000001,0.780000000000001,
0.785000000000001,0.790000000000001,0.795000000000001,0.800000000000001,
0.805000000000001,0.810000000000001,0.815000000000001,0.820000000000001,
0.825000000000001,0.830000000000001,0.835000000000001,0.840000000000001,
0.845000000000001,0.850000000000001,0.855000000000001,0.860000000000001,
0.865000000000001,0.870000000000001,0.875000000000001,0.880000000000001,
0.885000000000001,0.890000000000001,0.895000000000001,0.900000000000001,
0.905000000000001,0.910000000000001,0.915000000000001,0.920000000000001,
0.925000000000001,0.930000000000001,0.935000000000001,0.940000000000001,
0.945000000000001,0.950000000000001,0.955000000000001,0.960000000000001,
0.965000000000001,0.970000000000001,0.975000000000001,0.980000000000001,
0.985000000000001,0.990000000000001,0.995000000000001,1.),(0.,1.2),
 .UNSPECIFIED.)
GEOMETRIC_REPRESENTATION_ITEM()
RATIONAL_B_SPLINE_SURFACE(((1.,1.),(1.,1.),(1.,1.),(1.,1.),(1.,1.),(1.,
1.),(1.,1.),(1.,1.),(1.,1.),(1.,1.),(1.,1.),(1.,1.),(1.,1.),(1.,1.),(1.,
1.),(1.,1.),(1.,1.),(1.,1.),(1.,1.),(1.,1.),(1.,1.),(1.,1.),(1.,1.),(1.,
1.),(1.,1.),(1.,1.),(1.,1.),(1.,1.),(1.,1.),(1.,1.),(1.,1.),(1.,1.),(1.,
1.),(1.,1.),(1.,1.),(1.,1.),(1.,1.),(1.,1.),(1.,1.),(1.,1.),(1.,1.),(1.,
1.),(1.,1.),(1.,1.),(1.,1.),(1.,1.),(1.,1.),(1.,1.),(1.,1.),(1.,1.),(1.,
1.),(1.,1.),(1.,1.),(1.,1.),(1.,1.),(1.,1.),(1.,1.),(1.,1.),(1.,1.),(1.,
1.),(1.,1.),(1.,1.),(1.,1.),(1.,1.),(1.,1.),(1.,1.),(1.,1.),(1.,1.),(1.,
1.),(1.,1.),(1.,1.),(1.,1.),(1.,1.),(1.,1.),(1.,1.),(1.,1.),(1.,1.),(1.,
1.),(1.,1.),(1.,1.),(1.,1.),(1.,1.),(1.,1.),(1.,1.),(1.,1.),(1.,1.),(1.,
1.),(1.,1.),(1.,1.),(1.,1.),(1.,1.),(1.,1.),(1.,1.),(1.,1.),(1.,1.),(1.,
1.),(1.,1.),(1.,1.),(1.,1.),(1.,1.),(1.,1.),(1.,1.),(1.,1.),(1.,1.),(1.,
1.),(1.,1.),(1.,1.),(1.,1.),(1.,1.),(1.,1.),(1.,1.),(1.,1.),(1.,1.),(1.,
1.),(1.,1.),(1.,1.),(1.,1.),(1.,1.),(1.,1.),(1.,1.),(1.,1.),(1.,1.),(1.,
1.),(1.,1.),(1.,1.),(1.,1.),(1.,1.),(1.,1.),(1.,1.),(1.,1.),(1.,1.),(1.,
1.),(1.,1.),(1.,1.),(1.,1.),(1.,1.),(1.,1.),(1.,1.),(1.,1.),(1.,1.),(1.,
1.),(1.,1.),(1.,1.),(1.,1.),(1.,1.),(1.,1.),(1.,1.),(1.,1.),(1.,1.),(1.,
1.),(1.,1.),(1.,1.),(1.,1.),(1.,1.),(1.,1.),(1.,1.),(1.,1.),(1.,1.),(1.,
1.),(1.,1.),(1.,1.),(1.,1.),(1.,1.),(1.,1.),(1.,1.),(1.,1.),(1.,1.),(1.,
1.),(1.,1.),(1.,1.),(1.,1.),(1.,1.),(1.,1.),(1.,1.),(1.,1.),(1.,1.),(1.,
1.),(1.,1.),(1.,1.),(1.,1.),(1.,1.),(1.,1.),(1.,1.),(1.,1.),(1.,1.),(1.,
1.),(1.,1.),(1.,1.),(1.,1.),(1.,1.),(1.,1.),(1.,1.),(1.,1.),(1.,1.),(1.,
1.),(1.,1.),(1.,1.),(1.,1.),(1.,1.),(1.,1.),(1.,1.),(1.,1.),(1.,1.),(1.,
1.),(1.,1.)))
REPRESENTATION_ITEM('')
SURFACE()
);
#1077=(
BOUNDED_SURFACE()
B_SPLINE_SURFACE(5,1,((#217660,#217661),(#217662,#217663),(#217664,#217665),
(#217666,#217667),(#217668,#217669),(#217670,#217671),(#217672,#217673),
(#217674,#217675),(#217676,#217677),(#217678,#217679),(#217680,#217681),
(#217682,#217683),(#217684,#217685),(#217686,#217687),(#217688,#217689),
(#217690,#217691),(#217692,#217693),(#217694,#217695),(#217696,#217697),
(#217698,#217699),(#217700,#217701),(#217702,#217703),(#217704,#217705),
(#217706,#217707),(#217708,#217709),(#217710,#217711),(#217712,#217713),
(#217714,#217715),(#217716,#217717),(#217718,#217719),(#217720,#217721),
(#217722,#217723),(#217724,#217725),(#217726,#217727),(#217728,#217729),
(#217730,#217731),(#217732,#217733),(#217734,#217735),(#217736,#217737),
(#217738,#217739),(#217740,#217741),(#217742,#217743),(#217744,#217745),
(#217746,#217747),(#217748,#217749),(#217750,#217751),(#217752,#217753),
(#217754,#217755),(#217756,#217757),(#217758,#217759),(#217760,#217761),
(#217762,#217763),(#217764,#217765),(#217766,#217767),(#217768,#217769),
(#217770,#217771),(#217772,#217773),(#217774,#217775),(#217776,#217777),
(#217778,#217779),(#217780,#217781),(#217782,#217783),(#217784,#217785),
(#217786,#217787),(#217788,#217789),(#217790,#217791),(#217792,#217793),
(#217794,#217795),(#217796,#217797),(#217798,#217799),(#217800,#217801),
(#217802,#217803),(#217804,#217805),(#217806,#217807),(#217808,#217809),
(#217810,#217811),(#217812,#217813),(#217814,#217815),(#217816,#217817),
(#217818,#217819),(#217820,#217821),(#217822,#217823),(#217824,#217825),
(#217826,#217827),(#217828,#217829),(#217830,#217831),(#217832,#217833),
(#217834,#217835),(#217836,#217837),(#217838,#217839),(#217840,#217841),
(#217842,#217843),(#217844,#217845),(#217846,#217847),(#217848,#217849),
(#217850,#217851),(#217852,#217853),(#217854,#217855),(#217856,#217857),
(#217858,#217859),(#217860,#217861),(#217862,#217863),(#217864,#217865),
(#217866,#217867),(#217868,#217869),(#217870,#217871),(#217872,#217873),
(#217874,#217875),(#217876,#217877),(#217878,#217879),(#217880,#217881),
(#217882,#217883),(#217884,#217885),(#217886,#217887),(#217888,#217889),
(#217890,#217891),(#217892,#217893),(#217894,#217895),(#217896,#217897),
(#217898,#217899),(#217900,#217901),(#217902,#217903),(#217904,#217905),
(#217906,#217907),(#217908,#217909),(#217910,#217911),(#217912,#217913),
(#217914,#217915),(#217916,#217917),(#217918,#217919),(#217920,#217921),
(#217922,#217923),(#217924,#217925),(#217926,#217927),(#217928,#217929),
(#217930,#217931),(#217932,#217933),(#217934,#217935),(#217936,#217937),
(#217938,#217939),(#217940,#217941),(#217942,#217943),(#217944,#217945),
(#217946,#217947),(#217948,#217949),(#217950,#217951),(#217952,#217953),
(#217954,#217955),(#217956,#217957),(#217958,#217959),(#217960,#217961),
(#217962,#217963),(#217964,#217965),(#217966,#217967),(#217968,#217969),
(#217970,#217971),(#217972,#217973),(#217974,#217975),(#217976,#217977),
(#217978,#217979),(#217980,#217981),(#217982,#217983),(#217984,#217985),
(#217986,#217987),(#217988,#217989),(#217990,#217991),(#217992,#217993),
(#217994,#217995),(#217996,#217997),(#217998,#217999),(#218000,#218001),
(#218002,#218003),(#218004,#218005),(#218006,#218007),(#218008,#218009),
(#218010,#218011),(#218012,#218013),(#218014,#218015),(#218016,#218017),
(#218018,#218019),(#218020,#218021),(#218022,#218023),(#218024,#218025),
(#218026,#218027),(#218028,#218029),(#218030,#218031),(#218032,#218033),
(#218034,#218035),(#218036,#218037),(#218038,#218039),(#218040,#218041),
(#218042,#218043),(#218044,#218045),(#218046,#218047),(#218048,#218049),
(#218050,#218051),(#218052,#218053),(#218054,#218055),(#218056,#218057),
(#218058,#218059),(#218060,#218061),(#218062,#218063),(#218064,#218065),
(#218066,#218067),(#218068,#218069)),.UNSPECIFIED.,.F.,.F.,.F.)
B_SPLINE_SURFACE_WITH_KNOTS((6,1,1,1,1,1,1,1,1,1,1,1,1,1,1,1,1,1,1,1,1,
1,1,1,1,1,1,1,1,1,1,1,1,1,1,1,1,1,1,1,1,1,1,1,1,1,1,1,1,1,1,1,1,1,1,1,1,
1,1,1,1,1,1,1,1,1,1,1,1,1,1,1,1,1,1,1,1,1,1,1,1,1,1,1,1,1,1,1,1,1,1,1,1,
1,1,1,1,1,1,1,1,1,1,1,1,1,1,1,1,1,1,1,1,1,1,1,1,1,1,1,1,1,1,1,1,1,1,1,1,
1,1,1,1,1,1,1,1,1,1,1,1,1,1,1,1,1,1,1,1,1,1,1,1,1,1,1,1,1,1,1,1,1,1,1,1,
1,1,1,1,1,1,1,1,1,1,1,1,1,1,1,1,1,1,1,1,1,1,1,1,1,1,1,1,1,1,1,1,1,1,1,6),
(2,2),(-1.,-0.995000000000001,-0.990000000000001,-0.985000000000001,-0.980000000000001,
-0.975000000000001,-0.970000000000001,-0.965000000000001,-0.960000000000001,
-0.955000000000001,-0.950000000000001,-0.945000000000001,-0.940000000000001,
-0.935000000000001,-0.930000000000001,-0.925000000000001,-0.920000000000001,
-0.915000000000001,-0.910000000000001,-0.905000000000001,-0.900000000000001,
-0.895000000000001,-0.890000000000001,-0.885000000000001,-0.880000000000001,
-0.875000000000001,-0.870000000000001,-0.865000000000001,-0.860000000000001,
-0.855000000000001,-0.850000000000001,-0.845000000000001,-0.840000000000001,
-0.835000000000001,-0.830000000000001,-0.825000000000001,-0.820000000000001,
-0.815000000000001,-0.810000000000001,-0.805000000000001,-0.800000000000001,
-0.795000000000001,-0.790000000000001,-0.785000000000001,-0.780000000000001,
-0.775000000000001,-0.770000000000001,-0.765000000000001,-0.760000000000001,
-0.755000000000001,-0.750000000000001,-0.745000000000001,-0.740000000000001,
-0.735000000000001,-0.730000000000001,-0.725000000000001,-0.720000000000001,
-0.715000000000001,-0.710000000000001,-0.705000000000001,-0.700000000000001,
-0.695000000000001,-0.690000000000001,-0.685,-0.68,-0.675,-0.67,-0.665,
-0.66,-0.655,-0.65,-0.645,-0.64,-0.635,-0.63,-0.625,-0.62,-0.615,-0.61,
-0.605,-0.6,-0.595,-0.59,-0.585,-0.58,-0.575,-0.57,-0.565,-0.56,-0.555,
-0.55,-0.545,-0.54,-0.535,-0.53,-0.525,-0.52,-0.515,-0.51,-0.505,-0.5,-0.495,
-0.49,-0.485,-0.48,-0.475,-0.47,-0.465,-0.46,-0.455,-0.45,-0.445,-0.44,
-0.435,-0.43,-0.425,-0.42,-0.415,-0.41,-0.405,-0.4,-0.395,-0.39,-0.385,
-0.38,-0.375,-0.37,-0.365,-0.36,-0.355,-0.35,-0.345,-0.34,-0.335,-0.33,
-0.325,-0.32,-0.315,-0.31,-0.305,-0.3,-0.295,-0.29,-0.285,-0.28,-0.275,
-0.27,-0.265,-0.26,-0.255,-0.25,-0.245,-0.24,-0.235,-0.23,-0.225,-0.22,
-0.215,-0.21,-0.205,-0.2,-0.195,-0.19,-0.185,-0.18,-0.175,-0.17,-0.165,
-0.16,-0.155,-0.15,-0.145,-0.14,-0.135,-0.13,-0.125,-0.12,-0.115,-0.11,
-0.105,-0.1,-0.095,-0.09,-0.085,-0.08,-0.075,-0.07,-0.065,-0.06,-0.055,
-0.05,-0.045,-0.04,-0.035,-0.03,-0.025,-0.02,-0.015,-0.01,-0.005,0.),(0.,
1.2),.UNSPECIFIED.)
GEOMETRIC_REPRESENTATION_ITEM()
RATIONAL_B_SPLINE_SURFACE(((1.,1.),(1.,1.),(1.,1.),(1.,1.),(1.,1.),(1.,
1.),(1.,1.),(1.,1.),(1.,1.),(1.,1.),(1.,1.),(1.,1.),(1.,1.),(1.,1.),(1.,
1.),(1.,1.),(1.,1.),(1.,1.),(1.,1.),(1.,1.),(1.,1.),(1.,1.),(1.,1.),(1.,
1.),(1.,1.),(1.,1.),(1.,1.),(1.,1.),(1.,1.),(1.,1.),(1.,1.),(1.,1.),(1.,
1.),(1.,1.),(1.,1.),(1.,1.),(1.,1.),(1.,1.),(1.,1.),(1.,1.),(1.,1.),(1.,
1.),(1.,1.),(1.,1.),(1.,1.),(1.,1.),(1.,1.),(1.,1.),(1.,1.),(1.,1.),(1.,
1.),(1.,1.),(1.,1.),(1.,1.),(1.,1.),(1.,1.),(1.,1.),(1.,1.),(1.,1.),(1.,
1.),(1.,1.),(1.,1.),(1.,1.),(1.,1.),(1.,1.),(1.,1.),(1.,1.),(1.,1.),(1.,
1.),(1.,1.),(1.,1.),(1.,1.),(1.,1.),(1.,1.),(1.,1.),(1.,1.),(1.,1.),(1.,
1.),(1.,1.),(1.,1.),(1.,1.),(1.,1.),(1.,1.),(1.,1.),(1.,1.),(1.,1.),(1.,
1.),(1.,1.),(1.,1.),(1.,1.),(1.,1.),(1.,1.),(1.,1.),(1.,1.),(1.,1.),(1.,
1.),(1.,1.),(1.,1.),(1.,1.),(1.,1.),(1.,1.),(1.,1.),(1.,1.),(1.,1.),(1.,
1.),(1.,1.),(1.,1.),(1.,1.),(1.,1.),(1.,1.),(1.,1.),(1.,1.),(1.,1.),(1.,
1.),(1.,1.),(1.,1.),(1.,1.),(1.,1.),(1.,1.),(1.,1.),(1.,1.),(1.,1.),(1.,
1.),(1.,1.),(1.,1.),(1.,1.),(1.,1.),(1.,1.),(1.,1.),(1.,1.),(1.,1.),(1.,
1.),(1.,1.),(1.,1.),(1.,1.),(1.,1.),(1.,1.),(1.,1.),(1.,1.),(1.,1.),(1.,
1.),(1.,1.),(1.,1.),(1.,1.),(1.,1.),(1.,1.),(1.,1.),(1.,1.),(1.,1.),(1.,
1.),(1.,1.),(1.,1.),(1.,1.),(1.,1.),(1.,1.),(1.,1.),(1.,1.),(1.,1.),(1.,
1.),(1.,1.),(1.,1.),(1.,1.),(1.,1.),(1.,1.),(1.,1.),(1.,1.),(1.,1.),(1.,
1.),(1.,1.),(1.,1.),(1.,1.),(1.,1.),(1.,1.),(1.,1.),(1.,1.),(1.,1.),(1.,
1.),(1.,1.),(1.,1.),(1.,1.),(1.,1.),(1.,1.),(1.,1.),(1.,1.),(1.,1.),(1.,
1.),(1.,1.),(1.,1.),(1.,1.),(1.,1.),(1.,1.),(1.,1.),(1.,1.),(1.,1.),(1.,
1.),(1.,1.),(1.,1.),(1.,1.),(1.,1.),(1.,1.),(1.,1.),(1.,1.),(1.,1.),(1.,
1.),(1.,1.)))
REPRESENTATION_ITEM('')
SURFACE()
);
#1078=(
BOUNDED_SURFACE()
B_SPLINE_SURFACE(5,1,((#218483,#218484),(#218485,#218486),(#218487,#218488),
(#218489,#218490),(#218491,#218492),(#218493,#218494),(#218495,#218496),
(#218497,#218498),(#218499,#218500),(#218501,#218502),(#218503,#218504),
(#218505,#218506),(#218507,#218508),(#218509,#218510),(#218511,#218512),
(#218513,#218514),(#218515,#218516),(#218517,#218518),(#218519,#218520),
(#218521,#218522),(#218523,#218524),(#218525,#218526),(#218527,#218528),
(#218529,#218530),(#218531,#218532),(#218533,#218534),(#218535,#218536),
(#218537,#218538),(#218539,#218540),(#218541,#218542),(#218543,#218544),
(#218545,#218546),(#218547,#218548),(#218549,#218550),(#218551,#218552),
(#218553,#218554),(#218555,#218556),(#218557,#218558),(#218559,#218560),
(#218561,#218562),(#218563,#218564),(#218565,#218566),(#218567,#218568),
(#218569,#218570),(#218571,#218572),(#218573,#218574),(#218575,#218576),
(#218577,#218578),(#218579,#218580),(#218581,#218582),(#218583,#218584),
(#218585,#218586),(#218587,#218588),(#218589,#218590),(#218591,#218592),
(#218593,#218594),(#218595,#218596),(#218597,#218598),(#218599,#218600),
(#218601,#218602),(#218603,#218604),(#218605,#218606),(#218607,#218608),
(#218609,#218610),(#218611,#218612),(#218613,#218614),(#218615,#218616),
(#218617,#218618),(#218619,#218620),(#218621,#218622),(#218623,#218624),
(#218625,#218626),(#218627,#218628),(#218629,#218630),(#218631,#218632),
(#218633,#218634),(#218635,#218636),(#218637,#218638),(#218639,#218640),
(#218641,#218642),(#218643,#218644),(#218645,#218646),(#218647,#218648),
(#218649,#218650),(#218651,#218652),(#218653,#218654),(#218655,#218656),
(#218657,#218658),(#218659,#218660),(#218661,#218662),(#218663,#218664),
(#218665,#218666),(#218667,#218668),(#218669,#218670),(#218671,#218672),
(#218673,#218674),(#218675,#218676),(#218677,#218678),(#218679,#218680),
(#218681,#218682),(#218683,#218684),(#218685,#218686),(#218687,#218688),
(#218689,#218690),(#218691,#218692),(#218693,#218694),(#218695,#218696),
(#218697,#218698),(#218699,#218700),(#218701,#218702),(#218703,#218704),
(#218705,#218706),(#218707,#218708),(#218709,#218710),(#218711,#218712),
(#218713,#218714),(#218715,#218716),(#218717,#218718),(#218719,#218720),
(#218721,#218722),(#218723,#218724),(#218725,#218726),(#218727,#218728),
(#218729,#218730),(#218731,#218732),(#218733,#218734),(#218735,#218736),
(#218737,#218738),(#218739,#218740),(#218741,#218742),(#218743,#218744),
(#218745,#218746),(#218747,#218748),(#218749,#218750),(#218751,#218752),
(#218753,#218754),(#218755,#218756),(#218757,#218758),(#218759,#218760),
(#218761,#218762),(#218763,#218764),(#218765,#218766),(#218767,#218768),
(#218769,#218770),(#218771,#218772),(#218773,#218774),(#218775,#218776),
(#218777,#218778),(#218779,#218780),(#218781,#218782),(#218783,#218784),
(#218785,#218786),(#218787,#218788),(#218789,#218790),(#218791,#218792),
(#218793,#218794),(#218795,#218796),(#218797,#218798),(#218799,#218800),
(#218801,#218802),(#218803,#218804),(#218805,#218806),(#218807,#218808),
(#218809,#218810),(#218811,#218812),(#218813,#218814),(#218815,#218816),
(#218817,#218818),(#218819,#218820),(#218821,#218822),(#218823,#218824),
(#218825,#218826),(#218827,#218828),(#218829,#218830),(#218831,#218832),
(#218833,#218834),(#218835,#218836),(#218837,#218838),(#218839,#218840),
(#218841,#218842),(#218843,#218844),(#218845,#218846),(#218847,#218848),
(#218849,#218850),(#218851,#218852),(#218853,#218854),(#218855,#218856),
(#218857,#218858),(#218859,#218860),(#218861,#218862),(#218863,#218864),
(#218865,#218866),(#218867,#218868),(#218869,#218870),(#218871,#218872),
(#218873,#218874),(#218875,#218876),(#218877,#218878),(#218879,#218880),
(#218881,#218882),(#218883,#218884),(#218885,#218886),(#218887,#218888),
(#218889,#218890),(#218891,#218892)),.UNSPECIFIED.,.F.,.F.,.F.)
B_SPLINE_SURFACE_WITH_KNOTS((6,1,1,1,1,1,1,1,1,1,1,1,1,1,1,1,1,1,1,1,1,
1,1,1,1,1,1,1,1,1,1,1,1,1,1,1,1,1,1,1,1,1,1,1,1,1,1,1,1,1,1,1,1,1,1,1,1,
1,1,1,1,1,1,1,1,1,1,1,1,1,1,1,1,1,1,1,1,1,1,1,1,1,1,1,1,1,1,1,1,1,1,1,1,
1,1,1,1,1,1,1,1,1,1,1,1,1,1,1,1,1,1,1,1,1,1,1,1,1,1,1,1,1,1,1,1,1,1,1,1,
1,1,1,1,1,1,1,1,1,1,1,1,1,1,1,1,1,1,1,1,1,1,1,1,1,1,1,1,1,1,1,1,1,1,1,1,
1,1,1,1,1,1,1,1,1,1,1,1,1,1,1,1,1,1,1,1,1,1,1,1,1,1,1,1,1,1,1,1,1,1,1,6),
(2,2),(0.,0.005,0.01,0.015,0.02,0.025,0.03,0.035,0.04,0.045,0.05,0.055,
0.06,0.065,0.07,0.075,0.08,0.085,0.09,0.095,0.1,0.105,0.11,0.115,0.12,0.125,
0.13,0.135,0.14,0.145,0.15,0.155,0.16,0.165,0.17,0.175,0.18,0.185,0.19,
0.195,0.2,0.205,0.21,0.215,0.22,0.225,0.23,0.235,0.24,0.245,0.25,0.255,
0.26,0.265,0.27,0.275,0.28,0.285,0.29,0.295,0.3,0.305,0.31,0.315,0.32,0.325,
0.33,0.335,0.34,0.345,0.35,0.355,0.36,0.365,0.37,0.375,0.38,0.385,0.39,
0.395,0.4,0.405,0.41,0.415,0.42,0.425,0.43,0.435,0.44,0.445,0.45,0.455,
0.46,0.465,0.47,0.475,0.48,0.485,0.49,0.495,0.5,0.505,0.51,0.515,0.52,0.525,
0.53,0.535,0.54,0.545,0.55,0.555,0.56,0.565,0.57,0.575,0.58,0.585,0.59,
0.595,0.6,0.605,0.61,0.615,0.62,0.625,0.63,0.635,0.64,0.645,0.65,0.655,
0.66,0.665,0.67,0.675,0.68,0.685,0.690000000000001,0.695000000000001,0.700000000000001,
0.705000000000001,0.710000000000001,0.715000000000001,0.720000000000001,
0.725000000000001,0.730000000000001,0.735000000000001,0.740000000000001,
0.745000000000001,0.750000000000001,0.755000000000001,0.760000000000001,
0.765000000000001,0.770000000000001,0.775000000000001,0.780000000000001,
0.785000000000001,0.790000000000001,0.795000000000001,0.800000000000001,
0.805000000000001,0.810000000000001,0.815000000000001,0.820000000000001,
0.825000000000001,0.830000000000001,0.835000000000001,0.840000000000001,
0.845000000000001,0.850000000000001,0.855000000000001,0.860000000000001,
0.865000000000001,0.870000000000001,0.875000000000001,0.880000000000001,
0.885000000000001,0.890000000000001,0.895000000000001,0.900000000000001,
0.905000000000001,0.910000000000001,0.915000000000001,0.920000000000001,
0.925000000000001,0.930000000000001,0.935000000000001,0.940000000000001,
0.945000000000001,0.950000000000001,0.955000000000001,0.960000000000001,
0.965000000000001,0.970000000000001,0.975000000000001,0.980000000000001,
0.985000000000001,0.990000000000001,0.995000000000001,1.),(0.,1.2),
 .UNSPECIFIED.)
GEOMETRIC_REPRESENTATION_ITEM()
RATIONAL_B_SPLINE_SURFACE(((1.,1.),(1.,1.),(1.,1.),(1.,1.),(1.,1.),(1.,
1.),(1.,1.),(1.,1.),(1.,1.),(1.,1.),(1.,1.),(1.,1.),(1.,1.),(1.,1.),(1.,
1.),(1.,1.),(1.,1.),(1.,1.),(1.,1.),(1.,1.),(1.,1.),(1.,1.),(1.,1.),(1.,
1.),(1.,1.),(1.,1.),(1.,1.),(1.,1.),(1.,1.),(1.,1.),(1.,1.),(1.,1.),(1.,
1.),(1.,1.),(1.,1.),(1.,1.),(1.,1.),(1.,1.),(1.,1.),(1.,1.),(1.,1.),(1.,
1.),(1.,1.),(1.,1.),(1.,1.),(1.,1.),(1.,1.),(1.,1.),(1.,1.),(1.,1.),(1.,
1.),(1.,1.),(1.,1.),(1.,1.),(1.,1.),(1.,1.),(1.,1.),(1.,1.),(1.,1.),(1.,
1.),(1.,1.),(1.,1.),(1.,1.),(1.,1.),(1.,1.),(1.,1.),(1.,1.),(1.,1.),(1.,
1.),(1.,1.),(1.,1.),(1.,1.),(1.,1.),(1.,1.),(1.,1.),(1.,1.),(1.,1.),(1.,
1.),(1.,1.),(1.,1.),(1.,1.),(1.,1.),(1.,1.),(1.,1.),(1.,1.),(1.,1.),(1.,
1.),(1.,1.),(1.,1.),(1.,1.),(1.,1.),(1.,1.),(1.,1.),(1.,1.),(1.,1.),(1.,
1.),(1.,1.),(1.,1.),(1.,1.),(1.,1.),(1.,1.),(1.,1.),(1.,1.),(1.,1.),(1.,
1.),(1.,1.),(1.,1.),(1.,1.),(1.,1.),(1.,1.),(1.,1.),(1.,1.),(1.,1.),(1.,
1.),(1.,1.),(1.,1.),(1.,1.),(1.,1.),(1.,1.),(1.,1.),(1.,1.),(1.,1.),(1.,
1.),(1.,1.),(1.,1.),(1.,1.),(1.,1.),(1.,1.),(1.,1.),(1.,1.),(1.,1.),(1.,
1.),(1.,1.),(1.,1.),(1.,1.),(1.,1.),(1.,1.),(1.,1.),(1.,1.),(1.,1.),(1.,
1.),(1.,1.),(1.,1.),(1.,1.),(1.,1.),(1.,1.),(1.,1.),(1.,1.),(1.,1.),(1.,
1.),(1.,1.),(1.,1.),(1.,1.),(1.,1.),(1.,1.),(1.,1.),(1.,1.),(1.,1.),(1.,
1.),(1.,1.),(1.,1.),(1.,1.),(1.,1.),(1.,1.),(1.,1.),(1.,1.),(1.,1.),(1.,
1.),(1.,1.),(1.,1.),(1.,1.),(1.,1.),(1.,1.),(1.,1.),(1.,1.),(1.,1.),(1.,
1.),(1.,1.),(1.,1.),(1.,1.),(1.,1.),(1.,1.),(1.,1.),(1.,1.),(1.,1.),(1.,
1.),(1.,1.),(1.,1.),(1.,1.),(1.,1.),(1.,1.),(1.,1.),(1.,1.),(1.,1.),(1.,
1.),(1.,1.),(1.,1.),(1.,1.),(1.,1.),(1.,1.),(1.,1.),(1.,1.),(1.,1.),(1.,
1.),(1.,1.)))
REPRESENTATION_ITEM('')
SURFACE()
);
#1079=(
BOUNDED_SURFACE()
B_SPLINE_SURFACE(5,1,((#219312,#219313),(#219314,#219315),(#219316,#219317),
(#219318,#219319),(#219320,#219321),(#219322,#219323),(#219324,#219325),
(#219326,#219327),(#219328,#219329),(#219330,#219331),(#219332,#219333),
(#219334,#219335),(#219336,#219337),(#219338,#219339),(#219340,#219341),
(#219342,#219343),(#219344,#219345),(#219346,#219347),(#219348,#219349),
(#219350,#219351),(#219352,#219353),(#219354,#219355),(#219356,#219357),
(#219358,#219359),(#219360,#219361),(#219362,#219363),(#219364,#219365),
(#219366,#219367),(#219368,#219369),(#219370,#219371),(#219372,#219373),
(#219374,#219375),(#219376,#219377),(#219378,#219379),(#219380,#219381),
(#219382,#219383),(#219384,#219385),(#219386,#219387),(#219388,#219389),
(#219390,#219391),(#219392,#219393),(#219394,#219395),(#219396,#219397),
(#219398,#219399),(#219400,#219401),(#219402,#219403),(#219404,#219405),
(#219406,#219407),(#219408,#219409),(#219410,#219411),(#219412,#219413),
(#219414,#219415),(#219416,#219417),(#219418,#219419),(#219420,#219421),
(#219422,#219423),(#219424,#219425),(#219426,#219427),(#219428,#219429),
(#219430,#219431),(#219432,#219433),(#219434,#219435),(#219436,#219437),
(#219438,#219439),(#219440,#219441),(#219442,#219443),(#219444,#219445),
(#219446,#219447),(#219448,#219449),(#219450,#219451),(#219452,#219453),
(#219454,#219455),(#219456,#219457),(#219458,#219459),(#219460,#219461),
(#219462,#219463),(#219464,#219465),(#219466,#219467),(#219468,#219469),
(#219470,#219471),(#219472,#219473),(#219474,#219475),(#219476,#219477),
(#219478,#219479),(#219480,#219481),(#219482,#219483),(#219484,#219485),
(#219486,#219487),(#219488,#219489),(#219490,#219491),(#219492,#219493),
(#219494,#219495),(#219496,#219497),(#219498,#219499),(#219500,#219501),
(#219502,#219503),(#219504,#219505),(#219506,#219507),(#219508,#219509),
(#219510,#219511),(#219512,#219513),(#219514,#219515),(#219516,#219517),
(#219518,#219519),(#219520,#219521),(#219522,#219523),(#219524,#219525),
(#219526,#219527),(#219528,#219529),(#219530,#219531),(#219532,#219533),
(#219534,#219535),(#219536,#219537),(#219538,#219539),(#219540,#219541),
(#219542,#219543),(#219544,#219545),(#219546,#219547),(#219548,#219549),
(#219550,#219551),(#219552,#219553),(#219554,#219555),(#219556,#219557),
(#219558,#219559),(#219560,#219561),(#219562,#219563),(#219564,#219565),
(#219566,#219567),(#219568,#219569),(#219570,#219571),(#219572,#219573),
(#219574,#219575),(#219576,#219577),(#219578,#219579),(#219580,#219581),
(#219582,#219583),(#219584,#219585),(#219586,#219587),(#219588,#219589),
(#219590,#219591),(#219592,#219593),(#219594,#219595),(#219596,#219597),
(#219598,#219599),(#219600,#219601),(#219602,#219603),(#219604,#219605),
(#219606,#219607),(#219608,#219609),(#219610,#219611),(#219612,#219613),
(#219614,#219615),(#219616,#219617),(#219618,#219619),(#219620,#219621),
(#219622,#219623),(#219624,#219625),(#219626,#219627),(#219628,#219629),
(#219630,#219631),(#219632,#219633),(#219634,#219635),(#219636,#219637),
(#219638,#219639),(#219640,#219641),(#219642,#219643),(#219644,#219645),
(#219646,#219647),(#219648,#219649),(#219650,#219651),(#219652,#219653),
(#219654,#219655),(#219656,#219657),(#219658,#219659),(#219660,#219661),
(#219662,#219663),(#219664,#219665),(#219666,#219667),(#219668,#219669),
(#219670,#219671),(#219672,#219673),(#219674,#219675),(#219676,#219677),
(#219678,#219679),(#219680,#219681),(#219682,#219683),(#219684,#219685),
(#219686,#219687),(#219688,#219689),(#219690,#219691),(#219692,#219693),
(#219694,#219695),(#219696,#219697),(#219698,#219699),(#219700,#219701),
(#219702,#219703),(#219704,#219705),(#219706,#219707),(#219708,#219709),
(#219710,#219711),(#219712,#219713),(#219714,#219715),(#219716,#219717),
(#219718,#219719),(#219720,#219721)),.UNSPECIFIED.,.F.,.F.,.F.)
B_SPLINE_SURFACE_WITH_KNOTS((6,1,1,1,1,1,1,1,1,1,1,1,1,1,1,1,1,1,1,1,1,
1,1,1,1,1,1,1,1,1,1,1,1,1,1,1,1,1,1,1,1,1,1,1,1,1,1,1,1,1,1,1,1,1,1,1,1,
1,1,1,1,1,1,1,1,1,1,1,1,1,1,1,1,1,1,1,1,1,1,1,1,1,1,1,1,1,1,1,1,1,1,1,1,
1,1,1,1,1,1,1,1,1,1,1,1,1,1,1,1,1,1,1,1,1,1,1,1,1,1,1,1,1,1,1,1,1,1,1,1,
1,1,1,1,1,1,1,1,1,1,1,1,1,1,1,1,1,1,1,1,1,1,1,1,1,1,1,1,1,1,1,1,1,1,1,1,
1,1,1,1,1,1,1,1,1,1,1,1,1,1,1,1,1,1,1,1,1,1,1,1,1,1,1,1,1,1,1,1,1,1,1,6),
(2,2),(-1.,-0.995000000000001,-0.990000000000001,-0.985000000000001,-0.980000000000001,
-0.975000000000001,-0.970000000000001,-0.965000000000001,-0.960000000000001,
-0.955000000000001,-0.950000000000001,-0.945000000000001,-0.940000000000001,
-0.935000000000001,-0.930000000000001,-0.925000000000001,-0.920000000000001,
-0.915000000000001,-0.910000000000001,-0.905000000000001,-0.900000000000001,
-0.895000000000001,-0.890000000000001,-0.885000000000001,-0.880000000000001,
-0.875000000000001,-0.870000000000001,-0.865000000000001,-0.860000000000001,
-0.855000000000001,-0.850000000000001,-0.845000000000001,-0.840000000000001,
-0.835000000000001,-0.830000000000001,-0.825000000000001,-0.820000000000001,
-0.815000000000001,-0.810000000000001,-0.805000000000001,-0.800000000000001,
-0.795000000000001,-0.790000000000001,-0.785000000000001,-0.780000000000001,
-0.775000000000001,-0.770000000000001,-0.765000000000001,-0.760000000000001,
-0.755000000000001,-0.750000000000001,-0.745000000000001,-0.740000000000001,
-0.735000000000001,-0.730000000000001,-0.725000000000001,-0.720000000000001,
-0.715000000000001,-0.710000000000001,-0.705000000000001,-0.700000000000001,
-0.695000000000001,-0.690000000000001,-0.685,-0.68,-0.675,-0.67,-0.665,
-0.66,-0.655,-0.65,-0.645,-0.64,-0.635,-0.63,-0.625,-0.62,-0.615,-0.61,
-0.605,-0.6,-0.595,-0.59,-0.585,-0.58,-0.575,-0.57,-0.565,-0.56,-0.555,
-0.55,-0.545,-0.54,-0.535,-0.53,-0.525,-0.52,-0.515,-0.51,-0.505,-0.5,-0.495,
-0.49,-0.485,-0.48,-0.475,-0.47,-0.465,-0.46,-0.455,-0.45,-0.445,-0.44,
-0.435,-0.43,-0.425,-0.42,-0.415,-0.41,-0.405,-0.4,-0.395,-0.39,-0.385,
-0.38,-0.375,-0.37,-0.365,-0.36,-0.355,-0.35,-0.345,-0.34,-0.335,-0.33,
-0.325,-0.32,-0.315,-0.31,-0.305,-0.3,-0.295,-0.29,-0.285,-0.28,-0.275,
-0.27,-0.265,-0.26,-0.255,-0.25,-0.245,-0.24,-0.235,-0.23,-0.225,-0.22,
-0.215,-0.21,-0.205,-0.2,-0.195,-0.19,-0.185,-0.18,-0.175,-0.17,-0.165,
-0.16,-0.155,-0.15,-0.145,-0.14,-0.135,-0.13,-0.125,-0.12,-0.115,-0.11,
-0.105,-0.1,-0.095,-0.09,-0.085,-0.08,-0.075,-0.07,-0.065,-0.06,-0.055,
-0.05,-0.045,-0.04,-0.035,-0.03,-0.025,-0.02,-0.015,-0.01,-0.005,0.),(0.,
1.2),.UNSPECIFIED.)
GEOMETRIC_REPRESENTATION_ITEM()
RATIONAL_B_SPLINE_SURFACE(((1.,1.),(1.,1.),(1.,1.),(1.,1.),(1.,1.),(1.,
1.),(1.,1.),(1.,1.),(1.,1.),(1.,1.),(1.,1.),(1.,1.),(1.,1.),(1.,1.),(1.,
1.),(1.,1.),(1.,1.),(1.,1.),(1.,1.),(1.,1.),(1.,1.),(1.,1.),(1.,1.),(1.,
1.),(1.,1.),(1.,1.),(1.,1.),(1.,1.),(1.,1.),(1.,1.),(1.,1.),(1.,1.),(1.,
1.),(1.,1.),(1.,1.),(1.,1.),(1.,1.),(1.,1.),(1.,1.),(1.,1.),(1.,1.),(1.,
1.),(1.,1.),(1.,1.),(1.,1.),(1.,1.),(1.,1.),(1.,1.),(1.,1.),(1.,1.),(1.,
1.),(1.,1.),(1.,1.),(1.,1.),(1.,1.),(1.,1.),(1.,1.),(1.,1.),(1.,1.),(1.,
1.),(1.,1.),(1.,1.),(1.,1.),(1.,1.),(1.,1.),(1.,1.),(1.,1.),(1.,1.),(1.,
1.),(1.,1.),(1.,1.),(1.,1.),(1.,1.),(1.,1.),(1.,1.),(1.,1.),(1.,1.),(1.,
1.),(1.,1.),(1.,1.),(1.,1.),(1.,1.),(1.,1.),(1.,1.),(1.,1.),(1.,1.),(1.,
1.),(1.,1.),(1.,1.),(1.,1.),(1.,1.),(1.,1.),(1.,1.),(1.,1.),(1.,1.),(1.,
1.),(1.,1.),(1.,1.),(1.,1.),(1.,1.),(1.,1.),(1.,1.),(1.,1.),(1.,1.),(1.,
1.),(1.,1.),(1.,1.),(1.,1.),(1.,1.),(1.,1.),(1.,1.),(1.,1.),(1.,1.),(1.,
1.),(1.,1.),(1.,1.),(1.,1.),(1.,1.),(1.,1.),(1.,1.),(1.,1.),(1.,1.),(1.,
1.),(1.,1.),(1.,1.),(1.,1.),(1.,1.),(1.,1.),(1.,1.),(1.,1.),(1.,1.),(1.,
1.),(1.,1.),(1.,1.),(1.,1.),(1.,1.),(1.,1.),(1.,1.),(1.,1.),(1.,1.),(1.,
1.),(1.,1.),(1.,1.),(1.,1.),(1.,1.),(1.,1.),(1.,1.),(1.,1.),(1.,1.),(1.,
1.),(1.,1.),(1.,1.),(1.,1.),(1.,1.),(1.,1.),(1.,1.),(1.,1.),(1.,1.),(1.,
1.),(1.,1.),(1.,1.),(1.,1.),(1.,1.),(1.,1.),(1.,1.),(1.,1.),(1.,1.),(1.,
1.),(1.,1.),(1.,1.),(1.,1.),(1.,1.),(1.,1.),(1.,1.),(1.,1.),(1.,1.),(1.,
1.),(1.,1.),(1.,1.),(1.,1.),(1.,1.),(1.,1.),(1.,1.),(1.,1.),(1.,1.),(1.,
1.),(1.,1.),(1.,1.),(1.,1.),(1.,1.),(1.,1.),(1.,1.),(1.,1.),(1.,1.),(1.,
1.),(1.,1.),(1.,1.),(1.,1.),(1.,1.),(1.,1.),(1.,1.),(1.,1.),(1.,1.),(1.,
1.),(1.,1.)))
REPRESENTATION_ITEM('')
SURFACE()
);
#1080=(
BOUNDED_SURFACE()
B_SPLINE_SURFACE(5,1,((#220135,#220136),(#220137,#220138),(#220139,#220140),
(#220141,#220142),(#220143,#220144),(#220145,#220146),(#220147,#220148),
(#220149,#220150),(#220151,#220152),(#220153,#220154),(#220155,#220156),
(#220157,#220158),(#220159,#220160),(#220161,#220162),(#220163,#220164),
(#220165,#220166),(#220167,#220168),(#220169,#220170),(#220171,#220172),
(#220173,#220174),(#220175,#220176),(#220177,#220178),(#220179,#220180),
(#220181,#220182),(#220183,#220184),(#220185,#220186),(#220187,#220188),
(#220189,#220190),(#220191,#220192),(#220193,#220194),(#220195,#220196),
(#220197,#220198),(#220199,#220200),(#220201,#220202),(#220203,#220204),
(#220205,#220206),(#220207,#220208),(#220209,#220210),(#220211,#220212),
(#220213,#220214),(#220215,#220216),(#220217,#220218),(#220219,#220220),
(#220221,#220222),(#220223,#220224),(#220225,#220226),(#220227,#220228),
(#220229,#220230),(#220231,#220232),(#220233,#220234),(#220235,#220236),
(#220237,#220238),(#220239,#220240),(#220241,#220242),(#220243,#220244),
(#220245,#220246),(#220247,#220248),(#220249,#220250),(#220251,#220252),
(#220253,#220254),(#220255,#220256),(#220257,#220258),(#220259,#220260),
(#220261,#220262),(#220263,#220264),(#220265,#220266),(#220267,#220268),
(#220269,#220270),(#220271,#220272),(#220273,#220274),(#220275,#220276),
(#220277,#220278),(#220279,#220280),(#220281,#220282),(#220283,#220284),
(#220285,#220286),(#220287,#220288),(#220289,#220290),(#220291,#220292),
(#220293,#220294),(#220295,#220296),(#220297,#220298),(#220299,#220300),
(#220301,#220302),(#220303,#220304),(#220305,#220306),(#220307,#220308),
(#220309,#220310),(#220311,#220312),(#220313,#220314),(#220315,#220316),
(#220317,#220318),(#220319,#220320),(#220321,#220322),(#220323,#220324),
(#220325,#220326),(#220327,#220328),(#220329,#220330),(#220331,#220332),
(#220333,#220334),(#220335,#220336),(#220337,#220338),(#220339,#220340),
(#220341,#220342),(#220343,#220344),(#220345,#220346),(#220347,#220348),
(#220349,#220350),(#220351,#220352),(#220353,#220354),(#220355,#220356),
(#220357,#220358),(#220359,#220360),(#220361,#220362),(#220363,#220364),
(#220365,#220366),(#220367,#220368),(#220369,#220370),(#220371,#220372),
(#220373,#220374),(#220375,#220376),(#220377,#220378),(#220379,#220380),
(#220381,#220382),(#220383,#220384),(#220385,#220386),(#220387,#220388),
(#220389,#220390),(#220391,#220392),(#220393,#220394),(#220395,#220396),
(#220397,#220398),(#220399,#220400),(#220401,#220402),(#220403,#220404),
(#220405,#220406),(#220407,#220408),(#220409,#220410),(#220411,#220412),
(#220413,#220414),(#220415,#220416),(#220417,#220418),(#220419,#220420),
(#220421,#220422),(#220423,#220424),(#220425,#220426),(#220427,#220428),
(#220429,#220430),(#220431,#220432),(#220433,#220434),(#220435,#220436),
(#220437,#220438),(#220439,#220440),(#220441,#220442),(#220443,#220444),
(#220445,#220446),(#220447,#220448),(#220449,#220450),(#220451,#220452),
(#220453,#220454),(#220455,#220456),(#220457,#220458),(#220459,#220460),
(#220461,#220462),(#220463,#220464),(#220465,#220466),(#220467,#220468),
(#220469,#220470),(#220471,#220472),(#220473,#220474),(#220475,#220476),
(#220477,#220478),(#220479,#220480),(#220481,#220482),(#220483,#220484),
(#220485,#220486),(#220487,#220488),(#220489,#220490),(#220491,#220492),
(#220493,#220494),(#220495,#220496),(#220497,#220498),(#220499,#220500),
(#220501,#220502),(#220503,#220504),(#220505,#220506),(#220507,#220508),
(#220509,#220510),(#220511,#220512),(#220513,#220514),(#220515,#220516),
(#220517,#220518),(#220519,#220520),(#220521,#220522),(#220523,#220524),
(#220525,#220526),(#220527,#220528),(#220529,#220530),(#220531,#220532),
(#220533,#220534),(#220535,#220536),(#220537,#220538),(#220539,#220540),
(#220541,#220542),(#220543,#220544)),.UNSPECIFIED.,.F.,.F.,.F.)
B_SPLINE_SURFACE_WITH_KNOTS((6,1,1,1,1,1,1,1,1,1,1,1,1,1,1,1,1,1,1,1,1,
1,1,1,1,1,1,1,1,1,1,1,1,1,1,1,1,1,1,1,1,1,1,1,1,1,1,1,1,1,1,1,1,1,1,1,1,
1,1,1,1,1,1,1,1,1,1,1,1,1,1,1,1,1,1,1,1,1,1,1,1,1,1,1,1,1,1,1,1,1,1,1,1,
1,1,1,1,1,1,1,1,1,1,1,1,1,1,1,1,1,1,1,1,1,1,1,1,1,1,1,1,1,1,1,1,1,1,1,1,
1,1,1,1,1,1,1,1,1,1,1,1,1,1,1,1,1,1,1,1,1,1,1,1,1,1,1,1,1,1,1,1,1,1,1,1,
1,1,1,1,1,1,1,1,1,1,1,1,1,1,1,1,1,1,1,1,1,1,1,1,1,1,1,1,1,1,1,1,1,1,1,6),
(2,2),(0.,0.005,0.01,0.015,0.02,0.025,0.03,0.035,0.04,0.045,0.05,0.055,
0.06,0.065,0.07,0.075,0.08,0.085,0.09,0.095,0.1,0.105,0.11,0.115,0.12,0.125,
0.13,0.135,0.14,0.145,0.15,0.155,0.16,0.165,0.17,0.175,0.18,0.185,0.19,
0.195,0.2,0.205,0.21,0.215,0.22,0.225,0.23,0.235,0.24,0.245,0.25,0.255,
0.26,0.265,0.27,0.275,0.28,0.285,0.29,0.295,0.3,0.305,0.31,0.315,0.32,0.325,
0.33,0.335,0.34,0.345,0.35,0.355,0.36,0.365,0.37,0.375,0.38,0.385,0.39,
0.395,0.4,0.405,0.41,0.415,0.42,0.425,0.43,0.435,0.44,0.445,0.45,0.455,
0.46,0.465,0.47,0.475,0.48,0.485,0.49,0.495,0.5,0.505,0.51,0.515,0.52,0.525,
0.53,0.535,0.54,0.545,0.55,0.555,0.56,0.565,0.57,0.575,0.58,0.585,0.59,
0.595,0.6,0.605,0.61,0.615,0.62,0.625,0.63,0.635,0.64,0.645,0.65,0.655,
0.66,0.665,0.67,0.675,0.68,0.685,0.690000000000001,0.695000000000001,0.700000000000001,
0.705000000000001,0.710000000000001,0.715000000000001,0.720000000000001,
0.725000000000001,0.730000000000001,0.735000000000001,0.740000000000001,
0.745000000000001,0.750000000000001,0.755000000000001,0.760000000000001,
0.765000000000001,0.770000000000001,0.775000000000001,0.780000000000001,
0.785000000000001,0.790000000000001,0.795000000000001,0.800000000000001,
0.805000000000001,0.810000000000001,0.815000000000001,0.820000000000001,
0.825000000000001,0.830000000000001,0.835000000000001,0.840000000000001,
0.845000000000001,0.850000000000001,0.855000000000001,0.860000000000001,
0.865000000000001,0.870000000000001,0.875000000000001,0.880000000000001,
0.885000000000001,0.890000000000001,0.895000000000001,0.900000000000001,
0.905000000000001,0.910000000000001,0.915000000000001,0.920000000000001,
0.925000000000001,0.930000000000001,0.935000000000001,0.940000000000001,
0.945000000000001,0.950000000000001,0.955000000000001,0.960000000000001,
0.965000000000001,0.970000000000001,0.975000000000001,0.980000000000001,
0.985000000000001,0.990000000000001,0.995000000000001,1.),(0.,1.2),
 .UNSPECIFIED.)
GEOMETRIC_REPRESENTATION_ITEM()
RATIONAL_B_SPLINE_SURFACE(((1.,1.),(1.,1.),(1.,1.),(1.,1.),(1.,1.),(1.,
1.),(1.,1.),(1.,1.),(1.,1.),(1.,1.),(1.,1.),(1.,1.),(1.,1.),(1.,1.),(1.,
1.),(1.,1.),(1.,1.),(1.,1.),(1.,1.),(1.,1.),(1.,1.),(1.,1.),(1.,1.),(1.,
1.),(1.,1.),(1.,1.),(1.,1.),(1.,1.),(1.,1.),(1.,1.),(1.,1.),(1.,1.),(1.,
1.),(1.,1.),(1.,1.),(1.,1.),(1.,1.),(1.,1.),(1.,1.),(1.,1.),(1.,1.),(1.,
1.),(1.,1.),(1.,1.),(1.,1.),(1.,1.),(1.,1.),(1.,1.),(1.,1.),(1.,1.),(1.,
1.),(1.,1.),(1.,1.),(1.,1.),(1.,1.),(1.,1.),(1.,1.),(1.,1.),(1.,1.),(1.,
1.),(1.,1.),(1.,1.),(1.,1.),(1.,1.),(1.,1.),(1.,1.),(1.,1.),(1.,1.),(1.,
1.),(1.,1.),(1.,1.),(1.,1.),(1.,1.),(1.,1.),(1.,1.),(1.,1.),(1.,1.),(1.,
1.),(1.,1.),(1.,1.),(1.,1.),(1.,1.),(1.,1.),(1.,1.),(1.,1.),(1.,1.),(1.,
1.),(1.,1.),(1.,1.),(1.,1.),(1.,1.),(1.,1.),(1.,1.),(1.,1.),(1.,1.),(1.,
1.),(1.,1.),(1.,1.),(1.,1.),(1.,1.),(1.,1.),(1.,1.),(1.,1.),(1.,1.),(1.,
1.),(1.,1.),(1.,1.),(1.,1.),(1.,1.),(1.,1.),(1.,1.),(1.,1.),(1.,1.),(1.,
1.),(1.,1.),(1.,1.),(1.,1.),(1.,1.),(1.,1.),(1.,1.),(1.,1.),(1.,1.),(1.,
1.),(1.,1.),(1.,1.),(1.,1.),(1.,1.),(1.,1.),(1.,1.),(1.,1.),(1.,1.),(1.,
1.),(1.,1.),(1.,1.),(1.,1.),(1.,1.),(1.,1.),(1.,1.),(1.,1.),(1.,1.),(1.,
1.),(1.,1.),(1.,1.),(1.,1.),(1.,1.),(1.,1.),(1.,1.),(1.,1.),(1.,1.),(1.,
1.),(1.,1.),(1.,1.),(1.,1.),(1.,1.),(1.,1.),(1.,1.),(1.,1.),(1.,1.),(1.,
1.),(1.,1.),(1.,1.),(1.,1.),(1.,1.),(1.,1.),(1.,1.),(1.,1.),(1.,1.),(1.,
1.),(1.,1.),(1.,1.),(1.,1.),(1.,1.),(1.,1.),(1.,1.),(1.,1.),(1.,1.),(1.,
1.),(1.,1.),(1.,1.),(1.,1.),(1.,1.),(1.,1.),(1.,1.),(1.,1.),(1.,1.),(1.,
1.),(1.,1.),(1.,1.),(1.,1.),(1.,1.),(1.,1.),(1.,1.),(1.,1.),(1.,1.),(1.,
1.),(1.,1.),(1.,1.),(1.,1.),(1.,1.),(1.,1.),(1.,1.),(1.,1.),(1.,1.),(1.,
1.),(1.,1.)))
REPRESENTATION_ITEM('')
SURFACE()
);
#1081=(
BOUNDED_SURFACE()
B_SPLINE_SURFACE(5,1,((#220964,#220965),(#220966,#220967),(#220968,#220969),
(#220970,#220971),(#220972,#220973),(#220974,#220975),(#220976,#220977),
(#220978,#220979),(#220980,#220981),(#220982,#220983),(#220984,#220985),
(#220986,#220987),(#220988,#220989),(#220990,#220991),(#220992,#220993),
(#220994,#220995),(#220996,#220997),(#220998,#220999),(#221000,#221001),
(#221002,#221003),(#221004,#221005),(#221006,#221007),(#221008,#221009),
(#221010,#221011),(#221012,#221013),(#221014,#221015),(#221016,#221017),
(#221018,#221019),(#221020,#221021),(#221022,#221023),(#221024,#221025),
(#221026,#221027),(#221028,#221029),(#221030,#221031),(#221032,#221033),
(#221034,#221035),(#221036,#221037),(#221038,#221039),(#221040,#221041),
(#221042,#221043),(#221044,#221045),(#221046,#221047),(#221048,#221049),
(#221050,#221051),(#221052,#221053),(#221054,#221055),(#221056,#221057),
(#221058,#221059),(#221060,#221061),(#221062,#221063),(#221064,#221065),
(#221066,#221067),(#221068,#221069),(#221070,#221071),(#221072,#221073),
(#221074,#221075),(#221076,#221077),(#221078,#221079),(#221080,#221081),
(#221082,#221083),(#221084,#221085),(#221086,#221087),(#221088,#221089),
(#221090,#221091),(#221092,#221093),(#221094,#221095),(#221096,#221097),
(#221098,#221099),(#221100,#221101),(#221102,#221103),(#221104,#221105),
(#221106,#221107),(#221108,#221109),(#221110,#221111),(#221112,#221113),
(#221114,#221115),(#221116,#221117),(#221118,#221119),(#221120,#221121),
(#221122,#221123),(#221124,#221125),(#221126,#221127),(#221128,#221129),
(#221130,#221131),(#221132,#221133),(#221134,#221135),(#221136,#221137),
(#221138,#221139),(#221140,#221141),(#221142,#221143),(#221144,#221145),
(#221146,#221147),(#221148,#221149),(#221150,#221151),(#221152,#221153),
(#221154,#221155),(#221156,#221157),(#221158,#221159),(#221160,#221161),
(#221162,#221163),(#221164,#221165),(#221166,#221167),(#221168,#221169),
(#221170,#221171),(#221172,#221173),(#221174,#221175),(#221176,#221177),
(#221178,#221179),(#221180,#221181),(#221182,#221183),(#221184,#221185),
(#221186,#221187),(#221188,#221189),(#221190,#221191),(#221192,#221193),
(#221194,#221195),(#221196,#221197),(#221198,#221199),(#221200,#221201),
(#221202,#221203),(#221204,#221205),(#221206,#221207),(#221208,#221209),
(#221210,#221211),(#221212,#221213),(#221214,#221215),(#221216,#221217),
(#221218,#221219),(#221220,#221221),(#221222,#221223),(#221224,#221225),
(#221226,#221227),(#221228,#221229),(#221230,#221231),(#221232,#221233),
(#221234,#221235),(#221236,#221237),(#221238,#221239),(#221240,#221241),
(#221242,#221243),(#221244,#221245),(#221246,#221247),(#221248,#221249),
(#221250,#221251),(#221252,#221253),(#221254,#221255),(#221256,#221257),
(#221258,#221259),(#221260,#221261),(#221262,#221263),(#221264,#221265),
(#221266,#221267),(#221268,#221269),(#221270,#221271),(#221272,#221273),
(#221274,#221275),(#221276,#221277),(#221278,#221279),(#221280,#221281),
(#221282,#221283),(#221284,#221285),(#221286,#221287),(#221288,#221289),
(#221290,#221291),(#221292,#221293),(#221294,#221295),(#221296,#221297),
(#221298,#221299),(#221300,#221301),(#221302,#221303),(#221304,#221305),
(#221306,#221307),(#221308,#221309),(#221310,#221311),(#221312,#221313),
(#221314,#221315),(#221316,#221317),(#221318,#221319),(#221320,#221321),
(#221322,#221323),(#221324,#221325),(#221326,#221327),(#221328,#221329),
(#221330,#221331),(#221332,#221333),(#221334,#221335),(#221336,#221337),
(#221338,#221339),(#221340,#221341),(#221342,#221343),(#221344,#221345),
(#221346,#221347),(#221348,#221349),(#221350,#221351),(#221352,#221353),
(#221354,#221355),(#221356,#221357),(#221358,#221359),(#221360,#221361),
(#221362,#221363),(#221364,#221365),(#221366,#221367),(#221368,#221369),
(#221370,#221371),(#221372,#221373)),.UNSPECIFIED.,.F.,.F.,.F.)
B_SPLINE_SURFACE_WITH_KNOTS((6,1,1,1,1,1,1,1,1,1,1,1,1,1,1,1,1,1,1,1,1,
1,1,1,1,1,1,1,1,1,1,1,1,1,1,1,1,1,1,1,1,1,1,1,1,1,1,1,1,1,1,1,1,1,1,1,1,
1,1,1,1,1,1,1,1,1,1,1,1,1,1,1,1,1,1,1,1,1,1,1,1,1,1,1,1,1,1,1,1,1,1,1,1,
1,1,1,1,1,1,1,1,1,1,1,1,1,1,1,1,1,1,1,1,1,1,1,1,1,1,1,1,1,1,1,1,1,1,1,1,
1,1,1,1,1,1,1,1,1,1,1,1,1,1,1,1,1,1,1,1,1,1,1,1,1,1,1,1,1,1,1,1,1,1,1,1,
1,1,1,1,1,1,1,1,1,1,1,1,1,1,1,1,1,1,1,1,1,1,1,1,1,1,1,1,1,1,1,1,1,1,1,6),
(2,2),(-1.,-0.995000000000001,-0.990000000000001,-0.985000000000001,-0.980000000000001,
-0.975000000000001,-0.970000000000001,-0.965000000000001,-0.960000000000001,
-0.955000000000001,-0.950000000000001,-0.945000000000001,-0.940000000000001,
-0.935000000000001,-0.930000000000001,-0.925000000000001,-0.920000000000001,
-0.915000000000001,-0.910000000000001,-0.905000000000001,-0.900000000000001,
-0.895000000000001,-0.890000000000001,-0.885000000000001,-0.880000000000001,
-0.875000000000001,-0.870000000000001,-0.865000000000001,-0.860000000000001,
-0.855000000000001,-0.850000000000001,-0.845000000000001,-0.840000000000001,
-0.835000000000001,-0.830000000000001,-0.825000000000001,-0.820000000000001,
-0.815000000000001,-0.810000000000001,-0.805000000000001,-0.800000000000001,
-0.795000000000001,-0.790000000000001,-0.785000000000001,-0.780000000000001,
-0.775000000000001,-0.770000000000001,-0.765000000000001,-0.760000000000001,
-0.755000000000001,-0.750000000000001,-0.745000000000001,-0.740000000000001,
-0.735000000000001,-0.730000000000001,-0.725000000000001,-0.720000000000001,
-0.715000000000001,-0.710000000000001,-0.705000000000001,-0.700000000000001,
-0.695000000000001,-0.690000000000001,-0.685,-0.68,-0.675,-0.67,-0.665,
-0.66,-0.655,-0.65,-0.645,-0.64,-0.635,-0.63,-0.625,-0.62,-0.615,-0.61,
-0.605,-0.6,-0.595,-0.59,-0.585,-0.58,-0.575,-0.57,-0.565,-0.56,-0.555,
-0.55,-0.545,-0.54,-0.535,-0.53,-0.525,-0.52,-0.515,-0.51,-0.505,-0.5,-0.495,
-0.49,-0.485,-0.48,-0.475,-0.47,-0.465,-0.46,-0.455,-0.45,-0.445,-0.44,
-0.435,-0.43,-0.425,-0.42,-0.415,-0.41,-0.405,-0.4,-0.395,-0.39,-0.385,
-0.38,-0.375,-0.37,-0.365,-0.36,-0.355,-0.35,-0.345,-0.34,-0.335,-0.33,
-0.325,-0.32,-0.315,-0.31,-0.305,-0.3,-0.295,-0.29,-0.285,-0.28,-0.275,
-0.27,-0.265,-0.26,-0.255,-0.25,-0.245,-0.24,-0.235,-0.23,-0.225,-0.22,
-0.215,-0.21,-0.205,-0.2,-0.195,-0.19,-0.185,-0.18,-0.175,-0.17,-0.165,
-0.16,-0.155,-0.15,-0.145,-0.14,-0.135,-0.13,-0.125,-0.12,-0.115,-0.11,
-0.105,-0.1,-0.095,-0.09,-0.085,-0.08,-0.075,-0.07,-0.065,-0.06,-0.055,
-0.05,-0.045,-0.04,-0.035,-0.03,-0.025,-0.02,-0.015,-0.01,-0.005,0.),(0.,
1.2),.UNSPECIFIED.)
GEOMETRIC_REPRESENTATION_ITEM()
RATIONAL_B_SPLINE_SURFACE(((1.,1.),(1.,1.),(1.,1.),(1.,1.),(1.,1.),(1.,
1.),(1.,1.),(1.,1.),(1.,1.),(1.,1.),(1.,1.),(1.,1.),(1.,1.),(1.,1.),(1.,
1.),(1.,1.),(1.,1.),(1.,1.),(1.,1.),(1.,1.),(1.,1.),(1.,1.),(1.,1.),(1.,
1.),(1.,1.),(1.,1.),(1.,1.),(1.,1.),(1.,1.),(1.,1.),(1.,1.),(1.,1.),(1.,
1.),(1.,1.),(1.,1.),(1.,1.),(1.,1.),(1.,1.),(1.,1.),(1.,1.),(1.,1.),(1.,
1.),(1.,1.),(1.,1.),(1.,1.),(1.,1.),(1.,1.),(1.,1.),(1.,1.),(1.,1.),(1.,
1.),(1.,1.),(1.,1.),(1.,1.),(1.,1.),(1.,1.),(1.,1.),(1.,1.),(1.,1.),(1.,
1.),(1.,1.),(1.,1.),(1.,1.),(1.,1.),(1.,1.),(1.,1.),(1.,1.),(1.,1.),(1.,
1.),(1.,1.),(1.,1.),(1.,1.),(1.,1.),(1.,1.),(1.,1.),(1.,1.),(1.,1.),(1.,
1.),(1.,1.),(1.,1.),(1.,1.),(1.,1.),(1.,1.),(1.,1.),(1.,1.),(1.,1.),(1.,
1.),(1.,1.),(1.,1.),(1.,1.),(1.,1.),(1.,1.),(1.,1.),(1.,1.),(1.,1.),(1.,
1.),(1.,1.),(1.,1.),(1.,1.),(1.,1.),(1.,1.),(1.,1.),(1.,1.),(1.,1.),(1.,
1.),(1.,1.),(1.,1.),(1.,1.),(1.,1.),(1.,1.),(1.,1.),(1.,1.),(1.,1.),(1.,
1.),(1.,1.),(1.,1.),(1.,1.),(1.,1.),(1.,1.),(1.,1.),(1.,1.),(1.,1.),(1.,
1.),(1.,1.),(1.,1.),(1.,1.),(1.,1.),(1.,1.),(1.,1.),(1.,1.),(1.,1.),(1.,
1.),(1.,1.),(1.,1.),(1.,1.),(1.,1.),(1.,1.),(1.,1.),(1.,1.),(1.,1.),(1.,
1.),(1.,1.),(1.,1.),(1.,1.),(1.,1.),(1.,1.),(1.,1.),(1.,1.),(1.,1.),(1.,
1.),(1.,1.),(1.,1.),(1.,1.),(1.,1.),(1.,1.),(1.,1.),(1.,1.),(1.,1.),(1.,
1.),(1.,1.),(1.,1.),(1.,1.),(1.,1.),(1.,1.),(1.,1.),(1.,1.),(1.,1.),(1.,
1.),(1.,1.),(1.,1.),(1.,1.),(1.,1.),(1.,1.),(1.,1.),(1.,1.),(1.,1.),(1.,
1.),(1.,1.),(1.,1.),(1.,1.),(1.,1.),(1.,1.),(1.,1.),(1.,1.),(1.,1.),(1.,
1.),(1.,1.),(1.,1.),(1.,1.),(1.,1.),(1.,1.),(1.,1.),(1.,1.),(1.,1.),(1.,
1.),(1.,1.),(1.,1.),(1.,1.),(1.,1.),(1.,1.),(1.,1.),(1.,1.),(1.,1.),(1.,
1.),(1.,1.)))
REPRESENTATION_ITEM('')
SURFACE()
);
#1082=(
BOUNDED_SURFACE()
B_SPLINE_SURFACE(5,1,((#221787,#221788),(#221789,#221790),(#221791,#221792),
(#221793,#221794),(#221795,#221796),(#221797,#221798),(#221799,#221800),
(#221801,#221802),(#221803,#221804),(#221805,#221806),(#221807,#221808),
(#221809,#221810),(#221811,#221812),(#221813,#221814),(#221815,#221816),
(#221817,#221818),(#221819,#221820),(#221821,#221822),(#221823,#221824),
(#221825,#221826),(#221827,#221828),(#221829,#221830),(#221831,#221832),
(#221833,#221834),(#221835,#221836),(#221837,#221838),(#221839,#221840),
(#221841,#221842),(#221843,#221844),(#221845,#221846),(#221847,#221848),
(#221849,#221850),(#221851,#221852),(#221853,#221854),(#221855,#221856),
(#221857,#221858),(#221859,#221860),(#221861,#221862),(#221863,#221864),
(#221865,#221866),(#221867,#221868),(#221869,#221870),(#221871,#221872),
(#221873,#221874),(#221875,#221876),(#221877,#221878),(#221879,#221880),
(#221881,#221882),(#221883,#221884),(#221885,#221886),(#221887,#221888),
(#221889,#221890),(#221891,#221892),(#221893,#221894),(#221895,#221896),
(#221897,#221898),(#221899,#221900),(#221901,#221902),(#221903,#221904),
(#221905,#221906),(#221907,#221908),(#221909,#221910),(#221911,#221912),
(#221913,#221914),(#221915,#221916),(#221917,#221918),(#221919,#221920),
(#221921,#221922),(#221923,#221924),(#221925,#221926),(#221927,#221928),
(#221929,#221930),(#221931,#221932),(#221933,#221934),(#221935,#221936),
(#221937,#221938),(#221939,#221940),(#221941,#221942),(#221943,#221944),
(#221945,#221946),(#221947,#221948),(#221949,#221950),(#221951,#221952),
(#221953,#221954),(#221955,#221956),(#221957,#221958),(#221959,#221960),
(#221961,#221962),(#221963,#221964),(#221965,#221966),(#221967,#221968),
(#221969,#221970),(#221971,#221972),(#221973,#221974),(#221975,#221976),
(#221977,#221978),(#221979,#221980),(#221981,#221982),(#221983,#221984),
(#221985,#221986),(#221987,#221988),(#221989,#221990),(#221991,#221992),
(#221993,#221994),(#221995,#221996),(#221997,#221998),(#221999,#222000),
(#222001,#222002),(#222003,#222004),(#222005,#222006),(#222007,#222008),
(#222009,#222010),(#222011,#222012),(#222013,#222014),(#222015,#222016),
(#222017,#222018),(#222019,#222020),(#222021,#222022),(#222023,#222024),
(#222025,#222026),(#222027,#222028),(#222029,#222030),(#222031,#222032),
(#222033,#222034),(#222035,#222036),(#222037,#222038),(#222039,#222040),
(#222041,#222042),(#222043,#222044),(#222045,#222046),(#222047,#222048),
(#222049,#222050),(#222051,#222052),(#222053,#222054),(#222055,#222056),
(#222057,#222058),(#222059,#222060),(#222061,#222062),(#222063,#222064),
(#222065,#222066),(#222067,#222068),(#222069,#222070),(#222071,#222072),
(#222073,#222074),(#222075,#222076),(#222077,#222078),(#222079,#222080),
(#222081,#222082),(#222083,#222084),(#222085,#222086),(#222087,#222088),
(#222089,#222090),(#222091,#222092),(#222093,#222094),(#222095,#222096),
(#222097,#222098),(#222099,#222100),(#222101,#222102),(#222103,#222104),
(#222105,#222106),(#222107,#222108),(#222109,#222110),(#222111,#222112),
(#222113,#222114),(#222115,#222116),(#222117,#222118),(#222119,#222120),
(#222121,#222122),(#222123,#222124),(#222125,#222126),(#222127,#222128),
(#222129,#222130),(#222131,#222132),(#222133,#222134),(#222135,#222136),
(#222137,#222138),(#222139,#222140),(#222141,#222142),(#222143,#222144),
(#222145,#222146),(#222147,#222148),(#222149,#222150),(#222151,#222152),
(#222153,#222154),(#222155,#222156),(#222157,#222158),(#222159,#222160),
(#222161,#222162),(#222163,#222164),(#222165,#222166),(#222167,#222168),
(#222169,#222170),(#222171,#222172),(#222173,#222174),(#222175,#222176),
(#222177,#222178),(#222179,#222180),(#222181,#222182),(#222183,#222184),
(#222185,#222186),(#222187,#222188),(#222189,#222190),(#222191,#222192),
(#222193,#222194),(#222195,#222196)),.UNSPECIFIED.,.F.,.F.,.F.)
B_SPLINE_SURFACE_WITH_KNOTS((6,1,1,1,1,1,1,1,1,1,1,1,1,1,1,1,1,1,1,1,1,
1,1,1,1,1,1,1,1,1,1,1,1,1,1,1,1,1,1,1,1,1,1,1,1,1,1,1,1,1,1,1,1,1,1,1,1,
1,1,1,1,1,1,1,1,1,1,1,1,1,1,1,1,1,1,1,1,1,1,1,1,1,1,1,1,1,1,1,1,1,1,1,1,
1,1,1,1,1,1,1,1,1,1,1,1,1,1,1,1,1,1,1,1,1,1,1,1,1,1,1,1,1,1,1,1,1,1,1,1,
1,1,1,1,1,1,1,1,1,1,1,1,1,1,1,1,1,1,1,1,1,1,1,1,1,1,1,1,1,1,1,1,1,1,1,1,
1,1,1,1,1,1,1,1,1,1,1,1,1,1,1,1,1,1,1,1,1,1,1,1,1,1,1,1,1,1,1,1,1,1,1,6),
(2,2),(0.,0.005,0.01,0.015,0.02,0.025,0.03,0.035,0.04,0.045,0.05,0.055,
0.06,0.065,0.07,0.075,0.08,0.085,0.09,0.095,0.1,0.105,0.11,0.115,0.12,0.125,
0.13,0.135,0.14,0.145,0.15,0.155,0.16,0.165,0.17,0.175,0.18,0.185,0.19,
0.195,0.2,0.205,0.21,0.215,0.22,0.225,0.23,0.235,0.24,0.245,0.25,0.255,
0.26,0.265,0.27,0.275,0.28,0.285,0.29,0.295,0.3,0.305,0.31,0.315,0.32,0.325,
0.33,0.335,0.34,0.345,0.35,0.355,0.36,0.365,0.37,0.375,0.38,0.385,0.39,
0.395,0.4,0.405,0.41,0.415,0.42,0.425,0.43,0.435,0.44,0.445,0.45,0.455,
0.46,0.465,0.47,0.475,0.48,0.485,0.49,0.495,0.5,0.505,0.51,0.515,0.52,0.525,
0.53,0.535,0.54,0.545,0.55,0.555,0.56,0.565,0.57,0.575,0.58,0.585,0.59,
0.595,0.6,0.605,0.61,0.615,0.62,0.625,0.63,0.635,0.64,0.645,0.65,0.655,
0.66,0.665,0.67,0.675,0.68,0.685,0.690000000000001,0.695000000000001,0.700000000000001,
0.705000000000001,0.710000000000001,0.715000000000001,0.720000000000001,
0.725000000000001,0.730000000000001,0.735000000000001,0.740000000000001,
0.745000000000001,0.750000000000001,0.755000000000001,0.760000000000001,
0.765000000000001,0.770000000000001,0.775000000000001,0.780000000000001,
0.785000000000001,0.790000000000001,0.795000000000001,0.800000000000001,
0.805000000000001,0.810000000000001,0.815000000000001,0.820000000000001,
0.825000000000001,0.830000000000001,0.835000000000001,0.840000000000001,
0.845000000000001,0.850000000000001,0.855000000000001,0.860000000000001,
0.865000000000001,0.870000000000001,0.875000000000001,0.880000000000001,
0.885000000000001,0.890000000000001,0.895000000000001,0.900000000000001,
0.905000000000001,0.910000000000001,0.915000000000001,0.920000000000001,
0.925000000000001,0.930000000000001,0.935000000000001,0.940000000000001,
0.945000000000001,0.950000000000001,0.955000000000001,0.960000000000001,
0.965000000000001,0.970000000000001,0.975000000000001,0.980000000000001,
0.985000000000001,0.990000000000001,0.995000000000001,1.),(0.,1.2),
 .UNSPECIFIED.)
GEOMETRIC_REPRESENTATION_ITEM()
RATIONAL_B_SPLINE_SURFACE(((1.,1.),(1.,1.),(1.,1.),(1.,1.),(1.,1.),(1.,
1.),(1.,1.),(1.,1.),(1.,1.),(1.,1.),(1.,1.),(1.,1.),(1.,1.),(1.,1.),(1.,
1.),(1.,1.),(1.,1.),(1.,1.),(1.,1.),(1.,1.),(1.,1.),(1.,1.),(1.,1.),(1.,
1.),(1.,1.),(1.,1.),(1.,1.),(1.,1.),(1.,1.),(1.,1.),(1.,1.),(1.,1.),(1.,
1.),(1.,1.),(1.,1.),(1.,1.),(1.,1.),(1.,1.),(1.,1.),(1.,1.),(1.,1.),(1.,
1.),(1.,1.),(1.,1.),(1.,1.),(1.,1.),(1.,1.),(1.,1.),(1.,1.),(1.,1.),(1.,
1.),(1.,1.),(1.,1.),(1.,1.),(1.,1.),(1.,1.),(1.,1.),(1.,1.),(1.,1.),(1.,
1.),(1.,1.),(1.,1.),(1.,1.),(1.,1.),(1.,1.),(1.,1.),(1.,1.),(1.,1.),(1.,
1.),(1.,1.),(1.,1.),(1.,1.),(1.,1.),(1.,1.),(1.,1.),(1.,1.),(1.,1.),(1.,
1.),(1.,1.),(1.,1.),(1.,1.),(1.,1.),(1.,1.),(1.,1.),(1.,1.),(1.,1.),(1.,
1.),(1.,1.),(1.,1.),(1.,1.),(1.,1.),(1.,1.),(1.,1.),(1.,1.),(1.,1.),(1.,
1.),(1.,1.),(1.,1.),(1.,1.),(1.,1.),(1.,1.),(1.,1.),(1.,1.),(1.,1.),(1.,
1.),(1.,1.),(1.,1.),(1.,1.),(1.,1.),(1.,1.),(1.,1.),(1.,1.),(1.,1.),(1.,
1.),(1.,1.),(1.,1.),(1.,1.),(1.,1.),(1.,1.),(1.,1.),(1.,1.),(1.,1.),(1.,
1.),(1.,1.),(1.,1.),(1.,1.),(1.,1.),(1.,1.),(1.,1.),(1.,1.),(1.,1.),(1.,
1.),(1.,1.),(1.,1.),(1.,1.),(1.,1.),(1.,1.),(1.,1.),(1.,1.),(1.,1.),(1.,
1.),(1.,1.),(1.,1.),(1.,1.),(1.,1.),(1.,1.),(1.,1.),(1.,1.),(1.,1.),(1.,
1.),(1.,1.),(1.,1.),(1.,1.),(1.,1.),(1.,1.),(1.,1.),(1.,1.),(1.,1.),(1.,
1.),(1.,1.),(1.,1.),(1.,1.),(1.,1.),(1.,1.),(1.,1.),(1.,1.),(1.,1.),(1.,
1.),(1.,1.),(1.,1.),(1.,1.),(1.,1.),(1.,1.),(1.,1.),(1.,1.),(1.,1.),(1.,
1.),(1.,1.),(1.,1.),(1.,1.),(1.,1.),(1.,1.),(1.,1.),(1.,1.),(1.,1.),(1.,
1.),(1.,1.),(1.,1.),(1.,1.),(1.,1.),(1.,1.),(1.,1.),(1.,1.),(1.,1.),(1.,
1.),(1.,1.),(1.,1.),(1.,1.),(1.,1.),(1.,1.),(1.,1.),(1.,1.),(1.,1.),(1.,
1.),(1.,1.)))
REPRESENTATION_ITEM('')
SURFACE()
);
#1083=(
BOUNDED_SURFACE()
B_SPLINE_SURFACE(5,1,((#222616,#222617),(#222618,#222619),(#222620,#222621),
(#222622,#222623),(#222624,#222625),(#222626,#222627),(#222628,#222629),
(#222630,#222631),(#222632,#222633),(#222634,#222635),(#222636,#222637),
(#222638,#222639),(#222640,#222641),(#222642,#222643),(#222644,#222645),
(#222646,#222647),(#222648,#222649),(#222650,#222651),(#222652,#222653),
(#222654,#222655),(#222656,#222657),(#222658,#222659),(#222660,#222661),
(#222662,#222663),(#222664,#222665),(#222666,#222667),(#222668,#222669),
(#222670,#222671),(#222672,#222673),(#222674,#222675),(#222676,#222677),
(#222678,#222679),(#222680,#222681),(#222682,#222683),(#222684,#222685),
(#222686,#222687),(#222688,#222689),(#222690,#222691),(#222692,#222693),
(#222694,#222695),(#222696,#222697),(#222698,#222699),(#222700,#222701),
(#222702,#222703),(#222704,#222705),(#222706,#222707),(#222708,#222709),
(#222710,#222711),(#222712,#222713),(#222714,#222715),(#222716,#222717),
(#222718,#222719),(#222720,#222721),(#222722,#222723),(#222724,#222725),
(#222726,#222727),(#222728,#222729),(#222730,#222731),(#222732,#222733),
(#222734,#222735),(#222736,#222737),(#222738,#222739),(#222740,#222741),
(#222742,#222743),(#222744,#222745),(#222746,#222747),(#222748,#222749),
(#222750,#222751),(#222752,#222753),(#222754,#222755),(#222756,#222757),
(#222758,#222759),(#222760,#222761),(#222762,#222763),(#222764,#222765),
(#222766,#222767),(#222768,#222769),(#222770,#222771),(#222772,#222773),
(#222774,#222775),(#222776,#222777),(#222778,#222779),(#222780,#222781),
(#222782,#222783),(#222784,#222785),(#222786,#222787),(#222788,#222789),
(#222790,#222791),(#222792,#222793),(#222794,#222795),(#222796,#222797),
(#222798,#222799),(#222800,#222801),(#222802,#222803),(#222804,#222805),
(#222806,#222807),(#222808,#222809),(#222810,#222811),(#222812,#222813),
(#222814,#222815),(#222816,#222817),(#222818,#222819),(#222820,#222821),
(#222822,#222823),(#222824,#222825),(#222826,#222827),(#222828,#222829),
(#222830,#222831),(#222832,#222833),(#222834,#222835),(#222836,#222837),
(#222838,#222839),(#222840,#222841),(#222842,#222843),(#222844,#222845),
(#222846,#222847),(#222848,#222849),(#222850,#222851),(#222852,#222853),
(#222854,#222855),(#222856,#222857),(#222858,#222859),(#222860,#222861),
(#222862,#222863),(#222864,#222865),(#222866,#222867),(#222868,#222869),
(#222870,#222871),(#222872,#222873),(#222874,#222875),(#222876,#222877),
(#222878,#222879),(#222880,#222881),(#222882,#222883),(#222884,#222885),
(#222886,#222887),(#222888,#222889),(#222890,#222891),(#222892,#222893),
(#222894,#222895),(#222896,#222897),(#222898,#222899),(#222900,#222901),
(#222902,#222903),(#222904,#222905),(#222906,#222907),(#222908,#222909),
(#222910,#222911),(#222912,#222913),(#222914,#222915),(#222916,#222917),
(#222918,#222919),(#222920,#222921),(#222922,#222923),(#222924,#222925),
(#222926,#222927),(#222928,#222929),(#222930,#222931),(#222932,#222933),
(#222934,#222935),(#222936,#222937),(#222938,#222939),(#222940,#222941),
(#222942,#222943),(#222944,#222945),(#222946,#222947),(#222948,#222949),
(#222950,#222951),(#222952,#222953),(#222954,#222955),(#222956,#222957),
(#222958,#222959),(#222960,#222961),(#222962,#222963),(#222964,#222965),
(#222966,#222967),(#222968,#222969),(#222970,#222971),(#222972,#222973),
(#222974,#222975),(#222976,#222977),(#222978,#222979),(#222980,#222981),
(#222982,#222983),(#222984,#222985),(#222986,#222987),(#222988,#222989),
(#222990,#222991),(#222992,#222993),(#222994,#222995),(#222996,#222997),
(#222998,#222999),(#223000,#223001),(#223002,#223003),(#223004,#223005),
(#223006,#223007),(#223008,#223009),(#223010,#223011),(#223012,#223013),
(#223014,#223015),(#223016,#223017),(#223018,#223019),(#223020,#223021),
(#223022,#223023),(#223024,#223025)),.UNSPECIFIED.,.F.,.F.,.F.)
B_SPLINE_SURFACE_WITH_KNOTS((6,1,1,1,1,1,1,1,1,1,1,1,1,1,1,1,1,1,1,1,1,
1,1,1,1,1,1,1,1,1,1,1,1,1,1,1,1,1,1,1,1,1,1,1,1,1,1,1,1,1,1,1,1,1,1,1,1,
1,1,1,1,1,1,1,1,1,1,1,1,1,1,1,1,1,1,1,1,1,1,1,1,1,1,1,1,1,1,1,1,1,1,1,1,
1,1,1,1,1,1,1,1,1,1,1,1,1,1,1,1,1,1,1,1,1,1,1,1,1,1,1,1,1,1,1,1,1,1,1,1,
1,1,1,1,1,1,1,1,1,1,1,1,1,1,1,1,1,1,1,1,1,1,1,1,1,1,1,1,1,1,1,1,1,1,1,1,
1,1,1,1,1,1,1,1,1,1,1,1,1,1,1,1,1,1,1,1,1,1,1,1,1,1,1,1,1,1,1,1,1,1,1,6),
(2,2),(-1.,-0.995000000000001,-0.990000000000001,-0.985000000000001,-0.980000000000001,
-0.975000000000001,-0.970000000000001,-0.965000000000001,-0.960000000000001,
-0.955000000000001,-0.950000000000001,-0.945000000000001,-0.940000000000001,
-0.935000000000001,-0.930000000000001,-0.925000000000001,-0.920000000000001,
-0.915000000000001,-0.910000000000001,-0.905000000000001,-0.900000000000001,
-0.895000000000001,-0.890000000000001,-0.885000000000001,-0.880000000000001,
-0.875000000000001,-0.870000000000001,-0.865000000000001,-0.860000000000001,
-0.855000000000001,-0.850000000000001,-0.845000000000001,-0.840000000000001,
-0.835000000000001,-0.830000000000001,-0.825000000000001,-0.820000000000001,
-0.815000000000001,-0.810000000000001,-0.805000000000001,-0.800000000000001,
-0.795000000000001,-0.790000000000001,-0.785000000000001,-0.780000000000001,
-0.775000000000001,-0.770000000000001,-0.765000000000001,-0.760000000000001,
-0.755000000000001,-0.750000000000001,-0.745000000000001,-0.740000000000001,
-0.735000000000001,-0.730000000000001,-0.725000000000001,-0.720000000000001,
-0.715000000000001,-0.710000000000001,-0.705000000000001,-0.700000000000001,
-0.695000000000001,-0.690000000000001,-0.685,-0.68,-0.675,-0.67,-0.665,
-0.66,-0.655,-0.65,-0.645,-0.64,-0.635,-0.63,-0.625,-0.62,-0.615,-0.61,
-0.605,-0.6,-0.595,-0.59,-0.585,-0.58,-0.575,-0.57,-0.565,-0.56,-0.555,
-0.55,-0.545,-0.54,-0.535,-0.53,-0.525,-0.52,-0.515,-0.51,-0.505,-0.5,-0.495,
-0.49,-0.485,-0.48,-0.475,-0.47,-0.465,-0.46,-0.455,-0.45,-0.445,-0.44,
-0.435,-0.43,-0.425,-0.42,-0.415,-0.41,-0.405,-0.4,-0.395,-0.39,-0.385,
-0.38,-0.375,-0.37,-0.365,-0.36,-0.355,-0.35,-0.345,-0.34,-0.335,-0.33,
-0.325,-0.32,-0.315,-0.31,-0.305,-0.3,-0.295,-0.29,-0.285,-0.28,-0.275,
-0.27,-0.265,-0.26,-0.255,-0.25,-0.245,-0.24,-0.235,-0.23,-0.225,-0.22,
-0.215,-0.21,-0.205,-0.2,-0.195,-0.19,-0.185,-0.18,-0.175,-0.17,-0.165,
-0.16,-0.155,-0.15,-0.145,-0.14,-0.135,-0.13,-0.125,-0.12,-0.115,-0.11,
-0.105,-0.1,-0.095,-0.09,-0.085,-0.08,-0.075,-0.07,-0.065,-0.06,-0.055,
-0.05,-0.045,-0.04,-0.035,-0.03,-0.025,-0.02,-0.015,-0.01,-0.005,0.),(0.,
1.2),.UNSPECIFIED.)
GEOMETRIC_REPRESENTATION_ITEM()
RATIONAL_B_SPLINE_SURFACE(((1.,1.),(1.,1.),(1.,1.),(1.,1.),(1.,1.),(1.,
1.),(1.,1.),(1.,1.),(1.,1.),(1.,1.),(1.,1.),(1.,1.),(1.,1.),(1.,1.),(1.,
1.),(1.,1.),(1.,1.),(1.,1.),(1.,1.),(1.,1.),(1.,1.),(1.,1.),(1.,1.),(1.,
1.),(1.,1.),(1.,1.),(1.,1.),(1.,1.),(1.,1.),(1.,1.),(1.,1.),(1.,1.),(1.,
1.),(1.,1.),(1.,1.),(1.,1.),(1.,1.),(1.,1.),(1.,1.),(1.,1.),(1.,1.),(1.,
1.),(1.,1.),(1.,1.),(1.,1.),(1.,1.),(1.,1.),(1.,1.),(1.,1.),(1.,1.),(1.,
1.),(1.,1.),(1.,1.),(1.,1.),(1.,1.),(1.,1.),(1.,1.),(1.,1.),(1.,1.),(1.,
1.),(1.,1.),(1.,1.),(1.,1.),(1.,1.),(1.,1.),(1.,1.),(1.,1.),(1.,1.),(1.,
1.),(1.,1.),(1.,1.),(1.,1.),(1.,1.),(1.,1.),(1.,1.),(1.,1.),(1.,1.),(1.,
1.),(1.,1.),(1.,1.),(1.,1.),(1.,1.),(1.,1.),(1.,1.),(1.,1.),(1.,1.),(1.,
1.),(1.,1.),(1.,1.),(1.,1.),(1.,1.),(1.,1.),(1.,1.),(1.,1.),(1.,1.),(1.,
1.),(1.,1.),(1.,1.),(1.,1.),(1.,1.),(1.,1.),(1.,1.),(1.,1.),(1.,1.),(1.,
1.),(1.,1.),(1.,1.),(1.,1.),(1.,1.),(1.,1.),(1.,1.),(1.,1.),(1.,1.),(1.,
1.),(1.,1.),(1.,1.),(1.,1.),(1.,1.),(1.,1.),(1.,1.),(1.,1.),(1.,1.),(1.,
1.),(1.,1.),(1.,1.),(1.,1.),(1.,1.),(1.,1.),(1.,1.),(1.,1.),(1.,1.),(1.,
1.),(1.,1.),(1.,1.),(1.,1.),(1.,1.),(1.,1.),(1.,1.),(1.,1.),(1.,1.),(1.,
1.),(1.,1.),(1.,1.),(1.,1.),(1.,1.),(1.,1.),(1.,1.),(1.,1.),(1.,1.),(1.,
1.),(1.,1.),(1.,1.),(1.,1.),(1.,1.),(1.,1.),(1.,1.),(1.,1.),(1.,1.),(1.,
1.),(1.,1.),(1.,1.),(1.,1.),(1.,1.),(1.,1.),(1.,1.),(1.,1.),(1.,1.),(1.,
1.),(1.,1.),(1.,1.),(1.,1.),(1.,1.),(1.,1.),(1.,1.),(1.,1.),(1.,1.),(1.,
1.),(1.,1.),(1.,1.),(1.,1.),(1.,1.),(1.,1.),(1.,1.),(1.,1.),(1.,1.),(1.,
1.),(1.,1.),(1.,1.),(1.,1.),(1.,1.),(1.,1.),(1.,1.),(1.,1.),(1.,1.),(1.,
1.),(1.,1.),(1.,1.),(1.,1.),(1.,1.),(1.,1.),(1.,1.),(1.,1.),(1.,1.),(1.,
1.),(1.,1.)))
REPRESENTATION_ITEM('')
SURFACE()
);
#1084=(
BOUNDED_SURFACE()
B_SPLINE_SURFACE(5,1,((#223439,#223440),(#223441,#223442),(#223443,#223444),
(#223445,#223446),(#223447,#223448),(#223449,#223450),(#223451,#223452),
(#223453,#223454),(#223455,#223456),(#223457,#223458),(#223459,#223460),
(#223461,#223462),(#223463,#223464),(#223465,#223466),(#223467,#223468),
(#223469,#223470),(#223471,#223472),(#223473,#223474),(#223475,#223476),
(#223477,#223478),(#223479,#223480),(#223481,#223482),(#223483,#223484),
(#223485,#223486),(#223487,#223488),(#223489,#223490),(#223491,#223492),
(#223493,#223494),(#223495,#223496),(#223497,#223498),(#223499,#223500),
(#223501,#223502),(#223503,#223504),(#223505,#223506),(#223507,#223508),
(#223509,#223510),(#223511,#223512),(#223513,#223514),(#223515,#223516),
(#223517,#223518),(#223519,#223520),(#223521,#223522),(#223523,#223524),
(#223525,#223526),(#223527,#223528),(#223529,#223530),(#223531,#223532),
(#223533,#223534),(#223535,#223536),(#223537,#223538),(#223539,#223540),
(#223541,#223542),(#223543,#223544),(#223545,#223546),(#223547,#223548),
(#223549,#223550),(#223551,#223552),(#223553,#223554),(#223555,#223556),
(#223557,#223558),(#223559,#223560),(#223561,#223562),(#223563,#223564),
(#223565,#223566),(#223567,#223568),(#223569,#223570),(#223571,#223572),
(#223573,#223574),(#223575,#223576),(#223577,#223578),(#223579,#223580),
(#223581,#223582),(#223583,#223584),(#223585,#223586),(#223587,#223588),
(#223589,#223590),(#223591,#223592),(#223593,#223594),(#223595,#223596),
(#223597,#223598),(#223599,#223600),(#223601,#223602),(#223603,#223604),
(#223605,#223606),(#223607,#223608),(#223609,#223610),(#223611,#223612),
(#223613,#223614),(#223615,#223616),(#223617,#223618),(#223619,#223620),
(#223621,#223622),(#223623,#223624),(#223625,#223626),(#223627,#223628),
(#223629,#223630),(#223631,#223632),(#223633,#223634),(#223635,#223636),
(#223637,#223638),(#223639,#223640),(#223641,#223642),(#223643,#223644),
(#223645,#223646),(#223647,#223648),(#223649,#223650),(#223651,#223652),
(#223653,#223654),(#223655,#223656),(#223657,#223658),(#223659,#223660),
(#223661,#223662),(#223663,#223664),(#223665,#223666),(#223667,#223668),
(#223669,#223670),(#223671,#223672),(#223673,#223674),(#223675,#223676),
(#223677,#223678),(#223679,#223680),(#223681,#223682),(#223683,#223684),
(#223685,#223686),(#223687,#223688),(#223689,#223690),(#223691,#223692),
(#223693,#223694),(#223695,#223696),(#223697,#223698),(#223699,#223700),
(#223701,#223702),(#223703,#223704),(#223705,#223706),(#223707,#223708),
(#223709,#223710),(#223711,#223712),(#223713,#223714),(#223715,#223716),
(#223717,#223718),(#223719,#223720),(#223721,#223722),(#223723,#223724),
(#223725,#223726),(#223727,#223728),(#223729,#223730),(#223731,#223732),
(#223733,#223734),(#223735,#223736),(#223737,#223738),(#223739,#223740),
(#223741,#223742),(#223743,#223744),(#223745,#223746),(#223747,#223748),
(#223749,#223750),(#223751,#223752),(#223753,#223754),(#223755,#223756),
(#223757,#223758),(#223759,#223760),(#223761,#223762),(#223763,#223764),
(#223765,#223766),(#223767,#223768),(#223769,#223770),(#223771,#223772),
(#223773,#223774),(#223775,#223776),(#223777,#223778),(#223779,#223780),
(#223781,#223782),(#223783,#223784),(#223785,#223786),(#223787,#223788),
(#223789,#223790),(#223791,#223792),(#223793,#223794),(#223795,#223796),
(#223797,#223798),(#223799,#223800),(#223801,#223802),(#223803,#223804),
(#223805,#223806),(#223807,#223808),(#223809,#223810),(#223811,#223812),
(#223813,#223814),(#223815,#223816),(#223817,#223818),(#223819,#223820),
(#223821,#223822),(#223823,#223824),(#223825,#223826),(#223827,#223828),
(#223829,#223830),(#223831,#223832),(#223833,#223834),(#223835,#223836),
(#223837,#223838),(#223839,#223840),(#223841,#223842),(#223843,#223844),
(#223845,#223846),(#223847,#223848)),.UNSPECIFIED.,.F.,.F.,.F.)
B_SPLINE_SURFACE_WITH_KNOTS((6,1,1,1,1,1,1,1,1,1,1,1,1,1,1,1,1,1,1,1,1,
1,1,1,1,1,1,1,1,1,1,1,1,1,1,1,1,1,1,1,1,1,1,1,1,1,1,1,1,1,1,1,1,1,1,1,1,
1,1,1,1,1,1,1,1,1,1,1,1,1,1,1,1,1,1,1,1,1,1,1,1,1,1,1,1,1,1,1,1,1,1,1,1,
1,1,1,1,1,1,1,1,1,1,1,1,1,1,1,1,1,1,1,1,1,1,1,1,1,1,1,1,1,1,1,1,1,1,1,1,
1,1,1,1,1,1,1,1,1,1,1,1,1,1,1,1,1,1,1,1,1,1,1,1,1,1,1,1,1,1,1,1,1,1,1,1,
1,1,1,1,1,1,1,1,1,1,1,1,1,1,1,1,1,1,1,1,1,1,1,1,1,1,1,1,1,1,1,1,1,1,1,6),
(2,2),(0.,0.005,0.01,0.015,0.02,0.025,0.03,0.035,0.04,0.045,0.05,0.055,
0.06,0.065,0.07,0.075,0.08,0.085,0.09,0.095,0.1,0.105,0.11,0.115,0.12,0.125,
0.13,0.135,0.14,0.145,0.15,0.155,0.16,0.165,0.17,0.175,0.18,0.185,0.19,
0.195,0.2,0.205,0.21,0.215,0.22,0.225,0.23,0.235,0.24,0.245,0.25,0.255,
0.26,0.265,0.27,0.275,0.28,0.285,0.29,0.295,0.3,0.305,0.31,0.315,0.32,0.325,
0.33,0.335,0.34,0.345,0.35,0.355,0.36,0.365,0.37,0.375,0.38,0.385,0.39,
0.395,0.4,0.405,0.41,0.415,0.42,0.425,0.43,0.435,0.44,0.445,0.45,0.455,
0.46,0.465,0.47,0.475,0.48,0.485,0.49,0.495,0.5,0.505,0.51,0.515,0.52,0.525,
0.53,0.535,0.54,0.545,0.55,0.555,0.56,0.565,0.57,0.575,0.58,0.585,0.59,
0.595,0.6,0.605,0.61,0.615,0.62,0.625,0.63,0.635,0.64,0.645,0.65,0.655,
0.66,0.665,0.67,0.675,0.68,0.685,0.690000000000001,0.695000000000001,0.700000000000001,
0.705000000000001,0.710000000000001,0.715000000000001,0.720000000000001,
0.725000000000001,0.730000000000001,0.735000000000001,0.740000000000001,
0.745000000000001,0.750000000000001,0.755000000000001,0.760000000000001,
0.765000000000001,0.770000000000001,0.775000000000001,0.780000000000001,
0.785000000000001,0.790000000000001,0.795000000000001,0.800000000000001,
0.805000000000001,0.810000000000001,0.815000000000001,0.820000000000001,
0.825000000000001,0.830000000000001,0.835000000000001,0.840000000000001,
0.845000000000001,0.850000000000001,0.855000000000001,0.860000000000001,
0.865000000000001,0.870000000000001,0.875000000000001,0.880000000000001,
0.885000000000001,0.890000000000001,0.895000000000001,0.900000000000001,
0.905000000000001,0.910000000000001,0.915000000000001,0.920000000000001,
0.925000000000001,0.930000000000001,0.935000000000001,0.940000000000001,
0.945000000000001,0.950000000000001,0.955000000000001,0.960000000000001,
0.965000000000001,0.970000000000001,0.975000000000001,0.980000000000001,
0.985000000000001,0.990000000000001,0.995000000000001,1.),(0.,1.2),
 .UNSPECIFIED.)
GEOMETRIC_REPRESENTATION_ITEM()
RATIONAL_B_SPLINE_SURFACE(((1.,1.),(1.,1.),(1.,1.),(1.,1.),(1.,1.),(1.,
1.),(1.,1.),(1.,1.),(1.,1.),(1.,1.),(1.,1.),(1.,1.),(1.,1.),(1.,1.),(1.,
1.),(1.,1.),(1.,1.),(1.,1.),(1.,1.),(1.,1.),(1.,1.),(1.,1.),(1.,1.),(1.,
1.),(1.,1.),(1.,1.),(1.,1.),(1.,1.),(1.,1.),(1.,1.),(1.,1.),(1.,1.),(1.,
1.),(1.,1.),(1.,1.),(1.,1.),(1.,1.),(1.,1.),(1.,1.),(1.,1.),(1.,1.),(1.,
1.),(1.,1.),(1.,1.),(1.,1.),(1.,1.),(1.,1.),(1.,1.),(1.,1.),(1.,1.),(1.,
1.),(1.,1.),(1.,1.),(1.,1.),(1.,1.),(1.,1.),(1.,1.),(1.,1.),(1.,1.),(1.,
1.),(1.,1.),(1.,1.),(1.,1.),(1.,1.),(1.,1.),(1.,1.),(1.,1.),(1.,1.),(1.,
1.),(1.,1.),(1.,1.),(1.,1.),(1.,1.),(1.,1.),(1.,1.),(1.,1.),(1.,1.),(1.,
1.),(1.,1.),(1.,1.),(1.,1.),(1.,1.),(1.,1.),(1.,1.),(1.,1.),(1.,1.),(1.,
1.),(1.,1.),(1.,1.),(1.,1.),(1.,1.),(1.,1.),(1.,1.),(1.,1.),(1.,1.),(1.,
1.),(1.,1.),(1.,1.),(1.,1.),(1.,1.),(1.,1.),(1.,1.),(1.,1.),(1.,1.),(1.,
1.),(1.,1.),(1.,1.),(1.,1.),(1.,1.),(1.,1.),(1.,1.),(1.,1.),(1.,1.),(1.,
1.),(1.,1.),(1.,1.),(1.,1.),(1.,1.),(1.,1.),(1.,1.),(1.,1.),(1.,1.),(1.,
1.),(1.,1.),(1.,1.),(1.,1.),(1.,1.),(1.,1.),(1.,1.),(1.,1.),(1.,1.),(1.,
1.),(1.,1.),(1.,1.),(1.,1.),(1.,1.),(1.,1.),(1.,1.),(1.,1.),(1.,1.),(1.,
1.),(1.,1.),(1.,1.),(1.,1.),(1.,1.),(1.,1.),(1.,1.),(1.,1.),(1.,1.),(1.,
1.),(1.,1.),(1.,1.),(1.,1.),(1.,1.),(1.,1.),(1.,1.),(1.,1.),(1.,1.),(1.,
1.),(1.,1.),(1.,1.),(1.,1.),(1.,1.),(1.,1.),(1.,1.),(1.,1.),(1.,1.),(1.,
1.),(1.,1.),(1.,1.),(1.,1.),(1.,1.),(1.,1.),(1.,1.),(1.,1.),(1.,1.),(1.,
1.),(1.,1.),(1.,1.),(1.,1.),(1.,1.),(1.,1.),(1.,1.),(1.,1.),(1.,1.),(1.,
1.),(1.,1.),(1.,1.),(1.,1.),(1.,1.),(1.,1.),(1.,1.),(1.,1.),(1.,1.),(1.,
1.),(1.,1.),(1.,1.),(1.,1.),(1.,1.),(1.,1.),(1.,1.),(1.,1.),(1.,1.),(1.,
1.),(1.,1.)))
REPRESENTATION_ITEM('')
SURFACE()
);
#1085=(
BOUNDED_SURFACE()
B_SPLINE_SURFACE(5,1,((#224268,#224269),(#224270,#224271),(#224272,#224273),
(#224274,#224275),(#224276,#224277),(#224278,#224279),(#224280,#224281),
(#224282,#224283),(#224284,#224285),(#224286,#224287),(#224288,#224289),
(#224290,#224291),(#224292,#224293),(#224294,#224295),(#224296,#224297),
(#224298,#224299),(#224300,#224301),(#224302,#224303),(#224304,#224305),
(#224306,#224307),(#224308,#224309),(#224310,#224311),(#224312,#224313),
(#224314,#224315),(#224316,#224317),(#224318,#224319),(#224320,#224321),
(#224322,#224323),(#224324,#224325),(#224326,#224327),(#224328,#224329),
(#224330,#224331),(#224332,#224333),(#224334,#224335),(#224336,#224337),
(#224338,#224339),(#224340,#224341),(#224342,#224343),(#224344,#224345),
(#224346,#224347),(#224348,#224349),(#224350,#224351),(#224352,#224353),
(#224354,#224355),(#224356,#224357),(#224358,#224359),(#224360,#224361),
(#224362,#224363),(#224364,#224365),(#224366,#224367),(#224368,#224369),
(#224370,#224371),(#224372,#224373),(#224374,#224375),(#224376,#224377),
(#224378,#224379),(#224380,#224381),(#224382,#224383),(#224384,#224385),
(#224386,#224387),(#224388,#224389),(#224390,#224391),(#224392,#224393),
(#224394,#224395),(#224396,#224397),(#224398,#224399),(#224400,#224401),
(#224402,#224403),(#224404,#224405),(#224406,#224407),(#224408,#224409),
(#224410,#224411),(#224412,#224413),(#224414,#224415),(#224416,#224417),
(#224418,#224419),(#224420,#224421),(#224422,#224423),(#224424,#224425),
(#224426,#224427),(#224428,#224429),(#224430,#224431),(#224432,#224433),
(#224434,#224435),(#224436,#224437),(#224438,#224439),(#224440,#224441),
(#224442,#224443),(#224444,#224445),(#224446,#224447),(#224448,#224449),
(#224450,#224451),(#224452,#224453),(#224454,#224455),(#224456,#224457),
(#224458,#224459),(#224460,#224461),(#224462,#224463),(#224464,#224465),
(#224466,#224467),(#224468,#224469),(#224470,#224471),(#224472,#224473),
(#224474,#224475),(#224476,#224477),(#224478,#224479),(#224480,#224481),
(#224482,#224483),(#224484,#224485),(#224486,#224487),(#224488,#224489),
(#224490,#224491),(#224492,#224493),(#224494,#224495),(#224496,#224497),
(#224498,#224499),(#224500,#224501),(#224502,#224503),(#224504,#224505),
(#224506,#224507),(#224508,#224509),(#224510,#224511),(#224512,#224513),
(#224514,#224515),(#224516,#224517),(#224518,#224519),(#224520,#224521),
(#224522,#224523),(#224524,#224525),(#224526,#224527),(#224528,#224529),
(#224530,#224531),(#224532,#224533),(#224534,#224535),(#224536,#224537),
(#224538,#224539),(#224540,#224541),(#224542,#224543),(#224544,#224545),
(#224546,#224547),(#224548,#224549),(#224550,#224551),(#224552,#224553),
(#224554,#224555),(#224556,#224557),(#224558,#224559),(#224560,#224561),
(#224562,#224563),(#224564,#224565),(#224566,#224567),(#224568,#224569),
(#224570,#224571),(#224572,#224573),(#224574,#224575),(#224576,#224577),
(#224578,#224579),(#224580,#224581),(#224582,#224583),(#224584,#224585),
(#224586,#224587),(#224588,#224589),(#224590,#224591),(#224592,#224593),
(#224594,#224595),(#224596,#224597),(#224598,#224599),(#224600,#224601),
(#224602,#224603),(#224604,#224605),(#224606,#224607),(#224608,#224609),
(#224610,#224611),(#224612,#224613),(#224614,#224615),(#224616,#224617),
(#224618,#224619),(#224620,#224621),(#224622,#224623),(#224624,#224625),
(#224626,#224627),(#224628,#224629),(#224630,#224631),(#224632,#224633),
(#224634,#224635),(#224636,#224637),(#224638,#224639),(#224640,#224641),
(#224642,#224643),(#224644,#224645),(#224646,#224647),(#224648,#224649),
(#224650,#224651),(#224652,#224653),(#224654,#224655),(#224656,#224657),
(#224658,#224659),(#224660,#224661),(#224662,#224663),(#224664,#224665),
(#224666,#224667),(#224668,#224669),(#224670,#224671),(#224672,#224673),
(#224674,#224675),(#224676,#224677)),.UNSPECIFIED.,.F.,.F.,.F.)
B_SPLINE_SURFACE_WITH_KNOTS((6,1,1,1,1,1,1,1,1,1,1,1,1,1,1,1,1,1,1,1,1,
1,1,1,1,1,1,1,1,1,1,1,1,1,1,1,1,1,1,1,1,1,1,1,1,1,1,1,1,1,1,1,1,1,1,1,1,
1,1,1,1,1,1,1,1,1,1,1,1,1,1,1,1,1,1,1,1,1,1,1,1,1,1,1,1,1,1,1,1,1,1,1,1,
1,1,1,1,1,1,1,1,1,1,1,1,1,1,1,1,1,1,1,1,1,1,1,1,1,1,1,1,1,1,1,1,1,1,1,1,
1,1,1,1,1,1,1,1,1,1,1,1,1,1,1,1,1,1,1,1,1,1,1,1,1,1,1,1,1,1,1,1,1,1,1,1,
1,1,1,1,1,1,1,1,1,1,1,1,1,1,1,1,1,1,1,1,1,1,1,1,1,1,1,1,1,1,1,1,1,1,1,6),
(2,2),(-1.,-0.995000000000001,-0.990000000000001,-0.985000000000001,-0.980000000000001,
-0.975000000000001,-0.970000000000001,-0.965000000000001,-0.960000000000001,
-0.955000000000001,-0.950000000000001,-0.945000000000001,-0.940000000000001,
-0.935000000000001,-0.930000000000001,-0.925000000000001,-0.920000000000001,
-0.915000000000001,-0.910000000000001,-0.905000000000001,-0.900000000000001,
-0.895000000000001,-0.890000000000001,-0.885000000000001,-0.880000000000001,
-0.875000000000001,-0.870000000000001,-0.865000000000001,-0.860000000000001,
-0.855000000000001,-0.850000000000001,-0.845000000000001,-0.840000000000001,
-0.835000000000001,-0.830000000000001,-0.825000000000001,-0.820000000000001,
-0.815000000000001,-0.810000000000001,-0.805000000000001,-0.800000000000001,
-0.795000000000001,-0.790000000000001,-0.785000000000001,-0.780000000000001,
-0.775000000000001,-0.770000000000001,-0.765000000000001,-0.760000000000001,
-0.755000000000001,-0.750000000000001,-0.745000000000001,-0.740000000000001,
-0.735000000000001,-0.730000000000001,-0.725000000000001,-0.720000000000001,
-0.715000000000001,-0.710000000000001,-0.705000000000001,-0.700000000000001,
-0.695000000000001,-0.690000000000001,-0.685,-0.68,-0.675,-0.67,-0.665,
-0.66,-0.655,-0.65,-0.645,-0.64,-0.635,-0.63,-0.625,-0.62,-0.615,-0.61,
-0.605,-0.6,-0.595,-0.59,-0.585,-0.58,-0.575,-0.57,-0.565,-0.56,-0.555,
-0.55,-0.545,-0.54,-0.535,-0.53,-0.525,-0.52,-0.515,-0.51,-0.505,-0.5,-0.495,
-0.49,-0.485,-0.48,-0.475,-0.47,-0.465,-0.46,-0.455,-0.45,-0.445,-0.44,
-0.435,-0.43,-0.425,-0.42,-0.415,-0.41,-0.405,-0.4,-0.395,-0.39,-0.385,
-0.38,-0.375,-0.37,-0.365,-0.36,-0.355,-0.35,-0.345,-0.34,-0.335,-0.33,
-0.325,-0.32,-0.315,-0.31,-0.305,-0.3,-0.295,-0.29,-0.285,-0.28,-0.275,
-0.27,-0.265,-0.26,-0.255,-0.25,-0.245,-0.24,-0.235,-0.23,-0.225,-0.22,
-0.215,-0.21,-0.205,-0.2,-0.195,-0.19,-0.185,-0.18,-0.175,-0.17,-0.165,
-0.16,-0.155,-0.15,-0.145,-0.14,-0.135,-0.13,-0.125,-0.12,-0.115,-0.11,
-0.105,-0.1,-0.095,-0.09,-0.085,-0.08,-0.075,-0.07,-0.065,-0.06,-0.055,
-0.05,-0.045,-0.04,-0.035,-0.03,-0.025,-0.02,-0.015,-0.01,-0.005,0.),(0.,
1.2),.UNSPECIFIED.)
GEOMETRIC_REPRESENTATION_ITEM()
RATIONAL_B_SPLINE_SURFACE(((1.,1.),(1.,1.),(1.,1.),(1.,1.),(1.,1.),(1.,
1.),(1.,1.),(1.,1.),(1.,1.),(1.,1.),(1.,1.),(1.,1.),(1.,1.),(1.,1.),(1.,
1.),(1.,1.),(1.,1.),(1.,1.),(1.,1.),(1.,1.),(1.,1.),(1.,1.),(1.,1.),(1.,
1.),(1.,1.),(1.,1.),(1.,1.),(1.,1.),(1.,1.),(1.,1.),(1.,1.),(1.,1.),(1.,
1.),(1.,1.),(1.,1.),(1.,1.),(1.,1.),(1.,1.),(1.,1.),(1.,1.),(1.,1.),(1.,
1.),(1.,1.),(1.,1.),(1.,1.),(1.,1.),(1.,1.),(1.,1.),(1.,1.),(1.,1.),(1.,
1.),(1.,1.),(1.,1.),(1.,1.),(1.,1.),(1.,1.),(1.,1.),(1.,1.),(1.,1.),(1.,
1.),(1.,1.),(1.,1.),(1.,1.),(1.,1.),(1.,1.),(1.,1.),(1.,1.),(1.,1.),(1.,
1.),(1.,1.),(1.,1.),(1.,1.),(1.,1.),(1.,1.),(1.,1.),(1.,1.),(1.,1.),(1.,
1.),(1.,1.),(1.,1.),(1.,1.),(1.,1.),(1.,1.),(1.,1.),(1.,1.),(1.,1.),(1.,
1.),(1.,1.),(1.,1.),(1.,1.),(1.,1.),(1.,1.),(1.,1.),(1.,1.),(1.,1.),(1.,
1.),(1.,1.),(1.,1.),(1.,1.),(1.,1.),(1.,1.),(1.,1.),(1.,1.),(1.,1.),(1.,
1.),(1.,1.),(1.,1.),(1.,1.),(1.,1.),(1.,1.),(1.,1.),(1.,1.),(1.,1.),(1.,
1.),(1.,1.),(1.,1.),(1.,1.),(1.,1.),(1.,1.),(1.,1.),(1.,1.),(1.,1.),(1.,
1.),(1.,1.),(1.,1.),(1.,1.),(1.,1.),(1.,1.),(1.,1.),(1.,1.),(1.,1.),(1.,
1.),(1.,1.),(1.,1.),(1.,1.),(1.,1.),(1.,1.),(1.,1.),(1.,1.),(1.,1.),(1.,
1.),(1.,1.),(1.,1.),(1.,1.),(1.,1.),(1.,1.),(1.,1.),(1.,1.),(1.,1.),(1.,
1.),(1.,1.),(1.,1.),(1.,1.),(1.,1.),(1.,1.),(1.,1.),(1.,1.),(1.,1.),(1.,
1.),(1.,1.),(1.,1.),(1.,1.),(1.,1.),(1.,1.),(1.,1.),(1.,1.),(1.,1.),(1.,
1.),(1.,1.),(1.,1.),(1.,1.),(1.,1.),(1.,1.),(1.,1.),(1.,1.),(1.,1.),(1.,
1.),(1.,1.),(1.,1.),(1.,1.),(1.,1.),(1.,1.),(1.,1.),(1.,1.),(1.,1.),(1.,
1.),(1.,1.),(1.,1.),(1.,1.),(1.,1.),(1.,1.),(1.,1.),(1.,1.),(1.,1.),(1.,
1.),(1.,1.),(1.,1.),(1.,1.),(1.,1.),(1.,1.),(1.,1.),(1.,1.),(1.,1.),(1.,
1.),(1.,1.)))
REPRESENTATION_ITEM('')
SURFACE()
);
#1086=(
BOUNDED_SURFACE()
B_SPLINE_SURFACE(5,1,((#225091,#225092),(#225093,#225094),(#225095,#225096),
(#225097,#225098),(#225099,#225100),(#225101,#225102),(#225103,#225104),
(#225105,#225106),(#225107,#225108),(#225109,#225110),(#225111,#225112),
(#225113,#225114),(#225115,#225116),(#225117,#225118),(#225119,#225120),
(#225121,#225122),(#225123,#225124),(#225125,#225126),(#225127,#225128),
(#225129,#225130),(#225131,#225132),(#225133,#225134),(#225135,#225136),
(#225137,#225138),(#225139,#225140),(#225141,#225142),(#225143,#225144),
(#225145,#225146),(#225147,#225148),(#225149,#225150),(#225151,#225152),
(#225153,#225154),(#225155,#225156),(#225157,#225158),(#225159,#225160),
(#225161,#225162),(#225163,#225164),(#225165,#225166),(#225167,#225168),
(#225169,#225170),(#225171,#225172),(#225173,#225174),(#225175,#225176),
(#225177,#225178),(#225179,#225180),(#225181,#225182),(#225183,#225184),
(#225185,#225186),(#225187,#225188),(#225189,#225190),(#225191,#225192),
(#225193,#225194),(#225195,#225196),(#225197,#225198),(#225199,#225200),
(#225201,#225202),(#225203,#225204),(#225205,#225206),(#225207,#225208),
(#225209,#225210),(#225211,#225212),(#225213,#225214),(#225215,#225216),
(#225217,#225218),(#225219,#225220),(#225221,#225222),(#225223,#225224),
(#225225,#225226),(#225227,#225228),(#225229,#225230),(#225231,#225232),
(#225233,#225234),(#225235,#225236),(#225237,#225238),(#225239,#225240),
(#225241,#225242),(#225243,#225244),(#225245,#225246),(#225247,#225248),
(#225249,#225250),(#225251,#225252),(#225253,#225254),(#225255,#225256),
(#225257,#225258),(#225259,#225260),(#225261,#225262),(#225263,#225264),
(#225265,#225266),(#225267,#225268),(#225269,#225270),(#225271,#225272),
(#225273,#225274),(#225275,#225276),(#225277,#225278),(#225279,#225280),
(#225281,#225282),(#225283,#225284),(#225285,#225286),(#225287,#225288),
(#225289,#225290),(#225291,#225292),(#225293,#225294),(#225295,#225296),
(#225297,#225298),(#225299,#225300),(#225301,#225302),(#225303,#225304),
(#225305,#225306),(#225307,#225308),(#225309,#225310),(#225311,#225312),
(#225313,#225314),(#225315,#225316),(#225317,#225318),(#225319,#225320),
(#225321,#225322),(#225323,#225324),(#225325,#225326),(#225327,#225328),
(#225329,#225330),(#225331,#225332),(#225333,#225334),(#225335,#225336),
(#225337,#225338),(#225339,#225340),(#225341,#225342),(#225343,#225344),
(#225345,#225346),(#225347,#225348),(#225349,#225350),(#225351,#225352),
(#225353,#225354),(#225355,#225356),(#225357,#225358),(#225359,#225360),
(#225361,#225362),(#225363,#225364),(#225365,#225366),(#225367,#225368),
(#225369,#225370),(#225371,#225372),(#225373,#225374),(#225375,#225376),
(#225377,#225378),(#225379,#225380),(#225381,#225382),(#225383,#225384),
(#225385,#225386),(#225387,#225388),(#225389,#225390),(#225391,#225392),
(#225393,#225394),(#225395,#225396),(#225397,#225398),(#225399,#225400),
(#225401,#225402),(#225403,#225404),(#225405,#225406),(#225407,#225408),
(#225409,#225410),(#225411,#225412),(#225413,#225414),(#225415,#225416),
(#225417,#225418),(#225419,#225420),(#225421,#225422),(#225423,#225424),
(#225425,#225426),(#225427,#225428),(#225429,#225430),(#225431,#225432),
(#225433,#225434),(#225435,#225436),(#225437,#225438),(#225439,#225440),
(#225441,#225442),(#225443,#225444),(#225445,#225446),(#225447,#225448),
(#225449,#225450),(#225451,#225452),(#225453,#225454),(#225455,#225456),
(#225457,#225458),(#225459,#225460),(#225461,#225462),(#225463,#225464),
(#225465,#225466),(#225467,#225468),(#225469,#225470),(#225471,#225472),
(#225473,#225474),(#225475,#225476),(#225477,#225478),(#225479,#225480),
(#225481,#225482),(#225483,#225484),(#225485,#225486),(#225487,#225488),
(#225489,#225490),(#225491,#225492),(#225493,#225494),(#225495,#225496),
(#225497,#225498),(#225499,#225500)),.UNSPECIFIED.,.F.,.F.,.F.)
B_SPLINE_SURFACE_WITH_KNOTS((6,1,1,1,1,1,1,1,1,1,1,1,1,1,1,1,1,1,1,1,1,
1,1,1,1,1,1,1,1,1,1,1,1,1,1,1,1,1,1,1,1,1,1,1,1,1,1,1,1,1,1,1,1,1,1,1,1,
1,1,1,1,1,1,1,1,1,1,1,1,1,1,1,1,1,1,1,1,1,1,1,1,1,1,1,1,1,1,1,1,1,1,1,1,
1,1,1,1,1,1,1,1,1,1,1,1,1,1,1,1,1,1,1,1,1,1,1,1,1,1,1,1,1,1,1,1,1,1,1,1,
1,1,1,1,1,1,1,1,1,1,1,1,1,1,1,1,1,1,1,1,1,1,1,1,1,1,1,1,1,1,1,1,1,1,1,1,
1,1,1,1,1,1,1,1,1,1,1,1,1,1,1,1,1,1,1,1,1,1,1,1,1,1,1,1,1,1,1,1,1,1,1,6),
(2,2),(0.,0.005,0.01,0.015,0.02,0.025,0.03,0.035,0.04,0.045,0.05,0.055,
0.06,0.065,0.07,0.075,0.08,0.085,0.09,0.095,0.1,0.105,0.11,0.115,0.12,0.125,
0.13,0.135,0.14,0.145,0.15,0.155,0.16,0.165,0.17,0.175,0.18,0.185,0.19,
0.195,0.2,0.205,0.21,0.215,0.22,0.225,0.23,0.235,0.24,0.245,0.25,0.255,
0.26,0.265,0.27,0.275,0.28,0.285,0.29,0.295,0.3,0.305,0.31,0.315,0.32,0.325,
0.33,0.335,0.34,0.345,0.35,0.355,0.36,0.365,0.37,0.375,0.38,0.385,0.39,
0.395,0.4,0.405,0.41,0.415,0.42,0.425,0.43,0.435,0.44,0.445,0.45,0.455,
0.46,0.465,0.47,0.475,0.48,0.485,0.49,0.495,0.5,0.505,0.51,0.515,0.52,0.525,
0.53,0.535,0.54,0.545,0.55,0.555,0.56,0.565,0.57,0.575,0.58,0.585,0.59,
0.595,0.6,0.605,0.61,0.615,0.62,0.625,0.63,0.635,0.64,0.645,0.65,0.655,
0.66,0.665,0.67,0.675,0.68,0.685,0.690000000000001,0.695000000000001,0.700000000000001,
0.705000000000001,0.710000000000001,0.715000000000001,0.720000000000001,
0.725000000000001,0.730000000000001,0.735000000000001,0.740000000000001,
0.745000000000001,0.750000000000001,0.755000000000001,0.760000000000001,
0.765000000000001,0.770000000000001,0.775000000000001,0.780000000000001,
0.785000000000001,0.790000000000001,0.795000000000001,0.800000000000001,
0.805000000000001,0.810000000000001,0.815000000000001,0.820000000000001,
0.825000000000001,0.830000000000001,0.835000000000001,0.840000000000001,
0.845000000000001,0.850000000000001,0.855000000000001,0.860000000000001,
0.865000000000001,0.870000000000001,0.875000000000001,0.880000000000001,
0.885000000000001,0.890000000000001,0.895000000000001,0.900000000000001,
0.905000000000001,0.910000000000001,0.915000000000001,0.920000000000001,
0.925000000000001,0.930000000000001,0.935000000000001,0.940000000000001,
0.945000000000001,0.950000000000001,0.955000000000001,0.960000000000001,
0.965000000000001,0.970000000000001,0.975000000000001,0.980000000000001,
0.985000000000001,0.990000000000001,0.995000000000001,1.),(0.,1.2),
 .UNSPECIFIED.)
GEOMETRIC_REPRESENTATION_ITEM()
RATIONAL_B_SPLINE_SURFACE(((1.,1.),(1.,1.),(1.,1.),(1.,1.),(1.,1.),(1.,
1.),(1.,1.),(1.,1.),(1.,1.),(1.,1.),(1.,1.),(1.,1.),(1.,1.),(1.,1.),(1.,
1.),(1.,1.),(1.,1.),(1.,1.),(1.,1.),(1.,1.),(1.,1.),(1.,1.),(1.,1.),(1.,
1.),(1.,1.),(1.,1.),(1.,1.),(1.,1.),(1.,1.),(1.,1.),(1.,1.),(1.,1.),(1.,
1.),(1.,1.),(1.,1.),(1.,1.),(1.,1.),(1.,1.),(1.,1.),(1.,1.),(1.,1.),(1.,
1.),(1.,1.),(1.,1.),(1.,1.),(1.,1.),(1.,1.),(1.,1.),(1.,1.),(1.,1.),(1.,
1.),(1.,1.),(1.,1.),(1.,1.),(1.,1.),(1.,1.),(1.,1.),(1.,1.),(1.,1.),(1.,
1.),(1.,1.),(1.,1.),(1.,1.),(1.,1.),(1.,1.),(1.,1.),(1.,1.),(1.,1.),(1.,
1.),(1.,1.),(1.,1.),(1.,1.),(1.,1.),(1.,1.),(1.,1.),(1.,1.),(1.,1.),(1.,
1.),(1.,1.),(1.,1.),(1.,1.),(1.,1.),(1.,1.),(1.,1.),(1.,1.),(1.,1.),(1.,
1.),(1.,1.),(1.,1.),(1.,1.),(1.,1.),(1.,1.),(1.,1.),(1.,1.),(1.,1.),(1.,
1.),(1.,1.),(1.,1.),(1.,1.),(1.,1.),(1.,1.),(1.,1.),(1.,1.),(1.,1.),(1.,
1.),(1.,1.),(1.,1.),(1.,1.),(1.,1.),(1.,1.),(1.,1.),(1.,1.),(1.,1.),(1.,
1.),(1.,1.),(1.,1.),(1.,1.),(1.,1.),(1.,1.),(1.,1.),(1.,1.),(1.,1.),(1.,
1.),(1.,1.),(1.,1.),(1.,1.),(1.,1.),(1.,1.),(1.,1.),(1.,1.),(1.,1.),(1.,
1.),(1.,1.),(1.,1.),(1.,1.),(1.,1.),(1.,1.),(1.,1.),(1.,1.),(1.,1.),(1.,
1.),(1.,1.),(1.,1.),(1.,1.),(1.,1.),(1.,1.),(1.,1.),(1.,1.),(1.,1.),(1.,
1.),(1.,1.),(1.,1.),(1.,1.),(1.,1.),(1.,1.),(1.,1.),(1.,1.),(1.,1.),(1.,
1.),(1.,1.),(1.,1.),(1.,1.),(1.,1.),(1.,1.),(1.,1.),(1.,1.),(1.,1.),(1.,
1.),(1.,1.),(1.,1.),(1.,1.),(1.,1.),(1.,1.),(1.,1.),(1.,1.),(1.,1.),(1.,
1.),(1.,1.),(1.,1.),(1.,1.),(1.,1.),(1.,1.),(1.,1.),(1.,1.),(1.,1.),(1.,
1.),(1.,1.),(1.,1.),(1.,1.),(1.,1.),(1.,1.),(1.,1.),(1.,1.),(1.,1.),(1.,
1.),(1.,1.),(1.,1.),(1.,1.),(1.,1.),(1.,1.),(1.,1.),(1.,1.),(1.,1.),(1.,
1.),(1.,1.)))
REPRESENTATION_ITEM('')
SURFACE()
);
#1087=(
BOUNDED_SURFACE()
B_SPLINE_SURFACE(5,1,((#225920,#225921),(#225922,#225923),(#225924,#225925),
(#225926,#225927),(#225928,#225929),(#225930,#225931),(#225932,#225933),
(#225934,#225935),(#225936,#225937),(#225938,#225939),(#225940,#225941),
(#225942,#225943),(#225944,#225945),(#225946,#225947),(#225948,#225949),
(#225950,#225951),(#225952,#225953),(#225954,#225955),(#225956,#225957),
(#225958,#225959),(#225960,#225961),(#225962,#225963),(#225964,#225965),
(#225966,#225967),(#225968,#225969),(#225970,#225971),(#225972,#225973),
(#225974,#225975),(#225976,#225977),(#225978,#225979),(#225980,#225981),
(#225982,#225983),(#225984,#225985),(#225986,#225987),(#225988,#225989),
(#225990,#225991),(#225992,#225993),(#225994,#225995),(#225996,#225997),
(#225998,#225999),(#226000,#226001),(#226002,#226003),(#226004,#226005),
(#226006,#226007),(#226008,#226009),(#226010,#226011),(#226012,#226013),
(#226014,#226015),(#226016,#226017),(#226018,#226019),(#226020,#226021),
(#226022,#226023),(#226024,#226025),(#226026,#226027),(#226028,#226029),
(#226030,#226031),(#226032,#226033),(#226034,#226035),(#226036,#226037),
(#226038,#226039),(#226040,#226041),(#226042,#226043),(#226044,#226045),
(#226046,#226047),(#226048,#226049),(#226050,#226051),(#226052,#226053),
(#226054,#226055),(#226056,#226057),(#226058,#226059),(#226060,#226061),
(#226062,#226063),(#226064,#226065),(#226066,#226067),(#226068,#226069),
(#226070,#226071),(#226072,#226073),(#226074,#226075),(#226076,#226077),
(#226078,#226079),(#226080,#226081),(#226082,#226083),(#226084,#226085),
(#226086,#226087),(#226088,#226089),(#226090,#226091),(#226092,#226093),
(#226094,#226095),(#226096,#226097),(#226098,#226099),(#226100,#226101),
(#226102,#226103),(#226104,#226105),(#226106,#226107),(#226108,#226109),
(#226110,#226111),(#226112,#226113),(#226114,#226115),(#226116,#226117),
(#226118,#226119),(#226120,#226121),(#226122,#226123),(#226124,#226125),
(#226126,#226127),(#226128,#226129),(#226130,#226131),(#226132,#226133),
(#226134,#226135),(#226136,#226137),(#226138,#226139),(#226140,#226141),
(#226142,#226143),(#226144,#226145),(#226146,#226147),(#226148,#226149),
(#226150,#226151),(#226152,#226153),(#226154,#226155),(#226156,#226157),
(#226158,#226159),(#226160,#226161),(#226162,#226163),(#226164,#226165),
(#226166,#226167),(#226168,#226169),(#226170,#226171),(#226172,#226173),
(#226174,#226175),(#226176,#226177),(#226178,#226179),(#226180,#226181),
(#226182,#226183),(#226184,#226185),(#226186,#226187),(#226188,#226189),
(#226190,#226191),(#226192,#226193),(#226194,#226195),(#226196,#226197),
(#226198,#226199),(#226200,#226201),(#226202,#226203),(#226204,#226205),
(#226206,#226207),(#226208,#226209),(#226210,#226211),(#226212,#226213),
(#226214,#226215),(#226216,#226217),(#226218,#226219),(#226220,#226221),
(#226222,#226223),(#226224,#226225),(#226226,#226227),(#226228,#226229),
(#226230,#226231),(#226232,#226233),(#226234,#226235),(#226236,#226237),
(#226238,#226239),(#226240,#226241),(#226242,#226243),(#226244,#226245),
(#226246,#226247),(#226248,#226249),(#226250,#226251),(#226252,#226253),
(#226254,#226255),(#226256,#226257),(#226258,#226259),(#226260,#226261),
(#226262,#226263),(#226264,#226265),(#226266,#226267),(#226268,#226269),
(#226270,#226271),(#226272,#226273),(#226274,#226275),(#226276,#226277),
(#226278,#226279),(#226280,#226281),(#226282,#226283),(#226284,#226285),
(#226286,#226287),(#226288,#226289),(#226290,#226291),(#226292,#226293),
(#226294,#226295),(#226296,#226297),(#226298,#226299),(#226300,#226301),
(#226302,#226303),(#226304,#226305),(#226306,#226307),(#226308,#226309),
(#226310,#226311),(#226312,#226313),(#226314,#226315),(#226316,#226317),
(#226318,#226319),(#226320,#226321),(#226322,#226323),(#226324,#226325),
(#226326,#226327),(#226328,#226329)),.UNSPECIFIED.,.F.,.F.,.F.)
B_SPLINE_SURFACE_WITH_KNOTS((6,1,1,1,1,1,1,1,1,1,1,1,1,1,1,1,1,1,1,1,1,
1,1,1,1,1,1,1,1,1,1,1,1,1,1,1,1,1,1,1,1,1,1,1,1,1,1,1,1,1,1,1,1,1,1,1,1,
1,1,1,1,1,1,1,1,1,1,1,1,1,1,1,1,1,1,1,1,1,1,1,1,1,1,1,1,1,1,1,1,1,1,1,1,
1,1,1,1,1,1,1,1,1,1,1,1,1,1,1,1,1,1,1,1,1,1,1,1,1,1,1,1,1,1,1,1,1,1,1,1,
1,1,1,1,1,1,1,1,1,1,1,1,1,1,1,1,1,1,1,1,1,1,1,1,1,1,1,1,1,1,1,1,1,1,1,1,
1,1,1,1,1,1,1,1,1,1,1,1,1,1,1,1,1,1,1,1,1,1,1,1,1,1,1,1,1,1,1,1,1,1,1,6),
(2,2),(-1.,-0.995000000000001,-0.990000000000001,-0.985000000000001,-0.980000000000001,
-0.975000000000001,-0.970000000000001,-0.965000000000001,-0.960000000000001,
-0.955000000000001,-0.950000000000001,-0.945000000000001,-0.940000000000001,
-0.935000000000001,-0.930000000000001,-0.925000000000001,-0.920000000000001,
-0.915000000000001,-0.910000000000001,-0.905000000000001,-0.900000000000001,
-0.895000000000001,-0.890000000000001,-0.885000000000001,-0.880000000000001,
-0.875000000000001,-0.870000000000001,-0.865000000000001,-0.860000000000001,
-0.855000000000001,-0.850000000000001,-0.845000000000001,-0.840000000000001,
-0.835000000000001,-0.830000000000001,-0.825000000000001,-0.820000000000001,
-0.815000000000001,-0.810000000000001,-0.805000000000001,-0.800000000000001,
-0.795000000000001,-0.790000000000001,-0.785000000000001,-0.780000000000001,
-0.775000000000001,-0.770000000000001,-0.765000000000001,-0.760000000000001,
-0.755000000000001,-0.750000000000001,-0.745000000000001,-0.740000000000001,
-0.735000000000001,-0.730000000000001,-0.725000000000001,-0.720000000000001,
-0.715000000000001,-0.710000000000001,-0.705000000000001,-0.700000000000001,
-0.695000000000001,-0.690000000000001,-0.685,-0.68,-0.675,-0.67,-0.665,
-0.66,-0.655,-0.65,-0.645,-0.64,-0.635,-0.63,-0.625,-0.62,-0.615,-0.61,
-0.605,-0.6,-0.595,-0.59,-0.585,-0.58,-0.575,-0.57,-0.565,-0.56,-0.555,
-0.55,-0.545,-0.54,-0.535,-0.53,-0.525,-0.52,-0.515,-0.51,-0.505,-0.5,-0.495,
-0.49,-0.485,-0.48,-0.475,-0.47,-0.465,-0.46,-0.455,-0.45,-0.445,-0.44,
-0.435,-0.43,-0.425,-0.42,-0.415,-0.41,-0.405,-0.4,-0.395,-0.39,-0.385,
-0.38,-0.375,-0.37,-0.365,-0.36,-0.355,-0.35,-0.345,-0.34,-0.335,-0.33,
-0.325,-0.32,-0.315,-0.31,-0.305,-0.3,-0.295,-0.29,-0.285,-0.28,-0.275,
-0.27,-0.265,-0.26,-0.255,-0.25,-0.245,-0.24,-0.235,-0.23,-0.225,-0.22,
-0.215,-0.21,-0.205,-0.2,-0.195,-0.19,-0.185,-0.18,-0.175,-0.17,-0.165,
-0.16,-0.155,-0.15,-0.145,-0.14,-0.135,-0.13,-0.125,-0.12,-0.115,-0.11,
-0.105,-0.1,-0.095,-0.09,-0.085,-0.08,-0.075,-0.07,-0.065,-0.06,-0.055,
-0.05,-0.045,-0.04,-0.035,-0.03,-0.025,-0.02,-0.015,-0.01,-0.005,0.),(0.,
1.2),.UNSPECIFIED.)
GEOMETRIC_REPRESENTATION_ITEM()
RATIONAL_B_SPLINE_SURFACE(((1.,1.),(1.,1.),(1.,1.),(1.,1.),(1.,1.),(1.,
1.),(1.,1.),(1.,1.),(1.,1.),(1.,1.),(1.,1.),(1.,1.),(1.,1.),(1.,1.),(1.,
1.),(1.,1.),(1.,1.),(1.,1.),(1.,1.),(1.,1.),(1.,1.),(1.,1.),(1.,1.),(1.,
1.),(1.,1.),(1.,1.),(1.,1.),(1.,1.),(1.,1.),(1.,1.),(1.,1.),(1.,1.),(1.,
1.),(1.,1.),(1.,1.),(1.,1.),(1.,1.),(1.,1.),(1.,1.),(1.,1.),(1.,1.),(1.,
1.),(1.,1.),(1.,1.),(1.,1.),(1.,1.),(1.,1.),(1.,1.),(1.,1.),(1.,1.),(1.,
1.),(1.,1.),(1.,1.),(1.,1.),(1.,1.),(1.,1.),(1.,1.),(1.,1.),(1.,1.),(1.,
1.),(1.,1.),(1.,1.),(1.,1.),(1.,1.),(1.,1.),(1.,1.),(1.,1.),(1.,1.),(1.,
1.),(1.,1.),(1.,1.),(1.,1.),(1.,1.),(1.,1.),(1.,1.),(1.,1.),(1.,1.),(1.,
1.),(1.,1.),(1.,1.),(1.,1.),(1.,1.),(1.,1.),(1.,1.),(1.,1.),(1.,1.),(1.,
1.),(1.,1.),(1.,1.),(1.,1.),(1.,1.),(1.,1.),(1.,1.),(1.,1.),(1.,1.),(1.,
1.),(1.,1.),(1.,1.),(1.,1.),(1.,1.),(1.,1.),(1.,1.),(1.,1.),(1.,1.),(1.,
1.),(1.,1.),(1.,1.),(1.,1.),(1.,1.),(1.,1.),(1.,1.),(1.,1.),(1.,1.),(1.,
1.),(1.,1.),(1.,1.),(1.,1.),(1.,1.),(1.,1.),(1.,1.),(1.,1.),(1.,1.),(1.,
1.),(1.,1.),(1.,1.),(1.,1.),(1.,1.),(1.,1.),(1.,1.),(1.,1.),(1.,1.),(1.,
1.),(1.,1.),(1.,1.),(1.,1.),(1.,1.),(1.,1.),(1.,1.),(1.,1.),(1.,1.),(1.,
1.),(1.,1.),(1.,1.),(1.,1.),(1.,1.),(1.,1.),(1.,1.),(1.,1.),(1.,1.),(1.,
1.),(1.,1.),(1.,1.),(1.,1.),(1.,1.),(1.,1.),(1.,1.),(1.,1.),(1.,1.),(1.,
1.),(1.,1.),(1.,1.),(1.,1.),(1.,1.),(1.,1.),(1.,1.),(1.,1.),(1.,1.),(1.,
1.),(1.,1.),(1.,1.),(1.,1.),(1.,1.),(1.,1.),(1.,1.),(1.,1.),(1.,1.),(1.,
1.),(1.,1.),(1.,1.),(1.,1.),(1.,1.),(1.,1.),(1.,1.),(1.,1.),(1.,1.),(1.,
1.),(1.,1.),(1.,1.),(1.,1.),(1.,1.),(1.,1.),(1.,1.),(1.,1.),(1.,1.),(1.,
1.),(1.,1.),(1.,1.),(1.,1.),(1.,1.),(1.,1.),(1.,1.),(1.,1.),(1.,1.),(1.,
1.),(1.,1.)))
REPRESENTATION_ITEM('')
SURFACE()
);
#1088=(
BOUNDED_SURFACE()
B_SPLINE_SURFACE(5,1,((#226743,#226744),(#226745,#226746),(#226747,#226748),
(#226749,#226750),(#226751,#226752),(#226753,#226754),(#226755,#226756),
(#226757,#226758),(#226759,#226760),(#226761,#226762),(#226763,#226764),
(#226765,#226766),(#226767,#226768),(#226769,#226770),(#226771,#226772),
(#226773,#226774),(#226775,#226776),(#226777,#226778),(#226779,#226780),
(#226781,#226782),(#226783,#226784),(#226785,#226786),(#226787,#226788),
(#226789,#226790),(#226791,#226792),(#226793,#226794),(#226795,#226796),
(#226797,#226798),(#226799,#226800),(#226801,#226802),(#226803,#226804),
(#226805,#226806),(#226807,#226808),(#226809,#226810),(#226811,#226812),
(#226813,#226814),(#226815,#226816),(#226817,#226818),(#226819,#226820),
(#226821,#226822),(#226823,#226824),(#226825,#226826),(#226827,#226828),
(#226829,#226830),(#226831,#226832),(#226833,#226834),(#226835,#226836),
(#226837,#226838),(#226839,#226840),(#226841,#226842),(#226843,#226844),
(#226845,#226846),(#226847,#226848),(#226849,#226850),(#226851,#226852),
(#226853,#226854),(#226855,#226856),(#226857,#226858),(#226859,#226860),
(#226861,#226862),(#226863,#226864),(#226865,#226866),(#226867,#226868),
(#226869,#226870),(#226871,#226872),(#226873,#226874),(#226875,#226876),
(#226877,#226878),(#226879,#226880),(#226881,#226882),(#226883,#226884),
(#226885,#226886),(#226887,#226888),(#226889,#226890),(#226891,#226892),
(#226893,#226894),(#226895,#226896),(#226897,#226898),(#226899,#226900),
(#226901,#226902),(#226903,#226904),(#226905,#226906),(#226907,#226908),
(#226909,#226910),(#226911,#226912),(#226913,#226914),(#226915,#226916),
(#226917,#226918),(#226919,#226920),(#226921,#226922),(#226923,#226924),
(#226925,#226926),(#226927,#226928),(#226929,#226930),(#226931,#226932),
(#226933,#226934),(#226935,#226936),(#226937,#226938),(#226939,#226940),
(#226941,#226942),(#226943,#226944),(#226945,#226946),(#226947,#226948),
(#226949,#226950),(#226951,#226952),(#226953,#226954),(#226955,#226956),
(#226957,#226958),(#226959,#226960),(#226961,#226962),(#226963,#226964),
(#226965,#226966),(#226967,#226968),(#226969,#226970),(#226971,#226972),
(#226973,#226974),(#226975,#226976),(#226977,#226978),(#226979,#226980),
(#226981,#226982),(#226983,#226984),(#226985,#226986),(#226987,#226988),
(#226989,#226990),(#226991,#226992),(#226993,#226994),(#226995,#226996),
(#226997,#226998),(#226999,#227000),(#227001,#227002),(#227003,#227004),
(#227005,#227006),(#227007,#227008),(#227009,#227010),(#227011,#227012),
(#227013,#227014),(#227015,#227016),(#227017,#227018),(#227019,#227020),
(#227021,#227022),(#227023,#227024),(#227025,#227026),(#227027,#227028),
(#227029,#227030),(#227031,#227032),(#227033,#227034),(#227035,#227036),
(#227037,#227038),(#227039,#227040),(#227041,#227042),(#227043,#227044),
(#227045,#227046),(#227047,#227048),(#227049,#227050),(#227051,#227052),
(#227053,#227054),(#227055,#227056),(#227057,#227058),(#227059,#227060),
(#227061,#227062),(#227063,#227064),(#227065,#227066),(#227067,#227068),
(#227069,#227070),(#227071,#227072),(#227073,#227074),(#227075,#227076),
(#227077,#227078),(#227079,#227080),(#227081,#227082),(#227083,#227084),
(#227085,#227086),(#227087,#227088),(#227089,#227090),(#227091,#227092),
(#227093,#227094),(#227095,#227096),(#227097,#227098),(#227099,#227100),
(#227101,#227102),(#227103,#227104),(#227105,#227106),(#227107,#227108),
(#227109,#227110),(#227111,#227112),(#227113,#227114),(#227115,#227116),
(#227117,#227118),(#227119,#227120),(#227121,#227122),(#227123,#227124),
(#227125,#227126),(#227127,#227128),(#227129,#227130),(#227131,#227132),
(#227133,#227134),(#227135,#227136),(#227137,#227138),(#227139,#227140),
(#227141,#227142),(#227143,#227144),(#227145,#227146),(#227147,#227148),
(#227149,#227150),(#227151,#227152)),.UNSPECIFIED.,.F.,.F.,.F.)
B_SPLINE_SURFACE_WITH_KNOTS((6,1,1,1,1,1,1,1,1,1,1,1,1,1,1,1,1,1,1,1,1,
1,1,1,1,1,1,1,1,1,1,1,1,1,1,1,1,1,1,1,1,1,1,1,1,1,1,1,1,1,1,1,1,1,1,1,1,
1,1,1,1,1,1,1,1,1,1,1,1,1,1,1,1,1,1,1,1,1,1,1,1,1,1,1,1,1,1,1,1,1,1,1,1,
1,1,1,1,1,1,1,1,1,1,1,1,1,1,1,1,1,1,1,1,1,1,1,1,1,1,1,1,1,1,1,1,1,1,1,1,
1,1,1,1,1,1,1,1,1,1,1,1,1,1,1,1,1,1,1,1,1,1,1,1,1,1,1,1,1,1,1,1,1,1,1,1,
1,1,1,1,1,1,1,1,1,1,1,1,1,1,1,1,1,1,1,1,1,1,1,1,1,1,1,1,1,1,1,1,1,1,1,6),
(2,2),(0.,0.005,0.01,0.015,0.02,0.025,0.03,0.035,0.04,0.045,0.05,0.055,
0.06,0.065,0.07,0.075,0.08,0.085,0.09,0.095,0.1,0.105,0.11,0.115,0.12,0.125,
0.13,0.135,0.14,0.145,0.15,0.155,0.16,0.165,0.17,0.175,0.18,0.185,0.19,
0.195,0.2,0.205,0.21,0.215,0.22,0.225,0.23,0.235,0.24,0.245,0.25,0.255,
0.26,0.265,0.27,0.275,0.28,0.285,0.29,0.295,0.3,0.305,0.31,0.315,0.32,0.325,
0.33,0.335,0.34,0.345,0.35,0.355,0.36,0.365,0.37,0.375,0.38,0.385,0.39,
0.395,0.4,0.405,0.41,0.415,0.42,0.425,0.43,0.435,0.44,0.445,0.45,0.455,
0.46,0.465,0.47,0.475,0.48,0.485,0.49,0.495,0.5,0.505,0.51,0.515,0.52,0.525,
0.53,0.535,0.54,0.545,0.55,0.555,0.56,0.565,0.57,0.575,0.58,0.585,0.59,
0.595,0.6,0.605,0.61,0.615,0.62,0.625,0.63,0.635,0.64,0.645,0.65,0.655,
0.66,0.665,0.67,0.675,0.68,0.685,0.690000000000001,0.695000000000001,0.700000000000001,
0.705000000000001,0.710000000000001,0.715000000000001,0.720000000000001,
0.725000000000001,0.730000000000001,0.735000000000001,0.740000000000001,
0.745000000000001,0.750000000000001,0.755000000000001,0.760000000000001,
0.765000000000001,0.770000000000001,0.775000000000001,0.780000000000001,
0.785000000000001,0.790000000000001,0.795000000000001,0.800000000000001,
0.805000000000001,0.810000000000001,0.815000000000001,0.820000000000001,
0.825000000000001,0.830000000000001,0.835000000000001,0.840000000000001,
0.845000000000001,0.850000000000001,0.855000000000001,0.860000000000001,
0.865000000000001,0.870000000000001,0.875000000000001,0.880000000000001,
0.885000000000001,0.890000000000001,0.895000000000001,0.900000000000001,
0.905000000000001,0.910000000000001,0.915000000000001,0.920000000000001,
0.925000000000001,0.930000000000001,0.935000000000001,0.940000000000001,
0.945000000000001,0.950000000000001,0.955000000000001,0.960000000000001,
0.965000000000001,0.970000000000001,0.975000000000001,0.980000000000001,
0.985000000000001,0.990000000000001,0.995000000000001,1.),(0.,1.2),
 .UNSPECIFIED.)
GEOMETRIC_REPRESENTATION_ITEM()
RATIONAL_B_SPLINE_SURFACE(((1.,1.),(1.,1.),(1.,1.),(1.,1.),(1.,1.),(1.,
1.),(1.,1.),(1.,1.),(1.,1.),(1.,1.),(1.,1.),(1.,1.),(1.,1.),(1.,1.),(1.,
1.),(1.,1.),(1.,1.),(1.,1.),(1.,1.),(1.,1.),(1.,1.),(1.,1.),(1.,1.),(1.,
1.),(1.,1.),(1.,1.),(1.,1.),(1.,1.),(1.,1.),(1.,1.),(1.,1.),(1.,1.),(1.,
1.),(1.,1.),(1.,1.),(1.,1.),(1.,1.),(1.,1.),(1.,1.),(1.,1.),(1.,1.),(1.,
1.),(1.,1.),(1.,1.),(1.,1.),(1.,1.),(1.,1.),(1.,1.),(1.,1.),(1.,1.),(1.,
1.),(1.,1.),(1.,1.),(1.,1.),(1.,1.),(1.,1.),(1.,1.),(1.,1.),(1.,1.),(1.,
1.),(1.,1.),(1.,1.),(1.,1.),(1.,1.),(1.,1.),(1.,1.),(1.,1.),(1.,1.),(1.,
1.),(1.,1.),(1.,1.),(1.,1.),(1.,1.),(1.,1.),(1.,1.),(1.,1.),(1.,1.),(1.,
1.),(1.,1.),(1.,1.),(1.,1.),(1.,1.),(1.,1.),(1.,1.),(1.,1.),(1.,1.),(1.,
1.),(1.,1.),(1.,1.),(1.,1.),(1.,1.),(1.,1.),(1.,1.),(1.,1.),(1.,1.),(1.,
1.),(1.,1.),(1.,1.),(1.,1.),(1.,1.),(1.,1.),(1.,1.),(1.,1.),(1.,1.),(1.,
1.),(1.,1.),(1.,1.),(1.,1.),(1.,1.),(1.,1.),(1.,1.),(1.,1.),(1.,1.),(1.,
1.),(1.,1.),(1.,1.),(1.,1.),(1.,1.),(1.,1.),(1.,1.),(1.,1.),(1.,1.),(1.,
1.),(1.,1.),(1.,1.),(1.,1.),(1.,1.),(1.,1.),(1.,1.),(1.,1.),(1.,1.),(1.,
1.),(1.,1.),(1.,1.),(1.,1.),(1.,1.),(1.,1.),(1.,1.),(1.,1.),(1.,1.),(1.,
1.),(1.,1.),(1.,1.),(1.,1.),(1.,1.),(1.,1.),(1.,1.),(1.,1.),(1.,1.),(1.,
1.),(1.,1.),(1.,1.),(1.,1.),(1.,1.),(1.,1.),(1.,1.),(1.,1.),(1.,1.),(1.,
1.),(1.,1.),(1.,1.),(1.,1.),(1.,1.),(1.,1.),(1.,1.),(1.,1.),(1.,1.),(1.,
1.),(1.,1.),(1.,1.),(1.,1.),(1.,1.),(1.,1.),(1.,1.),(1.,1.),(1.,1.),(1.,
1.),(1.,1.),(1.,1.),(1.,1.),(1.,1.),(1.,1.),(1.,1.),(1.,1.),(1.,1.),(1.,
1.),(1.,1.),(1.,1.),(1.,1.),(1.,1.),(1.,1.),(1.,1.),(1.,1.),(1.,1.),(1.,
1.),(1.,1.),(1.,1.),(1.,1.),(1.,1.),(1.,1.),(1.,1.),(1.,1.),(1.,1.),(1.,
1.),(1.,1.)))
REPRESENTATION_ITEM('')
SURFACE()
);
#1089=(
BOUNDED_SURFACE()
B_SPLINE_SURFACE(5,1,((#227572,#227573),(#227574,#227575),(#227576,#227577),
(#227578,#227579),(#227580,#227581),(#227582,#227583),(#227584,#227585),
(#227586,#227587),(#227588,#227589),(#227590,#227591),(#227592,#227593),
(#227594,#227595),(#227596,#227597),(#227598,#227599),(#227600,#227601),
(#227602,#227603),(#227604,#227605),(#227606,#227607),(#227608,#227609),
(#227610,#227611),(#227612,#227613),(#227614,#227615),(#227616,#227617),
(#227618,#227619),(#227620,#227621),(#227622,#227623),(#227624,#227625),
(#227626,#227627),(#227628,#227629),(#227630,#227631),(#227632,#227633),
(#227634,#227635),(#227636,#227637),(#227638,#227639),(#227640,#227641),
(#227642,#227643),(#227644,#227645),(#227646,#227647),(#227648,#227649),
(#227650,#227651),(#227652,#227653),(#227654,#227655),(#227656,#227657),
(#227658,#227659),(#227660,#227661),(#227662,#227663),(#227664,#227665),
(#227666,#227667),(#227668,#227669),(#227670,#227671),(#227672,#227673),
(#227674,#227675),(#227676,#227677),(#227678,#227679),(#227680,#227681),
(#227682,#227683),(#227684,#227685),(#227686,#227687),(#227688,#227689),
(#227690,#227691),(#227692,#227693),(#227694,#227695),(#227696,#227697),
(#227698,#227699),(#227700,#227701),(#227702,#227703),(#227704,#227705),
(#227706,#227707),(#227708,#227709),(#227710,#227711),(#227712,#227713),
(#227714,#227715),(#227716,#227717),(#227718,#227719),(#227720,#227721),
(#227722,#227723),(#227724,#227725),(#227726,#227727),(#227728,#227729),
(#227730,#227731),(#227732,#227733),(#227734,#227735),(#227736,#227737),
(#227738,#227739),(#227740,#227741),(#227742,#227743),(#227744,#227745),
(#227746,#227747),(#227748,#227749),(#227750,#227751),(#227752,#227753),
(#227754,#227755),(#227756,#227757),(#227758,#227759),(#227760,#227761),
(#227762,#227763),(#227764,#227765),(#227766,#227767),(#227768,#227769),
(#227770,#227771),(#227772,#227773),(#227774,#227775),(#227776,#227777),
(#227778,#227779),(#227780,#227781),(#227782,#227783),(#227784,#227785),
(#227786,#227787),(#227788,#227789),(#227790,#227791),(#227792,#227793),
(#227794,#227795),(#227796,#227797),(#227798,#227799),(#227800,#227801),
(#227802,#227803),(#227804,#227805),(#227806,#227807),(#227808,#227809),
(#227810,#227811),(#227812,#227813),(#227814,#227815),(#227816,#227817),
(#227818,#227819),(#227820,#227821),(#227822,#227823),(#227824,#227825),
(#227826,#227827),(#227828,#227829),(#227830,#227831),(#227832,#227833),
(#227834,#227835),(#227836,#227837),(#227838,#227839),(#227840,#227841),
(#227842,#227843),(#227844,#227845),(#227846,#227847),(#227848,#227849),
(#227850,#227851),(#227852,#227853),(#227854,#227855),(#227856,#227857),
(#227858,#227859),(#227860,#227861),(#227862,#227863),(#227864,#227865),
(#227866,#227867),(#227868,#227869),(#227870,#227871),(#227872,#227873),
(#227874,#227875),(#227876,#227877),(#227878,#227879),(#227880,#227881),
(#227882,#227883),(#227884,#227885),(#227886,#227887),(#227888,#227889),
(#227890,#227891),(#227892,#227893),(#227894,#227895),(#227896,#227897),
(#227898,#227899),(#227900,#227901),(#227902,#227903),(#227904,#227905),
(#227906,#227907),(#227908,#227909),(#227910,#227911),(#227912,#227913),
(#227914,#227915),(#227916,#227917),(#227918,#227919),(#227920,#227921),
(#227922,#227923),(#227924,#227925),(#227926,#227927),(#227928,#227929),
(#227930,#227931),(#227932,#227933),(#227934,#227935),(#227936,#227937),
(#227938,#227939),(#227940,#227941),(#227942,#227943),(#227944,#227945),
(#227946,#227947),(#227948,#227949),(#227950,#227951),(#227952,#227953),
(#227954,#227955),(#227956,#227957),(#227958,#227959),(#227960,#227961),
(#227962,#227963),(#227964,#227965),(#227966,#227967),(#227968,#227969),
(#227970,#227971),(#227972,#227973),(#227974,#227975),(#227976,#227977),
(#227978,#227979),(#227980,#227981)),.UNSPECIFIED.,.F.,.F.,.F.)
B_SPLINE_SURFACE_WITH_KNOTS((6,1,1,1,1,1,1,1,1,1,1,1,1,1,1,1,1,1,1,1,1,
1,1,1,1,1,1,1,1,1,1,1,1,1,1,1,1,1,1,1,1,1,1,1,1,1,1,1,1,1,1,1,1,1,1,1,1,
1,1,1,1,1,1,1,1,1,1,1,1,1,1,1,1,1,1,1,1,1,1,1,1,1,1,1,1,1,1,1,1,1,1,1,1,
1,1,1,1,1,1,1,1,1,1,1,1,1,1,1,1,1,1,1,1,1,1,1,1,1,1,1,1,1,1,1,1,1,1,1,1,
1,1,1,1,1,1,1,1,1,1,1,1,1,1,1,1,1,1,1,1,1,1,1,1,1,1,1,1,1,1,1,1,1,1,1,1,
1,1,1,1,1,1,1,1,1,1,1,1,1,1,1,1,1,1,1,1,1,1,1,1,1,1,1,1,1,1,1,1,1,1,1,6),
(2,2),(-1.,-0.995000000000001,-0.990000000000001,-0.985000000000001,-0.980000000000001,
-0.975000000000001,-0.970000000000001,-0.965000000000001,-0.960000000000001,
-0.955000000000001,-0.950000000000001,-0.945000000000001,-0.940000000000001,
-0.935000000000001,-0.930000000000001,-0.925000000000001,-0.920000000000001,
-0.915000000000001,-0.910000000000001,-0.905000000000001,-0.900000000000001,
-0.895000000000001,-0.890000000000001,-0.885000000000001,-0.880000000000001,
-0.875000000000001,-0.870000000000001,-0.865000000000001,-0.860000000000001,
-0.855000000000001,-0.850000000000001,-0.845000000000001,-0.840000000000001,
-0.835000000000001,-0.830000000000001,-0.825000000000001,-0.820000000000001,
-0.815000000000001,-0.810000000000001,-0.805000000000001,-0.800000000000001,
-0.795000000000001,-0.790000000000001,-0.785000000000001,-0.780000000000001,
-0.775000000000001,-0.770000000000001,-0.765000000000001,-0.760000000000001,
-0.755000000000001,-0.750000000000001,-0.745000000000001,-0.740000000000001,
-0.735000000000001,-0.730000000000001,-0.725000000000001,-0.720000000000001,
-0.715000000000001,-0.710000000000001,-0.705000000000001,-0.700000000000001,
-0.695000000000001,-0.690000000000001,-0.685,-0.68,-0.675,-0.67,-0.665,
-0.66,-0.655,-0.65,-0.645,-0.64,-0.635,-0.63,-0.625,-0.62,-0.615,-0.61,
-0.605,-0.6,-0.595,-0.59,-0.585,-0.58,-0.575,-0.57,-0.565,-0.56,-0.555,
-0.55,-0.545,-0.54,-0.535,-0.53,-0.525,-0.52,-0.515,-0.51,-0.505,-0.5,-0.495,
-0.49,-0.485,-0.48,-0.475,-0.47,-0.465,-0.46,-0.455,-0.45,-0.445,-0.44,
-0.435,-0.43,-0.425,-0.42,-0.415,-0.41,-0.405,-0.4,-0.395,-0.39,-0.385,
-0.38,-0.375,-0.37,-0.365,-0.36,-0.355,-0.35,-0.345,-0.34,-0.335,-0.33,
-0.325,-0.32,-0.315,-0.31,-0.305,-0.3,-0.295,-0.29,-0.285,-0.28,-0.275,
-0.27,-0.265,-0.26,-0.255,-0.25,-0.245,-0.24,-0.235,-0.23,-0.225,-0.22,
-0.215,-0.21,-0.205,-0.2,-0.195,-0.19,-0.185,-0.18,-0.175,-0.17,-0.165,
-0.16,-0.155,-0.15,-0.145,-0.14,-0.135,-0.13,-0.125,-0.12,-0.115,-0.11,
-0.105,-0.1,-0.095,-0.09,-0.085,-0.08,-0.075,-0.07,-0.065,-0.06,-0.055,
-0.05,-0.045,-0.04,-0.035,-0.03,-0.025,-0.02,-0.015,-0.01,-0.005,0.),(0.,
1.2),.UNSPECIFIED.)
GEOMETRIC_REPRESENTATION_ITEM()
RATIONAL_B_SPLINE_SURFACE(((1.,1.),(1.,1.),(1.,1.),(1.,1.),(1.,1.),(1.,
1.),(1.,1.),(1.,1.),(1.,1.),(1.,1.),(1.,1.),(1.,1.),(1.,1.),(1.,1.),(1.,
1.),(1.,1.),(1.,1.),(1.,1.),(1.,1.),(1.,1.),(1.,1.),(1.,1.),(1.,1.),(1.,
1.),(1.,1.),(1.,1.),(1.,1.),(1.,1.),(1.,1.),(1.,1.),(1.,1.),(1.,1.),(1.,
1.),(1.,1.),(1.,1.),(1.,1.),(1.,1.),(1.,1.),(1.,1.),(1.,1.),(1.,1.),(1.,
1.),(1.,1.),(1.,1.),(1.,1.),(1.,1.),(1.,1.),(1.,1.),(1.,1.),(1.,1.),(1.,
1.),(1.,1.),(1.,1.),(1.,1.),(1.,1.),(1.,1.),(1.,1.),(1.,1.),(1.,1.),(1.,
1.),(1.,1.),(1.,1.),(1.,1.),(1.,1.),(1.,1.),(1.,1.),(1.,1.),(1.,1.),(1.,
1.),(1.,1.),(1.,1.),(1.,1.),(1.,1.),(1.,1.),(1.,1.),(1.,1.),(1.,1.),(1.,
1.),(1.,1.),(1.,1.),(1.,1.),(1.,1.),(1.,1.),(1.,1.),(1.,1.),(1.,1.),(1.,
1.),(1.,1.),(1.,1.),(1.,1.),(1.,1.),(1.,1.),(1.,1.),(1.,1.),(1.,1.),(1.,
1.),(1.,1.),(1.,1.),(1.,1.),(1.,1.),(1.,1.),(1.,1.),(1.,1.),(1.,1.),(1.,
1.),(1.,1.),(1.,1.),(1.,1.),(1.,1.),(1.,1.),(1.,1.),(1.,1.),(1.,1.),(1.,
1.),(1.,1.),(1.,1.),(1.,1.),(1.,1.),(1.,1.),(1.,1.),(1.,1.),(1.,1.),(1.,
1.),(1.,1.),(1.,1.),(1.,1.),(1.,1.),(1.,1.),(1.,1.),(1.,1.),(1.,1.),(1.,
1.),(1.,1.),(1.,1.),(1.,1.),(1.,1.),(1.,1.),(1.,1.),(1.,1.),(1.,1.),(1.,
1.),(1.,1.),(1.,1.),(1.,1.),(1.,1.),(1.,1.),(1.,1.),(1.,1.),(1.,1.),(1.,
1.),(1.,1.),(1.,1.),(1.,1.),(1.,1.),(1.,1.),(1.,1.),(1.,1.),(1.,1.),(1.,
1.),(1.,1.),(1.,1.),(1.,1.),(1.,1.),(1.,1.),(1.,1.),(1.,1.),(1.,1.),(1.,
1.),(1.,1.),(1.,1.),(1.,1.),(1.,1.),(1.,1.),(1.,1.),(1.,1.),(1.,1.),(1.,
1.),(1.,1.),(1.,1.),(1.,1.),(1.,1.),(1.,1.),(1.,1.),(1.,1.),(1.,1.),(1.,
1.),(1.,1.),(1.,1.),(1.,1.),(1.,1.),(1.,1.),(1.,1.),(1.,1.),(1.,1.),(1.,
1.),(1.,1.),(1.,1.),(1.,1.),(1.,1.),(1.,1.),(1.,1.),(1.,1.),(1.,1.),(1.,
1.),(1.,1.)))
REPRESENTATION_ITEM('')
SURFACE()
);
#1090=(
BOUNDED_SURFACE()
B_SPLINE_SURFACE(5,1,((#228395,#228396),(#228397,#228398),(#228399,#228400),
(#228401,#228402),(#228403,#228404),(#228405,#228406),(#228407,#228408),
(#228409,#228410),(#228411,#228412),(#228413,#228414),(#228415,#228416),
(#228417,#228418),(#228419,#228420),(#228421,#228422),(#228423,#228424),
(#228425,#228426),(#228427,#228428),(#228429,#228430),(#228431,#228432),
(#228433,#228434),(#228435,#228436),(#228437,#228438),(#228439,#228440),
(#228441,#228442),(#228443,#228444),(#228445,#228446),(#228447,#228448),
(#228449,#228450),(#228451,#228452),(#228453,#228454),(#228455,#228456),
(#228457,#228458),(#228459,#228460),(#228461,#228462),(#228463,#228464),
(#228465,#228466),(#228467,#228468),(#228469,#228470),(#228471,#228472),
(#228473,#228474),(#228475,#228476),(#228477,#228478),(#228479,#228480),
(#228481,#228482),(#228483,#228484),(#228485,#228486),(#228487,#228488),
(#228489,#228490),(#228491,#228492),(#228493,#228494),(#228495,#228496),
(#228497,#228498),(#228499,#228500),(#228501,#228502),(#228503,#228504),
(#228505,#228506),(#228507,#228508),(#228509,#228510),(#228511,#228512),
(#228513,#228514),(#228515,#228516),(#228517,#228518),(#228519,#228520),
(#228521,#228522),(#228523,#228524),(#228525,#228526),(#228527,#228528),
(#228529,#228530),(#228531,#228532),(#228533,#228534),(#228535,#228536),
(#228537,#228538),(#228539,#228540),(#228541,#228542),(#228543,#228544),
(#228545,#228546),(#228547,#228548),(#228549,#228550),(#228551,#228552),
(#228553,#228554),(#228555,#228556),(#228557,#228558),(#228559,#228560),
(#228561,#228562),(#228563,#228564),(#228565,#228566),(#228567,#228568),
(#228569,#228570),(#228571,#228572),(#228573,#228574),(#228575,#228576),
(#228577,#228578),(#228579,#228580),(#228581,#228582),(#228583,#228584),
(#228585,#228586),(#228587,#228588),(#228589,#228590),(#228591,#228592),
(#228593,#228594),(#228595,#228596),(#228597,#228598),(#228599,#228600),
(#228601,#228602),(#228603,#228604),(#228605,#228606),(#228607,#228608),
(#228609,#228610),(#228611,#228612),(#228613,#228614),(#228615,#228616),
(#228617,#228618),(#228619,#228620),(#228621,#228622),(#228623,#228624),
(#228625,#228626),(#228627,#228628),(#228629,#228630),(#228631,#228632),
(#228633,#228634),(#228635,#228636),(#228637,#228638),(#228639,#228640),
(#228641,#228642),(#228643,#228644),(#228645,#228646),(#228647,#228648),
(#228649,#228650),(#228651,#228652),(#228653,#228654),(#228655,#228656),
(#228657,#228658),(#228659,#228660),(#228661,#228662),(#228663,#228664),
(#228665,#228666),(#228667,#228668),(#228669,#228670),(#228671,#228672),
(#228673,#228674),(#228675,#228676),(#228677,#228678),(#228679,#228680),
(#228681,#228682),(#228683,#228684),(#228685,#228686),(#228687,#228688),
(#228689,#228690),(#228691,#228692),(#228693,#228694),(#228695,#228696),
(#228697,#228698),(#228699,#228700),(#228701,#228702),(#228703,#228704),
(#228705,#228706),(#228707,#228708),(#228709,#228710),(#228711,#228712),
(#228713,#228714),(#228715,#228716),(#228717,#228718),(#228719,#228720),
(#228721,#228722),(#228723,#228724),(#228725,#228726),(#228727,#228728),
(#228729,#228730),(#228731,#228732),(#228733,#228734),(#228735,#228736),
(#228737,#228738),(#228739,#228740),(#228741,#228742),(#228743,#228744),
(#228745,#228746),(#228747,#228748),(#228749,#228750),(#228751,#228752),
(#228753,#228754),(#228755,#228756),(#228757,#228758),(#228759,#228760),
(#228761,#228762),(#228763,#228764),(#228765,#228766),(#228767,#228768),
(#228769,#228770),(#228771,#228772),(#228773,#228774),(#228775,#228776),
(#228777,#228778),(#228779,#228780),(#228781,#228782),(#228783,#228784),
(#228785,#228786),(#228787,#228788),(#228789,#228790),(#228791,#228792),
(#228793,#228794),(#228795,#228796),(#228797,#228798),(#228799,#228800),
(#228801,#228802),(#228803,#228804)),.UNSPECIFIED.,.F.,.F.,.F.)
B_SPLINE_SURFACE_WITH_KNOTS((6,1,1,1,1,1,1,1,1,1,1,1,1,1,1,1,1,1,1,1,1,
1,1,1,1,1,1,1,1,1,1,1,1,1,1,1,1,1,1,1,1,1,1,1,1,1,1,1,1,1,1,1,1,1,1,1,1,
1,1,1,1,1,1,1,1,1,1,1,1,1,1,1,1,1,1,1,1,1,1,1,1,1,1,1,1,1,1,1,1,1,1,1,1,
1,1,1,1,1,1,1,1,1,1,1,1,1,1,1,1,1,1,1,1,1,1,1,1,1,1,1,1,1,1,1,1,1,1,1,1,
1,1,1,1,1,1,1,1,1,1,1,1,1,1,1,1,1,1,1,1,1,1,1,1,1,1,1,1,1,1,1,1,1,1,1,1,
1,1,1,1,1,1,1,1,1,1,1,1,1,1,1,1,1,1,1,1,1,1,1,1,1,1,1,1,1,1,1,1,1,1,1,6),
(2,2),(0.,0.005,0.01,0.015,0.02,0.025,0.03,0.035,0.04,0.045,0.05,0.055,
0.06,0.065,0.07,0.075,0.08,0.085,0.09,0.095,0.1,0.105,0.11,0.115,0.12,0.125,
0.13,0.135,0.14,0.145,0.15,0.155,0.16,0.165,0.17,0.175,0.18,0.185,0.19,
0.195,0.2,0.205,0.21,0.215,0.22,0.225,0.23,0.235,0.24,0.245,0.25,0.255,
0.26,0.265,0.27,0.275,0.28,0.285,0.29,0.295,0.3,0.305,0.31,0.315,0.32,0.325,
0.33,0.335,0.34,0.345,0.35,0.355,0.36,0.365,0.37,0.375,0.38,0.385,0.39,
0.395,0.4,0.405,0.41,0.415,0.42,0.425,0.43,0.435,0.44,0.445,0.45,0.455,
0.46,0.465,0.47,0.475,0.48,0.485,0.49,0.495,0.5,0.505,0.51,0.515,0.52,0.525,
0.53,0.535,0.54,0.545,0.55,0.555,0.56,0.565,0.57,0.575,0.58,0.585,0.59,
0.595,0.6,0.605,0.61,0.615,0.62,0.625,0.63,0.635,0.64,0.645,0.65,0.655,
0.66,0.665,0.67,0.675,0.68,0.685,0.690000000000001,0.695000000000001,0.700000000000001,
0.705000000000001,0.710000000000001,0.715000000000001,0.720000000000001,
0.725000000000001,0.730000000000001,0.735000000000001,0.740000000000001,
0.745000000000001,0.750000000000001,0.755000000000001,0.760000000000001,
0.765000000000001,0.770000000000001,0.775000000000001,0.780000000000001,
0.785000000000001,0.790000000000001,0.795000000000001,0.800000000000001,
0.805000000000001,0.810000000000001,0.815000000000001,0.820000000000001,
0.825000000000001,0.830000000000001,0.835000000000001,0.840000000000001,
0.845000000000001,0.850000000000001,0.855000000000001,0.860000000000001,
0.865000000000001,0.870000000000001,0.875000000000001,0.880000000000001,
0.885000000000001,0.890000000000001,0.895000000000001,0.900000000000001,
0.905000000000001,0.910000000000001,0.915000000000001,0.920000000000001,
0.925000000000001,0.930000000000001,0.935000000000001,0.940000000000001,
0.945000000000001,0.950000000000001,0.955000000000001,0.960000000000001,
0.965000000000001,0.970000000000001,0.975000000000001,0.980000000000001,
0.985000000000001,0.990000000000001,0.995000000000001,1.),(0.,1.2),
 .UNSPECIFIED.)
GEOMETRIC_REPRESENTATION_ITEM()
RATIONAL_B_SPLINE_SURFACE(((1.,1.),(1.,1.),(1.,1.),(1.,1.),(1.,1.),(1.,
1.),(1.,1.),(1.,1.),(1.,1.),(1.,1.),(1.,1.),(1.,1.),(1.,1.),(1.,1.),(1.,
1.),(1.,1.),(1.,1.),(1.,1.),(1.,1.),(1.,1.),(1.,1.),(1.,1.),(1.,1.),(1.,
1.),(1.,1.),(1.,1.),(1.,1.),(1.,1.),(1.,1.),(1.,1.),(1.,1.),(1.,1.),(1.,
1.),(1.,1.),(1.,1.),(1.,1.),(1.,1.),(1.,1.),(1.,1.),(1.,1.),(1.,1.),(1.,
1.),(1.,1.),(1.,1.),(1.,1.),(1.,1.),(1.,1.),(1.,1.),(1.,1.),(1.,1.),(1.,
1.),(1.,1.),(1.,1.),(1.,1.),(1.,1.),(1.,1.),(1.,1.),(1.,1.),(1.,1.),(1.,
1.),(1.,1.),(1.,1.),(1.,1.),(1.,1.),(1.,1.),(1.,1.),(1.,1.),(1.,1.),(1.,
1.),(1.,1.),(1.,1.),(1.,1.),(1.,1.),(1.,1.),(1.,1.),(1.,1.),(1.,1.),(1.,
1.),(1.,1.),(1.,1.),(1.,1.),(1.,1.),(1.,1.),(1.,1.),(1.,1.),(1.,1.),(1.,
1.),(1.,1.),(1.,1.),(1.,1.),(1.,1.),(1.,1.),(1.,1.),(1.,1.),(1.,1.),(1.,
1.),(1.,1.),(1.,1.),(1.,1.),(1.,1.),(1.,1.),(1.,1.),(1.,1.),(1.,1.),(1.,
1.),(1.,1.),(1.,1.),(1.,1.),(1.,1.),(1.,1.),(1.,1.),(1.,1.),(1.,1.),(1.,
1.),(1.,1.),(1.,1.),(1.,1.),(1.,1.),(1.,1.),(1.,1.),(1.,1.),(1.,1.),(1.,
1.),(1.,1.),(1.,1.),(1.,1.),(1.,1.),(1.,1.),(1.,1.),(1.,1.),(1.,1.),(1.,
1.),(1.,1.),(1.,1.),(1.,1.),(1.,1.),(1.,1.),(1.,1.),(1.,1.),(1.,1.),(1.,
1.),(1.,1.),(1.,1.),(1.,1.),(1.,1.),(1.,1.),(1.,1.),(1.,1.),(1.,1.),(1.,
1.),(1.,1.),(1.,1.),(1.,1.),(1.,1.),(1.,1.),(1.,1.),(1.,1.),(1.,1.),(1.,
1.),(1.,1.),(1.,1.),(1.,1.),(1.,1.),(1.,1.),(1.,1.),(1.,1.),(1.,1.),(1.,
1.),(1.,1.),(1.,1.),(1.,1.),(1.,1.),(1.,1.),(1.,1.),(1.,1.),(1.,1.),(1.,
1.),(1.,1.),(1.,1.),(1.,1.),(1.,1.),(1.,1.),(1.,1.),(1.,1.),(1.,1.),(1.,
1.),(1.,1.),(1.,1.),(1.,1.),(1.,1.),(1.,1.),(1.,1.),(1.,1.),(1.,1.),(1.,
1.),(1.,1.),(1.,1.),(1.,1.),(1.,1.),(1.,1.),(1.,1.),(1.,1.),(1.,1.),(1.,
1.),(1.,1.)))
REPRESENTATION_ITEM('')
SURFACE()
);
#1091=(
BOUNDED_SURFACE()
B_SPLINE_SURFACE(5,1,((#229224,#229225),(#229226,#229227),(#229228,#229229),
(#229230,#229231),(#229232,#229233),(#229234,#229235),(#229236,#229237),
(#229238,#229239),(#229240,#229241),(#229242,#229243),(#229244,#229245),
(#229246,#229247),(#229248,#229249),(#229250,#229251),(#229252,#229253),
(#229254,#229255),(#229256,#229257),(#229258,#229259),(#229260,#229261),
(#229262,#229263),(#229264,#229265),(#229266,#229267),(#229268,#229269),
(#229270,#229271),(#229272,#229273),(#229274,#229275),(#229276,#229277),
(#229278,#229279),(#229280,#229281),(#229282,#229283),(#229284,#229285),
(#229286,#229287),(#229288,#229289),(#229290,#229291),(#229292,#229293),
(#229294,#229295),(#229296,#229297),(#229298,#229299),(#229300,#229301),
(#229302,#229303),(#229304,#229305),(#229306,#229307),(#229308,#229309),
(#229310,#229311),(#229312,#229313),(#229314,#229315),(#229316,#229317),
(#229318,#229319),(#229320,#229321),(#229322,#229323),(#229324,#229325),
(#229326,#229327),(#229328,#229329),(#229330,#229331),(#229332,#229333),
(#229334,#229335),(#229336,#229337),(#229338,#229339),(#229340,#229341),
(#229342,#229343),(#229344,#229345),(#229346,#229347),(#229348,#229349),
(#229350,#229351),(#229352,#229353),(#229354,#229355),(#229356,#229357),
(#229358,#229359),(#229360,#229361),(#229362,#229363),(#229364,#229365),
(#229366,#229367),(#229368,#229369),(#229370,#229371),(#229372,#229373),
(#229374,#229375),(#229376,#229377),(#229378,#229379),(#229380,#229381),
(#229382,#229383),(#229384,#229385),(#229386,#229387),(#229388,#229389),
(#229390,#229391),(#229392,#229393),(#229394,#229395),(#229396,#229397),
(#229398,#229399),(#229400,#229401),(#229402,#229403),(#229404,#229405),
(#229406,#229407),(#229408,#229409),(#229410,#229411),(#229412,#229413),
(#229414,#229415),(#229416,#229417),(#229418,#229419),(#229420,#229421),
(#229422,#229423),(#229424,#229425),(#229426,#229427),(#229428,#229429),
(#229430,#229431),(#229432,#229433),(#229434,#229435),(#229436,#229437),
(#229438,#229439),(#229440,#229441),(#229442,#229443),(#229444,#229445),
(#229446,#229447),(#229448,#229449),(#229450,#229451),(#229452,#229453),
(#229454,#229455),(#229456,#229457),(#229458,#229459),(#229460,#229461),
(#229462,#229463),(#229464,#229465),(#229466,#229467),(#229468,#229469),
(#229470,#229471),(#229472,#229473),(#229474,#229475),(#229476,#229477),
(#229478,#229479),(#229480,#229481),(#229482,#229483),(#229484,#229485),
(#229486,#229487),(#229488,#229489),(#229490,#229491),(#229492,#229493),
(#229494,#229495),(#229496,#229497),(#229498,#229499),(#229500,#229501),
(#229502,#229503),(#229504,#229505),(#229506,#229507),(#229508,#229509),
(#229510,#229511),(#229512,#229513),(#229514,#229515),(#229516,#229517),
(#229518,#229519),(#229520,#229521),(#229522,#229523),(#229524,#229525),
(#229526,#229527),(#229528,#229529),(#229530,#229531),(#229532,#229533),
(#229534,#229535),(#229536,#229537),(#229538,#229539),(#229540,#229541),
(#229542,#229543),(#229544,#229545),(#229546,#229547),(#229548,#229549),
(#229550,#229551),(#229552,#229553),(#229554,#229555),(#229556,#229557),
(#229558,#229559),(#229560,#229561),(#229562,#229563),(#229564,#229565),
(#229566,#229567),(#229568,#229569),(#229570,#229571),(#229572,#229573),
(#229574,#229575),(#229576,#229577),(#229578,#229579),(#229580,#229581),
(#229582,#229583),(#229584,#229585),(#229586,#229587),(#229588,#229589),
(#229590,#229591),(#229592,#229593),(#229594,#229595),(#229596,#229597),
(#229598,#229599),(#229600,#229601),(#229602,#229603),(#229604,#229605),
(#229606,#229607),(#229608,#229609),(#229610,#229611),(#229612,#229613),
(#229614,#229615),(#229616,#229617),(#229618,#229619),(#229620,#229621),
(#229622,#229623),(#229624,#229625),(#229626,#229627),(#229628,#229629),
(#229630,#229631),(#229632,#229633)),.UNSPECIFIED.,.F.,.F.,.F.)
B_SPLINE_SURFACE_WITH_KNOTS((6,1,1,1,1,1,1,1,1,1,1,1,1,1,1,1,1,1,1,1,1,
1,1,1,1,1,1,1,1,1,1,1,1,1,1,1,1,1,1,1,1,1,1,1,1,1,1,1,1,1,1,1,1,1,1,1,1,
1,1,1,1,1,1,1,1,1,1,1,1,1,1,1,1,1,1,1,1,1,1,1,1,1,1,1,1,1,1,1,1,1,1,1,1,
1,1,1,1,1,1,1,1,1,1,1,1,1,1,1,1,1,1,1,1,1,1,1,1,1,1,1,1,1,1,1,1,1,1,1,1,
1,1,1,1,1,1,1,1,1,1,1,1,1,1,1,1,1,1,1,1,1,1,1,1,1,1,1,1,1,1,1,1,1,1,1,1,
1,1,1,1,1,1,1,1,1,1,1,1,1,1,1,1,1,1,1,1,1,1,1,1,1,1,1,1,1,1,1,1,1,1,1,6),
(2,2),(-1.,-0.995000000000001,-0.990000000000001,-0.985000000000001,-0.980000000000001,
-0.975000000000001,-0.970000000000001,-0.965000000000001,-0.960000000000001,
-0.955000000000001,-0.950000000000001,-0.945000000000001,-0.940000000000001,
-0.935000000000001,-0.930000000000001,-0.925000000000001,-0.920000000000001,
-0.915000000000001,-0.910000000000001,-0.905000000000001,-0.900000000000001,
-0.895000000000001,-0.890000000000001,-0.885000000000001,-0.880000000000001,
-0.875000000000001,-0.870000000000001,-0.865000000000001,-0.860000000000001,
-0.855000000000001,-0.850000000000001,-0.845000000000001,-0.840000000000001,
-0.835000000000001,-0.830000000000001,-0.825000000000001,-0.820000000000001,
-0.815000000000001,-0.810000000000001,-0.805000000000001,-0.800000000000001,
-0.795000000000001,-0.790000000000001,-0.785000000000001,-0.780000000000001,
-0.775000000000001,-0.770000000000001,-0.765000000000001,-0.760000000000001,
-0.755000000000001,-0.750000000000001,-0.745000000000001,-0.740000000000001,
-0.735000000000001,-0.730000000000001,-0.725000000000001,-0.720000000000001,
-0.715000000000001,-0.710000000000001,-0.705000000000001,-0.700000000000001,
-0.695000000000001,-0.690000000000001,-0.685,-0.68,-0.675,-0.67,-0.665,
-0.66,-0.655,-0.65,-0.645,-0.64,-0.635,-0.63,-0.625,-0.62,-0.615,-0.61,
-0.605,-0.6,-0.595,-0.59,-0.585,-0.58,-0.575,-0.57,-0.565,-0.56,-0.555,
-0.55,-0.545,-0.54,-0.535,-0.53,-0.525,-0.52,-0.515,-0.51,-0.505,-0.5,-0.495,
-0.49,-0.485,-0.48,-0.475,-0.47,-0.465,-0.46,-0.455,-0.45,-0.445,-0.44,
-0.435,-0.43,-0.425,-0.42,-0.415,-0.41,-0.405,-0.4,-0.395,-0.39,-0.385,
-0.38,-0.375,-0.37,-0.365,-0.36,-0.355,-0.35,-0.345,-0.34,-0.335,-0.33,
-0.325,-0.32,-0.315,-0.31,-0.305,-0.3,-0.295,-0.29,-0.285,-0.28,-0.275,
-0.27,-0.265,-0.26,-0.255,-0.25,-0.245,-0.24,-0.235,-0.23,-0.225,-0.22,
-0.215,-0.21,-0.205,-0.2,-0.195,-0.19,-0.185,-0.18,-0.175,-0.17,-0.165,
-0.16,-0.155,-0.15,-0.145,-0.14,-0.135,-0.13,-0.125,-0.12,-0.115,-0.11,
-0.105,-0.1,-0.095,-0.09,-0.085,-0.08,-0.075,-0.07,-0.065,-0.06,-0.055,
-0.05,-0.045,-0.04,-0.035,-0.03,-0.025,-0.02,-0.015,-0.01,-0.005,0.),(0.,
1.2),.UNSPECIFIED.)
GEOMETRIC_REPRESENTATION_ITEM()
RATIONAL_B_SPLINE_SURFACE(((1.,1.),(1.,1.),(1.,1.),(1.,1.),(1.,1.),(1.,
1.),(1.,1.),(1.,1.),(1.,1.),(1.,1.),(1.,1.),(1.,1.),(1.,1.),(1.,1.),(1.,
1.),(1.,1.),(1.,1.),(1.,1.),(1.,1.),(1.,1.),(1.,1.),(1.,1.),(1.,1.),(1.,
1.),(1.,1.),(1.,1.),(1.,1.),(1.,1.),(1.,1.),(1.,1.),(1.,1.),(1.,1.),(1.,
1.),(1.,1.),(1.,1.),(1.,1.),(1.,1.),(1.,1.),(1.,1.),(1.,1.),(1.,1.),(1.,
1.),(1.,1.),(1.,1.),(1.,1.),(1.,1.),(1.,1.),(1.,1.),(1.,1.),(1.,1.),(1.,
1.),(1.,1.),(1.,1.),(1.,1.),(1.,1.),(1.,1.),(1.,1.),(1.,1.),(1.,1.),(1.,
1.),(1.,1.),(1.,1.),(1.,1.),(1.,1.),(1.,1.),(1.,1.),(1.,1.),(1.,1.),(1.,
1.),(1.,1.),(1.,1.),(1.,1.),(1.,1.),(1.,1.),(1.,1.),(1.,1.),(1.,1.),(1.,
1.),(1.,1.),(1.,1.),(1.,1.),(1.,1.),(1.,1.),(1.,1.),(1.,1.),(1.,1.),(1.,
1.),(1.,1.),(1.,1.),(1.,1.),(1.,1.),(1.,1.),(1.,1.),(1.,1.),(1.,1.),(1.,
1.),(1.,1.),(1.,1.),(1.,1.),(1.,1.),(1.,1.),(1.,1.),(1.,1.),(1.,1.),(1.,
1.),(1.,1.),(1.,1.),(1.,1.),(1.,1.),(1.,1.),(1.,1.),(1.,1.),(1.,1.),(1.,
1.),(1.,1.),(1.,1.),(1.,1.),(1.,1.),(1.,1.),(1.,1.),(1.,1.),(1.,1.),(1.,
1.),(1.,1.),(1.,1.),(1.,1.),(1.,1.),(1.,1.),(1.,1.),(1.,1.),(1.,1.),(1.,
1.),(1.,1.),(1.,1.),(1.,1.),(1.,1.),(1.,1.),(1.,1.),(1.,1.),(1.,1.),(1.,
1.),(1.,1.),(1.,1.),(1.,1.),(1.,1.),(1.,1.),(1.,1.),(1.,1.),(1.,1.),(1.,
1.),(1.,1.),(1.,1.),(1.,1.),(1.,1.),(1.,1.),(1.,1.),(1.,1.),(1.,1.),(1.,
1.),(1.,1.),(1.,1.),(1.,1.),(1.,1.),(1.,1.),(1.,1.),(1.,1.),(1.,1.),(1.,
1.),(1.,1.),(1.,1.),(1.,1.),(1.,1.),(1.,1.),(1.,1.),(1.,1.),(1.,1.),(1.,
1.),(1.,1.),(1.,1.),(1.,1.),(1.,1.),(1.,1.),(1.,1.),(1.,1.),(1.,1.),(1.,
1.),(1.,1.),(1.,1.),(1.,1.),(1.,1.),(1.,1.),(1.,1.),(1.,1.),(1.,1.),(1.,
1.),(1.,1.),(1.,1.),(1.,1.),(1.,1.),(1.,1.),(1.,1.),(1.,1.),(1.,1.),(1.,
1.),(1.,1.)))
REPRESENTATION_ITEM('')
SURFACE()
);
#1092=(
BOUNDED_SURFACE()
B_SPLINE_SURFACE(5,1,((#230047,#230048),(#230049,#230050),(#230051,#230052),
(#230053,#230054),(#230055,#230056),(#230057,#230058),(#230059,#230060),
(#230061,#230062),(#230063,#230064),(#230065,#230066),(#230067,#230068),
(#230069,#230070),(#230071,#230072),(#230073,#230074),(#230075,#230076),
(#230077,#230078),(#230079,#230080),(#230081,#230082),(#230083,#230084),
(#230085,#230086),(#230087,#230088),(#230089,#230090),(#230091,#230092),
(#230093,#230094),(#230095,#230096),(#230097,#230098),(#230099,#230100),
(#230101,#230102),(#230103,#230104),(#230105,#230106),(#230107,#230108),
(#230109,#230110),(#230111,#230112),(#230113,#230114),(#230115,#230116),
(#230117,#230118),(#230119,#230120),(#230121,#230122),(#230123,#230124),
(#230125,#230126),(#230127,#230128),(#230129,#230130),(#230131,#230132),
(#230133,#230134),(#230135,#230136),(#230137,#230138),(#230139,#230140),
(#230141,#230142),(#230143,#230144),(#230145,#230146),(#230147,#230148),
(#230149,#230150),(#230151,#230152),(#230153,#230154),(#230155,#230156),
(#230157,#230158),(#230159,#230160),(#230161,#230162),(#230163,#230164),
(#230165,#230166),(#230167,#230168),(#230169,#230170),(#230171,#230172),
(#230173,#230174),(#230175,#230176),(#230177,#230178),(#230179,#230180),
(#230181,#230182),(#230183,#230184),(#230185,#230186),(#230187,#230188),
(#230189,#230190),(#230191,#230192),(#230193,#230194),(#230195,#230196),
(#230197,#230198),(#230199,#230200),(#230201,#230202),(#230203,#230204),
(#230205,#230206),(#230207,#230208),(#230209,#230210),(#230211,#230212),
(#230213,#230214),(#230215,#230216),(#230217,#230218),(#230219,#230220),
(#230221,#230222),(#230223,#230224),(#230225,#230226),(#230227,#230228),
(#230229,#230230),(#230231,#230232),(#230233,#230234),(#230235,#230236),
(#230237,#230238),(#230239,#230240),(#230241,#230242),(#230243,#230244),
(#230245,#230246),(#230247,#230248),(#230249,#230250),(#230251,#230252),
(#230253,#230254),(#230255,#230256),(#230257,#230258),(#230259,#230260),
(#230261,#230262),(#230263,#230264),(#230265,#230266),(#230267,#230268),
(#230269,#230270),(#230271,#230272),(#230273,#230274),(#230275,#230276),
(#230277,#230278),(#230279,#230280),(#230281,#230282),(#230283,#230284),
(#230285,#230286),(#230287,#230288),(#230289,#230290),(#230291,#230292),
(#230293,#230294),(#230295,#230296),(#230297,#230298),(#230299,#230300),
(#230301,#230302),(#230303,#230304),(#230305,#230306),(#230307,#230308),
(#230309,#230310),(#230311,#230312),(#230313,#230314),(#230315,#230316),
(#230317,#230318),(#230319,#230320),(#230321,#230322),(#230323,#230324),
(#230325,#230326),(#230327,#230328),(#230329,#230330),(#230331,#230332),
(#230333,#230334),(#230335,#230336),(#230337,#230338),(#230339,#230340),
(#230341,#230342),(#230343,#230344),(#230345,#230346),(#230347,#230348),
(#230349,#230350),(#230351,#230352),(#230353,#230354),(#230355,#230356),
(#230357,#230358),(#230359,#230360),(#230361,#230362),(#230363,#230364),
(#230365,#230366),(#230367,#230368),(#230369,#230370),(#230371,#230372),
(#230373,#230374),(#230375,#230376),(#230377,#230378),(#230379,#230380),
(#230381,#230382),(#230383,#230384),(#230385,#230386),(#230387,#230388),
(#230389,#230390),(#230391,#230392),(#230393,#230394),(#230395,#230396),
(#230397,#230398),(#230399,#230400),(#230401,#230402),(#230403,#230404),
(#230405,#230406),(#230407,#230408),(#230409,#230410),(#230411,#230412),
(#230413,#230414),(#230415,#230416),(#230417,#230418),(#230419,#230420),
(#230421,#230422),(#230423,#230424),(#230425,#230426),(#230427,#230428),
(#230429,#230430),(#230431,#230432),(#230433,#230434),(#230435,#230436),
(#230437,#230438),(#230439,#230440),(#230441,#230442),(#230443,#230444),
(#230445,#230446),(#230447,#230448),(#230449,#230450),(#230451,#230452),
(#230453,#230454),(#230455,#230456)),.UNSPECIFIED.,.F.,.F.,.F.)
B_SPLINE_SURFACE_WITH_KNOTS((6,1,1,1,1,1,1,1,1,1,1,1,1,1,1,1,1,1,1,1,1,
1,1,1,1,1,1,1,1,1,1,1,1,1,1,1,1,1,1,1,1,1,1,1,1,1,1,1,1,1,1,1,1,1,1,1,1,
1,1,1,1,1,1,1,1,1,1,1,1,1,1,1,1,1,1,1,1,1,1,1,1,1,1,1,1,1,1,1,1,1,1,1,1,
1,1,1,1,1,1,1,1,1,1,1,1,1,1,1,1,1,1,1,1,1,1,1,1,1,1,1,1,1,1,1,1,1,1,1,1,
1,1,1,1,1,1,1,1,1,1,1,1,1,1,1,1,1,1,1,1,1,1,1,1,1,1,1,1,1,1,1,1,1,1,1,1,
1,1,1,1,1,1,1,1,1,1,1,1,1,1,1,1,1,1,1,1,1,1,1,1,1,1,1,1,1,1,1,1,1,1,1,6),
(2,2),(0.,0.005,0.01,0.015,0.02,0.025,0.03,0.035,0.04,0.045,0.05,0.055,
0.06,0.065,0.07,0.075,0.08,0.085,0.09,0.095,0.1,0.105,0.11,0.115,0.12,0.125,
0.13,0.135,0.14,0.145,0.15,0.155,0.16,0.165,0.17,0.175,0.18,0.185,0.19,
0.195,0.2,0.205,0.21,0.215,0.22,0.225,0.23,0.235,0.24,0.245,0.25,0.255,
0.26,0.265,0.27,0.275,0.28,0.285,0.29,0.295,0.3,0.305,0.31,0.315,0.32,0.325,
0.33,0.335,0.34,0.345,0.35,0.355,0.36,0.365,0.37,0.375,0.38,0.385,0.39,
0.395,0.4,0.405,0.41,0.415,0.42,0.425,0.43,0.435,0.44,0.445,0.45,0.455,
0.46,0.465,0.47,0.475,0.48,0.485,0.49,0.495,0.5,0.505,0.51,0.515,0.52,0.525,
0.53,0.535,0.54,0.545,0.55,0.555,0.56,0.565,0.57,0.575,0.58,0.585,0.59,
0.595,0.6,0.605,0.61,0.615,0.62,0.625,0.63,0.635,0.64,0.645,0.65,0.655,
0.66,0.665,0.67,0.675,0.68,0.685,0.690000000000001,0.695000000000001,0.700000000000001,
0.705000000000001,0.710000000000001,0.715000000000001,0.720000000000001,
0.725000000000001,0.730000000000001,0.735000000000001,0.740000000000001,
0.745000000000001,0.750000000000001,0.755000000000001,0.760000000000001,
0.765000000000001,0.770000000000001,0.775000000000001,0.780000000000001,
0.785000000000001,0.790000000000001,0.795000000000001,0.800000000000001,
0.805000000000001,0.810000000000001,0.815000000000001,0.820000000000001,
0.825000000000001,0.830000000000001,0.835000000000001,0.840000000000001,
0.845000000000001,0.850000000000001,0.855000000000001,0.860000000000001,
0.865000000000001,0.870000000000001,0.875000000000001,0.880000000000001,
0.885000000000001,0.890000000000001,0.895000000000001,0.900000000000001,
0.905000000000001,0.910000000000001,0.915000000000001,0.920000000000001,
0.925000000000001,0.930000000000001,0.935000000000001,0.940000000000001,
0.945000000000001,0.950000000000001,0.955000000000001,0.960000000000001,
0.965000000000001,0.970000000000001,0.975000000000001,0.980000000000001,
0.985000000000001,0.990000000000001,0.995000000000001,1.),(0.,1.2),
 .UNSPECIFIED.)
GEOMETRIC_REPRESENTATION_ITEM()
RATIONAL_B_SPLINE_SURFACE(((1.,1.),(1.,1.),(1.,1.),(1.,1.),(1.,1.),(1.,
1.),(1.,1.),(1.,1.),(1.,1.),(1.,1.),(1.,1.),(1.,1.),(1.,1.),(1.,1.),(1.,
1.),(1.,1.),(1.,1.),(1.,1.),(1.,1.),(1.,1.),(1.,1.),(1.,1.),(1.,1.),(1.,
1.),(1.,1.),(1.,1.),(1.,1.),(1.,1.),(1.,1.),(1.,1.),(1.,1.),(1.,1.),(1.,
1.),(1.,1.),(1.,1.),(1.,1.),(1.,1.),(1.,1.),(1.,1.),(1.,1.),(1.,1.),(1.,
1.),(1.,1.),(1.,1.),(1.,1.),(1.,1.),(1.,1.),(1.,1.),(1.,1.),(1.,1.),(1.,
1.),(1.,1.),(1.,1.),(1.,1.),(1.,1.),(1.,1.),(1.,1.),(1.,1.),(1.,1.),(1.,
1.),(1.,1.),(1.,1.),(1.,1.),(1.,1.),(1.,1.),(1.,1.),(1.,1.),(1.,1.),(1.,
1.),(1.,1.),(1.,1.),(1.,1.),(1.,1.),(1.,1.),(1.,1.),(1.,1.),(1.,1.),(1.,
1.),(1.,1.),(1.,1.),(1.,1.),(1.,1.),(1.,1.),(1.,1.),(1.,1.),(1.,1.),(1.,
1.),(1.,1.),(1.,1.),(1.,1.),(1.,1.),(1.,1.),(1.,1.),(1.,1.),(1.,1.),(1.,
1.),(1.,1.),(1.,1.),(1.,1.),(1.,1.),(1.,1.),(1.,1.),(1.,1.),(1.,1.),(1.,
1.),(1.,1.),(1.,1.),(1.,1.),(1.,1.),(1.,1.),(1.,1.),(1.,1.),(1.,1.),(1.,
1.),(1.,1.),(1.,1.),(1.,1.),(1.,1.),(1.,1.),(1.,1.),(1.,1.),(1.,1.),(1.,
1.),(1.,1.),(1.,1.),(1.,1.),(1.,1.),(1.,1.),(1.,1.),(1.,1.),(1.,1.),(1.,
1.),(1.,1.),(1.,1.),(1.,1.),(1.,1.),(1.,1.),(1.,1.),(1.,1.),(1.,1.),(1.,
1.),(1.,1.),(1.,1.),(1.,1.),(1.,1.),(1.,1.),(1.,1.),(1.,1.),(1.,1.),(1.,
1.),(1.,1.),(1.,1.),(1.,1.),(1.,1.),(1.,1.),(1.,1.),(1.,1.),(1.,1.),(1.,
1.),(1.,1.),(1.,1.),(1.,1.),(1.,1.),(1.,1.),(1.,1.),(1.,1.),(1.,1.),(1.,
1.),(1.,1.),(1.,1.),(1.,1.),(1.,1.),(1.,1.),(1.,1.),(1.,1.),(1.,1.),(1.,
1.),(1.,1.),(1.,1.),(1.,1.),(1.,1.),(1.,1.),(1.,1.),(1.,1.),(1.,1.),(1.,
1.),(1.,1.),(1.,1.),(1.,1.),(1.,1.),(1.,1.),(1.,1.),(1.,1.),(1.,1.),(1.,
1.),(1.,1.),(1.,1.),(1.,1.),(1.,1.),(1.,1.),(1.,1.),(1.,1.),(1.,1.),(1.,
1.),(1.,1.)))
REPRESENTATION_ITEM('')
SURFACE()
);
#1093=(
BOUNDED_SURFACE()
B_SPLINE_SURFACE(5,1,((#230876,#230877),(#230878,#230879),(#230880,#230881),
(#230882,#230883),(#230884,#230885),(#230886,#230887),(#230888,#230889),
(#230890,#230891),(#230892,#230893),(#230894,#230895),(#230896,#230897),
(#230898,#230899),(#230900,#230901),(#230902,#230903),(#230904,#230905),
(#230906,#230907),(#230908,#230909),(#230910,#230911),(#230912,#230913),
(#230914,#230915),(#230916,#230917),(#230918,#230919),(#230920,#230921),
(#230922,#230923),(#230924,#230925),(#230926,#230927),(#230928,#230929),
(#230930,#230931),(#230932,#230933),(#230934,#230935),(#230936,#230937),
(#230938,#230939),(#230940,#230941),(#230942,#230943),(#230944,#230945),
(#230946,#230947),(#230948,#230949),(#230950,#230951),(#230952,#230953),
(#230954,#230955),(#230956,#230957),(#230958,#230959),(#230960,#230961),
(#230962,#230963),(#230964,#230965),(#230966,#230967),(#230968,#230969),
(#230970,#230971),(#230972,#230973),(#230974,#230975),(#230976,#230977),
(#230978,#230979),(#230980,#230981),(#230982,#230983),(#230984,#230985),
(#230986,#230987),(#230988,#230989),(#230990,#230991),(#230992,#230993),
(#230994,#230995),(#230996,#230997),(#230998,#230999),(#231000,#231001),
(#231002,#231003),(#231004,#231005),(#231006,#231007),(#231008,#231009),
(#231010,#231011),(#231012,#231013),(#231014,#231015),(#231016,#231017),
(#231018,#231019),(#231020,#231021),(#231022,#231023),(#231024,#231025),
(#231026,#231027),(#231028,#231029),(#231030,#231031),(#231032,#231033),
(#231034,#231035),(#231036,#231037),(#231038,#231039),(#231040,#231041),
(#231042,#231043),(#231044,#231045),(#231046,#231047),(#231048,#231049),
(#231050,#231051),(#231052,#231053),(#231054,#231055),(#231056,#231057),
(#231058,#231059),(#231060,#231061),(#231062,#231063),(#231064,#231065),
(#231066,#231067),(#231068,#231069),(#231070,#231071),(#231072,#231073),
(#231074,#231075),(#231076,#231077),(#231078,#231079),(#231080,#231081),
(#231082,#231083),(#231084,#231085),(#231086,#231087),(#231088,#231089),
(#231090,#231091),(#231092,#231093),(#231094,#231095),(#231096,#231097),
(#231098,#231099),(#231100,#231101),(#231102,#231103),(#231104,#231105),
(#231106,#231107),(#231108,#231109),(#231110,#231111),(#231112,#231113),
(#231114,#231115),(#231116,#231117),(#231118,#231119),(#231120,#231121),
(#231122,#231123),(#231124,#231125),(#231126,#231127),(#231128,#231129),
(#231130,#231131),(#231132,#231133),(#231134,#231135),(#231136,#231137),
(#231138,#231139),(#231140,#231141),(#231142,#231143),(#231144,#231145),
(#231146,#231147),(#231148,#231149),(#231150,#231151),(#231152,#231153),
(#231154,#231155),(#231156,#231157),(#231158,#231159),(#231160,#231161),
(#231162,#231163),(#231164,#231165),(#231166,#231167),(#231168,#231169),
(#231170,#231171),(#231172,#231173),(#231174,#231175),(#231176,#231177),
(#231178,#231179),(#231180,#231181),(#231182,#231183),(#231184,#231185),
(#231186,#231187),(#231188,#231189),(#231190,#231191),(#231192,#231193),
(#231194,#231195),(#231196,#231197),(#231198,#231199),(#231200,#231201),
(#231202,#231203),(#231204,#231205),(#231206,#231207),(#231208,#231209),
(#231210,#231211),(#231212,#231213),(#231214,#231215),(#231216,#231217),
(#231218,#231219),(#231220,#231221),(#231222,#231223),(#231224,#231225),
(#231226,#231227),(#231228,#231229),(#231230,#231231),(#231232,#231233),
(#231234,#231235),(#231236,#231237),(#231238,#231239),(#231240,#231241),
(#231242,#231243),(#231244,#231245),(#231246,#231247),(#231248,#231249),
(#231250,#231251),(#231252,#231253),(#231254,#231255),(#231256,#231257),
(#231258,#231259),(#231260,#231261),(#231262,#231263),(#231264,#231265),
(#231266,#231267),(#231268,#231269),(#231270,#231271),(#231272,#231273),
(#231274,#231275),(#231276,#231277),(#231278,#231279),(#231280,#231281),
(#231282,#231283),(#231284,#231285)),.UNSPECIFIED.,.F.,.F.,.F.)
B_SPLINE_SURFACE_WITH_KNOTS((6,1,1,1,1,1,1,1,1,1,1,1,1,1,1,1,1,1,1,1,1,
1,1,1,1,1,1,1,1,1,1,1,1,1,1,1,1,1,1,1,1,1,1,1,1,1,1,1,1,1,1,1,1,1,1,1,1,
1,1,1,1,1,1,1,1,1,1,1,1,1,1,1,1,1,1,1,1,1,1,1,1,1,1,1,1,1,1,1,1,1,1,1,1,
1,1,1,1,1,1,1,1,1,1,1,1,1,1,1,1,1,1,1,1,1,1,1,1,1,1,1,1,1,1,1,1,1,1,1,1,
1,1,1,1,1,1,1,1,1,1,1,1,1,1,1,1,1,1,1,1,1,1,1,1,1,1,1,1,1,1,1,1,1,1,1,1,
1,1,1,1,1,1,1,1,1,1,1,1,1,1,1,1,1,1,1,1,1,1,1,1,1,1,1,1,1,1,1,1,1,1,1,6),
(2,2),(-1.,-0.995000000000001,-0.990000000000001,-0.985000000000001,-0.980000000000001,
-0.975000000000001,-0.970000000000001,-0.965000000000001,-0.960000000000001,
-0.955000000000001,-0.950000000000001,-0.945000000000001,-0.940000000000001,
-0.935000000000001,-0.930000000000001,-0.925000000000001,-0.920000000000001,
-0.915000000000001,-0.910000000000001,-0.905000000000001,-0.900000000000001,
-0.895000000000001,-0.890000000000001,-0.885000000000001,-0.880000000000001,
-0.875000000000001,-0.870000000000001,-0.865000000000001,-0.860000000000001,
-0.855000000000001,-0.850000000000001,-0.845000000000001,-0.840000000000001,
-0.835000000000001,-0.830000000000001,-0.825000000000001,-0.820000000000001,
-0.815000000000001,-0.810000000000001,-0.805000000000001,-0.800000000000001,
-0.795000000000001,-0.790000000000001,-0.785000000000001,-0.780000000000001,
-0.775000000000001,-0.770000000000001,-0.765000000000001,-0.760000000000001,
-0.755000000000001,-0.750000000000001,-0.745000000000001,-0.740000000000001,
-0.735000000000001,-0.730000000000001,-0.725000000000001,-0.720000000000001,
-0.715000000000001,-0.710000000000001,-0.705000000000001,-0.700000000000001,
-0.695000000000001,-0.690000000000001,-0.685,-0.68,-0.675,-0.67,-0.665,
-0.66,-0.655,-0.65,-0.645,-0.64,-0.635,-0.63,-0.625,-0.62,-0.615,-0.61,
-0.605,-0.6,-0.595,-0.59,-0.585,-0.58,-0.575,-0.57,-0.565,-0.56,-0.555,
-0.55,-0.545,-0.54,-0.535,-0.53,-0.525,-0.52,-0.515,-0.51,-0.505,-0.5,-0.495,
-0.49,-0.485,-0.48,-0.475,-0.47,-0.465,-0.46,-0.455,-0.45,-0.445,-0.44,
-0.435,-0.43,-0.425,-0.42,-0.415,-0.41,-0.405,-0.4,-0.395,-0.39,-0.385,
-0.38,-0.375,-0.37,-0.365,-0.36,-0.355,-0.35,-0.345,-0.34,-0.335,-0.33,
-0.325,-0.32,-0.315,-0.31,-0.305,-0.3,-0.295,-0.29,-0.285,-0.28,-0.275,
-0.27,-0.265,-0.26,-0.255,-0.25,-0.245,-0.24,-0.235,-0.23,-0.225,-0.22,
-0.215,-0.21,-0.205,-0.2,-0.195,-0.19,-0.185,-0.18,-0.175,-0.17,-0.165,
-0.16,-0.155,-0.15,-0.145,-0.14,-0.135,-0.13,-0.125,-0.12,-0.115,-0.11,
-0.105,-0.1,-0.095,-0.09,-0.085,-0.08,-0.075,-0.07,-0.065,-0.06,-0.055,
-0.05,-0.045,-0.04,-0.035,-0.03,-0.025,-0.02,-0.015,-0.01,-0.005,0.),(0.,
1.2),.UNSPECIFIED.)
GEOMETRIC_REPRESENTATION_ITEM()
RATIONAL_B_SPLINE_SURFACE(((1.,1.),(1.,1.),(1.,1.),(1.,1.),(1.,1.),(1.,
1.),(1.,1.),(1.,1.),(1.,1.),(1.,1.),(1.,1.),(1.,1.),(1.,1.),(1.,1.),(1.,
1.),(1.,1.),(1.,1.),(1.,1.),(1.,1.),(1.,1.),(1.,1.),(1.,1.),(1.,1.),(1.,
1.),(1.,1.),(1.,1.),(1.,1.),(1.,1.),(1.,1.),(1.,1.),(1.,1.),(1.,1.),(1.,
1.),(1.,1.),(1.,1.),(1.,1.),(1.,1.),(1.,1.),(1.,1.),(1.,1.),(1.,1.),(1.,
1.),(1.,1.),(1.,1.),(1.,1.),(1.,1.),(1.,1.),(1.,1.),(1.,1.),(1.,1.),(1.,
1.),(1.,1.),(1.,1.),(1.,1.),(1.,1.),(1.,1.),(1.,1.),(1.,1.),(1.,1.),(1.,
1.),(1.,1.),(1.,1.),(1.,1.),(1.,1.),(1.,1.),(1.,1.),(1.,1.),(1.,1.),(1.,
1.),(1.,1.),(1.,1.),(1.,1.),(1.,1.),(1.,1.),(1.,1.),(1.,1.),(1.,1.),(1.,
1.),(1.,1.),(1.,1.),(1.,1.),(1.,1.),(1.,1.),(1.,1.),(1.,1.),(1.,1.),(1.,
1.),(1.,1.),(1.,1.),(1.,1.),(1.,1.),(1.,1.),(1.,1.),(1.,1.),(1.,1.),(1.,
1.),(1.,1.),(1.,1.),(1.,1.),(1.,1.),(1.,1.),(1.,1.),(1.,1.),(1.,1.),(1.,
1.),(1.,1.),(1.,1.),(1.,1.),(1.,1.),(1.,1.),(1.,1.),(1.,1.),(1.,1.),(1.,
1.),(1.,1.),(1.,1.),(1.,1.),(1.,1.),(1.,1.),(1.,1.),(1.,1.),(1.,1.),(1.,
1.),(1.,1.),(1.,1.),(1.,1.),(1.,1.),(1.,1.),(1.,1.),(1.,1.),(1.,1.),(1.,
1.),(1.,1.),(1.,1.),(1.,1.),(1.,1.),(1.,1.),(1.,1.),(1.,1.),(1.,1.),(1.,
1.),(1.,1.),(1.,1.),(1.,1.),(1.,1.),(1.,1.),(1.,1.),(1.,1.),(1.,1.),(1.,
1.),(1.,1.),(1.,1.),(1.,1.),(1.,1.),(1.,1.),(1.,1.),(1.,1.),(1.,1.),(1.,
1.),(1.,1.),(1.,1.),(1.,1.),(1.,1.),(1.,1.),(1.,1.),(1.,1.),(1.,1.),(1.,
1.),(1.,1.),(1.,1.),(1.,1.),(1.,1.),(1.,1.),(1.,1.),(1.,1.),(1.,1.),(1.,
1.),(1.,1.),(1.,1.),(1.,1.),(1.,1.),(1.,1.),(1.,1.),(1.,1.),(1.,1.),(1.,
1.),(1.,1.),(1.,1.),(1.,1.),(1.,1.),(1.,1.),(1.,1.),(1.,1.),(1.,1.),(1.,
1.),(1.,1.),(1.,1.),(1.,1.),(1.,1.),(1.,1.),(1.,1.),(1.,1.),(1.,1.),(1.,
1.),(1.,1.)))
REPRESENTATION_ITEM('')
SURFACE()
);
#1094=(
BOUNDED_SURFACE()
B_SPLINE_SURFACE(5,1,((#231699,#231700),(#231701,#231702),(#231703,#231704),
(#231705,#231706),(#231707,#231708),(#231709,#231710),(#231711,#231712),
(#231713,#231714),(#231715,#231716),(#231717,#231718),(#231719,#231720),
(#231721,#231722),(#231723,#231724),(#231725,#231726),(#231727,#231728),
(#231729,#231730),(#231731,#231732),(#231733,#231734),(#231735,#231736),
(#231737,#231738),(#231739,#231740),(#231741,#231742),(#231743,#231744),
(#231745,#231746),(#231747,#231748),(#231749,#231750),(#231751,#231752),
(#231753,#231754),(#231755,#231756),(#231757,#231758),(#231759,#231760),
(#231761,#231762),(#231763,#231764),(#231765,#231766),(#231767,#231768),
(#231769,#231770),(#231771,#231772),(#231773,#231774),(#231775,#231776),
(#231777,#231778),(#231779,#231780),(#231781,#231782),(#231783,#231784),
(#231785,#231786),(#231787,#231788),(#231789,#231790),(#231791,#231792),
(#231793,#231794),(#231795,#231796),(#231797,#231798),(#231799,#231800),
(#231801,#231802),(#231803,#231804),(#231805,#231806),(#231807,#231808),
(#231809,#231810),(#231811,#231812),(#231813,#231814),(#231815,#231816),
(#231817,#231818),(#231819,#231820),(#231821,#231822),(#231823,#231824),
(#231825,#231826),(#231827,#231828),(#231829,#231830),(#231831,#231832),
(#231833,#231834),(#231835,#231836),(#231837,#231838),(#231839,#231840),
(#231841,#231842),(#231843,#231844),(#231845,#231846),(#231847,#231848),
(#231849,#231850),(#231851,#231852),(#231853,#231854),(#231855,#231856),
(#231857,#231858),(#231859,#231860),(#231861,#231862),(#231863,#231864),
(#231865,#231866),(#231867,#231868),(#231869,#231870),(#231871,#231872),
(#231873,#231874),(#231875,#231876),(#231877,#231878),(#231879,#231880),
(#231881,#231882),(#231883,#231884),(#231885,#231886),(#231887,#231888),
(#231889,#231890),(#231891,#231892),(#231893,#231894),(#231895,#231896),
(#231897,#231898),(#231899,#231900),(#231901,#231902),(#231903,#231904),
(#231905,#231906),(#231907,#231908),(#231909,#231910),(#231911,#231912),
(#231913,#231914),(#231915,#231916),(#231917,#231918),(#231919,#231920),
(#231921,#231922),(#231923,#231924),(#231925,#231926),(#231927,#231928),
(#231929,#231930),(#231931,#231932),(#231933,#231934),(#231935,#231936),
(#231937,#231938),(#231939,#231940),(#231941,#231942),(#231943,#231944),
(#231945,#231946),(#231947,#231948),(#231949,#231950),(#231951,#231952),
(#231953,#231954),(#231955,#231956),(#231957,#231958),(#231959,#231960),
(#231961,#231962),(#231963,#231964),(#231965,#231966),(#231967,#231968),
(#231969,#231970),(#231971,#231972),(#231973,#231974),(#231975,#231976),
(#231977,#231978),(#231979,#231980),(#231981,#231982),(#231983,#231984),
(#231985,#231986),(#231987,#231988),(#231989,#231990),(#231991,#231992),
(#231993,#231994),(#231995,#231996),(#231997,#231998),(#231999,#232000),
(#232001,#232002),(#232003,#232004),(#232005,#232006),(#232007,#232008),
(#232009,#232010),(#232011,#232012),(#232013,#232014),(#232015,#232016),
(#232017,#232018),(#232019,#232020),(#232021,#232022),(#232023,#232024),
(#232025,#232026),(#232027,#232028),(#232029,#232030),(#232031,#232032),
(#232033,#232034),(#232035,#232036),(#232037,#232038),(#232039,#232040),
(#232041,#232042),(#232043,#232044),(#232045,#232046),(#232047,#232048),
(#232049,#232050),(#232051,#232052),(#232053,#232054),(#232055,#232056),
(#232057,#232058),(#232059,#232060),(#232061,#232062),(#232063,#232064),
(#232065,#232066),(#232067,#232068),(#232069,#232070),(#232071,#232072),
(#232073,#232074),(#232075,#232076),(#232077,#232078),(#232079,#232080),
(#232081,#232082),(#232083,#232084),(#232085,#232086),(#232087,#232088),
(#232089,#232090),(#232091,#232092),(#232093,#232094),(#232095,#232096),
(#232097,#232098),(#232099,#232100),(#232101,#232102),(#232103,#232104),
(#232105,#232106),(#232107,#232108)),.UNSPECIFIED.,.F.,.F.,.F.)
B_SPLINE_SURFACE_WITH_KNOTS((6,1,1,1,1,1,1,1,1,1,1,1,1,1,1,1,1,1,1,1,1,
1,1,1,1,1,1,1,1,1,1,1,1,1,1,1,1,1,1,1,1,1,1,1,1,1,1,1,1,1,1,1,1,1,1,1,1,
1,1,1,1,1,1,1,1,1,1,1,1,1,1,1,1,1,1,1,1,1,1,1,1,1,1,1,1,1,1,1,1,1,1,1,1,
1,1,1,1,1,1,1,1,1,1,1,1,1,1,1,1,1,1,1,1,1,1,1,1,1,1,1,1,1,1,1,1,1,1,1,1,
1,1,1,1,1,1,1,1,1,1,1,1,1,1,1,1,1,1,1,1,1,1,1,1,1,1,1,1,1,1,1,1,1,1,1,1,
1,1,1,1,1,1,1,1,1,1,1,1,1,1,1,1,1,1,1,1,1,1,1,1,1,1,1,1,1,1,1,1,1,1,1,6),
(2,2),(0.,0.005,0.01,0.015,0.02,0.025,0.03,0.035,0.04,0.045,0.05,0.055,
0.06,0.065,0.07,0.075,0.08,0.085,0.09,0.095,0.1,0.105,0.11,0.115,0.12,0.125,
0.13,0.135,0.14,0.145,0.15,0.155,0.16,0.165,0.17,0.175,0.18,0.185,0.19,
0.195,0.2,0.205,0.21,0.215,0.22,0.225,0.23,0.235,0.24,0.245,0.25,0.255,
0.26,0.265,0.27,0.275,0.28,0.285,0.29,0.295,0.3,0.305,0.31,0.315,0.32,0.325,
0.33,0.335,0.34,0.345,0.35,0.355,0.36,0.365,0.37,0.375,0.38,0.385,0.39,
0.395,0.4,0.405,0.41,0.415,0.42,0.425,0.43,0.435,0.44,0.445,0.45,0.455,
0.46,0.465,0.47,0.475,0.48,0.485,0.49,0.495,0.5,0.505,0.51,0.515,0.52,0.525,
0.53,0.535,0.54,0.545,0.55,0.555,0.56,0.565,0.57,0.575,0.58,0.585,0.59,
0.595,0.6,0.605,0.61,0.615,0.62,0.625,0.63,0.635,0.64,0.645,0.65,0.655,
0.66,0.665,0.67,0.675,0.68,0.685,0.690000000000001,0.695000000000001,0.700000000000001,
0.705000000000001,0.710000000000001,0.715000000000001,0.720000000000001,
0.725000000000001,0.730000000000001,0.735000000000001,0.740000000000001,
0.745000000000001,0.750000000000001,0.755000000000001,0.760000000000001,
0.765000000000001,0.770000000000001,0.775000000000001,0.780000000000001,
0.785000000000001,0.790000000000001,0.795000000000001,0.800000000000001,
0.805000000000001,0.810000000000001,0.815000000000001,0.820000000000001,
0.825000000000001,0.830000000000001,0.835000000000001,0.840000000000001,
0.845000000000001,0.850000000000001,0.855000000000001,0.860000000000001,
0.865000000000001,0.870000000000001,0.875000000000001,0.880000000000001,
0.885000000000001,0.890000000000001,0.895000000000001,0.900000000000001,
0.905000000000001,0.910000000000001,0.915000000000001,0.920000000000001,
0.925000000000001,0.930000000000001,0.935000000000001,0.940000000000001,
0.945000000000001,0.950000000000001,0.955000000000001,0.960000000000001,
0.965000000000001,0.970000000000001,0.975000000000001,0.980000000000001,
0.985000000000001,0.990000000000001,0.995000000000001,1.),(0.,1.2),
 .UNSPECIFIED.)
GEOMETRIC_REPRESENTATION_ITEM()
RATIONAL_B_SPLINE_SURFACE(((1.,1.),(1.,1.),(1.,1.),(1.,1.),(1.,1.),(1.,
1.),(1.,1.),(1.,1.),(1.,1.),(1.,1.),(1.,1.),(1.,1.),(1.,1.),(1.,1.),(1.,
1.),(1.,1.),(1.,1.),(1.,1.),(1.,1.),(1.,1.),(1.,1.),(1.,1.),(1.,1.),(1.,
1.),(1.,1.),(1.,1.),(1.,1.),(1.,1.),(1.,1.),(1.,1.),(1.,1.),(1.,1.),(1.,
1.),(1.,1.),(1.,1.),(1.,1.),(1.,1.),(1.,1.),(1.,1.),(1.,1.),(1.,1.),(1.,
1.),(1.,1.),(1.,1.),(1.,1.),(1.,1.),(1.,1.),(1.,1.),(1.,1.),(1.,1.),(1.,
1.),(1.,1.),(1.,1.),(1.,1.),(1.,1.),(1.,1.),(1.,1.),(1.,1.),(1.,1.),(1.,
1.),(1.,1.),(1.,1.),(1.,1.),(1.,1.),(1.,1.),(1.,1.),(1.,1.),(1.,1.),(1.,
1.),(1.,1.),(1.,1.),(1.,1.),(1.,1.),(1.,1.),(1.,1.),(1.,1.),(1.,1.),(1.,
1.),(1.,1.),(1.,1.),(1.,1.),(1.,1.),(1.,1.),(1.,1.),(1.,1.),(1.,1.),(1.,
1.),(1.,1.),(1.,1.),(1.,1.),(1.,1.),(1.,1.),(1.,1.),(1.,1.),(1.,1.),(1.,
1.),(1.,1.),(1.,1.),(1.,1.),(1.,1.),(1.,1.),(1.,1.),(1.,1.),(1.,1.),(1.,
1.),(1.,1.),(1.,1.),(1.,1.),(1.,1.),(1.,1.),(1.,1.),(1.,1.),(1.,1.),(1.,
1.),(1.,1.),(1.,1.),(1.,1.),(1.,1.),(1.,1.),(1.,1.),(1.,1.),(1.,1.),(1.,
1.),(1.,1.),(1.,1.),(1.,1.),(1.,1.),(1.,1.),(1.,1.),(1.,1.),(1.,1.),(1.,
1.),(1.,1.),(1.,1.),(1.,1.),(1.,1.),(1.,1.),(1.,1.),(1.,1.),(1.,1.),(1.,
1.),(1.,1.),(1.,1.),(1.,1.),(1.,1.),(1.,1.),(1.,1.),(1.,1.),(1.,1.),(1.,
1.),(1.,1.),(1.,1.),(1.,1.),(1.,1.),(1.,1.),(1.,1.),(1.,1.),(1.,1.),(1.,
1.),(1.,1.),(1.,1.),(1.,1.),(1.,1.),(1.,1.),(1.,1.),(1.,1.),(1.,1.),(1.,
1.),(1.,1.),(1.,1.),(1.,1.),(1.,1.),(1.,1.),(1.,1.),(1.,1.),(1.,1.),(1.,
1.),(1.,1.),(1.,1.),(1.,1.),(1.,1.),(1.,1.),(1.,1.),(1.,1.),(1.,1.),(1.,
1.),(1.,1.),(1.,1.),(1.,1.),(1.,1.),(1.,1.),(1.,1.),(1.,1.),(1.,1.),(1.,
1.),(1.,1.),(1.,1.),(1.,1.),(1.,1.),(1.,1.),(1.,1.),(1.,1.),(1.,1.),(1.,
1.),(1.,1.)))
REPRESENTATION_ITEM('')
SURFACE()
);
#1095=(
BOUNDED_SURFACE()
B_SPLINE_SURFACE(5,1,((#232528,#232529),(#232530,#232531),(#232532,#232533),
(#232534,#232535),(#232536,#232537),(#232538,#232539),(#232540,#232541),
(#232542,#232543),(#232544,#232545),(#232546,#232547),(#232548,#232549),
(#232550,#232551),(#232552,#232553),(#232554,#232555),(#232556,#232557),
(#232558,#232559),(#232560,#232561),(#232562,#232563),(#232564,#232565),
(#232566,#232567),(#232568,#232569),(#232570,#232571),(#232572,#232573),
(#232574,#232575),(#232576,#232577),(#232578,#232579),(#232580,#232581),
(#232582,#232583),(#232584,#232585),(#232586,#232587),(#232588,#232589),
(#232590,#232591),(#232592,#232593),(#232594,#232595),(#232596,#232597),
(#232598,#232599),(#232600,#232601),(#232602,#232603),(#232604,#232605),
(#232606,#232607),(#232608,#232609),(#232610,#232611),(#232612,#232613),
(#232614,#232615),(#232616,#232617),(#232618,#232619),(#232620,#232621),
(#232622,#232623),(#232624,#232625),(#232626,#232627),(#232628,#232629),
(#232630,#232631),(#232632,#232633),(#232634,#232635),(#232636,#232637),
(#232638,#232639),(#232640,#232641),(#232642,#232643),(#232644,#232645),
(#232646,#232647),(#232648,#232649),(#232650,#232651),(#232652,#232653),
(#232654,#232655),(#232656,#232657),(#232658,#232659),(#232660,#232661),
(#232662,#232663),(#232664,#232665),(#232666,#232667),(#232668,#232669),
(#232670,#232671),(#232672,#232673),(#232674,#232675),(#232676,#232677),
(#232678,#232679),(#232680,#232681),(#232682,#232683),(#232684,#232685),
(#232686,#232687),(#232688,#232689),(#232690,#232691),(#232692,#232693),
(#232694,#232695),(#232696,#232697),(#232698,#232699),(#232700,#232701),
(#232702,#232703),(#232704,#232705),(#232706,#232707),(#232708,#232709),
(#232710,#232711),(#232712,#232713),(#232714,#232715),(#232716,#232717),
(#232718,#232719),(#232720,#232721),(#232722,#232723),(#232724,#232725),
(#232726,#232727),(#232728,#232729),(#232730,#232731),(#232732,#232733),
(#232734,#232735),(#232736,#232737),(#232738,#232739),(#232740,#232741),
(#232742,#232743),(#232744,#232745),(#232746,#232747),(#232748,#232749),
(#232750,#232751),(#232752,#232753),(#232754,#232755),(#232756,#232757),
(#232758,#232759),(#232760,#232761),(#232762,#232763),(#232764,#232765),
(#232766,#232767),(#232768,#232769),(#232770,#232771),(#232772,#232773),
(#232774,#232775),(#232776,#232777),(#232778,#232779),(#232780,#232781),
(#232782,#232783),(#232784,#232785),(#232786,#232787),(#232788,#232789),
(#232790,#232791),(#232792,#232793),(#232794,#232795),(#232796,#232797),
(#232798,#232799),(#232800,#232801),(#232802,#232803),(#232804,#232805),
(#232806,#232807),(#232808,#232809),(#232810,#232811),(#232812,#232813),
(#232814,#232815),(#232816,#232817),(#232818,#232819),(#232820,#232821),
(#232822,#232823),(#232824,#232825),(#232826,#232827),(#232828,#232829),
(#232830,#232831),(#232832,#232833),(#232834,#232835),(#232836,#232837),
(#232838,#232839),(#232840,#232841),(#232842,#232843),(#232844,#232845),
(#232846,#232847),(#232848,#232849),(#232850,#232851),(#232852,#232853),
(#232854,#232855),(#232856,#232857),(#232858,#232859),(#232860,#232861),
(#232862,#232863),(#232864,#232865),(#232866,#232867),(#232868,#232869),
(#232870,#232871),(#232872,#232873),(#232874,#232875),(#232876,#232877),
(#232878,#232879),(#232880,#232881),(#232882,#232883),(#232884,#232885),
(#232886,#232887),(#232888,#232889),(#232890,#232891),(#232892,#232893),
(#232894,#232895),(#232896,#232897),(#232898,#232899),(#232900,#232901),
(#232902,#232903),(#232904,#232905),(#232906,#232907),(#232908,#232909),
(#232910,#232911),(#232912,#232913),(#232914,#232915),(#232916,#232917),
(#232918,#232919),(#232920,#232921),(#232922,#232923),(#232924,#232925),
(#232926,#232927),(#232928,#232929),(#232930,#232931),(#232932,#232933),
(#232934,#232935),(#232936,#232937)),.UNSPECIFIED.,.F.,.F.,.F.)
B_SPLINE_SURFACE_WITH_KNOTS((6,1,1,1,1,1,1,1,1,1,1,1,1,1,1,1,1,1,1,1,1,
1,1,1,1,1,1,1,1,1,1,1,1,1,1,1,1,1,1,1,1,1,1,1,1,1,1,1,1,1,1,1,1,1,1,1,1,
1,1,1,1,1,1,1,1,1,1,1,1,1,1,1,1,1,1,1,1,1,1,1,1,1,1,1,1,1,1,1,1,1,1,1,1,
1,1,1,1,1,1,1,1,1,1,1,1,1,1,1,1,1,1,1,1,1,1,1,1,1,1,1,1,1,1,1,1,1,1,1,1,
1,1,1,1,1,1,1,1,1,1,1,1,1,1,1,1,1,1,1,1,1,1,1,1,1,1,1,1,1,1,1,1,1,1,1,1,
1,1,1,1,1,1,1,1,1,1,1,1,1,1,1,1,1,1,1,1,1,1,1,1,1,1,1,1,1,1,1,1,1,1,1,6),
(2,2),(-1.,-0.995000000000001,-0.990000000000001,-0.985000000000001,-0.980000000000001,
-0.975000000000001,-0.970000000000001,-0.965000000000001,-0.960000000000001,
-0.955000000000001,-0.950000000000001,-0.945000000000001,-0.940000000000001,
-0.935000000000001,-0.930000000000001,-0.925000000000001,-0.920000000000001,
-0.915000000000001,-0.910000000000001,-0.905000000000001,-0.900000000000001,
-0.895000000000001,-0.890000000000001,-0.885000000000001,-0.880000000000001,
-0.875000000000001,-0.870000000000001,-0.865000000000001,-0.860000000000001,
-0.855000000000001,-0.850000000000001,-0.845000000000001,-0.840000000000001,
-0.835000000000001,-0.830000000000001,-0.825000000000001,-0.820000000000001,
-0.815000000000001,-0.810000000000001,-0.805000000000001,-0.800000000000001,
-0.795000000000001,-0.790000000000001,-0.785000000000001,-0.780000000000001,
-0.775000000000001,-0.770000000000001,-0.765000000000001,-0.760000000000001,
-0.755000000000001,-0.750000000000001,-0.745000000000001,-0.740000000000001,
-0.735000000000001,-0.730000000000001,-0.725000000000001,-0.720000000000001,
-0.715000000000001,-0.710000000000001,-0.705000000000001,-0.700000000000001,
-0.695000000000001,-0.690000000000001,-0.685,-0.68,-0.675,-0.67,-0.665,
-0.66,-0.655,-0.65,-0.645,-0.64,-0.635,-0.63,-0.625,-0.62,-0.615,-0.61,
-0.605,-0.6,-0.595,-0.59,-0.585,-0.58,-0.575,-0.57,-0.565,-0.56,-0.555,
-0.55,-0.545,-0.54,-0.535,-0.53,-0.525,-0.52,-0.515,-0.51,-0.505,-0.5,-0.495,
-0.49,-0.485,-0.48,-0.475,-0.47,-0.465,-0.46,-0.455,-0.45,-0.445,-0.44,
-0.435,-0.43,-0.425,-0.42,-0.415,-0.41,-0.405,-0.4,-0.395,-0.39,-0.385,
-0.38,-0.375,-0.37,-0.365,-0.36,-0.355,-0.35,-0.345,-0.34,-0.335,-0.33,
-0.325,-0.32,-0.315,-0.31,-0.305,-0.3,-0.295,-0.29,-0.285,-0.28,-0.275,
-0.27,-0.265,-0.26,-0.255,-0.25,-0.245,-0.24,-0.235,-0.23,-0.225,-0.22,
-0.215,-0.21,-0.205,-0.2,-0.195,-0.19,-0.185,-0.18,-0.175,-0.17,-0.165,
-0.16,-0.155,-0.15,-0.145,-0.14,-0.135,-0.13,-0.125,-0.12,-0.115,-0.11,
-0.105,-0.1,-0.095,-0.09,-0.085,-0.08,-0.075,-0.07,-0.065,-0.06,-0.055,
-0.05,-0.045,-0.04,-0.035,-0.03,-0.025,-0.02,-0.015,-0.01,-0.005,0.),(0.,
1.2),.UNSPECIFIED.)
GEOMETRIC_REPRESENTATION_ITEM()
RATIONAL_B_SPLINE_SURFACE(((1.,1.),(1.,1.),(1.,1.),(1.,1.),(1.,1.),(1.,
1.),(1.,1.),(1.,1.),(1.,1.),(1.,1.),(1.,1.),(1.,1.),(1.,1.),(1.,1.),(1.,
1.),(1.,1.),(1.,1.),(1.,1.),(1.,1.),(1.,1.),(1.,1.),(1.,1.),(1.,1.),(1.,
1.),(1.,1.),(1.,1.),(1.,1.),(1.,1.),(1.,1.),(1.,1.),(1.,1.),(1.,1.),(1.,
1.),(1.,1.),(1.,1.),(1.,1.),(1.,1.),(1.,1.),(1.,1.),(1.,1.),(1.,1.),(1.,
1.),(1.,1.),(1.,1.),(1.,1.),(1.,1.),(1.,1.),(1.,1.),(1.,1.),(1.,1.),(1.,
1.),(1.,1.),(1.,1.),(1.,1.),(1.,1.),(1.,1.),(1.,1.),(1.,1.),(1.,1.),(1.,
1.),(1.,1.),(1.,1.),(1.,1.),(1.,1.),(1.,1.),(1.,1.),(1.,1.),(1.,1.),(1.,
1.),(1.,1.),(1.,1.),(1.,1.),(1.,1.),(1.,1.),(1.,1.),(1.,1.),(1.,1.),(1.,
1.),(1.,1.),(1.,1.),(1.,1.),(1.,1.),(1.,1.),(1.,1.),(1.,1.),(1.,1.),(1.,
1.),(1.,1.),(1.,1.),(1.,1.),(1.,1.),(1.,1.),(1.,1.),(1.,1.),(1.,1.),(1.,
1.),(1.,1.),(1.,1.),(1.,1.),(1.,1.),(1.,1.),(1.,1.),(1.,1.),(1.,1.),(1.,
1.),(1.,1.),(1.,1.),(1.,1.),(1.,1.),(1.,1.),(1.,1.),(1.,1.),(1.,1.),(1.,
1.),(1.,1.),(1.,1.),(1.,1.),(1.,1.),(1.,1.),(1.,1.),(1.,1.),(1.,1.),(1.,
1.),(1.,1.),(1.,1.),(1.,1.),(1.,1.),(1.,1.),(1.,1.),(1.,1.),(1.,1.),(1.,
1.),(1.,1.),(1.,1.),(1.,1.),(1.,1.),(1.,1.),(1.,1.),(1.,1.),(1.,1.),(1.,
1.),(1.,1.),(1.,1.),(1.,1.),(1.,1.),(1.,1.),(1.,1.),(1.,1.),(1.,1.),(1.,
1.),(1.,1.),(1.,1.),(1.,1.),(1.,1.),(1.,1.),(1.,1.),(1.,1.),(1.,1.),(1.,
1.),(1.,1.),(1.,1.),(1.,1.),(1.,1.),(1.,1.),(1.,1.),(1.,1.),(1.,1.),(1.,
1.),(1.,1.),(1.,1.),(1.,1.),(1.,1.),(1.,1.),(1.,1.),(1.,1.),(1.,1.),(1.,
1.),(1.,1.),(1.,1.),(1.,1.),(1.,1.),(1.,1.),(1.,1.),(1.,1.),(1.,1.),(1.,
1.),(1.,1.),(1.,1.),(1.,1.),(1.,1.),(1.,1.),(1.,1.),(1.,1.),(1.,1.),(1.,
1.),(1.,1.),(1.,1.),(1.,1.),(1.,1.),(1.,1.),(1.,1.),(1.,1.),(1.,1.),(1.,
1.),(1.,1.)))
REPRESENTATION_ITEM('')
SURFACE()
);
#1096=(
BOUNDED_SURFACE()
B_SPLINE_SURFACE(5,1,((#233351,#233352),(#233353,#233354),(#233355,#233356),
(#233357,#233358),(#233359,#233360),(#233361,#233362),(#233363,#233364),
(#233365,#233366),(#233367,#233368),(#233369,#233370),(#233371,#233372),
(#233373,#233374),(#233375,#233376),(#233377,#233378),(#233379,#233380),
(#233381,#233382),(#233383,#233384),(#233385,#233386),(#233387,#233388),
(#233389,#233390),(#233391,#233392),(#233393,#233394),(#233395,#233396),
(#233397,#233398),(#233399,#233400),(#233401,#233402),(#233403,#233404),
(#233405,#233406),(#233407,#233408),(#233409,#233410),(#233411,#233412),
(#233413,#233414),(#233415,#233416),(#233417,#233418),(#233419,#233420),
(#233421,#233422),(#233423,#233424),(#233425,#233426),(#233427,#233428),
(#233429,#233430),(#233431,#233432),(#233433,#233434),(#233435,#233436),
(#233437,#233438),(#233439,#233440),(#233441,#233442),(#233443,#233444),
(#233445,#233446),(#233447,#233448),(#233449,#233450),(#233451,#233452),
(#233453,#233454),(#233455,#233456),(#233457,#233458),(#233459,#233460),
(#233461,#233462),(#233463,#233464),(#233465,#233466),(#233467,#233468),
(#233469,#233470),(#233471,#233472),(#233473,#233474),(#233475,#233476),
(#233477,#233478),(#233479,#233480),(#233481,#233482),(#233483,#233484),
(#233485,#233486),(#233487,#233488),(#233489,#233490),(#233491,#233492),
(#233493,#233494),(#233495,#233496),(#233497,#233498),(#233499,#233500),
(#233501,#233502),(#233503,#233504),(#233505,#233506),(#233507,#233508),
(#233509,#233510),(#233511,#233512),(#233513,#233514),(#233515,#233516),
(#233517,#233518),(#233519,#233520),(#233521,#233522),(#233523,#233524),
(#233525,#233526),(#233527,#233528),(#233529,#233530),(#233531,#233532),
(#233533,#233534),(#233535,#233536),(#233537,#233538),(#233539,#233540),
(#233541,#233542),(#233543,#233544),(#233545,#233546),(#233547,#233548),
(#233549,#233550),(#233551,#233552),(#233553,#233554),(#233555,#233556),
(#233557,#233558),(#233559,#233560),(#233561,#233562),(#233563,#233564),
(#233565,#233566),(#233567,#233568),(#233569,#233570),(#233571,#233572),
(#233573,#233574),(#233575,#233576),(#233577,#233578),(#233579,#233580),
(#233581,#233582),(#233583,#233584),(#233585,#233586),(#233587,#233588),
(#233589,#233590),(#233591,#233592),(#233593,#233594),(#233595,#233596),
(#233597,#233598),(#233599,#233600),(#233601,#233602),(#233603,#233604),
(#233605,#233606),(#233607,#233608),(#233609,#233610),(#233611,#233612),
(#233613,#233614),(#233615,#233616),(#233617,#233618),(#233619,#233620),
(#233621,#233622),(#233623,#233624),(#233625,#233626),(#233627,#233628),
(#233629,#233630),(#233631,#233632),(#233633,#233634),(#233635,#233636),
(#233637,#233638),(#233639,#233640),(#233641,#233642),(#233643,#233644),
(#233645,#233646),(#233647,#233648),(#233649,#233650),(#233651,#233652),
(#233653,#233654),(#233655,#233656),(#233657,#233658),(#233659,#233660),
(#233661,#233662),(#233663,#233664),(#233665,#233666),(#233667,#233668),
(#233669,#233670),(#233671,#233672),(#233673,#233674),(#233675,#233676),
(#233677,#233678),(#233679,#233680),(#233681,#233682),(#233683,#233684),
(#233685,#233686),(#233687,#233688),(#233689,#233690),(#233691,#233692),
(#233693,#233694),(#233695,#233696),(#233697,#233698),(#233699,#233700),
(#233701,#233702),(#233703,#233704),(#233705,#233706),(#233707,#233708),
(#233709,#233710),(#233711,#233712),(#233713,#233714),(#233715,#233716),
(#233717,#233718),(#233719,#233720),(#233721,#233722),(#233723,#233724),
(#233725,#233726),(#233727,#233728),(#233729,#233730),(#233731,#233732),
(#233733,#233734),(#233735,#233736),(#233737,#233738),(#233739,#233740),
(#233741,#233742),(#233743,#233744),(#233745,#233746),(#233747,#233748),
(#233749,#233750),(#233751,#233752),(#233753,#233754),(#233755,#233756),
(#233757,#233758),(#233759,#233760)),.UNSPECIFIED.,.F.,.F.,.F.)
B_SPLINE_SURFACE_WITH_KNOTS((6,1,1,1,1,1,1,1,1,1,1,1,1,1,1,1,1,1,1,1,1,
1,1,1,1,1,1,1,1,1,1,1,1,1,1,1,1,1,1,1,1,1,1,1,1,1,1,1,1,1,1,1,1,1,1,1,1,
1,1,1,1,1,1,1,1,1,1,1,1,1,1,1,1,1,1,1,1,1,1,1,1,1,1,1,1,1,1,1,1,1,1,1,1,
1,1,1,1,1,1,1,1,1,1,1,1,1,1,1,1,1,1,1,1,1,1,1,1,1,1,1,1,1,1,1,1,1,1,1,1,
1,1,1,1,1,1,1,1,1,1,1,1,1,1,1,1,1,1,1,1,1,1,1,1,1,1,1,1,1,1,1,1,1,1,1,1,
1,1,1,1,1,1,1,1,1,1,1,1,1,1,1,1,1,1,1,1,1,1,1,1,1,1,1,1,1,1,1,1,1,1,1,6),
(2,2),(0.,0.005,0.01,0.015,0.02,0.025,0.03,0.035,0.04,0.045,0.05,0.055,
0.06,0.065,0.07,0.075,0.08,0.085,0.09,0.095,0.1,0.105,0.11,0.115,0.12,0.125,
0.13,0.135,0.14,0.145,0.15,0.155,0.16,0.165,0.17,0.175,0.18,0.185,0.19,
0.195,0.2,0.205,0.21,0.215,0.22,0.225,0.23,0.235,0.24,0.245,0.25,0.255,
0.26,0.265,0.27,0.275,0.28,0.285,0.29,0.295,0.3,0.305,0.31,0.315,0.32,0.325,
0.33,0.335,0.34,0.345,0.35,0.355,0.36,0.365,0.37,0.375,0.38,0.385,0.39,
0.395,0.4,0.405,0.41,0.415,0.42,0.425,0.43,0.435,0.44,0.445,0.45,0.455,
0.46,0.465,0.47,0.475,0.48,0.485,0.49,0.495,0.5,0.505,0.51,0.515,0.52,0.525,
0.53,0.535,0.54,0.545,0.55,0.555,0.56,0.565,0.57,0.575,0.58,0.585,0.59,
0.595,0.6,0.605,0.61,0.615,0.62,0.625,0.63,0.635,0.64,0.645,0.65,0.655,
0.66,0.665,0.67,0.675,0.68,0.685,0.690000000000001,0.695000000000001,0.700000000000001,
0.705000000000001,0.710000000000001,0.715000000000001,0.720000000000001,
0.725000000000001,0.730000000000001,0.735000000000001,0.740000000000001,
0.745000000000001,0.750000000000001,0.755000000000001,0.760000000000001,
0.765000000000001,0.770000000000001,0.775000000000001,0.780000000000001,
0.785000000000001,0.790000000000001,0.795000000000001,0.800000000000001,
0.805000000000001,0.810000000000001,0.815000000000001,0.820000000000001,
0.825000000000001,0.830000000000001,0.835000000000001,0.840000000000001,
0.845000000000001,0.850000000000001,0.855000000000001,0.860000000000001,
0.865000000000001,0.870000000000001,0.875000000000001,0.880000000000001,
0.885000000000001,0.890000000000001,0.895000000000001,0.900000000000001,
0.905000000000001,0.910000000000001,0.915000000000001,0.920000000000001,
0.925000000000001,0.930000000000001,0.935000000000001,0.940000000000001,
0.945000000000001,0.950000000000001,0.955000000000001,0.960000000000001,
0.965000000000001,0.970000000000001,0.975000000000001,0.980000000000001,
0.985000000000001,0.990000000000001,0.995000000000001,1.),(0.,1.2),
 .UNSPECIFIED.)
GEOMETRIC_REPRESENTATION_ITEM()
RATIONAL_B_SPLINE_SURFACE(((1.,1.),(1.,1.),(1.,1.),(1.,1.),(1.,1.),(1.,
1.),(1.,1.),(1.,1.),(1.,1.),(1.,1.),(1.,1.),(1.,1.),(1.,1.),(1.,1.),(1.,
1.),(1.,1.),(1.,1.),(1.,1.),(1.,1.),(1.,1.),(1.,1.),(1.,1.),(1.,1.),(1.,
1.),(1.,1.),(1.,1.),(1.,1.),(1.,1.),(1.,1.),(1.,1.),(1.,1.),(1.,1.),(1.,
1.),(1.,1.),(1.,1.),(1.,1.),(1.,1.),(1.,1.),(1.,1.),(1.,1.),(1.,1.),(1.,
1.),(1.,1.),(1.,1.),(1.,1.),(1.,1.),(1.,1.),(1.,1.),(1.,1.),(1.,1.),(1.,
1.),(1.,1.),(1.,1.),(1.,1.),(1.,1.),(1.,1.),(1.,1.),(1.,1.),(1.,1.),(1.,
1.),(1.,1.),(1.,1.),(1.,1.),(1.,1.),(1.,1.),(1.,1.),(1.,1.),(1.,1.),(1.,
1.),(1.,1.),(1.,1.),(1.,1.),(1.,1.),(1.,1.),(1.,1.),(1.,1.),(1.,1.),(1.,
1.),(1.,1.),(1.,1.),(1.,1.),(1.,1.),(1.,1.),(1.,1.),(1.,1.),(1.,1.),(1.,
1.),(1.,1.),(1.,1.),(1.,1.),(1.,1.),(1.,1.),(1.,1.),(1.,1.),(1.,1.),(1.,
1.),(1.,1.),(1.,1.),(1.,1.),(1.,1.),(1.,1.),(1.,1.),(1.,1.),(1.,1.),(1.,
1.),(1.,1.),(1.,1.),(1.,1.),(1.,1.),(1.,1.),(1.,1.),(1.,1.),(1.,1.),(1.,
1.),(1.,1.),(1.,1.),(1.,1.),(1.,1.),(1.,1.),(1.,1.),(1.,1.),(1.,1.),(1.,
1.),(1.,1.),(1.,1.),(1.,1.),(1.,1.),(1.,1.),(1.,1.),(1.,1.),(1.,1.),(1.,
1.),(1.,1.),(1.,1.),(1.,1.),(1.,1.),(1.,1.),(1.,1.),(1.,1.),(1.,1.),(1.,
1.),(1.,1.),(1.,1.),(1.,1.),(1.,1.),(1.,1.),(1.,1.),(1.,1.),(1.,1.),(1.,
1.),(1.,1.),(1.,1.),(1.,1.),(1.,1.),(1.,1.),(1.,1.),(1.,1.),(1.,1.),(1.,
1.),(1.,1.),(1.,1.),(1.,1.),(1.,1.),(1.,1.),(1.,1.),(1.,1.),(1.,1.),(1.,
1.),(1.,1.),(1.,1.),(1.,1.),(1.,1.),(1.,1.),(1.,1.),(1.,1.),(1.,1.),(1.,
1.),(1.,1.),(1.,1.),(1.,1.),(1.,1.),(1.,1.),(1.,1.),(1.,1.),(1.,1.),(1.,
1.),(1.,1.),(1.,1.),(1.,1.),(1.,1.),(1.,1.),(1.,1.),(1.,1.),(1.,1.),(1.,
1.),(1.,1.),(1.,1.),(1.,1.),(1.,1.),(1.,1.),(1.,1.),(1.,1.),(1.,1.),(1.,
1.),(1.,1.)))
REPRESENTATION_ITEM('')
SURFACE()
);
#1097=(
BOUNDED_SURFACE()
B_SPLINE_SURFACE(5,1,((#234180,#234181),(#234182,#234183),(#234184,#234185),
(#234186,#234187),(#234188,#234189),(#234190,#234191),(#234192,#234193),
(#234194,#234195),(#234196,#234197),(#234198,#234199),(#234200,#234201),
(#234202,#234203),(#234204,#234205),(#234206,#234207),(#234208,#234209),
(#234210,#234211),(#234212,#234213),(#234214,#234215),(#234216,#234217),
(#234218,#234219),(#234220,#234221),(#234222,#234223),(#234224,#234225),
(#234226,#234227),(#234228,#234229),(#234230,#234231),(#234232,#234233),
(#234234,#234235),(#234236,#234237),(#234238,#234239),(#234240,#234241),
(#234242,#234243),(#234244,#234245),(#234246,#234247),(#234248,#234249),
(#234250,#234251),(#234252,#234253),(#234254,#234255),(#234256,#234257),
(#234258,#234259),(#234260,#234261),(#234262,#234263),(#234264,#234265),
(#234266,#234267),(#234268,#234269),(#234270,#234271),(#234272,#234273),
(#234274,#234275),(#234276,#234277),(#234278,#234279),(#234280,#234281),
(#234282,#234283),(#234284,#234285),(#234286,#234287),(#234288,#234289),
(#234290,#234291),(#234292,#234293),(#234294,#234295),(#234296,#234297),
(#234298,#234299),(#234300,#234301),(#234302,#234303),(#234304,#234305),
(#234306,#234307),(#234308,#234309),(#234310,#234311),(#234312,#234313),
(#234314,#234315),(#234316,#234317),(#234318,#234319),(#234320,#234321),
(#234322,#234323),(#234324,#234325),(#234326,#234327),(#234328,#234329),
(#234330,#234331),(#234332,#234333),(#234334,#234335),(#234336,#234337),
(#234338,#234339),(#234340,#234341),(#234342,#234343),(#234344,#234345),
(#234346,#234347),(#234348,#234349),(#234350,#234351),(#234352,#234353),
(#234354,#234355),(#234356,#234357),(#234358,#234359),(#234360,#234361),
(#234362,#234363),(#234364,#234365),(#234366,#234367),(#234368,#234369),
(#234370,#234371),(#234372,#234373),(#234374,#234375),(#234376,#234377),
(#234378,#234379),(#234380,#234381),(#234382,#234383),(#234384,#234385),
(#234386,#234387),(#234388,#234389),(#234390,#234391),(#234392,#234393),
(#234394,#234395),(#234396,#234397),(#234398,#234399),(#234400,#234401),
(#234402,#234403),(#234404,#234405),(#234406,#234407),(#234408,#234409),
(#234410,#234411),(#234412,#234413),(#234414,#234415),(#234416,#234417),
(#234418,#234419),(#234420,#234421),(#234422,#234423),(#234424,#234425),
(#234426,#234427),(#234428,#234429),(#234430,#234431),(#234432,#234433),
(#234434,#234435),(#234436,#234437),(#234438,#234439),(#234440,#234441),
(#234442,#234443),(#234444,#234445),(#234446,#234447),(#234448,#234449),
(#234450,#234451),(#234452,#234453),(#234454,#234455),(#234456,#234457),
(#234458,#234459),(#234460,#234461),(#234462,#234463),(#234464,#234465),
(#234466,#234467),(#234468,#234469),(#234470,#234471),(#234472,#234473),
(#234474,#234475),(#234476,#234477),(#234478,#234479),(#234480,#234481),
(#234482,#234483),(#234484,#234485),(#234486,#234487),(#234488,#234489),
(#234490,#234491),(#234492,#234493),(#234494,#234495),(#234496,#234497),
(#234498,#234499),(#234500,#234501),(#234502,#234503),(#234504,#234505),
(#234506,#234507),(#234508,#234509),(#234510,#234511),(#234512,#234513),
(#234514,#234515),(#234516,#234517),(#234518,#234519),(#234520,#234521),
(#234522,#234523),(#234524,#234525),(#234526,#234527),(#234528,#234529),
(#234530,#234531),(#234532,#234533),(#234534,#234535),(#234536,#234537),
(#234538,#234539),(#234540,#234541),(#234542,#234543),(#234544,#234545),
(#234546,#234547),(#234548,#234549),(#234550,#234551),(#234552,#234553),
(#234554,#234555),(#234556,#234557),(#234558,#234559),(#234560,#234561),
(#234562,#234563),(#234564,#234565),(#234566,#234567),(#234568,#234569),
(#234570,#234571),(#234572,#234573),(#234574,#234575),(#234576,#234577),
(#234578,#234579),(#234580,#234581),(#234582,#234583),(#234584,#234585),
(#234586,#234587),(#234588,#234589)),.UNSPECIFIED.,.F.,.F.,.F.)
B_SPLINE_SURFACE_WITH_KNOTS((6,1,1,1,1,1,1,1,1,1,1,1,1,1,1,1,1,1,1,1,1,
1,1,1,1,1,1,1,1,1,1,1,1,1,1,1,1,1,1,1,1,1,1,1,1,1,1,1,1,1,1,1,1,1,1,1,1,
1,1,1,1,1,1,1,1,1,1,1,1,1,1,1,1,1,1,1,1,1,1,1,1,1,1,1,1,1,1,1,1,1,1,1,1,
1,1,1,1,1,1,1,1,1,1,1,1,1,1,1,1,1,1,1,1,1,1,1,1,1,1,1,1,1,1,1,1,1,1,1,1,
1,1,1,1,1,1,1,1,1,1,1,1,1,1,1,1,1,1,1,1,1,1,1,1,1,1,1,1,1,1,1,1,1,1,1,1,
1,1,1,1,1,1,1,1,1,1,1,1,1,1,1,1,1,1,1,1,1,1,1,1,1,1,1,1,1,1,1,1,1,1,1,6),
(2,2),(-1.,-0.995000000000001,-0.990000000000001,-0.985000000000001,-0.980000000000001,
-0.975000000000001,-0.970000000000001,-0.965000000000001,-0.960000000000001,
-0.955000000000001,-0.950000000000001,-0.945000000000001,-0.940000000000001,
-0.935000000000001,-0.930000000000001,-0.925000000000001,-0.920000000000001,
-0.915000000000001,-0.910000000000001,-0.905000000000001,-0.900000000000001,
-0.895000000000001,-0.890000000000001,-0.885000000000001,-0.880000000000001,
-0.875000000000001,-0.870000000000001,-0.865000000000001,-0.860000000000001,
-0.855000000000001,-0.850000000000001,-0.845000000000001,-0.840000000000001,
-0.835000000000001,-0.830000000000001,-0.825000000000001,-0.820000000000001,
-0.815000000000001,-0.810000000000001,-0.805000000000001,-0.800000000000001,
-0.795000000000001,-0.790000000000001,-0.785000000000001,-0.780000000000001,
-0.775000000000001,-0.770000000000001,-0.765000000000001,-0.760000000000001,
-0.755000000000001,-0.750000000000001,-0.745000000000001,-0.740000000000001,
-0.735000000000001,-0.730000000000001,-0.725000000000001,-0.720000000000001,
-0.715000000000001,-0.710000000000001,-0.705000000000001,-0.700000000000001,
-0.695000000000001,-0.690000000000001,-0.685,-0.68,-0.675,-0.67,-0.665,
-0.66,-0.655,-0.65,-0.645,-0.64,-0.635,-0.63,-0.625,-0.62,-0.615,-0.61,
-0.605,-0.6,-0.595,-0.59,-0.585,-0.58,-0.575,-0.57,-0.565,-0.56,-0.555,
-0.55,-0.545,-0.54,-0.535,-0.53,-0.525,-0.52,-0.515,-0.51,-0.505,-0.5,-0.495,
-0.49,-0.485,-0.48,-0.475,-0.47,-0.465,-0.46,-0.455,-0.45,-0.445,-0.44,
-0.435,-0.43,-0.425,-0.42,-0.415,-0.41,-0.405,-0.4,-0.395,-0.39,-0.385,
-0.38,-0.375,-0.37,-0.365,-0.36,-0.355,-0.35,-0.345,-0.34,-0.335,-0.33,
-0.325,-0.32,-0.315,-0.31,-0.305,-0.3,-0.295,-0.29,-0.285,-0.28,-0.275,
-0.27,-0.265,-0.26,-0.255,-0.25,-0.245,-0.24,-0.235,-0.23,-0.225,-0.22,
-0.215,-0.21,-0.205,-0.2,-0.195,-0.19,-0.185,-0.18,-0.175,-0.17,-0.165,
-0.16,-0.155,-0.15,-0.145,-0.14,-0.135,-0.13,-0.125,-0.12,-0.115,-0.11,
-0.105,-0.1,-0.095,-0.09,-0.085,-0.08,-0.075,-0.07,-0.065,-0.06,-0.055,
-0.05,-0.045,-0.04,-0.035,-0.03,-0.025,-0.02,-0.015,-0.01,-0.005,0.),(0.,
1.2),.UNSPECIFIED.)
GEOMETRIC_REPRESENTATION_ITEM()
RATIONAL_B_SPLINE_SURFACE(((1.,1.),(1.,1.),(1.,1.),(1.,1.),(1.,1.),(1.,
1.),(1.,1.),(1.,1.),(1.,1.),(1.,1.),(1.,1.),(1.,1.),(1.,1.),(1.,1.),(1.,
1.),(1.,1.),(1.,1.),(1.,1.),(1.,1.),(1.,1.),(1.,1.),(1.,1.),(1.,1.),(1.,
1.),(1.,1.),(1.,1.),(1.,1.),(1.,1.),(1.,1.),(1.,1.),(1.,1.),(1.,1.),(1.,
1.),(1.,1.),(1.,1.),(1.,1.),(1.,1.),(1.,1.),(1.,1.),(1.,1.),(1.,1.),(1.,
1.),(1.,1.),(1.,1.),(1.,1.),(1.,1.),(1.,1.),(1.,1.),(1.,1.),(1.,1.),(1.,
1.),(1.,1.),(1.,1.),(1.,1.),(1.,1.),(1.,1.),(1.,1.),(1.,1.),(1.,1.),(1.,
1.),(1.,1.),(1.,1.),(1.,1.),(1.,1.),(1.,1.),(1.,1.),(1.,1.),(1.,1.),(1.,
1.),(1.,1.),(1.,1.),(1.,1.),(1.,1.),(1.,1.),(1.,1.),(1.,1.),(1.,1.),(1.,
1.),(1.,1.),(1.,1.),(1.,1.),(1.,1.),(1.,1.),(1.,1.),(1.,1.),(1.,1.),(1.,
1.),(1.,1.),(1.,1.),(1.,1.),(1.,1.),(1.,1.),(1.,1.),(1.,1.),(1.,1.),(1.,
1.),(1.,1.),(1.,1.),(1.,1.),(1.,1.),(1.,1.),(1.,1.),(1.,1.),(1.,1.),(1.,
1.),(1.,1.),(1.,1.),(1.,1.),(1.,1.),(1.,1.),(1.,1.),(1.,1.),(1.,1.),(1.,
1.),(1.,1.),(1.,1.),(1.,1.),(1.,1.),(1.,1.),(1.,1.),(1.,1.),(1.,1.),(1.,
1.),(1.,1.),(1.,1.),(1.,1.),(1.,1.),(1.,1.),(1.,1.),(1.,1.),(1.,1.),(1.,
1.),(1.,1.),(1.,1.),(1.,1.),(1.,1.),(1.,1.),(1.,1.),(1.,1.),(1.,1.),(1.,
1.),(1.,1.),(1.,1.),(1.,1.),(1.,1.),(1.,1.),(1.,1.),(1.,1.),(1.,1.),(1.,
1.),(1.,1.),(1.,1.),(1.,1.),(1.,1.),(1.,1.),(1.,1.),(1.,1.),(1.,1.),(1.,
1.),(1.,1.),(1.,1.),(1.,1.),(1.,1.),(1.,1.),(1.,1.),(1.,1.),(1.,1.),(1.,
1.),(1.,1.),(1.,1.),(1.,1.),(1.,1.),(1.,1.),(1.,1.),(1.,1.),(1.,1.),(1.,
1.),(1.,1.),(1.,1.),(1.,1.),(1.,1.),(1.,1.),(1.,1.),(1.,1.),(1.,1.),(1.,
1.),(1.,1.),(1.,1.),(1.,1.),(1.,1.),(1.,1.),(1.,1.),(1.,1.),(1.,1.),(1.,
1.),(1.,1.),(1.,1.),(1.,1.),(1.,1.),(1.,1.),(1.,1.),(1.,1.),(1.,1.),(1.,
1.),(1.,1.)))
REPRESENTATION_ITEM('')
SURFACE()
);
#1098=(
BOUNDED_SURFACE()
B_SPLINE_SURFACE(5,1,((#235003,#235004),(#235005,#235006),(#235007,#235008),
(#235009,#235010),(#235011,#235012),(#235013,#235014),(#235015,#235016),
(#235017,#235018),(#235019,#235020),(#235021,#235022),(#235023,#235024),
(#235025,#235026),(#235027,#235028),(#235029,#235030),(#235031,#235032),
(#235033,#235034),(#235035,#235036),(#235037,#235038),(#235039,#235040),
(#235041,#235042),(#235043,#235044),(#235045,#235046),(#235047,#235048),
(#235049,#235050),(#235051,#235052),(#235053,#235054),(#235055,#235056),
(#235057,#235058),(#235059,#235060),(#235061,#235062),(#235063,#235064),
(#235065,#235066),(#235067,#235068),(#235069,#235070),(#235071,#235072),
(#235073,#235074),(#235075,#235076),(#235077,#235078),(#235079,#235080),
(#235081,#235082),(#235083,#235084),(#235085,#235086),(#235087,#235088),
(#235089,#235090),(#235091,#235092),(#235093,#235094),(#235095,#235096),
(#235097,#235098),(#235099,#235100),(#235101,#235102),(#235103,#235104),
(#235105,#235106),(#235107,#235108),(#235109,#235110),(#235111,#235112),
(#235113,#235114),(#235115,#235116),(#235117,#235118),(#235119,#235120),
(#235121,#235122),(#235123,#235124),(#235125,#235126),(#235127,#235128),
(#235129,#235130),(#235131,#235132),(#235133,#235134),(#235135,#235136),
(#235137,#235138),(#235139,#235140),(#235141,#235142),(#235143,#235144),
(#235145,#235146),(#235147,#235148),(#235149,#235150),(#235151,#235152),
(#235153,#235154),(#235155,#235156),(#235157,#235158),(#235159,#235160),
(#235161,#235162),(#235163,#235164),(#235165,#235166),(#235167,#235168),
(#235169,#235170),(#235171,#235172),(#235173,#235174),(#235175,#235176),
(#235177,#235178),(#235179,#235180),(#235181,#235182),(#235183,#235184),
(#235185,#235186),(#235187,#235188),(#235189,#235190),(#235191,#235192),
(#235193,#235194),(#235195,#235196),(#235197,#235198),(#235199,#235200),
(#235201,#235202),(#235203,#235204),(#235205,#235206),(#235207,#235208),
(#235209,#235210),(#235211,#235212),(#235213,#235214),(#235215,#235216),
(#235217,#235218),(#235219,#235220),(#235221,#235222),(#235223,#235224),
(#235225,#235226),(#235227,#235228),(#235229,#235230),(#235231,#235232),
(#235233,#235234),(#235235,#235236),(#235237,#235238),(#235239,#235240),
(#235241,#235242),(#235243,#235244),(#235245,#235246),(#235247,#235248),
(#235249,#235250),(#235251,#235252),(#235253,#235254),(#235255,#235256),
(#235257,#235258),(#235259,#235260),(#235261,#235262),(#235263,#235264),
(#235265,#235266),(#235267,#235268),(#235269,#235270),(#235271,#235272),
(#235273,#235274),(#235275,#235276),(#235277,#235278),(#235279,#235280),
(#235281,#235282),(#235283,#235284),(#235285,#235286),(#235287,#235288),
(#235289,#235290),(#235291,#235292),(#235293,#235294),(#235295,#235296),
(#235297,#235298),(#235299,#235300),(#235301,#235302),(#235303,#235304),
(#235305,#235306),(#235307,#235308),(#235309,#235310),(#235311,#235312),
(#235313,#235314),(#235315,#235316),(#235317,#235318),(#235319,#235320),
(#235321,#235322),(#235323,#235324),(#235325,#235326),(#235327,#235328),
(#235329,#235330),(#235331,#235332),(#235333,#235334),(#235335,#235336),
(#235337,#235338),(#235339,#235340),(#235341,#235342),(#235343,#235344),
(#235345,#235346),(#235347,#235348),(#235349,#235350),(#235351,#235352),
(#235353,#235354),(#235355,#235356),(#235357,#235358),(#235359,#235360),
(#235361,#235362),(#235363,#235364),(#235365,#235366),(#235367,#235368),
(#235369,#235370),(#235371,#235372),(#235373,#235374),(#235375,#235376),
(#235377,#235378),(#235379,#235380),(#235381,#235382),(#235383,#235384),
(#235385,#235386),(#235387,#235388),(#235389,#235390),(#235391,#235392),
(#235393,#235394),(#235395,#235396),(#235397,#235398),(#235399,#235400),
(#235401,#235402),(#235403,#235404),(#235405,#235406),(#235407,#235408),
(#235409,#235410),(#235411,#235412)),.UNSPECIFIED.,.F.,.F.,.F.)
B_SPLINE_SURFACE_WITH_KNOTS((6,1,1,1,1,1,1,1,1,1,1,1,1,1,1,1,1,1,1,1,1,
1,1,1,1,1,1,1,1,1,1,1,1,1,1,1,1,1,1,1,1,1,1,1,1,1,1,1,1,1,1,1,1,1,1,1,1,
1,1,1,1,1,1,1,1,1,1,1,1,1,1,1,1,1,1,1,1,1,1,1,1,1,1,1,1,1,1,1,1,1,1,1,1,
1,1,1,1,1,1,1,1,1,1,1,1,1,1,1,1,1,1,1,1,1,1,1,1,1,1,1,1,1,1,1,1,1,1,1,1,
1,1,1,1,1,1,1,1,1,1,1,1,1,1,1,1,1,1,1,1,1,1,1,1,1,1,1,1,1,1,1,1,1,1,1,1,
1,1,1,1,1,1,1,1,1,1,1,1,1,1,1,1,1,1,1,1,1,1,1,1,1,1,1,1,1,1,1,1,1,1,1,6),
(2,2),(0.,0.005,0.01,0.015,0.02,0.025,0.03,0.035,0.04,0.045,0.05,0.055,
0.06,0.065,0.07,0.075,0.08,0.085,0.09,0.095,0.1,0.105,0.11,0.115,0.12,0.125,
0.13,0.135,0.14,0.145,0.15,0.155,0.16,0.165,0.17,0.175,0.18,0.185,0.19,
0.195,0.2,0.205,0.21,0.215,0.22,0.225,0.23,0.235,0.24,0.245,0.25,0.255,
0.26,0.265,0.27,0.275,0.28,0.285,0.29,0.295,0.3,0.305,0.31,0.315,0.32,0.325,
0.33,0.335,0.34,0.345,0.35,0.355,0.36,0.365,0.37,0.375,0.38,0.385,0.39,
0.395,0.4,0.405,0.41,0.415,0.42,0.425,0.43,0.435,0.44,0.445,0.45,0.455,
0.46,0.465,0.47,0.475,0.48,0.485,0.49,0.495,0.5,0.505,0.51,0.515,0.52,0.525,
0.53,0.535,0.54,0.545,0.55,0.555,0.56,0.565,0.57,0.575,0.58,0.585,0.59,
0.595,0.6,0.605,0.61,0.615,0.62,0.625,0.63,0.635,0.64,0.645,0.65,0.655,
0.66,0.665,0.67,0.675,0.68,0.685,0.690000000000001,0.695000000000001,0.700000000000001,
0.705000000000001,0.710000000000001,0.715000000000001,0.720000000000001,
0.725000000000001,0.730000000000001,0.735000000000001,0.740000000000001,
0.745000000000001,0.750000000000001,0.755000000000001,0.760000000000001,
0.765000000000001,0.770000000000001,0.775000000000001,0.780000000000001,
0.785000000000001,0.790000000000001,0.795000000000001,0.800000000000001,
0.805000000000001,0.810000000000001,0.815000000000001,0.820000000000001,
0.825000000000001,0.830000000000001,0.835000000000001,0.840000000000001,
0.845000000000001,0.850000000000001,0.855000000000001,0.860000000000001,
0.865000000000001,0.870000000000001,0.875000000000001,0.880000000000001,
0.885000000000001,0.890000000000001,0.895000000000001,0.900000000000001,
0.905000000000001,0.910000000000001,0.915000000000001,0.920000000000001,
0.925000000000001,0.930000000000001,0.935000000000001,0.940000000000001,
0.945000000000001,0.950000000000001,0.955000000000001,0.960000000000001,
0.965000000000001,0.970000000000001,0.975000000000001,0.980000000000001,
0.985000000000001,0.990000000000001,0.995000000000001,1.),(0.,1.2),
 .UNSPECIFIED.)
GEOMETRIC_REPRESENTATION_ITEM()
RATIONAL_B_SPLINE_SURFACE(((1.,1.),(1.,1.),(1.,1.),(1.,1.),(1.,1.),(1.,
1.),(1.,1.),(1.,1.),(1.,1.),(1.,1.),(1.,1.),(1.,1.),(1.,1.),(1.,1.),(1.,
1.),(1.,1.),(1.,1.),(1.,1.),(1.,1.),(1.,1.),(1.,1.),(1.,1.),(1.,1.),(1.,
1.),(1.,1.),(1.,1.),(1.,1.),(1.,1.),(1.,1.),(1.,1.),(1.,1.),(1.,1.),(1.,
1.),(1.,1.),(1.,1.),(1.,1.),(1.,1.),(1.,1.),(1.,1.),(1.,1.),(1.,1.),(1.,
1.),(1.,1.),(1.,1.),(1.,1.),(1.,1.),(1.,1.),(1.,1.),(1.,1.),(1.,1.),(1.,
1.),(1.,1.),(1.,1.),(1.,1.),(1.,1.),(1.,1.),(1.,1.),(1.,1.),(1.,1.),(1.,
1.),(1.,1.),(1.,1.),(1.,1.),(1.,1.),(1.,1.),(1.,1.),(1.,1.),(1.,1.),(1.,
1.),(1.,1.),(1.,1.),(1.,1.),(1.,1.),(1.,1.),(1.,1.),(1.,1.),(1.,1.),(1.,
1.),(1.,1.),(1.,1.),(1.,1.),(1.,1.),(1.,1.),(1.,1.),(1.,1.),(1.,1.),(1.,
1.),(1.,1.),(1.,1.),(1.,1.),(1.,1.),(1.,1.),(1.,1.),(1.,1.),(1.,1.),(1.,
1.),(1.,1.),(1.,1.),(1.,1.),(1.,1.),(1.,1.),(1.,1.),(1.,1.),(1.,1.),(1.,
1.),(1.,1.),(1.,1.),(1.,1.),(1.,1.),(1.,1.),(1.,1.),(1.,1.),(1.,1.),(1.,
1.),(1.,1.),(1.,1.),(1.,1.),(1.,1.),(1.,1.),(1.,1.),(1.,1.),(1.,1.),(1.,
1.),(1.,1.),(1.,1.),(1.,1.),(1.,1.),(1.,1.),(1.,1.),(1.,1.),(1.,1.),(1.,
1.),(1.,1.),(1.,1.),(1.,1.),(1.,1.),(1.,1.),(1.,1.),(1.,1.),(1.,1.),(1.,
1.),(1.,1.),(1.,1.),(1.,1.),(1.,1.),(1.,1.),(1.,1.),(1.,1.),(1.,1.),(1.,
1.),(1.,1.),(1.,1.),(1.,1.),(1.,1.),(1.,1.),(1.,1.),(1.,1.),(1.,1.),(1.,
1.),(1.,1.),(1.,1.),(1.,1.),(1.,1.),(1.,1.),(1.,1.),(1.,1.),(1.,1.),(1.,
1.),(1.,1.),(1.,1.),(1.,1.),(1.,1.),(1.,1.),(1.,1.),(1.,1.),(1.,1.),(1.,
1.),(1.,1.),(1.,1.),(1.,1.),(1.,1.),(1.,1.),(1.,1.),(1.,1.),(1.,1.),(1.,
1.),(1.,1.),(1.,1.),(1.,1.),(1.,1.),(1.,1.),(1.,1.),(1.,1.),(1.,1.),(1.,
1.),(1.,1.),(1.,1.),(1.,1.),(1.,1.),(1.,1.),(1.,1.),(1.,1.),(1.,1.),(1.,
1.),(1.,1.)))
REPRESENTATION_ITEM('')
SURFACE()
);
#1099=(
BOUNDED_SURFACE()
B_SPLINE_SURFACE(5,1,((#235832,#235833),(#235834,#235835),(#235836,#235837),
(#235838,#235839),(#235840,#235841),(#235842,#235843),(#235844,#235845),
(#235846,#235847),(#235848,#235849),(#235850,#235851),(#235852,#235853),
(#235854,#235855),(#235856,#235857),(#235858,#235859),(#235860,#235861),
(#235862,#235863),(#235864,#235865),(#235866,#235867),(#235868,#235869),
(#235870,#235871),(#235872,#235873),(#235874,#235875),(#235876,#235877),
(#235878,#235879),(#235880,#235881),(#235882,#235883),(#235884,#235885),
(#235886,#235887),(#235888,#235889),(#235890,#235891),(#235892,#235893),
(#235894,#235895),(#235896,#235897),(#235898,#235899),(#235900,#235901),
(#235902,#235903),(#235904,#235905),(#235906,#235907),(#235908,#235909),
(#235910,#235911),(#235912,#235913),(#235914,#235915),(#235916,#235917),
(#235918,#235919),(#235920,#235921),(#235922,#235923),(#235924,#235925),
(#235926,#235927),(#235928,#235929),(#235930,#235931),(#235932,#235933),
(#235934,#235935),(#235936,#235937),(#235938,#235939),(#235940,#235941),
(#235942,#235943),(#235944,#235945),(#235946,#235947),(#235948,#235949),
(#235950,#235951),(#235952,#235953),(#235954,#235955),(#235956,#235957),
(#235958,#235959),(#235960,#235961),(#235962,#235963),(#235964,#235965),
(#235966,#235967),(#235968,#235969),(#235970,#235971),(#235972,#235973),
(#235974,#235975),(#235976,#235977),(#235978,#235979),(#235980,#235981),
(#235982,#235983),(#235984,#235985),(#235986,#235987),(#235988,#235989),
(#235990,#235991),(#235992,#235993),(#235994,#235995),(#235996,#235997),
(#235998,#235999),(#236000,#236001),(#236002,#236003),(#236004,#236005),
(#236006,#236007),(#236008,#236009),(#236010,#236011),(#236012,#236013),
(#236014,#236015),(#236016,#236017),(#236018,#236019),(#236020,#236021),
(#236022,#236023),(#236024,#236025),(#236026,#236027),(#236028,#236029),
(#236030,#236031),(#236032,#236033),(#236034,#236035),(#236036,#236037),
(#236038,#236039),(#236040,#236041),(#236042,#236043),(#236044,#236045),
(#236046,#236047),(#236048,#236049),(#236050,#236051),(#236052,#236053),
(#236054,#236055),(#236056,#236057),(#236058,#236059),(#236060,#236061),
(#236062,#236063),(#236064,#236065),(#236066,#236067),(#236068,#236069),
(#236070,#236071),(#236072,#236073),(#236074,#236075),(#236076,#236077),
(#236078,#236079),(#236080,#236081),(#236082,#236083),(#236084,#236085),
(#236086,#236087),(#236088,#236089),(#236090,#236091),(#236092,#236093),
(#236094,#236095),(#236096,#236097),(#236098,#236099),(#236100,#236101),
(#236102,#236103),(#236104,#236105),(#236106,#236107),(#236108,#236109),
(#236110,#236111),(#236112,#236113),(#236114,#236115),(#236116,#236117),
(#236118,#236119),(#236120,#236121),(#236122,#236123),(#236124,#236125),
(#236126,#236127),(#236128,#236129),(#236130,#236131),(#236132,#236133),
(#236134,#236135),(#236136,#236137),(#236138,#236139),(#236140,#236141),
(#236142,#236143),(#236144,#236145),(#236146,#236147),(#236148,#236149),
(#236150,#236151),(#236152,#236153),(#236154,#236155),(#236156,#236157),
(#236158,#236159),(#236160,#236161),(#236162,#236163),(#236164,#236165),
(#236166,#236167),(#236168,#236169),(#236170,#236171),(#236172,#236173),
(#236174,#236175),(#236176,#236177),(#236178,#236179),(#236180,#236181),
(#236182,#236183),(#236184,#236185),(#236186,#236187),(#236188,#236189),
(#236190,#236191),(#236192,#236193),(#236194,#236195),(#236196,#236197),
(#236198,#236199),(#236200,#236201),(#236202,#236203),(#236204,#236205),
(#236206,#236207),(#236208,#236209),(#236210,#236211),(#236212,#236213),
(#236214,#236215),(#236216,#236217),(#236218,#236219),(#236220,#236221),
(#236222,#236223),(#236224,#236225),(#236226,#236227),(#236228,#236229),
(#236230,#236231),(#236232,#236233),(#236234,#236235),(#236236,#236237),
(#236238,#236239),(#236240,#236241)),.UNSPECIFIED.,.F.,.F.,.F.)
B_SPLINE_SURFACE_WITH_KNOTS((6,1,1,1,1,1,1,1,1,1,1,1,1,1,1,1,1,1,1,1,1,
1,1,1,1,1,1,1,1,1,1,1,1,1,1,1,1,1,1,1,1,1,1,1,1,1,1,1,1,1,1,1,1,1,1,1,1,
1,1,1,1,1,1,1,1,1,1,1,1,1,1,1,1,1,1,1,1,1,1,1,1,1,1,1,1,1,1,1,1,1,1,1,1,
1,1,1,1,1,1,1,1,1,1,1,1,1,1,1,1,1,1,1,1,1,1,1,1,1,1,1,1,1,1,1,1,1,1,1,1,
1,1,1,1,1,1,1,1,1,1,1,1,1,1,1,1,1,1,1,1,1,1,1,1,1,1,1,1,1,1,1,1,1,1,1,1,
1,1,1,1,1,1,1,1,1,1,1,1,1,1,1,1,1,1,1,1,1,1,1,1,1,1,1,1,1,1,1,1,1,1,1,6),
(2,2),(-1.,-0.995000000000001,-0.990000000000001,-0.985000000000001,-0.980000000000001,
-0.975000000000001,-0.970000000000001,-0.965000000000001,-0.960000000000001,
-0.955000000000001,-0.950000000000001,-0.945000000000001,-0.940000000000001,
-0.935000000000001,-0.930000000000001,-0.925000000000001,-0.920000000000001,
-0.915000000000001,-0.910000000000001,-0.905000000000001,-0.900000000000001,
-0.895000000000001,-0.890000000000001,-0.885000000000001,-0.880000000000001,
-0.875000000000001,-0.870000000000001,-0.865000000000001,-0.860000000000001,
-0.855000000000001,-0.850000000000001,-0.845000000000001,-0.840000000000001,
-0.835000000000001,-0.830000000000001,-0.825000000000001,-0.820000000000001,
-0.815000000000001,-0.810000000000001,-0.805000000000001,-0.800000000000001,
-0.795000000000001,-0.790000000000001,-0.785000000000001,-0.780000000000001,
-0.775000000000001,-0.770000000000001,-0.765000000000001,-0.760000000000001,
-0.755000000000001,-0.750000000000001,-0.745000000000001,-0.740000000000001,
-0.735000000000001,-0.730000000000001,-0.725000000000001,-0.720000000000001,
-0.715000000000001,-0.710000000000001,-0.705000000000001,-0.700000000000001,
-0.695000000000001,-0.690000000000001,-0.685,-0.68,-0.675,-0.67,-0.665,
-0.66,-0.655,-0.65,-0.645,-0.64,-0.635,-0.63,-0.625,-0.62,-0.615,-0.61,
-0.605,-0.6,-0.595,-0.59,-0.585,-0.58,-0.575,-0.57,-0.565,-0.56,-0.555,
-0.55,-0.545,-0.54,-0.535,-0.53,-0.525,-0.52,-0.515,-0.51,-0.505,-0.5,-0.495,
-0.49,-0.485,-0.48,-0.475,-0.47,-0.465,-0.46,-0.455,-0.45,-0.445,-0.44,
-0.435,-0.43,-0.425,-0.42,-0.415,-0.41,-0.405,-0.4,-0.395,-0.39,-0.385,
-0.38,-0.375,-0.37,-0.365,-0.36,-0.355,-0.35,-0.345,-0.34,-0.335,-0.33,
-0.325,-0.32,-0.315,-0.31,-0.305,-0.3,-0.295,-0.29,-0.285,-0.28,-0.275,
-0.27,-0.265,-0.26,-0.255,-0.25,-0.245,-0.24,-0.235,-0.23,-0.225,-0.22,
-0.215,-0.21,-0.205,-0.2,-0.195,-0.19,-0.185,-0.18,-0.175,-0.17,-0.165,
-0.16,-0.155,-0.15,-0.145,-0.14,-0.135,-0.13,-0.125,-0.12,-0.115,-0.11,
-0.105,-0.1,-0.095,-0.09,-0.085,-0.08,-0.075,-0.07,-0.065,-0.06,-0.055,
-0.05,-0.045,-0.04,-0.035,-0.03,-0.025,-0.02,-0.015,-0.01,-0.005,0.),(0.,
1.2),.UNSPECIFIED.)
GEOMETRIC_REPRESENTATION_ITEM()
RATIONAL_B_SPLINE_SURFACE(((1.,1.),(1.,1.),(1.,1.),(1.,1.),(1.,1.),(1.,
1.),(1.,1.),(1.,1.),(1.,1.),(1.,1.),(1.,1.),(1.,1.),(1.,1.),(1.,1.),(1.,
1.),(1.,1.),(1.,1.),(1.,1.),(1.,1.),(1.,1.),(1.,1.),(1.,1.),(1.,1.),(1.,
1.),(1.,1.),(1.,1.),(1.,1.),(1.,1.),(1.,1.),(1.,1.),(1.,1.),(1.,1.),(1.,
1.),(1.,1.),(1.,1.),(1.,1.),(1.,1.),(1.,1.),(1.,1.),(1.,1.),(1.,1.),(1.,
1.),(1.,1.),(1.,1.),(1.,1.),(1.,1.),(1.,1.),(1.,1.),(1.,1.),(1.,1.),(1.,
1.),(1.,1.),(1.,1.),(1.,1.),(1.,1.),(1.,1.),(1.,1.),(1.,1.),(1.,1.),(1.,
1.),(1.,1.),(1.,1.),(1.,1.),(1.,1.),(1.,1.),(1.,1.),(1.,1.),(1.,1.),(1.,
1.),(1.,1.),(1.,1.),(1.,1.),(1.,1.),(1.,1.),(1.,1.),(1.,1.),(1.,1.),(1.,
1.),(1.,1.),(1.,1.),(1.,1.),(1.,1.),(1.,1.),(1.,1.),(1.,1.),(1.,1.),(1.,
1.),(1.,1.),(1.,1.),(1.,1.),(1.,1.),(1.,1.),(1.,1.),(1.,1.),(1.,1.),(1.,
1.),(1.,1.),(1.,1.),(1.,1.),(1.,1.),(1.,1.),(1.,1.),(1.,1.),(1.,1.),(1.,
1.),(1.,1.),(1.,1.),(1.,1.),(1.,1.),(1.,1.),(1.,1.),(1.,1.),(1.,1.),(1.,
1.),(1.,1.),(1.,1.),(1.,1.),(1.,1.),(1.,1.),(1.,1.),(1.,1.),(1.,1.),(1.,
1.),(1.,1.),(1.,1.),(1.,1.),(1.,1.),(1.,1.),(1.,1.),(1.,1.),(1.,1.),(1.,
1.),(1.,1.),(1.,1.),(1.,1.),(1.,1.),(1.,1.),(1.,1.),(1.,1.),(1.,1.),(1.,
1.),(1.,1.),(1.,1.),(1.,1.),(1.,1.),(1.,1.),(1.,1.),(1.,1.),(1.,1.),(1.,
1.),(1.,1.),(1.,1.),(1.,1.),(1.,1.),(1.,1.),(1.,1.),(1.,1.),(1.,1.),(1.,
1.),(1.,1.),(1.,1.),(1.,1.),(1.,1.),(1.,1.),(1.,1.),(1.,1.),(1.,1.),(1.,
1.),(1.,1.),(1.,1.),(1.,1.),(1.,1.),(1.,1.),(1.,1.),(1.,1.),(1.,1.),(1.,
1.),(1.,1.),(1.,1.),(1.,1.),(1.,1.),(1.,1.),(1.,1.),(1.,1.),(1.,1.),(1.,
1.),(1.,1.),(1.,1.),(1.,1.),(1.,1.),(1.,1.),(1.,1.),(1.,1.),(1.,1.),(1.,
1.),(1.,1.),(1.,1.),(1.,1.),(1.,1.),(1.,1.),(1.,1.),(1.,1.),(1.,1.),(1.,
1.),(1.,1.)))
REPRESENTATION_ITEM('')
SURFACE()
);
#1100=(
BOUNDED_SURFACE()
B_SPLINE_SURFACE(5,1,((#236655,#236656),(#236657,#236658),(#236659,#236660),
(#236661,#236662),(#236663,#236664),(#236665,#236666),(#236667,#236668),
(#236669,#236670),(#236671,#236672),(#236673,#236674),(#236675,#236676),
(#236677,#236678),(#236679,#236680),(#236681,#236682),(#236683,#236684),
(#236685,#236686),(#236687,#236688),(#236689,#236690),(#236691,#236692),
(#236693,#236694),(#236695,#236696),(#236697,#236698),(#236699,#236700),
(#236701,#236702),(#236703,#236704),(#236705,#236706),(#236707,#236708),
(#236709,#236710),(#236711,#236712),(#236713,#236714),(#236715,#236716),
(#236717,#236718),(#236719,#236720),(#236721,#236722),(#236723,#236724),
(#236725,#236726),(#236727,#236728),(#236729,#236730),(#236731,#236732),
(#236733,#236734),(#236735,#236736),(#236737,#236738),(#236739,#236740),
(#236741,#236742),(#236743,#236744),(#236745,#236746),(#236747,#236748),
(#236749,#236750),(#236751,#236752),(#236753,#236754),(#236755,#236756),
(#236757,#236758),(#236759,#236760),(#236761,#236762),(#236763,#236764),
(#236765,#236766),(#236767,#236768),(#236769,#236770),(#236771,#236772),
(#236773,#236774),(#236775,#236776),(#236777,#236778),(#236779,#236780),
(#236781,#236782),(#236783,#236784),(#236785,#236786),(#236787,#236788),
(#236789,#236790),(#236791,#236792),(#236793,#236794),(#236795,#236796),
(#236797,#236798),(#236799,#236800),(#236801,#236802),(#236803,#236804),
(#236805,#236806),(#236807,#236808),(#236809,#236810),(#236811,#236812),
(#236813,#236814),(#236815,#236816),(#236817,#236818),(#236819,#236820),
(#236821,#236822),(#236823,#236824),(#236825,#236826),(#236827,#236828),
(#236829,#236830),(#236831,#236832),(#236833,#236834),(#236835,#236836),
(#236837,#236838),(#236839,#236840),(#236841,#236842),(#236843,#236844),
(#236845,#236846),(#236847,#236848),(#236849,#236850),(#236851,#236852),
(#236853,#236854),(#236855,#236856),(#236857,#236858),(#236859,#236860),
(#236861,#236862),(#236863,#236864),(#236865,#236866),(#236867,#236868),
(#236869,#236870),(#236871,#236872),(#236873,#236874),(#236875,#236876),
(#236877,#236878),(#236879,#236880),(#236881,#236882),(#236883,#236884),
(#236885,#236886),(#236887,#236888),(#236889,#236890),(#236891,#236892),
(#236893,#236894),(#236895,#236896),(#236897,#236898),(#236899,#236900),
(#236901,#236902),(#236903,#236904),(#236905,#236906),(#236907,#236908),
(#236909,#236910),(#236911,#236912),(#236913,#236914),(#236915,#236916),
(#236917,#236918),(#236919,#236920),(#236921,#236922),(#236923,#236924),
(#236925,#236926),(#236927,#236928),(#236929,#236930),(#236931,#236932),
(#236933,#236934),(#236935,#236936),(#236937,#236938),(#236939,#236940),
(#236941,#236942),(#236943,#236944),(#236945,#236946),(#236947,#236948),
(#236949,#236950),(#236951,#236952),(#236953,#236954),(#236955,#236956),
(#236957,#236958),(#236959,#236960),(#236961,#236962),(#236963,#236964),
(#236965,#236966),(#236967,#236968),(#236969,#236970),(#236971,#236972),
(#236973,#236974),(#236975,#236976),(#236977,#236978),(#236979,#236980),
(#236981,#236982),(#236983,#236984),(#236985,#236986),(#236987,#236988),
(#236989,#236990),(#236991,#236992),(#236993,#236994),(#236995,#236996),
(#236997,#236998),(#236999,#237000),(#237001,#237002),(#237003,#237004),
(#237005,#237006),(#237007,#237008),(#237009,#237010),(#237011,#237012),
(#237013,#237014),(#237015,#237016),(#237017,#237018),(#237019,#237020),
(#237021,#237022),(#237023,#237024),(#237025,#237026),(#237027,#237028),
(#237029,#237030),(#237031,#237032),(#237033,#237034),(#237035,#237036),
(#237037,#237038),(#237039,#237040),(#237041,#237042),(#237043,#237044),
(#237045,#237046),(#237047,#237048),(#237049,#237050),(#237051,#237052),
(#237053,#237054),(#237055,#237056),(#237057,#237058),(#237059,#237060),
(#237061,#237062),(#237063,#237064)),.UNSPECIFIED.,.F.,.F.,.F.)
B_SPLINE_SURFACE_WITH_KNOTS((6,1,1,1,1,1,1,1,1,1,1,1,1,1,1,1,1,1,1,1,1,
1,1,1,1,1,1,1,1,1,1,1,1,1,1,1,1,1,1,1,1,1,1,1,1,1,1,1,1,1,1,1,1,1,1,1,1,
1,1,1,1,1,1,1,1,1,1,1,1,1,1,1,1,1,1,1,1,1,1,1,1,1,1,1,1,1,1,1,1,1,1,1,1,
1,1,1,1,1,1,1,1,1,1,1,1,1,1,1,1,1,1,1,1,1,1,1,1,1,1,1,1,1,1,1,1,1,1,1,1,
1,1,1,1,1,1,1,1,1,1,1,1,1,1,1,1,1,1,1,1,1,1,1,1,1,1,1,1,1,1,1,1,1,1,1,1,
1,1,1,1,1,1,1,1,1,1,1,1,1,1,1,1,1,1,1,1,1,1,1,1,1,1,1,1,1,1,1,1,1,1,1,6),
(2,2),(0.,0.005,0.01,0.015,0.02,0.025,0.03,0.035,0.04,0.045,0.05,0.055,
0.06,0.065,0.07,0.075,0.08,0.085,0.09,0.095,0.1,0.105,0.11,0.115,0.12,0.125,
0.13,0.135,0.14,0.145,0.15,0.155,0.16,0.165,0.17,0.175,0.18,0.185,0.19,
0.195,0.2,0.205,0.21,0.215,0.22,0.225,0.23,0.235,0.24,0.245,0.25,0.255,
0.26,0.265,0.27,0.275,0.28,0.285,0.29,0.295,0.3,0.305,0.31,0.315,0.32,0.325,
0.33,0.335,0.34,0.345,0.35,0.355,0.36,0.365,0.37,0.375,0.38,0.385,0.39,
0.395,0.4,0.405,0.41,0.415,0.42,0.425,0.43,0.435,0.44,0.445,0.45,0.455,
0.46,0.465,0.47,0.475,0.48,0.485,0.49,0.495,0.5,0.505,0.51,0.515,0.52,0.525,
0.53,0.535,0.54,0.545,0.55,0.555,0.56,0.565,0.57,0.575,0.58,0.585,0.59,
0.595,0.6,0.605,0.61,0.615,0.62,0.625,0.63,0.635,0.64,0.645,0.65,0.655,
0.66,0.665,0.67,0.675,0.68,0.685,0.690000000000001,0.695000000000001,0.700000000000001,
0.705000000000001,0.710000000000001,0.715000000000001,0.720000000000001,
0.725000000000001,0.730000000000001,0.735000000000001,0.740000000000001,
0.745000000000001,0.750000000000001,0.755000000000001,0.760000000000001,
0.765000000000001,0.770000000000001,0.775000000000001,0.780000000000001,
0.785000000000001,0.790000000000001,0.795000000000001,0.800000000000001,
0.805000000000001,0.810000000000001,0.815000000000001,0.820000000000001,
0.825000000000001,0.830000000000001,0.835000000000001,0.840000000000001,
0.845000000000001,0.850000000000001,0.855000000000001,0.860000000000001,
0.865000000000001,0.870000000000001,0.875000000000001,0.880000000000001,
0.885000000000001,0.890000000000001,0.895000000000001,0.900000000000001,
0.905000000000001,0.910000000000001,0.915000000000001,0.920000000000001,
0.925000000000001,0.930000000000001,0.935000000000001,0.940000000000001,
0.945000000000001,0.950000000000001,0.955000000000001,0.960000000000001,
0.965000000000001,0.970000000000001,0.975000000000001,0.980000000000001,
0.985000000000001,0.990000000000001,0.995000000000001,1.),(0.,1.2),
 .UNSPECIFIED.)
GEOMETRIC_REPRESENTATION_ITEM()
RATIONAL_B_SPLINE_SURFACE(((1.,1.),(1.,1.),(1.,1.),(1.,1.),(1.,1.),(1.,
1.),(1.,1.),(1.,1.),(1.,1.),(1.,1.),(1.,1.),(1.,1.),(1.,1.),(1.,1.),(1.,
1.),(1.,1.),(1.,1.),(1.,1.),(1.,1.),(1.,1.),(1.,1.),(1.,1.),(1.,1.),(1.,
1.),(1.,1.),(1.,1.),(1.,1.),(1.,1.),(1.,1.),(1.,1.),(1.,1.),(1.,1.),(1.,
1.),(1.,1.),(1.,1.),(1.,1.),(1.,1.),(1.,1.),(1.,1.),(1.,1.),(1.,1.),(1.,
1.),(1.,1.),(1.,1.),(1.,1.),(1.,1.),(1.,1.),(1.,1.),(1.,1.),(1.,1.),(1.,
1.),(1.,1.),(1.,1.),(1.,1.),(1.,1.),(1.,1.),(1.,1.),(1.,1.),(1.,1.),(1.,
1.),(1.,1.),(1.,1.),(1.,1.),(1.,1.),(1.,1.),(1.,1.),(1.,1.),(1.,1.),(1.,
1.),(1.,1.),(1.,1.),(1.,1.),(1.,1.),(1.,1.),(1.,1.),(1.,1.),(1.,1.),(1.,
1.),(1.,1.),(1.,1.),(1.,1.),(1.,1.),(1.,1.),(1.,1.),(1.,1.),(1.,1.),(1.,
1.),(1.,1.),(1.,1.),(1.,1.),(1.,1.),(1.,1.),(1.,1.),(1.,1.),(1.,1.),(1.,
1.),(1.,1.),(1.,1.),(1.,1.),(1.,1.),(1.,1.),(1.,1.),(1.,1.),(1.,1.),(1.,
1.),(1.,1.),(1.,1.),(1.,1.),(1.,1.),(1.,1.),(1.,1.),(1.,1.),(1.,1.),(1.,
1.),(1.,1.),(1.,1.),(1.,1.),(1.,1.),(1.,1.),(1.,1.),(1.,1.),(1.,1.),(1.,
1.),(1.,1.),(1.,1.),(1.,1.),(1.,1.),(1.,1.),(1.,1.),(1.,1.),(1.,1.),(1.,
1.),(1.,1.),(1.,1.),(1.,1.),(1.,1.),(1.,1.),(1.,1.),(1.,1.),(1.,1.),(1.,
1.),(1.,1.),(1.,1.),(1.,1.),(1.,1.),(1.,1.),(1.,1.),(1.,1.),(1.,1.),(1.,
1.),(1.,1.),(1.,1.),(1.,1.),(1.,1.),(1.,1.),(1.,1.),(1.,1.),(1.,1.),(1.,
1.),(1.,1.),(1.,1.),(1.,1.),(1.,1.),(1.,1.),(1.,1.),(1.,1.),(1.,1.),(1.,
1.),(1.,1.),(1.,1.),(1.,1.),(1.,1.),(1.,1.),(1.,1.),(1.,1.),(1.,1.),(1.,
1.),(1.,1.),(1.,1.),(1.,1.),(1.,1.),(1.,1.),(1.,1.),(1.,1.),(1.,1.),(1.,
1.),(1.,1.),(1.,1.),(1.,1.),(1.,1.),(1.,1.),(1.,1.),(1.,1.),(1.,1.),(1.,
1.),(1.,1.),(1.,1.),(1.,1.),(1.,1.),(1.,1.),(1.,1.),(1.,1.),(1.,1.),(1.,
1.),(1.,1.)))
REPRESENTATION_ITEM('')
SURFACE()
);
#1101=(
BOUNDED_SURFACE()
B_SPLINE_SURFACE(5,1,((#237484,#237485),(#237486,#237487),(#237488,#237489),
(#237490,#237491),(#237492,#237493),(#237494,#237495),(#237496,#237497),
(#237498,#237499),(#237500,#237501),(#237502,#237503),(#237504,#237505),
(#237506,#237507),(#237508,#237509),(#237510,#237511),(#237512,#237513),
(#237514,#237515),(#237516,#237517),(#237518,#237519),(#237520,#237521),
(#237522,#237523),(#237524,#237525),(#237526,#237527),(#237528,#237529),
(#237530,#237531),(#237532,#237533),(#237534,#237535),(#237536,#237537),
(#237538,#237539),(#237540,#237541),(#237542,#237543),(#237544,#237545),
(#237546,#237547),(#237548,#237549),(#237550,#237551),(#237552,#237553),
(#237554,#237555),(#237556,#237557),(#237558,#237559),(#237560,#237561),
(#237562,#237563),(#237564,#237565),(#237566,#237567),(#237568,#237569),
(#237570,#237571),(#237572,#237573),(#237574,#237575),(#237576,#237577),
(#237578,#237579),(#237580,#237581),(#237582,#237583),(#237584,#237585),
(#237586,#237587),(#237588,#237589),(#237590,#237591),(#237592,#237593),
(#237594,#237595),(#237596,#237597),(#237598,#237599),(#237600,#237601),
(#237602,#237603),(#237604,#237605),(#237606,#237607),(#237608,#237609),
(#237610,#237611),(#237612,#237613),(#237614,#237615),(#237616,#237617),
(#237618,#237619),(#237620,#237621),(#237622,#237623),(#237624,#237625),
(#237626,#237627),(#237628,#237629),(#237630,#237631),(#237632,#237633),
(#237634,#237635),(#237636,#237637),(#237638,#237639),(#237640,#237641),
(#237642,#237643),(#237644,#237645),(#237646,#237647),(#237648,#237649),
(#237650,#237651),(#237652,#237653),(#237654,#237655),(#237656,#237657),
(#237658,#237659),(#237660,#237661),(#237662,#237663),(#237664,#237665),
(#237666,#237667),(#237668,#237669),(#237670,#237671),(#237672,#237673),
(#237674,#237675),(#237676,#237677),(#237678,#237679),(#237680,#237681),
(#237682,#237683),(#237684,#237685),(#237686,#237687),(#237688,#237689),
(#237690,#237691),(#237692,#237693),(#237694,#237695),(#237696,#237697),
(#237698,#237699),(#237700,#237701),(#237702,#237703),(#237704,#237705),
(#237706,#237707),(#237708,#237709),(#237710,#237711),(#237712,#237713),
(#237714,#237715),(#237716,#237717),(#237718,#237719),(#237720,#237721),
(#237722,#237723),(#237724,#237725),(#237726,#237727),(#237728,#237729),
(#237730,#237731),(#237732,#237733),(#237734,#237735),(#237736,#237737),
(#237738,#237739),(#237740,#237741),(#237742,#237743),(#237744,#237745),
(#237746,#237747),(#237748,#237749),(#237750,#237751),(#237752,#237753),
(#237754,#237755),(#237756,#237757),(#237758,#237759),(#237760,#237761),
(#237762,#237763),(#237764,#237765),(#237766,#237767),(#237768,#237769),
(#237770,#237771),(#237772,#237773),(#237774,#237775),(#237776,#237777),
(#237778,#237779),(#237780,#237781),(#237782,#237783),(#237784,#237785),
(#237786,#237787),(#237788,#237789),(#237790,#237791),(#237792,#237793),
(#237794,#237795),(#237796,#237797),(#237798,#237799),(#237800,#237801),
(#237802,#237803),(#237804,#237805),(#237806,#237807),(#237808,#237809),
(#237810,#237811),(#237812,#237813),(#237814,#237815),(#237816,#237817),
(#237818,#237819),(#237820,#237821),(#237822,#237823),(#237824,#237825),
(#237826,#237827),(#237828,#237829),(#237830,#237831),(#237832,#237833),
(#237834,#237835),(#237836,#237837),(#237838,#237839),(#237840,#237841),
(#237842,#237843),(#237844,#237845),(#237846,#237847),(#237848,#237849),
(#237850,#237851),(#237852,#237853),(#237854,#237855),(#237856,#237857),
(#237858,#237859),(#237860,#237861),(#237862,#237863),(#237864,#237865),
(#237866,#237867),(#237868,#237869),(#237870,#237871),(#237872,#237873),
(#237874,#237875),(#237876,#237877),(#237878,#237879),(#237880,#237881),
(#237882,#237883),(#237884,#237885),(#237886,#237887),(#237888,#237889),
(#237890,#237891),(#237892,#237893)),.UNSPECIFIED.,.F.,.F.,.F.)
B_SPLINE_SURFACE_WITH_KNOTS((6,1,1,1,1,1,1,1,1,1,1,1,1,1,1,1,1,1,1,1,1,
1,1,1,1,1,1,1,1,1,1,1,1,1,1,1,1,1,1,1,1,1,1,1,1,1,1,1,1,1,1,1,1,1,1,1,1,
1,1,1,1,1,1,1,1,1,1,1,1,1,1,1,1,1,1,1,1,1,1,1,1,1,1,1,1,1,1,1,1,1,1,1,1,
1,1,1,1,1,1,1,1,1,1,1,1,1,1,1,1,1,1,1,1,1,1,1,1,1,1,1,1,1,1,1,1,1,1,1,1,
1,1,1,1,1,1,1,1,1,1,1,1,1,1,1,1,1,1,1,1,1,1,1,1,1,1,1,1,1,1,1,1,1,1,1,1,
1,1,1,1,1,1,1,1,1,1,1,1,1,1,1,1,1,1,1,1,1,1,1,1,1,1,1,1,1,1,1,1,1,1,1,6),
(2,2),(-1.,-0.995000000000001,-0.990000000000001,-0.985000000000001,-0.980000000000001,
-0.975000000000001,-0.970000000000001,-0.965000000000001,-0.960000000000001,
-0.955000000000001,-0.950000000000001,-0.945000000000001,-0.940000000000001,
-0.935000000000001,-0.930000000000001,-0.925000000000001,-0.920000000000001,
-0.915000000000001,-0.910000000000001,-0.905000000000001,-0.900000000000001,
-0.895000000000001,-0.890000000000001,-0.885000000000001,-0.880000000000001,
-0.875000000000001,-0.870000000000001,-0.865000000000001,-0.860000000000001,
-0.855000000000001,-0.850000000000001,-0.845000000000001,-0.840000000000001,
-0.835000000000001,-0.830000000000001,-0.825000000000001,-0.820000000000001,
-0.815000000000001,-0.810000000000001,-0.805000000000001,-0.800000000000001,
-0.795000000000001,-0.790000000000001,-0.785000000000001,-0.780000000000001,
-0.775000000000001,-0.770000000000001,-0.765000000000001,-0.760000000000001,
-0.755000000000001,-0.750000000000001,-0.745000000000001,-0.740000000000001,
-0.735000000000001,-0.730000000000001,-0.725000000000001,-0.720000000000001,
-0.715000000000001,-0.710000000000001,-0.705000000000001,-0.700000000000001,
-0.695000000000001,-0.690000000000001,-0.685,-0.68,-0.675,-0.67,-0.665,
-0.66,-0.655,-0.65,-0.645,-0.64,-0.635,-0.63,-0.625,-0.62,-0.615,-0.61,
-0.605,-0.6,-0.595,-0.59,-0.585,-0.58,-0.575,-0.57,-0.565,-0.56,-0.555,
-0.55,-0.545,-0.54,-0.535,-0.53,-0.525,-0.52,-0.515,-0.51,-0.505,-0.5,-0.495,
-0.49,-0.485,-0.48,-0.475,-0.47,-0.465,-0.46,-0.455,-0.45,-0.445,-0.44,
-0.435,-0.43,-0.425,-0.42,-0.415,-0.41,-0.405,-0.4,-0.395,-0.39,-0.385,
-0.38,-0.375,-0.37,-0.365,-0.36,-0.355,-0.35,-0.345,-0.34,-0.335,-0.33,
-0.325,-0.32,-0.315,-0.31,-0.305,-0.3,-0.295,-0.29,-0.285,-0.28,-0.275,
-0.27,-0.265,-0.26,-0.255,-0.25,-0.245,-0.24,-0.235,-0.23,-0.225,-0.22,
-0.215,-0.21,-0.205,-0.2,-0.195,-0.19,-0.185,-0.18,-0.175,-0.17,-0.165,
-0.16,-0.155,-0.15,-0.145,-0.14,-0.135,-0.13,-0.125,-0.12,-0.115,-0.11,
-0.105,-0.1,-0.095,-0.09,-0.085,-0.08,-0.075,-0.07,-0.065,-0.06,-0.055,
-0.05,-0.045,-0.04,-0.035,-0.03,-0.025,-0.02,-0.015,-0.01,-0.005,0.),(0.,
1.2),.UNSPECIFIED.)
GEOMETRIC_REPRESENTATION_ITEM()
RATIONAL_B_SPLINE_SURFACE(((1.,1.),(1.,1.),(1.,1.),(1.,1.),(1.,1.),(1.,
1.),(1.,1.),(1.,1.),(1.,1.),(1.,1.),(1.,1.),(1.,1.),(1.,1.),(1.,1.),(1.,
1.),(1.,1.),(1.,1.),(1.,1.),(1.,1.),(1.,1.),(1.,1.),(1.,1.),(1.,1.),(1.,
1.),(1.,1.),(1.,1.),(1.,1.),(1.,1.),(1.,1.),(1.,1.),(1.,1.),(1.,1.),(1.,
1.),(1.,1.),(1.,1.),(1.,1.),(1.,1.),(1.,1.),(1.,1.),(1.,1.),(1.,1.),(1.,
1.),(1.,1.),(1.,1.),(1.,1.),(1.,1.),(1.,1.),(1.,1.),(1.,1.),(1.,1.),(1.,
1.),(1.,1.),(1.,1.),(1.,1.),(1.,1.),(1.,1.),(1.,1.),(1.,1.),(1.,1.),(1.,
1.),(1.,1.),(1.,1.),(1.,1.),(1.,1.),(1.,1.),(1.,1.),(1.,1.),(1.,1.),(1.,
1.),(1.,1.),(1.,1.),(1.,1.),(1.,1.),(1.,1.),(1.,1.),(1.,1.),(1.,1.),(1.,
1.),(1.,1.),(1.,1.),(1.,1.),(1.,1.),(1.,1.),(1.,1.),(1.,1.),(1.,1.),(1.,
1.),(1.,1.),(1.,1.),(1.,1.),(1.,1.),(1.,1.),(1.,1.),(1.,1.),(1.,1.),(1.,
1.),(1.,1.),(1.,1.),(1.,1.),(1.,1.),(1.,1.),(1.,1.),(1.,1.),(1.,1.),(1.,
1.),(1.,1.),(1.,1.),(1.,1.),(1.,1.),(1.,1.),(1.,1.),(1.,1.),(1.,1.),(1.,
1.),(1.,1.),(1.,1.),(1.,1.),(1.,1.),(1.,1.),(1.,1.),(1.,1.),(1.,1.),(1.,
1.),(1.,1.),(1.,1.),(1.,1.),(1.,1.),(1.,1.),(1.,1.),(1.,1.),(1.,1.),(1.,
1.),(1.,1.),(1.,1.),(1.,1.),(1.,1.),(1.,1.),(1.,1.),(1.,1.),(1.,1.),(1.,
1.),(1.,1.),(1.,1.),(1.,1.),(1.,1.),(1.,1.),(1.,1.),(1.,1.),(1.,1.),(1.,
1.),(1.,1.),(1.,1.),(1.,1.),(1.,1.),(1.,1.),(1.,1.),(1.,1.),(1.,1.),(1.,
1.),(1.,1.),(1.,1.),(1.,1.),(1.,1.),(1.,1.),(1.,1.),(1.,1.),(1.,1.),(1.,
1.),(1.,1.),(1.,1.),(1.,1.),(1.,1.),(1.,1.),(1.,1.),(1.,1.),(1.,1.),(1.,
1.),(1.,1.),(1.,1.),(1.,1.),(1.,1.),(1.,1.),(1.,1.),(1.,1.),(1.,1.),(1.,
1.),(1.,1.),(1.,1.),(1.,1.),(1.,1.),(1.,1.),(1.,1.),(1.,1.),(1.,1.),(1.,
1.),(1.,1.),(1.,1.),(1.,1.),(1.,1.),(1.,1.),(1.,1.),(1.,1.),(1.,1.),(1.,
1.),(1.,1.)))
REPRESENTATION_ITEM('')
SURFACE()
);
#1102=(
BOUNDED_SURFACE()
B_SPLINE_SURFACE(5,1,((#238307,#238308),(#238309,#238310),(#238311,#238312),
(#238313,#238314),(#238315,#238316),(#238317,#238318),(#238319,#238320),
(#238321,#238322),(#238323,#238324),(#238325,#238326),(#238327,#238328),
(#238329,#238330),(#238331,#238332),(#238333,#238334),(#238335,#238336),
(#238337,#238338),(#238339,#238340),(#238341,#238342),(#238343,#238344),
(#238345,#238346),(#238347,#238348),(#238349,#238350),(#238351,#238352),
(#238353,#238354),(#238355,#238356),(#238357,#238358),(#238359,#238360),
(#238361,#238362),(#238363,#238364),(#238365,#238366),(#238367,#238368),
(#238369,#238370),(#238371,#238372),(#238373,#238374),(#238375,#238376),
(#238377,#238378),(#238379,#238380),(#238381,#238382),(#238383,#238384),
(#238385,#238386),(#238387,#238388),(#238389,#238390),(#238391,#238392),
(#238393,#238394),(#238395,#238396),(#238397,#238398),(#238399,#238400),
(#238401,#238402),(#238403,#238404),(#238405,#238406),(#238407,#238408),
(#238409,#238410),(#238411,#238412),(#238413,#238414),(#238415,#238416),
(#238417,#238418),(#238419,#238420),(#238421,#238422),(#238423,#238424),
(#238425,#238426),(#238427,#238428),(#238429,#238430),(#238431,#238432),
(#238433,#238434),(#238435,#238436),(#238437,#238438),(#238439,#238440),
(#238441,#238442),(#238443,#238444),(#238445,#238446),(#238447,#238448),
(#238449,#238450),(#238451,#238452),(#238453,#238454),(#238455,#238456),
(#238457,#238458),(#238459,#238460),(#238461,#238462),(#238463,#238464),
(#238465,#238466),(#238467,#238468),(#238469,#238470),(#238471,#238472),
(#238473,#238474),(#238475,#238476),(#238477,#238478),(#238479,#238480),
(#238481,#238482),(#238483,#238484),(#238485,#238486),(#238487,#238488),
(#238489,#238490),(#238491,#238492),(#238493,#238494),(#238495,#238496),
(#238497,#238498),(#238499,#238500),(#238501,#238502),(#238503,#238504),
(#238505,#238506),(#238507,#238508),(#238509,#238510),(#238511,#238512),
(#238513,#238514),(#238515,#238516),(#238517,#238518),(#238519,#238520),
(#238521,#238522),(#238523,#238524),(#238525,#238526),(#238527,#238528),
(#238529,#238530),(#238531,#238532),(#238533,#238534),(#238535,#238536),
(#238537,#238538),(#238539,#238540),(#238541,#238542),(#238543,#238544),
(#238545,#238546),(#238547,#238548),(#238549,#238550),(#238551,#238552),
(#238553,#238554),(#238555,#238556),(#238557,#238558),(#238559,#238560),
(#238561,#238562),(#238563,#238564),(#238565,#238566),(#238567,#238568),
(#238569,#238570),(#238571,#238572),(#238573,#238574),(#238575,#238576),
(#238577,#238578),(#238579,#238580),(#238581,#238582),(#238583,#238584),
(#238585,#238586),(#238587,#238588),(#238589,#238590),(#238591,#238592),
(#238593,#238594),(#238595,#238596),(#238597,#238598),(#238599,#238600),
(#238601,#238602),(#238603,#238604),(#238605,#238606),(#238607,#238608),
(#238609,#238610),(#238611,#238612),(#238613,#238614),(#238615,#238616),
(#238617,#238618),(#238619,#238620),(#238621,#238622),(#238623,#238624),
(#238625,#238626),(#238627,#238628),(#238629,#238630),(#238631,#238632),
(#238633,#238634),(#238635,#238636),(#238637,#238638),(#238639,#238640),
(#238641,#238642),(#238643,#238644),(#238645,#238646),(#238647,#238648),
(#238649,#238650),(#238651,#238652),(#238653,#238654),(#238655,#238656),
(#238657,#238658),(#238659,#238660),(#238661,#238662),(#238663,#238664),
(#238665,#238666),(#238667,#238668),(#238669,#238670),(#238671,#238672),
(#238673,#238674),(#238675,#238676),(#238677,#238678),(#238679,#238680),
(#238681,#238682),(#238683,#238684),(#238685,#238686),(#238687,#238688),
(#238689,#238690),(#238691,#238692),(#238693,#238694),(#238695,#238696),
(#238697,#238698),(#238699,#238700),(#238701,#238702),(#238703,#238704),
(#238705,#238706),(#238707,#238708),(#238709,#238710),(#238711,#238712),
(#238713,#238714),(#238715,#238716)),.UNSPECIFIED.,.F.,.F.,.F.)
B_SPLINE_SURFACE_WITH_KNOTS((6,1,1,1,1,1,1,1,1,1,1,1,1,1,1,1,1,1,1,1,1,
1,1,1,1,1,1,1,1,1,1,1,1,1,1,1,1,1,1,1,1,1,1,1,1,1,1,1,1,1,1,1,1,1,1,1,1,
1,1,1,1,1,1,1,1,1,1,1,1,1,1,1,1,1,1,1,1,1,1,1,1,1,1,1,1,1,1,1,1,1,1,1,1,
1,1,1,1,1,1,1,1,1,1,1,1,1,1,1,1,1,1,1,1,1,1,1,1,1,1,1,1,1,1,1,1,1,1,1,1,
1,1,1,1,1,1,1,1,1,1,1,1,1,1,1,1,1,1,1,1,1,1,1,1,1,1,1,1,1,1,1,1,1,1,1,1,
1,1,1,1,1,1,1,1,1,1,1,1,1,1,1,1,1,1,1,1,1,1,1,1,1,1,1,1,1,1,1,1,1,1,1,6),
(2,2),(0.,0.005,0.01,0.015,0.02,0.025,0.03,0.035,0.04,0.045,0.05,0.055,
0.06,0.065,0.07,0.075,0.08,0.085,0.09,0.095,0.1,0.105,0.11,0.115,0.12,0.125,
0.13,0.135,0.14,0.145,0.15,0.155,0.16,0.165,0.17,0.175,0.18,0.185,0.19,
0.195,0.2,0.205,0.21,0.215,0.22,0.225,0.23,0.235,0.24,0.245,0.25,0.255,
0.26,0.265,0.27,0.275,0.28,0.285,0.29,0.295,0.3,0.305,0.31,0.315,0.32,0.325,
0.33,0.335,0.34,0.345,0.35,0.355,0.36,0.365,0.37,0.375,0.38,0.385,0.39,
0.395,0.4,0.405,0.41,0.415,0.42,0.425,0.43,0.435,0.44,0.445,0.45,0.455,
0.46,0.465,0.47,0.475,0.48,0.485,0.49,0.495,0.5,0.505,0.51,0.515,0.52,0.525,
0.53,0.535,0.54,0.545,0.55,0.555,0.56,0.565,0.57,0.575,0.58,0.585,0.59,
0.595,0.6,0.605,0.61,0.615,0.62,0.625,0.63,0.635,0.64,0.645,0.65,0.655,
0.66,0.665,0.67,0.675,0.68,0.685,0.690000000000001,0.695000000000001,0.700000000000001,
0.705000000000001,0.710000000000001,0.715000000000001,0.720000000000001,
0.725000000000001,0.730000000000001,0.735000000000001,0.740000000000001,
0.745000000000001,0.750000000000001,0.755000000000001,0.760000000000001,
0.765000000000001,0.770000000000001,0.775000000000001,0.780000000000001,
0.785000000000001,0.790000000000001,0.795000000000001,0.800000000000001,
0.805000000000001,0.810000000000001,0.815000000000001,0.820000000000001,
0.825000000000001,0.830000000000001,0.835000000000001,0.840000000000001,
0.845000000000001,0.850000000000001,0.855000000000001,0.860000000000001,
0.865000000000001,0.870000000000001,0.875000000000001,0.880000000000001,
0.885000000000001,0.890000000000001,0.895000000000001,0.900000000000001,
0.905000000000001,0.910000000000001,0.915000000000001,0.920000000000001,
0.925000000000001,0.930000000000001,0.935000000000001,0.940000000000001,
0.945000000000001,0.950000000000001,0.955000000000001,0.960000000000001,
0.965000000000001,0.970000000000001,0.975000000000001,0.980000000000001,
0.985000000000001,0.990000000000001,0.995000000000001,1.),(0.,1.2),
 .UNSPECIFIED.)
GEOMETRIC_REPRESENTATION_ITEM()
RATIONAL_B_SPLINE_SURFACE(((1.,1.),(1.,1.),(1.,1.),(1.,1.),(1.,1.),(1.,
1.),(1.,1.),(1.,1.),(1.,1.),(1.,1.),(1.,1.),(1.,1.),(1.,1.),(1.,1.),(1.,
1.),(1.,1.),(1.,1.),(1.,1.),(1.,1.),(1.,1.),(1.,1.),(1.,1.),(1.,1.),(1.,
1.),(1.,1.),(1.,1.),(1.,1.),(1.,1.),(1.,1.),(1.,1.),(1.,1.),(1.,1.),(1.,
1.),(1.,1.),(1.,1.),(1.,1.),(1.,1.),(1.,1.),(1.,1.),(1.,1.),(1.,1.),(1.,
1.),(1.,1.),(1.,1.),(1.,1.),(1.,1.),(1.,1.),(1.,1.),(1.,1.),(1.,1.),(1.,
1.),(1.,1.),(1.,1.),(1.,1.),(1.,1.),(1.,1.),(1.,1.),(1.,1.),(1.,1.),(1.,
1.),(1.,1.),(1.,1.),(1.,1.),(1.,1.),(1.,1.),(1.,1.),(1.,1.),(1.,1.),(1.,
1.),(1.,1.),(1.,1.),(1.,1.),(1.,1.),(1.,1.),(1.,1.),(1.,1.),(1.,1.),(1.,
1.),(1.,1.),(1.,1.),(1.,1.),(1.,1.),(1.,1.),(1.,1.),(1.,1.),(1.,1.),(1.,
1.),(1.,1.),(1.,1.),(1.,1.),(1.,1.),(1.,1.),(1.,1.),(1.,1.),(1.,1.),(1.,
1.),(1.,1.),(1.,1.),(1.,1.),(1.,1.),(1.,1.),(1.,1.),(1.,1.),(1.,1.),(1.,
1.),(1.,1.),(1.,1.),(1.,1.),(1.,1.),(1.,1.),(1.,1.),(1.,1.),(1.,1.),(1.,
1.),(1.,1.),(1.,1.),(1.,1.),(1.,1.),(1.,1.),(1.,1.),(1.,1.),(1.,1.),(1.,
1.),(1.,1.),(1.,1.),(1.,1.),(1.,1.),(1.,1.),(1.,1.),(1.,1.),(1.,1.),(1.,
1.),(1.,1.),(1.,1.),(1.,1.),(1.,1.),(1.,1.),(1.,1.),(1.,1.),(1.,1.),(1.,
1.),(1.,1.),(1.,1.),(1.,1.),(1.,1.),(1.,1.),(1.,1.),(1.,1.),(1.,1.),(1.,
1.),(1.,1.),(1.,1.),(1.,1.),(1.,1.),(1.,1.),(1.,1.),(1.,1.),(1.,1.),(1.,
1.),(1.,1.),(1.,1.),(1.,1.),(1.,1.),(1.,1.),(1.,1.),(1.,1.),(1.,1.),(1.,
1.),(1.,1.),(1.,1.),(1.,1.),(1.,1.),(1.,1.),(1.,1.),(1.,1.),(1.,1.),(1.,
1.),(1.,1.),(1.,1.),(1.,1.),(1.,1.),(1.,1.),(1.,1.),(1.,1.),(1.,1.),(1.,
1.),(1.,1.),(1.,1.),(1.,1.),(1.,1.),(1.,1.),(1.,1.),(1.,1.),(1.,1.),(1.,
1.),(1.,1.),(1.,1.),(1.,1.),(1.,1.),(1.,1.),(1.,1.),(1.,1.),(1.,1.),(1.,
1.),(1.,1.)))
REPRESENTATION_ITEM('')
SURFACE()
);
#1103=(
BOUNDED_SURFACE()
B_SPLINE_SURFACE(5,1,((#239136,#239137),(#239138,#239139),(#239140,#239141),
(#239142,#239143),(#239144,#239145),(#239146,#239147),(#239148,#239149),
(#239150,#239151),(#239152,#239153),(#239154,#239155),(#239156,#239157),
(#239158,#239159),(#239160,#239161),(#239162,#239163),(#239164,#239165),
(#239166,#239167),(#239168,#239169),(#239170,#239171),(#239172,#239173),
(#239174,#239175),(#239176,#239177),(#239178,#239179),(#239180,#239181),
(#239182,#239183),(#239184,#239185),(#239186,#239187),(#239188,#239189),
(#239190,#239191),(#239192,#239193),(#239194,#239195),(#239196,#239197),
(#239198,#239199),(#239200,#239201),(#239202,#239203),(#239204,#239205),
(#239206,#239207),(#239208,#239209),(#239210,#239211),(#239212,#239213),
(#239214,#239215),(#239216,#239217),(#239218,#239219),(#239220,#239221),
(#239222,#239223),(#239224,#239225),(#239226,#239227),(#239228,#239229),
(#239230,#239231),(#239232,#239233),(#239234,#239235),(#239236,#239237),
(#239238,#239239),(#239240,#239241),(#239242,#239243),(#239244,#239245),
(#239246,#239247),(#239248,#239249),(#239250,#239251),(#239252,#239253),
(#239254,#239255),(#239256,#239257),(#239258,#239259),(#239260,#239261),
(#239262,#239263),(#239264,#239265),(#239266,#239267),(#239268,#239269),
(#239270,#239271),(#239272,#239273),(#239274,#239275),(#239276,#239277),
(#239278,#239279),(#239280,#239281),(#239282,#239283),(#239284,#239285),
(#239286,#239287),(#239288,#239289),(#239290,#239291),(#239292,#239293),
(#239294,#239295),(#239296,#239297),(#239298,#239299),(#239300,#239301),
(#239302,#239303),(#239304,#239305),(#239306,#239307),(#239308,#239309),
(#239310,#239311),(#239312,#239313),(#239314,#239315),(#239316,#239317),
(#239318,#239319),(#239320,#239321),(#239322,#239323),(#239324,#239325),
(#239326,#239327),(#239328,#239329),(#239330,#239331),(#239332,#239333),
(#239334,#239335),(#239336,#239337),(#239338,#239339),(#239340,#239341),
(#239342,#239343),(#239344,#239345),(#239346,#239347),(#239348,#239349),
(#239350,#239351),(#239352,#239353),(#239354,#239355),(#239356,#239357),
(#239358,#239359),(#239360,#239361),(#239362,#239363),(#239364,#239365),
(#239366,#239367),(#239368,#239369),(#239370,#239371),(#239372,#239373),
(#239374,#239375),(#239376,#239377),(#239378,#239379),(#239380,#239381),
(#239382,#239383),(#239384,#239385),(#239386,#239387),(#239388,#239389),
(#239390,#239391),(#239392,#239393),(#239394,#239395),(#239396,#239397),
(#239398,#239399),(#239400,#239401),(#239402,#239403),(#239404,#239405),
(#239406,#239407),(#239408,#239409),(#239410,#239411),(#239412,#239413),
(#239414,#239415),(#239416,#239417),(#239418,#239419),(#239420,#239421),
(#239422,#239423),(#239424,#239425),(#239426,#239427),(#239428,#239429),
(#239430,#239431),(#239432,#239433),(#239434,#239435),(#239436,#239437),
(#239438,#239439),(#239440,#239441),(#239442,#239443),(#239444,#239445),
(#239446,#239447),(#239448,#239449),(#239450,#239451),(#239452,#239453),
(#239454,#239455),(#239456,#239457),(#239458,#239459),(#239460,#239461),
(#239462,#239463),(#239464,#239465),(#239466,#239467),(#239468,#239469),
(#239470,#239471),(#239472,#239473),(#239474,#239475),(#239476,#239477),
(#239478,#239479),(#239480,#239481),(#239482,#239483),(#239484,#239485),
(#239486,#239487),(#239488,#239489),(#239490,#239491),(#239492,#239493),
(#239494,#239495),(#239496,#239497),(#239498,#239499),(#239500,#239501),
(#239502,#239503),(#239504,#239505),(#239506,#239507),(#239508,#239509),
(#239510,#239511),(#239512,#239513),(#239514,#239515),(#239516,#239517),
(#239518,#239519),(#239520,#239521),(#239522,#239523),(#239524,#239525),
(#239526,#239527),(#239528,#239529),(#239530,#239531),(#239532,#239533),
(#239534,#239535),(#239536,#239537),(#239538,#239539),(#239540,#239541),
(#239542,#239543),(#239544,#239545)),.UNSPECIFIED.,.F.,.F.,.F.)
B_SPLINE_SURFACE_WITH_KNOTS((6,1,1,1,1,1,1,1,1,1,1,1,1,1,1,1,1,1,1,1,1,
1,1,1,1,1,1,1,1,1,1,1,1,1,1,1,1,1,1,1,1,1,1,1,1,1,1,1,1,1,1,1,1,1,1,1,1,
1,1,1,1,1,1,1,1,1,1,1,1,1,1,1,1,1,1,1,1,1,1,1,1,1,1,1,1,1,1,1,1,1,1,1,1,
1,1,1,1,1,1,1,1,1,1,1,1,1,1,1,1,1,1,1,1,1,1,1,1,1,1,1,1,1,1,1,1,1,1,1,1,
1,1,1,1,1,1,1,1,1,1,1,1,1,1,1,1,1,1,1,1,1,1,1,1,1,1,1,1,1,1,1,1,1,1,1,1,
1,1,1,1,1,1,1,1,1,1,1,1,1,1,1,1,1,1,1,1,1,1,1,1,1,1,1,1,1,1,1,1,1,1,1,6),
(2,2),(-1.,-0.995000000000001,-0.990000000000001,-0.985000000000001,-0.980000000000001,
-0.975000000000001,-0.970000000000001,-0.965000000000001,-0.960000000000001,
-0.955000000000001,-0.950000000000001,-0.945000000000001,-0.940000000000001,
-0.935000000000001,-0.930000000000001,-0.925000000000001,-0.920000000000001,
-0.915000000000001,-0.910000000000001,-0.905000000000001,-0.900000000000001,
-0.895000000000001,-0.890000000000001,-0.885000000000001,-0.880000000000001,
-0.875000000000001,-0.870000000000001,-0.865000000000001,-0.860000000000001,
-0.855000000000001,-0.850000000000001,-0.845000000000001,-0.840000000000001,
-0.835000000000001,-0.830000000000001,-0.825000000000001,-0.820000000000001,
-0.815000000000001,-0.810000000000001,-0.805000000000001,-0.800000000000001,
-0.795000000000001,-0.790000000000001,-0.785000000000001,-0.780000000000001,
-0.775000000000001,-0.770000000000001,-0.765000000000001,-0.760000000000001,
-0.755000000000001,-0.750000000000001,-0.745000000000001,-0.740000000000001,
-0.735000000000001,-0.730000000000001,-0.725000000000001,-0.720000000000001,
-0.715000000000001,-0.710000000000001,-0.705000000000001,-0.700000000000001,
-0.695000000000001,-0.690000000000001,-0.685,-0.68,-0.675,-0.67,-0.665,
-0.66,-0.655,-0.65,-0.645,-0.64,-0.635,-0.63,-0.625,-0.62,-0.615,-0.61,
-0.605,-0.6,-0.595,-0.59,-0.585,-0.58,-0.575,-0.57,-0.565,-0.56,-0.555,
-0.55,-0.545,-0.54,-0.535,-0.53,-0.525,-0.52,-0.515,-0.51,-0.505,-0.5,-0.495,
-0.49,-0.485,-0.48,-0.475,-0.47,-0.465,-0.46,-0.455,-0.45,-0.445,-0.44,
-0.435,-0.43,-0.425,-0.42,-0.415,-0.41,-0.405,-0.4,-0.395,-0.39,-0.385,
-0.38,-0.375,-0.37,-0.365,-0.36,-0.355,-0.35,-0.345,-0.34,-0.335,-0.33,
-0.325,-0.32,-0.315,-0.31,-0.305,-0.3,-0.295,-0.29,-0.285,-0.28,-0.275,
-0.27,-0.265,-0.26,-0.255,-0.25,-0.245,-0.24,-0.235,-0.23,-0.225,-0.22,
-0.215,-0.21,-0.205,-0.2,-0.195,-0.19,-0.185,-0.18,-0.175,-0.17,-0.165,
-0.16,-0.155,-0.15,-0.145,-0.14,-0.135,-0.13,-0.125,-0.12,-0.115,-0.11,
-0.105,-0.1,-0.095,-0.09,-0.085,-0.08,-0.075,-0.07,-0.065,-0.06,-0.055,
-0.05,-0.045,-0.04,-0.035,-0.03,-0.025,-0.02,-0.015,-0.01,-0.005,0.),(0.,
1.2),.UNSPECIFIED.)
GEOMETRIC_REPRESENTATION_ITEM()
RATIONAL_B_SPLINE_SURFACE(((1.,1.),(1.,1.),(1.,1.),(1.,1.),(1.,1.),(1.,
1.),(1.,1.),(1.,1.),(1.,1.),(1.,1.),(1.,1.),(1.,1.),(1.,1.),(1.,1.),(1.,
1.),(1.,1.),(1.,1.),(1.,1.),(1.,1.),(1.,1.),(1.,1.),(1.,1.),(1.,1.),(1.,
1.),(1.,1.),(1.,1.),(1.,1.),(1.,1.),(1.,1.),(1.,1.),(1.,1.),(1.,1.),(1.,
1.),(1.,1.),(1.,1.),(1.,1.),(1.,1.),(1.,1.),(1.,1.),(1.,1.),(1.,1.),(1.,
1.),(1.,1.),(1.,1.),(1.,1.),(1.,1.),(1.,1.),(1.,1.),(1.,1.),(1.,1.),(1.,
1.),(1.,1.),(1.,1.),(1.,1.),(1.,1.),(1.,1.),(1.,1.),(1.,1.),(1.,1.),(1.,
1.),(1.,1.),(1.,1.),(1.,1.),(1.,1.),(1.,1.),(1.,1.),(1.,1.),(1.,1.),(1.,
1.),(1.,1.),(1.,1.),(1.,1.),(1.,1.),(1.,1.),(1.,1.),(1.,1.),(1.,1.),(1.,
1.),(1.,1.),(1.,1.),(1.,1.),(1.,1.),(1.,1.),(1.,1.),(1.,1.),(1.,1.),(1.,
1.),(1.,1.),(1.,1.),(1.,1.),(1.,1.),(1.,1.),(1.,1.),(1.,1.),(1.,1.),(1.,
1.),(1.,1.),(1.,1.),(1.,1.),(1.,1.),(1.,1.),(1.,1.),(1.,1.),(1.,1.),(1.,
1.),(1.,1.),(1.,1.),(1.,1.),(1.,1.),(1.,1.),(1.,1.),(1.,1.),(1.,1.),(1.,
1.),(1.,1.),(1.,1.),(1.,1.),(1.,1.),(1.,1.),(1.,1.),(1.,1.),(1.,1.),(1.,
1.),(1.,1.),(1.,1.),(1.,1.),(1.,1.),(1.,1.),(1.,1.),(1.,1.),(1.,1.),(1.,
1.),(1.,1.),(1.,1.),(1.,1.),(1.,1.),(1.,1.),(1.,1.),(1.,1.),(1.,1.),(1.,
1.),(1.,1.),(1.,1.),(1.,1.),(1.,1.),(1.,1.),(1.,1.),(1.,1.),(1.,1.),(1.,
1.),(1.,1.),(1.,1.),(1.,1.),(1.,1.),(1.,1.),(1.,1.),(1.,1.),(1.,1.),(1.,
1.),(1.,1.),(1.,1.),(1.,1.),(1.,1.),(1.,1.),(1.,1.),(1.,1.),(1.,1.),(1.,
1.),(1.,1.),(1.,1.),(1.,1.),(1.,1.),(1.,1.),(1.,1.),(1.,1.),(1.,1.),(1.,
1.),(1.,1.),(1.,1.),(1.,1.),(1.,1.),(1.,1.),(1.,1.),(1.,1.),(1.,1.),(1.,
1.),(1.,1.),(1.,1.),(1.,1.),(1.,1.),(1.,1.),(1.,1.),(1.,1.),(1.,1.),(1.,
1.),(1.,1.),(1.,1.),(1.,1.),(1.,1.),(1.,1.),(1.,1.),(1.,1.),(1.,1.),(1.,
1.),(1.,1.)))
REPRESENTATION_ITEM('')
SURFACE()
);
#1104=(
BOUNDED_SURFACE()
B_SPLINE_SURFACE(5,1,((#239959,#239960),(#239961,#239962),(#239963,#239964),
(#239965,#239966),(#239967,#239968),(#239969,#239970),(#239971,#239972),
(#239973,#239974),(#239975,#239976),(#239977,#239978),(#239979,#239980),
(#239981,#239982),(#239983,#239984),(#239985,#239986),(#239987,#239988),
(#239989,#239990),(#239991,#239992),(#239993,#239994),(#239995,#239996),
(#239997,#239998),(#239999,#240000),(#240001,#240002),(#240003,#240004),
(#240005,#240006),(#240007,#240008),(#240009,#240010),(#240011,#240012),
(#240013,#240014),(#240015,#240016),(#240017,#240018),(#240019,#240020),
(#240021,#240022),(#240023,#240024),(#240025,#240026),(#240027,#240028),
(#240029,#240030),(#240031,#240032),(#240033,#240034),(#240035,#240036),
(#240037,#240038),(#240039,#240040),(#240041,#240042),(#240043,#240044),
(#240045,#240046),(#240047,#240048),(#240049,#240050),(#240051,#240052),
(#240053,#240054),(#240055,#240056),(#240057,#240058),(#240059,#240060),
(#240061,#240062),(#240063,#240064),(#240065,#240066),(#240067,#240068),
(#240069,#240070),(#240071,#240072),(#240073,#240074),(#240075,#240076),
(#240077,#240078),(#240079,#240080),(#240081,#240082),(#240083,#240084),
(#240085,#240086),(#240087,#240088),(#240089,#240090),(#240091,#240092),
(#240093,#240094),(#240095,#240096),(#240097,#240098),(#240099,#240100),
(#240101,#240102),(#240103,#240104),(#240105,#240106),(#240107,#240108),
(#240109,#240110),(#240111,#240112),(#240113,#240114),(#240115,#240116),
(#240117,#240118),(#240119,#240120),(#240121,#240122),(#240123,#240124),
(#240125,#240126),(#240127,#240128),(#240129,#240130),(#240131,#240132),
(#240133,#240134),(#240135,#240136),(#240137,#240138),(#240139,#240140),
(#240141,#240142),(#240143,#240144),(#240145,#240146),(#240147,#240148),
(#240149,#240150),(#240151,#240152),(#240153,#240154),(#240155,#240156),
(#240157,#240158),(#240159,#240160),(#240161,#240162),(#240163,#240164),
(#240165,#240166),(#240167,#240168),(#240169,#240170),(#240171,#240172),
(#240173,#240174),(#240175,#240176),(#240177,#240178),(#240179,#240180),
(#240181,#240182),(#240183,#240184),(#240185,#240186),(#240187,#240188),
(#240189,#240190),(#240191,#240192),(#240193,#240194),(#240195,#240196),
(#240197,#240198),(#240199,#240200),(#240201,#240202),(#240203,#240204),
(#240205,#240206),(#240207,#240208),(#240209,#240210),(#240211,#240212),
(#240213,#240214),(#240215,#240216),(#240217,#240218),(#240219,#240220),
(#240221,#240222),(#240223,#240224),(#240225,#240226),(#240227,#240228),
(#240229,#240230),(#240231,#240232),(#240233,#240234),(#240235,#240236),
(#240237,#240238),(#240239,#240240),(#240241,#240242),(#240243,#240244),
(#240245,#240246),(#240247,#240248),(#240249,#240250),(#240251,#240252),
(#240253,#240254),(#240255,#240256),(#240257,#240258),(#240259,#240260),
(#240261,#240262),(#240263,#240264),(#240265,#240266),(#240267,#240268),
(#240269,#240270),(#240271,#240272),(#240273,#240274),(#240275,#240276),
(#240277,#240278),(#240279,#240280),(#240281,#240282),(#240283,#240284),
(#240285,#240286),(#240287,#240288),(#240289,#240290),(#240291,#240292),
(#240293,#240294),(#240295,#240296),(#240297,#240298),(#240299,#240300),
(#240301,#240302),(#240303,#240304),(#240305,#240306),(#240307,#240308),
(#240309,#240310),(#240311,#240312),(#240313,#240314),(#240315,#240316),
(#240317,#240318),(#240319,#240320),(#240321,#240322),(#240323,#240324),
(#240325,#240326),(#240327,#240328),(#240329,#240330),(#240331,#240332),
(#240333,#240334),(#240335,#240336),(#240337,#240338),(#240339,#240340),
(#240341,#240342),(#240343,#240344),(#240345,#240346),(#240347,#240348),
(#240349,#240350),(#240351,#240352),(#240353,#240354),(#240355,#240356),
(#240357,#240358),(#240359,#240360),(#240361,#240362),(#240363,#240364),
(#240365,#240366),(#240367,#240368)),.UNSPECIFIED.,.F.,.F.,.F.)
B_SPLINE_SURFACE_WITH_KNOTS((6,1,1,1,1,1,1,1,1,1,1,1,1,1,1,1,1,1,1,1,1,
1,1,1,1,1,1,1,1,1,1,1,1,1,1,1,1,1,1,1,1,1,1,1,1,1,1,1,1,1,1,1,1,1,1,1,1,
1,1,1,1,1,1,1,1,1,1,1,1,1,1,1,1,1,1,1,1,1,1,1,1,1,1,1,1,1,1,1,1,1,1,1,1,
1,1,1,1,1,1,1,1,1,1,1,1,1,1,1,1,1,1,1,1,1,1,1,1,1,1,1,1,1,1,1,1,1,1,1,1,
1,1,1,1,1,1,1,1,1,1,1,1,1,1,1,1,1,1,1,1,1,1,1,1,1,1,1,1,1,1,1,1,1,1,1,1,
1,1,1,1,1,1,1,1,1,1,1,1,1,1,1,1,1,1,1,1,1,1,1,1,1,1,1,1,1,1,1,1,1,1,1,6),
(2,2),(0.,0.005,0.01,0.015,0.02,0.025,0.03,0.035,0.04,0.045,0.05,0.055,
0.06,0.065,0.07,0.075,0.08,0.085,0.09,0.095,0.1,0.105,0.11,0.115,0.12,0.125,
0.13,0.135,0.14,0.145,0.15,0.155,0.16,0.165,0.17,0.175,0.18,0.185,0.19,
0.195,0.2,0.205,0.21,0.215,0.22,0.225,0.23,0.235,0.24,0.245,0.25,0.255,
0.26,0.265,0.27,0.275,0.28,0.285,0.29,0.295,0.3,0.305,0.31,0.315,0.32,0.325,
0.33,0.335,0.34,0.345,0.35,0.355,0.36,0.365,0.37,0.375,0.38,0.385,0.39,
0.395,0.4,0.405,0.41,0.415,0.42,0.425,0.43,0.435,0.44,0.445,0.45,0.455,
0.46,0.465,0.47,0.475,0.48,0.485,0.49,0.495,0.5,0.505,0.51,0.515,0.52,0.525,
0.53,0.535,0.54,0.545,0.55,0.555,0.56,0.565,0.57,0.575,0.58,0.585,0.59,
0.595,0.6,0.605,0.61,0.615,0.62,0.625,0.63,0.635,0.64,0.645,0.65,0.655,
0.66,0.665,0.67,0.675,0.68,0.685,0.690000000000001,0.695000000000001,0.700000000000001,
0.705000000000001,0.710000000000001,0.715000000000001,0.720000000000001,
0.725000000000001,0.730000000000001,0.735000000000001,0.740000000000001,
0.745000000000001,0.750000000000001,0.755000000000001,0.760000000000001,
0.765000000000001,0.770000000000001,0.775000000000001,0.780000000000001,
0.785000000000001,0.790000000000001,0.795000000000001,0.800000000000001,
0.805000000000001,0.810000000000001,0.815000000000001,0.820000000000001,
0.825000000000001,0.830000000000001,0.835000000000001,0.840000000000001,
0.845000000000001,0.850000000000001,0.855000000000001,0.860000000000001,
0.865000000000001,0.870000000000001,0.875000000000001,0.880000000000001,
0.885000000000001,0.890000000000001,0.895000000000001,0.900000000000001,
0.905000000000001,0.910000000000001,0.915000000000001,0.920000000000001,
0.925000000000001,0.930000000000001,0.935000000000001,0.940000000000001,
0.945000000000001,0.950000000000001,0.955000000000001,0.960000000000001,
0.965000000000001,0.970000000000001,0.975000000000001,0.980000000000001,
0.985000000000001,0.990000000000001,0.995000000000001,1.),(0.,1.2),
 .UNSPECIFIED.)
GEOMETRIC_REPRESENTATION_ITEM()
RATIONAL_B_SPLINE_SURFACE(((1.,1.),(1.,1.),(1.,1.),(1.,1.),(1.,1.),(1.,
1.),(1.,1.),(1.,1.),(1.,1.),(1.,1.),(1.,1.),(1.,1.),(1.,1.),(1.,1.),(1.,
1.),(1.,1.),(1.,1.),(1.,1.),(1.,1.),(1.,1.),(1.,1.),(1.,1.),(1.,1.),(1.,
1.),(1.,1.),(1.,1.),(1.,1.),(1.,1.),(1.,1.),(1.,1.),(1.,1.),(1.,1.),(1.,
1.),(1.,1.),(1.,1.),(1.,1.),(1.,1.),(1.,1.),(1.,1.),(1.,1.),(1.,1.),(1.,
1.),(1.,1.),(1.,1.),(1.,1.),(1.,1.),(1.,1.),(1.,1.),(1.,1.),(1.,1.),(1.,
1.),(1.,1.),(1.,1.),(1.,1.),(1.,1.),(1.,1.),(1.,1.),(1.,1.),(1.,1.),(1.,
1.),(1.,1.),(1.,1.),(1.,1.),(1.,1.),(1.,1.),(1.,1.),(1.,1.),(1.,1.),(1.,
1.),(1.,1.),(1.,1.),(1.,1.),(1.,1.),(1.,1.),(1.,1.),(1.,1.),(1.,1.),(1.,
1.),(1.,1.),(1.,1.),(1.,1.),(1.,1.),(1.,1.),(1.,1.),(1.,1.),(1.,1.),(1.,
1.),(1.,1.),(1.,1.),(1.,1.),(1.,1.),(1.,1.),(1.,1.),(1.,1.),(1.,1.),(1.,
1.),(1.,1.),(1.,1.),(1.,1.),(1.,1.),(1.,1.),(1.,1.),(1.,1.),(1.,1.),(1.,
1.),(1.,1.),(1.,1.),(1.,1.),(1.,1.),(1.,1.),(1.,1.),(1.,1.),(1.,1.),(1.,
1.),(1.,1.),(1.,1.),(1.,1.),(1.,1.),(1.,1.),(1.,1.),(1.,1.),(1.,1.),(1.,
1.),(1.,1.),(1.,1.),(1.,1.),(1.,1.),(1.,1.),(1.,1.),(1.,1.),(1.,1.),(1.,
1.),(1.,1.),(1.,1.),(1.,1.),(1.,1.),(1.,1.),(1.,1.),(1.,1.),(1.,1.),(1.,
1.),(1.,1.),(1.,1.),(1.,1.),(1.,1.),(1.,1.),(1.,1.),(1.,1.),(1.,1.),(1.,
1.),(1.,1.),(1.,1.),(1.,1.),(1.,1.),(1.,1.),(1.,1.),(1.,1.),(1.,1.),(1.,
1.),(1.,1.),(1.,1.),(1.,1.),(1.,1.),(1.,1.),(1.,1.),(1.,1.),(1.,1.),(1.,
1.),(1.,1.),(1.,1.),(1.,1.),(1.,1.),(1.,1.),(1.,1.),(1.,1.),(1.,1.),(1.,
1.),(1.,1.),(1.,1.),(1.,1.),(1.,1.),(1.,1.),(1.,1.),(1.,1.),(1.,1.),(1.,
1.),(1.,1.),(1.,1.),(1.,1.),(1.,1.),(1.,1.),(1.,1.),(1.,1.),(1.,1.),(1.,
1.),(1.,1.),(1.,1.),(1.,1.),(1.,1.),(1.,1.),(1.,1.),(1.,1.),(1.,1.),(1.,
1.),(1.,1.)))
REPRESENTATION_ITEM('')
SURFACE()
);
#1105=(
BOUNDED_SURFACE()
B_SPLINE_SURFACE(5,1,((#240788,#240789),(#240790,#240791),(#240792,#240793),
(#240794,#240795),(#240796,#240797),(#240798,#240799),(#240800,#240801),
(#240802,#240803),(#240804,#240805),(#240806,#240807),(#240808,#240809),
(#240810,#240811),(#240812,#240813),(#240814,#240815),(#240816,#240817),
(#240818,#240819),(#240820,#240821),(#240822,#240823),(#240824,#240825),
(#240826,#240827),(#240828,#240829),(#240830,#240831),(#240832,#240833),
(#240834,#240835),(#240836,#240837),(#240838,#240839),(#240840,#240841),
(#240842,#240843),(#240844,#240845),(#240846,#240847),(#240848,#240849),
(#240850,#240851),(#240852,#240853),(#240854,#240855),(#240856,#240857),
(#240858,#240859),(#240860,#240861),(#240862,#240863),(#240864,#240865),
(#240866,#240867),(#240868,#240869),(#240870,#240871),(#240872,#240873),
(#240874,#240875),(#240876,#240877),(#240878,#240879),(#240880,#240881),
(#240882,#240883),(#240884,#240885),(#240886,#240887),(#240888,#240889),
(#240890,#240891),(#240892,#240893),(#240894,#240895),(#240896,#240897),
(#240898,#240899),(#240900,#240901),(#240902,#240903),(#240904,#240905),
(#240906,#240907),(#240908,#240909),(#240910,#240911),(#240912,#240913),
(#240914,#240915),(#240916,#240917),(#240918,#240919),(#240920,#240921),
(#240922,#240923),(#240924,#240925),(#240926,#240927),(#240928,#240929),
(#240930,#240931),(#240932,#240933),(#240934,#240935),(#240936,#240937),
(#240938,#240939),(#240940,#240941),(#240942,#240943),(#240944,#240945),
(#240946,#240947),(#240948,#240949),(#240950,#240951),(#240952,#240953),
(#240954,#240955),(#240956,#240957),(#240958,#240959),(#240960,#240961),
(#240962,#240963),(#240964,#240965),(#240966,#240967),(#240968,#240969),
(#240970,#240971),(#240972,#240973),(#240974,#240975),(#240976,#240977),
(#240978,#240979),(#240980,#240981),(#240982,#240983),(#240984,#240985),
(#240986,#240987),(#240988,#240989),(#240990,#240991),(#240992,#240993),
(#240994,#240995),(#240996,#240997),(#240998,#240999),(#241000,#241001),
(#241002,#241003),(#241004,#241005),(#241006,#241007),(#241008,#241009),
(#241010,#241011),(#241012,#241013),(#241014,#241015),(#241016,#241017),
(#241018,#241019),(#241020,#241021),(#241022,#241023),(#241024,#241025),
(#241026,#241027),(#241028,#241029),(#241030,#241031),(#241032,#241033),
(#241034,#241035),(#241036,#241037),(#241038,#241039),(#241040,#241041),
(#241042,#241043),(#241044,#241045),(#241046,#241047),(#241048,#241049),
(#241050,#241051),(#241052,#241053),(#241054,#241055),(#241056,#241057),
(#241058,#241059),(#241060,#241061),(#241062,#241063),(#241064,#241065),
(#241066,#241067),(#241068,#241069),(#241070,#241071),(#241072,#241073),
(#241074,#241075),(#241076,#241077),(#241078,#241079),(#241080,#241081),
(#241082,#241083),(#241084,#241085),(#241086,#241087),(#241088,#241089),
(#241090,#241091),(#241092,#241093),(#241094,#241095),(#241096,#241097),
(#241098,#241099),(#241100,#241101),(#241102,#241103),(#241104,#241105),
(#241106,#241107),(#241108,#241109),(#241110,#241111),(#241112,#241113),
(#241114,#241115),(#241116,#241117),(#241118,#241119),(#241120,#241121),
(#241122,#241123),(#241124,#241125),(#241126,#241127),(#241128,#241129),
(#241130,#241131),(#241132,#241133),(#241134,#241135),(#241136,#241137),
(#241138,#241139),(#241140,#241141),(#241142,#241143),(#241144,#241145),
(#241146,#241147),(#241148,#241149),(#241150,#241151),(#241152,#241153),
(#241154,#241155),(#241156,#241157),(#241158,#241159),(#241160,#241161),
(#241162,#241163),(#241164,#241165),(#241166,#241167),(#241168,#241169),
(#241170,#241171),(#241172,#241173),(#241174,#241175),(#241176,#241177),
(#241178,#241179),(#241180,#241181),(#241182,#241183),(#241184,#241185),
(#241186,#241187),(#241188,#241189),(#241190,#241191),(#241192,#241193),
(#241194,#241195),(#241196,#241197)),.UNSPECIFIED.,.F.,.F.,.F.)
B_SPLINE_SURFACE_WITH_KNOTS((6,1,1,1,1,1,1,1,1,1,1,1,1,1,1,1,1,1,1,1,1,
1,1,1,1,1,1,1,1,1,1,1,1,1,1,1,1,1,1,1,1,1,1,1,1,1,1,1,1,1,1,1,1,1,1,1,1,
1,1,1,1,1,1,1,1,1,1,1,1,1,1,1,1,1,1,1,1,1,1,1,1,1,1,1,1,1,1,1,1,1,1,1,1,
1,1,1,1,1,1,1,1,1,1,1,1,1,1,1,1,1,1,1,1,1,1,1,1,1,1,1,1,1,1,1,1,1,1,1,1,
1,1,1,1,1,1,1,1,1,1,1,1,1,1,1,1,1,1,1,1,1,1,1,1,1,1,1,1,1,1,1,1,1,1,1,1,
1,1,1,1,1,1,1,1,1,1,1,1,1,1,1,1,1,1,1,1,1,1,1,1,1,1,1,1,1,1,1,1,1,1,1,6),
(2,2),(-1.,-0.995000000000001,-0.990000000000001,-0.985000000000001,-0.980000000000001,
-0.975000000000001,-0.970000000000001,-0.965000000000001,-0.960000000000001,
-0.955000000000001,-0.950000000000001,-0.945000000000001,-0.940000000000001,
-0.935000000000001,-0.930000000000001,-0.925000000000001,-0.920000000000001,
-0.915000000000001,-0.910000000000001,-0.905000000000001,-0.900000000000001,
-0.895000000000001,-0.890000000000001,-0.885000000000001,-0.880000000000001,
-0.875000000000001,-0.870000000000001,-0.865000000000001,-0.860000000000001,
-0.855000000000001,-0.850000000000001,-0.845000000000001,-0.840000000000001,
-0.835000000000001,-0.830000000000001,-0.825000000000001,-0.820000000000001,
-0.815000000000001,-0.810000000000001,-0.805000000000001,-0.800000000000001,
-0.795000000000001,-0.790000000000001,-0.785000000000001,-0.780000000000001,
-0.775000000000001,-0.770000000000001,-0.765000000000001,-0.760000000000001,
-0.755000000000001,-0.750000000000001,-0.745000000000001,-0.740000000000001,
-0.735000000000001,-0.730000000000001,-0.725000000000001,-0.720000000000001,
-0.715000000000001,-0.710000000000001,-0.705000000000001,-0.700000000000001,
-0.695000000000001,-0.690000000000001,-0.685,-0.68,-0.675,-0.67,-0.665,
-0.66,-0.655,-0.65,-0.645,-0.64,-0.635,-0.63,-0.625,-0.62,-0.615,-0.61,
-0.605,-0.6,-0.595,-0.59,-0.585,-0.58,-0.575,-0.57,-0.565,-0.56,-0.555,
-0.55,-0.545,-0.54,-0.535,-0.53,-0.525,-0.52,-0.515,-0.51,-0.505,-0.5,-0.495,
-0.49,-0.485,-0.48,-0.475,-0.47,-0.465,-0.46,-0.455,-0.45,-0.445,-0.44,
-0.435,-0.43,-0.425,-0.42,-0.415,-0.41,-0.405,-0.4,-0.395,-0.39,-0.385,
-0.38,-0.375,-0.37,-0.365,-0.36,-0.355,-0.35,-0.345,-0.34,-0.335,-0.33,
-0.325,-0.32,-0.315,-0.31,-0.305,-0.3,-0.295,-0.29,-0.285,-0.28,-0.275,
-0.27,-0.265,-0.26,-0.255,-0.25,-0.245,-0.24,-0.235,-0.23,-0.225,-0.22,
-0.215,-0.21,-0.205,-0.2,-0.195,-0.19,-0.185,-0.18,-0.175,-0.17,-0.165,
-0.16,-0.155,-0.15,-0.145,-0.14,-0.135,-0.13,-0.125,-0.12,-0.115,-0.11,
-0.105,-0.1,-0.095,-0.09,-0.085,-0.08,-0.075,-0.07,-0.065,-0.06,-0.055,
-0.05,-0.045,-0.04,-0.035,-0.03,-0.025,-0.02,-0.015,-0.01,-0.005,0.),(0.,
1.2),.UNSPECIFIED.)
GEOMETRIC_REPRESENTATION_ITEM()
RATIONAL_B_SPLINE_SURFACE(((1.,1.),(1.,1.),(1.,1.),(1.,1.),(1.,1.),(1.,
1.),(1.,1.),(1.,1.),(1.,1.),(1.,1.),(1.,1.),(1.,1.),(1.,1.),(1.,1.),(1.,
1.),(1.,1.),(1.,1.),(1.,1.),(1.,1.),(1.,1.),(1.,1.),(1.,1.),(1.,1.),(1.,
1.),(1.,1.),(1.,1.),(1.,1.),(1.,1.),(1.,1.),(1.,1.),(1.,1.),(1.,1.),(1.,
1.),(1.,1.),(1.,1.),(1.,1.),(1.,1.),(1.,1.),(1.,1.),(1.,1.),(1.,1.),(1.,
1.),(1.,1.),(1.,1.),(1.,1.),(1.,1.),(1.,1.),(1.,1.),(1.,1.),(1.,1.),(1.,
1.),(1.,1.),(1.,1.),(1.,1.),(1.,1.),(1.,1.),(1.,1.),(1.,1.),(1.,1.),(1.,
1.),(1.,1.),(1.,1.),(1.,1.),(1.,1.),(1.,1.),(1.,1.),(1.,1.),(1.,1.),(1.,
1.),(1.,1.),(1.,1.),(1.,1.),(1.,1.),(1.,1.),(1.,1.),(1.,1.),(1.,1.),(1.,
1.),(1.,1.),(1.,1.),(1.,1.),(1.,1.),(1.,1.),(1.,1.),(1.,1.),(1.,1.),(1.,
1.),(1.,1.),(1.,1.),(1.,1.),(1.,1.),(1.,1.),(1.,1.),(1.,1.),(1.,1.),(1.,
1.),(1.,1.),(1.,1.),(1.,1.),(1.,1.),(1.,1.),(1.,1.),(1.,1.),(1.,1.),(1.,
1.),(1.,1.),(1.,1.),(1.,1.),(1.,1.),(1.,1.),(1.,1.),(1.,1.),(1.,1.),(1.,
1.),(1.,1.),(1.,1.),(1.,1.),(1.,1.),(1.,1.),(1.,1.),(1.,1.),(1.,1.),(1.,
1.),(1.,1.),(1.,1.),(1.,1.),(1.,1.),(1.,1.),(1.,1.),(1.,1.),(1.,1.),(1.,
1.),(1.,1.),(1.,1.),(1.,1.),(1.,1.),(1.,1.),(1.,1.),(1.,1.),(1.,1.),(1.,
1.),(1.,1.),(1.,1.),(1.,1.),(1.,1.),(1.,1.),(1.,1.),(1.,1.),(1.,1.),(1.,
1.),(1.,1.),(1.,1.),(1.,1.),(1.,1.),(1.,1.),(1.,1.),(1.,1.),(1.,1.),(1.,
1.),(1.,1.),(1.,1.),(1.,1.),(1.,1.),(1.,1.),(1.,1.),(1.,1.),(1.,1.),(1.,
1.),(1.,1.),(1.,1.),(1.,1.),(1.,1.),(1.,1.),(1.,1.),(1.,1.),(1.,1.),(1.,
1.),(1.,1.),(1.,1.),(1.,1.),(1.,1.),(1.,1.),(1.,1.),(1.,1.),(1.,1.),(1.,
1.),(1.,1.),(1.,1.),(1.,1.),(1.,1.),(1.,1.),(1.,1.),(1.,1.),(1.,1.),(1.,
1.),(1.,1.),(1.,1.),(1.,1.),(1.,1.),(1.,1.),(1.,1.),(1.,1.),(1.,1.),(1.,
1.),(1.,1.)))
REPRESENTATION_ITEM('')
SURFACE()
);
#1106=(
BOUNDED_SURFACE()
B_SPLINE_SURFACE(5,1,((#241611,#241612),(#241613,#241614),(#241615,#241616),
(#241617,#241618),(#241619,#241620),(#241621,#241622),(#241623,#241624),
(#241625,#241626),(#241627,#241628),(#241629,#241630),(#241631,#241632),
(#241633,#241634),(#241635,#241636),(#241637,#241638),(#241639,#241640),
(#241641,#241642),(#241643,#241644),(#241645,#241646),(#241647,#241648),
(#241649,#241650),(#241651,#241652),(#241653,#241654),(#241655,#241656),
(#241657,#241658),(#241659,#241660),(#241661,#241662),(#241663,#241664),
(#241665,#241666),(#241667,#241668),(#241669,#241670),(#241671,#241672),
(#241673,#241674),(#241675,#241676),(#241677,#241678),(#241679,#241680),
(#241681,#241682),(#241683,#241684),(#241685,#241686),(#241687,#241688),
(#241689,#241690),(#241691,#241692),(#241693,#241694),(#241695,#241696),
(#241697,#241698),(#241699,#241700),(#241701,#241702),(#241703,#241704),
(#241705,#241706),(#241707,#241708),(#241709,#241710),(#241711,#241712),
(#241713,#241714),(#241715,#241716),(#241717,#241718),(#241719,#241720),
(#241721,#241722),(#241723,#241724),(#241725,#241726),(#241727,#241728),
(#241729,#241730),(#241731,#241732),(#241733,#241734),(#241735,#241736),
(#241737,#241738),(#241739,#241740),(#241741,#241742),(#241743,#241744),
(#241745,#241746),(#241747,#241748),(#241749,#241750),(#241751,#241752),
(#241753,#241754),(#241755,#241756),(#241757,#241758),(#241759,#241760),
(#241761,#241762),(#241763,#241764),(#241765,#241766),(#241767,#241768),
(#241769,#241770),(#241771,#241772),(#241773,#241774),(#241775,#241776),
(#241777,#241778),(#241779,#241780),(#241781,#241782),(#241783,#241784),
(#241785,#241786),(#241787,#241788),(#241789,#241790),(#241791,#241792),
(#241793,#241794),(#241795,#241796),(#241797,#241798),(#241799,#241800),
(#241801,#241802),(#241803,#241804),(#241805,#241806),(#241807,#241808),
(#241809,#241810),(#241811,#241812),(#241813,#241814),(#241815,#241816),
(#241817,#241818),(#241819,#241820),(#241821,#241822),(#241823,#241824),
(#241825,#241826),(#241827,#241828),(#241829,#241830),(#241831,#241832),
(#241833,#241834),(#241835,#241836),(#241837,#241838),(#241839,#241840),
(#241841,#241842),(#241843,#241844),(#241845,#241846),(#241847,#241848),
(#241849,#241850),(#241851,#241852),(#241853,#241854),(#241855,#241856),
(#241857,#241858),(#241859,#241860),(#241861,#241862),(#241863,#241864),
(#241865,#241866),(#241867,#241868),(#241869,#241870),(#241871,#241872),
(#241873,#241874),(#241875,#241876),(#241877,#241878),(#241879,#241880),
(#241881,#241882),(#241883,#241884),(#241885,#241886),(#241887,#241888),
(#241889,#241890),(#241891,#241892),(#241893,#241894),(#241895,#241896),
(#241897,#241898),(#241899,#241900),(#241901,#241902),(#241903,#241904),
(#241905,#241906),(#241907,#241908),(#241909,#241910),(#241911,#241912),
(#241913,#241914),(#241915,#241916),(#241917,#241918),(#241919,#241920),
(#241921,#241922),(#241923,#241924),(#241925,#241926),(#241927,#241928),
(#241929,#241930),(#241931,#241932),(#241933,#241934),(#241935,#241936),
(#241937,#241938),(#241939,#241940),(#241941,#241942),(#241943,#241944),
(#241945,#241946),(#241947,#241948),(#241949,#241950),(#241951,#241952),
(#241953,#241954),(#241955,#241956),(#241957,#241958),(#241959,#241960),
(#241961,#241962),(#241963,#241964),(#241965,#241966),(#241967,#241968),
(#241969,#241970),(#241971,#241972),(#241973,#241974),(#241975,#241976),
(#241977,#241978),(#241979,#241980),(#241981,#241982),(#241983,#241984),
(#241985,#241986),(#241987,#241988),(#241989,#241990),(#241991,#241992),
(#241993,#241994),(#241995,#241996),(#241997,#241998),(#241999,#242000),
(#242001,#242002),(#242003,#242004),(#242005,#242006),(#242007,#242008),
(#242009,#242010),(#242011,#242012),(#242013,#242014),(#242015,#242016),
(#242017,#242018),(#242019,#242020)),.UNSPECIFIED.,.F.,.F.,.F.)
B_SPLINE_SURFACE_WITH_KNOTS((6,1,1,1,1,1,1,1,1,1,1,1,1,1,1,1,1,1,1,1,1,
1,1,1,1,1,1,1,1,1,1,1,1,1,1,1,1,1,1,1,1,1,1,1,1,1,1,1,1,1,1,1,1,1,1,1,1,
1,1,1,1,1,1,1,1,1,1,1,1,1,1,1,1,1,1,1,1,1,1,1,1,1,1,1,1,1,1,1,1,1,1,1,1,
1,1,1,1,1,1,1,1,1,1,1,1,1,1,1,1,1,1,1,1,1,1,1,1,1,1,1,1,1,1,1,1,1,1,1,1,
1,1,1,1,1,1,1,1,1,1,1,1,1,1,1,1,1,1,1,1,1,1,1,1,1,1,1,1,1,1,1,1,1,1,1,1,
1,1,1,1,1,1,1,1,1,1,1,1,1,1,1,1,1,1,1,1,1,1,1,1,1,1,1,1,1,1,1,1,1,1,1,6),
(2,2),(0.,0.005,0.01,0.015,0.02,0.025,0.03,0.035,0.04,0.045,0.05,0.055,
0.06,0.065,0.07,0.075,0.08,0.085,0.09,0.095,0.1,0.105,0.11,0.115,0.12,0.125,
0.13,0.135,0.14,0.145,0.15,0.155,0.16,0.165,0.17,0.175,0.18,0.185,0.19,
0.195,0.2,0.205,0.21,0.215,0.22,0.225,0.23,0.235,0.24,0.245,0.25,0.255,
0.26,0.265,0.27,0.275,0.28,0.285,0.29,0.295,0.3,0.305,0.31,0.315,0.32,0.325,
0.33,0.335,0.34,0.345,0.35,0.355,0.36,0.365,0.37,0.375,0.38,0.385,0.39,
0.395,0.4,0.405,0.41,0.415,0.42,0.425,0.43,0.435,0.44,0.445,0.45,0.455,
0.46,0.465,0.47,0.475,0.48,0.485,0.49,0.495,0.5,0.505,0.51,0.515,0.52,0.525,
0.53,0.535,0.54,0.545,0.55,0.555,0.56,0.565,0.57,0.575,0.58,0.585,0.59,
0.595,0.6,0.605,0.61,0.615,0.62,0.625,0.63,0.635,0.64,0.645,0.65,0.655,
0.66,0.665,0.67,0.675,0.68,0.685,0.690000000000001,0.695000000000001,0.700000000000001,
0.705000000000001,0.710000000000001,0.715000000000001,0.720000000000001,
0.725000000000001,0.730000000000001,0.735000000000001,0.740000000000001,
0.745000000000001,0.750000000000001,0.755000000000001,0.760000000000001,
0.765000000000001,0.770000000000001,0.775000000000001,0.780000000000001,
0.785000000000001,0.790000000000001,0.795000000000001,0.800000000000001,
0.805000000000001,0.810000000000001,0.815000000000001,0.820000000000001,
0.825000000000001,0.830000000000001,0.835000000000001,0.840000000000001,
0.845000000000001,0.850000000000001,0.855000000000001,0.860000000000001,
0.865000000000001,0.870000000000001,0.875000000000001,0.880000000000001,
0.885000000000001,0.890000000000001,0.895000000000001,0.900000000000001,
0.905000000000001,0.910000000000001,0.915000000000001,0.920000000000001,
0.925000000000001,0.930000000000001,0.935000000000001,0.940000000000001,
0.945000000000001,0.950000000000001,0.955000000000001,0.960000000000001,
0.965000000000001,0.970000000000001,0.975000000000001,0.980000000000001,
0.985000000000001,0.990000000000001,0.995000000000001,1.),(0.,1.2),
 .UNSPECIFIED.)
GEOMETRIC_REPRESENTATION_ITEM()
RATIONAL_B_SPLINE_SURFACE(((1.,1.),(1.,1.),(1.,1.),(1.,1.),(1.,1.),(1.,
1.),(1.,1.),(1.,1.),(1.,1.),(1.,1.),(1.,1.),(1.,1.),(1.,1.),(1.,1.),(1.,
1.),(1.,1.),(1.,1.),(1.,1.),(1.,1.),(1.,1.),(1.,1.),(1.,1.),(1.,1.),(1.,
1.),(1.,1.),(1.,1.),(1.,1.),(1.,1.),(1.,1.),(1.,1.),(1.,1.),(1.,1.),(1.,
1.),(1.,1.),(1.,1.),(1.,1.),(1.,1.),(1.,1.),(1.,1.),(1.,1.),(1.,1.),(1.,
1.),(1.,1.),(1.,1.),(1.,1.),(1.,1.),(1.,1.),(1.,1.),(1.,1.),(1.,1.),(1.,
1.),(1.,1.),(1.,1.),(1.,1.),(1.,1.),(1.,1.),(1.,1.),(1.,1.),(1.,1.),(1.,
1.),(1.,1.),(1.,1.),(1.,1.),(1.,1.),(1.,1.),(1.,1.),(1.,1.),(1.,1.),(1.,
1.),(1.,1.),(1.,1.),(1.,1.),(1.,1.),(1.,1.),(1.,1.),(1.,1.),(1.,1.),(1.,
1.),(1.,1.),(1.,1.),(1.,1.),(1.,1.),(1.,1.),(1.,1.),(1.,1.),(1.,1.),(1.,
1.),(1.,1.),(1.,1.),(1.,1.),(1.,1.),(1.,1.),(1.,1.),(1.,1.),(1.,1.),(1.,
1.),(1.,1.),(1.,1.),(1.,1.),(1.,1.),(1.,1.),(1.,1.),(1.,1.),(1.,1.),(1.,
1.),(1.,1.),(1.,1.),(1.,1.),(1.,1.),(1.,1.),(1.,1.),(1.,1.),(1.,1.),(1.,
1.),(1.,1.),(1.,1.),(1.,1.),(1.,1.),(1.,1.),(1.,1.),(1.,1.),(1.,1.),(1.,
1.),(1.,1.),(1.,1.),(1.,1.),(1.,1.),(1.,1.),(1.,1.),(1.,1.),(1.,1.),(1.,
1.),(1.,1.),(1.,1.),(1.,1.),(1.,1.),(1.,1.),(1.,1.),(1.,1.),(1.,1.),(1.,
1.),(1.,1.),(1.,1.),(1.,1.),(1.,1.),(1.,1.),(1.,1.),(1.,1.),(1.,1.),(1.,
1.),(1.,1.),(1.,1.),(1.,1.),(1.,1.),(1.,1.),(1.,1.),(1.,1.),(1.,1.),(1.,
1.),(1.,1.),(1.,1.),(1.,1.),(1.,1.),(1.,1.),(1.,1.),(1.,1.),(1.,1.),(1.,
1.),(1.,1.),(1.,1.),(1.,1.),(1.,1.),(1.,1.),(1.,1.),(1.,1.),(1.,1.),(1.,
1.),(1.,1.),(1.,1.),(1.,1.),(1.,1.),(1.,1.),(1.,1.),(1.,1.),(1.,1.),(1.,
1.),(1.,1.),(1.,1.),(1.,1.),(1.,1.),(1.,1.),(1.,1.),(1.,1.),(1.,1.),(1.,
1.),(1.,1.),(1.,1.),(1.,1.),(1.,1.),(1.,1.),(1.,1.),(1.,1.),(1.,1.),(1.,
1.),(1.,1.)))
REPRESENTATION_ITEM('')
SURFACE()
);
#1107=(
BOUNDED_SURFACE()
B_SPLINE_SURFACE(5,1,((#242440,#242441),(#242442,#242443),(#242444,#242445),
(#242446,#242447),(#242448,#242449),(#242450,#242451),(#242452,#242453),
(#242454,#242455),(#242456,#242457),(#242458,#242459),(#242460,#242461),
(#242462,#242463),(#242464,#242465),(#242466,#242467),(#242468,#242469),
(#242470,#242471),(#242472,#242473),(#242474,#242475),(#242476,#242477),
(#242478,#242479),(#242480,#242481),(#242482,#242483),(#242484,#242485),
(#242486,#242487),(#242488,#242489),(#242490,#242491),(#242492,#242493),
(#242494,#242495),(#242496,#242497),(#242498,#242499),(#242500,#242501),
(#242502,#242503),(#242504,#242505),(#242506,#242507),(#242508,#242509),
(#242510,#242511),(#242512,#242513),(#242514,#242515),(#242516,#242517),
(#242518,#242519),(#242520,#242521),(#242522,#242523),(#242524,#242525),
(#242526,#242527),(#242528,#242529),(#242530,#242531),(#242532,#242533),
(#242534,#242535),(#242536,#242537),(#242538,#242539),(#242540,#242541),
(#242542,#242543),(#242544,#242545),(#242546,#242547),(#242548,#242549),
(#242550,#242551),(#242552,#242553),(#242554,#242555),(#242556,#242557),
(#242558,#242559),(#242560,#242561),(#242562,#242563),(#242564,#242565),
(#242566,#242567),(#242568,#242569),(#242570,#242571),(#242572,#242573),
(#242574,#242575),(#242576,#242577),(#242578,#242579),(#242580,#242581),
(#242582,#242583),(#242584,#242585),(#242586,#242587),(#242588,#242589),
(#242590,#242591),(#242592,#242593),(#242594,#242595),(#242596,#242597),
(#242598,#242599),(#242600,#242601),(#242602,#242603),(#242604,#242605),
(#242606,#242607),(#242608,#242609),(#242610,#242611),(#242612,#242613),
(#242614,#242615),(#242616,#242617),(#242618,#242619),(#242620,#242621),
(#242622,#242623),(#242624,#242625),(#242626,#242627),(#242628,#242629),
(#242630,#242631),(#242632,#242633),(#242634,#242635),(#242636,#242637),
(#242638,#242639),(#242640,#242641),(#242642,#242643),(#242644,#242645),
(#242646,#242647),(#242648,#242649),(#242650,#242651),(#242652,#242653),
(#242654,#242655),(#242656,#242657),(#242658,#242659),(#242660,#242661),
(#242662,#242663),(#242664,#242665),(#242666,#242667),(#242668,#242669),
(#242670,#242671),(#242672,#242673),(#242674,#242675),(#242676,#242677),
(#242678,#242679),(#242680,#242681),(#242682,#242683),(#242684,#242685),
(#242686,#242687),(#242688,#242689),(#242690,#242691),(#242692,#242693),
(#242694,#242695),(#242696,#242697),(#242698,#242699),(#242700,#242701),
(#242702,#242703),(#242704,#242705),(#242706,#242707),(#242708,#242709),
(#242710,#242711),(#242712,#242713),(#242714,#242715),(#242716,#242717),
(#242718,#242719),(#242720,#242721),(#242722,#242723),(#242724,#242725),
(#242726,#242727),(#242728,#242729),(#242730,#242731),(#242732,#242733),
(#242734,#242735),(#242736,#242737),(#242738,#242739),(#242740,#242741),
(#242742,#242743),(#242744,#242745),(#242746,#242747),(#242748,#242749),
(#242750,#242751),(#242752,#242753),(#242754,#242755),(#242756,#242757),
(#242758,#242759),(#242760,#242761),(#242762,#242763),(#242764,#242765),
(#242766,#242767),(#242768,#242769),(#242770,#242771),(#242772,#242773),
(#242774,#242775),(#242776,#242777),(#242778,#242779),(#242780,#242781),
(#242782,#242783),(#242784,#242785),(#242786,#242787),(#242788,#242789),
(#242790,#242791),(#242792,#242793),(#242794,#242795),(#242796,#242797),
(#242798,#242799),(#242800,#242801),(#242802,#242803),(#242804,#242805),
(#242806,#242807),(#242808,#242809),(#242810,#242811),(#242812,#242813),
(#242814,#242815),(#242816,#242817),(#242818,#242819),(#242820,#242821),
(#242822,#242823),(#242824,#242825),(#242826,#242827),(#242828,#242829),
(#242830,#242831),(#242832,#242833),(#242834,#242835),(#242836,#242837),
(#242838,#242839),(#242840,#242841),(#242842,#242843),(#242844,#242845),
(#242846,#242847),(#242848,#242849)),.UNSPECIFIED.,.F.,.F.,.F.)
B_SPLINE_SURFACE_WITH_KNOTS((6,1,1,1,1,1,1,1,1,1,1,1,1,1,1,1,1,1,1,1,1,
1,1,1,1,1,1,1,1,1,1,1,1,1,1,1,1,1,1,1,1,1,1,1,1,1,1,1,1,1,1,1,1,1,1,1,1,
1,1,1,1,1,1,1,1,1,1,1,1,1,1,1,1,1,1,1,1,1,1,1,1,1,1,1,1,1,1,1,1,1,1,1,1,
1,1,1,1,1,1,1,1,1,1,1,1,1,1,1,1,1,1,1,1,1,1,1,1,1,1,1,1,1,1,1,1,1,1,1,1,
1,1,1,1,1,1,1,1,1,1,1,1,1,1,1,1,1,1,1,1,1,1,1,1,1,1,1,1,1,1,1,1,1,1,1,1,
1,1,1,1,1,1,1,1,1,1,1,1,1,1,1,1,1,1,1,1,1,1,1,1,1,1,1,1,1,1,1,1,1,1,1,6),
(2,2),(-1.,-0.995000000000001,-0.990000000000001,-0.985000000000001,-0.980000000000001,
-0.975000000000001,-0.970000000000001,-0.965000000000001,-0.960000000000001,
-0.955000000000001,-0.950000000000001,-0.945000000000001,-0.940000000000001,
-0.935000000000001,-0.930000000000001,-0.925000000000001,-0.920000000000001,
-0.915000000000001,-0.910000000000001,-0.905000000000001,-0.900000000000001,
-0.895000000000001,-0.890000000000001,-0.885000000000001,-0.880000000000001,
-0.875000000000001,-0.870000000000001,-0.865000000000001,-0.860000000000001,
-0.855000000000001,-0.850000000000001,-0.845000000000001,-0.840000000000001,
-0.835000000000001,-0.830000000000001,-0.825000000000001,-0.820000000000001,
-0.815000000000001,-0.810000000000001,-0.805000000000001,-0.800000000000001,
-0.795000000000001,-0.790000000000001,-0.785000000000001,-0.780000000000001,
-0.775000000000001,-0.770000000000001,-0.765000000000001,-0.760000000000001,
-0.755000000000001,-0.750000000000001,-0.745000000000001,-0.740000000000001,
-0.735000000000001,-0.730000000000001,-0.725000000000001,-0.720000000000001,
-0.715000000000001,-0.710000000000001,-0.705000000000001,-0.700000000000001,
-0.695000000000001,-0.690000000000001,-0.685,-0.68,-0.675,-0.67,-0.665,
-0.66,-0.655,-0.65,-0.645,-0.64,-0.635,-0.63,-0.625,-0.62,-0.615,-0.61,
-0.605,-0.6,-0.595,-0.59,-0.585,-0.58,-0.575,-0.57,-0.565,-0.56,-0.555,
-0.55,-0.545,-0.54,-0.535,-0.53,-0.525,-0.52,-0.515,-0.51,-0.505,-0.5,-0.495,
-0.49,-0.485,-0.48,-0.475,-0.47,-0.465,-0.46,-0.455,-0.45,-0.445,-0.44,
-0.435,-0.43,-0.425,-0.42,-0.415,-0.41,-0.405,-0.4,-0.395,-0.39,-0.385,
-0.38,-0.375,-0.37,-0.365,-0.36,-0.355,-0.35,-0.345,-0.34,-0.335,-0.33,
-0.325,-0.32,-0.315,-0.31,-0.305,-0.3,-0.295,-0.29,-0.285,-0.28,-0.275,
-0.27,-0.265,-0.26,-0.255,-0.25,-0.245,-0.24,-0.235,-0.23,-0.225,-0.22,
-0.215,-0.21,-0.205,-0.2,-0.195,-0.19,-0.185,-0.18,-0.175,-0.17,-0.165,
-0.16,-0.155,-0.15,-0.145,-0.14,-0.135,-0.13,-0.125,-0.12,-0.115,-0.11,
-0.105,-0.1,-0.095,-0.09,-0.085,-0.08,-0.075,-0.07,-0.065,-0.06,-0.055,
-0.05,-0.045,-0.04,-0.035,-0.03,-0.025,-0.02,-0.015,-0.01,-0.005,0.),(0.,
1.2),.UNSPECIFIED.)
GEOMETRIC_REPRESENTATION_ITEM()
RATIONAL_B_SPLINE_SURFACE(((1.,1.),(1.,1.),(1.,1.),(1.,1.),(1.,1.),(1.,
1.),(1.,1.),(1.,1.),(1.,1.),(1.,1.),(1.,1.),(1.,1.),(1.,1.),(1.,1.),(1.,
1.),(1.,1.),(1.,1.),(1.,1.),(1.,1.),(1.,1.),(1.,1.),(1.,1.),(1.,1.),(1.,
1.),(1.,1.),(1.,1.),(1.,1.),(1.,1.),(1.,1.),(1.,1.),(1.,1.),(1.,1.),(1.,
1.),(1.,1.),(1.,1.),(1.,1.),(1.,1.),(1.,1.),(1.,1.),(1.,1.),(1.,1.),(1.,
1.),(1.,1.),(1.,1.),(1.,1.),(1.,1.),(1.,1.),(1.,1.),(1.,1.),(1.,1.),(1.,
1.),(1.,1.),(1.,1.),(1.,1.),(1.,1.),(1.,1.),(1.,1.),(1.,1.),(1.,1.),(1.,
1.),(1.,1.),(1.,1.),(1.,1.),(1.,1.),(1.,1.),(1.,1.),(1.,1.),(1.,1.),(1.,
1.),(1.,1.),(1.,1.),(1.,1.),(1.,1.),(1.,1.),(1.,1.),(1.,1.),(1.,1.),(1.,
1.),(1.,1.),(1.,1.),(1.,1.),(1.,1.),(1.,1.),(1.,1.),(1.,1.),(1.,1.),(1.,
1.),(1.,1.),(1.,1.),(1.,1.),(1.,1.),(1.,1.),(1.,1.),(1.,1.),(1.,1.),(1.,
1.),(1.,1.),(1.,1.),(1.,1.),(1.,1.),(1.,1.),(1.,1.),(1.,1.),(1.,1.),(1.,
1.),(1.,1.),(1.,1.),(1.,1.),(1.,1.),(1.,1.),(1.,1.),(1.,1.),(1.,1.),(1.,
1.),(1.,1.),(1.,1.),(1.,1.),(1.,1.),(1.,1.),(1.,1.),(1.,1.),(1.,1.),(1.,
1.),(1.,1.),(1.,1.),(1.,1.),(1.,1.),(1.,1.),(1.,1.),(1.,1.),(1.,1.),(1.,
1.),(1.,1.),(1.,1.),(1.,1.),(1.,1.),(1.,1.),(1.,1.),(1.,1.),(1.,1.),(1.,
1.),(1.,1.),(1.,1.),(1.,1.),(1.,1.),(1.,1.),(1.,1.),(1.,1.),(1.,1.),(1.,
1.),(1.,1.),(1.,1.),(1.,1.),(1.,1.),(1.,1.),(1.,1.),(1.,1.),(1.,1.),(1.,
1.),(1.,1.),(1.,1.),(1.,1.),(1.,1.),(1.,1.),(1.,1.),(1.,1.),(1.,1.),(1.,
1.),(1.,1.),(1.,1.),(1.,1.),(1.,1.),(1.,1.),(1.,1.),(1.,1.),(1.,1.),(1.,
1.),(1.,1.),(1.,1.),(1.,1.),(1.,1.),(1.,1.),(1.,1.),(1.,1.),(1.,1.),(1.,
1.),(1.,1.),(1.,1.),(1.,1.),(1.,1.),(1.,1.),(1.,1.),(1.,1.),(1.,1.),(1.,
1.),(1.,1.),(1.,1.),(1.,1.),(1.,1.),(1.,1.),(1.,1.),(1.,1.),(1.,1.),(1.,
1.),(1.,1.)))
REPRESENTATION_ITEM('')
SURFACE()
);
#1108=(
BOUNDED_SURFACE()
B_SPLINE_SURFACE(5,1,((#243263,#243264),(#243265,#243266),(#243267,#243268),
(#243269,#243270),(#243271,#243272),(#243273,#243274),(#243275,#243276),
(#243277,#243278),(#243279,#243280),(#243281,#243282),(#243283,#243284),
(#243285,#243286),(#243287,#243288),(#243289,#243290),(#243291,#243292),
(#243293,#243294),(#243295,#243296),(#243297,#243298),(#243299,#243300),
(#243301,#243302),(#243303,#243304),(#243305,#243306),(#243307,#243308),
(#243309,#243310),(#243311,#243312),(#243313,#243314),(#243315,#243316),
(#243317,#243318),(#243319,#243320),(#243321,#243322),(#243323,#243324),
(#243325,#243326),(#243327,#243328),(#243329,#243330),(#243331,#243332),
(#243333,#243334),(#243335,#243336),(#243337,#243338),(#243339,#243340),
(#243341,#243342),(#243343,#243344),(#243345,#243346),(#243347,#243348),
(#243349,#243350),(#243351,#243352),(#243353,#243354),(#243355,#243356),
(#243357,#243358),(#243359,#243360),(#243361,#243362),(#243363,#243364),
(#243365,#243366),(#243367,#243368),(#243369,#243370),(#243371,#243372),
(#243373,#243374),(#243375,#243376),(#243377,#243378),(#243379,#243380),
(#243381,#243382),(#243383,#243384),(#243385,#243386),(#243387,#243388),
(#243389,#243390),(#243391,#243392),(#243393,#243394),(#243395,#243396),
(#243397,#243398),(#243399,#243400),(#243401,#243402),(#243403,#243404),
(#243405,#243406),(#243407,#243408),(#243409,#243410),(#243411,#243412),
(#243413,#243414),(#243415,#243416),(#243417,#243418),(#243419,#243420),
(#243421,#243422),(#243423,#243424),(#243425,#243426),(#243427,#243428),
(#243429,#243430),(#243431,#243432),(#243433,#243434),(#243435,#243436),
(#243437,#243438),(#243439,#243440),(#243441,#243442),(#243443,#243444),
(#243445,#243446),(#243447,#243448),(#243449,#243450),(#243451,#243452),
(#243453,#243454),(#243455,#243456),(#243457,#243458),(#243459,#243460),
(#243461,#243462),(#243463,#243464),(#243465,#243466),(#243467,#243468),
(#243469,#243470),(#243471,#243472),(#243473,#243474),(#243475,#243476),
(#243477,#243478),(#243479,#243480),(#243481,#243482),(#243483,#243484),
(#243485,#243486),(#243487,#243488),(#243489,#243490),(#243491,#243492),
(#243493,#243494),(#243495,#243496),(#243497,#243498),(#243499,#243500),
(#243501,#243502),(#243503,#243504),(#243505,#243506),(#243507,#243508),
(#243509,#243510),(#243511,#243512),(#243513,#243514),(#243515,#243516),
(#243517,#243518),(#243519,#243520),(#243521,#243522),(#243523,#243524),
(#243525,#243526),(#243527,#243528),(#243529,#243530),(#243531,#243532),
(#243533,#243534),(#243535,#243536),(#243537,#243538),(#243539,#243540),
(#243541,#243542),(#243543,#243544),(#243545,#243546),(#243547,#243548),
(#243549,#243550),(#243551,#243552),(#243553,#243554),(#243555,#243556),
(#243557,#243558),(#243559,#243560),(#243561,#243562),(#243563,#243564),
(#243565,#243566),(#243567,#243568),(#243569,#243570),(#243571,#243572),
(#243573,#243574),(#243575,#243576),(#243577,#243578),(#243579,#243580),
(#243581,#243582),(#243583,#243584),(#243585,#243586),(#243587,#243588),
(#243589,#243590),(#243591,#243592),(#243593,#243594),(#243595,#243596),
(#243597,#243598),(#243599,#243600),(#243601,#243602),(#243603,#243604),
(#243605,#243606),(#243607,#243608),(#243609,#243610),(#243611,#243612),
(#243613,#243614),(#243615,#243616),(#243617,#243618),(#243619,#243620),
(#243621,#243622),(#243623,#243624),(#243625,#243626),(#243627,#243628),
(#243629,#243630),(#243631,#243632),(#243633,#243634),(#243635,#243636),
(#243637,#243638),(#243639,#243640),(#243641,#243642),(#243643,#243644),
(#243645,#243646),(#243647,#243648),(#243649,#243650),(#243651,#243652),
(#243653,#243654),(#243655,#243656),(#243657,#243658),(#243659,#243660),
(#243661,#243662),(#243663,#243664),(#243665,#243666),(#243667,#243668),
(#243669,#243670),(#243671,#243672)),.UNSPECIFIED.,.F.,.F.,.F.)
B_SPLINE_SURFACE_WITH_KNOTS((6,1,1,1,1,1,1,1,1,1,1,1,1,1,1,1,1,1,1,1,1,
1,1,1,1,1,1,1,1,1,1,1,1,1,1,1,1,1,1,1,1,1,1,1,1,1,1,1,1,1,1,1,1,1,1,1,1,
1,1,1,1,1,1,1,1,1,1,1,1,1,1,1,1,1,1,1,1,1,1,1,1,1,1,1,1,1,1,1,1,1,1,1,1,
1,1,1,1,1,1,1,1,1,1,1,1,1,1,1,1,1,1,1,1,1,1,1,1,1,1,1,1,1,1,1,1,1,1,1,1,
1,1,1,1,1,1,1,1,1,1,1,1,1,1,1,1,1,1,1,1,1,1,1,1,1,1,1,1,1,1,1,1,1,1,1,1,
1,1,1,1,1,1,1,1,1,1,1,1,1,1,1,1,1,1,1,1,1,1,1,1,1,1,1,1,1,1,1,1,1,1,1,6),
(2,2),(0.,0.005,0.01,0.015,0.02,0.025,0.03,0.035,0.04,0.045,0.05,0.055,
0.06,0.065,0.07,0.075,0.08,0.085,0.09,0.095,0.1,0.105,0.11,0.115,0.12,0.125,
0.13,0.135,0.14,0.145,0.15,0.155,0.16,0.165,0.17,0.175,0.18,0.185,0.19,
0.195,0.2,0.205,0.21,0.215,0.22,0.225,0.23,0.235,0.24,0.245,0.25,0.255,
0.26,0.265,0.27,0.275,0.28,0.285,0.29,0.295,0.3,0.305,0.31,0.315,0.32,0.325,
0.33,0.335,0.34,0.345,0.35,0.355,0.36,0.365,0.37,0.375,0.38,0.385,0.39,
0.395,0.4,0.405,0.41,0.415,0.42,0.425,0.43,0.435,0.44,0.445,0.45,0.455,
0.46,0.465,0.47,0.475,0.48,0.485,0.49,0.495,0.5,0.505,0.51,0.515,0.52,0.525,
0.53,0.535,0.54,0.545,0.55,0.555,0.56,0.565,0.57,0.575,0.58,0.585,0.59,
0.595,0.6,0.605,0.61,0.615,0.62,0.625,0.63,0.635,0.64,0.645,0.65,0.655,
0.66,0.665,0.67,0.675,0.68,0.685,0.690000000000001,0.695000000000001,0.700000000000001,
0.705000000000001,0.710000000000001,0.715000000000001,0.720000000000001,
0.725000000000001,0.730000000000001,0.735000000000001,0.740000000000001,
0.745000000000001,0.750000000000001,0.755000000000001,0.760000000000001,
0.765000000000001,0.770000000000001,0.775000000000001,0.780000000000001,
0.785000000000001,0.790000000000001,0.795000000000001,0.800000000000001,
0.805000000000001,0.810000000000001,0.815000000000001,0.820000000000001,
0.825000000000001,0.830000000000001,0.835000000000001,0.840000000000001,
0.845000000000001,0.850000000000001,0.855000000000001,0.860000000000001,
0.865000000000001,0.870000000000001,0.875000000000001,0.880000000000001,
0.885000000000001,0.890000000000001,0.895000000000001,0.900000000000001,
0.905000000000001,0.910000000000001,0.915000000000001,0.920000000000001,
0.925000000000001,0.930000000000001,0.935000000000001,0.940000000000001,
0.945000000000001,0.950000000000001,0.955000000000001,0.960000000000001,
0.965000000000001,0.970000000000001,0.975000000000001,0.980000000000001,
0.985000000000001,0.990000000000001,0.995000000000001,1.),(0.,1.2),
 .UNSPECIFIED.)
GEOMETRIC_REPRESENTATION_ITEM()
RATIONAL_B_SPLINE_SURFACE(((1.,1.),(1.,1.),(1.,1.),(1.,1.),(1.,1.),(1.,
1.),(1.,1.),(1.,1.),(1.,1.),(1.,1.),(1.,1.),(1.,1.),(1.,1.),(1.,1.),(1.,
1.),(1.,1.),(1.,1.),(1.,1.),(1.,1.),(1.,1.),(1.,1.),(1.,1.),(1.,1.),(1.,
1.),(1.,1.),(1.,1.),(1.,1.),(1.,1.),(1.,1.),(1.,1.),(1.,1.),(1.,1.),(1.,
1.),(1.,1.),(1.,1.),(1.,1.),(1.,1.),(1.,1.),(1.,1.),(1.,1.),(1.,1.),(1.,
1.),(1.,1.),(1.,1.),(1.,1.),(1.,1.),(1.,1.),(1.,1.),(1.,1.),(1.,1.),(1.,
1.),(1.,1.),(1.,1.),(1.,1.),(1.,1.),(1.,1.),(1.,1.),(1.,1.),(1.,1.),(1.,
1.),(1.,1.),(1.,1.),(1.,1.),(1.,1.),(1.,1.),(1.,1.),(1.,1.),(1.,1.),(1.,
1.),(1.,1.),(1.,1.),(1.,1.),(1.,1.),(1.,1.),(1.,1.),(1.,1.),(1.,1.),(1.,
1.),(1.,1.),(1.,1.),(1.,1.),(1.,1.),(1.,1.),(1.,1.),(1.,1.),(1.,1.),(1.,
1.),(1.,1.),(1.,1.),(1.,1.),(1.,1.),(1.,1.),(1.,1.),(1.,1.),(1.,1.),(1.,
1.),(1.,1.),(1.,1.),(1.,1.),(1.,1.),(1.,1.),(1.,1.),(1.,1.),(1.,1.),(1.,
1.),(1.,1.),(1.,1.),(1.,1.),(1.,1.),(1.,1.),(1.,1.),(1.,1.),(1.,1.),(1.,
1.),(1.,1.),(1.,1.),(1.,1.),(1.,1.),(1.,1.),(1.,1.),(1.,1.),(1.,1.),(1.,
1.),(1.,1.),(1.,1.),(1.,1.),(1.,1.),(1.,1.),(1.,1.),(1.,1.),(1.,1.),(1.,
1.),(1.,1.),(1.,1.),(1.,1.),(1.,1.),(1.,1.),(1.,1.),(1.,1.),(1.,1.),(1.,
1.),(1.,1.),(1.,1.),(1.,1.),(1.,1.),(1.,1.),(1.,1.),(1.,1.),(1.,1.),(1.,
1.),(1.,1.),(1.,1.),(1.,1.),(1.,1.),(1.,1.),(1.,1.),(1.,1.),(1.,1.),(1.,
1.),(1.,1.),(1.,1.),(1.,1.),(1.,1.),(1.,1.),(1.,1.),(1.,1.),(1.,1.),(1.,
1.),(1.,1.),(1.,1.),(1.,1.),(1.,1.),(1.,1.),(1.,1.),(1.,1.),(1.,1.),(1.,
1.),(1.,1.),(1.,1.),(1.,1.),(1.,1.),(1.,1.),(1.,1.),(1.,1.),(1.,1.),(1.,
1.),(1.,1.),(1.,1.),(1.,1.),(1.,1.),(1.,1.),(1.,1.),(1.,1.),(1.,1.),(1.,
1.),(1.,1.),(1.,1.),(1.,1.),(1.,1.),(1.,1.),(1.,1.),(1.,1.),(1.,1.),(1.,
1.),(1.,1.)))
REPRESENTATION_ITEM('')
SURFACE()
);
#1109=(
BOUNDED_SURFACE()
B_SPLINE_SURFACE(5,1,((#244092,#244093),(#244094,#244095),(#244096,#244097),
(#244098,#244099),(#244100,#244101),(#244102,#244103),(#244104,#244105),
(#244106,#244107),(#244108,#244109),(#244110,#244111),(#244112,#244113),
(#244114,#244115),(#244116,#244117),(#244118,#244119),(#244120,#244121),
(#244122,#244123),(#244124,#244125),(#244126,#244127),(#244128,#244129),
(#244130,#244131),(#244132,#244133),(#244134,#244135),(#244136,#244137),
(#244138,#244139),(#244140,#244141),(#244142,#244143),(#244144,#244145),
(#244146,#244147),(#244148,#244149),(#244150,#244151),(#244152,#244153),
(#244154,#244155),(#244156,#244157),(#244158,#244159),(#244160,#244161),
(#244162,#244163),(#244164,#244165),(#244166,#244167),(#244168,#244169),
(#244170,#244171),(#244172,#244173),(#244174,#244175),(#244176,#244177),
(#244178,#244179),(#244180,#244181),(#244182,#244183),(#244184,#244185),
(#244186,#244187),(#244188,#244189),(#244190,#244191),(#244192,#244193),
(#244194,#244195),(#244196,#244197),(#244198,#244199),(#244200,#244201),
(#244202,#244203),(#244204,#244205),(#244206,#244207),(#244208,#244209),
(#244210,#244211),(#244212,#244213),(#244214,#244215),(#244216,#244217),
(#244218,#244219),(#244220,#244221),(#244222,#244223),(#244224,#244225),
(#244226,#244227),(#244228,#244229),(#244230,#244231),(#244232,#244233),
(#244234,#244235),(#244236,#244237),(#244238,#244239),(#244240,#244241),
(#244242,#244243),(#244244,#244245),(#244246,#244247),(#244248,#244249),
(#244250,#244251),(#244252,#244253),(#244254,#244255),(#244256,#244257),
(#244258,#244259),(#244260,#244261),(#244262,#244263),(#244264,#244265),
(#244266,#244267),(#244268,#244269),(#244270,#244271),(#244272,#244273),
(#244274,#244275),(#244276,#244277),(#244278,#244279),(#244280,#244281),
(#244282,#244283),(#244284,#244285),(#244286,#244287),(#244288,#244289),
(#244290,#244291),(#244292,#244293),(#244294,#244295),(#244296,#244297),
(#244298,#244299),(#244300,#244301),(#244302,#244303),(#244304,#244305),
(#244306,#244307),(#244308,#244309),(#244310,#244311),(#244312,#244313),
(#244314,#244315),(#244316,#244317),(#244318,#244319),(#244320,#244321),
(#244322,#244323),(#244324,#244325),(#244326,#244327),(#244328,#244329),
(#244330,#244331),(#244332,#244333),(#244334,#244335),(#244336,#244337),
(#244338,#244339),(#244340,#244341),(#244342,#244343),(#244344,#244345),
(#244346,#244347),(#244348,#244349),(#244350,#244351),(#244352,#244353),
(#244354,#244355),(#244356,#244357),(#244358,#244359),(#244360,#244361),
(#244362,#244363),(#244364,#244365),(#244366,#244367),(#244368,#244369),
(#244370,#244371),(#244372,#244373),(#244374,#244375),(#244376,#244377),
(#244378,#244379),(#244380,#244381),(#244382,#244383),(#244384,#244385),
(#244386,#244387),(#244388,#244389),(#244390,#244391),(#244392,#244393),
(#244394,#244395),(#244396,#244397),(#244398,#244399),(#244400,#244401),
(#244402,#244403),(#244404,#244405),(#244406,#244407),(#244408,#244409),
(#244410,#244411),(#244412,#244413),(#244414,#244415),(#244416,#244417),
(#244418,#244419),(#244420,#244421),(#244422,#244423),(#244424,#244425),
(#244426,#244427),(#244428,#244429),(#244430,#244431),(#244432,#244433),
(#244434,#244435),(#244436,#244437),(#244438,#244439),(#244440,#244441),
(#244442,#244443),(#244444,#244445),(#244446,#244447),(#244448,#244449),
(#244450,#244451),(#244452,#244453),(#244454,#244455),(#244456,#244457),
(#244458,#244459),(#244460,#244461),(#244462,#244463),(#244464,#244465),
(#244466,#244467),(#244468,#244469),(#244470,#244471),(#244472,#244473),
(#244474,#244475),(#244476,#244477),(#244478,#244479),(#244480,#244481),
(#244482,#244483),(#244484,#244485),(#244486,#244487),(#244488,#244489),
(#244490,#244491),(#244492,#244493),(#244494,#244495),(#244496,#244497),
(#244498,#244499),(#244500,#244501)),.UNSPECIFIED.,.F.,.F.,.F.)
B_SPLINE_SURFACE_WITH_KNOTS((6,1,1,1,1,1,1,1,1,1,1,1,1,1,1,1,1,1,1,1,1,
1,1,1,1,1,1,1,1,1,1,1,1,1,1,1,1,1,1,1,1,1,1,1,1,1,1,1,1,1,1,1,1,1,1,1,1,
1,1,1,1,1,1,1,1,1,1,1,1,1,1,1,1,1,1,1,1,1,1,1,1,1,1,1,1,1,1,1,1,1,1,1,1,
1,1,1,1,1,1,1,1,1,1,1,1,1,1,1,1,1,1,1,1,1,1,1,1,1,1,1,1,1,1,1,1,1,1,1,1,
1,1,1,1,1,1,1,1,1,1,1,1,1,1,1,1,1,1,1,1,1,1,1,1,1,1,1,1,1,1,1,1,1,1,1,1,
1,1,1,1,1,1,1,1,1,1,1,1,1,1,1,1,1,1,1,1,1,1,1,1,1,1,1,1,1,1,1,1,1,1,1,6),
(2,2),(-1.,-0.995000000000001,-0.990000000000001,-0.985000000000001,-0.980000000000001,
-0.975000000000001,-0.970000000000001,-0.965000000000001,-0.960000000000001,
-0.955000000000001,-0.950000000000001,-0.945000000000001,-0.940000000000001,
-0.935000000000001,-0.930000000000001,-0.925000000000001,-0.920000000000001,
-0.915000000000001,-0.910000000000001,-0.905000000000001,-0.900000000000001,
-0.895000000000001,-0.890000000000001,-0.885000000000001,-0.880000000000001,
-0.875000000000001,-0.870000000000001,-0.865000000000001,-0.860000000000001,
-0.855000000000001,-0.850000000000001,-0.845000000000001,-0.840000000000001,
-0.835000000000001,-0.830000000000001,-0.825000000000001,-0.820000000000001,
-0.815000000000001,-0.810000000000001,-0.805000000000001,-0.800000000000001,
-0.795000000000001,-0.790000000000001,-0.785000000000001,-0.780000000000001,
-0.775000000000001,-0.770000000000001,-0.765000000000001,-0.760000000000001,
-0.755000000000001,-0.750000000000001,-0.745000000000001,-0.740000000000001,
-0.735000000000001,-0.730000000000001,-0.725000000000001,-0.720000000000001,
-0.715000000000001,-0.710000000000001,-0.705000000000001,-0.700000000000001,
-0.695000000000001,-0.690000000000001,-0.685,-0.68,-0.675,-0.67,-0.665,
-0.66,-0.655,-0.65,-0.645,-0.64,-0.635,-0.63,-0.625,-0.62,-0.615,-0.61,
-0.605,-0.6,-0.595,-0.59,-0.585,-0.58,-0.575,-0.57,-0.565,-0.56,-0.555,
-0.55,-0.545,-0.54,-0.535,-0.53,-0.525,-0.52,-0.515,-0.51,-0.505,-0.5,-0.495,
-0.49,-0.485,-0.48,-0.475,-0.47,-0.465,-0.46,-0.455,-0.45,-0.445,-0.44,
-0.435,-0.43,-0.425,-0.42,-0.415,-0.41,-0.405,-0.4,-0.395,-0.39,-0.385,
-0.38,-0.375,-0.37,-0.365,-0.36,-0.355,-0.35,-0.345,-0.34,-0.335,-0.33,
-0.325,-0.32,-0.315,-0.31,-0.305,-0.3,-0.295,-0.29,-0.285,-0.28,-0.275,
-0.27,-0.265,-0.26,-0.255,-0.25,-0.245,-0.24,-0.235,-0.23,-0.225,-0.22,
-0.215,-0.21,-0.205,-0.2,-0.195,-0.19,-0.185,-0.18,-0.175,-0.17,-0.165,
-0.16,-0.155,-0.15,-0.145,-0.14,-0.135,-0.13,-0.125,-0.12,-0.115,-0.11,
-0.105,-0.1,-0.095,-0.09,-0.085,-0.08,-0.075,-0.07,-0.065,-0.06,-0.055,
-0.05,-0.045,-0.04,-0.035,-0.03,-0.025,-0.02,-0.015,-0.01,-0.005,0.),(0.,
1.2),.UNSPECIFIED.)
GEOMETRIC_REPRESENTATION_ITEM()
RATIONAL_B_SPLINE_SURFACE(((1.,1.),(1.,1.),(1.,1.),(1.,1.),(1.,1.),(1.,
1.),(1.,1.),(1.,1.),(1.,1.),(1.,1.),(1.,1.),(1.,1.),(1.,1.),(1.,1.),(1.,
1.),(1.,1.),(1.,1.),(1.,1.),(1.,1.),(1.,1.),(1.,1.),(1.,1.),(1.,1.),(1.,
1.),(1.,1.),(1.,1.),(1.,1.),(1.,1.),(1.,1.),(1.,1.),(1.,1.),(1.,1.),(1.,
1.),(1.,1.),(1.,1.),(1.,1.),(1.,1.),(1.,1.),(1.,1.),(1.,1.),(1.,1.),(1.,
1.),(1.,1.),(1.,1.),(1.,1.),(1.,1.),(1.,1.),(1.,1.),(1.,1.),(1.,1.),(1.,
1.),(1.,1.),(1.,1.),(1.,1.),(1.,1.),(1.,1.),(1.,1.),(1.,1.),(1.,1.),(1.,
1.),(1.,1.),(1.,1.),(1.,1.),(1.,1.),(1.,1.),(1.,1.),(1.,1.),(1.,1.),(1.,
1.),(1.,1.),(1.,1.),(1.,1.),(1.,1.),(1.,1.),(1.,1.),(1.,1.),(1.,1.),(1.,
1.),(1.,1.),(1.,1.),(1.,1.),(1.,1.),(1.,1.),(1.,1.),(1.,1.),(1.,1.),(1.,
1.),(1.,1.),(1.,1.),(1.,1.),(1.,1.),(1.,1.),(1.,1.),(1.,1.),(1.,1.),(1.,
1.),(1.,1.),(1.,1.),(1.,1.),(1.,1.),(1.,1.),(1.,1.),(1.,1.),(1.,1.),(1.,
1.),(1.,1.),(1.,1.),(1.,1.),(1.,1.),(1.,1.),(1.,1.),(1.,1.),(1.,1.),(1.,
1.),(1.,1.),(1.,1.),(1.,1.),(1.,1.),(1.,1.),(1.,1.),(1.,1.),(1.,1.),(1.,
1.),(1.,1.),(1.,1.),(1.,1.),(1.,1.),(1.,1.),(1.,1.),(1.,1.),(1.,1.),(1.,
1.),(1.,1.),(1.,1.),(1.,1.),(1.,1.),(1.,1.),(1.,1.),(1.,1.),(1.,1.),(1.,
1.),(1.,1.),(1.,1.),(1.,1.),(1.,1.),(1.,1.),(1.,1.),(1.,1.),(1.,1.),(1.,
1.),(1.,1.),(1.,1.),(1.,1.),(1.,1.),(1.,1.),(1.,1.),(1.,1.),(1.,1.),(1.,
1.),(1.,1.),(1.,1.),(1.,1.),(1.,1.),(1.,1.),(1.,1.),(1.,1.),(1.,1.),(1.,
1.),(1.,1.),(1.,1.),(1.,1.),(1.,1.),(1.,1.),(1.,1.),(1.,1.),(1.,1.),(1.,
1.),(1.,1.),(1.,1.),(1.,1.),(1.,1.),(1.,1.),(1.,1.),(1.,1.),(1.,1.),(1.,
1.),(1.,1.),(1.,1.),(1.,1.),(1.,1.),(1.,1.),(1.,1.),(1.,1.),(1.,1.),(1.,
1.),(1.,1.),(1.,1.),(1.,1.),(1.,1.),(1.,1.),(1.,1.),(1.,1.),(1.,1.),(1.,
1.),(1.,1.)))
REPRESENTATION_ITEM('')
SURFACE()
);
#1110=(
BOUNDED_SURFACE()
B_SPLINE_SURFACE(5,1,((#244915,#244916),(#244917,#244918),(#244919,#244920),
(#244921,#244922),(#244923,#244924),(#244925,#244926),(#244927,#244928),
(#244929,#244930),(#244931,#244932),(#244933,#244934),(#244935,#244936),
(#244937,#244938),(#244939,#244940),(#244941,#244942),(#244943,#244944),
(#244945,#244946),(#244947,#244948),(#244949,#244950),(#244951,#244952),
(#244953,#244954),(#244955,#244956),(#244957,#244958),(#244959,#244960),
(#244961,#244962),(#244963,#244964),(#244965,#244966),(#244967,#244968),
(#244969,#244970),(#244971,#244972),(#244973,#244974),(#244975,#244976),
(#244977,#244978),(#244979,#244980),(#244981,#244982),(#244983,#244984),
(#244985,#244986),(#244987,#244988),(#244989,#244990),(#244991,#244992),
(#244993,#244994),(#244995,#244996),(#244997,#244998),(#244999,#245000),
(#245001,#245002),(#245003,#245004),(#245005,#245006),(#245007,#245008),
(#245009,#245010),(#245011,#245012),(#245013,#245014),(#245015,#245016),
(#245017,#245018),(#245019,#245020),(#245021,#245022),(#245023,#245024),
(#245025,#245026),(#245027,#245028),(#245029,#245030),(#245031,#245032),
(#245033,#245034),(#245035,#245036),(#245037,#245038),(#245039,#245040),
(#245041,#245042),(#245043,#245044),(#245045,#245046),(#245047,#245048),
(#245049,#245050),(#245051,#245052),(#245053,#245054),(#245055,#245056),
(#245057,#245058),(#245059,#245060),(#245061,#245062),(#245063,#245064),
(#245065,#245066),(#245067,#245068),(#245069,#245070),(#245071,#245072),
(#245073,#245074),(#245075,#245076),(#245077,#245078),(#245079,#245080),
(#245081,#245082),(#245083,#245084),(#245085,#245086),(#245087,#245088),
(#245089,#245090),(#245091,#245092),(#245093,#245094),(#245095,#245096),
(#245097,#245098),(#245099,#245100),(#245101,#245102),(#245103,#245104),
(#245105,#245106),(#245107,#245108),(#245109,#245110),(#245111,#245112),
(#245113,#245114),(#245115,#245116),(#245117,#245118),(#245119,#245120),
(#245121,#245122),(#245123,#245124),(#245125,#245126),(#245127,#245128),
(#245129,#245130),(#245131,#245132),(#245133,#245134),(#245135,#245136),
(#245137,#245138),(#245139,#245140),(#245141,#245142),(#245143,#245144),
(#245145,#245146),(#245147,#245148),(#245149,#245150),(#245151,#245152),
(#245153,#245154),(#245155,#245156),(#245157,#245158),(#245159,#245160),
(#245161,#245162),(#245163,#245164),(#245165,#245166),(#245167,#245168),
(#245169,#245170),(#245171,#245172),(#245173,#245174),(#245175,#245176),
(#245177,#245178),(#245179,#245180),(#245181,#245182),(#245183,#245184),
(#245185,#245186),(#245187,#245188),(#245189,#245190),(#245191,#245192),
(#245193,#245194),(#245195,#245196),(#245197,#245198),(#245199,#245200),
(#245201,#245202),(#245203,#245204),(#245205,#245206),(#245207,#245208),
(#245209,#245210),(#245211,#245212),(#245213,#245214),(#245215,#245216),
(#245217,#245218),(#245219,#245220),(#245221,#245222),(#245223,#245224),
(#245225,#245226),(#245227,#245228),(#245229,#245230),(#245231,#245232),
(#245233,#245234),(#245235,#245236),(#245237,#245238),(#245239,#245240),
(#245241,#245242),(#245243,#245244),(#245245,#245246),(#245247,#245248),
(#245249,#245250),(#245251,#245252),(#245253,#245254),(#245255,#245256),
(#245257,#245258),(#245259,#245260),(#245261,#245262),(#245263,#245264),
(#245265,#245266),(#245267,#245268),(#245269,#245270),(#245271,#245272),
(#245273,#245274),(#245275,#245276),(#245277,#245278),(#245279,#245280),
(#245281,#245282),(#245283,#245284),(#245285,#245286),(#245287,#245288),
(#245289,#245290),(#245291,#245292),(#245293,#245294),(#245295,#245296),
(#245297,#245298),(#245299,#245300),(#245301,#245302),(#245303,#245304),
(#245305,#245306),(#245307,#245308),(#245309,#245310),(#245311,#245312),
(#245313,#245314),(#245315,#245316),(#245317,#245318),(#245319,#245320),
(#245321,#245322),(#245323,#245324)),.UNSPECIFIED.,.F.,.F.,.F.)
B_SPLINE_SURFACE_WITH_KNOTS((6,1,1,1,1,1,1,1,1,1,1,1,1,1,1,1,1,1,1,1,1,
1,1,1,1,1,1,1,1,1,1,1,1,1,1,1,1,1,1,1,1,1,1,1,1,1,1,1,1,1,1,1,1,1,1,1,1,
1,1,1,1,1,1,1,1,1,1,1,1,1,1,1,1,1,1,1,1,1,1,1,1,1,1,1,1,1,1,1,1,1,1,1,1,
1,1,1,1,1,1,1,1,1,1,1,1,1,1,1,1,1,1,1,1,1,1,1,1,1,1,1,1,1,1,1,1,1,1,1,1,
1,1,1,1,1,1,1,1,1,1,1,1,1,1,1,1,1,1,1,1,1,1,1,1,1,1,1,1,1,1,1,1,1,1,1,1,
1,1,1,1,1,1,1,1,1,1,1,1,1,1,1,1,1,1,1,1,1,1,1,1,1,1,1,1,1,1,1,1,1,1,1,6),
(2,2),(0.,0.005,0.01,0.015,0.02,0.025,0.03,0.035,0.04,0.045,0.05,0.055,
0.06,0.065,0.07,0.075,0.08,0.085,0.09,0.095,0.1,0.105,0.11,0.115,0.12,0.125,
0.13,0.135,0.14,0.145,0.15,0.155,0.16,0.165,0.17,0.175,0.18,0.185,0.19,
0.195,0.2,0.205,0.21,0.215,0.22,0.225,0.23,0.235,0.24,0.245,0.25,0.255,
0.26,0.265,0.27,0.275,0.28,0.285,0.29,0.295,0.3,0.305,0.31,0.315,0.32,0.325,
0.33,0.335,0.34,0.345,0.35,0.355,0.36,0.365,0.37,0.375,0.38,0.385,0.39,
0.395,0.4,0.405,0.41,0.415,0.42,0.425,0.43,0.435,0.44,0.445,0.45,0.455,
0.46,0.465,0.47,0.475,0.48,0.485,0.49,0.495,0.5,0.505,0.51,0.515,0.52,0.525,
0.53,0.535,0.54,0.545,0.55,0.555,0.56,0.565,0.57,0.575,0.58,0.585,0.59,
0.595,0.6,0.605,0.61,0.615,0.62,0.625,0.63,0.635,0.64,0.645,0.65,0.655,
0.66,0.665,0.67,0.675,0.68,0.685,0.690000000000001,0.695000000000001,0.700000000000001,
0.705000000000001,0.710000000000001,0.715000000000001,0.720000000000001,
0.725000000000001,0.730000000000001,0.735000000000001,0.740000000000001,
0.745000000000001,0.750000000000001,0.755000000000001,0.760000000000001,
0.765000000000001,0.770000000000001,0.775000000000001,0.780000000000001,
0.785000000000001,0.790000000000001,0.795000000000001,0.800000000000001,
0.805000000000001,0.810000000000001,0.815000000000001,0.820000000000001,
0.825000000000001,0.830000000000001,0.835000000000001,0.840000000000001,
0.845000000000001,0.850000000000001,0.855000000000001,0.860000000000001,
0.865000000000001,0.870000000000001,0.875000000000001,0.880000000000001,
0.885000000000001,0.890000000000001,0.895000000000001,0.900000000000001,
0.905000000000001,0.910000000000001,0.915000000000001,0.920000000000001,
0.925000000000001,0.930000000000001,0.935000000000001,0.940000000000001,
0.945000000000001,0.950000000000001,0.955000000000001,0.960000000000001,
0.965000000000001,0.970000000000001,0.975000000000001,0.980000000000001,
0.985000000000001,0.990000000000001,0.995000000000001,1.),(0.,1.2),
 .UNSPECIFIED.)
GEOMETRIC_REPRESENTATION_ITEM()
RATIONAL_B_SPLINE_SURFACE(((1.,1.),(1.,1.),(1.,1.),(1.,1.),(1.,1.),(1.,
1.),(1.,1.),(1.,1.),(1.,1.),(1.,1.),(1.,1.),(1.,1.),(1.,1.),(1.,1.),(1.,
1.),(1.,1.),(1.,1.),(1.,1.),(1.,1.),(1.,1.),(1.,1.),(1.,1.),(1.,1.),(1.,
1.),(1.,1.),(1.,1.),(1.,1.),(1.,1.),(1.,1.),(1.,1.),(1.,1.),(1.,1.),(1.,
1.),(1.,1.),(1.,1.),(1.,1.),(1.,1.),(1.,1.),(1.,1.),(1.,1.),(1.,1.),(1.,
1.),(1.,1.),(1.,1.),(1.,1.),(1.,1.),(1.,1.),(1.,1.),(1.,1.),(1.,1.),(1.,
1.),(1.,1.),(1.,1.),(1.,1.),(1.,1.),(1.,1.),(1.,1.),(1.,1.),(1.,1.),(1.,
1.),(1.,1.),(1.,1.),(1.,1.),(1.,1.),(1.,1.),(1.,1.),(1.,1.),(1.,1.),(1.,
1.),(1.,1.),(1.,1.),(1.,1.),(1.,1.),(1.,1.),(1.,1.),(1.,1.),(1.,1.),(1.,
1.),(1.,1.),(1.,1.),(1.,1.),(1.,1.),(1.,1.),(1.,1.),(1.,1.),(1.,1.),(1.,
1.),(1.,1.),(1.,1.),(1.,1.),(1.,1.),(1.,1.),(1.,1.),(1.,1.),(1.,1.),(1.,
1.),(1.,1.),(1.,1.),(1.,1.),(1.,1.),(1.,1.),(1.,1.),(1.,1.),(1.,1.),(1.,
1.),(1.,1.),(1.,1.),(1.,1.),(1.,1.),(1.,1.),(1.,1.),(1.,1.),(1.,1.),(1.,
1.),(1.,1.),(1.,1.),(1.,1.),(1.,1.),(1.,1.),(1.,1.),(1.,1.),(1.,1.),(1.,
1.),(1.,1.),(1.,1.),(1.,1.),(1.,1.),(1.,1.),(1.,1.),(1.,1.),(1.,1.),(1.,
1.),(1.,1.),(1.,1.),(1.,1.),(1.,1.),(1.,1.),(1.,1.),(1.,1.),(1.,1.),(1.,
1.),(1.,1.),(1.,1.),(1.,1.),(1.,1.),(1.,1.),(1.,1.),(1.,1.),(1.,1.),(1.,
1.),(1.,1.),(1.,1.),(1.,1.),(1.,1.),(1.,1.),(1.,1.),(1.,1.),(1.,1.),(1.,
1.),(1.,1.),(1.,1.),(1.,1.),(1.,1.),(1.,1.),(1.,1.),(1.,1.),(1.,1.),(1.,
1.),(1.,1.),(1.,1.),(1.,1.),(1.,1.),(1.,1.),(1.,1.),(1.,1.),(1.,1.),(1.,
1.),(1.,1.),(1.,1.),(1.,1.),(1.,1.),(1.,1.),(1.,1.),(1.,1.),(1.,1.),(1.,
1.),(1.,1.),(1.,1.),(1.,1.),(1.,1.),(1.,1.),(1.,1.),(1.,1.),(1.,1.),(1.,
1.),(1.,1.),(1.,1.),(1.,1.),(1.,1.),(1.,1.),(1.,1.),(1.,1.),(1.,1.),(1.,
1.),(1.,1.)))
REPRESENTATION_ITEM('')
SURFACE()
);
#1111=(
BOUNDED_SURFACE()
B_SPLINE_SURFACE(5,1,((#245744,#245745),(#245746,#245747),(#245748,#245749),
(#245750,#245751),(#245752,#245753),(#245754,#245755),(#245756,#245757),
(#245758,#245759),(#245760,#245761),(#245762,#245763),(#245764,#245765),
(#245766,#245767),(#245768,#245769),(#245770,#245771),(#245772,#245773),
(#245774,#245775),(#245776,#245777),(#245778,#245779),(#245780,#245781),
(#245782,#245783),(#245784,#245785),(#245786,#245787),(#245788,#245789),
(#245790,#245791),(#245792,#245793),(#245794,#245795),(#245796,#245797),
(#245798,#245799),(#245800,#245801),(#245802,#245803),(#245804,#245805),
(#245806,#245807),(#245808,#245809),(#245810,#245811),(#245812,#245813),
(#245814,#245815),(#245816,#245817),(#245818,#245819),(#245820,#245821),
(#245822,#245823),(#245824,#245825),(#245826,#245827),(#245828,#245829),
(#245830,#245831),(#245832,#245833),(#245834,#245835),(#245836,#245837),
(#245838,#245839),(#245840,#245841),(#245842,#245843),(#245844,#245845),
(#245846,#245847),(#245848,#245849),(#245850,#245851),(#245852,#245853),
(#245854,#245855),(#245856,#245857),(#245858,#245859),(#245860,#245861),
(#245862,#245863),(#245864,#245865),(#245866,#245867),(#245868,#245869),
(#245870,#245871),(#245872,#245873),(#245874,#245875),(#245876,#245877),
(#245878,#245879),(#245880,#245881),(#245882,#245883),(#245884,#245885),
(#245886,#245887),(#245888,#245889),(#245890,#245891),(#245892,#245893),
(#245894,#245895),(#245896,#245897),(#245898,#245899),(#245900,#245901),
(#245902,#245903),(#245904,#245905),(#245906,#245907),(#245908,#245909),
(#245910,#245911),(#245912,#245913),(#245914,#245915),(#245916,#245917),
(#245918,#245919),(#245920,#245921),(#245922,#245923),(#245924,#245925),
(#245926,#245927),(#245928,#245929),(#245930,#245931),(#245932,#245933),
(#245934,#245935),(#245936,#245937),(#245938,#245939),(#245940,#245941),
(#245942,#245943),(#245944,#245945),(#245946,#245947),(#245948,#245949),
(#245950,#245951),(#245952,#245953),(#245954,#245955),(#245956,#245957),
(#245958,#245959),(#245960,#245961),(#245962,#245963),(#245964,#245965),
(#245966,#245967),(#245968,#245969),(#245970,#245971),(#245972,#245973),
(#245974,#245975),(#245976,#245977),(#245978,#245979),(#245980,#245981),
(#245982,#245983),(#245984,#245985),(#245986,#245987),(#245988,#245989),
(#245990,#245991),(#245992,#245993),(#245994,#245995),(#245996,#245997),
(#245998,#245999),(#246000,#246001),(#246002,#246003),(#246004,#246005),
(#246006,#246007),(#246008,#246009),(#246010,#246011),(#246012,#246013),
(#246014,#246015),(#246016,#246017),(#246018,#246019),(#246020,#246021),
(#246022,#246023),(#246024,#246025),(#246026,#246027),(#246028,#246029),
(#246030,#246031),(#246032,#246033),(#246034,#246035),(#246036,#246037),
(#246038,#246039),(#246040,#246041),(#246042,#246043),(#246044,#246045),
(#246046,#246047),(#246048,#246049),(#246050,#246051),(#246052,#246053),
(#246054,#246055),(#246056,#246057),(#246058,#246059),(#246060,#246061),
(#246062,#246063),(#246064,#246065),(#246066,#246067),(#246068,#246069),
(#246070,#246071),(#246072,#246073),(#246074,#246075),(#246076,#246077),
(#246078,#246079),(#246080,#246081),(#246082,#246083),(#246084,#246085),
(#246086,#246087),(#246088,#246089),(#246090,#246091),(#246092,#246093),
(#246094,#246095),(#246096,#246097),(#246098,#246099),(#246100,#246101),
(#246102,#246103),(#246104,#246105),(#246106,#246107),(#246108,#246109),
(#246110,#246111),(#246112,#246113),(#246114,#246115),(#246116,#246117),
(#246118,#246119),(#246120,#246121),(#246122,#246123),(#246124,#246125),
(#246126,#246127),(#246128,#246129),(#246130,#246131),(#246132,#246133),
(#246134,#246135),(#246136,#246137),(#246138,#246139),(#246140,#246141),
(#246142,#246143),(#246144,#246145),(#246146,#246147),(#246148,#246149),
(#246150,#246151),(#246152,#246153)),.UNSPECIFIED.,.F.,.F.,.F.)
B_SPLINE_SURFACE_WITH_KNOTS((6,1,1,1,1,1,1,1,1,1,1,1,1,1,1,1,1,1,1,1,1,
1,1,1,1,1,1,1,1,1,1,1,1,1,1,1,1,1,1,1,1,1,1,1,1,1,1,1,1,1,1,1,1,1,1,1,1,
1,1,1,1,1,1,1,1,1,1,1,1,1,1,1,1,1,1,1,1,1,1,1,1,1,1,1,1,1,1,1,1,1,1,1,1,
1,1,1,1,1,1,1,1,1,1,1,1,1,1,1,1,1,1,1,1,1,1,1,1,1,1,1,1,1,1,1,1,1,1,1,1,
1,1,1,1,1,1,1,1,1,1,1,1,1,1,1,1,1,1,1,1,1,1,1,1,1,1,1,1,1,1,1,1,1,1,1,1,
1,1,1,1,1,1,1,1,1,1,1,1,1,1,1,1,1,1,1,1,1,1,1,1,1,1,1,1,1,1,1,1,1,1,1,6),
(2,2),(-1.,-0.995000000000001,-0.990000000000001,-0.985000000000001,-0.980000000000001,
-0.975000000000001,-0.970000000000001,-0.965000000000001,-0.960000000000001,
-0.955000000000001,-0.950000000000001,-0.945000000000001,-0.940000000000001,
-0.935000000000001,-0.930000000000001,-0.925000000000001,-0.920000000000001,
-0.915000000000001,-0.910000000000001,-0.905000000000001,-0.900000000000001,
-0.895000000000001,-0.890000000000001,-0.885000000000001,-0.880000000000001,
-0.875000000000001,-0.870000000000001,-0.865000000000001,-0.860000000000001,
-0.855000000000001,-0.850000000000001,-0.845000000000001,-0.840000000000001,
-0.835000000000001,-0.830000000000001,-0.825000000000001,-0.820000000000001,
-0.815000000000001,-0.810000000000001,-0.805000000000001,-0.800000000000001,
-0.795000000000001,-0.790000000000001,-0.785000000000001,-0.780000000000001,
-0.775000000000001,-0.770000000000001,-0.765000000000001,-0.760000000000001,
-0.755000000000001,-0.750000000000001,-0.745000000000001,-0.740000000000001,
-0.735000000000001,-0.730000000000001,-0.725000000000001,-0.720000000000001,
-0.715000000000001,-0.710000000000001,-0.705000000000001,-0.700000000000001,
-0.695000000000001,-0.690000000000001,-0.685,-0.68,-0.675,-0.67,-0.665,
-0.66,-0.655,-0.65,-0.645,-0.64,-0.635,-0.63,-0.625,-0.62,-0.615,-0.61,
-0.605,-0.6,-0.595,-0.59,-0.585,-0.58,-0.575,-0.57,-0.565,-0.56,-0.555,
-0.55,-0.545,-0.54,-0.535,-0.53,-0.525,-0.52,-0.515,-0.51,-0.505,-0.5,-0.495,
-0.49,-0.485,-0.48,-0.475,-0.47,-0.465,-0.46,-0.455,-0.45,-0.445,-0.44,
-0.435,-0.43,-0.425,-0.42,-0.415,-0.41,-0.405,-0.4,-0.395,-0.39,-0.385,
-0.38,-0.375,-0.37,-0.365,-0.36,-0.355,-0.35,-0.345,-0.34,-0.335,-0.33,
-0.325,-0.32,-0.315,-0.31,-0.305,-0.3,-0.295,-0.29,-0.285,-0.28,-0.275,
-0.27,-0.265,-0.26,-0.255,-0.25,-0.245,-0.24,-0.235,-0.23,-0.225,-0.22,
-0.215,-0.21,-0.205,-0.2,-0.195,-0.19,-0.185,-0.18,-0.175,-0.17,-0.165,
-0.16,-0.155,-0.15,-0.145,-0.14,-0.135,-0.13,-0.125,-0.12,-0.115,-0.11,
-0.105,-0.1,-0.095,-0.09,-0.085,-0.08,-0.075,-0.07,-0.065,-0.06,-0.055,
-0.05,-0.045,-0.04,-0.035,-0.03,-0.025,-0.02,-0.015,-0.01,-0.005,0.),(0.,
1.2),.UNSPECIFIED.)
GEOMETRIC_REPRESENTATION_ITEM()
RATIONAL_B_SPLINE_SURFACE(((1.,1.),(1.,1.),(1.,1.),(1.,1.),(1.,1.),(1.,
1.),(1.,1.),(1.,1.),(1.,1.),(1.,1.),(1.,1.),(1.,1.),(1.,1.),(1.,1.),(1.,
1.),(1.,1.),(1.,1.),(1.,1.),(1.,1.),(1.,1.),(1.,1.),(1.,1.),(1.,1.),(1.,
1.),(1.,1.),(1.,1.),(1.,1.),(1.,1.),(1.,1.),(1.,1.),(1.,1.),(1.,1.),(1.,
1.),(1.,1.),(1.,1.),(1.,1.),(1.,1.),(1.,1.),(1.,1.),(1.,1.),(1.,1.),(1.,
1.),(1.,1.),(1.,1.),(1.,1.),(1.,1.),(1.,1.),(1.,1.),(1.,1.),(1.,1.),(1.,
1.),(1.,1.),(1.,1.),(1.,1.),(1.,1.),(1.,1.),(1.,1.),(1.,1.),(1.,1.),(1.,
1.),(1.,1.),(1.,1.),(1.,1.),(1.,1.),(1.,1.),(1.,1.),(1.,1.),(1.,1.),(1.,
1.),(1.,1.),(1.,1.),(1.,1.),(1.,1.),(1.,1.),(1.,1.),(1.,1.),(1.,1.),(1.,
1.),(1.,1.),(1.,1.),(1.,1.),(1.,1.),(1.,1.),(1.,1.),(1.,1.),(1.,1.),(1.,
1.),(1.,1.),(1.,1.),(1.,1.),(1.,1.),(1.,1.),(1.,1.),(1.,1.),(1.,1.),(1.,
1.),(1.,1.),(1.,1.),(1.,1.),(1.,1.),(1.,1.),(1.,1.),(1.,1.),(1.,1.),(1.,
1.),(1.,1.),(1.,1.),(1.,1.),(1.,1.),(1.,1.),(1.,1.),(1.,1.),(1.,1.),(1.,
1.),(1.,1.),(1.,1.),(1.,1.),(1.,1.),(1.,1.),(1.,1.),(1.,1.),(1.,1.),(1.,
1.),(1.,1.),(1.,1.),(1.,1.),(1.,1.),(1.,1.),(1.,1.),(1.,1.),(1.,1.),(1.,
1.),(1.,1.),(1.,1.),(1.,1.),(1.,1.),(1.,1.),(1.,1.),(1.,1.),(1.,1.),(1.,
1.),(1.,1.),(1.,1.),(1.,1.),(1.,1.),(1.,1.),(1.,1.),(1.,1.),(1.,1.),(1.,
1.),(1.,1.),(1.,1.),(1.,1.),(1.,1.),(1.,1.),(1.,1.),(1.,1.),(1.,1.),(1.,
1.),(1.,1.),(1.,1.),(1.,1.),(1.,1.),(1.,1.),(1.,1.),(1.,1.),(1.,1.),(1.,
1.),(1.,1.),(1.,1.),(1.,1.),(1.,1.),(1.,1.),(1.,1.),(1.,1.),(1.,1.),(1.,
1.),(1.,1.),(1.,1.),(1.,1.),(1.,1.),(1.,1.),(1.,1.),(1.,1.),(1.,1.),(1.,
1.),(1.,1.),(1.,1.),(1.,1.),(1.,1.),(1.,1.),(1.,1.),(1.,1.),(1.,1.),(1.,
1.),(1.,1.),(1.,1.),(1.,1.),(1.,1.),(1.,1.),(1.,1.),(1.,1.),(1.,1.),(1.,
1.),(1.,1.)))
REPRESENTATION_ITEM('')
SURFACE()
);
#1112=(
BOUNDED_SURFACE()
B_SPLINE_SURFACE(5,1,((#246567,#246568),(#246569,#246570),(#246571,#246572),
(#246573,#246574),(#246575,#246576),(#246577,#246578),(#246579,#246580),
(#246581,#246582),(#246583,#246584),(#246585,#246586),(#246587,#246588),
(#246589,#246590),(#246591,#246592),(#246593,#246594),(#246595,#246596),
(#246597,#246598),(#246599,#246600),(#246601,#246602),(#246603,#246604),
(#246605,#246606),(#246607,#246608),(#246609,#246610),(#246611,#246612),
(#246613,#246614),(#246615,#246616),(#246617,#246618),(#246619,#246620),
(#246621,#246622),(#246623,#246624),(#246625,#246626),(#246627,#246628),
(#246629,#246630),(#246631,#246632),(#246633,#246634),(#246635,#246636),
(#246637,#246638),(#246639,#246640),(#246641,#246642),(#246643,#246644),
(#246645,#246646),(#246647,#246648),(#246649,#246650),(#246651,#246652),
(#246653,#246654),(#246655,#246656),(#246657,#246658),(#246659,#246660),
(#246661,#246662),(#246663,#246664),(#246665,#246666),(#246667,#246668),
(#246669,#246670),(#246671,#246672),(#246673,#246674),(#246675,#246676),
(#246677,#246678),(#246679,#246680),(#246681,#246682),(#246683,#246684),
(#246685,#246686),(#246687,#246688),(#246689,#246690),(#246691,#246692),
(#246693,#246694),(#246695,#246696),(#246697,#246698),(#246699,#246700),
(#246701,#246702),(#246703,#246704),(#246705,#246706),(#246707,#246708),
(#246709,#246710),(#246711,#246712),(#246713,#246714),(#246715,#246716),
(#246717,#246718),(#246719,#246720),(#246721,#246722),(#246723,#246724),
(#246725,#246726),(#246727,#246728),(#246729,#246730),(#246731,#246732),
(#246733,#246734),(#246735,#246736),(#246737,#246738),(#246739,#246740),
(#246741,#246742),(#246743,#246744),(#246745,#246746),(#246747,#246748),
(#246749,#246750),(#246751,#246752),(#246753,#246754),(#246755,#246756),
(#246757,#246758),(#246759,#246760),(#246761,#246762),(#246763,#246764),
(#246765,#246766),(#246767,#246768),(#246769,#246770),(#246771,#246772),
(#246773,#246774),(#246775,#246776),(#246777,#246778),(#246779,#246780),
(#246781,#246782),(#246783,#246784),(#246785,#246786),(#246787,#246788),
(#246789,#246790),(#246791,#246792),(#246793,#246794),(#246795,#246796),
(#246797,#246798),(#246799,#246800),(#246801,#246802),(#246803,#246804),
(#246805,#246806),(#246807,#246808),(#246809,#246810),(#246811,#246812),
(#246813,#246814),(#246815,#246816),(#246817,#246818),(#246819,#246820),
(#246821,#246822),(#246823,#246824),(#246825,#246826),(#246827,#246828),
(#246829,#246830),(#246831,#246832),(#246833,#246834),(#246835,#246836),
(#246837,#246838),(#246839,#246840),(#246841,#246842),(#246843,#246844),
(#246845,#246846),(#246847,#246848),(#246849,#246850),(#246851,#246852),
(#246853,#246854),(#246855,#246856),(#246857,#246858),(#246859,#246860),
(#246861,#246862),(#246863,#246864),(#246865,#246866),(#246867,#246868),
(#246869,#246870),(#246871,#246872),(#246873,#246874),(#246875,#246876),
(#246877,#246878),(#246879,#246880),(#246881,#246882),(#246883,#246884),
(#246885,#246886),(#246887,#246888),(#246889,#246890),(#246891,#246892),
(#246893,#246894),(#246895,#246896),(#246897,#246898),(#246899,#246900),
(#246901,#246902),(#246903,#246904),(#246905,#246906),(#246907,#246908),
(#246909,#246910),(#246911,#246912),(#246913,#246914),(#246915,#246916),
(#246917,#246918),(#246919,#246920),(#246921,#246922),(#246923,#246924),
(#246925,#246926),(#246927,#246928),(#246929,#246930),(#246931,#246932),
(#246933,#246934),(#246935,#246936),(#246937,#246938),(#246939,#246940),
(#246941,#246942),(#246943,#246944),(#246945,#246946),(#246947,#246948),
(#246949,#246950),(#246951,#246952),(#246953,#246954),(#246955,#246956),
(#246957,#246958),(#246959,#246960),(#246961,#246962),(#246963,#246964),
(#246965,#246966),(#246967,#246968),(#246969,#246970),(#246971,#246972),
(#246973,#246974),(#246975,#246976)),.UNSPECIFIED.,.F.,.F.,.F.)
B_SPLINE_SURFACE_WITH_KNOTS((6,1,1,1,1,1,1,1,1,1,1,1,1,1,1,1,1,1,1,1,1,
1,1,1,1,1,1,1,1,1,1,1,1,1,1,1,1,1,1,1,1,1,1,1,1,1,1,1,1,1,1,1,1,1,1,1,1,
1,1,1,1,1,1,1,1,1,1,1,1,1,1,1,1,1,1,1,1,1,1,1,1,1,1,1,1,1,1,1,1,1,1,1,1,
1,1,1,1,1,1,1,1,1,1,1,1,1,1,1,1,1,1,1,1,1,1,1,1,1,1,1,1,1,1,1,1,1,1,1,1,
1,1,1,1,1,1,1,1,1,1,1,1,1,1,1,1,1,1,1,1,1,1,1,1,1,1,1,1,1,1,1,1,1,1,1,1,
1,1,1,1,1,1,1,1,1,1,1,1,1,1,1,1,1,1,1,1,1,1,1,1,1,1,1,1,1,1,1,1,1,1,1,6),
(2,2),(0.,0.005,0.01,0.015,0.02,0.025,0.03,0.035,0.04,0.045,0.05,0.055,
0.06,0.065,0.07,0.075,0.08,0.085,0.09,0.095,0.1,0.105,0.11,0.115,0.12,0.125,
0.13,0.135,0.14,0.145,0.15,0.155,0.16,0.165,0.17,0.175,0.18,0.185,0.19,
0.195,0.2,0.205,0.21,0.215,0.22,0.225,0.23,0.235,0.24,0.245,0.25,0.255,
0.26,0.265,0.27,0.275,0.28,0.285,0.29,0.295,0.3,0.305,0.31,0.315,0.32,0.325,
0.33,0.335,0.34,0.345,0.35,0.355,0.36,0.365,0.37,0.375,0.38,0.385,0.39,
0.395,0.4,0.405,0.41,0.415,0.42,0.425,0.43,0.435,0.44,0.445,0.45,0.455,
0.46,0.465,0.47,0.475,0.48,0.485,0.49,0.495,0.5,0.505,0.51,0.515,0.52,0.525,
0.53,0.535,0.54,0.545,0.55,0.555,0.56,0.565,0.57,0.575,0.58,0.585,0.59,
0.595,0.6,0.605,0.61,0.615,0.62,0.625,0.63,0.635,0.64,0.645,0.65,0.655,
0.66,0.665,0.67,0.675,0.68,0.685,0.690000000000001,0.695000000000001,0.700000000000001,
0.705000000000001,0.710000000000001,0.715000000000001,0.720000000000001,
0.725000000000001,0.730000000000001,0.735000000000001,0.740000000000001,
0.745000000000001,0.750000000000001,0.755000000000001,0.760000000000001,
0.765000000000001,0.770000000000001,0.775000000000001,0.780000000000001,
0.785000000000001,0.790000000000001,0.795000000000001,0.800000000000001,
0.805000000000001,0.810000000000001,0.815000000000001,0.820000000000001,
0.825000000000001,0.830000000000001,0.835000000000001,0.840000000000001,
0.845000000000001,0.850000000000001,0.855000000000001,0.860000000000001,
0.865000000000001,0.870000000000001,0.875000000000001,0.880000000000001,
0.885000000000001,0.890000000000001,0.895000000000001,0.900000000000001,
0.905000000000001,0.910000000000001,0.915000000000001,0.920000000000001,
0.925000000000001,0.930000000000001,0.935000000000001,0.940000000000001,
0.945000000000001,0.950000000000001,0.955000000000001,0.960000000000001,
0.965000000000001,0.970000000000001,0.975000000000001,0.980000000000001,
0.985000000000001,0.990000000000001,0.995000000000001,1.),(0.,1.2),
 .UNSPECIFIED.)
GEOMETRIC_REPRESENTATION_ITEM()
RATIONAL_B_SPLINE_SURFACE(((1.,1.),(1.,1.),(1.,1.),(1.,1.),(1.,1.),(1.,
1.),(1.,1.),(1.,1.),(1.,1.),(1.,1.),(1.,1.),(1.,1.),(1.,1.),(1.,1.),(1.,
1.),(1.,1.),(1.,1.),(1.,1.),(1.,1.),(1.,1.),(1.,1.),(1.,1.),(1.,1.),(1.,
1.),(1.,1.),(1.,1.),(1.,1.),(1.,1.),(1.,1.),(1.,1.),(1.,1.),(1.,1.),(1.,
1.),(1.,1.),(1.,1.),(1.,1.),(1.,1.),(1.,1.),(1.,1.),(1.,1.),(1.,1.),(1.,
1.),(1.,1.),(1.,1.),(1.,1.),(1.,1.),(1.,1.),(1.,1.),(1.,1.),(1.,1.),(1.,
1.),(1.,1.),(1.,1.),(1.,1.),(1.,1.),(1.,1.),(1.,1.),(1.,1.),(1.,1.),(1.,
1.),(1.,1.),(1.,1.),(1.,1.),(1.,1.),(1.,1.),(1.,1.),(1.,1.),(1.,1.),(1.,
1.),(1.,1.),(1.,1.),(1.,1.),(1.,1.),(1.,1.),(1.,1.),(1.,1.),(1.,1.),(1.,
1.),(1.,1.),(1.,1.),(1.,1.),(1.,1.),(1.,1.),(1.,1.),(1.,1.),(1.,1.),(1.,
1.),(1.,1.),(1.,1.),(1.,1.),(1.,1.),(1.,1.),(1.,1.),(1.,1.),(1.,1.),(1.,
1.),(1.,1.),(1.,1.),(1.,1.),(1.,1.),(1.,1.),(1.,1.),(1.,1.),(1.,1.),(1.,
1.),(1.,1.),(1.,1.),(1.,1.),(1.,1.),(1.,1.),(1.,1.),(1.,1.),(1.,1.),(1.,
1.),(1.,1.),(1.,1.),(1.,1.),(1.,1.),(1.,1.),(1.,1.),(1.,1.),(1.,1.),(1.,
1.),(1.,1.),(1.,1.),(1.,1.),(1.,1.),(1.,1.),(1.,1.),(1.,1.),(1.,1.),(1.,
1.),(1.,1.),(1.,1.),(1.,1.),(1.,1.),(1.,1.),(1.,1.),(1.,1.),(1.,1.),(1.,
1.),(1.,1.),(1.,1.),(1.,1.),(1.,1.),(1.,1.),(1.,1.),(1.,1.),(1.,1.),(1.,
1.),(1.,1.),(1.,1.),(1.,1.),(1.,1.),(1.,1.),(1.,1.),(1.,1.),(1.,1.),(1.,
1.),(1.,1.),(1.,1.),(1.,1.),(1.,1.),(1.,1.),(1.,1.),(1.,1.),(1.,1.),(1.,
1.),(1.,1.),(1.,1.),(1.,1.),(1.,1.),(1.,1.),(1.,1.),(1.,1.),(1.,1.),(1.,
1.),(1.,1.),(1.,1.),(1.,1.),(1.,1.),(1.,1.),(1.,1.),(1.,1.),(1.,1.),(1.,
1.),(1.,1.),(1.,1.),(1.,1.),(1.,1.),(1.,1.),(1.,1.),(1.,1.),(1.,1.),(1.,
1.),(1.,1.),(1.,1.),(1.,1.),(1.,1.),(1.,1.),(1.,1.),(1.,1.),(1.,1.),(1.,
1.),(1.,1.)))
REPRESENTATION_ITEM('')
SURFACE()
);
#1113=(
BOUNDED_SURFACE()
B_SPLINE_SURFACE(5,1,((#247396,#247397),(#247398,#247399),(#247400,#247401),
(#247402,#247403),(#247404,#247405),(#247406,#247407),(#247408,#247409),
(#247410,#247411),(#247412,#247413),(#247414,#247415),(#247416,#247417),
(#247418,#247419),(#247420,#247421),(#247422,#247423),(#247424,#247425),
(#247426,#247427),(#247428,#247429),(#247430,#247431),(#247432,#247433),
(#247434,#247435),(#247436,#247437),(#247438,#247439),(#247440,#247441),
(#247442,#247443),(#247444,#247445),(#247446,#247447),(#247448,#247449),
(#247450,#247451),(#247452,#247453),(#247454,#247455),(#247456,#247457),
(#247458,#247459),(#247460,#247461),(#247462,#247463),(#247464,#247465),
(#247466,#247467),(#247468,#247469),(#247470,#247471),(#247472,#247473),
(#247474,#247475),(#247476,#247477),(#247478,#247479),(#247480,#247481),
(#247482,#247483),(#247484,#247485),(#247486,#247487),(#247488,#247489),
(#247490,#247491),(#247492,#247493),(#247494,#247495),(#247496,#247497),
(#247498,#247499),(#247500,#247501),(#247502,#247503),(#247504,#247505),
(#247506,#247507),(#247508,#247509),(#247510,#247511),(#247512,#247513),
(#247514,#247515),(#247516,#247517),(#247518,#247519),(#247520,#247521),
(#247522,#247523),(#247524,#247525),(#247526,#247527),(#247528,#247529),
(#247530,#247531),(#247532,#247533),(#247534,#247535),(#247536,#247537),
(#247538,#247539),(#247540,#247541),(#247542,#247543),(#247544,#247545),
(#247546,#247547),(#247548,#247549),(#247550,#247551),(#247552,#247553),
(#247554,#247555),(#247556,#247557),(#247558,#247559),(#247560,#247561),
(#247562,#247563),(#247564,#247565),(#247566,#247567),(#247568,#247569),
(#247570,#247571),(#247572,#247573),(#247574,#247575),(#247576,#247577),
(#247578,#247579),(#247580,#247581),(#247582,#247583),(#247584,#247585),
(#247586,#247587),(#247588,#247589),(#247590,#247591),(#247592,#247593),
(#247594,#247595),(#247596,#247597),(#247598,#247599),(#247600,#247601),
(#247602,#247603),(#247604,#247605),(#247606,#247607),(#247608,#247609),
(#247610,#247611),(#247612,#247613),(#247614,#247615),(#247616,#247617),
(#247618,#247619),(#247620,#247621),(#247622,#247623),(#247624,#247625),
(#247626,#247627),(#247628,#247629),(#247630,#247631),(#247632,#247633),
(#247634,#247635),(#247636,#247637),(#247638,#247639),(#247640,#247641),
(#247642,#247643),(#247644,#247645),(#247646,#247647),(#247648,#247649),
(#247650,#247651),(#247652,#247653),(#247654,#247655),(#247656,#247657),
(#247658,#247659),(#247660,#247661),(#247662,#247663),(#247664,#247665),
(#247666,#247667),(#247668,#247669),(#247670,#247671),(#247672,#247673),
(#247674,#247675),(#247676,#247677),(#247678,#247679),(#247680,#247681),
(#247682,#247683),(#247684,#247685),(#247686,#247687),(#247688,#247689),
(#247690,#247691),(#247692,#247693),(#247694,#247695),(#247696,#247697),
(#247698,#247699),(#247700,#247701),(#247702,#247703),(#247704,#247705),
(#247706,#247707),(#247708,#247709),(#247710,#247711),(#247712,#247713),
(#247714,#247715),(#247716,#247717),(#247718,#247719),(#247720,#247721),
(#247722,#247723),(#247724,#247725),(#247726,#247727),(#247728,#247729),
(#247730,#247731),(#247732,#247733),(#247734,#247735),(#247736,#247737),
(#247738,#247739),(#247740,#247741),(#247742,#247743),(#247744,#247745),
(#247746,#247747),(#247748,#247749),(#247750,#247751),(#247752,#247753),
(#247754,#247755),(#247756,#247757),(#247758,#247759),(#247760,#247761),
(#247762,#247763),(#247764,#247765),(#247766,#247767),(#247768,#247769),
(#247770,#247771),(#247772,#247773),(#247774,#247775),(#247776,#247777),
(#247778,#247779),(#247780,#247781),(#247782,#247783),(#247784,#247785),
(#247786,#247787),(#247788,#247789),(#247790,#247791),(#247792,#247793),
(#247794,#247795),(#247796,#247797),(#247798,#247799),(#247800,#247801),
(#247802,#247803),(#247804,#247805)),.UNSPECIFIED.,.F.,.F.,.F.)
B_SPLINE_SURFACE_WITH_KNOTS((6,1,1,1,1,1,1,1,1,1,1,1,1,1,1,1,1,1,1,1,1,
1,1,1,1,1,1,1,1,1,1,1,1,1,1,1,1,1,1,1,1,1,1,1,1,1,1,1,1,1,1,1,1,1,1,1,1,
1,1,1,1,1,1,1,1,1,1,1,1,1,1,1,1,1,1,1,1,1,1,1,1,1,1,1,1,1,1,1,1,1,1,1,1,
1,1,1,1,1,1,1,1,1,1,1,1,1,1,1,1,1,1,1,1,1,1,1,1,1,1,1,1,1,1,1,1,1,1,1,1,
1,1,1,1,1,1,1,1,1,1,1,1,1,1,1,1,1,1,1,1,1,1,1,1,1,1,1,1,1,1,1,1,1,1,1,1,
1,1,1,1,1,1,1,1,1,1,1,1,1,1,1,1,1,1,1,1,1,1,1,1,1,1,1,1,1,1,1,1,1,1,1,6),
(2,2),(-1.,-0.995000000000001,-0.990000000000001,-0.985000000000001,-0.980000000000001,
-0.975000000000001,-0.970000000000001,-0.965000000000001,-0.960000000000001,
-0.955000000000001,-0.950000000000001,-0.945000000000001,-0.940000000000001,
-0.935000000000001,-0.930000000000001,-0.925000000000001,-0.920000000000001,
-0.915000000000001,-0.910000000000001,-0.905000000000001,-0.900000000000001,
-0.895000000000001,-0.890000000000001,-0.885000000000001,-0.880000000000001,
-0.875000000000001,-0.870000000000001,-0.865000000000001,-0.860000000000001,
-0.855000000000001,-0.850000000000001,-0.845000000000001,-0.840000000000001,
-0.835000000000001,-0.830000000000001,-0.825000000000001,-0.820000000000001,
-0.815000000000001,-0.810000000000001,-0.805000000000001,-0.800000000000001,
-0.795000000000001,-0.790000000000001,-0.785000000000001,-0.780000000000001,
-0.775000000000001,-0.770000000000001,-0.765000000000001,-0.760000000000001,
-0.755000000000001,-0.750000000000001,-0.745000000000001,-0.740000000000001,
-0.735000000000001,-0.730000000000001,-0.725000000000001,-0.720000000000001,
-0.715000000000001,-0.710000000000001,-0.705000000000001,-0.700000000000001,
-0.695000000000001,-0.690000000000001,-0.685,-0.68,-0.675,-0.67,-0.665,
-0.66,-0.655,-0.65,-0.645,-0.64,-0.635,-0.63,-0.625,-0.62,-0.615,-0.61,
-0.605,-0.6,-0.595,-0.59,-0.585,-0.58,-0.575,-0.57,-0.565,-0.56,-0.555,
-0.55,-0.545,-0.54,-0.535,-0.53,-0.525,-0.52,-0.515,-0.51,-0.505,-0.5,-0.495,
-0.49,-0.485,-0.48,-0.475,-0.47,-0.465,-0.46,-0.455,-0.45,-0.445,-0.44,
-0.435,-0.43,-0.425,-0.42,-0.415,-0.41,-0.405,-0.4,-0.395,-0.39,-0.385,
-0.38,-0.375,-0.37,-0.365,-0.36,-0.355,-0.35,-0.345,-0.34,-0.335,-0.33,
-0.325,-0.32,-0.315,-0.31,-0.305,-0.3,-0.295,-0.29,-0.285,-0.28,-0.275,
-0.27,-0.265,-0.26,-0.255,-0.25,-0.245,-0.24,-0.235,-0.23,-0.225,-0.22,
-0.215,-0.21,-0.205,-0.2,-0.195,-0.19,-0.185,-0.18,-0.175,-0.17,-0.165,
-0.16,-0.155,-0.15,-0.145,-0.14,-0.135,-0.13,-0.125,-0.12,-0.115,-0.11,
-0.105,-0.1,-0.095,-0.09,-0.085,-0.08,-0.075,-0.07,-0.065,-0.06,-0.055,
-0.05,-0.045,-0.04,-0.035,-0.03,-0.025,-0.02,-0.015,-0.01,-0.005,0.),(0.,
1.2),.UNSPECIFIED.)
GEOMETRIC_REPRESENTATION_ITEM()
RATIONAL_B_SPLINE_SURFACE(((1.,1.),(1.,1.),(1.,1.),(1.,1.),(1.,1.),(1.,
1.),(1.,1.),(1.,1.),(1.,1.),(1.,1.),(1.,1.),(1.,1.),(1.,1.),(1.,1.),(1.,
1.),(1.,1.),(1.,1.),(1.,1.),(1.,1.),(1.,1.),(1.,1.),(1.,1.),(1.,1.),(1.,
1.),(1.,1.),(1.,1.),(1.,1.),(1.,1.),(1.,1.),(1.,1.),(1.,1.),(1.,1.),(1.,
1.),(1.,1.),(1.,1.),(1.,1.),(1.,1.),(1.,1.),(1.,1.),(1.,1.),(1.,1.),(1.,
1.),(1.,1.),(1.,1.),(1.,1.),(1.,1.),(1.,1.),(1.,1.),(1.,1.),(1.,1.),(1.,
1.),(1.,1.),(1.,1.),(1.,1.),(1.,1.),(1.,1.),(1.,1.),(1.,1.),(1.,1.),(1.,
1.),(1.,1.),(1.,1.),(1.,1.),(1.,1.),(1.,1.),(1.,1.),(1.,1.),(1.,1.),(1.,
1.),(1.,1.),(1.,1.),(1.,1.),(1.,1.),(1.,1.),(1.,1.),(1.,1.),(1.,1.),(1.,
1.),(1.,1.),(1.,1.),(1.,1.),(1.,1.),(1.,1.),(1.,1.),(1.,1.),(1.,1.),(1.,
1.),(1.,1.),(1.,1.),(1.,1.),(1.,1.),(1.,1.),(1.,1.),(1.,1.),(1.,1.),(1.,
1.),(1.,1.),(1.,1.),(1.,1.),(1.,1.),(1.,1.),(1.,1.),(1.,1.),(1.,1.),(1.,
1.),(1.,1.),(1.,1.),(1.,1.),(1.,1.),(1.,1.),(1.,1.),(1.,1.),(1.,1.),(1.,
1.),(1.,1.),(1.,1.),(1.,1.),(1.,1.),(1.,1.),(1.,1.),(1.,1.),(1.,1.),(1.,
1.),(1.,1.),(1.,1.),(1.,1.),(1.,1.),(1.,1.),(1.,1.),(1.,1.),(1.,1.),(1.,
1.),(1.,1.),(1.,1.),(1.,1.),(1.,1.),(1.,1.),(1.,1.),(1.,1.),(1.,1.),(1.,
1.),(1.,1.),(1.,1.),(1.,1.),(1.,1.),(1.,1.),(1.,1.),(1.,1.),(1.,1.),(1.,
1.),(1.,1.),(1.,1.),(1.,1.),(1.,1.),(1.,1.),(1.,1.),(1.,1.),(1.,1.),(1.,
1.),(1.,1.),(1.,1.),(1.,1.),(1.,1.),(1.,1.),(1.,1.),(1.,1.),(1.,1.),(1.,
1.),(1.,1.),(1.,1.),(1.,1.),(1.,1.),(1.,1.),(1.,1.),(1.,1.),(1.,1.),(1.,
1.),(1.,1.),(1.,1.),(1.,1.),(1.,1.),(1.,1.),(1.,1.),(1.,1.),(1.,1.),(1.,
1.),(1.,1.),(1.,1.),(1.,1.),(1.,1.),(1.,1.),(1.,1.),(1.,1.),(1.,1.),(1.,
1.),(1.,1.),(1.,1.),(1.,1.),(1.,1.),(1.,1.),(1.,1.),(1.,1.),(1.,1.),(1.,
1.),(1.,1.)))
REPRESENTATION_ITEM('')
SURFACE()
);
#1114=(
BOUNDED_SURFACE()
B_SPLINE_SURFACE(5,1,((#248219,#248220),(#248221,#248222),(#248223,#248224),
(#248225,#248226),(#248227,#248228),(#248229,#248230),(#248231,#248232),
(#248233,#248234),(#248235,#248236),(#248237,#248238),(#248239,#248240),
(#248241,#248242),(#248243,#248244),(#248245,#248246),(#248247,#248248),
(#248249,#248250),(#248251,#248252),(#248253,#248254),(#248255,#248256),
(#248257,#248258),(#248259,#248260),(#248261,#248262),(#248263,#248264),
(#248265,#248266),(#248267,#248268),(#248269,#248270),(#248271,#248272),
(#248273,#248274),(#248275,#248276),(#248277,#248278),(#248279,#248280),
(#248281,#248282),(#248283,#248284),(#248285,#248286),(#248287,#248288),
(#248289,#248290),(#248291,#248292),(#248293,#248294),(#248295,#248296),
(#248297,#248298),(#248299,#248300),(#248301,#248302),(#248303,#248304),
(#248305,#248306),(#248307,#248308),(#248309,#248310),(#248311,#248312),
(#248313,#248314),(#248315,#248316),(#248317,#248318),(#248319,#248320),
(#248321,#248322),(#248323,#248324),(#248325,#248326),(#248327,#248328),
(#248329,#248330),(#248331,#248332),(#248333,#248334),(#248335,#248336),
(#248337,#248338),(#248339,#248340),(#248341,#248342),(#248343,#248344),
(#248345,#248346),(#248347,#248348),(#248349,#248350),(#248351,#248352),
(#248353,#248354),(#248355,#248356),(#248357,#248358),(#248359,#248360),
(#248361,#248362),(#248363,#248364),(#248365,#248366),(#248367,#248368),
(#248369,#248370),(#248371,#248372),(#248373,#248374),(#248375,#248376),
(#248377,#248378),(#248379,#248380),(#248381,#248382),(#248383,#248384),
(#248385,#248386),(#248387,#248388),(#248389,#248390),(#248391,#248392),
(#248393,#248394),(#248395,#248396),(#248397,#248398),(#248399,#248400),
(#248401,#248402),(#248403,#248404),(#248405,#248406),(#248407,#248408),
(#248409,#248410),(#248411,#248412),(#248413,#248414),(#248415,#248416),
(#248417,#248418),(#248419,#248420),(#248421,#248422),(#248423,#248424),
(#248425,#248426),(#248427,#248428),(#248429,#248430),(#248431,#248432),
(#248433,#248434),(#248435,#248436),(#248437,#248438),(#248439,#248440),
(#248441,#248442),(#248443,#248444),(#248445,#248446),(#248447,#248448),
(#248449,#248450),(#248451,#248452),(#248453,#248454),(#248455,#248456),
(#248457,#248458),(#248459,#248460),(#248461,#248462),(#248463,#248464),
(#248465,#248466),(#248467,#248468),(#248469,#248470),(#248471,#248472),
(#248473,#248474),(#248475,#248476),(#248477,#248478),(#248479,#248480),
(#248481,#248482),(#248483,#248484),(#248485,#248486),(#248487,#248488),
(#248489,#248490),(#248491,#248492),(#248493,#248494),(#248495,#248496),
(#248497,#248498),(#248499,#248500),(#248501,#248502),(#248503,#248504),
(#248505,#248506),(#248507,#248508),(#248509,#248510),(#248511,#248512),
(#248513,#248514),(#248515,#248516),(#248517,#248518),(#248519,#248520),
(#248521,#248522),(#248523,#248524),(#248525,#248526),(#248527,#248528),
(#248529,#248530),(#248531,#248532),(#248533,#248534),(#248535,#248536),
(#248537,#248538),(#248539,#248540),(#248541,#248542),(#248543,#248544),
(#248545,#248546),(#248547,#248548),(#248549,#248550),(#248551,#248552),
(#248553,#248554),(#248555,#248556),(#248557,#248558),(#248559,#248560),
(#248561,#248562),(#248563,#248564),(#248565,#248566),(#248567,#248568),
(#248569,#248570),(#248571,#248572),(#248573,#248574),(#248575,#248576),
(#248577,#248578),(#248579,#248580),(#248581,#248582),(#248583,#248584),
(#248585,#248586),(#248587,#248588),(#248589,#248590),(#248591,#248592),
(#248593,#248594),(#248595,#248596),(#248597,#248598),(#248599,#248600),
(#248601,#248602),(#248603,#248604),(#248605,#248606),(#248607,#248608),
(#248609,#248610),(#248611,#248612),(#248613,#248614),(#248615,#248616),
(#248617,#248618),(#248619,#248620),(#248621,#248622),(#248623,#248624),
(#248625,#248626),(#248627,#248628)),.UNSPECIFIED.,.F.,.F.,.F.)
B_SPLINE_SURFACE_WITH_KNOTS((6,1,1,1,1,1,1,1,1,1,1,1,1,1,1,1,1,1,1,1,1,
1,1,1,1,1,1,1,1,1,1,1,1,1,1,1,1,1,1,1,1,1,1,1,1,1,1,1,1,1,1,1,1,1,1,1,1,
1,1,1,1,1,1,1,1,1,1,1,1,1,1,1,1,1,1,1,1,1,1,1,1,1,1,1,1,1,1,1,1,1,1,1,1,
1,1,1,1,1,1,1,1,1,1,1,1,1,1,1,1,1,1,1,1,1,1,1,1,1,1,1,1,1,1,1,1,1,1,1,1,
1,1,1,1,1,1,1,1,1,1,1,1,1,1,1,1,1,1,1,1,1,1,1,1,1,1,1,1,1,1,1,1,1,1,1,1,
1,1,1,1,1,1,1,1,1,1,1,1,1,1,1,1,1,1,1,1,1,1,1,1,1,1,1,1,1,1,1,1,1,1,1,6),
(2,2),(0.,0.005,0.01,0.015,0.02,0.025,0.03,0.035,0.04,0.045,0.05,0.055,
0.06,0.065,0.07,0.075,0.08,0.085,0.09,0.095,0.1,0.105,0.11,0.115,0.12,0.125,
0.13,0.135,0.14,0.145,0.15,0.155,0.16,0.165,0.17,0.175,0.18,0.185,0.19,
0.195,0.2,0.205,0.21,0.215,0.22,0.225,0.23,0.235,0.24,0.245,0.25,0.255,
0.26,0.265,0.27,0.275,0.28,0.285,0.29,0.295,0.3,0.305,0.31,0.315,0.32,0.325,
0.33,0.335,0.34,0.345,0.35,0.355,0.36,0.365,0.37,0.375,0.38,0.385,0.39,
0.395,0.4,0.405,0.41,0.415,0.42,0.425,0.43,0.435,0.44,0.445,0.45,0.455,
0.46,0.465,0.47,0.475,0.48,0.485,0.49,0.495,0.5,0.505,0.51,0.515,0.52,0.525,
0.53,0.535,0.54,0.545,0.55,0.555,0.56,0.565,0.57,0.575,0.58,0.585,0.59,
0.595,0.6,0.605,0.61,0.615,0.62,0.625,0.63,0.635,0.64,0.645,0.65,0.655,
0.66,0.665,0.67,0.675,0.68,0.685,0.690000000000001,0.695000000000001,0.700000000000001,
0.705000000000001,0.710000000000001,0.715000000000001,0.720000000000001,
0.725000000000001,0.730000000000001,0.735000000000001,0.740000000000001,
0.745000000000001,0.750000000000001,0.755000000000001,0.760000000000001,
0.765000000000001,0.770000000000001,0.775000000000001,0.780000000000001,
0.785000000000001,0.790000000000001,0.795000000000001,0.800000000000001,
0.805000000000001,0.810000000000001,0.815000000000001,0.820000000000001,
0.825000000000001,0.830000000000001,0.835000000000001,0.840000000000001,
0.845000000000001,0.850000000000001,0.855000000000001,0.860000000000001,
0.865000000000001,0.870000000000001,0.875000000000001,0.880000000000001,
0.885000000000001,0.890000000000001,0.895000000000001,0.900000000000001,
0.905000000000001,0.910000000000001,0.915000000000001,0.920000000000001,
0.925000000000001,0.930000000000001,0.935000000000001,0.940000000000001,
0.945000000000001,0.950000000000001,0.955000000000001,0.960000000000001,
0.965000000000001,0.970000000000001,0.975000000000001,0.980000000000001,
0.985000000000001,0.990000000000001,0.995000000000001,1.),(0.,1.2),
 .UNSPECIFIED.)
GEOMETRIC_REPRESENTATION_ITEM()
RATIONAL_B_SPLINE_SURFACE(((1.,1.),(1.,1.),(1.,1.),(1.,1.),(1.,1.),(1.,
1.),(1.,1.),(1.,1.),(1.,1.),(1.,1.),(1.,1.),(1.,1.),(1.,1.),(1.,1.),(1.,
1.),(1.,1.),(1.,1.),(1.,1.),(1.,1.),(1.,1.),(1.,1.),(1.,1.),(1.,1.),(1.,
1.),(1.,1.),(1.,1.),(1.,1.),(1.,1.),(1.,1.),(1.,1.),(1.,1.),(1.,1.),(1.,
1.),(1.,1.),(1.,1.),(1.,1.),(1.,1.),(1.,1.),(1.,1.),(1.,1.),(1.,1.),(1.,
1.),(1.,1.),(1.,1.),(1.,1.),(1.,1.),(1.,1.),(1.,1.),(1.,1.),(1.,1.),(1.,
1.),(1.,1.),(1.,1.),(1.,1.),(1.,1.),(1.,1.),(1.,1.),(1.,1.),(1.,1.),(1.,
1.),(1.,1.),(1.,1.),(1.,1.),(1.,1.),(1.,1.),(1.,1.),(1.,1.),(1.,1.),(1.,
1.),(1.,1.),(1.,1.),(1.,1.),(1.,1.),(1.,1.),(1.,1.),(1.,1.),(1.,1.),(1.,
1.),(1.,1.),(1.,1.),(1.,1.),(1.,1.),(1.,1.),(1.,1.),(1.,1.),(1.,1.),(1.,
1.),(1.,1.),(1.,1.),(1.,1.),(1.,1.),(1.,1.),(1.,1.),(1.,1.),(1.,1.),(1.,
1.),(1.,1.),(1.,1.),(1.,1.),(1.,1.),(1.,1.),(1.,1.),(1.,1.),(1.,1.),(1.,
1.),(1.,1.),(1.,1.),(1.,1.),(1.,1.),(1.,1.),(1.,1.),(1.,1.),(1.,1.),(1.,
1.),(1.,1.),(1.,1.),(1.,1.),(1.,1.),(1.,1.),(1.,1.),(1.,1.),(1.,1.),(1.,
1.),(1.,1.),(1.,1.),(1.,1.),(1.,1.),(1.,1.),(1.,1.),(1.,1.),(1.,1.),(1.,
1.),(1.,1.),(1.,1.),(1.,1.),(1.,1.),(1.,1.),(1.,1.),(1.,1.),(1.,1.),(1.,
1.),(1.,1.),(1.,1.),(1.,1.),(1.,1.),(1.,1.),(1.,1.),(1.,1.),(1.,1.),(1.,
1.),(1.,1.),(1.,1.),(1.,1.),(1.,1.),(1.,1.),(1.,1.),(1.,1.),(1.,1.),(1.,
1.),(1.,1.),(1.,1.),(1.,1.),(1.,1.),(1.,1.),(1.,1.),(1.,1.),(1.,1.),(1.,
1.),(1.,1.),(1.,1.),(1.,1.),(1.,1.),(1.,1.),(1.,1.),(1.,1.),(1.,1.),(1.,
1.),(1.,1.),(1.,1.),(1.,1.),(1.,1.),(1.,1.),(1.,1.),(1.,1.),(1.,1.),(1.,
1.),(1.,1.),(1.,1.),(1.,1.),(1.,1.),(1.,1.),(1.,1.),(1.,1.),(1.,1.),(1.,
1.),(1.,1.),(1.,1.),(1.,1.),(1.,1.),(1.,1.),(1.,1.),(1.,1.),(1.,1.),(1.,
1.),(1.,1.)))
REPRESENTATION_ITEM('')
SURFACE()
);
#1115=(
BOUNDED_SURFACE()
B_SPLINE_SURFACE(5,1,((#249048,#249049),(#249050,#249051),(#249052,#249053),
(#249054,#249055),(#249056,#249057),(#249058,#249059),(#249060,#249061),
(#249062,#249063),(#249064,#249065),(#249066,#249067),(#249068,#249069),
(#249070,#249071),(#249072,#249073),(#249074,#249075),(#249076,#249077),
(#249078,#249079),(#249080,#249081),(#249082,#249083),(#249084,#249085),
(#249086,#249087),(#249088,#249089),(#249090,#249091),(#249092,#249093),
(#249094,#249095),(#249096,#249097),(#249098,#249099),(#249100,#249101),
(#249102,#249103),(#249104,#249105),(#249106,#249107),(#249108,#249109),
(#249110,#249111),(#249112,#249113),(#249114,#249115),(#249116,#249117),
(#249118,#249119),(#249120,#249121),(#249122,#249123),(#249124,#249125),
(#249126,#249127),(#249128,#249129),(#249130,#249131),(#249132,#249133),
(#249134,#249135),(#249136,#249137),(#249138,#249139),(#249140,#249141),
(#249142,#249143),(#249144,#249145),(#249146,#249147),(#249148,#249149),
(#249150,#249151),(#249152,#249153),(#249154,#249155),(#249156,#249157),
(#249158,#249159),(#249160,#249161),(#249162,#249163),(#249164,#249165),
(#249166,#249167),(#249168,#249169),(#249170,#249171),(#249172,#249173),
(#249174,#249175),(#249176,#249177),(#249178,#249179),(#249180,#249181),
(#249182,#249183),(#249184,#249185),(#249186,#249187),(#249188,#249189),
(#249190,#249191),(#249192,#249193),(#249194,#249195),(#249196,#249197),
(#249198,#249199),(#249200,#249201),(#249202,#249203),(#249204,#249205),
(#249206,#249207),(#249208,#249209),(#249210,#249211),(#249212,#249213),
(#249214,#249215),(#249216,#249217),(#249218,#249219),(#249220,#249221),
(#249222,#249223),(#249224,#249225),(#249226,#249227),(#249228,#249229),
(#249230,#249231),(#249232,#249233),(#249234,#249235),(#249236,#249237),
(#249238,#249239),(#249240,#249241),(#249242,#249243),(#249244,#249245),
(#249246,#249247),(#249248,#249249),(#249250,#249251),(#249252,#249253),
(#249254,#249255),(#249256,#249257),(#249258,#249259),(#249260,#249261),
(#249262,#249263),(#249264,#249265),(#249266,#249267),(#249268,#249269),
(#249270,#249271),(#249272,#249273),(#249274,#249275),(#249276,#249277),
(#249278,#249279),(#249280,#249281),(#249282,#249283),(#249284,#249285),
(#249286,#249287),(#249288,#249289),(#249290,#249291),(#249292,#249293),
(#249294,#249295),(#249296,#249297),(#249298,#249299),(#249300,#249301),
(#249302,#249303),(#249304,#249305),(#249306,#249307),(#249308,#249309),
(#249310,#249311),(#249312,#249313),(#249314,#249315),(#249316,#249317),
(#249318,#249319),(#249320,#249321),(#249322,#249323),(#249324,#249325),
(#249326,#249327),(#249328,#249329),(#249330,#249331),(#249332,#249333),
(#249334,#249335),(#249336,#249337),(#249338,#249339),(#249340,#249341),
(#249342,#249343),(#249344,#249345),(#249346,#249347),(#249348,#249349),
(#249350,#249351),(#249352,#249353),(#249354,#249355),(#249356,#249357),
(#249358,#249359),(#249360,#249361),(#249362,#249363),(#249364,#249365),
(#249366,#249367),(#249368,#249369),(#249370,#249371),(#249372,#249373),
(#249374,#249375),(#249376,#249377),(#249378,#249379),(#249380,#249381),
(#249382,#249383),(#249384,#249385),(#249386,#249387),(#249388,#249389),
(#249390,#249391),(#249392,#249393),(#249394,#249395),(#249396,#249397),
(#249398,#249399),(#249400,#249401),(#249402,#249403),(#249404,#249405),
(#249406,#249407),(#249408,#249409),(#249410,#249411),(#249412,#249413),
(#249414,#249415),(#249416,#249417),(#249418,#249419),(#249420,#249421),
(#249422,#249423),(#249424,#249425),(#249426,#249427),(#249428,#249429),
(#249430,#249431),(#249432,#249433),(#249434,#249435),(#249436,#249437),
(#249438,#249439),(#249440,#249441),(#249442,#249443),(#249444,#249445),
(#249446,#249447),(#249448,#249449),(#249450,#249451),(#249452,#249453),
(#249454,#249455),(#249456,#249457)),.UNSPECIFIED.,.F.,.F.,.F.)
B_SPLINE_SURFACE_WITH_KNOTS((6,1,1,1,1,1,1,1,1,1,1,1,1,1,1,1,1,1,1,1,1,
1,1,1,1,1,1,1,1,1,1,1,1,1,1,1,1,1,1,1,1,1,1,1,1,1,1,1,1,1,1,1,1,1,1,1,1,
1,1,1,1,1,1,1,1,1,1,1,1,1,1,1,1,1,1,1,1,1,1,1,1,1,1,1,1,1,1,1,1,1,1,1,1,
1,1,1,1,1,1,1,1,1,1,1,1,1,1,1,1,1,1,1,1,1,1,1,1,1,1,1,1,1,1,1,1,1,1,1,1,
1,1,1,1,1,1,1,1,1,1,1,1,1,1,1,1,1,1,1,1,1,1,1,1,1,1,1,1,1,1,1,1,1,1,1,1,
1,1,1,1,1,1,1,1,1,1,1,1,1,1,1,1,1,1,1,1,1,1,1,1,1,1,1,1,1,1,1,1,1,1,1,6),
(2,2),(-1.,-0.995000000000001,-0.990000000000001,-0.985000000000001,-0.980000000000001,
-0.975000000000001,-0.970000000000001,-0.965000000000001,-0.960000000000001,
-0.955000000000001,-0.950000000000001,-0.945000000000001,-0.940000000000001,
-0.935000000000001,-0.930000000000001,-0.925000000000001,-0.920000000000001,
-0.915000000000001,-0.910000000000001,-0.905000000000001,-0.900000000000001,
-0.895000000000001,-0.890000000000001,-0.885000000000001,-0.880000000000001,
-0.875000000000001,-0.870000000000001,-0.865000000000001,-0.860000000000001,
-0.855000000000001,-0.850000000000001,-0.845000000000001,-0.840000000000001,
-0.835000000000001,-0.830000000000001,-0.825000000000001,-0.820000000000001,
-0.815000000000001,-0.810000000000001,-0.805000000000001,-0.800000000000001,
-0.795000000000001,-0.790000000000001,-0.785000000000001,-0.780000000000001,
-0.775000000000001,-0.770000000000001,-0.765000000000001,-0.760000000000001,
-0.755000000000001,-0.750000000000001,-0.745000000000001,-0.740000000000001,
-0.735000000000001,-0.730000000000001,-0.725000000000001,-0.720000000000001,
-0.715000000000001,-0.710000000000001,-0.705000000000001,-0.700000000000001,
-0.695000000000001,-0.690000000000001,-0.685,-0.68,-0.675,-0.67,-0.665,
-0.66,-0.655,-0.65,-0.645,-0.64,-0.635,-0.63,-0.625,-0.62,-0.615,-0.61,
-0.605,-0.6,-0.595,-0.59,-0.585,-0.58,-0.575,-0.57,-0.565,-0.56,-0.555,
-0.55,-0.545,-0.54,-0.535,-0.53,-0.525,-0.52,-0.515,-0.51,-0.505,-0.5,-0.495,
-0.49,-0.485,-0.48,-0.475,-0.47,-0.465,-0.46,-0.455,-0.45,-0.445,-0.44,
-0.435,-0.43,-0.425,-0.42,-0.415,-0.41,-0.405,-0.4,-0.395,-0.39,-0.385,
-0.38,-0.375,-0.37,-0.365,-0.36,-0.355,-0.35,-0.345,-0.34,-0.335,-0.33,
-0.325,-0.32,-0.315,-0.31,-0.305,-0.3,-0.295,-0.29,-0.285,-0.28,-0.275,
-0.27,-0.265,-0.26,-0.255,-0.25,-0.245,-0.24,-0.235,-0.23,-0.225,-0.22,
-0.215,-0.21,-0.205,-0.2,-0.195,-0.19,-0.185,-0.18,-0.175,-0.17,-0.165,
-0.16,-0.155,-0.15,-0.145,-0.14,-0.135,-0.13,-0.125,-0.12,-0.115,-0.11,
-0.105,-0.1,-0.095,-0.09,-0.085,-0.08,-0.075,-0.07,-0.065,-0.06,-0.055,
-0.05,-0.045,-0.04,-0.035,-0.03,-0.025,-0.02,-0.015,-0.01,-0.005,0.),(0.,
1.2),.UNSPECIFIED.)
GEOMETRIC_REPRESENTATION_ITEM()
RATIONAL_B_SPLINE_SURFACE(((1.,1.),(1.,1.),(1.,1.),(1.,1.),(1.,1.),(1.,
1.),(1.,1.),(1.,1.),(1.,1.),(1.,1.),(1.,1.),(1.,1.),(1.,1.),(1.,1.),(1.,
1.),(1.,1.),(1.,1.),(1.,1.),(1.,1.),(1.,1.),(1.,1.),(1.,1.),(1.,1.),(1.,
1.),(1.,1.),(1.,1.),(1.,1.),(1.,1.),(1.,1.),(1.,1.),(1.,1.),(1.,1.),(1.,
1.),(1.,1.),(1.,1.),(1.,1.),(1.,1.),(1.,1.),(1.,1.),(1.,1.),(1.,1.),(1.,
1.),(1.,1.),(1.,1.),(1.,1.),(1.,1.),(1.,1.),(1.,1.),(1.,1.),(1.,1.),(1.,
1.),(1.,1.),(1.,1.),(1.,1.),(1.,1.),(1.,1.),(1.,1.),(1.,1.),(1.,1.),(1.,
1.),(1.,1.),(1.,1.),(1.,1.),(1.,1.),(1.,1.),(1.,1.),(1.,1.),(1.,1.),(1.,
1.),(1.,1.),(1.,1.),(1.,1.),(1.,1.),(1.,1.),(1.,1.),(1.,1.),(1.,1.),(1.,
1.),(1.,1.),(1.,1.),(1.,1.),(1.,1.),(1.,1.),(1.,1.),(1.,1.),(1.,1.),(1.,
1.),(1.,1.),(1.,1.),(1.,1.),(1.,1.),(1.,1.),(1.,1.),(1.,1.),(1.,1.),(1.,
1.),(1.,1.),(1.,1.),(1.,1.),(1.,1.),(1.,1.),(1.,1.),(1.,1.),(1.,1.),(1.,
1.),(1.,1.),(1.,1.),(1.,1.),(1.,1.),(1.,1.),(1.,1.),(1.,1.),(1.,1.),(1.,
1.),(1.,1.),(1.,1.),(1.,1.),(1.,1.),(1.,1.),(1.,1.),(1.,1.),(1.,1.),(1.,
1.),(1.,1.),(1.,1.),(1.,1.),(1.,1.),(1.,1.),(1.,1.),(1.,1.),(1.,1.),(1.,
1.),(1.,1.),(1.,1.),(1.,1.),(1.,1.),(1.,1.),(1.,1.),(1.,1.),(1.,1.),(1.,
1.),(1.,1.),(1.,1.),(1.,1.),(1.,1.),(1.,1.),(1.,1.),(1.,1.),(1.,1.),(1.,
1.),(1.,1.),(1.,1.),(1.,1.),(1.,1.),(1.,1.),(1.,1.),(1.,1.),(1.,1.),(1.,
1.),(1.,1.),(1.,1.),(1.,1.),(1.,1.),(1.,1.),(1.,1.),(1.,1.),(1.,1.),(1.,
1.),(1.,1.),(1.,1.),(1.,1.),(1.,1.),(1.,1.),(1.,1.),(1.,1.),(1.,1.),(1.,
1.),(1.,1.),(1.,1.),(1.,1.),(1.,1.),(1.,1.),(1.,1.),(1.,1.),(1.,1.),(1.,
1.),(1.,1.),(1.,1.),(1.,1.),(1.,1.),(1.,1.),(1.,1.),(1.,1.),(1.,1.),(1.,
1.),(1.,1.),(1.,1.),(1.,1.),(1.,1.),(1.,1.),(1.,1.),(1.,1.),(1.,1.),(1.,
1.),(1.,1.)))
REPRESENTATION_ITEM('')
SURFACE()
);
#1116=(
BOUNDED_SURFACE()
B_SPLINE_SURFACE(5,1,((#249871,#249872),(#249873,#249874),(#249875,#249876),
(#249877,#249878),(#249879,#249880),(#249881,#249882),(#249883,#249884),
(#249885,#249886),(#249887,#249888),(#249889,#249890),(#249891,#249892),
(#249893,#249894),(#249895,#249896),(#249897,#249898),(#249899,#249900),
(#249901,#249902),(#249903,#249904),(#249905,#249906),(#249907,#249908),
(#249909,#249910),(#249911,#249912),(#249913,#249914),(#249915,#249916),
(#249917,#249918),(#249919,#249920),(#249921,#249922),(#249923,#249924),
(#249925,#249926),(#249927,#249928),(#249929,#249930),(#249931,#249932),
(#249933,#249934),(#249935,#249936),(#249937,#249938),(#249939,#249940),
(#249941,#249942),(#249943,#249944),(#249945,#249946),(#249947,#249948),
(#249949,#249950),(#249951,#249952),(#249953,#249954),(#249955,#249956),
(#249957,#249958),(#249959,#249960),(#249961,#249962),(#249963,#249964),
(#249965,#249966),(#249967,#249968),(#249969,#249970),(#249971,#249972),
(#249973,#249974),(#249975,#249976),(#249977,#249978),(#249979,#249980),
(#249981,#249982),(#249983,#249984),(#249985,#249986),(#249987,#249988),
(#249989,#249990),(#249991,#249992),(#249993,#249994),(#249995,#249996),
(#249997,#249998),(#249999,#250000),(#250001,#250002),(#250003,#250004),
(#250005,#250006),(#250007,#250008),(#250009,#250010),(#250011,#250012),
(#250013,#250014),(#250015,#250016),(#250017,#250018),(#250019,#250020),
(#250021,#250022),(#250023,#250024),(#250025,#250026),(#250027,#250028),
(#250029,#250030),(#250031,#250032),(#250033,#250034),(#250035,#250036),
(#250037,#250038),(#250039,#250040),(#250041,#250042),(#250043,#250044),
(#250045,#250046),(#250047,#250048),(#250049,#250050),(#250051,#250052),
(#250053,#250054),(#250055,#250056),(#250057,#250058),(#250059,#250060),
(#250061,#250062),(#250063,#250064),(#250065,#250066),(#250067,#250068),
(#250069,#250070),(#250071,#250072),(#250073,#250074),(#250075,#250076),
(#250077,#250078),(#250079,#250080),(#250081,#250082),(#250083,#250084),
(#250085,#250086),(#250087,#250088),(#250089,#250090),(#250091,#250092),
(#250093,#250094),(#250095,#250096),(#250097,#250098),(#250099,#250100),
(#250101,#250102),(#250103,#250104),(#250105,#250106),(#250107,#250108),
(#250109,#250110),(#250111,#250112),(#250113,#250114),(#250115,#250116),
(#250117,#250118),(#250119,#250120),(#250121,#250122),(#250123,#250124),
(#250125,#250126),(#250127,#250128),(#250129,#250130),(#250131,#250132),
(#250133,#250134),(#250135,#250136),(#250137,#250138),(#250139,#250140),
(#250141,#250142),(#250143,#250144),(#250145,#250146),(#250147,#250148),
(#250149,#250150),(#250151,#250152),(#250153,#250154),(#250155,#250156),
(#250157,#250158),(#250159,#250160),(#250161,#250162),(#250163,#250164),
(#250165,#250166),(#250167,#250168),(#250169,#250170),(#250171,#250172),
(#250173,#250174),(#250175,#250176),(#250177,#250178),(#250179,#250180),
(#250181,#250182),(#250183,#250184),(#250185,#250186),(#250187,#250188),
(#250189,#250190),(#250191,#250192),(#250193,#250194),(#250195,#250196),
(#250197,#250198),(#250199,#250200),(#250201,#250202),(#250203,#250204),
(#250205,#250206),(#250207,#250208),(#250209,#250210),(#250211,#250212),
(#250213,#250214),(#250215,#250216),(#250217,#250218),(#250219,#250220),
(#250221,#250222),(#250223,#250224),(#250225,#250226),(#250227,#250228),
(#250229,#250230),(#250231,#250232),(#250233,#250234),(#250235,#250236),
(#250237,#250238),(#250239,#250240),(#250241,#250242),(#250243,#250244),
(#250245,#250246),(#250247,#250248),(#250249,#250250),(#250251,#250252),
(#250253,#250254),(#250255,#250256),(#250257,#250258),(#250259,#250260),
(#250261,#250262),(#250263,#250264),(#250265,#250266),(#250267,#250268),
(#250269,#250270),(#250271,#250272),(#250273,#250274),(#250275,#250276),
(#250277,#250278),(#250279,#250280)),.UNSPECIFIED.,.F.,.F.,.F.)
B_SPLINE_SURFACE_WITH_KNOTS((6,1,1,1,1,1,1,1,1,1,1,1,1,1,1,1,1,1,1,1,1,
1,1,1,1,1,1,1,1,1,1,1,1,1,1,1,1,1,1,1,1,1,1,1,1,1,1,1,1,1,1,1,1,1,1,1,1,
1,1,1,1,1,1,1,1,1,1,1,1,1,1,1,1,1,1,1,1,1,1,1,1,1,1,1,1,1,1,1,1,1,1,1,1,
1,1,1,1,1,1,1,1,1,1,1,1,1,1,1,1,1,1,1,1,1,1,1,1,1,1,1,1,1,1,1,1,1,1,1,1,
1,1,1,1,1,1,1,1,1,1,1,1,1,1,1,1,1,1,1,1,1,1,1,1,1,1,1,1,1,1,1,1,1,1,1,1,
1,1,1,1,1,1,1,1,1,1,1,1,1,1,1,1,1,1,1,1,1,1,1,1,1,1,1,1,1,1,1,1,1,1,1,6),
(2,2),(0.,0.005,0.01,0.015,0.02,0.025,0.03,0.035,0.04,0.045,0.05,0.055,
0.06,0.065,0.07,0.075,0.08,0.085,0.09,0.095,0.1,0.105,0.11,0.115,0.12,0.125,
0.13,0.135,0.14,0.145,0.15,0.155,0.16,0.165,0.17,0.175,0.18,0.185,0.19,
0.195,0.2,0.205,0.21,0.215,0.22,0.225,0.23,0.235,0.24,0.245,0.25,0.255,
0.26,0.265,0.27,0.275,0.28,0.285,0.29,0.295,0.3,0.305,0.31,0.315,0.32,0.325,
0.33,0.335,0.34,0.345,0.35,0.355,0.36,0.365,0.37,0.375,0.38,0.385,0.39,
0.395,0.4,0.405,0.41,0.415,0.42,0.425,0.43,0.435,0.44,0.445,0.45,0.455,
0.46,0.465,0.47,0.475,0.48,0.485,0.49,0.495,0.5,0.505,0.51,0.515,0.52,0.525,
0.53,0.535,0.54,0.545,0.55,0.555,0.56,0.565,0.57,0.575,0.58,0.585,0.59,
0.595,0.6,0.605,0.61,0.615,0.62,0.625,0.63,0.635,0.64,0.645,0.65,0.655,
0.66,0.665,0.67,0.675,0.68,0.685,0.690000000000001,0.695000000000001,0.700000000000001,
0.705000000000001,0.710000000000001,0.715000000000001,0.720000000000001,
0.725000000000001,0.730000000000001,0.735000000000001,0.740000000000001,
0.745000000000001,0.750000000000001,0.755000000000001,0.760000000000001,
0.765000000000001,0.770000000000001,0.775000000000001,0.780000000000001,
0.785000000000001,0.790000000000001,0.795000000000001,0.800000000000001,
0.805000000000001,0.810000000000001,0.815000000000001,0.820000000000001,
0.825000000000001,0.830000000000001,0.835000000000001,0.840000000000001,
0.845000000000001,0.850000000000001,0.855000000000001,0.860000000000001,
0.865000000000001,0.870000000000001,0.875000000000001,0.880000000000001,
0.885000000000001,0.890000000000001,0.895000000000001,0.900000000000001,
0.905000000000001,0.910000000000001,0.915000000000001,0.920000000000001,
0.925000000000001,0.930000000000001,0.935000000000001,0.940000000000001,
0.945000000000001,0.950000000000001,0.955000000000001,0.960000000000001,
0.965000000000001,0.970000000000001,0.975000000000001,0.980000000000001,
0.985000000000001,0.990000000000001,0.995000000000001,1.),(0.,1.2),
 .UNSPECIFIED.)
GEOMETRIC_REPRESENTATION_ITEM()
RATIONAL_B_SPLINE_SURFACE(((1.,1.),(1.,1.),(1.,1.),(1.,1.),(1.,1.),(1.,
1.),(1.,1.),(1.,1.),(1.,1.),(1.,1.),(1.,1.),(1.,1.),(1.,1.),(1.,1.),(1.,
1.),(1.,1.),(1.,1.),(1.,1.),(1.,1.),(1.,1.),(1.,1.),(1.,1.),(1.,1.),(1.,
1.),(1.,1.),(1.,1.),(1.,1.),(1.,1.),(1.,1.),(1.,1.),(1.,1.),(1.,1.),(1.,
1.),(1.,1.),(1.,1.),(1.,1.),(1.,1.),(1.,1.),(1.,1.),(1.,1.),(1.,1.),(1.,
1.),(1.,1.),(1.,1.),(1.,1.),(1.,1.),(1.,1.),(1.,1.),(1.,1.),(1.,1.),(1.,
1.),(1.,1.),(1.,1.),(1.,1.),(1.,1.),(1.,1.),(1.,1.),(1.,1.),(1.,1.),(1.,
1.),(1.,1.),(1.,1.),(1.,1.),(1.,1.),(1.,1.),(1.,1.),(1.,1.),(1.,1.),(1.,
1.),(1.,1.),(1.,1.),(1.,1.),(1.,1.),(1.,1.),(1.,1.),(1.,1.),(1.,1.),(1.,
1.),(1.,1.),(1.,1.),(1.,1.),(1.,1.),(1.,1.),(1.,1.),(1.,1.),(1.,1.),(1.,
1.),(1.,1.),(1.,1.),(1.,1.),(1.,1.),(1.,1.),(1.,1.),(1.,1.),(1.,1.),(1.,
1.),(1.,1.),(1.,1.),(1.,1.),(1.,1.),(1.,1.),(1.,1.),(1.,1.),(1.,1.),(1.,
1.),(1.,1.),(1.,1.),(1.,1.),(1.,1.),(1.,1.),(1.,1.),(1.,1.),(1.,1.),(1.,
1.),(1.,1.),(1.,1.),(1.,1.),(1.,1.),(1.,1.),(1.,1.),(1.,1.),(1.,1.),(1.,
1.),(1.,1.),(1.,1.),(1.,1.),(1.,1.),(1.,1.),(1.,1.),(1.,1.),(1.,1.),(1.,
1.),(1.,1.),(1.,1.),(1.,1.),(1.,1.),(1.,1.),(1.,1.),(1.,1.),(1.,1.),(1.,
1.),(1.,1.),(1.,1.),(1.,1.),(1.,1.),(1.,1.),(1.,1.),(1.,1.),(1.,1.),(1.,
1.),(1.,1.),(1.,1.),(1.,1.),(1.,1.),(1.,1.),(1.,1.),(1.,1.),(1.,1.),(1.,
1.),(1.,1.),(1.,1.),(1.,1.),(1.,1.),(1.,1.),(1.,1.),(1.,1.),(1.,1.),(1.,
1.),(1.,1.),(1.,1.),(1.,1.),(1.,1.),(1.,1.),(1.,1.),(1.,1.),(1.,1.),(1.,
1.),(1.,1.),(1.,1.),(1.,1.),(1.,1.),(1.,1.),(1.,1.),(1.,1.),(1.,1.),(1.,
1.),(1.,1.),(1.,1.),(1.,1.),(1.,1.),(1.,1.),(1.,1.),(1.,1.),(1.,1.),(1.,
1.),(1.,1.),(1.,1.),(1.,1.),(1.,1.),(1.,1.),(1.,1.),(1.,1.),(1.,1.),(1.,
1.),(1.,1.)))
REPRESENTATION_ITEM('')
SURFACE()
);
#1117=(
BOUNDED_SURFACE()
B_SPLINE_SURFACE(5,1,((#250700,#250701),(#250702,#250703),(#250704,#250705),
(#250706,#250707),(#250708,#250709),(#250710,#250711),(#250712,#250713),
(#250714,#250715),(#250716,#250717),(#250718,#250719),(#250720,#250721),
(#250722,#250723),(#250724,#250725),(#250726,#250727),(#250728,#250729),
(#250730,#250731),(#250732,#250733),(#250734,#250735),(#250736,#250737),
(#250738,#250739),(#250740,#250741),(#250742,#250743),(#250744,#250745),
(#250746,#250747),(#250748,#250749),(#250750,#250751),(#250752,#250753),
(#250754,#250755),(#250756,#250757),(#250758,#250759),(#250760,#250761),
(#250762,#250763),(#250764,#250765),(#250766,#250767),(#250768,#250769),
(#250770,#250771),(#250772,#250773),(#250774,#250775),(#250776,#250777),
(#250778,#250779),(#250780,#250781),(#250782,#250783),(#250784,#250785),
(#250786,#250787),(#250788,#250789),(#250790,#250791),(#250792,#250793),
(#250794,#250795),(#250796,#250797),(#250798,#250799),(#250800,#250801),
(#250802,#250803),(#250804,#250805),(#250806,#250807),(#250808,#250809),
(#250810,#250811),(#250812,#250813),(#250814,#250815),(#250816,#250817),
(#250818,#250819),(#250820,#250821),(#250822,#250823),(#250824,#250825),
(#250826,#250827),(#250828,#250829),(#250830,#250831),(#250832,#250833),
(#250834,#250835),(#250836,#250837),(#250838,#250839),(#250840,#250841),
(#250842,#250843),(#250844,#250845),(#250846,#250847),(#250848,#250849),
(#250850,#250851),(#250852,#250853),(#250854,#250855),(#250856,#250857),
(#250858,#250859),(#250860,#250861),(#250862,#250863),(#250864,#250865),
(#250866,#250867),(#250868,#250869),(#250870,#250871),(#250872,#250873),
(#250874,#250875),(#250876,#250877),(#250878,#250879),(#250880,#250881),
(#250882,#250883),(#250884,#250885),(#250886,#250887),(#250888,#250889),
(#250890,#250891),(#250892,#250893),(#250894,#250895),(#250896,#250897),
(#250898,#250899),(#250900,#250901),(#250902,#250903),(#250904,#250905),
(#250906,#250907),(#250908,#250909),(#250910,#250911),(#250912,#250913),
(#250914,#250915),(#250916,#250917),(#250918,#250919),(#250920,#250921),
(#250922,#250923),(#250924,#250925),(#250926,#250927),(#250928,#250929),
(#250930,#250931),(#250932,#250933),(#250934,#250935),(#250936,#250937),
(#250938,#250939),(#250940,#250941),(#250942,#250943),(#250944,#250945),
(#250946,#250947),(#250948,#250949),(#250950,#250951),(#250952,#250953),
(#250954,#250955),(#250956,#250957),(#250958,#250959),(#250960,#250961),
(#250962,#250963),(#250964,#250965),(#250966,#250967),(#250968,#250969),
(#250970,#250971),(#250972,#250973),(#250974,#250975),(#250976,#250977),
(#250978,#250979),(#250980,#250981),(#250982,#250983),(#250984,#250985),
(#250986,#250987),(#250988,#250989),(#250990,#250991),(#250992,#250993),
(#250994,#250995),(#250996,#250997),(#250998,#250999),(#251000,#251001),
(#251002,#251003),(#251004,#251005),(#251006,#251007),(#251008,#251009),
(#251010,#251011),(#251012,#251013),(#251014,#251015),(#251016,#251017),
(#251018,#251019),(#251020,#251021),(#251022,#251023),(#251024,#251025),
(#251026,#251027),(#251028,#251029),(#251030,#251031),(#251032,#251033),
(#251034,#251035),(#251036,#251037),(#251038,#251039),(#251040,#251041),
(#251042,#251043),(#251044,#251045),(#251046,#251047),(#251048,#251049),
(#251050,#251051),(#251052,#251053),(#251054,#251055),(#251056,#251057),
(#251058,#251059),(#251060,#251061),(#251062,#251063),(#251064,#251065),
(#251066,#251067),(#251068,#251069),(#251070,#251071),(#251072,#251073),
(#251074,#251075),(#251076,#251077),(#251078,#251079),(#251080,#251081),
(#251082,#251083),(#251084,#251085),(#251086,#251087),(#251088,#251089),
(#251090,#251091),(#251092,#251093),(#251094,#251095),(#251096,#251097),
(#251098,#251099),(#251100,#251101),(#251102,#251103),(#251104,#251105),
(#251106,#251107),(#251108,#251109)),.UNSPECIFIED.,.F.,.F.,.F.)
B_SPLINE_SURFACE_WITH_KNOTS((6,1,1,1,1,1,1,1,1,1,1,1,1,1,1,1,1,1,1,1,1,
1,1,1,1,1,1,1,1,1,1,1,1,1,1,1,1,1,1,1,1,1,1,1,1,1,1,1,1,1,1,1,1,1,1,1,1,
1,1,1,1,1,1,1,1,1,1,1,1,1,1,1,1,1,1,1,1,1,1,1,1,1,1,1,1,1,1,1,1,1,1,1,1,
1,1,1,1,1,1,1,1,1,1,1,1,1,1,1,1,1,1,1,1,1,1,1,1,1,1,1,1,1,1,1,1,1,1,1,1,
1,1,1,1,1,1,1,1,1,1,1,1,1,1,1,1,1,1,1,1,1,1,1,1,1,1,1,1,1,1,1,1,1,1,1,1,
1,1,1,1,1,1,1,1,1,1,1,1,1,1,1,1,1,1,1,1,1,1,1,1,1,1,1,1,1,1,1,1,1,1,1,6),
(2,2),(-1.,-0.995000000000001,-0.990000000000001,-0.985000000000001,-0.980000000000001,
-0.975000000000001,-0.970000000000001,-0.965000000000001,-0.960000000000001,
-0.955000000000001,-0.950000000000001,-0.945000000000001,-0.940000000000001,
-0.935000000000001,-0.930000000000001,-0.925000000000001,-0.920000000000001,
-0.915000000000001,-0.910000000000001,-0.905000000000001,-0.900000000000001,
-0.895000000000001,-0.890000000000001,-0.885000000000001,-0.880000000000001,
-0.875000000000001,-0.870000000000001,-0.865000000000001,-0.860000000000001,
-0.855000000000001,-0.850000000000001,-0.845000000000001,-0.840000000000001,
-0.835000000000001,-0.830000000000001,-0.825000000000001,-0.820000000000001,
-0.815000000000001,-0.810000000000001,-0.805000000000001,-0.800000000000001,
-0.795000000000001,-0.790000000000001,-0.785000000000001,-0.780000000000001,
-0.775000000000001,-0.770000000000001,-0.765000000000001,-0.760000000000001,
-0.755000000000001,-0.750000000000001,-0.745000000000001,-0.740000000000001,
-0.735000000000001,-0.730000000000001,-0.725000000000001,-0.720000000000001,
-0.715000000000001,-0.710000000000001,-0.705000000000001,-0.700000000000001,
-0.695000000000001,-0.690000000000001,-0.685,-0.68,-0.675,-0.67,-0.665,
-0.66,-0.655,-0.65,-0.645,-0.64,-0.635,-0.63,-0.625,-0.62,-0.615,-0.61,
-0.605,-0.6,-0.595,-0.59,-0.585,-0.58,-0.575,-0.57,-0.565,-0.56,-0.555,
-0.55,-0.545,-0.54,-0.535,-0.53,-0.525,-0.52,-0.515,-0.51,-0.505,-0.5,-0.495,
-0.49,-0.485,-0.48,-0.475,-0.47,-0.465,-0.46,-0.455,-0.45,-0.445,-0.44,
-0.435,-0.43,-0.425,-0.42,-0.415,-0.41,-0.405,-0.4,-0.395,-0.39,-0.385,
-0.38,-0.375,-0.37,-0.365,-0.36,-0.355,-0.35,-0.345,-0.34,-0.335,-0.33,
-0.325,-0.32,-0.315,-0.31,-0.305,-0.3,-0.295,-0.29,-0.285,-0.28,-0.275,
-0.27,-0.265,-0.26,-0.255,-0.25,-0.245,-0.24,-0.235,-0.23,-0.225,-0.22,
-0.215,-0.21,-0.205,-0.2,-0.195,-0.19,-0.185,-0.18,-0.175,-0.17,-0.165,
-0.16,-0.155,-0.15,-0.145,-0.14,-0.135,-0.13,-0.125,-0.12,-0.115,-0.11,
-0.105,-0.1,-0.095,-0.09,-0.085,-0.08,-0.075,-0.07,-0.065,-0.06,-0.055,
-0.05,-0.045,-0.04,-0.035,-0.03,-0.025,-0.02,-0.015,-0.01,-0.005,0.),(0.,
1.2),.UNSPECIFIED.)
GEOMETRIC_REPRESENTATION_ITEM()
RATIONAL_B_SPLINE_SURFACE(((1.,1.),(1.,1.),(1.,1.),(1.,1.),(1.,1.),(1.,
1.),(1.,1.),(1.,1.),(1.,1.),(1.,1.),(1.,1.),(1.,1.),(1.,1.),(1.,1.),(1.,
1.),(1.,1.),(1.,1.),(1.,1.),(1.,1.),(1.,1.),(1.,1.),(1.,1.),(1.,1.),(1.,
1.),(1.,1.),(1.,1.),(1.,1.),(1.,1.),(1.,1.),(1.,1.),(1.,1.),(1.,1.),(1.,
1.),(1.,1.),(1.,1.),(1.,1.),(1.,1.),(1.,1.),(1.,1.),(1.,1.),(1.,1.),(1.,
1.),(1.,1.),(1.,1.),(1.,1.),(1.,1.),(1.,1.),(1.,1.),(1.,1.),(1.,1.),(1.,
1.),(1.,1.),(1.,1.),(1.,1.),(1.,1.),(1.,1.),(1.,1.),(1.,1.),(1.,1.),(1.,
1.),(1.,1.),(1.,1.),(1.,1.),(1.,1.),(1.,1.),(1.,1.),(1.,1.),(1.,1.),(1.,
1.),(1.,1.),(1.,1.),(1.,1.),(1.,1.),(1.,1.),(1.,1.),(1.,1.),(1.,1.),(1.,
1.),(1.,1.),(1.,1.),(1.,1.),(1.,1.),(1.,1.),(1.,1.),(1.,1.),(1.,1.),(1.,
1.),(1.,1.),(1.,1.),(1.,1.),(1.,1.),(1.,1.),(1.,1.),(1.,1.),(1.,1.),(1.,
1.),(1.,1.),(1.,1.),(1.,1.),(1.,1.),(1.,1.),(1.,1.),(1.,1.),(1.,1.),(1.,
1.),(1.,1.),(1.,1.),(1.,1.),(1.,1.),(1.,1.),(1.,1.),(1.,1.),(1.,1.),(1.,
1.),(1.,1.),(1.,1.),(1.,1.),(1.,1.),(1.,1.),(1.,1.),(1.,1.),(1.,1.),(1.,
1.),(1.,1.),(1.,1.),(1.,1.),(1.,1.),(1.,1.),(1.,1.),(1.,1.),(1.,1.),(1.,
1.),(1.,1.),(1.,1.),(1.,1.),(1.,1.),(1.,1.),(1.,1.),(1.,1.),(1.,1.),(1.,
1.),(1.,1.),(1.,1.),(1.,1.),(1.,1.),(1.,1.),(1.,1.),(1.,1.),(1.,1.),(1.,
1.),(1.,1.),(1.,1.),(1.,1.),(1.,1.),(1.,1.),(1.,1.),(1.,1.),(1.,1.),(1.,
1.),(1.,1.),(1.,1.),(1.,1.),(1.,1.),(1.,1.),(1.,1.),(1.,1.),(1.,1.),(1.,
1.),(1.,1.),(1.,1.),(1.,1.),(1.,1.),(1.,1.),(1.,1.),(1.,1.),(1.,1.),(1.,
1.),(1.,1.),(1.,1.),(1.,1.),(1.,1.),(1.,1.),(1.,1.),(1.,1.),(1.,1.),(1.,
1.),(1.,1.),(1.,1.),(1.,1.),(1.,1.),(1.,1.),(1.,1.),(1.,1.),(1.,1.),(1.,
1.),(1.,1.),(1.,1.),(1.,1.),(1.,1.),(1.,1.),(1.,1.),(1.,1.),(1.,1.),(1.,
1.),(1.,1.)))
REPRESENTATION_ITEM('')
SURFACE()
);
#1118=(
BOUNDED_SURFACE()
B_SPLINE_SURFACE(5,1,((#251523,#251524),(#251525,#251526),(#251527,#251528),
(#251529,#251530),(#251531,#251532),(#251533,#251534),(#251535,#251536),
(#251537,#251538),(#251539,#251540),(#251541,#251542),(#251543,#251544),
(#251545,#251546),(#251547,#251548),(#251549,#251550),(#251551,#251552),
(#251553,#251554),(#251555,#251556),(#251557,#251558),(#251559,#251560),
(#251561,#251562),(#251563,#251564),(#251565,#251566),(#251567,#251568),
(#251569,#251570),(#251571,#251572),(#251573,#251574),(#251575,#251576),
(#251577,#251578),(#251579,#251580),(#251581,#251582),(#251583,#251584),
(#251585,#251586),(#251587,#251588),(#251589,#251590),(#251591,#251592),
(#251593,#251594),(#251595,#251596),(#251597,#251598),(#251599,#251600),
(#251601,#251602),(#251603,#251604),(#251605,#251606),(#251607,#251608),
(#251609,#251610),(#251611,#251612),(#251613,#251614),(#251615,#251616),
(#251617,#251618),(#251619,#251620),(#251621,#251622),(#251623,#251624),
(#251625,#251626),(#251627,#251628),(#251629,#251630),(#251631,#251632),
(#251633,#251634),(#251635,#251636),(#251637,#251638),(#251639,#251640),
(#251641,#251642),(#251643,#251644),(#251645,#251646),(#251647,#251648),
(#251649,#251650),(#251651,#251652),(#251653,#251654),(#251655,#251656),
(#251657,#251658),(#251659,#251660),(#251661,#251662),(#251663,#251664),
(#251665,#251666),(#251667,#251668),(#251669,#251670),(#251671,#251672),
(#251673,#251674),(#251675,#251676),(#251677,#251678),(#251679,#251680),
(#251681,#251682),(#251683,#251684),(#251685,#251686),(#251687,#251688),
(#251689,#251690),(#251691,#251692),(#251693,#251694),(#251695,#251696),
(#251697,#251698),(#251699,#251700),(#251701,#251702),(#251703,#251704),
(#251705,#251706),(#251707,#251708),(#251709,#251710),(#251711,#251712),
(#251713,#251714),(#251715,#251716),(#251717,#251718),(#251719,#251720),
(#251721,#251722),(#251723,#251724),(#251725,#251726),(#251727,#251728),
(#251729,#251730),(#251731,#251732),(#251733,#251734),(#251735,#251736),
(#251737,#251738),(#251739,#251740),(#251741,#251742),(#251743,#251744),
(#251745,#251746),(#251747,#251748),(#251749,#251750),(#251751,#251752),
(#251753,#251754),(#251755,#251756),(#251757,#251758),(#251759,#251760),
(#251761,#251762),(#251763,#251764),(#251765,#251766),(#251767,#251768),
(#251769,#251770),(#251771,#251772),(#251773,#251774),(#251775,#251776),
(#251777,#251778),(#251779,#251780),(#251781,#251782),(#251783,#251784),
(#251785,#251786),(#251787,#251788),(#251789,#251790),(#251791,#251792),
(#251793,#251794),(#251795,#251796),(#251797,#251798),(#251799,#251800),
(#251801,#251802),(#251803,#251804),(#251805,#251806),(#251807,#251808),
(#251809,#251810),(#251811,#251812),(#251813,#251814),(#251815,#251816),
(#251817,#251818),(#251819,#251820),(#251821,#251822),(#251823,#251824),
(#251825,#251826),(#251827,#251828),(#251829,#251830),(#251831,#251832),
(#251833,#251834),(#251835,#251836),(#251837,#251838),(#251839,#251840),
(#251841,#251842),(#251843,#251844),(#251845,#251846),(#251847,#251848),
(#251849,#251850),(#251851,#251852),(#251853,#251854),(#251855,#251856),
(#251857,#251858),(#251859,#251860),(#251861,#251862),(#251863,#251864),
(#251865,#251866),(#251867,#251868),(#251869,#251870),(#251871,#251872),
(#251873,#251874),(#251875,#251876),(#251877,#251878),(#251879,#251880),
(#251881,#251882),(#251883,#251884),(#251885,#251886),(#251887,#251888),
(#251889,#251890),(#251891,#251892),(#251893,#251894),(#251895,#251896),
(#251897,#251898),(#251899,#251900),(#251901,#251902),(#251903,#251904),
(#251905,#251906),(#251907,#251908),(#251909,#251910),(#251911,#251912),
(#251913,#251914),(#251915,#251916),(#251917,#251918),(#251919,#251920),
(#251921,#251922),(#251923,#251924),(#251925,#251926),(#251927,#251928),
(#251929,#251930),(#251931,#251932)),.UNSPECIFIED.,.F.,.F.,.F.)
B_SPLINE_SURFACE_WITH_KNOTS((6,1,1,1,1,1,1,1,1,1,1,1,1,1,1,1,1,1,1,1,1,
1,1,1,1,1,1,1,1,1,1,1,1,1,1,1,1,1,1,1,1,1,1,1,1,1,1,1,1,1,1,1,1,1,1,1,1,
1,1,1,1,1,1,1,1,1,1,1,1,1,1,1,1,1,1,1,1,1,1,1,1,1,1,1,1,1,1,1,1,1,1,1,1,
1,1,1,1,1,1,1,1,1,1,1,1,1,1,1,1,1,1,1,1,1,1,1,1,1,1,1,1,1,1,1,1,1,1,1,1,
1,1,1,1,1,1,1,1,1,1,1,1,1,1,1,1,1,1,1,1,1,1,1,1,1,1,1,1,1,1,1,1,1,1,1,1,
1,1,1,1,1,1,1,1,1,1,1,1,1,1,1,1,1,1,1,1,1,1,1,1,1,1,1,1,1,1,1,1,1,1,1,6),
(2,2),(0.,0.005,0.01,0.015,0.02,0.025,0.03,0.035,0.04,0.045,0.05,0.055,
0.06,0.065,0.07,0.075,0.08,0.085,0.09,0.095,0.1,0.105,0.11,0.115,0.12,0.125,
0.13,0.135,0.14,0.145,0.15,0.155,0.16,0.165,0.17,0.175,0.18,0.185,0.19,
0.195,0.2,0.205,0.21,0.215,0.22,0.225,0.23,0.235,0.24,0.245,0.25,0.255,
0.26,0.265,0.27,0.275,0.28,0.285,0.29,0.295,0.3,0.305,0.31,0.315,0.32,0.325,
0.33,0.335,0.34,0.345,0.35,0.355,0.36,0.365,0.37,0.375,0.38,0.385,0.39,
0.395,0.4,0.405,0.41,0.415,0.42,0.425,0.43,0.435,0.44,0.445,0.45,0.455,
0.46,0.465,0.47,0.475,0.48,0.485,0.49,0.495,0.5,0.505,0.51,0.515,0.52,0.525,
0.53,0.535,0.54,0.545,0.55,0.555,0.56,0.565,0.57,0.575,0.58,0.585,0.59,
0.595,0.6,0.605,0.61,0.615,0.62,0.625,0.63,0.635,0.64,0.645,0.65,0.655,
0.66,0.665,0.67,0.675,0.68,0.685,0.690000000000001,0.695000000000001,0.700000000000001,
0.705000000000001,0.710000000000001,0.715000000000001,0.720000000000001,
0.725000000000001,0.730000000000001,0.735000000000001,0.740000000000001,
0.745000000000001,0.750000000000001,0.755000000000001,0.760000000000001,
0.765000000000001,0.770000000000001,0.775000000000001,0.780000000000001,
0.785000000000001,0.790000000000001,0.795000000000001,0.800000000000001,
0.805000000000001,0.810000000000001,0.815000000000001,0.820000000000001,
0.825000000000001,0.830000000000001,0.835000000000001,0.840000000000001,
0.845000000000001,0.850000000000001,0.855000000000001,0.860000000000001,
0.865000000000001,0.870000000000001,0.875000000000001,0.880000000000001,
0.885000000000001,0.890000000000001,0.895000000000001,0.900000000000001,
0.905000000000001,0.910000000000001,0.915000000000001,0.920000000000001,
0.925000000000001,0.930000000000001,0.935000000000001,0.940000000000001,
0.945000000000001,0.950000000000001,0.955000000000001,0.960000000000001,
0.965000000000001,0.970000000000001,0.975000000000001,0.980000000000001,
0.985000000000001,0.990000000000001,0.995000000000001,1.),(0.,1.2),
 .UNSPECIFIED.)
GEOMETRIC_REPRESENTATION_ITEM()
RATIONAL_B_SPLINE_SURFACE(((1.,1.),(1.,1.),(1.,1.),(1.,1.),(1.,1.),(1.,
1.),(1.,1.),(1.,1.),(1.,1.),(1.,1.),(1.,1.),(1.,1.),(1.,1.),(1.,1.),(1.,
1.),(1.,1.),(1.,1.),(1.,1.),(1.,1.),(1.,1.),(1.,1.),(1.,1.),(1.,1.),(1.,
1.),(1.,1.),(1.,1.),(1.,1.),(1.,1.),(1.,1.),(1.,1.),(1.,1.),(1.,1.),(1.,
1.),(1.,1.),(1.,1.),(1.,1.),(1.,1.),(1.,1.),(1.,1.),(1.,1.),(1.,1.),(1.,
1.),(1.,1.),(1.,1.),(1.,1.),(1.,1.),(1.,1.),(1.,1.),(1.,1.),(1.,1.),(1.,
1.),(1.,1.),(1.,1.),(1.,1.),(1.,1.),(1.,1.),(1.,1.),(1.,1.),(1.,1.),(1.,
1.),(1.,1.),(1.,1.),(1.,1.),(1.,1.),(1.,1.),(1.,1.),(1.,1.),(1.,1.),(1.,
1.),(1.,1.),(1.,1.),(1.,1.),(1.,1.),(1.,1.),(1.,1.),(1.,1.),(1.,1.),(1.,
1.),(1.,1.),(1.,1.),(1.,1.),(1.,1.),(1.,1.),(1.,1.),(1.,1.),(1.,1.),(1.,
1.),(1.,1.),(1.,1.),(1.,1.),(1.,1.),(1.,1.),(1.,1.),(1.,1.),(1.,1.),(1.,
1.),(1.,1.),(1.,1.),(1.,1.),(1.,1.),(1.,1.),(1.,1.),(1.,1.),(1.,1.),(1.,
1.),(1.,1.),(1.,1.),(1.,1.),(1.,1.),(1.,1.),(1.,1.),(1.,1.),(1.,1.),(1.,
1.),(1.,1.),(1.,1.),(1.,1.),(1.,1.),(1.,1.),(1.,1.),(1.,1.),(1.,1.),(1.,
1.),(1.,1.),(1.,1.),(1.,1.),(1.,1.),(1.,1.),(1.,1.),(1.,1.),(1.,1.),(1.,
1.),(1.,1.),(1.,1.),(1.,1.),(1.,1.),(1.,1.),(1.,1.),(1.,1.),(1.,1.),(1.,
1.),(1.,1.),(1.,1.),(1.,1.),(1.,1.),(1.,1.),(1.,1.),(1.,1.),(1.,1.),(1.,
1.),(1.,1.),(1.,1.),(1.,1.),(1.,1.),(1.,1.),(1.,1.),(1.,1.),(1.,1.),(1.,
1.),(1.,1.),(1.,1.),(1.,1.),(1.,1.),(1.,1.),(1.,1.),(1.,1.),(1.,1.),(1.,
1.),(1.,1.),(1.,1.),(1.,1.),(1.,1.),(1.,1.),(1.,1.),(1.,1.),(1.,1.),(1.,
1.),(1.,1.),(1.,1.),(1.,1.),(1.,1.),(1.,1.),(1.,1.),(1.,1.),(1.,1.),(1.,
1.),(1.,1.),(1.,1.),(1.,1.),(1.,1.),(1.,1.),(1.,1.),(1.,1.),(1.,1.),(1.,
1.),(1.,1.),(1.,1.),(1.,1.),(1.,1.),(1.,1.),(1.,1.),(1.,1.),(1.,1.),(1.,
1.),(1.,1.)))
REPRESENTATION_ITEM('')
SURFACE()
);
#1119=(
BOUNDED_SURFACE()
B_SPLINE_SURFACE(5,1,((#252352,#252353),(#252354,#252355),(#252356,#252357),
(#252358,#252359),(#252360,#252361),(#252362,#252363),(#252364,#252365),
(#252366,#252367),(#252368,#252369),(#252370,#252371),(#252372,#252373),
(#252374,#252375),(#252376,#252377),(#252378,#252379),(#252380,#252381),
(#252382,#252383),(#252384,#252385),(#252386,#252387),(#252388,#252389),
(#252390,#252391),(#252392,#252393),(#252394,#252395),(#252396,#252397),
(#252398,#252399),(#252400,#252401),(#252402,#252403),(#252404,#252405),
(#252406,#252407),(#252408,#252409),(#252410,#252411),(#252412,#252413),
(#252414,#252415),(#252416,#252417),(#252418,#252419),(#252420,#252421),
(#252422,#252423),(#252424,#252425),(#252426,#252427),(#252428,#252429),
(#252430,#252431),(#252432,#252433),(#252434,#252435),(#252436,#252437),
(#252438,#252439),(#252440,#252441),(#252442,#252443),(#252444,#252445),
(#252446,#252447),(#252448,#252449),(#252450,#252451),(#252452,#252453),
(#252454,#252455),(#252456,#252457),(#252458,#252459),(#252460,#252461),
(#252462,#252463),(#252464,#252465),(#252466,#252467),(#252468,#252469),
(#252470,#252471),(#252472,#252473),(#252474,#252475),(#252476,#252477),
(#252478,#252479),(#252480,#252481),(#252482,#252483),(#252484,#252485),
(#252486,#252487),(#252488,#252489),(#252490,#252491),(#252492,#252493),
(#252494,#252495),(#252496,#252497),(#252498,#252499),(#252500,#252501),
(#252502,#252503),(#252504,#252505),(#252506,#252507),(#252508,#252509),
(#252510,#252511),(#252512,#252513),(#252514,#252515),(#252516,#252517),
(#252518,#252519),(#252520,#252521),(#252522,#252523),(#252524,#252525),
(#252526,#252527),(#252528,#252529),(#252530,#252531),(#252532,#252533),
(#252534,#252535),(#252536,#252537),(#252538,#252539),(#252540,#252541),
(#252542,#252543),(#252544,#252545),(#252546,#252547),(#252548,#252549),
(#252550,#252551),(#252552,#252553),(#252554,#252555),(#252556,#252557),
(#252558,#252559),(#252560,#252561),(#252562,#252563),(#252564,#252565),
(#252566,#252567),(#252568,#252569),(#252570,#252571),(#252572,#252573),
(#252574,#252575),(#252576,#252577),(#252578,#252579),(#252580,#252581),
(#252582,#252583),(#252584,#252585),(#252586,#252587),(#252588,#252589),
(#252590,#252591),(#252592,#252593),(#252594,#252595),(#252596,#252597),
(#252598,#252599),(#252600,#252601),(#252602,#252603),(#252604,#252605),
(#252606,#252607),(#252608,#252609),(#252610,#252611),(#252612,#252613),
(#252614,#252615),(#252616,#252617),(#252618,#252619),(#252620,#252621),
(#252622,#252623),(#252624,#252625),(#252626,#252627),(#252628,#252629),
(#252630,#252631),(#252632,#252633),(#252634,#252635),(#252636,#252637),
(#252638,#252639),(#252640,#252641),(#252642,#252643),(#252644,#252645),
(#252646,#252647),(#252648,#252649),(#252650,#252651),(#252652,#252653),
(#252654,#252655),(#252656,#252657),(#252658,#252659),(#252660,#252661),
(#252662,#252663),(#252664,#252665),(#252666,#252667),(#252668,#252669),
(#252670,#252671),(#252672,#252673),(#252674,#252675),(#252676,#252677),
(#252678,#252679),(#252680,#252681),(#252682,#252683),(#252684,#252685),
(#252686,#252687),(#252688,#252689),(#252690,#252691),(#252692,#252693),
(#252694,#252695),(#252696,#252697),(#252698,#252699),(#252700,#252701),
(#252702,#252703),(#252704,#252705),(#252706,#252707),(#252708,#252709),
(#252710,#252711),(#252712,#252713),(#252714,#252715),(#252716,#252717),
(#252718,#252719),(#252720,#252721),(#252722,#252723),(#252724,#252725),
(#252726,#252727),(#252728,#252729),(#252730,#252731),(#252732,#252733),
(#252734,#252735),(#252736,#252737),(#252738,#252739),(#252740,#252741),
(#252742,#252743),(#252744,#252745),(#252746,#252747),(#252748,#252749),
(#252750,#252751),(#252752,#252753),(#252754,#252755),(#252756,#252757),
(#252758,#252759),(#252760,#252761)),.UNSPECIFIED.,.F.,.F.,.F.)
B_SPLINE_SURFACE_WITH_KNOTS((6,1,1,1,1,1,1,1,1,1,1,1,1,1,1,1,1,1,1,1,1,
1,1,1,1,1,1,1,1,1,1,1,1,1,1,1,1,1,1,1,1,1,1,1,1,1,1,1,1,1,1,1,1,1,1,1,1,
1,1,1,1,1,1,1,1,1,1,1,1,1,1,1,1,1,1,1,1,1,1,1,1,1,1,1,1,1,1,1,1,1,1,1,1,
1,1,1,1,1,1,1,1,1,1,1,1,1,1,1,1,1,1,1,1,1,1,1,1,1,1,1,1,1,1,1,1,1,1,1,1,
1,1,1,1,1,1,1,1,1,1,1,1,1,1,1,1,1,1,1,1,1,1,1,1,1,1,1,1,1,1,1,1,1,1,1,1,
1,1,1,1,1,1,1,1,1,1,1,1,1,1,1,1,1,1,1,1,1,1,1,1,1,1,1,1,1,1,1,1,1,1,1,6),
(2,2),(-1.,-0.995000000000001,-0.990000000000001,-0.985000000000001,-0.980000000000001,
-0.975000000000001,-0.970000000000001,-0.965000000000001,-0.960000000000001,
-0.955000000000001,-0.950000000000001,-0.945000000000001,-0.940000000000001,
-0.935000000000001,-0.930000000000001,-0.925000000000001,-0.920000000000001,
-0.915000000000001,-0.910000000000001,-0.905000000000001,-0.900000000000001,
-0.895000000000001,-0.890000000000001,-0.885000000000001,-0.880000000000001,
-0.875000000000001,-0.870000000000001,-0.865000000000001,-0.860000000000001,
-0.855000000000001,-0.850000000000001,-0.845000000000001,-0.840000000000001,
-0.835000000000001,-0.830000000000001,-0.825000000000001,-0.820000000000001,
-0.815000000000001,-0.810000000000001,-0.805000000000001,-0.800000000000001,
-0.795000000000001,-0.790000000000001,-0.785000000000001,-0.780000000000001,
-0.775000000000001,-0.770000000000001,-0.765000000000001,-0.760000000000001,
-0.755000000000001,-0.750000000000001,-0.745000000000001,-0.740000000000001,
-0.735000000000001,-0.730000000000001,-0.725000000000001,-0.720000000000001,
-0.715000000000001,-0.710000000000001,-0.705000000000001,-0.700000000000001,
-0.695000000000001,-0.690000000000001,-0.685,-0.68,-0.675,-0.67,-0.665,
-0.66,-0.655,-0.65,-0.645,-0.64,-0.635,-0.63,-0.625,-0.62,-0.615,-0.61,
-0.605,-0.6,-0.595,-0.59,-0.585,-0.58,-0.575,-0.57,-0.565,-0.56,-0.555,
-0.55,-0.545,-0.54,-0.535,-0.53,-0.525,-0.52,-0.515,-0.51,-0.505,-0.5,-0.495,
-0.49,-0.485,-0.48,-0.475,-0.47,-0.465,-0.46,-0.455,-0.45,-0.445,-0.44,
-0.435,-0.43,-0.425,-0.42,-0.415,-0.41,-0.405,-0.4,-0.395,-0.39,-0.385,
-0.38,-0.375,-0.37,-0.365,-0.36,-0.355,-0.35,-0.345,-0.34,-0.335,-0.33,
-0.325,-0.32,-0.315,-0.31,-0.305,-0.3,-0.295,-0.29,-0.285,-0.28,-0.275,
-0.27,-0.265,-0.26,-0.255,-0.25,-0.245,-0.24,-0.235,-0.23,-0.225,-0.22,
-0.215,-0.21,-0.205,-0.2,-0.195,-0.19,-0.185,-0.18,-0.175,-0.17,-0.165,
-0.16,-0.155,-0.15,-0.145,-0.14,-0.135,-0.13,-0.125,-0.12,-0.115,-0.11,
-0.105,-0.1,-0.095,-0.09,-0.085,-0.08,-0.075,-0.07,-0.065,-0.06,-0.055,
-0.05,-0.045,-0.04,-0.035,-0.03,-0.025,-0.02,-0.015,-0.01,-0.005,0.),(0.,
1.2),.UNSPECIFIED.)
GEOMETRIC_REPRESENTATION_ITEM()
RATIONAL_B_SPLINE_SURFACE(((1.,1.),(1.,1.),(1.,1.),(1.,1.),(1.,1.),(1.,
1.),(1.,1.),(1.,1.),(1.,1.),(1.,1.),(1.,1.),(1.,1.),(1.,1.),(1.,1.),(1.,
1.),(1.,1.),(1.,1.),(1.,1.),(1.,1.),(1.,1.),(1.,1.),(1.,1.),(1.,1.),(1.,
1.),(1.,1.),(1.,1.),(1.,1.),(1.,1.),(1.,1.),(1.,1.),(1.,1.),(1.,1.),(1.,
1.),(1.,1.),(1.,1.),(1.,1.),(1.,1.),(1.,1.),(1.,1.),(1.,1.),(1.,1.),(1.,
1.),(1.,1.),(1.,1.),(1.,1.),(1.,1.),(1.,1.),(1.,1.),(1.,1.),(1.,1.),(1.,
1.),(1.,1.),(1.,1.),(1.,1.),(1.,1.),(1.,1.),(1.,1.),(1.,1.),(1.,1.),(1.,
1.),(1.,1.),(1.,1.),(1.,1.),(1.,1.),(1.,1.),(1.,1.),(1.,1.),(1.,1.),(1.,
1.),(1.,1.),(1.,1.),(1.,1.),(1.,1.),(1.,1.),(1.,1.),(1.,1.),(1.,1.),(1.,
1.),(1.,1.),(1.,1.),(1.,1.),(1.,1.),(1.,1.),(1.,1.),(1.,1.),(1.,1.),(1.,
1.),(1.,1.),(1.,1.),(1.,1.),(1.,1.),(1.,1.),(1.,1.),(1.,1.),(1.,1.),(1.,
1.),(1.,1.),(1.,1.),(1.,1.),(1.,1.),(1.,1.),(1.,1.),(1.,1.),(1.,1.),(1.,
1.),(1.,1.),(1.,1.),(1.,1.),(1.,1.),(1.,1.),(1.,1.),(1.,1.),(1.,1.),(1.,
1.),(1.,1.),(1.,1.),(1.,1.),(1.,1.),(1.,1.),(1.,1.),(1.,1.),(1.,1.),(1.,
1.),(1.,1.),(1.,1.),(1.,1.),(1.,1.),(1.,1.),(1.,1.),(1.,1.),(1.,1.),(1.,
1.),(1.,1.),(1.,1.),(1.,1.),(1.,1.),(1.,1.),(1.,1.),(1.,1.),(1.,1.),(1.,
1.),(1.,1.),(1.,1.),(1.,1.),(1.,1.),(1.,1.),(1.,1.),(1.,1.),(1.,1.),(1.,
1.),(1.,1.),(1.,1.),(1.,1.),(1.,1.),(1.,1.),(1.,1.),(1.,1.),(1.,1.),(1.,
1.),(1.,1.),(1.,1.),(1.,1.),(1.,1.),(1.,1.),(1.,1.),(1.,1.),(1.,1.),(1.,
1.),(1.,1.),(1.,1.),(1.,1.),(1.,1.),(1.,1.),(1.,1.),(1.,1.),(1.,1.),(1.,
1.),(1.,1.),(1.,1.),(1.,1.),(1.,1.),(1.,1.),(1.,1.),(1.,1.),(1.,1.),(1.,
1.),(1.,1.),(1.,1.),(1.,1.),(1.,1.),(1.,1.),(1.,1.),(1.,1.),(1.,1.),(1.,
1.),(1.,1.),(1.,1.),(1.,1.),(1.,1.),(1.,1.),(1.,1.),(1.,1.),(1.,1.),(1.,
1.),(1.,1.)))
REPRESENTATION_ITEM('')
SURFACE()
);
#1120=(
BOUNDED_SURFACE()
B_SPLINE_SURFACE(5,1,((#253175,#253176),(#253177,#253178),(#253179,#253180),
(#253181,#253182),(#253183,#253184),(#253185,#253186),(#253187,#253188),
(#253189,#253190),(#253191,#253192),(#253193,#253194),(#253195,#253196),
(#253197,#253198),(#253199,#253200),(#253201,#253202),(#253203,#253204),
(#253205,#253206),(#253207,#253208),(#253209,#253210),(#253211,#253212),
(#253213,#253214),(#253215,#253216),(#253217,#253218),(#253219,#253220),
(#253221,#253222),(#253223,#253224),(#253225,#253226),(#253227,#253228),
(#253229,#253230),(#253231,#253232),(#253233,#253234),(#253235,#253236),
(#253237,#253238),(#253239,#253240),(#253241,#253242),(#253243,#253244),
(#253245,#253246),(#253247,#253248),(#253249,#253250),(#253251,#253252),
(#253253,#253254),(#253255,#253256),(#253257,#253258),(#253259,#253260),
(#253261,#253262),(#253263,#253264),(#253265,#253266),(#253267,#253268),
(#253269,#253270),(#253271,#253272),(#253273,#253274),(#253275,#253276),
(#253277,#253278),(#253279,#253280),(#253281,#253282),(#253283,#253284),
(#253285,#253286),(#253287,#253288),(#253289,#253290),(#253291,#253292),
(#253293,#253294),(#253295,#253296),(#253297,#253298),(#253299,#253300),
(#253301,#253302),(#253303,#253304),(#253305,#253306),(#253307,#253308),
(#253309,#253310),(#253311,#253312),(#253313,#253314),(#253315,#253316),
(#253317,#253318),(#253319,#253320),(#253321,#253322),(#253323,#253324),
(#253325,#253326),(#253327,#253328),(#253329,#253330),(#253331,#253332),
(#253333,#253334),(#253335,#253336),(#253337,#253338),(#253339,#253340),
(#253341,#253342),(#253343,#253344),(#253345,#253346),(#253347,#253348),
(#253349,#253350),(#253351,#253352),(#253353,#253354),(#253355,#253356),
(#253357,#253358),(#253359,#253360),(#253361,#253362),(#253363,#253364),
(#253365,#253366),(#253367,#253368),(#253369,#253370),(#253371,#253372),
(#253373,#253374),(#253375,#253376),(#253377,#253378),(#253379,#253380),
(#253381,#253382),(#253383,#253384),(#253385,#253386),(#253387,#253388),
(#253389,#253390),(#253391,#253392),(#253393,#253394),(#253395,#253396),
(#253397,#253398),(#253399,#253400),(#253401,#253402),(#253403,#253404),
(#253405,#253406),(#253407,#253408),(#253409,#253410),(#253411,#253412),
(#253413,#253414),(#253415,#253416),(#253417,#253418),(#253419,#253420),
(#253421,#253422),(#253423,#253424),(#253425,#253426),(#253427,#253428),
(#253429,#253430),(#253431,#253432),(#253433,#253434),(#253435,#253436),
(#253437,#253438),(#253439,#253440),(#253441,#253442),(#253443,#253444),
(#253445,#253446),(#253447,#253448),(#253449,#253450),(#253451,#253452),
(#253453,#253454),(#253455,#253456),(#253457,#253458),(#253459,#253460),
(#253461,#253462),(#253463,#253464),(#253465,#253466),(#253467,#253468),
(#253469,#253470),(#253471,#253472),(#253473,#253474),(#253475,#253476),
(#253477,#253478),(#253479,#253480),(#253481,#253482),(#253483,#253484),
(#253485,#253486),(#253487,#253488),(#253489,#253490),(#253491,#253492),
(#253493,#253494),(#253495,#253496),(#253497,#253498),(#253499,#253500),
(#253501,#253502),(#253503,#253504),(#253505,#253506),(#253507,#253508),
(#253509,#253510),(#253511,#253512),(#253513,#253514),(#253515,#253516),
(#253517,#253518),(#253519,#253520),(#253521,#253522),(#253523,#253524),
(#253525,#253526),(#253527,#253528),(#253529,#253530),(#253531,#253532),
(#253533,#253534),(#253535,#253536),(#253537,#253538),(#253539,#253540),
(#253541,#253542),(#253543,#253544),(#253545,#253546),(#253547,#253548),
(#253549,#253550),(#253551,#253552),(#253553,#253554),(#253555,#253556),
(#253557,#253558),(#253559,#253560),(#253561,#253562),(#253563,#253564),
(#253565,#253566),(#253567,#253568),(#253569,#253570),(#253571,#253572),
(#253573,#253574),(#253575,#253576),(#253577,#253578),(#253579,#253580),
(#253581,#253582),(#253583,#253584)),.UNSPECIFIED.,.F.,.F.,.F.)
B_SPLINE_SURFACE_WITH_KNOTS((6,1,1,1,1,1,1,1,1,1,1,1,1,1,1,1,1,1,1,1,1,
1,1,1,1,1,1,1,1,1,1,1,1,1,1,1,1,1,1,1,1,1,1,1,1,1,1,1,1,1,1,1,1,1,1,1,1,
1,1,1,1,1,1,1,1,1,1,1,1,1,1,1,1,1,1,1,1,1,1,1,1,1,1,1,1,1,1,1,1,1,1,1,1,
1,1,1,1,1,1,1,1,1,1,1,1,1,1,1,1,1,1,1,1,1,1,1,1,1,1,1,1,1,1,1,1,1,1,1,1,
1,1,1,1,1,1,1,1,1,1,1,1,1,1,1,1,1,1,1,1,1,1,1,1,1,1,1,1,1,1,1,1,1,1,1,1,
1,1,1,1,1,1,1,1,1,1,1,1,1,1,1,1,1,1,1,1,1,1,1,1,1,1,1,1,1,1,1,1,1,1,1,6),
(2,2),(0.,0.005,0.01,0.015,0.02,0.025,0.03,0.035,0.04,0.045,0.05,0.055,
0.06,0.065,0.07,0.075,0.08,0.085,0.09,0.095,0.1,0.105,0.11,0.115,0.12,0.125,
0.13,0.135,0.14,0.145,0.15,0.155,0.16,0.165,0.17,0.175,0.18,0.185,0.19,
0.195,0.2,0.205,0.21,0.215,0.22,0.225,0.23,0.235,0.24,0.245,0.25,0.255,
0.26,0.265,0.27,0.275,0.28,0.285,0.29,0.295,0.3,0.305,0.31,0.315,0.32,0.325,
0.33,0.335,0.34,0.345,0.35,0.355,0.36,0.365,0.37,0.375,0.38,0.385,0.39,
0.395,0.4,0.405,0.41,0.415,0.42,0.425,0.43,0.435,0.44,0.445,0.45,0.455,
0.46,0.465,0.47,0.475,0.48,0.485,0.49,0.495,0.5,0.505,0.51,0.515,0.52,0.525,
0.53,0.535,0.54,0.545,0.55,0.555,0.56,0.565,0.57,0.575,0.58,0.585,0.59,
0.595,0.6,0.605,0.61,0.615,0.62,0.625,0.63,0.635,0.64,0.645,0.65,0.655,
0.66,0.665,0.67,0.675,0.68,0.685,0.690000000000001,0.695000000000001,0.700000000000001,
0.705000000000001,0.710000000000001,0.715000000000001,0.720000000000001,
0.725000000000001,0.730000000000001,0.735000000000001,0.740000000000001,
0.745000000000001,0.750000000000001,0.755000000000001,0.760000000000001,
0.765000000000001,0.770000000000001,0.775000000000001,0.780000000000001,
0.785000000000001,0.790000000000001,0.795000000000001,0.800000000000001,
0.805000000000001,0.810000000000001,0.815000000000001,0.820000000000001,
0.825000000000001,0.830000000000001,0.835000000000001,0.840000000000001,
0.845000000000001,0.850000000000001,0.855000000000001,0.860000000000001,
0.865000000000001,0.870000000000001,0.875000000000001,0.880000000000001,
0.885000000000001,0.890000000000001,0.895000000000001,0.900000000000001,
0.905000000000001,0.910000000000001,0.915000000000001,0.920000000000001,
0.925000000000001,0.930000000000001,0.935000000000001,0.940000000000001,
0.945000000000001,0.950000000000001,0.955000000000001,0.960000000000001,
0.965000000000001,0.970000000000001,0.975000000000001,0.980000000000001,
0.985000000000001,0.990000000000001,0.995000000000001,1.),(0.,1.2),
 .UNSPECIFIED.)
GEOMETRIC_REPRESENTATION_ITEM()
RATIONAL_B_SPLINE_SURFACE(((1.,1.),(1.,1.),(1.,1.),(1.,1.),(1.,1.),(1.,
1.),(1.,1.),(1.,1.),(1.,1.),(1.,1.),(1.,1.),(1.,1.),(1.,1.),(1.,1.),(1.,
1.),(1.,1.),(1.,1.),(1.,1.),(1.,1.),(1.,1.),(1.,1.),(1.,1.),(1.,1.),(1.,
1.),(1.,1.),(1.,1.),(1.,1.),(1.,1.),(1.,1.),(1.,1.),(1.,1.),(1.,1.),(1.,
1.),(1.,1.),(1.,1.),(1.,1.),(1.,1.),(1.,1.),(1.,1.),(1.,1.),(1.,1.),(1.,
1.),(1.,1.),(1.,1.),(1.,1.),(1.,1.),(1.,1.),(1.,1.),(1.,1.),(1.,1.),(1.,
1.),(1.,1.),(1.,1.),(1.,1.),(1.,1.),(1.,1.),(1.,1.),(1.,1.),(1.,1.),(1.,
1.),(1.,1.),(1.,1.),(1.,1.),(1.,1.),(1.,1.),(1.,1.),(1.,1.),(1.,1.),(1.,
1.),(1.,1.),(1.,1.),(1.,1.),(1.,1.),(1.,1.),(1.,1.),(1.,1.),(1.,1.),(1.,
1.),(1.,1.),(1.,1.),(1.,1.),(1.,1.),(1.,1.),(1.,1.),(1.,1.),(1.,1.),(1.,
1.),(1.,1.),(1.,1.),(1.,1.),(1.,1.),(1.,1.),(1.,1.),(1.,1.),(1.,1.),(1.,
1.),(1.,1.),(1.,1.),(1.,1.),(1.,1.),(1.,1.),(1.,1.),(1.,1.),(1.,1.),(1.,
1.),(1.,1.),(1.,1.),(1.,1.),(1.,1.),(1.,1.),(1.,1.),(1.,1.),(1.,1.),(1.,
1.),(1.,1.),(1.,1.),(1.,1.),(1.,1.),(1.,1.),(1.,1.),(1.,1.),(1.,1.),(1.,
1.),(1.,1.),(1.,1.),(1.,1.),(1.,1.),(1.,1.),(1.,1.),(1.,1.),(1.,1.),(1.,
1.),(1.,1.),(1.,1.),(1.,1.),(1.,1.),(1.,1.),(1.,1.),(1.,1.),(1.,1.),(1.,
1.),(1.,1.),(1.,1.),(1.,1.),(1.,1.),(1.,1.),(1.,1.),(1.,1.),(1.,1.),(1.,
1.),(1.,1.),(1.,1.),(1.,1.),(1.,1.),(1.,1.),(1.,1.),(1.,1.),(1.,1.),(1.,
1.),(1.,1.),(1.,1.),(1.,1.),(1.,1.),(1.,1.),(1.,1.),(1.,1.),(1.,1.),(1.,
1.),(1.,1.),(1.,1.),(1.,1.),(1.,1.),(1.,1.),(1.,1.),(1.,1.),(1.,1.),(1.,
1.),(1.,1.),(1.,1.),(1.,1.),(1.,1.),(1.,1.),(1.,1.),(1.,1.),(1.,1.),(1.,
1.),(1.,1.),(1.,1.),(1.,1.),(1.,1.),(1.,1.),(1.,1.),(1.,1.),(1.,1.),(1.,
1.),(1.,1.),(1.,1.),(1.,1.),(1.,1.),(1.,1.),(1.,1.),(1.,1.),(1.,1.),(1.,
1.),(1.,1.)))
REPRESENTATION_ITEM('')
SURFACE()
);
#1121=(
BOUNDED_SURFACE()
B_SPLINE_SURFACE(5,1,((#254933,#254934),(#254935,#254936),(#254937,#254938),
(#254939,#254940),(#254941,#254942),(#254943,#254944),(#254945,#254946),
(#254947,#254948),(#254949,#254950),(#254951,#254952),(#254953,#254954),
(#254955,#254956),(#254957,#254958),(#254959,#254960),(#254961,#254962),
(#254963,#254964),(#254965,#254966),(#254967,#254968),(#254969,#254970),
(#254971,#254972),(#254973,#254974),(#254975,#254976),(#254977,#254978),
(#254979,#254980),(#254981,#254982),(#254983,#254984),(#254985,#254986),
(#254987,#254988),(#254989,#254990),(#254991,#254992),(#254993,#254994),
(#254995,#254996),(#254997,#254998),(#254999,#255000),(#255001,#255002),
(#255003,#255004),(#255005,#255006),(#255007,#255008),(#255009,#255010),
(#255011,#255012),(#255013,#255014),(#255015,#255016),(#255017,#255018),
(#255019,#255020),(#255021,#255022),(#255023,#255024),(#255025,#255026),
(#255027,#255028),(#255029,#255030),(#255031,#255032),(#255033,#255034),
(#255035,#255036),(#255037,#255038),(#255039,#255040),(#255041,#255042),
(#255043,#255044),(#255045,#255046),(#255047,#255048),(#255049,#255050),
(#255051,#255052),(#255053,#255054),(#255055,#255056),(#255057,#255058),
(#255059,#255060),(#255061,#255062),(#255063,#255064),(#255065,#255066),
(#255067,#255068),(#255069,#255070),(#255071,#255072),(#255073,#255074),
(#255075,#255076),(#255077,#255078),(#255079,#255080),(#255081,#255082),
(#255083,#255084),(#255085,#255086),(#255087,#255088),(#255089,#255090),
(#255091,#255092),(#255093,#255094),(#255095,#255096),(#255097,#255098),
(#255099,#255100),(#255101,#255102),(#255103,#255104),(#255105,#255106),
(#255107,#255108),(#255109,#255110),(#255111,#255112),(#255113,#255114),
(#255115,#255116),(#255117,#255118),(#255119,#255120),(#255121,#255122),
(#255123,#255124),(#255125,#255126),(#255127,#255128),(#255129,#255130),
(#255131,#255132),(#255133,#255134),(#255135,#255136),(#255137,#255138),
(#255139,#255140),(#255141,#255142),(#255143,#255144),(#255145,#255146),
(#255147,#255148),(#255149,#255150),(#255151,#255152),(#255153,#255154),
(#255155,#255156),(#255157,#255158),(#255159,#255160),(#255161,#255162),
(#255163,#255164),(#255165,#255166),(#255167,#255168),(#255169,#255170),
(#255171,#255172),(#255173,#255174),(#255175,#255176),(#255177,#255178),
(#255179,#255180),(#255181,#255182),(#255183,#255184),(#255185,#255186),
(#255187,#255188),(#255189,#255190),(#255191,#255192),(#255193,#255194),
(#255195,#255196),(#255197,#255198),(#255199,#255200),(#255201,#255202),
(#255203,#255204),(#255205,#255206),(#255207,#255208),(#255209,#255210),
(#255211,#255212),(#255213,#255214),(#255215,#255216),(#255217,#255218),
(#255219,#255220),(#255221,#255222),(#255223,#255224),(#255225,#255226),
(#255227,#255228),(#255229,#255230),(#255231,#255232),(#255233,#255234),
(#255235,#255236),(#255237,#255238),(#255239,#255240),(#255241,#255242),
(#255243,#255244),(#255245,#255246),(#255247,#255248),(#255249,#255250),
(#255251,#255252),(#255253,#255254),(#255255,#255256),(#255257,#255258),
(#255259,#255260),(#255261,#255262),(#255263,#255264),(#255265,#255266),
(#255267,#255268),(#255269,#255270),(#255271,#255272),(#255273,#255274),
(#255275,#255276),(#255277,#255278),(#255279,#255280),(#255281,#255282),
(#255283,#255284),(#255285,#255286),(#255287,#255288),(#255289,#255290),
(#255291,#255292),(#255293,#255294),(#255295,#255296),(#255297,#255298),
(#255299,#255300),(#255301,#255302),(#255303,#255304),(#255305,#255306),
(#255307,#255308),(#255309,#255310),(#255311,#255312),(#255313,#255314),
(#255315,#255316),(#255317,#255318),(#255319,#255320),(#255321,#255322),
(#255323,#255324),(#255325,#255326),(#255327,#255328),(#255329,#255330),
(#255331,#255332),(#255333,#255334),(#255335,#255336),(#255337,#255338),
(#255339,#255340),(#255341,#255342)),.UNSPECIFIED.,.F.,.F.,.F.)
B_SPLINE_SURFACE_WITH_KNOTS((6,1,1,1,1,1,1,1,1,1,1,1,1,1,1,1,1,1,1,1,1,
1,1,1,1,1,1,1,1,1,1,1,1,1,1,1,1,1,1,1,1,1,1,1,1,1,1,1,1,1,1,1,1,1,1,1,1,
1,1,1,1,1,1,1,1,1,1,1,1,1,1,1,1,1,1,1,1,1,1,1,1,1,1,1,1,1,1,1,1,1,1,1,1,
1,1,1,1,1,1,1,1,1,1,1,1,1,1,1,1,1,1,1,1,1,1,1,1,1,1,1,1,1,1,1,1,1,1,1,1,
1,1,1,1,1,1,1,1,1,1,1,1,1,1,1,1,1,1,1,1,1,1,1,1,1,1,1,1,1,1,1,1,1,1,1,1,
1,1,1,1,1,1,1,1,1,1,1,1,1,1,1,1,1,1,1,1,1,1,1,1,1,1,1,1,1,1,1,1,1,1,1,6),
(2,2),(-1.,-0.995000000000001,-0.990000000000001,-0.985000000000001,-0.980000000000001,
-0.975000000000001,-0.970000000000001,-0.965000000000001,-0.960000000000001,
-0.955000000000001,-0.950000000000001,-0.945000000000001,-0.940000000000001,
-0.935000000000001,-0.930000000000001,-0.925000000000001,-0.920000000000001,
-0.915000000000001,-0.910000000000001,-0.905000000000001,-0.900000000000001,
-0.895000000000001,-0.890000000000001,-0.885000000000001,-0.880000000000001,
-0.875000000000001,-0.870000000000001,-0.865000000000001,-0.860000000000001,
-0.855000000000001,-0.850000000000001,-0.845000000000001,-0.840000000000001,
-0.835000000000001,-0.830000000000001,-0.825000000000001,-0.820000000000001,
-0.815000000000001,-0.810000000000001,-0.805000000000001,-0.800000000000001,
-0.795000000000001,-0.790000000000001,-0.785000000000001,-0.780000000000001,
-0.775000000000001,-0.770000000000001,-0.765000000000001,-0.760000000000001,
-0.755000000000001,-0.750000000000001,-0.745000000000001,-0.740000000000001,
-0.735000000000001,-0.730000000000001,-0.725000000000001,-0.720000000000001,
-0.715000000000001,-0.710000000000001,-0.705000000000001,-0.700000000000001,
-0.695000000000001,-0.690000000000001,-0.685,-0.68,-0.675,-0.67,-0.665,
-0.66,-0.655,-0.65,-0.645,-0.64,-0.635,-0.63,-0.625,-0.62,-0.615,-0.61,
-0.605,-0.6,-0.595,-0.59,-0.585,-0.58,-0.575,-0.57,-0.565,-0.56,-0.555,
-0.55,-0.545,-0.54,-0.535,-0.53,-0.525,-0.52,-0.515,-0.51,-0.505,-0.5,-0.495,
-0.49,-0.485,-0.48,-0.475,-0.47,-0.465,-0.46,-0.455,-0.45,-0.445,-0.44,
-0.435,-0.43,-0.425,-0.42,-0.415,-0.41,-0.405,-0.4,-0.395,-0.39,-0.385,
-0.38,-0.375,-0.37,-0.365,-0.36,-0.355,-0.35,-0.345,-0.34,-0.335,-0.33,
-0.325,-0.32,-0.315,-0.31,-0.305,-0.3,-0.295,-0.29,-0.285,-0.28,-0.275,
-0.27,-0.265,-0.26,-0.255,-0.25,-0.245,-0.24,-0.235,-0.23,-0.225,-0.22,
-0.215,-0.21,-0.205,-0.2,-0.195,-0.19,-0.185,-0.18,-0.175,-0.17,-0.165,
-0.16,-0.155,-0.15,-0.145,-0.14,-0.135,-0.13,-0.125,-0.12,-0.115,-0.11,
-0.105,-0.1,-0.095,-0.09,-0.085,-0.08,-0.075,-0.07,-0.065,-0.06,-0.055,
-0.05,-0.045,-0.04,-0.035,-0.03,-0.025,-0.02,-0.015,-0.01,-0.005,0.),(0.,
1.2),.UNSPECIFIED.)
GEOMETRIC_REPRESENTATION_ITEM()
RATIONAL_B_SPLINE_SURFACE(((1.,1.),(1.,1.),(1.,1.),(1.,1.),(1.,1.),(1.,
1.),(1.,1.),(1.,1.),(1.,1.),(1.,1.),(1.,1.),(1.,1.),(1.,1.),(1.,1.),(1.,
1.),(1.,1.),(1.,1.),(1.,1.),(1.,1.),(1.,1.),(1.,1.),(1.,1.),(1.,1.),(1.,
1.),(1.,1.),(1.,1.),(1.,1.),(1.,1.),(1.,1.),(1.,1.),(1.,1.),(1.,1.),(1.,
1.),(1.,1.),(1.,1.),(1.,1.),(1.,1.),(1.,1.),(1.,1.),(1.,1.),(1.,1.),(1.,
1.),(1.,1.),(1.,1.),(1.,1.),(1.,1.),(1.,1.),(1.,1.),(1.,1.),(1.,1.),(1.,
1.),(1.,1.),(1.,1.),(1.,1.),(1.,1.),(1.,1.),(1.,1.),(1.,1.),(1.,1.),(1.,
1.),(1.,1.),(1.,1.),(1.,1.),(1.,1.),(1.,1.),(1.,1.),(1.,1.),(1.,1.),(1.,
1.),(1.,1.),(1.,1.),(1.,1.),(1.,1.),(1.,1.),(1.,1.),(1.,1.),(1.,1.),(1.,
1.),(1.,1.),(1.,1.),(1.,1.),(1.,1.),(1.,1.),(1.,1.),(1.,1.),(1.,1.),(1.,
1.),(1.,1.),(1.,1.),(1.,1.),(1.,1.),(1.,1.),(1.,1.),(1.,1.),(1.,1.),(1.,
1.),(1.,1.),(1.,1.),(1.,1.),(1.,1.),(1.,1.),(1.,1.),(1.,1.),(1.,1.),(1.,
1.),(1.,1.),(1.,1.),(1.,1.),(1.,1.),(1.,1.),(1.,1.),(1.,1.),(1.,1.),(1.,
1.),(1.,1.),(1.,1.),(1.,1.),(1.,1.),(1.,1.),(1.,1.),(1.,1.),(1.,1.),(1.,
1.),(1.,1.),(1.,1.),(1.,1.),(1.,1.),(1.,1.),(1.,1.),(1.,1.),(1.,1.),(1.,
1.),(1.,1.),(1.,1.),(1.,1.),(1.,1.),(1.,1.),(1.,1.),(1.,1.),(1.,1.),(1.,
1.),(1.,1.),(1.,1.),(1.,1.),(1.,1.),(1.,1.),(1.,1.),(1.,1.),(1.,1.),(1.,
1.),(1.,1.),(1.,1.),(1.,1.),(1.,1.),(1.,1.),(1.,1.),(1.,1.),(1.,1.),(1.,
1.),(1.,1.),(1.,1.),(1.,1.),(1.,1.),(1.,1.),(1.,1.),(1.,1.),(1.,1.),(1.,
1.),(1.,1.),(1.,1.),(1.,1.),(1.,1.),(1.,1.),(1.,1.),(1.,1.),(1.,1.),(1.,
1.),(1.,1.),(1.,1.),(1.,1.),(1.,1.),(1.,1.),(1.,1.),(1.,1.),(1.,1.),(1.,
1.),(1.,1.),(1.,1.),(1.,1.),(1.,1.),(1.,1.),(1.,1.),(1.,1.),(1.,1.),(1.,
1.),(1.,1.),(1.,1.),(1.,1.),(1.,1.),(1.,1.),(1.,1.),(1.,1.),(1.,1.),(1.,
1.),(1.,1.)))
REPRESENTATION_ITEM('')
SURFACE()
);
#1122=(
BOUNDED_SURFACE()
B_SPLINE_SURFACE(5,1,((#255343,#255344),(#255345,#255346),(#255347,#255348),
(#255349,#255350),(#255351,#255352),(#255353,#255354),(#255355,#255356),
(#255357,#255358),(#255359,#255360),(#255361,#255362),(#255363,#255364),
(#255365,#255366),(#255367,#255368),(#255369,#255370),(#255371,#255372),
(#255373,#255374),(#255375,#255376),(#255377,#255378),(#255379,#255380),
(#255381,#255382),(#255383,#255384),(#255385,#255386),(#255387,#255388),
(#255389,#255390),(#255391,#255392),(#255393,#255394),(#255395,#255396),
(#255397,#255398),(#255399,#255400),(#255401,#255402),(#255403,#255404),
(#255405,#255406),(#255407,#255408),(#255409,#255410),(#255411,#255412),
(#255413,#255414),(#255415,#255416),(#255417,#255418),(#255419,#255420),
(#255421,#255422),(#255423,#255424),(#255425,#255426),(#255427,#255428),
(#255429,#255430),(#255431,#255432),(#255433,#255434),(#255435,#255436),
(#255437,#255438),(#255439,#255440),(#255441,#255442),(#255443,#255444),
(#255445,#255446),(#255447,#255448),(#255449,#255450),(#255451,#255452),
(#255453,#255454),(#255455,#255456),(#255457,#255458),(#255459,#255460),
(#255461,#255462),(#255463,#255464),(#255465,#255466),(#255467,#255468),
(#255469,#255470),(#255471,#255472),(#255473,#255474),(#255475,#255476),
(#255477,#255478),(#255479,#255480),(#255481,#255482),(#255483,#255484),
(#255485,#255486),(#255487,#255488),(#255489,#255490),(#255491,#255492),
(#255493,#255494),(#255495,#255496),(#255497,#255498),(#255499,#255500),
(#255501,#255502),(#255503,#255504),(#255505,#255506),(#255507,#255508),
(#255509,#255510),(#255511,#255512),(#255513,#255514),(#255515,#255516),
(#255517,#255518),(#255519,#255520),(#255521,#255522),(#255523,#255524),
(#255525,#255526),(#255527,#255528),(#255529,#255530),(#255531,#255532),
(#255533,#255534),(#255535,#255536),(#255537,#255538),(#255539,#255540),
(#255541,#255542),(#255543,#255544),(#255545,#255546),(#255547,#255548),
(#255549,#255550),(#255551,#255552),(#255553,#255554),(#255555,#255556),
(#255557,#255558),(#255559,#255560),(#255561,#255562),(#255563,#255564),
(#255565,#255566),(#255567,#255568),(#255569,#255570),(#255571,#255572),
(#255573,#255574),(#255575,#255576),(#255577,#255578),(#255579,#255580),
(#255581,#255582),(#255583,#255584),(#255585,#255586),(#255587,#255588),
(#255589,#255590),(#255591,#255592),(#255593,#255594),(#255595,#255596),
(#255597,#255598),(#255599,#255600),(#255601,#255602),(#255603,#255604),
(#255605,#255606),(#255607,#255608),(#255609,#255610),(#255611,#255612),
(#255613,#255614),(#255615,#255616),(#255617,#255618),(#255619,#255620),
(#255621,#255622),(#255623,#255624),(#255625,#255626),(#255627,#255628),
(#255629,#255630),(#255631,#255632),(#255633,#255634),(#255635,#255636),
(#255637,#255638),(#255639,#255640),(#255641,#255642),(#255643,#255644),
(#255645,#255646),(#255647,#255648),(#255649,#255650),(#255651,#255652),
(#255653,#255654),(#255655,#255656),(#255657,#255658),(#255659,#255660),
(#255661,#255662),(#255663,#255664),(#255665,#255666),(#255667,#255668),
(#255669,#255670),(#255671,#255672),(#255673,#255674),(#255675,#255676),
(#255677,#255678),(#255679,#255680),(#255681,#255682),(#255683,#255684),
(#255685,#255686),(#255687,#255688),(#255689,#255690),(#255691,#255692),
(#255693,#255694),(#255695,#255696),(#255697,#255698),(#255699,#255700),
(#255701,#255702),(#255703,#255704),(#255705,#255706),(#255707,#255708),
(#255709,#255710),(#255711,#255712),(#255713,#255714),(#255715,#255716),
(#255717,#255718),(#255719,#255720),(#255721,#255722),(#255723,#255724),
(#255725,#255726),(#255727,#255728),(#255729,#255730),(#255731,#255732),
(#255733,#255734),(#255735,#255736),(#255737,#255738),(#255739,#255740),
(#255741,#255742),(#255743,#255744),(#255745,#255746),(#255747,#255748),
(#255749,#255750),(#255751,#255752)),.UNSPECIFIED.,.F.,.F.,.F.)
B_SPLINE_SURFACE_WITH_KNOTS((6,1,1,1,1,1,1,1,1,1,1,1,1,1,1,1,1,1,1,1,1,
1,1,1,1,1,1,1,1,1,1,1,1,1,1,1,1,1,1,1,1,1,1,1,1,1,1,1,1,1,1,1,1,1,1,1,1,
1,1,1,1,1,1,1,1,1,1,1,1,1,1,1,1,1,1,1,1,1,1,1,1,1,1,1,1,1,1,1,1,1,1,1,1,
1,1,1,1,1,1,1,1,1,1,1,1,1,1,1,1,1,1,1,1,1,1,1,1,1,1,1,1,1,1,1,1,1,1,1,1,
1,1,1,1,1,1,1,1,1,1,1,1,1,1,1,1,1,1,1,1,1,1,1,1,1,1,1,1,1,1,1,1,1,1,1,1,
1,1,1,1,1,1,1,1,1,1,1,1,1,1,1,1,1,1,1,1,1,1,1,1,1,1,1,1,1,1,1,1,1,1,1,6),
(2,2),(0.,0.005,0.01,0.015,0.02,0.025,0.03,0.035,0.04,0.045,0.05,0.055,
0.06,0.065,0.07,0.075,0.08,0.085,0.09,0.095,0.1,0.105,0.11,0.115,0.12,0.125,
0.13,0.135,0.14,0.145,0.15,0.155,0.16,0.165,0.17,0.175,0.18,0.185,0.19,
0.195,0.2,0.205,0.21,0.215,0.22,0.225,0.23,0.235,0.24,0.245,0.25,0.255,
0.26,0.265,0.27,0.275,0.28,0.285,0.29,0.295,0.3,0.305,0.31,0.315,0.32,0.325,
0.33,0.335,0.34,0.345,0.35,0.355,0.36,0.365,0.37,0.375,0.38,0.385,0.39,
0.395,0.4,0.405,0.41,0.415,0.42,0.425,0.43,0.435,0.44,0.445,0.45,0.455,
0.46,0.465,0.47,0.475,0.48,0.485,0.49,0.495,0.5,0.505,0.51,0.515,0.52,0.525,
0.53,0.535,0.54,0.545,0.55,0.555,0.56,0.565,0.57,0.575,0.58,0.585,0.59,
0.595,0.6,0.605,0.61,0.615,0.62,0.625,0.63,0.635,0.64,0.645,0.65,0.655,
0.66,0.665,0.67,0.675,0.68,0.685,0.690000000000001,0.695000000000001,0.700000000000001,
0.705000000000001,0.710000000000001,0.715000000000001,0.720000000000001,
0.725000000000001,0.730000000000001,0.735000000000001,0.740000000000001,
0.745000000000001,0.750000000000001,0.755000000000001,0.760000000000001,
0.765000000000001,0.770000000000001,0.775000000000001,0.780000000000001,
0.785000000000001,0.790000000000001,0.795000000000001,0.800000000000001,
0.805000000000001,0.810000000000001,0.815000000000001,0.820000000000001,
0.825000000000001,0.830000000000001,0.835000000000001,0.840000000000001,
0.845000000000001,0.850000000000001,0.855000000000001,0.860000000000001,
0.865000000000001,0.870000000000001,0.875000000000001,0.880000000000001,
0.885000000000001,0.890000000000001,0.895000000000001,0.900000000000001,
0.905000000000001,0.910000000000001,0.915000000000001,0.920000000000001,
0.925000000000001,0.930000000000001,0.935000000000001,0.940000000000001,
0.945000000000001,0.950000000000001,0.955000000000001,0.960000000000001,
0.965000000000001,0.970000000000001,0.975000000000001,0.980000000000001,
0.985000000000001,0.990000000000001,0.995000000000001,1.),(0.,1.2),
 .UNSPECIFIED.)
GEOMETRIC_REPRESENTATION_ITEM()
RATIONAL_B_SPLINE_SURFACE(((1.,1.),(1.,1.),(1.,1.),(1.,1.),(1.,1.),(1.,
1.),(1.,1.),(1.,1.),(1.,1.),(1.,1.),(1.,1.),(1.,1.),(1.,1.),(1.,1.),(1.,
1.),(1.,1.),(1.,1.),(1.,1.),(1.,1.),(1.,1.),(1.,1.),(1.,1.),(1.,1.),(1.,
1.),(1.,1.),(1.,1.),(1.,1.),(1.,1.),(1.,1.),(1.,1.),(1.,1.),(1.,1.),(1.,
1.),(1.,1.),(1.,1.),(1.,1.),(1.,1.),(1.,1.),(1.,1.),(1.,1.),(1.,1.),(1.,
1.),(1.,1.),(1.,1.),(1.,1.),(1.,1.),(1.,1.),(1.,1.),(1.,1.),(1.,1.),(1.,
1.),(1.,1.),(1.,1.),(1.,1.),(1.,1.),(1.,1.),(1.,1.),(1.,1.),(1.,1.),(1.,
1.),(1.,1.),(1.,1.),(1.,1.),(1.,1.),(1.,1.),(1.,1.),(1.,1.),(1.,1.),(1.,
1.),(1.,1.),(1.,1.),(1.,1.),(1.,1.),(1.,1.),(1.,1.),(1.,1.),(1.,1.),(1.,
1.),(1.,1.),(1.,1.),(1.,1.),(1.,1.),(1.,1.),(1.,1.),(1.,1.),(1.,1.),(1.,
1.),(1.,1.),(1.,1.),(1.,1.),(1.,1.),(1.,1.),(1.,1.),(1.,1.),(1.,1.),(1.,
1.),(1.,1.),(1.,1.),(1.,1.),(1.,1.),(1.,1.),(1.,1.),(1.,1.),(1.,1.),(1.,
1.),(1.,1.),(1.,1.),(1.,1.),(1.,1.),(1.,1.),(1.,1.),(1.,1.),(1.,1.),(1.,
1.),(1.,1.),(1.,1.),(1.,1.),(1.,1.),(1.,1.),(1.,1.),(1.,1.),(1.,1.),(1.,
1.),(1.,1.),(1.,1.),(1.,1.),(1.,1.),(1.,1.),(1.,1.),(1.,1.),(1.,1.),(1.,
1.),(1.,1.),(1.,1.),(1.,1.),(1.,1.),(1.,1.),(1.,1.),(1.,1.),(1.,1.),(1.,
1.),(1.,1.),(1.,1.),(1.,1.),(1.,1.),(1.,1.),(1.,1.),(1.,1.),(1.,1.),(1.,
1.),(1.,1.),(1.,1.),(1.,1.),(1.,1.),(1.,1.),(1.,1.),(1.,1.),(1.,1.),(1.,
1.),(1.,1.),(1.,1.),(1.,1.),(1.,1.),(1.,1.),(1.,1.),(1.,1.),(1.,1.),(1.,
1.),(1.,1.),(1.,1.),(1.,1.),(1.,1.),(1.,1.),(1.,1.),(1.,1.),(1.,1.),(1.,
1.),(1.,1.),(1.,1.),(1.,1.),(1.,1.),(1.,1.),(1.,1.),(1.,1.),(1.,1.),(1.,
1.),(1.,1.),(1.,1.),(1.,1.),(1.,1.),(1.,1.),(1.,1.),(1.,1.),(1.,1.),(1.,
1.),(1.,1.),(1.,1.),(1.,1.),(1.,1.),(1.,1.),(1.,1.),(1.,1.),(1.,1.),(1.,
1.),(1.,1.)))
REPRESENTATION_ITEM('')
SURFACE()
);
#1129=SHAPE_REPRESENTATION_RELATIONSHIP('SRR','None',#259376,#1149);
#1149=ADVANCED_BREP_SHAPE_REPRESENTATION('',(#1189),#259210);
#1169=STYLED_ITEM('',(#259484),#1189);
#1189=MANIFOLD_SOLID_BREP('Gear blank',#25156);
#1283=FACE_BOUND('',#4293,.T.);
#1284=FACE_BOUND('',#4295,.T.);
#1585=PLANE('',#26663);
#1586=PLANE('',#26673);
#1587=PLANE('',#26683);
#1588=PLANE('',#26693);
#1589=PLANE('',#26703);
#1590=PLANE('',#26713);
#1591=PLANE('',#26723);
#1592=PLANE('',#26733);
#1593=PLANE('',#26743);
#1594=PLANE('',#26753);
#1595=PLANE('',#26763);
#1596=PLANE('',#26773);
#1597=PLANE('',#26783);
#1598=PLANE('',#26793);
#1599=PLANE('',#26803);
#1600=PLANE('',#26813);
#1601=PLANE('',#26823);
#1602=PLANE('',#26833);
#1603=PLANE('',#26843);
#1604=PLANE('',#26853);
#1605=PLANE('',#26863);
#1606=PLANE('',#26873);
#1607=PLANE('',#26883);
#1608=PLANE('',#26890);
#1609=PLANE('',#26891);
#1610=PLANE('',#26892);
#1611=PLANE('',#26893);
#1612=PLANE('',#26894);
#1613=PLANE('',#26895);
#1614=PLANE('',#26896);
#1615=PLANE('',#26897);
#1616=PLANE('',#26898);
#1617=PLANE('',#26899);
#1618=PLANE('',#26900);
#1619=PLANE('',#26901);
#1620=PLANE('',#26902);
#1621=PLANE('',#26903);
#1622=PLANE('',#26904);
#1623=PLANE('',#26905);
#1624=PLANE('',#26906);
#1625=PLANE('',#26907);
#1626=PLANE('',#26908);
#1627=PLANE('',#26909);
#1628=PLANE('',#26910);
#1629=PLANE('',#26911);
#1630=PLANE('',#26912);
#1631=PLANE('',#26913);
#1632=PLANE('',#26942);
#1633=PLANE('',#26995);
#1634=PLANE('',#26998);
#2705=FACE_OUTER_BOUND('',#4131,.T.);
#2706=FACE_OUTER_BOUND('',#4132,.T.);
#2707=FACE_OUTER_BOUND('',#4133,.T.);
#2708=FACE_OUTER_BOUND('',#4134,.T.);
#2709=FACE_OUTER_BOUND('',#4135,.T.);
#2710=FACE_OUTER_BOUND('',#4136,.T.);
#2711=FACE_OUTER_BOUND('',#4137,.T.);
#2712=FACE_OUTER_BOUND('',#4138,.T.);
#2713=FACE_OUTER_BOUND('',#4139,.T.);
#2714=FACE_OUTER_BOUND('',#4140,.T.);
#2715=FACE_OUTER_BOUND('',#4141,.T.);
#2716=FACE_OUTER_BOUND('',#4142,.T.);
#2717=FACE_OUTER_BOUND('',#4143,.T.);
#2718=FACE_OUTER_BOUND('',#4144,.T.);
#2719=FACE_OUTER_BOUND('',#4145,.T.);
#2720=FACE_OUTER_BOUND('',#4146,.T.);
#2721=FACE_OUTER_BOUND('',#4147,.T.);
#2722=FACE_OUTER_BOUND('',#4148,.T.);
#2723=FACE_OUTER_BOUND('',#4149,.T.);
#2724=FACE_OUTER_BOUND('',#4150,.T.);
#2725=FACE_OUTER_BOUND('',#4151,.T.);
#2726=FACE_OUTER_BOUND('',#4152,.T.);
#2727=FACE_OUTER_BOUND('',#4153,.T.);
#2728=FACE_OUTER_BOUND('',#4154,.T.);
#2729=FACE_OUTER_BOUND('',#4155,.T.);
#2730=FACE_OUTER_BOUND('',#4156,.T.);
#2731=FACE_OUTER_BOUND('',#4157,.T.);
#2732=FACE_OUTER_BOUND('',#4158,.T.);
#2733=FACE_OUTER_BOUND('',#4159,.T.);
#2734=FACE_OUTER_BOUND('',#4160,.T.);
#2735=FACE_OUTER_BOUND('',#4161,.T.);
#2736=FACE_OUTER_BOUND('',#4162,.T.);
#2737=FACE_OUTER_BOUND('',#4163,.T.);
#2738=FACE_OUTER_BOUND('',#4164,.T.);
#2739=FACE_OUTER_BOUND('',#4165,.T.);
#2740=FACE_OUTER_BOUND('',#4166,.T.);
#2741=FACE_OUTER_BOUND('',#4167,.T.);
#2742=FACE_OUTER_BOUND('',#4168,.T.);
#2743=FACE_OUTER_BOUND('',#4169,.T.);
#2744=FACE_OUTER_BOUND('',#4170,.T.);
#2745=FACE_OUTER_BOUND('',#4171,.T.);
#2746=FACE_OUTER_BOUND('',#4172,.T.);
#2747=FACE_OUTER_BOUND('',#4173,.T.);
#2748=FACE_OUTER_BOUND('',#4174,.T.);
#2749=FACE_OUTER_BOUND('',#4175,.T.);
#2750=FACE_OUTER_BOUND('',#4176,.T.);
#2751=FACE_OUTER_BOUND('',#4177,.T.);
#2752=FACE_OUTER_BOUND('',#4178,.T.);
#2753=FACE_OUTER_BOUND('',#4179,.T.);
#2754=FACE_OUTER_BOUND('',#4180,.T.);
#2755=FACE_OUTER_BOUND('',#4181,.T.);
#2756=FACE_OUTER_BOUND('',#4182,.T.);
#2757=FACE_OUTER_BOUND('',#4183,.T.);
#2758=FACE_OUTER_BOUND('',#4184,.T.);
#2759=FACE_OUTER_BOUND('',#4185,.T.);
#2760=FACE_OUTER_BOUND('',#4186,.T.);
#2761=FACE_OUTER_BOUND('',#4187,.T.);
#2762=FACE_OUTER_BOUND('',#4188,.T.);
#2763=FACE_OUTER_BOUND('',#4189,.T.);
#2764=FACE_OUTER_BOUND('',#4190,.T.);
#2765=FACE_OUTER_BOUND('',#4191,.T.);
#2766=FACE_OUTER_BOUND('',#4192,.T.);
#2767=FACE_OUTER_BOUND('',#4193,.T.);
#2768=FACE_OUTER_BOUND('',#4194,.T.);
#2769=FACE_OUTER_BOUND('',#4195,.T.);
#2770=FACE_OUTER_BOUND('',#4196,.T.);
#2771=FACE_OUTER_BOUND('',#4197,.T.);
#2772=FACE_OUTER_BOUND('',#4198,.T.);
#2773=FACE_OUTER_BOUND('',#4199,.T.);
#2774=FACE_OUTER_BOUND('',#4200,.T.);
#2775=FACE_OUTER_BOUND('',#4201,.T.);
#2776=FACE_OUTER_BOUND('',#4202,.T.);
#2777=FACE_OUTER_BOUND('',#4203,.T.);
#2778=FACE_OUTER_BOUND('',#4204,.T.);
#2779=FACE_OUTER_BOUND('',#4205,.T.);
#2780=FACE_OUTER_BOUND('',#4206,.T.);
#2781=FACE_OUTER_BOUND('',#4207,.T.);
#2782=FACE_OUTER_BOUND('',#4208,.T.);
#2783=FACE_OUTER_BOUND('',#4209,.T.);
#2784=FACE_OUTER_BOUND('',#4210,.T.);
#2785=FACE_OUTER_BOUND('',#4211,.T.);
#2786=FACE_OUTER_BOUND('',#4212,.T.);
#2787=FACE_OUTER_BOUND('',#4213,.T.);
#2788=FACE_OUTER_BOUND('',#4214,.T.);
#2789=FACE_OUTER_BOUND('',#4215,.T.);
#2790=FACE_OUTER_BOUND('',#4216,.T.);
#2791=FACE_OUTER_BOUND('',#4217,.T.);
#2792=FACE_OUTER_BOUND('',#4218,.T.);
#2793=FACE_OUTER_BOUND('',#4219,.T.);
#2794=FACE_OUTER_BOUND('',#4220,.T.);
#2795=FACE_OUTER_BOUND('',#4221,.T.);
#2796=FACE_OUTER_BOUND('',#4222,.T.);
#2797=FACE_OUTER_BOUND('',#4223,.T.);
#2798=FACE_OUTER_BOUND('',#4224,.T.);
#2799=FACE_OUTER_BOUND('',#4225,.T.);
#2800=FACE_OUTER_BOUND('',#4226,.T.);
#2801=FACE_OUTER_BOUND('',#4227,.T.);
#2802=FACE_OUTER_BOUND('',#4228,.T.);
#2803=FACE_OUTER_BOUND('',#4229,.T.);
#2804=FACE_OUTER_BOUND('',#4230,.T.);
#2805=FACE_OUTER_BOUND('',#4231,.T.);
#2806=FACE_OUTER_BOUND('',#4232,.T.);
#2807=FACE_OUTER_BOUND('',#4233,.T.);
#2808=FACE_OUTER_BOUND('',#4234,.T.);
#2809=FACE_OUTER_BOUND('',#4235,.T.);
#2810=FACE_OUTER_BOUND('',#4236,.T.);
#2811=FACE_OUTER_BOUND('',#4237,.T.);
#2812=FACE_OUTER_BOUND('',#4238,.T.);
#2813=FACE_OUTER_BOUND('',#4239,.T.);
#2814=FACE_OUTER_BOUND('',#4240,.T.);
#2815=FACE_OUTER_BOUND('',#4241,.T.);
#2816=FACE_OUTER_BOUND('',#4242,.T.);
#2817=FACE_OUTER_BOUND('',#4243,.T.);
#2818=FACE_OUTER_BOUND('',#4244,.T.);
#2819=FACE_OUTER_BOUND('',#4245,.T.);
#2820=FACE_OUTER_BOUND('',#4246,.T.);
#2821=FACE_OUTER_BOUND('',#4247,.T.);
#2822=FACE_OUTER_BOUND('',#4248,.T.);
#2823=FACE_OUTER_BOUND('',#4249,.T.);
#2824=FACE_OUTER_BOUND('',#4250,.T.);
#2825=FACE_OUTER_BOUND('',#4251,.T.);
#2826=FACE_OUTER_BOUND('',#4252,.T.);
#2827=FACE_OUTER_BOUND('',#4253,.T.);
#2828=FACE_OUTER_BOUND('',#4254,.T.);
#2829=FACE_OUTER_BOUND('',#4255,.T.);
#2830=FACE_OUTER_BOUND('',#4256,.T.);
#2831=FACE_OUTER_BOUND('',#4257,.T.);
#2832=FACE_OUTER_BOUND('',#4258,.T.);
#2833=FACE_OUTER_BOUND('',#4259,.T.);
#2834=FACE_OUTER_BOUND('',#4260,.T.);
#2835=FACE_OUTER_BOUND('',#4261,.T.);
#2836=FACE_OUTER_BOUND('',#4262,.T.);
#2837=FACE_OUTER_BOUND('',#4263,.T.);
#2838=FACE_OUTER_BOUND('',#4264,.T.);
#2839=FACE_OUTER_BOUND('',#4265,.T.);
#2840=FACE_OUTER_BOUND('',#4266,.T.);
#2841=FACE_OUTER_BOUND('',#4267,.T.);
#2842=FACE_OUTER_BOUND('',#4268,.T.);
#2843=FACE_OUTER_BOUND('',#4269,.T.);
#2844=FACE_OUTER_BOUND('',#4270,.T.);
#2845=FACE_OUTER_BOUND('',#4271,.T.);
#2846=FACE_OUTER_BOUND('',#4272,.T.);
#2847=FACE_OUTER_BOUND('',#4273,.T.);
#2848=FACE_OUTER_BOUND('',#4274,.T.);
#2849=FACE_OUTER_BOUND('',#4275,.T.);
#2850=FACE_OUTER_BOUND('',#4276,.T.);
#2851=FACE_OUTER_BOUND('',#4277,.T.);
#2852=FACE_OUTER_BOUND('',#4278,.T.);
#2853=FACE_OUTER_BOUND('',#4279,.T.);
#2854=FACE_OUTER_BOUND('',#4280,.T.);
#2855=FACE_OUTER_BOUND('',#4281,.T.);
#2856=FACE_OUTER_BOUND('',#4282,.T.);
#2857=FACE_OUTER_BOUND('',#4283,.T.);
#2858=FACE_OUTER_BOUND('',#4284,.T.);
#2859=FACE_OUTER_BOUND('',#4285,.T.);
#2860=FACE_OUTER_BOUND('',#4286,.T.);
#2861=FACE_OUTER_BOUND('',#4287,.T.);
#2862=FACE_OUTER_BOUND('',#4288,.T.);
#2863=FACE_OUTER_BOUND('',#4289,.T.);
#2864=FACE_OUTER_BOUND('',#4290,.T.);
#2865=FACE_OUTER_BOUND('',#4291,.T.);
#2866=FACE_OUTER_BOUND('',#4292,.T.);
#2867=FACE_OUTER_BOUND('',#4294,.T.);
#2868=FACE_OUTER_BOUND('',#4296,.T.);
#2869=FACE_OUTER_BOUND('',#4297,.T.);
#2870=FACE_OUTER_BOUND('',#4298,.T.);
#2871=FACE_OUTER_BOUND('',#4299,.T.);
#2872=FACE_OUTER_BOUND('',#4300,.T.);
#2873=FACE_OUTER_BOUND('',#4301,.T.);
#2874=FACE_OUTER_BOUND('',#4302,.T.);
#2875=FACE_OUTER_BOUND('',#4303,.T.);
#2876=FACE_OUTER_BOUND('',#4304,.T.);
#2877=FACE_OUTER_BOUND('',#4305,.T.);
#2878=FACE_OUTER_BOUND('',#4306,.T.);
#2879=FACE_OUTER_BOUND('',#4307,.T.);
#2880=FACE_OUTER_BOUND('',#4308,.T.);
#2881=FACE_OUTER_BOUND('',#4309,.T.);
#2882=FACE_OUTER_BOUND('',#4310,.T.);
#2883=FACE_OUTER_BOUND('',#4311,.T.);
#2884=FACE_OUTER_BOUND('',#4312,.T.);
#2885=FACE_OUTER_BOUND('',#4313,.T.);
#2886=FACE_OUTER_BOUND('',#4314,.T.);
#2887=FACE_OUTER_BOUND('',#4315,.T.);
#2888=FACE_OUTER_BOUND('',#4316,.T.);
#2889=FACE_OUTER_BOUND('',#4317,.T.);
#2890=FACE_OUTER_BOUND('',#4318,.T.);
#2891=FACE_OUTER_BOUND('',#4319,.T.);
#2892=FACE_OUTER_BOUND('',#4320,.T.);
#2893=FACE_OUTER_BOUND('',#4321,.T.);
#2894=FACE_OUTER_BOUND('',#4322,.T.);
#2895=FACE_OUTER_BOUND('',#4323,.T.);
#2896=FACE_OUTER_BOUND('',#4324,.T.);
#2897=FACE_OUTER_BOUND('',#4325,.T.);
#2898=FACE_OUTER_BOUND('',#4326,.T.);
#2899=FACE_OUTER_BOUND('',#4327,.T.);
#4131=EDGE_LOOP('',(#21314,#21315,#21316,#21317));
#4132=EDGE_LOOP('',(#21318,#21319,#21320,#21321));
#4133=EDGE_LOOP('',(#21322,#21323,#21324,#21325));
#4134=EDGE_LOOP('',(#21326,#21327,#21328,#21329));
#4135=EDGE_LOOP('',(#21330,#21331,#21332,#21333));
#4136=EDGE_LOOP('',(#21334,#21335,#21336,#21337));
#4137=EDGE_LOOP('',(#21338,#21339,#21340,#21341));
#4138=EDGE_LOOP('',(#21342,#21343,#21344,#21345));
#4139=EDGE_LOOP('',(#21346,#21347,#21348,#21349));
#4140=EDGE_LOOP('',(#21350,#21351,#21352,#21353));
#4141=EDGE_LOOP('',(#21354,#21355,#21356,#21357));
#4142=EDGE_LOOP('',(#21358,#21359,#21360,#21361));
#4143=EDGE_LOOP('',(#21362,#21363,#21364,#21365));
#4144=EDGE_LOOP('',(#21366,#21367,#21368,#21369));
#4145=EDGE_LOOP('',(#21370,#21371,#21372,#21373));
#4146=EDGE_LOOP('',(#21374,#21375,#21376,#21377));
#4147=EDGE_LOOP('',(#21378,#21379,#21380,#21381));
#4148=EDGE_LOOP('',(#21382,#21383,#21384,#21385));
#4149=EDGE_LOOP('',(#21386,#21387,#21388,#21389));
#4150=EDGE_LOOP('',(#21390,#21391,#21392,#21393));
#4151=EDGE_LOOP('',(#21394,#21395,#21396,#21397));
#4152=EDGE_LOOP('',(#21398,#21399,#21400,#21401));
#4153=EDGE_LOOP('',(#21402,#21403,#21404,#21405));
#4154=EDGE_LOOP('',(#21406,#21407,#21408,#21409));
#4155=EDGE_LOOP('',(#21410,#21411,#21412,#21413));
#4156=EDGE_LOOP('',(#21414,#21415,#21416,#21417));
#4157=EDGE_LOOP('',(#21418,#21419,#21420,#21421));
#4158=EDGE_LOOP('',(#21422,#21423,#21424,#21425));
#4159=EDGE_LOOP('',(#21426,#21427,#21428,#21429));
#4160=EDGE_LOOP('',(#21430,#21431,#21432,#21433));
#4161=EDGE_LOOP('',(#21434,#21435,#21436,#21437));
#4162=EDGE_LOOP('',(#21438,#21439,#21440,#21441));
#4163=EDGE_LOOP('',(#21442,#21443,#21444,#21445));
#4164=EDGE_LOOP('',(#21446,#21447,#21448,#21449));
#4165=EDGE_LOOP('',(#21450,#21451,#21452,#21453));
#4166=EDGE_LOOP('',(#21454,#21455,#21456,#21457));
#4167=EDGE_LOOP('',(#21458,#21459,#21460,#21461));
#4168=EDGE_LOOP('',(#21462,#21463,#21464,#21465));
#4169=EDGE_LOOP('',(#21466,#21467,#21468,#21469));
#4170=EDGE_LOOP('',(#21470,#21471,#21472,#21473));
#4171=EDGE_LOOP('',(#21474,#21475,#21476,#21477));
#4172=EDGE_LOOP('',(#21478,#21479,#21480,#21481));
#4173=EDGE_LOOP('',(#21482,#21483,#21484,#21485));
#4174=EDGE_LOOP('',(#21486,#21487,#21488,#21489));
#4175=EDGE_LOOP('',(#21490,#21491,#21492,#21493));
#4176=EDGE_LOOP('',(#21494,#21495,#21496,#21497));
#4177=EDGE_LOOP('',(#21498,#21499,#21500,#21501));
#4178=EDGE_LOOP('',(#21502,#21503,#21504,#21505));
#4179=EDGE_LOOP('',(#21506,#21507,#21508,#21509));
#4180=EDGE_LOOP('',(#21510,#21511,#21512,#21513));
#4181=EDGE_LOOP('',(#21514,#21515,#21516,#21517));
#4182=EDGE_LOOP('',(#21518,#21519,#21520,#21521));
#4183=EDGE_LOOP('',(#21522,#21523,#21524,#21525));
#4184=EDGE_LOOP('',(#21526,#21527,#21528,#21529));
#4185=EDGE_LOOP('',(#21530,#21531,#21532,#21533));
#4186=EDGE_LOOP('',(#21534,#21535,#21536,#21537));
#4187=EDGE_LOOP('',(#21538,#21539,#21540,#21541));
#4188=EDGE_LOOP('',(#21542,#21543,#21544,#21545));
#4189=EDGE_LOOP('',(#21546,#21547,#21548,#21549));
#4190=EDGE_LOOP('',(#21550,#21551,#21552,#21553));
#4191=EDGE_LOOP('',(#21554,#21555,#21556,#21557));
#4192=EDGE_LOOP('',(#21558,#21559,#21560,#21561));
#4193=EDGE_LOOP('',(#21562,#21563,#21564,#21565));
#4194=EDGE_LOOP('',(#21566,#21567,#21568,#21569));
#4195=EDGE_LOOP('',(#21570,#21571,#21572,#21573));
#4196=EDGE_LOOP('',(#21574,#21575,#21576,#21577));
#4197=EDGE_LOOP('',(#21578,#21579,#21580,#21581));
#4198=EDGE_LOOP('',(#21582,#21583,#21584,#21585));
#4199=EDGE_LOOP('',(#21586,#21587,#21588,#21589));
#4200=EDGE_LOOP('',(#21590,#21591,#21592,#21593));
#4201=EDGE_LOOP('',(#21594,#21595,#21596,#21597));
#4202=EDGE_LOOP('',(#21598,#21599,#21600,#21601));
#4203=EDGE_LOOP('',(#21602,#21603,#21604,#21605));
#4204=EDGE_LOOP('',(#21606,#21607,#21608,#21609));
#4205=EDGE_LOOP('',(#21610,#21611,#21612,#21613));
#4206=EDGE_LOOP('',(#21614,#21615,#21616,#21617));
#4207=EDGE_LOOP('',(#21618,#21619,#21620,#21621));
#4208=EDGE_LOOP('',(#21622,#21623,#21624,#21625));
#4209=EDGE_LOOP('',(#21626,#21627,#21628,#21629));
#4210=EDGE_LOOP('',(#21630,#21631,#21632,#21633));
#4211=EDGE_LOOP('',(#21634,#21635,#21636,#21637));
#4212=EDGE_LOOP('',(#21638,#21639,#21640,#21641));
#4213=EDGE_LOOP('',(#21642,#21643,#21644,#21645));
#4214=EDGE_LOOP('',(#21646,#21647,#21648,#21649));
#4215=EDGE_LOOP('',(#21650,#21651,#21652,#21653));
#4216=EDGE_LOOP('',(#21654,#21655,#21656,#21657));
#4217=EDGE_LOOP('',(#21658,#21659,#21660,#21661));
#4218=EDGE_LOOP('',(#21662,#21663,#21664,#21665));
#4219=EDGE_LOOP('',(#21666,#21667,#21668,#21669));
#4220=EDGE_LOOP('',(#21670,#21671,#21672,#21673));
#4221=EDGE_LOOP('',(#21674,#21675,#21676,#21677));
#4222=EDGE_LOOP('',(#21678,#21679,#21680,#21681));
#4223=EDGE_LOOP('',(#21682,#21683,#21684,#21685));
#4224=EDGE_LOOP('',(#21686,#21687,#21688,#21689));
#4225=EDGE_LOOP('',(#21690,#21691,#21692,#21693));
#4226=EDGE_LOOP('',(#21694,#21695,#21696,#21697));
#4227=EDGE_LOOP('',(#21698,#21699,#21700,#21701));
#4228=EDGE_LOOP('',(#21702,#21703,#21704,#21705));
#4229=EDGE_LOOP('',(#21706,#21707,#21708,#21709));
#4230=EDGE_LOOP('',(#21710,#21711,#21712,#21713));
#4231=EDGE_LOOP('',(#21714,#21715,#21716,#21717));
#4232=EDGE_LOOP('',(#21718,#21719,#21720,#21721));
#4233=EDGE_LOOP('',(#21722,#21723,#21724,#21725));
#4234=EDGE_LOOP('',(#21726,#21727,#21728,#21729));
#4235=EDGE_LOOP('',(#21730,#21731,#21732,#21733));
#4236=EDGE_LOOP('',(#21734,#21735,#21736,#21737));
#4237=EDGE_LOOP('',(#21738,#21739,#21740,#21741));
#4238=EDGE_LOOP('',(#21742,#21743,#21744,#21745));
#4239=EDGE_LOOP('',(#21746,#21747,#21748,#21749));
#4240=EDGE_LOOP('',(#21750,#21751,#21752,#21753));
#4241=EDGE_LOOP('',(#21754,#21755,#21756,#21757));
#4242=EDGE_LOOP('',(#21758,#21759,#21760,#21761));
#4243=EDGE_LOOP('',(#21762,#21763,#21764,#21765));
#4244=EDGE_LOOP('',(#21766,#21767,#21768,#21769));
#4245=EDGE_LOOP('',(#21770,#21771,#21772,#21773));
#4246=EDGE_LOOP('',(#21774,#21775,#21776,#21777));
#4247=EDGE_LOOP('',(#21778,#21779,#21780,#21781));
#4248=EDGE_LOOP('',(#21782,#21783,#21784,#21785));
#4249=EDGE_LOOP('',(#21786,#21787,#21788,#21789));
#4250=EDGE_LOOP('',(#21790,#21791,#21792,#21793));
#4251=EDGE_LOOP('',(#21794,#21795,#21796,#21797));
#4252=EDGE_LOOP('',(#21798,#21799,#21800,#21801));
#4253=EDGE_LOOP('',(#21802,#21803,#21804,#21805));
#4254=EDGE_LOOP('',(#21806,#21807,#21808,#21809));
#4255=EDGE_LOOP('',(#21810,#21811,#21812,#21813));
#4256=EDGE_LOOP('',(#21814,#21815,#21816,#21817));
#4257=EDGE_LOOP('',(#21818,#21819,#21820,#21821));
#4258=EDGE_LOOP('',(#21822,#21823,#21824,#21825));
#4259=EDGE_LOOP('',(#21826,#21827,#21828,#21829));
#4260=EDGE_LOOP('',(#21830,#21831,#21832,#21833));
#4261=EDGE_LOOP('',(#21834,#21835,#21836,#21837));
#4262=EDGE_LOOP('',(#21838,#21839,#21840,#21841));
#4263=EDGE_LOOP('',(#21842,#21843,#21844,#21845));
#4264=EDGE_LOOP('',(#21846,#21847,#21848,#21849));
#4265=EDGE_LOOP('',(#21850,#21851,#21852,#21853));
#4266=EDGE_LOOP('',(#21854,#21855,#21856,#21857));
#4267=EDGE_LOOP('',(#21858,#21859,#21860,#21861));
#4268=EDGE_LOOP('',(#21862,#21863,#21864,#21865));
#4269=EDGE_LOOP('',(#21866,#21867,#21868,#21869));
#4270=EDGE_LOOP('',(#21870,#21871,#21872,#21873));
#4271=EDGE_LOOP('',(#21874,#21875,#21876,#21877));
#4272=EDGE_LOOP('',(#21878,#21879,#21880,#21881));
#4273=EDGE_LOOP('',(#21882,#21883,#21884,#21885));
#4274=EDGE_LOOP('',(#21886,#21887,#21888,#21889));
#4275=EDGE_LOOP('',(#21890,#21891,#21892,#21893));
#4276=EDGE_LOOP('',(#21894,#21895,#21896,#21897));
#4277=EDGE_LOOP('',(#21898,#21899,#21900,#21901));
#4278=EDGE_LOOP('',(#21902,#21903,#21904,#21905));
#4279=EDGE_LOOP('',(#21906,#21907,#21908,#21909));
#4280=EDGE_LOOP('',(#21910,#21911,#21912,#21913));
#4281=EDGE_LOOP('',(#21914,#21915,#21916,#21917));
#4282=EDGE_LOOP('',(#21918,#21919,#21920,#21921));
#4283=EDGE_LOOP('',(#21922,#21923,#21924,#21925));
#4284=EDGE_LOOP('',(#21926,#21927,#21928,#21929));
#4285=EDGE_LOOP('',(#21930,#21931,#21932,#21933));
#4286=EDGE_LOOP('',(#21934,#21935,#21936,#21937));
#4287=EDGE_LOOP('',(#21938,#21939,#21940,#21941));
#4288=EDGE_LOOP('',(#21942,#21943,#21944,#21945));
#4289=EDGE_LOOP('',(#21946,#21947,#21948,#21949));
#4290=EDGE_LOOP('',(#21950,#21951,#21952,#21953));
#4291=EDGE_LOOP('',(#21954,#21955,#21956,#21957));
#4292=EDGE_LOOP('',(#21958,#21959,#21960,#21961,#21962,#21963,#21964,#21965,
#21966,#21967,#21968,#21969,#21970,#21971,#21972,#21973,#21974,#21975,#21976,
#21977,#21978,#21979,#21980,#21981,#21982,#21983,#21984,#21985,#21986,#21987,
#21988,#21989,#21990,#21991,#21992,#21993,#21994,#21995,#21996,#21997,#21998,
#21999,#22000,#22001,#22002,#22003,#22004,#22005,#22006,#22007,#22008,#22009,
#22010,#22011,#22012,#22013,#22014,#22015,#22016,#22017,#22018,#22019,#22020,
#22021,#22022,#22023,#22024,#22025,#22026,#22027,#22028,#22029,#22030,#22031,
#22032,#22033,#22034,#22035,#22036,#22037,#22038,#22039,#22040,#22041,#22042,
#22043,#22044,#22045,#22046,#22047,#22048,#22049,#22050,#22051,#22052,#22053,
#22054,#22055,#22056,#22057,#22058,#22059,#22060,#22061,#22062,#22063,#22064,
#22065,#22066,#22067,#22068,#22069,#22070,#22071,#22072,#22073,#22074,#22075,
#22076,#22077,#22078,#22079,#22080,#22081,#22082,#22083,#22084,#22085,#22086,
#22087,#22088,#22089,#22090,#22091,#22092,#22093,#22094,#22095,#22096,#22097,
#22098,#22099,#22100,#22101,#22102,#22103,#22104,#22105,#22106,#22107,#22108,
#22109,#22110,#22111,#22112,#22113,#22114,#22115,#22116,#22117,#22118,#22119,
#22120,#22121,#22122,#22123,#22124,#22125,#22126,#22127,#22128,#22129,#22130,
#22131,#22132,#22133,#22134,#22135,#22136,#22137,#22138,#22139,#22140,#22141,
#22142,#22143,#22144,#22145,#22146,#22147,#22148,#22149));
#4293=EDGE_LOOP('',(#22150));
#4294=EDGE_LOOP('',(#22151,#22152,#22153,#22154,#22155,#22156,#22157,#22158,
#22159,#22160,#22161,#22162,#22163,#22164,#22165,#22166,#22167,#22168,#22169,
#22170,#22171,#22172,#22173,#22174,#22175,#22176,#22177,#22178,#22179,#22180,
#22181,#22182,#22183,#22184,#22185,#22186,#22187,#22188,#22189,#22190,#22191,
#22192,#22193,#22194,#22195,#22196,#22197,#22198,#22199,#22200,#22201,#22202,
#22203,#22204,#22205,#22206,#22207,#22208,#22209,#22210,#22211,#22212,#22213,
#22214,#22215,#22216,#22217,#22218,#22219,#22220,#22221,#22222,#22223,#22224,
#22225,#22226,#22227,#22228,#22229,#22230,#22231,#22232,#22233,#22234,#22235,
#22236,#22237,#22238,#22239,#22240,#22241,#22242,#22243,#22244,#22245,#22246,
#22247,#22248,#22249,#22250,#22251,#22252,#22253,#22254,#22255,#22256,#22257,
#22258,#22259,#22260,#22261,#22262,#22263,#22264,#22265,#22266,#22267,#22268,
#22269,#22270,#22271,#22272,#22273,#22274,#22275,#22276,#22277,#22278,#22279,
#22280,#22281,#22282,#22283,#22284,#22285,#22286,#22287,#22288,#22289,#22290,
#22291,#22292,#22293,#22294,#22295,#22296,#22297,#22298,#22299,#22300,#22301,
#22302,#22303,#22304,#22305,#22306,#22307,#22308,#22309,#22310,#22311,#22312,
#22313,#22314,#22315,#22316,#22317,#22318,#22319,#22320,#22321,#22322,#22323,
#22324,#22325,#22326,#22327,#22328,#22329,#22330,#22331,#22332,#22333,#22334,
#22335,#22336,#22337,#22338,#22339,#22340,#22341,#22342));
#4295=EDGE_LOOP('',(#22343));
#4296=EDGE_LOOP('',(#22344,#22345,#22346,#22347));
#4297=EDGE_LOOP('',(#22348,#22349,#22350,#22351));
#4298=EDGE_LOOP('',(#22352,#22353,#22354,#22355));
#4299=EDGE_LOOP('',(#22356,#22357,#22358,#22359));
#4300=EDGE_LOOP('',(#22360,#22361,#22362,#22363));
#4301=EDGE_LOOP('',(#22364,#22365,#22366,#22367));
#4302=EDGE_LOOP('',(#22368,#22369,#22370,#22371));
#4303=EDGE_LOOP('',(#22372,#22373,#22374,#22375));
#4304=EDGE_LOOP('',(#22376,#22377,#22378,#22379));
#4305=EDGE_LOOP('',(#22380,#22381,#22382,#22383));
#4306=EDGE_LOOP('',(#22384,#22385,#22386,#22387));
#4307=EDGE_LOOP('',(#22388,#22389,#22390,#22391));
#4308=EDGE_LOOP('',(#22392,#22393,#22394,#22395));
#4309=EDGE_LOOP('',(#22396,#22397,#22398,#22399));
#4310=EDGE_LOOP('',(#22400,#22401,#22402,#22403));
#4311=EDGE_LOOP('',(#22404,#22405,#22406,#22407));
#4312=EDGE_LOOP('',(#22408,#22409,#22410,#22411));
#4313=EDGE_LOOP('',(#22412,#22413,#22414,#22415));
#4314=EDGE_LOOP('',(#22416,#22417,#22418,#22419));
#4315=EDGE_LOOP('',(#22420,#22421,#22422,#22423));
#4316=EDGE_LOOP('',(#22424,#22425,#22426,#22427));
#4317=EDGE_LOOP('',(#22428,#22429,#22430,#22431));
#4318=EDGE_LOOP('',(#22432,#22433,#22434,#22435));
#4319=EDGE_LOOP('',(#22436,#22437,#22438,#22439));
#4320=EDGE_LOOP('',(#22440,#22441,#22442,#22443));
#4321=EDGE_LOOP('',(#22444,#22445,#22446,#22447));
#4322=EDGE_LOOP('',(#22448,#22449,#22450,#22451));
#4323=EDGE_LOOP('',(#22452,#22453,#22454,#22455));
#4324=EDGE_LOOP('',(#22456,#22457,#22458,#22459));
#4325=EDGE_LOOP('',(#22460,#22461,#22462,#22463));
#4326=EDGE_LOOP('',(#22464,#22465,#22466,#22467));
#4327=EDGE_LOOP('',(#22468,#22469,#22470,#22471));
#5111=CIRCLE('',#26661,0.5);
#5112=CIRCLE('',#26662,0.5);
#5113=CIRCLE('',#26665,0.5);
#5114=CIRCLE('',#26666,0.5);
#5115=CIRCLE('',#26668,21.4999999999992);
#5116=CIRCLE('',#26669,21.4999999999992);
#5117=CIRCLE('',#26671,0.5);
#5118=CIRCLE('',#26672,0.5);
#5119=CIRCLE('',#26675,0.5);
#5120=CIRCLE('',#26676,0.5);
#5121=CIRCLE('',#26678,21.4999999999992);
#5122=CIRCLE('',#26679,21.4999999999992);
#5123=CIRCLE('',#26681,0.5);
#5124=CIRCLE('',#26682,0.5);
#5125=CIRCLE('',#26685,0.5);
#5126=CIRCLE('',#26686,0.5);
#5127=CIRCLE('',#26688,21.4999999999992);
#5128=CIRCLE('',#26689,21.4999999999992);
#5129=CIRCLE('',#26691,0.5);
#5130=CIRCLE('',#26692,0.5);
#5131=CIRCLE('',#26695,0.5);
#5132=CIRCLE('',#26696,0.5);
#5133=CIRCLE('',#26698,21.4999999999992);
#5134=CIRCLE('',#26699,21.4999999999992);
#5135=CIRCLE('',#26701,0.5);
#5136=CIRCLE('',#26702,0.5);
#5137=CIRCLE('',#26705,0.5);
#5138=CIRCLE('',#26706,0.5);
#5139=CIRCLE('',#26708,21.4999999999992);
#5140=CIRCLE('',#26709,21.4999999999992);
#5141=CIRCLE('',#26711,0.5);
#5142=CIRCLE('',#26712,0.5);
#5143=CIRCLE('',#26715,0.5);
#5144=CIRCLE('',#26716,0.5);
#5145=CIRCLE('',#26718,21.4999999999992);
#5146=CIRCLE('',#26719,21.4999999999992);
#5147=CIRCLE('',#26721,0.5);
#5148=CIRCLE('',#26722,0.5);
#5149=CIRCLE('',#26725,0.5);
#5150=CIRCLE('',#26726,0.5);
#5151=CIRCLE('',#26728,21.4999999999992);
#5152=CIRCLE('',#26729,21.4999999999992);
#5153=CIRCLE('',#26731,0.5);
#5154=CIRCLE('',#26732,0.5);
#5155=CIRCLE('',#26735,0.5);
#5156=CIRCLE('',#26736,0.5);
#5157=CIRCLE('',#26738,21.4999999999992);
#5158=CIRCLE('',#26739,21.4999999999992);
#5159=CIRCLE('',#26741,0.5);
#5160=CIRCLE('',#26742,0.5);
#5161=CIRCLE('',#26745,0.5);
#5162=CIRCLE('',#26746,0.5);
#5163=CIRCLE('',#26748,21.4999999999992);
#5164=CIRCLE('',#26749,21.4999999999992);
#5165=CIRCLE('',#26751,0.5);
#5166=CIRCLE('',#26752,0.5);
#5167=CIRCLE('',#26755,0.5);
#5168=CIRCLE('',#26756,0.5);
#5169=CIRCLE('',#26758,21.4999999999992);
#5170=CIRCLE('',#26759,21.4999999999992);
#5171=CIRCLE('',#26761,0.5);
#5172=CIRCLE('',#26762,0.5);
#5173=CIRCLE('',#26765,0.5);
#5174=CIRCLE('',#26766,0.5);
#5175=CIRCLE('',#26768,21.4999999999992);
#5176=CIRCLE('',#26769,21.4999999999992);
#5177=CIRCLE('',#26771,0.5);
#5178=CIRCLE('',#26772,0.5);
#5179=CIRCLE('',#26775,0.5);
#5180=CIRCLE('',#26776,0.5);
#5181=CIRCLE('',#26778,21.4999999999992);
#5182=CIRCLE('',#26779,21.4999999999992);
#5183=CIRCLE('',#26781,0.5);
#5184=CIRCLE('',#26782,0.5);
#5185=CIRCLE('',#26785,0.5);
#5186=CIRCLE('',#26786,0.5);
#5187=CIRCLE('',#26788,21.4999999999992);
#5188=CIRCLE('',#26789,21.4999999999992);
#5189=CIRCLE('',#26791,0.5);
#5190=CIRCLE('',#26792,0.5);
#5191=CIRCLE('',#26795,0.5);
#5192=CIRCLE('',#26796,0.5);
#5193=CIRCLE('',#26798,21.4999999999992);
#5194=CIRCLE('',#26799,21.4999999999992);
#5195=CIRCLE('',#26801,0.5);
#5196=CIRCLE('',#26802,0.5);
#5197=CIRCLE('',#26805,0.5);
#5198=CIRCLE('',#26806,0.5);
#5199=CIRCLE('',#26808,21.4999999999992);
#5200=CIRCLE('',#26809,21.4999999999992);
#5201=CIRCLE('',#26811,0.5);
#5202=CIRCLE('',#26812,0.5);
#5203=CIRCLE('',#26815,0.5);
#5204=CIRCLE('',#26816,0.5);
#5205=CIRCLE('',#26818,21.4999999999992);
#5206=CIRCLE('',#26819,21.4999999999992);
#5207=CIRCLE('',#26821,0.5);
#5208=CIRCLE('',#26822,0.5);
#5209=CIRCLE('',#26825,0.5);
#5210=CIRCLE('',#26826,0.5);
#5211=CIRCLE('',#26828,21.4999999999992);
#5212=CIRCLE('',#26829,21.4999999999992);
#5213=CIRCLE('',#26831,0.5);
#5214=CIRCLE('',#26832,0.5);
#5215=CIRCLE('',#26835,0.5);
#5216=CIRCLE('',#26836,0.5);
#5217=CIRCLE('',#26838,21.4999999999992);
#5218=CIRCLE('',#26839,21.4999999999992);
#5219=CIRCLE('',#26841,0.5);
#5220=CIRCLE('',#26842,0.5);
#5221=CIRCLE('',#26845,0.5);
#5222=CIRCLE('',#26846,0.5);
#5223=CIRCLE('',#26848,21.4999999999992);
#5224=CIRCLE('',#26849,21.4999999999992);
#5225=CIRCLE('',#26851,0.5);
#5226=CIRCLE('',#26852,0.5);
#5227=CIRCLE('',#26855,0.5);
#5228=CIRCLE('',#26856,0.5);
#5229=CIRCLE('',#26858,21.4999999999992);
#5230=CIRCLE('',#26859,21.4999999999992);
#5231=CIRCLE('',#26861,0.5);
#5232=CIRCLE('',#26862,0.5);
#5233=CIRCLE('',#26865,0.5);
#5234=CIRCLE('',#26866,0.5);
#5235=CIRCLE('',#26868,21.4999999999992);
#5236=CIRCLE('',#26869,21.4999999999992);
#5237=CIRCLE('',#26871,0.5);
#5238=CIRCLE('',#26872,0.5);
#5239=CIRCLE('',#26875,0.5);
#5240=CIRCLE('',#26876,0.5);
#5241=CIRCLE('',#26878,21.4999999999992);
#5242=CIRCLE('',#26879,21.4999999999992);
#5243=CIRCLE('',#26881,0.5);
#5244=CIRCLE('',#26882,0.5);
#5245=CIRCLE('',#26885,0.5);
#5246=CIRCLE('',#26886,0.5);
#5247=CIRCLE('',#26888,21.4999999999992);
#5248=CIRCLE('',#26889,21.4999999999992);
#5249=CIRCLE('',#26914,26.);
#5250=CIRCLE('',#26915,26.);
#5251=CIRCLE('',#26916,26.);
#5252=CIRCLE('',#26917,26.);
#5253=CIRCLE('',#26918,26.);
#5254=CIRCLE('',#26919,26.);
#5255=CIRCLE('',#26920,26.);
#5256=CIRCLE('',#26921,26.);
#5257=CIRCLE('',#26922,26.);
#5258=CIRCLE('',#26923,26.);
#5259=CIRCLE('',#26924,26.);
#5260=CIRCLE('',#26925,26.);
#5261=CIRCLE('',#26926,26.);
#5262=CIRCLE('',#26927,26.);
#5263=CIRCLE('',#26928,26.);
#5264=CIRCLE('',#26929,26.);
#5265=CIRCLE('',#26930,26.);
#5266=CIRCLE('',#26931,26.);
#5267=CIRCLE('',#26932,26.);
#5268=CIRCLE('',#26933,26.);
#5269=CIRCLE('',#26934,26.);
#5270=CIRCLE('',#26935,26.);
#5271=CIRCLE('',#26936,26.);
#5272=CIRCLE('',#26937,0.5);
#5273=CIRCLE('',#26938,21.4999999999992);
#5274=CIRCLE('',#26939,0.5);
#5275=CIRCLE('',#26940,26.);
#5276=CIRCLE('',#26941,7.);
#5277=CIRCLE('',#26943,26.);
#5278=CIRCLE('',#26944,0.5);
#5279=CIRCLE('',#26945,21.4999999999992);
#5280=CIRCLE('',#26946,0.5);
#5281=CIRCLE('',#26947,26.);
#5282=CIRCLE('',#26948,26.);
#5283=CIRCLE('',#26949,26.);
#5284=CIRCLE('',#26950,26.);
#5285=CIRCLE('',#26951,26.);
#5286=CIRCLE('',#26952,26.);
#5287=CIRCLE('',#26953,26.);
#5288=CIRCLE('',#26954,26.);
#5289=CIRCLE('',#26955,26.);
#5290=CIRCLE('',#26956,26.);
#5291=CIRCLE('',#26957,26.);
#5292=CIRCLE('',#26958,26.);
#5293=CIRCLE('',#26959,26.);
#5294=CIRCLE('',#26960,26.);
#5295=CIRCLE('',#26961,26.);
#5296=CIRCLE('',#26962,26.);
#5297=CIRCLE('',#26963,26.);
#5298=CIRCLE('',#26964,26.);
#5299=CIRCLE('',#26965,26.);
#5300=CIRCLE('',#26966,26.);
#5301=CIRCLE('',#26967,26.);
#5302=CIRCLE('',#26968,26.);
#5303=CIRCLE('',#26969,26.);
#5304=CIRCLE('',#26970,7.);
#7428=LINE('',#215386,#8613);
#7429=LINE('',#215389,#8614);
#7430=LINE('',#215392,#8615);
#7431=LINE('',#215394,#8616);
#7432=LINE('',#215395,#8617);
#7433=LINE('',#215401,#8618);
#7434=LINE('',#215404,#8619);
#7435=LINE('',#215413,#8620);
#7436=LINE('',#215416,#8621);
#7437=LINE('',#215419,#8622);
#7438=LINE('',#215421,#8623);
#7439=LINE('',#215422,#8624);
#7440=LINE('',#215428,#8625);
#7441=LINE('',#215431,#8626);
#7442=LINE('',#215440,#8627);
#7443=LINE('',#215443,#8628);
#7444=LINE('',#215446,#8629);
#7445=LINE('',#215448,#8630);
#7446=LINE('',#215449,#8631);
#7447=LINE('',#215455,#8632);
#7448=LINE('',#215458,#8633);
#7449=LINE('',#215467,#8634);
#7450=LINE('',#215470,#8635);
#7451=LINE('',#215473,#8636);
#7452=LINE('',#215475,#8637);
#7453=LINE('',#215476,#8638);
#7454=LINE('',#215482,#8639);
#7455=LINE('',#215485,#8640);
#7456=LINE('',#215494,#8641);
#7457=LINE('',#215497,#8642);
#7458=LINE('',#215500,#8643);
#7459=LINE('',#215502,#8644);
#7460=LINE('',#215503,#8645);
#7461=LINE('',#215509,#8646);
#7462=LINE('',#215512,#8647);
#7463=LINE('',#215521,#8648);
#7464=LINE('',#215524,#8649);
#7465=LINE('',#215527,#8650);
#7466=LINE('',#215529,#8651);
#7467=LINE('',#215530,#8652);
#7468=LINE('',#215536,#8653);
#7469=LINE('',#215539,#8654);
#7470=LINE('',#215548,#8655);
#7471=LINE('',#215551,#8656);
#7472=LINE('',#215554,#8657);
#7473=LINE('',#215556,#8658);
#7474=LINE('',#215557,#8659);
#7475=LINE('',#215563,#8660);
#7476=LINE('',#215566,#8661);
#7477=LINE('',#215575,#8662);
#7478=LINE('',#215578,#8663);
#7479=LINE('',#215581,#8664);
#7480=LINE('',#215583,#8665);
#7481=LINE('',#215584,#8666);
#7482=LINE('',#215590,#8667);
#7483=LINE('',#215593,#8668);
#7484=LINE('',#215602,#8669);
#7485=LINE('',#215605,#8670);
#7486=LINE('',#215608,#8671);
#7487=LINE('',#215610,#8672);
#7488=LINE('',#215611,#8673);
#7489=LINE('',#215617,#8674);
#7490=LINE('',#215620,#8675);
#7491=LINE('',#215629,#8676);
#7492=LINE('',#215632,#8677);
#7493=LINE('',#215635,#8678);
#7494=LINE('',#215637,#8679);
#7495=LINE('',#215638,#8680);
#7496=LINE('',#215644,#8681);
#7497=LINE('',#215647,#8682);
#7498=LINE('',#215656,#8683);
#7499=LINE('',#215659,#8684);
#7500=LINE('',#215662,#8685);
#7501=LINE('',#215664,#8686);
#7502=LINE('',#215665,#8687);
#7503=LINE('',#215671,#8688);
#7504=LINE('',#215674,#8689);
#7505=LINE('',#215683,#8690);
#7506=LINE('',#215686,#8691);
#7507=LINE('',#215689,#8692);
#7508=LINE('',#215691,#8693);
#7509=LINE('',#215692,#8694);
#7510=LINE('',#215698,#8695);
#7511=LINE('',#215701,#8696);
#7512=LINE('',#215710,#8697);
#7513=LINE('',#215713,#8698);
#7514=LINE('',#215716,#8699);
#7515=LINE('',#215718,#8700);
#7516=LINE('',#215719,#8701);
#7517=LINE('',#215725,#8702);
#7518=LINE('',#215728,#8703);
#7519=LINE('',#215737,#8704);
#7520=LINE('',#215740,#8705);
#7521=LINE('',#215743,#8706);
#7522=LINE('',#215745,#8707);
#7523=LINE('',#215746,#8708);
#7524=LINE('',#215752,#8709);
#7525=LINE('',#215755,#8710);
#7526=LINE('',#215764,#8711);
#7527=LINE('',#215767,#8712);
#7528=LINE('',#215770,#8713);
#7529=LINE('',#215772,#8714);
#7530=LINE('',#215773,#8715);
#7531=LINE('',#215779,#8716);
#7532=LINE('',#215782,#8717);
#7533=LINE('',#215791,#8718);
#7534=LINE('',#215794,#8719);
#7535=LINE('',#215797,#8720);
#7536=LINE('',#215799,#8721);
#7537=LINE('',#215800,#8722);
#7538=LINE('',#215806,#8723);
#7539=LINE('',#215809,#8724);
#7540=LINE('',#215818,#8725);
#7541=LINE('',#215821,#8726);
#7542=LINE('',#215824,#8727);
#7543=LINE('',#215826,#8728);
#7544=LINE('',#215827,#8729);
#7545=LINE('',#215833,#8730);
#7546=LINE('',#215836,#8731);
#7547=LINE('',#215845,#8732);
#7548=LINE('',#215848,#8733);
#7549=LINE('',#215851,#8734);
#7550=LINE('',#215853,#8735);
#7551=LINE('',#215854,#8736);
#7552=LINE('',#215860,#8737);
#7553=LINE('',#215863,#8738);
#7554=LINE('',#215872,#8739);
#7555=LINE('',#215875,#8740);
#7556=LINE('',#215878,#8741);
#7557=LINE('',#215880,#8742);
#7558=LINE('',#215881,#8743);
#7559=LINE('',#215887,#8744);
#7560=LINE('',#215890,#8745);
#7561=LINE('',#215899,#8746);
#7562=LINE('',#215902,#8747);
#7563=LINE('',#215905,#8748);
#7564=LINE('',#215907,#8749);
#7565=LINE('',#215908,#8750);
#7566=LINE('',#215914,#8751);
#7567=LINE('',#215917,#8752);
#7568=LINE('',#215926,#8753);
#7569=LINE('',#215929,#8754);
#7570=LINE('',#215932,#8755);
#7571=LINE('',#215934,#8756);
#7572=LINE('',#215935,#8757);
#7573=LINE('',#215941,#8758);
#7574=LINE('',#215944,#8759);
#7575=LINE('',#215953,#8760);
#7576=LINE('',#215956,#8761);
#7577=LINE('',#215959,#8762);
#7578=LINE('',#215961,#8763);
#7579=LINE('',#215962,#8764);
#7580=LINE('',#215968,#8765);
#7581=LINE('',#215971,#8766);
#7582=LINE('',#215980,#8767);
#7583=LINE('',#215983,#8768);
#7584=LINE('',#215986,#8769);
#7585=LINE('',#215988,#8770);
#7586=LINE('',#215989,#8771);
#7587=LINE('',#215995,#8772);
#7588=LINE('',#215998,#8773);
#7589=LINE('',#216004,#8774);
#7590=LINE('',#216006,#8775);
#7591=LINE('',#216007,#8776);
#7592=LINE('',#216625,#8777);
#7593=LINE('',#217653,#8778);
#7594=LINE('',#217656,#8779);
#7595=LINE('',#217658,#8780);
#7596=LINE('',#217659,#8781);
#7597=LINE('',#218277,#8782);
#7598=LINE('',#219305,#8783);
#7599=LINE('',#219308,#8784);
#7600=LINE('',#219310,#8785);
#7601=LINE('',#219311,#8786);
#7602=LINE('',#219929,#8787);
#7603=LINE('',#220957,#8788);
#7604=LINE('',#220960,#8789);
#7605=LINE('',#220962,#8790);
#7606=LINE('',#220963,#8791);
#7607=LINE('',#221581,#8792);
#7608=LINE('',#222609,#8793);
#7609=LINE('',#222612,#8794);
#7610=LINE('',#222614,#8795);
#7611=LINE('',#222615,#8796);
#7612=LINE('',#223233,#8797);
#7613=LINE('',#224261,#8798);
#7614=LINE('',#224264,#8799);
#7615=LINE('',#224266,#8800);
#7616=LINE('',#224267,#8801);
#7617=LINE('',#224885,#8802);
#7618=LINE('',#225913,#8803);
#7619=LINE('',#225916,#8804);
#7620=LINE('',#225918,#8805);
#7621=LINE('',#225919,#8806);
#7622=LINE('',#226537,#8807);
#7623=LINE('',#227565,#8808);
#7624=LINE('',#227568,#8809);
#7625=LINE('',#227570,#8810);
#7626=LINE('',#227571,#8811);
#7627=LINE('',#228189,#8812);
#7628=LINE('',#229217,#8813);
#7629=LINE('',#229220,#8814);
#7630=LINE('',#229222,#8815);
#7631=LINE('',#229223,#8816);
#7632=LINE('',#229841,#8817);
#7633=LINE('',#230869,#8818);
#7634=LINE('',#230872,#8819);
#7635=LINE('',#230874,#8820);
#7636=LINE('',#230875,#8821);
#7637=LINE('',#231493,#8822);
#7638=LINE('',#232521,#8823);
#7639=LINE('',#232524,#8824);
#7640=LINE('',#232526,#8825);
#7641=LINE('',#232527,#8826);
#7642=LINE('',#233145,#8827);
#7643=LINE('',#234173,#8828);
#7644=LINE('',#234176,#8829);
#7645=LINE('',#234178,#8830);
#7646=LINE('',#234179,#8831);
#7647=LINE('',#234797,#8832);
#7648=LINE('',#235825,#8833);
#7649=LINE('',#235828,#8834);
#7650=LINE('',#235830,#8835);
#7651=LINE('',#235831,#8836);
#7652=LINE('',#236449,#8837);
#7653=LINE('',#237477,#8838);
#7654=LINE('',#237480,#8839);
#7655=LINE('',#237482,#8840);
#7656=LINE('',#237483,#8841);
#7657=LINE('',#238101,#8842);
#7658=LINE('',#239129,#8843);
#7659=LINE('',#239132,#8844);
#7660=LINE('',#239134,#8845);
#7661=LINE('',#239135,#8846);
#7662=LINE('',#239753,#8847);
#7663=LINE('',#240781,#8848);
#7664=LINE('',#240784,#8849);
#7665=LINE('',#240786,#8850);
#7666=LINE('',#240787,#8851);
#7667=LINE('',#241405,#8852);
#7668=LINE('',#242433,#8853);
#7669=LINE('',#242436,#8854);
#7670=LINE('',#242438,#8855);
#7671=LINE('',#242439,#8856);
#7672=LINE('',#243057,#8857);
#7673=LINE('',#244085,#8858);
#7674=LINE('',#244088,#8859);
#7675=LINE('',#244090,#8860);
#7676=LINE('',#244091,#8861);
#7677=LINE('',#244709,#8862);
#7678=LINE('',#245737,#8863);
#7679=LINE('',#245740,#8864);
#7680=LINE('',#245742,#8865);
#7681=LINE('',#245743,#8866);
#7682=LINE('',#246361,#8867);
#7683=LINE('',#247389,#8868);
#7684=LINE('',#247392,#8869);
#7685=LINE('',#247394,#8870);
#7686=LINE('',#247395,#8871);
#7687=LINE('',#248013,#8872);
#7688=LINE('',#249041,#8873);
#7689=LINE('',#249044,#8874);
#7690=LINE('',#249046,#8875);
#7691=LINE('',#249047,#8876);
#7692=LINE('',#249665,#8877);
#7693=LINE('',#250693,#8878);
#7694=LINE('',#250696,#8879);
#7695=LINE('',#250698,#8880);
#7696=LINE('',#250699,#8881);
#7697=LINE('',#251317,#8882);
#7698=LINE('',#252345,#8883);
#7699=LINE('',#252348,#8884);
#7700=LINE('',#252350,#8885);
#7701=LINE('',#252351,#8886);
#7702=LINE('',#252969,#8887);
#7703=LINE('',#253997,#8888);
#7704=LINE('',#254230,#8889);
#7705=LINE('',#254238,#8890);
#7706=LINE('',#254658,#8891);
#7707=LINE('',#254666,#8892);
#7708=LINE('',#254899,#8893);
#7709=LINE('',#254923,#8894);
#7710=LINE('',#254924,#8895);
#7711=LINE('',#254926,#8896);
#7712=LINE('',#254928,#8897);
#7713=LINE('',#254929,#8898);
#7714=LINE('',#254932,#8899);
#7715=LINE('',#255753,#8900);
#7716=LINE('',#255755,#8901);
#8613=VECTOR('',#30637,10.);
#8614=VECTOR('',#30640,10.);
#8615=VECTOR('',#30643,10.);
#8616=VECTOR('',#30644,10.);
#8617=VECTOR('',#30645,10.);
#8618=VECTOR('',#30650,10.);
#8619=VECTOR('',#30653,10.);
#8620=VECTOR('',#30664,10.);
#8621=VECTOR('',#30667,10.);
#8622=VECTOR('',#30670,10.);
#8623=VECTOR('',#30671,10.);
#8624=VECTOR('',#30672,10.);
#8625=VECTOR('',#30677,10.);
#8626=VECTOR('',#30680,10.);
#8627=VECTOR('',#30691,10.);
#8628=VECTOR('',#30694,10.);
#8629=VECTOR('',#30697,10.);
#8630=VECTOR('',#30698,10.);
#8631=VECTOR('',#30699,10.);
#8632=VECTOR('',#30704,10.);
#8633=VECTOR('',#30707,10.);
#8634=VECTOR('',#30718,10.);
#8635=VECTOR('',#30721,10.);
#8636=VECTOR('',#30724,10.);
#8637=VECTOR('',#30725,10.);
#8638=VECTOR('',#30726,10.);
#8639=VECTOR('',#30731,10.);
#8640=VECTOR('',#30734,10.);
#8641=VECTOR('',#30745,10.);
#8642=VECTOR('',#30748,10.);
#8643=VECTOR('',#30751,10.);
#8644=VECTOR('',#30752,10.);
#8645=VECTOR('',#30753,10.);
#8646=VECTOR('',#30758,10.);
#8647=VECTOR('',#30761,10.);
#8648=VECTOR('',#30772,10.);
#8649=VECTOR('',#30775,10.);
#8650=VECTOR('',#30778,10.);
#8651=VECTOR('',#30779,10.);
#8652=VECTOR('',#30780,10.);
#8653=VECTOR('',#30785,10.);
#8654=VECTOR('',#30788,10.);
#8655=VECTOR('',#30799,10.);
#8656=VECTOR('',#30802,10.);
#8657=VECTOR('',#30805,10.);
#8658=VECTOR('',#30806,10.);
#8659=VECTOR('',#30807,10.);
#8660=VECTOR('',#30812,10.);
#8661=VECTOR('',#30815,10.);
#8662=VECTOR('',#30826,10.);
#8663=VECTOR('',#30829,10.);
#8664=VECTOR('',#30832,10.);
#8665=VECTOR('',#30833,10.);
#8666=VECTOR('',#30834,10.);
#8667=VECTOR('',#30839,10.);
#8668=VECTOR('',#30842,10.);
#8669=VECTOR('',#30853,10.);
#8670=VECTOR('',#30856,10.);
#8671=VECTOR('',#30859,10.);
#8672=VECTOR('',#30860,10.);
#8673=VECTOR('',#30861,10.);
#8674=VECTOR('',#30866,10.);
#8675=VECTOR('',#30869,10.);
#8676=VECTOR('',#30880,10.);
#8677=VECTOR('',#30883,10.);
#8678=VECTOR('',#30886,10.);
#8679=VECTOR('',#30887,10.);
#8680=VECTOR('',#30888,10.);
#8681=VECTOR('',#30893,10.);
#8682=VECTOR('',#30896,10.);
#8683=VECTOR('',#30907,10.);
#8684=VECTOR('',#30910,10.);
#8685=VECTOR('',#30913,10.);
#8686=VECTOR('',#30914,10.);
#8687=VECTOR('',#30915,10.);
#8688=VECTOR('',#30920,10.);
#8689=VECTOR('',#30923,10.);
#8690=VECTOR('',#30934,10.);
#8691=VECTOR('',#30937,10.);
#8692=VECTOR('',#30940,10.);
#8693=VECTOR('',#30941,10.);
#8694=VECTOR('',#30942,10.);
#8695=VECTOR('',#30947,10.);
#8696=VECTOR('',#30950,10.);
#8697=VECTOR('',#30961,10.);
#8698=VECTOR('',#30964,10.);
#8699=VECTOR('',#30967,10.);
#8700=VECTOR('',#30968,10.);
#8701=VECTOR('',#30969,10.);
#8702=VECTOR('',#30974,10.);
#8703=VECTOR('',#30977,10.);
#8704=VECTOR('',#30988,10.);
#8705=VECTOR('',#30991,10.);
#8706=VECTOR('',#30994,10.);
#8707=VECTOR('',#30995,10.);
#8708=VECTOR('',#30996,10.);
#8709=VECTOR('',#31001,10.);
#8710=VECTOR('',#31004,10.);
#8711=VECTOR('',#31015,10.);
#8712=VECTOR('',#31018,10.);
#8713=VECTOR('',#31021,10.);
#8714=VECTOR('',#31022,10.);
#8715=VECTOR('',#31023,10.);
#8716=VECTOR('',#31028,10.);
#8717=VECTOR('',#31031,10.);
#8718=VECTOR('',#31042,10.);
#8719=VECTOR('',#31045,10.);
#8720=VECTOR('',#31048,10.);
#8721=VECTOR('',#31049,10.);
#8722=VECTOR('',#31050,10.);
#8723=VECTOR('',#31055,10.);
#8724=VECTOR('',#31058,10.);
#8725=VECTOR('',#31069,10.);
#8726=VECTOR('',#31072,10.);
#8727=VECTOR('',#31075,10.);
#8728=VECTOR('',#31076,10.);
#8729=VECTOR('',#31077,10.);
#8730=VECTOR('',#31082,10.);
#8731=VECTOR('',#31085,10.);
#8732=VECTOR('',#31096,10.);
#8733=VECTOR('',#31099,10.);
#8734=VECTOR('',#31102,10.);
#8735=VECTOR('',#31103,10.);
#8736=VECTOR('',#31104,10.);
#8737=VECTOR('',#31109,10.);
#8738=VECTOR('',#31112,10.);
#8739=VECTOR('',#31123,10.);
#8740=VECTOR('',#31126,10.);
#8741=VECTOR('',#31129,10.);
#8742=VECTOR('',#31130,10.);
#8743=VECTOR('',#31131,10.);
#8744=VECTOR('',#31136,10.);
#8745=VECTOR('',#31139,10.);
#8746=VECTOR('',#31150,10.);
#8747=VECTOR('',#31153,10.);
#8748=VECTOR('',#31156,10.);
#8749=VECTOR('',#31157,10.);
#8750=VECTOR('',#31158,10.);
#8751=VECTOR('',#31163,10.);
#8752=VECTOR('',#31166,10.);
#8753=VECTOR('',#31177,10.);
#8754=VECTOR('',#31180,10.);
#8755=VECTOR('',#31183,10.);
#8756=VECTOR('',#31184,10.);
#8757=VECTOR('',#31185,10.);
#8758=VECTOR('',#31190,10.);
#8759=VECTOR('',#31193,10.);
#8760=VECTOR('',#31204,10.);
#8761=VECTOR('',#31207,10.);
#8762=VECTOR('',#31210,10.);
#8763=VECTOR('',#31211,10.);
#8764=VECTOR('',#31212,10.);
#8765=VECTOR('',#31217,10.);
#8766=VECTOR('',#31220,10.);
#8767=VECTOR('',#31231,10.);
#8768=VECTOR('',#31234,10.);
#8769=VECTOR('',#31237,10.);
#8770=VECTOR('',#31238,10.);
#8771=VECTOR('',#31239,10.);
#8772=VECTOR('',#31244,10.);
#8773=VECTOR('',#31247,10.);
#8774=VECTOR('',#31256,10.);
#8775=VECTOR('',#31257,10.);
#8776=VECTOR('',#31258,10.);
#8777=VECTOR('',#31259,10.);
#8778=VECTOR('',#31260,10.);
#8779=VECTOR('',#31263,10.);
#8780=VECTOR('',#31264,10.);
#8781=VECTOR('',#31265,10.);
#8782=VECTOR('',#31266,10.);
#8783=VECTOR('',#31267,10.);
#8784=VECTOR('',#31270,10.);
#8785=VECTOR('',#31271,10.);
#8786=VECTOR('',#31272,10.);
#8787=VECTOR('',#31273,10.);
#8788=VECTOR('',#31274,10.);
#8789=VECTOR('',#31277,10.);
#8790=VECTOR('',#31278,10.);
#8791=VECTOR('',#31279,10.);
#8792=VECTOR('',#31280,10.);
#8793=VECTOR('',#31281,10.);
#8794=VECTOR('',#31284,10.);
#8795=VECTOR('',#31285,10.);
#8796=VECTOR('',#31286,10.);
#8797=VECTOR('',#31287,10.);
#8798=VECTOR('',#31288,10.);
#8799=VECTOR('',#31291,10.);
#8800=VECTOR('',#31292,10.);
#8801=VECTOR('',#31293,10.);
#8802=VECTOR('',#31294,10.);
#8803=VECTOR('',#31295,10.);
#8804=VECTOR('',#31298,10.);
#8805=VECTOR('',#31299,10.);
#8806=VECTOR('',#31300,10.);
#8807=VECTOR('',#31301,10.);
#8808=VECTOR('',#31302,10.);
#8809=VECTOR('',#31305,10.);
#8810=VECTOR('',#31306,10.);
#8811=VECTOR('',#31307,10.);
#8812=VECTOR('',#31308,10.);
#8813=VECTOR('',#31309,10.);
#8814=VECTOR('',#31312,10.);
#8815=VECTOR('',#31313,10.);
#8816=VECTOR('',#31314,10.);
#8817=VECTOR('',#31315,10.);
#8818=VECTOR('',#31316,10.);
#8819=VECTOR('',#31319,10.);
#8820=VECTOR('',#31320,10.);
#8821=VECTOR('',#31321,10.);
#8822=VECTOR('',#31322,10.);
#8823=VECTOR('',#31323,10.);
#8824=VECTOR('',#31326,10.);
#8825=VECTOR('',#31327,10.);
#8826=VECTOR('',#31328,10.);
#8827=VECTOR('',#31329,10.);
#8828=VECTOR('',#31330,10.);
#8829=VECTOR('',#31333,10.);
#8830=VECTOR('',#31334,10.);
#8831=VECTOR('',#31335,10.);
#8832=VECTOR('',#31336,10.);
#8833=VECTOR('',#31337,10.);
#8834=VECTOR('',#31340,10.);
#8835=VECTOR('',#31341,10.);
#8836=VECTOR('',#31342,10.);
#8837=VECTOR('',#31343,10.);
#8838=VECTOR('',#31344,10.);
#8839=VECTOR('',#31347,10.);
#8840=VECTOR('',#31348,10.);
#8841=VECTOR('',#31349,10.);
#8842=VECTOR('',#31350,10.);
#8843=VECTOR('',#31351,10.);
#8844=VECTOR('',#31354,10.);
#8845=VECTOR('',#31355,10.);
#8846=VECTOR('',#31356,10.);
#8847=VECTOR('',#31357,10.);
#8848=VECTOR('',#31358,10.);
#8849=VECTOR('',#31361,10.);
#8850=VECTOR('',#31362,10.);
#8851=VECTOR('',#31363,10.);
#8852=VECTOR('',#31364,10.);
#8853=VECTOR('',#31365,10.);
#8854=VECTOR('',#31368,10.);
#8855=VECTOR('',#31369,10.);
#8856=VECTOR('',#31370,10.);
#8857=VECTOR('',#31371,10.);
#8858=VECTOR('',#31372,10.);
#8859=VECTOR('',#31375,10.);
#8860=VECTOR('',#31376,10.);
#8861=VECTOR('',#31377,10.);
#8862=VECTOR('',#31378,10.);
#8863=VECTOR('',#31379,10.);
#8864=VECTOR('',#31382,10.);
#8865=VECTOR('',#31383,10.);
#8866=VECTOR('',#31384,10.);
#8867=VECTOR('',#31385,10.);
#8868=VECTOR('',#31386,10.);
#8869=VECTOR('',#31389,10.);
#8870=VECTOR('',#31390,10.);
#8871=VECTOR('',#31391,10.);
#8872=VECTOR('',#31392,10.);
#8873=VECTOR('',#31393,10.);
#8874=VECTOR('',#31396,10.);
#8875=VECTOR('',#31397,10.);
#8876=VECTOR('',#31398,10.);
#8877=VECTOR('',#31399,10.);
#8878=VECTOR('',#31400,10.);
#8879=VECTOR('',#31403,10.);
#8880=VECTOR('',#31404,10.);
#8881=VECTOR('',#31405,10.);
#8882=VECTOR('',#31406,10.);
#8883=VECTOR('',#31407,10.);
#8884=VECTOR('',#31410,10.);
#8885=VECTOR('',#31411,10.);
#8886=VECTOR('',#31412,10.);
#8887=VECTOR('',#31413,10.);
#8888=VECTOR('',#31414,10.);
#8889=VECTOR('',#31463,10.);
#8890=VECTOR('',#31470,10.);
#8891=VECTOR('',#31479,10.);
#8892=VECTOR('',#31486,10.);
#8893=VECTOR('',#31537,10.);
#8894=VECTOR('',#31584,10.);
#8895=VECTOR('',#31585,10.);
#8896=VECTOR('',#31588,10.);
#8897=VECTOR('',#31591,10.);
#8898=VECTOR('',#31592,10.);
#8899=VECTOR('',#31597,10.);
#8900=VECTOR('',#31598,10.);
#8901=VECTOR('',#31601,7.);
#11009=VERTEX_POINT('',#215382);
#11010=VERTEX_POINT('',#215383);
#11011=VERTEX_POINT('',#215385);
#11012=VERTEX_POINT('',#215387);
#11013=VERTEX_POINT('',#215391);
#11014=VERTEX_POINT('',#215393);
#11015=VERTEX_POINT('',#215397);
#11016=VERTEX_POINT('',#215398);
#11017=VERTEX_POINT('',#215400);
#11018=VERTEX_POINT('',#215402);
#11019=VERTEX_POINT('',#215409);
#11020=VERTEX_POINT('',#215410);
#11021=VERTEX_POINT('',#215412);
#11022=VERTEX_POINT('',#215414);
#11023=VERTEX_POINT('',#215418);
#11024=VERTEX_POINT('',#215420);
#11025=VERTEX_POINT('',#215424);
#11026=VERTEX_POINT('',#215425);
#11027=VERTEX_POINT('',#215427);
#11028=VERTEX_POINT('',#215429);
#11029=VERTEX_POINT('',#215436);
#11030=VERTEX_POINT('',#215437);
#11031=VERTEX_POINT('',#215439);
#11032=VERTEX_POINT('',#215441);
#11033=VERTEX_POINT('',#215445);
#11034=VERTEX_POINT('',#215447);
#11035=VERTEX_POINT('',#215451);
#11036=VERTEX_POINT('',#215452);
#11037=VERTEX_POINT('',#215454);
#11038=VERTEX_POINT('',#215456);
#11039=VERTEX_POINT('',#215463);
#11040=VERTEX_POINT('',#215464);
#11041=VERTEX_POINT('',#215466);
#11042=VERTEX_POINT('',#215468);
#11043=VERTEX_POINT('',#215472);
#11044=VERTEX_POINT('',#215474);
#11045=VERTEX_POINT('',#215478);
#11046=VERTEX_POINT('',#215479);
#11047=VERTEX_POINT('',#215481);
#11048=VERTEX_POINT('',#215483);
#11049=VERTEX_POINT('',#215490);
#11050=VERTEX_POINT('',#215491);
#11051=VERTEX_POINT('',#215493);
#11052=VERTEX_POINT('',#215495);
#11053=VERTEX_POINT('',#215499);
#11054=VERTEX_POINT('',#215501);
#11055=VERTEX_POINT('',#215505);
#11056=VERTEX_POINT('',#215506);
#11057=VERTEX_POINT('',#215508);
#11058=VERTEX_POINT('',#215510);
#11059=VERTEX_POINT('',#215517);
#11060=VERTEX_POINT('',#215518);
#11061=VERTEX_POINT('',#215520);
#11062=VERTEX_POINT('',#215522);
#11063=VERTEX_POINT('',#215526);
#11064=VERTEX_POINT('',#215528);
#11065=VERTEX_POINT('',#215532);
#11066=VERTEX_POINT('',#215533);
#11067=VERTEX_POINT('',#215535);
#11068=VERTEX_POINT('',#215537);
#11069=VERTEX_POINT('',#215544);
#11070=VERTEX_POINT('',#215545);
#11071=VERTEX_POINT('',#215547);
#11072=VERTEX_POINT('',#215549);
#11073=VERTEX_POINT('',#215553);
#11074=VERTEX_POINT('',#215555);
#11075=VERTEX_POINT('',#215559);
#11076=VERTEX_POINT('',#215560);
#11077=VERTEX_POINT('',#215562);
#11078=VERTEX_POINT('',#215564);
#11079=VERTEX_POINT('',#215571);
#11080=VERTEX_POINT('',#215572);
#11081=VERTEX_POINT('',#215574);
#11082=VERTEX_POINT('',#215576);
#11083=VERTEX_POINT('',#215580);
#11084=VERTEX_POINT('',#215582);
#11085=VERTEX_POINT('',#215586);
#11086=VERTEX_POINT('',#215587);
#11087=VERTEX_POINT('',#215589);
#11088=VERTEX_POINT('',#215591);
#11089=VERTEX_POINT('',#215598);
#11090=VERTEX_POINT('',#215599);
#11091=VERTEX_POINT('',#215601);
#11092=VERTEX_POINT('',#215603);
#11093=VERTEX_POINT('',#215607);
#11094=VERTEX_POINT('',#215609);
#11095=VERTEX_POINT('',#215613);
#11096=VERTEX_POINT('',#215614);
#11097=VERTEX_POINT('',#215616);
#11098=VERTEX_POINT('',#215618);
#11099=VERTEX_POINT('',#215625);
#11100=VERTEX_POINT('',#215626);
#11101=VERTEX_POINT('',#215628);
#11102=VERTEX_POINT('',#215630);
#11103=VERTEX_POINT('',#215634);
#11104=VERTEX_POINT('',#215636);
#11105=VERTEX_POINT('',#215640);
#11106=VERTEX_POINT('',#215641);
#11107=VERTEX_POINT('',#215643);
#11108=VERTEX_POINT('',#215645);
#11109=VERTEX_POINT('',#215652);
#11110=VERTEX_POINT('',#215653);
#11111=VERTEX_POINT('',#215655);
#11112=VERTEX_POINT('',#215657);
#11113=VERTEX_POINT('',#215661);
#11114=VERTEX_POINT('',#215663);
#11115=VERTEX_POINT('',#215667);
#11116=VERTEX_POINT('',#215668);
#11117=VERTEX_POINT('',#215670);
#11118=VERTEX_POINT('',#215672);
#11119=VERTEX_POINT('',#215679);
#11120=VERTEX_POINT('',#215680);
#11121=VERTEX_POINT('',#215682);
#11122=VERTEX_POINT('',#215684);
#11123=VERTEX_POINT('',#215688);
#11124=VERTEX_POINT('',#215690);
#11125=VERTEX_POINT('',#215694);
#11126=VERTEX_POINT('',#215695);
#11127=VERTEX_POINT('',#215697);
#11128=VERTEX_POINT('',#215699);
#11129=VERTEX_POINT('',#215706);
#11130=VERTEX_POINT('',#215707);
#11131=VERTEX_POINT('',#215709);
#11132=VERTEX_POINT('',#215711);
#11133=VERTEX_POINT('',#215715);
#11134=VERTEX_POINT('',#215717);
#11135=VERTEX_POINT('',#215721);
#11136=VERTEX_POINT('',#215722);
#11137=VERTEX_POINT('',#215724);
#11138=VERTEX_POINT('',#215726);
#11139=VERTEX_POINT('',#215733);
#11140=VERTEX_POINT('',#215734);
#11141=VERTEX_POINT('',#215736);
#11142=VERTEX_POINT('',#215738);
#11143=VERTEX_POINT('',#215742);
#11144=VERTEX_POINT('',#215744);
#11145=VERTEX_POINT('',#215748);
#11146=VERTEX_POINT('',#215749);
#11147=VERTEX_POINT('',#215751);
#11148=VERTEX_POINT('',#215753);
#11149=VERTEX_POINT('',#215760);
#11150=VERTEX_POINT('',#215761);
#11151=VERTEX_POINT('',#215763);
#11152=VERTEX_POINT('',#215765);
#11153=VERTEX_POINT('',#215769);
#11154=VERTEX_POINT('',#215771);
#11155=VERTEX_POINT('',#215775);
#11156=VERTEX_POINT('',#215776);
#11157=VERTEX_POINT('',#215778);
#11158=VERTEX_POINT('',#215780);
#11159=VERTEX_POINT('',#215787);
#11160=VERTEX_POINT('',#215788);
#11161=VERTEX_POINT('',#215790);
#11162=VERTEX_POINT('',#215792);
#11163=VERTEX_POINT('',#215796);
#11164=VERTEX_POINT('',#215798);
#11165=VERTEX_POINT('',#215802);
#11166=VERTEX_POINT('',#215803);
#11167=VERTEX_POINT('',#215805);
#11168=VERTEX_POINT('',#215807);
#11169=VERTEX_POINT('',#215814);
#11170=VERTEX_POINT('',#215815);
#11171=VERTEX_POINT('',#215817);
#11172=VERTEX_POINT('',#215819);
#11173=VERTEX_POINT('',#215823);
#11174=VERTEX_POINT('',#215825);
#11175=VERTEX_POINT('',#215829);
#11176=VERTEX_POINT('',#215830);
#11177=VERTEX_POINT('',#215832);
#11178=VERTEX_POINT('',#215834);
#11179=VERTEX_POINT('',#215841);
#11180=VERTEX_POINT('',#215842);
#11181=VERTEX_POINT('',#215844);
#11182=VERTEX_POINT('',#215846);
#11183=VERTEX_POINT('',#215850);
#11184=VERTEX_POINT('',#215852);
#11185=VERTEX_POINT('',#215856);
#11186=VERTEX_POINT('',#215857);
#11187=VERTEX_POINT('',#215859);
#11188=VERTEX_POINT('',#215861);
#11189=VERTEX_POINT('',#215868);
#11190=VERTEX_POINT('',#215869);
#11191=VERTEX_POINT('',#215871);
#11192=VERTEX_POINT('',#215873);
#11193=VERTEX_POINT('',#215877);
#11194=VERTEX_POINT('',#215879);
#11195=VERTEX_POINT('',#215883);
#11196=VERTEX_POINT('',#215884);
#11197=VERTEX_POINT('',#215886);
#11198=VERTEX_POINT('',#215888);
#11199=VERTEX_POINT('',#215895);
#11200=VERTEX_POINT('',#215896);
#11201=VERTEX_POINT('',#215898);
#11202=VERTEX_POINT('',#215900);
#11203=VERTEX_POINT('',#215904);
#11204=VERTEX_POINT('',#215906);
#11205=VERTEX_POINT('',#215910);
#11206=VERTEX_POINT('',#215911);
#11207=VERTEX_POINT('',#215913);
#11208=VERTEX_POINT('',#215915);
#11209=VERTEX_POINT('',#215922);
#11210=VERTEX_POINT('',#215923);
#11211=VERTEX_POINT('',#215925);
#11212=VERTEX_POINT('',#215927);
#11213=VERTEX_POINT('',#215931);
#11214=VERTEX_POINT('',#215933);
#11215=VERTEX_POINT('',#215937);
#11216=VERTEX_POINT('',#215938);
#11217=VERTEX_POINT('',#215940);
#11218=VERTEX_POINT('',#215942);
#11219=VERTEX_POINT('',#215949);
#11220=VERTEX_POINT('',#215950);
#11221=VERTEX_POINT('',#215952);
#11222=VERTEX_POINT('',#215954);
#11223=VERTEX_POINT('',#215958);
#11224=VERTEX_POINT('',#215960);
#11225=VERTEX_POINT('',#215964);
#11226=VERTEX_POINT('',#215965);
#11227=VERTEX_POINT('',#215967);
#11228=VERTEX_POINT('',#215969);
#11229=VERTEX_POINT('',#215976);
#11230=VERTEX_POINT('',#215977);
#11231=VERTEX_POINT('',#215979);
#11232=VERTEX_POINT('',#215981);
#11233=VERTEX_POINT('',#215985);
#11234=VERTEX_POINT('',#215987);
#11235=VERTEX_POINT('',#215991);
#11236=VERTEX_POINT('',#215992);
#11237=VERTEX_POINT('',#215994);
#11238=VERTEX_POINT('',#215996);
#11239=VERTEX_POINT('',#216003);
#11240=VERTEX_POINT('',#216005);
#11241=VERTEX_POINT('',#216418);
#11242=VERTEX_POINT('',#216624);
#11243=VERTEX_POINT('',#217241);
#11244=VERTEX_POINT('',#217447);
#11245=VERTEX_POINT('',#217655);
#11246=VERTEX_POINT('',#217657);
#11247=VERTEX_POINT('',#218070);
#11248=VERTEX_POINT('',#218276);
#11249=VERTEX_POINT('',#218893);
#11250=VERTEX_POINT('',#219099);
#11251=VERTEX_POINT('',#219307);
#11252=VERTEX_POINT('',#219309);
#11253=VERTEX_POINT('',#219722);
#11254=VERTEX_POINT('',#219928);
#11255=VERTEX_POINT('',#220545);
#11256=VERTEX_POINT('',#220751);
#11257=VERTEX_POINT('',#220959);
#11258=VERTEX_POINT('',#220961);
#11259=VERTEX_POINT('',#221374);
#11260=VERTEX_POINT('',#221580);
#11261=VERTEX_POINT('',#222197);
#11262=VERTEX_POINT('',#222403);
#11263=VERTEX_POINT('',#222611);
#11264=VERTEX_POINT('',#222613);
#11265=VERTEX_POINT('',#223026);
#11266=VERTEX_POINT('',#223232);
#11267=VERTEX_POINT('',#223849);
#11268=VERTEX_POINT('',#224055);
#11269=VERTEX_POINT('',#224263);
#11270=VERTEX_POINT('',#224265);
#11271=VERTEX_POINT('',#224678);
#11272=VERTEX_POINT('',#224884);
#11273=VERTEX_POINT('',#225501);
#11274=VERTEX_POINT('',#225707);
#11275=VERTEX_POINT('',#225915);
#11276=VERTEX_POINT('',#225917);
#11277=VERTEX_POINT('',#226330);
#11278=VERTEX_POINT('',#226536);
#11279=VERTEX_POINT('',#227153);
#11280=VERTEX_POINT('',#227359);
#11281=VERTEX_POINT('',#227567);
#11282=VERTEX_POINT('',#227569);
#11283=VERTEX_POINT('',#227982);
#11284=VERTEX_POINT('',#228188);
#11285=VERTEX_POINT('',#228805);
#11286=VERTEX_POINT('',#229011);
#11287=VERTEX_POINT('',#229219);
#11288=VERTEX_POINT('',#229221);
#11289=VERTEX_POINT('',#229634);
#11290=VERTEX_POINT('',#229840);
#11291=VERTEX_POINT('',#230457);
#11292=VERTEX_POINT('',#230663);
#11293=VERTEX_POINT('',#230871);
#11294=VERTEX_POINT('',#230873);
#11295=VERTEX_POINT('',#231286);
#11296=VERTEX_POINT('',#231492);
#11297=VERTEX_POINT('',#232109);
#11298=VERTEX_POINT('',#232315);
#11299=VERTEX_POINT('',#232523);
#11300=VERTEX_POINT('',#232525);
#11301=VERTEX_POINT('',#232938);
#11302=VERTEX_POINT('',#233144);
#11303=VERTEX_POINT('',#233761);
#11304=VERTEX_POINT('',#233967);
#11305=VERTEX_POINT('',#234175);
#11306=VERTEX_POINT('',#234177);
#11307=VERTEX_POINT('',#234590);
#11308=VERTEX_POINT('',#234796);
#11309=VERTEX_POINT('',#235413);
#11310=VERTEX_POINT('',#235619);
#11311=VERTEX_POINT('',#235827);
#11312=VERTEX_POINT('',#235829);
#11313=VERTEX_POINT('',#236242);
#11314=VERTEX_POINT('',#236448);
#11315=VERTEX_POINT('',#237065);
#11316=VERTEX_POINT('',#237271);
#11317=VERTEX_POINT('',#237479);
#11318=VERTEX_POINT('',#237481);
#11319=VERTEX_POINT('',#237894);
#11320=VERTEX_POINT('',#238100);
#11321=VERTEX_POINT('',#238717);
#11322=VERTEX_POINT('',#238923);
#11323=VERTEX_POINT('',#239131);
#11324=VERTEX_POINT('',#239133);
#11325=VERTEX_POINT('',#239546);
#11326=VERTEX_POINT('',#239752);
#11327=VERTEX_POINT('',#240369);
#11328=VERTEX_POINT('',#240575);
#11329=VERTEX_POINT('',#240783);
#11330=VERTEX_POINT('',#240785);
#11331=VERTEX_POINT('',#241198);
#11332=VERTEX_POINT('',#241404);
#11333=VERTEX_POINT('',#242021);
#11334=VERTEX_POINT('',#242227);
#11335=VERTEX_POINT('',#242435);
#11336=VERTEX_POINT('',#242437);
#11337=VERTEX_POINT('',#242850);
#11338=VERTEX_POINT('',#243056);
#11339=VERTEX_POINT('',#243673);
#11340=VERTEX_POINT('',#243879);
#11341=VERTEX_POINT('',#244087);
#11342=VERTEX_POINT('',#244089);
#11343=VERTEX_POINT('',#244502);
#11344=VERTEX_POINT('',#244708);
#11345=VERTEX_POINT('',#245325);
#11346=VERTEX_POINT('',#245531);
#11347=VERTEX_POINT('',#245739);
#11348=VERTEX_POINT('',#245741);
#11349=VERTEX_POINT('',#246154);
#11350=VERTEX_POINT('',#246360);
#11351=VERTEX_POINT('',#246977);
#11352=VERTEX_POINT('',#247183);
#11353=VERTEX_POINT('',#247391);
#11354=VERTEX_POINT('',#247393);
#11355=VERTEX_POINT('',#247806);
#11356=VERTEX_POINT('',#248012);
#11357=VERTEX_POINT('',#248629);
#11358=VERTEX_POINT('',#248835);
#11359=VERTEX_POINT('',#249043);
#11360=VERTEX_POINT('',#249045);
#11361=VERTEX_POINT('',#249458);
#11362=VERTEX_POINT('',#249664);
#11363=VERTEX_POINT('',#250281);
#11364=VERTEX_POINT('',#250487);
#11365=VERTEX_POINT('',#250695);
#11366=VERTEX_POINT('',#250697);
#11367=VERTEX_POINT('',#251110);
#11368=VERTEX_POINT('',#251316);
#11369=VERTEX_POINT('',#251933);
#11370=VERTEX_POINT('',#252139);
#11371=VERTEX_POINT('',#252347);
#11372=VERTEX_POINT('',#252349);
#11373=VERTEX_POINT('',#252762);
#11374=VERTEX_POINT('',#252968);
#11375=VERTEX_POINT('',#253585);
#11376=VERTEX_POINT('',#253791);
#11377=VERTEX_POINT('',#254021);
#11378=VERTEX_POINT('',#254023);
#11379=VERTEX_POINT('',#254229);
#11380=VERTEX_POINT('',#254231);
#11381=VERTEX_POINT('',#254233);
#11382=VERTEX_POINT('',#254235);
#11383=VERTEX_POINT('',#254237);
#11384=VERTEX_POINT('',#254239);
#11385=VERTEX_POINT('',#254446);
#11386=VERTEX_POINT('',#254449);
#11387=VERTEX_POINT('',#254451);
#11388=VERTEX_POINT('',#254657);
#11389=VERTEX_POINT('',#254659);
#11390=VERTEX_POINT('',#254661);
#11391=VERTEX_POINT('',#254663);
#11392=VERTEX_POINT('',#254665);
#11393=VERTEX_POINT('',#254667);
#11394=VERTEX_POINT('',#254896);
#14542=EDGE_CURVE('',#11009,#11010,#5111,.T.);
#14543=EDGE_CURVE('',#11010,#11011,#7428,.T.);
#14544=EDGE_CURVE('',#11011,#11012,#5112,.T.);
#14545=EDGE_CURVE('',#11012,#11009,#7429,.T.);
#14546=EDGE_CURVE('',#11013,#11010,#7430,.T.);
#14547=EDGE_CURVE('',#11013,#11014,#7431,.T.);
#14548=EDGE_CURVE('',#11011,#11014,#7432,.T.);
#14549=EDGE_CURVE('',#11015,#11016,#5113,.T.);
#14550=EDGE_CURVE('',#11016,#11017,#7433,.T.);
#14551=EDGE_CURVE('',#11017,#11018,#5114,.T.);
#14552=EDGE_CURVE('',#11018,#11015,#7434,.T.);
#14553=EDGE_CURVE('',#11017,#11012,#5115,.T.);
#14554=EDGE_CURVE('',#11009,#11016,#5116,.T.);
#14555=EDGE_CURVE('',#11019,#11020,#5117,.T.);
#14556=EDGE_CURVE('',#11020,#11021,#7435,.T.);
#14557=EDGE_CURVE('',#11021,#11022,#5118,.T.);
#14558=EDGE_CURVE('',#11022,#11019,#7436,.T.);
#14559=EDGE_CURVE('',#11023,#11020,#7437,.T.);
#14560=EDGE_CURVE('',#11023,#11024,#7438,.T.);
#14561=EDGE_CURVE('',#11021,#11024,#7439,.T.);
#14562=EDGE_CURVE('',#11025,#11026,#5119,.T.);
#14563=EDGE_CURVE('',#11026,#11027,#7440,.T.);
#14564=EDGE_CURVE('',#11027,#11028,#5120,.T.);
#14565=EDGE_CURVE('',#11028,#11025,#7441,.T.);
#14566=EDGE_CURVE('',#11027,#11022,#5121,.T.);
#14567=EDGE_CURVE('',#11019,#11026,#5122,.T.);
#14568=EDGE_CURVE('',#11029,#11030,#5123,.T.);
#14569=EDGE_CURVE('',#11030,#11031,#7442,.T.);
#14570=EDGE_CURVE('',#11031,#11032,#5124,.T.);
#14571=EDGE_CURVE('',#11032,#11029,#7443,.T.);
#14572=EDGE_CURVE('',#11033,#11030,#7444,.T.);
#14573=EDGE_CURVE('',#11033,#11034,#7445,.T.);
#14574=EDGE_CURVE('',#11031,#11034,#7446,.T.);
#14575=EDGE_CURVE('',#11035,#11036,#5125,.T.);
#14576=EDGE_CURVE('',#11036,#11037,#7447,.T.);
#14577=EDGE_CURVE('',#11037,#11038,#5126,.T.);
#14578=EDGE_CURVE('',#11038,#11035,#7448,.T.);
#14579=EDGE_CURVE('',#11037,#11032,#5127,.T.);
#14580=EDGE_CURVE('',#11029,#11036,#5128,.T.);
#14581=EDGE_CURVE('',#11039,#11040,#5129,.T.);
#14582=EDGE_CURVE('',#11040,#11041,#7449,.T.);
#14583=EDGE_CURVE('',#11041,#11042,#5130,.T.);
#14584=EDGE_CURVE('',#11042,#11039,#7450,.T.);
#14585=EDGE_CURVE('',#11043,#11040,#7451,.T.);
#14586=EDGE_CURVE('',#11043,#11044,#7452,.T.);
#14587=EDGE_CURVE('',#11041,#11044,#7453,.T.);
#14588=EDGE_CURVE('',#11045,#11046,#5131,.T.);
#14589=EDGE_CURVE('',#11046,#11047,#7454,.T.);
#14590=EDGE_CURVE('',#11047,#11048,#5132,.T.);
#14591=EDGE_CURVE('',#11048,#11045,#7455,.T.);
#14592=EDGE_CURVE('',#11047,#11042,#5133,.T.);
#14593=EDGE_CURVE('',#11039,#11046,#5134,.T.);
#14594=EDGE_CURVE('',#11049,#11050,#5135,.T.);
#14595=EDGE_CURVE('',#11050,#11051,#7456,.T.);
#14596=EDGE_CURVE('',#11051,#11052,#5136,.T.);
#14597=EDGE_CURVE('',#11052,#11049,#7457,.T.);
#14598=EDGE_CURVE('',#11053,#11050,#7458,.T.);
#14599=EDGE_CURVE('',#11053,#11054,#7459,.T.);
#14600=EDGE_CURVE('',#11051,#11054,#7460,.T.);
#14601=EDGE_CURVE('',#11055,#11056,#5137,.T.);
#14602=EDGE_CURVE('',#11056,#11057,#7461,.T.);
#14603=EDGE_CURVE('',#11057,#11058,#5138,.T.);
#14604=EDGE_CURVE('',#11058,#11055,#7462,.T.);
#14605=EDGE_CURVE('',#11057,#11052,#5139,.T.);
#14606=EDGE_CURVE('',#11049,#11056,#5140,.T.);
#14607=EDGE_CURVE('',#11059,#11060,#5141,.T.);
#14608=EDGE_CURVE('',#11060,#11061,#7463,.T.);
#14609=EDGE_CURVE('',#11061,#11062,#5142,.T.);
#14610=EDGE_CURVE('',#11062,#11059,#7464,.T.);
#14611=EDGE_CURVE('',#11063,#11060,#7465,.T.);
#14612=EDGE_CURVE('',#11063,#11064,#7466,.T.);
#14613=EDGE_CURVE('',#11061,#11064,#7467,.T.);
#14614=EDGE_CURVE('',#11065,#11066,#5143,.T.);
#14615=EDGE_CURVE('',#11066,#11067,#7468,.T.);
#14616=EDGE_CURVE('',#11067,#11068,#5144,.T.);
#14617=EDGE_CURVE('',#11068,#11065,#7469,.T.);
#14618=EDGE_CURVE('',#11067,#11062,#5145,.T.);
#14619=EDGE_CURVE('',#11059,#11066,#5146,.T.);
#14620=EDGE_CURVE('',#11069,#11070,#5147,.T.);
#14621=EDGE_CURVE('',#11070,#11071,#7470,.T.);
#14622=EDGE_CURVE('',#11071,#11072,#5148,.T.);
#14623=EDGE_CURVE('',#11072,#11069,#7471,.T.);
#14624=EDGE_CURVE('',#11073,#11070,#7472,.T.);
#14625=EDGE_CURVE('',#11073,#11074,#7473,.T.);
#14626=EDGE_CURVE('',#11071,#11074,#7474,.T.);
#14627=EDGE_CURVE('',#11075,#11076,#5149,.T.);
#14628=EDGE_CURVE('',#11076,#11077,#7475,.T.);
#14629=EDGE_CURVE('',#11077,#11078,#5150,.T.);
#14630=EDGE_CURVE('',#11078,#11075,#7476,.T.);
#14631=EDGE_CURVE('',#11077,#11072,#5151,.T.);
#14632=EDGE_CURVE('',#11069,#11076,#5152,.T.);
#14633=EDGE_CURVE('',#11079,#11080,#5153,.T.);
#14634=EDGE_CURVE('',#11080,#11081,#7477,.T.);
#14635=EDGE_CURVE('',#11081,#11082,#5154,.T.);
#14636=EDGE_CURVE('',#11082,#11079,#7478,.T.);
#14637=EDGE_CURVE('',#11083,#11080,#7479,.T.);
#14638=EDGE_CURVE('',#11083,#11084,#7480,.T.);
#14639=EDGE_CURVE('',#11081,#11084,#7481,.T.);
#14640=EDGE_CURVE('',#11085,#11086,#5155,.T.);
#14641=EDGE_CURVE('',#11086,#11087,#7482,.T.);
#14642=EDGE_CURVE('',#11087,#11088,#5156,.T.);
#14643=EDGE_CURVE('',#11088,#11085,#7483,.T.);
#14644=EDGE_CURVE('',#11087,#11082,#5157,.T.);
#14645=EDGE_CURVE('',#11079,#11086,#5158,.T.);
#14646=EDGE_CURVE('',#11089,#11090,#5159,.T.);
#14647=EDGE_CURVE('',#11090,#11091,#7484,.T.);
#14648=EDGE_CURVE('',#11091,#11092,#5160,.T.);
#14649=EDGE_CURVE('',#11092,#11089,#7485,.T.);
#14650=EDGE_CURVE('',#11093,#11090,#7486,.T.);
#14651=EDGE_CURVE('',#11093,#11094,#7487,.T.);
#14652=EDGE_CURVE('',#11091,#11094,#7488,.T.);
#14653=EDGE_CURVE('',#11095,#11096,#5161,.T.);
#14654=EDGE_CURVE('',#11096,#11097,#7489,.T.);
#14655=EDGE_CURVE('',#11097,#11098,#5162,.T.);
#14656=EDGE_CURVE('',#11098,#11095,#7490,.T.);
#14657=EDGE_CURVE('',#11097,#11092,#5163,.T.);
#14658=EDGE_CURVE('',#11089,#11096,#5164,.T.);
#14659=EDGE_CURVE('',#11099,#11100,#5165,.T.);
#14660=EDGE_CURVE('',#11100,#11101,#7491,.T.);
#14661=EDGE_CURVE('',#11101,#11102,#5166,.T.);
#14662=EDGE_CURVE('',#11102,#11099,#7492,.T.);
#14663=EDGE_CURVE('',#11103,#11100,#7493,.T.);
#14664=EDGE_CURVE('',#11103,#11104,#7494,.T.);
#14665=EDGE_CURVE('',#11101,#11104,#7495,.T.);
#14666=EDGE_CURVE('',#11105,#11106,#5167,.T.);
#14667=EDGE_CURVE('',#11106,#11107,#7496,.T.);
#14668=EDGE_CURVE('',#11107,#11108,#5168,.T.);
#14669=EDGE_CURVE('',#11108,#11105,#7497,.T.);
#14670=EDGE_CURVE('',#11107,#11102,#5169,.T.);
#14671=EDGE_CURVE('',#11099,#11106,#5170,.T.);
#14672=EDGE_CURVE('',#11109,#11110,#5171,.T.);
#14673=EDGE_CURVE('',#11110,#11111,#7498,.T.);
#14674=EDGE_CURVE('',#11111,#11112,#5172,.T.);
#14675=EDGE_CURVE('',#11112,#11109,#7499,.T.);
#14676=EDGE_CURVE('',#11113,#11110,#7500,.T.);
#14677=EDGE_CURVE('',#11113,#11114,#7501,.T.);
#14678=EDGE_CURVE('',#11111,#11114,#7502,.T.);
#14679=EDGE_CURVE('',#11115,#11116,#5173,.T.);
#14680=EDGE_CURVE('',#11116,#11117,#7503,.T.);
#14681=EDGE_CURVE('',#11117,#11118,#5174,.T.);
#14682=EDGE_CURVE('',#11118,#11115,#7504,.T.);
#14683=EDGE_CURVE('',#11117,#11112,#5175,.T.);
#14684=EDGE_CURVE('',#11109,#11116,#5176,.T.);
#14685=EDGE_CURVE('',#11119,#11120,#5177,.T.);
#14686=EDGE_CURVE('',#11120,#11121,#7505,.T.);
#14687=EDGE_CURVE('',#11121,#11122,#5178,.T.);
#14688=EDGE_CURVE('',#11122,#11119,#7506,.T.);
#14689=EDGE_CURVE('',#11123,#11120,#7507,.T.);
#14690=EDGE_CURVE('',#11123,#11124,#7508,.T.);
#14691=EDGE_CURVE('',#11121,#11124,#7509,.T.);
#14692=EDGE_CURVE('',#11125,#11126,#5179,.T.);
#14693=EDGE_CURVE('',#11126,#11127,#7510,.T.);
#14694=EDGE_CURVE('',#11127,#11128,#5180,.T.);
#14695=EDGE_CURVE('',#11128,#11125,#7511,.T.);
#14696=EDGE_CURVE('',#11127,#11122,#5181,.T.);
#14697=EDGE_CURVE('',#11119,#11126,#5182,.T.);
#14698=EDGE_CURVE('',#11129,#11130,#5183,.T.);
#14699=EDGE_CURVE('',#11130,#11131,#7512,.T.);
#14700=EDGE_CURVE('',#11131,#11132,#5184,.T.);
#14701=EDGE_CURVE('',#11132,#11129,#7513,.T.);
#14702=EDGE_CURVE('',#11133,#11130,#7514,.T.);
#14703=EDGE_CURVE('',#11133,#11134,#7515,.T.);
#14704=EDGE_CURVE('',#11131,#11134,#7516,.T.);
#14705=EDGE_CURVE('',#11135,#11136,#5185,.T.);
#14706=EDGE_CURVE('',#11136,#11137,#7517,.T.);
#14707=EDGE_CURVE('',#11137,#11138,#5186,.T.);
#14708=EDGE_CURVE('',#11138,#11135,#7518,.T.);
#14709=EDGE_CURVE('',#11137,#11132,#5187,.T.);
#14710=EDGE_CURVE('',#11129,#11136,#5188,.T.);
#14711=EDGE_CURVE('',#11139,#11140,#5189,.T.);
#14712=EDGE_CURVE('',#11140,#11141,#7519,.T.);
#14713=EDGE_CURVE('',#11141,#11142,#5190,.T.);
#14714=EDGE_CURVE('',#11142,#11139,#7520,.T.);
#14715=EDGE_CURVE('',#11143,#11140,#7521,.T.);
#14716=EDGE_CURVE('',#11143,#11144,#7522,.T.);
#14717=EDGE_CURVE('',#11141,#11144,#7523,.T.);
#14718=EDGE_CURVE('',#11145,#11146,#5191,.T.);
#14719=EDGE_CURVE('',#11146,#11147,#7524,.T.);
#14720=EDGE_CURVE('',#11147,#11148,#5192,.T.);
#14721=EDGE_CURVE('',#11148,#11145,#7525,.T.);
#14722=EDGE_CURVE('',#11147,#11142,#5193,.T.);
#14723=EDGE_CURVE('',#11139,#11146,#5194,.T.);
#14724=EDGE_CURVE('',#11149,#11150,#5195,.T.);
#14725=EDGE_CURVE('',#11150,#11151,#7526,.T.);
#14726=EDGE_CURVE('',#11151,#11152,#5196,.T.);
#14727=EDGE_CURVE('',#11152,#11149,#7527,.T.);
#14728=EDGE_CURVE('',#11153,#11150,#7528,.T.);
#14729=EDGE_CURVE('',#11153,#11154,#7529,.T.);
#14730=EDGE_CURVE('',#11151,#11154,#7530,.T.);
#14731=EDGE_CURVE('',#11155,#11156,#5197,.T.);
#14732=EDGE_CURVE('',#11156,#11157,#7531,.T.);
#14733=EDGE_CURVE('',#11157,#11158,#5198,.T.);
#14734=EDGE_CURVE('',#11158,#11155,#7532,.T.);
#14735=EDGE_CURVE('',#11157,#11152,#5199,.T.);
#14736=EDGE_CURVE('',#11149,#11156,#5200,.T.);
#14737=EDGE_CURVE('',#11159,#11160,#5201,.T.);
#14738=EDGE_CURVE('',#11160,#11161,#7533,.T.);
#14739=EDGE_CURVE('',#11161,#11162,#5202,.T.);
#14740=EDGE_CURVE('',#11162,#11159,#7534,.T.);
#14741=EDGE_CURVE('',#11163,#11160,#7535,.T.);
#14742=EDGE_CURVE('',#11163,#11164,#7536,.T.);
#14743=EDGE_CURVE('',#11161,#11164,#7537,.T.);
#14744=EDGE_CURVE('',#11165,#11166,#5203,.T.);
#14745=EDGE_CURVE('',#11166,#11167,#7538,.T.);
#14746=EDGE_CURVE('',#11167,#11168,#5204,.T.);
#14747=EDGE_CURVE('',#11168,#11165,#7539,.T.);
#14748=EDGE_CURVE('',#11167,#11162,#5205,.T.);
#14749=EDGE_CURVE('',#11159,#11166,#5206,.T.);
#14750=EDGE_CURVE('',#11169,#11170,#5207,.T.);
#14751=EDGE_CURVE('',#11170,#11171,#7540,.T.);
#14752=EDGE_CURVE('',#11171,#11172,#5208,.T.);
#14753=EDGE_CURVE('',#11172,#11169,#7541,.T.);
#14754=EDGE_CURVE('',#11173,#11170,#7542,.T.);
#14755=EDGE_CURVE('',#11173,#11174,#7543,.T.);
#14756=EDGE_CURVE('',#11171,#11174,#7544,.T.);
#14757=EDGE_CURVE('',#11175,#11176,#5209,.T.);
#14758=EDGE_CURVE('',#11176,#11177,#7545,.T.);
#14759=EDGE_CURVE('',#11177,#11178,#5210,.T.);
#14760=EDGE_CURVE('',#11178,#11175,#7546,.T.);
#14761=EDGE_CURVE('',#11177,#11172,#5211,.T.);
#14762=EDGE_CURVE('',#11169,#11176,#5212,.T.);
#14763=EDGE_CURVE('',#11179,#11180,#5213,.T.);
#14764=EDGE_CURVE('',#11180,#11181,#7547,.T.);
#14765=EDGE_CURVE('',#11181,#11182,#5214,.T.);
#14766=EDGE_CURVE('',#11182,#11179,#7548,.T.);
#14767=EDGE_CURVE('',#11183,#11180,#7549,.T.);
#14768=EDGE_CURVE('',#11183,#11184,#7550,.T.);
#14769=EDGE_CURVE('',#11181,#11184,#7551,.T.);
#14770=EDGE_CURVE('',#11185,#11186,#5215,.T.);
#14771=EDGE_CURVE('',#11186,#11187,#7552,.T.);
#14772=EDGE_CURVE('',#11187,#11188,#5216,.T.);
#14773=EDGE_CURVE('',#11188,#11185,#7553,.T.);
#14774=EDGE_CURVE('',#11187,#11182,#5217,.T.);
#14775=EDGE_CURVE('',#11179,#11186,#5218,.T.);
#14776=EDGE_CURVE('',#11189,#11190,#5219,.T.);
#14777=EDGE_CURVE('',#11190,#11191,#7554,.T.);
#14778=EDGE_CURVE('',#11191,#11192,#5220,.T.);
#14779=EDGE_CURVE('',#11192,#11189,#7555,.T.);
#14780=EDGE_CURVE('',#11193,#11190,#7556,.T.);
#14781=EDGE_CURVE('',#11193,#11194,#7557,.T.);
#14782=EDGE_CURVE('',#11191,#11194,#7558,.T.);
#14783=EDGE_CURVE('',#11195,#11196,#5221,.T.);
#14784=EDGE_CURVE('',#11196,#11197,#7559,.T.);
#14785=EDGE_CURVE('',#11197,#11198,#5222,.T.);
#14786=EDGE_CURVE('',#11198,#11195,#7560,.T.);
#14787=EDGE_CURVE('',#11197,#11192,#5223,.T.);
#14788=EDGE_CURVE('',#11189,#11196,#5224,.T.);
#14789=EDGE_CURVE('',#11199,#11200,#5225,.T.);
#14790=EDGE_CURVE('',#11200,#11201,#7561,.T.);
#14791=EDGE_CURVE('',#11201,#11202,#5226,.T.);
#14792=EDGE_CURVE('',#11202,#11199,#7562,.T.);
#14793=EDGE_CURVE('',#11203,#11200,#7563,.T.);
#14794=EDGE_CURVE('',#11203,#11204,#7564,.T.);
#14795=EDGE_CURVE('',#11201,#11204,#7565,.T.);
#14796=EDGE_CURVE('',#11205,#11206,#5227,.T.);
#14797=EDGE_CURVE('',#11206,#11207,#7566,.T.);
#14798=EDGE_CURVE('',#11207,#11208,#5228,.T.);
#14799=EDGE_CURVE('',#11208,#11205,#7567,.T.);
#14800=EDGE_CURVE('',#11207,#11202,#5229,.T.);
#14801=EDGE_CURVE('',#11199,#11206,#5230,.T.);
#14802=EDGE_CURVE('',#11209,#11210,#5231,.T.);
#14803=EDGE_CURVE('',#11210,#11211,#7568,.T.);
#14804=EDGE_CURVE('',#11211,#11212,#5232,.T.);
#14805=EDGE_CURVE('',#11212,#11209,#7569,.T.);
#14806=EDGE_CURVE('',#11213,#11210,#7570,.T.);
#14807=EDGE_CURVE('',#11213,#11214,#7571,.T.);
#14808=EDGE_CURVE('',#11211,#11214,#7572,.T.);
#14809=EDGE_CURVE('',#11215,#11216,#5233,.T.);
#14810=EDGE_CURVE('',#11216,#11217,#7573,.T.);
#14811=EDGE_CURVE('',#11217,#11218,#5234,.T.);
#14812=EDGE_CURVE('',#11218,#11215,#7574,.T.);
#14813=EDGE_CURVE('',#11217,#11212,#5235,.T.);
#14814=EDGE_CURVE('',#11209,#11216,#5236,.T.);
#14815=EDGE_CURVE('',#11219,#11220,#5237,.T.);
#14816=EDGE_CURVE('',#11220,#11221,#7575,.T.);
#14817=EDGE_CURVE('',#11221,#11222,#5238,.T.);
#14818=EDGE_CURVE('',#11222,#11219,#7576,.T.);
#14819=EDGE_CURVE('',#11223,#11220,#7577,.T.);
#14820=EDGE_CURVE('',#11223,#11224,#7578,.T.);
#14821=EDGE_CURVE('',#11221,#11224,#7579,.T.);
#14822=EDGE_CURVE('',#11225,#11226,#5239,.T.);
#14823=EDGE_CURVE('',#11226,#11227,#7580,.T.);
#14824=EDGE_CURVE('',#11227,#11228,#5240,.T.);
#14825=EDGE_CURVE('',#11228,#11225,#7581,.T.);
#14826=EDGE_CURVE('',#11227,#11222,#5241,.T.);
#14827=EDGE_CURVE('',#11219,#11226,#5242,.T.);
#14828=EDGE_CURVE('',#11229,#11230,#5243,.T.);
#14829=EDGE_CURVE('',#11230,#11231,#7582,.T.);
#14830=EDGE_CURVE('',#11231,#11232,#5244,.T.);
#14831=EDGE_CURVE('',#11232,#11229,#7583,.T.);
#14832=EDGE_CURVE('',#11233,#11230,#7584,.T.);
#14833=EDGE_CURVE('',#11233,#11234,#7585,.T.);
#14834=EDGE_CURVE('',#11231,#11234,#7586,.T.);
#14835=EDGE_CURVE('',#11235,#11236,#5245,.T.);
#14836=EDGE_CURVE('',#11236,#11237,#7587,.T.);
#14837=EDGE_CURVE('',#11237,#11238,#5246,.T.);
#14838=EDGE_CURVE('',#11238,#11235,#7588,.T.);
#14839=EDGE_CURVE('',#11237,#11232,#5247,.T.);
#14840=EDGE_CURVE('',#11229,#11236,#5248,.T.);
#14841=EDGE_CURVE('',#11239,#11018,#7589,.T.);
#14842=EDGE_CURVE('',#11240,#11239,#7590,.T.);
#14843=EDGE_CURVE('',#11015,#11240,#7591,.T.);
#14844=EDGE_CURVE('',#11241,#11013,#787,.T.);
#14845=EDGE_CURVE('',#11242,#11241,#7592,.T.);
#14846=EDGE_CURVE('',#11014,#11242,#788,.T.);
#14847=EDGE_CURVE('',#11240,#11243,#789,.T.);
#14848=EDGE_CURVE('',#11244,#11239,#790,.T.);
#14849=EDGE_CURVE('',#11243,#11244,#7593,.T.);
#14850=EDGE_CURVE('',#11245,#11028,#7594,.T.);
#14851=EDGE_CURVE('',#11246,#11245,#7595,.T.);
#14852=EDGE_CURVE('',#11025,#11246,#7596,.T.);
#14853=EDGE_CURVE('',#11247,#11023,#791,.T.);
#14854=EDGE_CURVE('',#11248,#11247,#7597,.T.);
#14855=EDGE_CURVE('',#11024,#11248,#792,.T.);
#14856=EDGE_CURVE('',#11246,#11249,#793,.T.);
#14857=EDGE_CURVE('',#11250,#11245,#794,.T.);
#14858=EDGE_CURVE('',#11249,#11250,#7598,.T.);
#14859=EDGE_CURVE('',#11251,#11038,#7599,.T.);
#14860=EDGE_CURVE('',#11252,#11251,#7600,.T.);
#14861=EDGE_CURVE('',#11035,#11252,#7601,.T.);
#14862=EDGE_CURVE('',#11253,#11033,#795,.T.);
#14863=EDGE_CURVE('',#11254,#11253,#7602,.T.);
#14864=EDGE_CURVE('',#11034,#11254,#796,.T.);
#14865=EDGE_CURVE('',#11252,#11255,#797,.T.);
#14866=EDGE_CURVE('',#11256,#11251,#798,.T.);
#14867=EDGE_CURVE('',#11255,#11256,#7603,.T.);
#14868=EDGE_CURVE('',#11257,#11048,#7604,.T.);
#14869=EDGE_CURVE('',#11258,#11257,#7605,.T.);
#14870=EDGE_CURVE('',#11045,#11258,#7606,.T.);
#14871=EDGE_CURVE('',#11259,#11043,#799,.T.);
#14872=EDGE_CURVE('',#11260,#11259,#7607,.T.);
#14873=EDGE_CURVE('',#11044,#11260,#800,.T.);
#14874=EDGE_CURVE('',#11258,#11261,#801,.T.);
#14875=EDGE_CURVE('',#11262,#11257,#802,.T.);
#14876=EDGE_CURVE('',#11261,#11262,#7608,.T.);
#14877=EDGE_CURVE('',#11263,#11058,#7609,.T.);
#14878=EDGE_CURVE('',#11264,#11263,#7610,.T.);
#14879=EDGE_CURVE('',#11055,#11264,#7611,.T.);
#14880=EDGE_CURVE('',#11265,#11053,#803,.T.);
#14881=EDGE_CURVE('',#11266,#11265,#7612,.T.);
#14882=EDGE_CURVE('',#11054,#11266,#804,.T.);
#14883=EDGE_CURVE('',#11264,#11267,#805,.T.);
#14884=EDGE_CURVE('',#11268,#11263,#806,.T.);
#14885=EDGE_CURVE('',#11267,#11268,#7613,.T.);
#14886=EDGE_CURVE('',#11269,#11068,#7614,.T.);
#14887=EDGE_CURVE('',#11270,#11269,#7615,.T.);
#14888=EDGE_CURVE('',#11065,#11270,#7616,.T.);
#14889=EDGE_CURVE('',#11271,#11063,#807,.T.);
#14890=EDGE_CURVE('',#11272,#11271,#7617,.T.);
#14891=EDGE_CURVE('',#11064,#11272,#808,.T.);
#14892=EDGE_CURVE('',#11270,#11273,#809,.T.);
#14893=EDGE_CURVE('',#11274,#11269,#810,.T.);
#14894=EDGE_CURVE('',#11273,#11274,#7618,.T.);
#14895=EDGE_CURVE('',#11275,#11078,#7619,.T.);
#14896=EDGE_CURVE('',#11276,#11275,#7620,.T.);
#14897=EDGE_CURVE('',#11075,#11276,#7621,.T.);
#14898=EDGE_CURVE('',#11277,#11073,#811,.T.);
#14899=EDGE_CURVE('',#11278,#11277,#7622,.T.);
#14900=EDGE_CURVE('',#11074,#11278,#812,.T.);
#14901=EDGE_CURVE('',#11276,#11279,#813,.T.);
#14902=EDGE_CURVE('',#11280,#11275,#814,.T.);
#14903=EDGE_CURVE('',#11279,#11280,#7623,.T.);
#14904=EDGE_CURVE('',#11281,#11088,#7624,.T.);
#14905=EDGE_CURVE('',#11282,#11281,#7625,.T.);
#14906=EDGE_CURVE('',#11085,#11282,#7626,.T.);
#14907=EDGE_CURVE('',#11283,#11083,#815,.T.);
#14908=EDGE_CURVE('',#11284,#11283,#7627,.T.);
#14909=EDGE_CURVE('',#11084,#11284,#816,.T.);
#14910=EDGE_CURVE('',#11282,#11285,#817,.T.);
#14911=EDGE_CURVE('',#11286,#11281,#818,.T.);
#14912=EDGE_CURVE('',#11285,#11286,#7628,.T.);
#14913=EDGE_CURVE('',#11287,#11098,#7629,.T.);
#14914=EDGE_CURVE('',#11288,#11287,#7630,.T.);
#14915=EDGE_CURVE('',#11095,#11288,#7631,.T.);
#14916=EDGE_CURVE('',#11289,#11093,#819,.T.);
#14917=EDGE_CURVE('',#11290,#11289,#7632,.T.);
#14918=EDGE_CURVE('',#11094,#11290,#820,.T.);
#14919=EDGE_CURVE('',#11288,#11291,#821,.T.);
#14920=EDGE_CURVE('',#11292,#11287,#822,.T.);
#14921=EDGE_CURVE('',#11291,#11292,#7633,.T.);
#14922=EDGE_CURVE('',#11293,#11108,#7634,.T.);
#14923=EDGE_CURVE('',#11294,#11293,#7635,.T.);
#14924=EDGE_CURVE('',#11105,#11294,#7636,.T.);
#14925=EDGE_CURVE('',#11295,#11103,#823,.T.);
#14926=EDGE_CURVE('',#11296,#11295,#7637,.T.);
#14927=EDGE_CURVE('',#11104,#11296,#824,.T.);
#14928=EDGE_CURVE('',#11294,#11297,#825,.T.);
#14929=EDGE_CURVE('',#11298,#11293,#826,.T.);
#14930=EDGE_CURVE('',#11297,#11298,#7638,.T.);
#14931=EDGE_CURVE('',#11299,#11118,#7639,.T.);
#14932=EDGE_CURVE('',#11300,#11299,#7640,.T.);
#14933=EDGE_CURVE('',#11115,#11300,#7641,.T.);
#14934=EDGE_CURVE('',#11301,#11113,#827,.T.);
#14935=EDGE_CURVE('',#11302,#11301,#7642,.T.);
#14936=EDGE_CURVE('',#11114,#11302,#828,.T.);
#14937=EDGE_CURVE('',#11300,#11303,#829,.T.);
#14938=EDGE_CURVE('',#11304,#11299,#830,.T.);
#14939=EDGE_CURVE('',#11303,#11304,#7643,.T.);
#14940=EDGE_CURVE('',#11305,#11128,#7644,.T.);
#14941=EDGE_CURVE('',#11306,#11305,#7645,.T.);
#14942=EDGE_CURVE('',#11125,#11306,#7646,.T.);
#14943=EDGE_CURVE('',#11307,#11123,#831,.T.);
#14944=EDGE_CURVE('',#11308,#11307,#7647,.T.);
#14945=EDGE_CURVE('',#11124,#11308,#832,.T.);
#14946=EDGE_CURVE('',#11306,#11309,#833,.T.);
#14947=EDGE_CURVE('',#11310,#11305,#834,.T.);
#14948=EDGE_CURVE('',#11309,#11310,#7648,.T.);
#14949=EDGE_CURVE('',#11311,#11138,#7649,.T.);
#14950=EDGE_CURVE('',#11312,#11311,#7650,.T.);
#14951=EDGE_CURVE('',#11135,#11312,#7651,.T.);
#14952=EDGE_CURVE('',#11313,#11133,#835,.T.);
#14953=EDGE_CURVE('',#11314,#11313,#7652,.T.);
#14954=EDGE_CURVE('',#11134,#11314,#836,.T.);
#14955=EDGE_CURVE('',#11312,#11315,#837,.T.);
#14956=EDGE_CURVE('',#11316,#11311,#838,.T.);
#14957=EDGE_CURVE('',#11315,#11316,#7653,.T.);
#14958=EDGE_CURVE('',#11317,#11148,#7654,.T.);
#14959=EDGE_CURVE('',#11318,#11317,#7655,.T.);
#14960=EDGE_CURVE('',#11145,#11318,#7656,.T.);
#14961=EDGE_CURVE('',#11319,#11143,#839,.T.);
#14962=EDGE_CURVE('',#11320,#11319,#7657,.T.);
#14963=EDGE_CURVE('',#11144,#11320,#840,.T.);
#14964=EDGE_CURVE('',#11318,#11321,#841,.T.);
#14965=EDGE_CURVE('',#11322,#11317,#842,.T.);
#14966=EDGE_CURVE('',#11321,#11322,#7658,.T.);
#14967=EDGE_CURVE('',#11323,#11158,#7659,.T.);
#14968=EDGE_CURVE('',#11324,#11323,#7660,.T.);
#14969=EDGE_CURVE('',#11155,#11324,#7661,.T.);
#14970=EDGE_CURVE('',#11325,#11153,#843,.T.);
#14971=EDGE_CURVE('',#11326,#11325,#7662,.T.);
#14972=EDGE_CURVE('',#11154,#11326,#844,.T.);
#14973=EDGE_CURVE('',#11324,#11327,#845,.T.);
#14974=EDGE_CURVE('',#11328,#11323,#846,.T.);
#14975=EDGE_CURVE('',#11327,#11328,#7663,.T.);
#14976=EDGE_CURVE('',#11329,#11168,#7664,.T.);
#14977=EDGE_CURVE('',#11330,#11329,#7665,.T.);
#14978=EDGE_CURVE('',#11165,#11330,#7666,.T.);
#14979=EDGE_CURVE('',#11331,#11163,#847,.T.);
#14980=EDGE_CURVE('',#11332,#11331,#7667,.T.);
#14981=EDGE_CURVE('',#11164,#11332,#848,.T.);
#14982=EDGE_CURVE('',#11330,#11333,#849,.T.);
#14983=EDGE_CURVE('',#11334,#11329,#850,.T.);
#14984=EDGE_CURVE('',#11333,#11334,#7668,.T.);
#14985=EDGE_CURVE('',#11335,#11178,#7669,.T.);
#14986=EDGE_CURVE('',#11336,#11335,#7670,.T.);
#14987=EDGE_CURVE('',#11175,#11336,#7671,.T.);
#14988=EDGE_CURVE('',#11337,#11173,#851,.T.);
#14989=EDGE_CURVE('',#11338,#11337,#7672,.T.);
#14990=EDGE_CURVE('',#11174,#11338,#852,.T.);
#14991=EDGE_CURVE('',#11336,#11339,#853,.T.);
#14992=EDGE_CURVE('',#11340,#11335,#854,.T.);
#14993=EDGE_CURVE('',#11339,#11340,#7673,.T.);
#14994=EDGE_CURVE('',#11341,#11188,#7674,.T.);
#14995=EDGE_CURVE('',#11342,#11341,#7675,.T.);
#14996=EDGE_CURVE('',#11185,#11342,#7676,.T.);
#14997=EDGE_CURVE('',#11343,#11183,#855,.T.);
#14998=EDGE_CURVE('',#11344,#11343,#7677,.T.);
#14999=EDGE_CURVE('',#11184,#11344,#856,.T.);
#15000=EDGE_CURVE('',#11342,#11345,#857,.T.);
#15001=EDGE_CURVE('',#11346,#11341,#858,.T.);
#15002=EDGE_CURVE('',#11345,#11346,#7678,.T.);
#15003=EDGE_CURVE('',#11347,#11198,#7679,.T.);
#15004=EDGE_CURVE('',#11348,#11347,#7680,.T.);
#15005=EDGE_CURVE('',#11195,#11348,#7681,.T.);
#15006=EDGE_CURVE('',#11349,#11193,#859,.T.);
#15007=EDGE_CURVE('',#11350,#11349,#7682,.T.);
#15008=EDGE_CURVE('',#11194,#11350,#860,.T.);
#15009=EDGE_CURVE('',#11348,#11351,#861,.T.);
#15010=EDGE_CURVE('',#11352,#11347,#862,.T.);
#15011=EDGE_CURVE('',#11351,#11352,#7683,.T.);
#15012=EDGE_CURVE('',#11353,#11208,#7684,.T.);
#15013=EDGE_CURVE('',#11354,#11353,#7685,.T.);
#15014=EDGE_CURVE('',#11205,#11354,#7686,.T.);
#15015=EDGE_CURVE('',#11355,#11203,#863,.T.);
#15016=EDGE_CURVE('',#11356,#11355,#7687,.T.);
#15017=EDGE_CURVE('',#11204,#11356,#864,.T.);
#15018=EDGE_CURVE('',#11354,#11357,#865,.T.);
#15019=EDGE_CURVE('',#11358,#11353,#866,.T.);
#15020=EDGE_CURVE('',#11357,#11358,#7688,.T.);
#15021=EDGE_CURVE('',#11359,#11218,#7689,.T.);
#15022=EDGE_CURVE('',#11360,#11359,#7690,.T.);
#15023=EDGE_CURVE('',#11215,#11360,#7691,.T.);
#15024=EDGE_CURVE('',#11361,#11213,#867,.T.);
#15025=EDGE_CURVE('',#11362,#11361,#7692,.T.);
#15026=EDGE_CURVE('',#11214,#11362,#868,.T.);
#15027=EDGE_CURVE('',#11360,#11363,#869,.T.);
#15028=EDGE_CURVE('',#11364,#11359,#870,.T.);
#15029=EDGE_CURVE('',#11363,#11364,#7693,.T.);
#15030=EDGE_CURVE('',#11365,#11228,#7694,.T.);
#15031=EDGE_CURVE('',#11366,#11365,#7695,.T.);
#15032=EDGE_CURVE('',#11225,#11366,#7696,.T.);
#15033=EDGE_CURVE('',#11367,#11223,#871,.T.);
#15034=EDGE_CURVE('',#11368,#11367,#7697,.T.);
#15035=EDGE_CURVE('',#11224,#11368,#872,.T.);
#15036=EDGE_CURVE('',#11366,#11369,#873,.T.);
#15037=EDGE_CURVE('',#11370,#11365,#874,.T.);
#15038=EDGE_CURVE('',#11369,#11370,#7698,.T.);
#15039=EDGE_CURVE('',#11371,#11238,#7699,.T.);
#15040=EDGE_CURVE('',#11372,#11371,#7700,.T.);
#15041=EDGE_CURVE('',#11235,#11372,#7701,.T.);
#15042=EDGE_CURVE('',#11373,#11233,#875,.T.);
#15043=EDGE_CURVE('',#11374,#11373,#7702,.T.);
#15044=EDGE_CURVE('',#11234,#11374,#876,.T.);
#15045=EDGE_CURVE('',#11372,#11375,#877,.T.);
#15046=EDGE_CURVE('',#11376,#11371,#878,.T.);
#15047=EDGE_CURVE('',#11375,#11376,#7703,.T.);
#15048=EDGE_CURVE('',#11247,#11243,#5249,.T.);
#15049=EDGE_CURVE('',#11253,#11249,#5250,.T.);
#15050=EDGE_CURVE('',#11259,#11255,#5251,.T.);
#15051=EDGE_CURVE('',#11265,#11261,#5252,.T.);
#15052=EDGE_CURVE('',#11271,#11267,#5253,.T.);
#15053=EDGE_CURVE('',#11277,#11273,#5254,.T.);
#15054=EDGE_CURVE('',#11283,#11279,#5255,.T.);
#15055=EDGE_CURVE('',#11289,#11285,#5256,.T.);
#15056=EDGE_CURVE('',#11295,#11291,#5257,.T.);
#15057=EDGE_CURVE('',#11301,#11297,#5258,.T.);
#15058=EDGE_CURVE('',#11307,#11303,#5259,.T.);
#15059=EDGE_CURVE('',#11313,#11309,#5260,.T.);
#15060=EDGE_CURVE('',#11319,#11315,#5261,.T.);
#15061=EDGE_CURVE('',#11325,#11321,#5262,.T.);
#15062=EDGE_CURVE('',#11331,#11327,#5263,.T.);
#15063=EDGE_CURVE('',#11337,#11333,#5264,.T.);
#15064=EDGE_CURVE('',#11343,#11339,#5265,.T.);
#15065=EDGE_CURVE('',#11349,#11345,#5266,.T.);
#15066=EDGE_CURVE('',#11355,#11351,#5267,.T.);
#15067=EDGE_CURVE('',#11361,#11357,#5268,.T.);
#15068=EDGE_CURVE('',#11367,#11363,#5269,.T.);
#15069=EDGE_CURVE('',#11373,#11369,#5270,.T.);
#15070=EDGE_CURVE('',#11377,#11375,#5271,.T.);
#15071=EDGE_CURVE('',#11377,#11378,#879,.T.);
#15072=EDGE_CURVE('',#11378,#11379,#7704,.T.);
#15073=EDGE_CURVE('',#11380,#11379,#5272,.T.);
#15074=EDGE_CURVE('',#11380,#11381,#5273,.T.);
#15075=EDGE_CURVE('',#11382,#11381,#5274,.T.);
#15076=EDGE_CURVE('',#11382,#11383,#7705,.T.);
#15077=EDGE_CURVE('',#11383,#11384,#880,.T.);
#15078=EDGE_CURVE('',#11241,#11384,#5275,.T.);
#15079=EDGE_CURVE('',#11385,#11385,#5276,.T.);
#15080=EDGE_CURVE('',#11242,#11386,#5277,.T.);
#15081=EDGE_CURVE('',#11386,#11387,#881,.T.);
#15082=EDGE_CURVE('',#11387,#11388,#7706,.T.);
#15083=EDGE_CURVE('',#11389,#11388,#5278,.T.);
#15084=EDGE_CURVE('',#11389,#11390,#5279,.T.);
#15085=EDGE_CURVE('',#11391,#11390,#5280,.T.);
#15086=EDGE_CURVE('',#11391,#11392,#7707,.T.);
#15087=EDGE_CURVE('',#11392,#11393,#882,.T.);
#15088=EDGE_CURVE('',#11393,#11376,#5281,.T.);
#15089=EDGE_CURVE('',#11374,#11370,#5282,.T.);
#15090=EDGE_CURVE('',#11368,#11364,#5283,.T.);
#15091=EDGE_CURVE('',#11362,#11358,#5284,.T.);
#15092=EDGE_CURVE('',#11356,#11352,#5285,.T.);
#15093=EDGE_CURVE('',#11350,#11346,#5286,.T.);
#15094=EDGE_CURVE('',#11344,#11340,#5287,.T.);
#15095=EDGE_CURVE('',#11338,#11334,#5288,.T.);
#15096=EDGE_CURVE('',#11332,#11328,#5289,.T.);
#15097=EDGE_CURVE('',#11326,#11322,#5290,.T.);
#15098=EDGE_CURVE('',#11320,#11316,#5291,.T.);
#15099=EDGE_CURVE('',#11314,#11310,#5292,.T.);
#15100=EDGE_CURVE('',#11308,#11304,#5293,.T.);
#15101=EDGE_CURVE('',#11302,#11298,#5294,.T.);
#15102=EDGE_CURVE('',#11296,#11292,#5295,.T.);
#15103=EDGE_CURVE('',#11290,#11286,#5296,.T.);
#15104=EDGE_CURVE('',#11284,#11280,#5297,.T.);
#15105=EDGE_CURVE('',#11278,#11274,#5298,.T.);
#15106=EDGE_CURVE('',#11272,#11268,#5299,.T.);
#15107=EDGE_CURVE('',#11266,#11262,#5300,.T.);
#15108=EDGE_CURVE('',#11260,#11256,#5301,.T.);
#15109=EDGE_CURVE('',#11254,#11250,#5302,.T.);
#15110=EDGE_CURVE('',#11248,#11244,#5303,.T.);
#15111=EDGE_CURVE('',#11394,#11394,#5304,.T.);
#15112=EDGE_CURVE('',#11393,#11377,#7708,.T.);
#15113=EDGE_CURVE('',#11379,#11391,#7709,.T.);
#15114=EDGE_CURVE('',#11390,#11380,#7710,.T.);
#15115=EDGE_CURVE('',#11378,#11392,#7711,.T.);
#15116=EDGE_CURVE('',#11381,#11389,#7712,.T.);
#15117=EDGE_CURVE('',#11388,#11382,#7713,.T.);
#15118=EDGE_CURVE('',#11383,#11387,#7714,.T.);
#15119=EDGE_CURVE('',#11384,#11386,#7715,.T.);
#15120=EDGE_CURVE('',#11394,#11385,#7716,.T.);
#21314=ORIENTED_EDGE('',*,*,#14542,.T.);
#21315=ORIENTED_EDGE('',*,*,#14543,.T.);
#21316=ORIENTED_EDGE('',*,*,#14544,.T.);
#21317=ORIENTED_EDGE('',*,*,#14545,.T.);
#21318=ORIENTED_EDGE('',*,*,#14543,.F.);
#21319=ORIENTED_EDGE('',*,*,#14546,.F.);
#21320=ORIENTED_EDGE('',*,*,#14547,.T.);
#21321=ORIENTED_EDGE('',*,*,#14548,.F.);
#21322=ORIENTED_EDGE('',*,*,#14549,.T.);
#21323=ORIENTED_EDGE('',*,*,#14550,.T.);
#21324=ORIENTED_EDGE('',*,*,#14551,.T.);
#21325=ORIENTED_EDGE('',*,*,#14552,.T.);
#21326=ORIENTED_EDGE('',*,*,#14545,.F.);
#21327=ORIENTED_EDGE('',*,*,#14553,.F.);
#21328=ORIENTED_EDGE('',*,*,#14550,.F.);
#21329=ORIENTED_EDGE('',*,*,#14554,.F.);
#21330=ORIENTED_EDGE('',*,*,#14555,.T.);
#21331=ORIENTED_EDGE('',*,*,#14556,.T.);
#21332=ORIENTED_EDGE('',*,*,#14557,.T.);
#21333=ORIENTED_EDGE('',*,*,#14558,.T.);
#21334=ORIENTED_EDGE('',*,*,#14556,.F.);
#21335=ORIENTED_EDGE('',*,*,#14559,.F.);
#21336=ORIENTED_EDGE('',*,*,#14560,.T.);
#21337=ORIENTED_EDGE('',*,*,#14561,.F.);
#21338=ORIENTED_EDGE('',*,*,#14562,.T.);
#21339=ORIENTED_EDGE('',*,*,#14563,.T.);
#21340=ORIENTED_EDGE('',*,*,#14564,.T.);
#21341=ORIENTED_EDGE('',*,*,#14565,.T.);
#21342=ORIENTED_EDGE('',*,*,#14558,.F.);
#21343=ORIENTED_EDGE('',*,*,#14566,.F.);
#21344=ORIENTED_EDGE('',*,*,#14563,.F.);
#21345=ORIENTED_EDGE('',*,*,#14567,.F.);
#21346=ORIENTED_EDGE('',*,*,#14568,.T.);
#21347=ORIENTED_EDGE('',*,*,#14569,.T.);
#21348=ORIENTED_EDGE('',*,*,#14570,.T.);
#21349=ORIENTED_EDGE('',*,*,#14571,.T.);
#21350=ORIENTED_EDGE('',*,*,#14569,.F.);
#21351=ORIENTED_EDGE('',*,*,#14572,.F.);
#21352=ORIENTED_EDGE('',*,*,#14573,.T.);
#21353=ORIENTED_EDGE('',*,*,#14574,.F.);
#21354=ORIENTED_EDGE('',*,*,#14575,.T.);
#21355=ORIENTED_EDGE('',*,*,#14576,.T.);
#21356=ORIENTED_EDGE('',*,*,#14577,.T.);
#21357=ORIENTED_EDGE('',*,*,#14578,.T.);
#21358=ORIENTED_EDGE('',*,*,#14571,.F.);
#21359=ORIENTED_EDGE('',*,*,#14579,.F.);
#21360=ORIENTED_EDGE('',*,*,#14576,.F.);
#21361=ORIENTED_EDGE('',*,*,#14580,.F.);
#21362=ORIENTED_EDGE('',*,*,#14581,.T.);
#21363=ORIENTED_EDGE('',*,*,#14582,.T.);
#21364=ORIENTED_EDGE('',*,*,#14583,.T.);
#21365=ORIENTED_EDGE('',*,*,#14584,.T.);
#21366=ORIENTED_EDGE('',*,*,#14582,.F.);
#21367=ORIENTED_EDGE('',*,*,#14585,.F.);
#21368=ORIENTED_EDGE('',*,*,#14586,.T.);
#21369=ORIENTED_EDGE('',*,*,#14587,.F.);
#21370=ORIENTED_EDGE('',*,*,#14588,.T.);
#21371=ORIENTED_EDGE('',*,*,#14589,.T.);
#21372=ORIENTED_EDGE('',*,*,#14590,.T.);
#21373=ORIENTED_EDGE('',*,*,#14591,.T.);
#21374=ORIENTED_EDGE('',*,*,#14584,.F.);
#21375=ORIENTED_EDGE('',*,*,#14592,.F.);
#21376=ORIENTED_EDGE('',*,*,#14589,.F.);
#21377=ORIENTED_EDGE('',*,*,#14593,.F.);
#21378=ORIENTED_EDGE('',*,*,#14594,.T.);
#21379=ORIENTED_EDGE('',*,*,#14595,.T.);
#21380=ORIENTED_EDGE('',*,*,#14596,.T.);
#21381=ORIENTED_EDGE('',*,*,#14597,.T.);
#21382=ORIENTED_EDGE('',*,*,#14595,.F.);
#21383=ORIENTED_EDGE('',*,*,#14598,.F.);
#21384=ORIENTED_EDGE('',*,*,#14599,.T.);
#21385=ORIENTED_EDGE('',*,*,#14600,.F.);
#21386=ORIENTED_EDGE('',*,*,#14601,.T.);
#21387=ORIENTED_EDGE('',*,*,#14602,.T.);
#21388=ORIENTED_EDGE('',*,*,#14603,.T.);
#21389=ORIENTED_EDGE('',*,*,#14604,.T.);
#21390=ORIENTED_EDGE('',*,*,#14597,.F.);
#21391=ORIENTED_EDGE('',*,*,#14605,.F.);
#21392=ORIENTED_EDGE('',*,*,#14602,.F.);
#21393=ORIENTED_EDGE('',*,*,#14606,.F.);
#21394=ORIENTED_EDGE('',*,*,#14607,.T.);
#21395=ORIENTED_EDGE('',*,*,#14608,.T.);
#21396=ORIENTED_EDGE('',*,*,#14609,.T.);
#21397=ORIENTED_EDGE('',*,*,#14610,.T.);
#21398=ORIENTED_EDGE('',*,*,#14608,.F.);
#21399=ORIENTED_EDGE('',*,*,#14611,.F.);
#21400=ORIENTED_EDGE('',*,*,#14612,.T.);
#21401=ORIENTED_EDGE('',*,*,#14613,.F.);
#21402=ORIENTED_EDGE('',*,*,#14614,.T.);
#21403=ORIENTED_EDGE('',*,*,#14615,.T.);
#21404=ORIENTED_EDGE('',*,*,#14616,.T.);
#21405=ORIENTED_EDGE('',*,*,#14617,.T.);
#21406=ORIENTED_EDGE('',*,*,#14610,.F.);
#21407=ORIENTED_EDGE('',*,*,#14618,.F.);
#21408=ORIENTED_EDGE('',*,*,#14615,.F.);
#21409=ORIENTED_EDGE('',*,*,#14619,.F.);
#21410=ORIENTED_EDGE('',*,*,#14620,.T.);
#21411=ORIENTED_EDGE('',*,*,#14621,.T.);
#21412=ORIENTED_EDGE('',*,*,#14622,.T.);
#21413=ORIENTED_EDGE('',*,*,#14623,.T.);
#21414=ORIENTED_EDGE('',*,*,#14621,.F.);
#21415=ORIENTED_EDGE('',*,*,#14624,.F.);
#21416=ORIENTED_EDGE('',*,*,#14625,.T.);
#21417=ORIENTED_EDGE('',*,*,#14626,.F.);
#21418=ORIENTED_EDGE('',*,*,#14627,.T.);
#21419=ORIENTED_EDGE('',*,*,#14628,.T.);
#21420=ORIENTED_EDGE('',*,*,#14629,.T.);
#21421=ORIENTED_EDGE('',*,*,#14630,.T.);
#21422=ORIENTED_EDGE('',*,*,#14623,.F.);
#21423=ORIENTED_EDGE('',*,*,#14631,.F.);
#21424=ORIENTED_EDGE('',*,*,#14628,.F.);
#21425=ORIENTED_EDGE('',*,*,#14632,.F.);
#21426=ORIENTED_EDGE('',*,*,#14633,.T.);
#21427=ORIENTED_EDGE('',*,*,#14634,.T.);
#21428=ORIENTED_EDGE('',*,*,#14635,.T.);
#21429=ORIENTED_EDGE('',*,*,#14636,.T.);
#21430=ORIENTED_EDGE('',*,*,#14634,.F.);
#21431=ORIENTED_EDGE('',*,*,#14637,.F.);
#21432=ORIENTED_EDGE('',*,*,#14638,.T.);
#21433=ORIENTED_EDGE('',*,*,#14639,.F.);
#21434=ORIENTED_EDGE('',*,*,#14640,.T.);
#21435=ORIENTED_EDGE('',*,*,#14641,.T.);
#21436=ORIENTED_EDGE('',*,*,#14642,.T.);
#21437=ORIENTED_EDGE('',*,*,#14643,.T.);
#21438=ORIENTED_EDGE('',*,*,#14636,.F.);
#21439=ORIENTED_EDGE('',*,*,#14644,.F.);
#21440=ORIENTED_EDGE('',*,*,#14641,.F.);
#21441=ORIENTED_EDGE('',*,*,#14645,.F.);
#21442=ORIENTED_EDGE('',*,*,#14646,.T.);
#21443=ORIENTED_EDGE('',*,*,#14647,.T.);
#21444=ORIENTED_EDGE('',*,*,#14648,.T.);
#21445=ORIENTED_EDGE('',*,*,#14649,.T.);
#21446=ORIENTED_EDGE('',*,*,#14647,.F.);
#21447=ORIENTED_EDGE('',*,*,#14650,.F.);
#21448=ORIENTED_EDGE('',*,*,#14651,.T.);
#21449=ORIENTED_EDGE('',*,*,#14652,.F.);
#21450=ORIENTED_EDGE('',*,*,#14653,.T.);
#21451=ORIENTED_EDGE('',*,*,#14654,.T.);
#21452=ORIENTED_EDGE('',*,*,#14655,.T.);
#21453=ORIENTED_EDGE('',*,*,#14656,.T.);
#21454=ORIENTED_EDGE('',*,*,#14649,.F.);
#21455=ORIENTED_EDGE('',*,*,#14657,.F.);
#21456=ORIENTED_EDGE('',*,*,#14654,.F.);
#21457=ORIENTED_EDGE('',*,*,#14658,.F.);
#21458=ORIENTED_EDGE('',*,*,#14659,.T.);
#21459=ORIENTED_EDGE('',*,*,#14660,.T.);
#21460=ORIENTED_EDGE('',*,*,#14661,.T.);
#21461=ORIENTED_EDGE('',*,*,#14662,.T.);
#21462=ORIENTED_EDGE('',*,*,#14660,.F.);
#21463=ORIENTED_EDGE('',*,*,#14663,.F.);
#21464=ORIENTED_EDGE('',*,*,#14664,.T.);
#21465=ORIENTED_EDGE('',*,*,#14665,.F.);
#21466=ORIENTED_EDGE('',*,*,#14666,.T.);
#21467=ORIENTED_EDGE('',*,*,#14667,.T.);
#21468=ORIENTED_EDGE('',*,*,#14668,.T.);
#21469=ORIENTED_EDGE('',*,*,#14669,.T.);
#21470=ORIENTED_EDGE('',*,*,#14662,.F.);
#21471=ORIENTED_EDGE('',*,*,#14670,.F.);
#21472=ORIENTED_EDGE('',*,*,#14667,.F.);
#21473=ORIENTED_EDGE('',*,*,#14671,.F.);
#21474=ORIENTED_EDGE('',*,*,#14672,.T.);
#21475=ORIENTED_EDGE('',*,*,#14673,.T.);
#21476=ORIENTED_EDGE('',*,*,#14674,.T.);
#21477=ORIENTED_EDGE('',*,*,#14675,.T.);
#21478=ORIENTED_EDGE('',*,*,#14673,.F.);
#21479=ORIENTED_EDGE('',*,*,#14676,.F.);
#21480=ORIENTED_EDGE('',*,*,#14677,.T.);
#21481=ORIENTED_EDGE('',*,*,#14678,.F.);
#21482=ORIENTED_EDGE('',*,*,#14679,.T.);
#21483=ORIENTED_EDGE('',*,*,#14680,.T.);
#21484=ORIENTED_EDGE('',*,*,#14681,.T.);
#21485=ORIENTED_EDGE('',*,*,#14682,.T.);
#21486=ORIENTED_EDGE('',*,*,#14675,.F.);
#21487=ORIENTED_EDGE('',*,*,#14683,.F.);
#21488=ORIENTED_EDGE('',*,*,#14680,.F.);
#21489=ORIENTED_EDGE('',*,*,#14684,.F.);
#21490=ORIENTED_EDGE('',*,*,#14685,.T.);
#21491=ORIENTED_EDGE('',*,*,#14686,.T.);
#21492=ORIENTED_EDGE('',*,*,#14687,.T.);
#21493=ORIENTED_EDGE('',*,*,#14688,.T.);
#21494=ORIENTED_EDGE('',*,*,#14686,.F.);
#21495=ORIENTED_EDGE('',*,*,#14689,.F.);
#21496=ORIENTED_EDGE('',*,*,#14690,.T.);
#21497=ORIENTED_EDGE('',*,*,#14691,.F.);
#21498=ORIENTED_EDGE('',*,*,#14692,.T.);
#21499=ORIENTED_EDGE('',*,*,#14693,.T.);
#21500=ORIENTED_EDGE('',*,*,#14694,.T.);
#21501=ORIENTED_EDGE('',*,*,#14695,.T.);
#21502=ORIENTED_EDGE('',*,*,#14688,.F.);
#21503=ORIENTED_EDGE('',*,*,#14696,.F.);
#21504=ORIENTED_EDGE('',*,*,#14693,.F.);
#21505=ORIENTED_EDGE('',*,*,#14697,.F.);
#21506=ORIENTED_EDGE('',*,*,#14698,.T.);
#21507=ORIENTED_EDGE('',*,*,#14699,.T.);
#21508=ORIENTED_EDGE('',*,*,#14700,.T.);
#21509=ORIENTED_EDGE('',*,*,#14701,.T.);
#21510=ORIENTED_EDGE('',*,*,#14699,.F.);
#21511=ORIENTED_EDGE('',*,*,#14702,.F.);
#21512=ORIENTED_EDGE('',*,*,#14703,.T.);
#21513=ORIENTED_EDGE('',*,*,#14704,.F.);
#21514=ORIENTED_EDGE('',*,*,#14705,.T.);
#21515=ORIENTED_EDGE('',*,*,#14706,.T.);
#21516=ORIENTED_EDGE('',*,*,#14707,.T.);
#21517=ORIENTED_EDGE('',*,*,#14708,.T.);
#21518=ORIENTED_EDGE('',*,*,#14701,.F.);
#21519=ORIENTED_EDGE('',*,*,#14709,.F.);
#21520=ORIENTED_EDGE('',*,*,#14706,.F.);
#21521=ORIENTED_EDGE('',*,*,#14710,.F.);
#21522=ORIENTED_EDGE('',*,*,#14711,.T.);
#21523=ORIENTED_EDGE('',*,*,#14712,.T.);
#21524=ORIENTED_EDGE('',*,*,#14713,.T.);
#21525=ORIENTED_EDGE('',*,*,#14714,.T.);
#21526=ORIENTED_EDGE('',*,*,#14712,.F.);
#21527=ORIENTED_EDGE('',*,*,#14715,.F.);
#21528=ORIENTED_EDGE('',*,*,#14716,.T.);
#21529=ORIENTED_EDGE('',*,*,#14717,.F.);
#21530=ORIENTED_EDGE('',*,*,#14718,.T.);
#21531=ORIENTED_EDGE('',*,*,#14719,.T.);
#21532=ORIENTED_EDGE('',*,*,#14720,.T.);
#21533=ORIENTED_EDGE('',*,*,#14721,.T.);
#21534=ORIENTED_EDGE('',*,*,#14714,.F.);
#21535=ORIENTED_EDGE('',*,*,#14722,.F.);
#21536=ORIENTED_EDGE('',*,*,#14719,.F.);
#21537=ORIENTED_EDGE('',*,*,#14723,.F.);
#21538=ORIENTED_EDGE('',*,*,#14724,.T.);
#21539=ORIENTED_EDGE('',*,*,#14725,.T.);
#21540=ORIENTED_EDGE('',*,*,#14726,.T.);
#21541=ORIENTED_EDGE('',*,*,#14727,.T.);
#21542=ORIENTED_EDGE('',*,*,#14725,.F.);
#21543=ORIENTED_EDGE('',*,*,#14728,.F.);
#21544=ORIENTED_EDGE('',*,*,#14729,.T.);
#21545=ORIENTED_EDGE('',*,*,#14730,.F.);
#21546=ORIENTED_EDGE('',*,*,#14731,.T.);
#21547=ORIENTED_EDGE('',*,*,#14732,.T.);
#21548=ORIENTED_EDGE('',*,*,#14733,.T.);
#21549=ORIENTED_EDGE('',*,*,#14734,.T.);
#21550=ORIENTED_EDGE('',*,*,#14727,.F.);
#21551=ORIENTED_EDGE('',*,*,#14735,.F.);
#21552=ORIENTED_EDGE('',*,*,#14732,.F.);
#21553=ORIENTED_EDGE('',*,*,#14736,.F.);
#21554=ORIENTED_EDGE('',*,*,#14737,.T.);
#21555=ORIENTED_EDGE('',*,*,#14738,.T.);
#21556=ORIENTED_EDGE('',*,*,#14739,.T.);
#21557=ORIENTED_EDGE('',*,*,#14740,.T.);
#21558=ORIENTED_EDGE('',*,*,#14738,.F.);
#21559=ORIENTED_EDGE('',*,*,#14741,.F.);
#21560=ORIENTED_EDGE('',*,*,#14742,.T.);
#21561=ORIENTED_EDGE('',*,*,#14743,.F.);
#21562=ORIENTED_EDGE('',*,*,#14744,.T.);
#21563=ORIENTED_EDGE('',*,*,#14745,.T.);
#21564=ORIENTED_EDGE('',*,*,#14746,.T.);
#21565=ORIENTED_EDGE('',*,*,#14747,.T.);
#21566=ORIENTED_EDGE('',*,*,#14740,.F.);
#21567=ORIENTED_EDGE('',*,*,#14748,.F.);
#21568=ORIENTED_EDGE('',*,*,#14745,.F.);
#21569=ORIENTED_EDGE('',*,*,#14749,.F.);
#21570=ORIENTED_EDGE('',*,*,#14750,.T.);
#21571=ORIENTED_EDGE('',*,*,#14751,.T.);
#21572=ORIENTED_EDGE('',*,*,#14752,.T.);
#21573=ORIENTED_EDGE('',*,*,#14753,.T.);
#21574=ORIENTED_EDGE('',*,*,#14751,.F.);
#21575=ORIENTED_EDGE('',*,*,#14754,.F.);
#21576=ORIENTED_EDGE('',*,*,#14755,.T.);
#21577=ORIENTED_EDGE('',*,*,#14756,.F.);
#21578=ORIENTED_EDGE('',*,*,#14757,.T.);
#21579=ORIENTED_EDGE('',*,*,#14758,.T.);
#21580=ORIENTED_EDGE('',*,*,#14759,.T.);
#21581=ORIENTED_EDGE('',*,*,#14760,.T.);
#21582=ORIENTED_EDGE('',*,*,#14753,.F.);
#21583=ORIENTED_EDGE('',*,*,#14761,.F.);
#21584=ORIENTED_EDGE('',*,*,#14758,.F.);
#21585=ORIENTED_EDGE('',*,*,#14762,.F.);
#21586=ORIENTED_EDGE('',*,*,#14763,.T.);
#21587=ORIENTED_EDGE('',*,*,#14764,.T.);
#21588=ORIENTED_EDGE('',*,*,#14765,.T.);
#21589=ORIENTED_EDGE('',*,*,#14766,.T.);
#21590=ORIENTED_EDGE('',*,*,#14764,.F.);
#21591=ORIENTED_EDGE('',*,*,#14767,.F.);
#21592=ORIENTED_EDGE('',*,*,#14768,.T.);
#21593=ORIENTED_EDGE('',*,*,#14769,.F.);
#21594=ORIENTED_EDGE('',*,*,#14770,.T.);
#21595=ORIENTED_EDGE('',*,*,#14771,.T.);
#21596=ORIENTED_EDGE('',*,*,#14772,.T.);
#21597=ORIENTED_EDGE('',*,*,#14773,.T.);
#21598=ORIENTED_EDGE('',*,*,#14766,.F.);
#21599=ORIENTED_EDGE('',*,*,#14774,.F.);
#21600=ORIENTED_EDGE('',*,*,#14771,.F.);
#21601=ORIENTED_EDGE('',*,*,#14775,.F.);
#21602=ORIENTED_EDGE('',*,*,#14776,.T.);
#21603=ORIENTED_EDGE('',*,*,#14777,.T.);
#21604=ORIENTED_EDGE('',*,*,#14778,.T.);
#21605=ORIENTED_EDGE('',*,*,#14779,.T.);
#21606=ORIENTED_EDGE('',*,*,#14777,.F.);
#21607=ORIENTED_EDGE('',*,*,#14780,.F.);
#21608=ORIENTED_EDGE('',*,*,#14781,.T.);
#21609=ORIENTED_EDGE('',*,*,#14782,.F.);
#21610=ORIENTED_EDGE('',*,*,#14783,.T.);
#21611=ORIENTED_EDGE('',*,*,#14784,.T.);
#21612=ORIENTED_EDGE('',*,*,#14785,.T.);
#21613=ORIENTED_EDGE('',*,*,#14786,.T.);
#21614=ORIENTED_EDGE('',*,*,#14779,.F.);
#21615=ORIENTED_EDGE('',*,*,#14787,.F.);
#21616=ORIENTED_EDGE('',*,*,#14784,.F.);
#21617=ORIENTED_EDGE('',*,*,#14788,.F.);
#21618=ORIENTED_EDGE('',*,*,#14789,.T.);
#21619=ORIENTED_EDGE('',*,*,#14790,.T.);
#21620=ORIENTED_EDGE('',*,*,#14791,.T.);
#21621=ORIENTED_EDGE('',*,*,#14792,.T.);
#21622=ORIENTED_EDGE('',*,*,#14790,.F.);
#21623=ORIENTED_EDGE('',*,*,#14793,.F.);
#21624=ORIENTED_EDGE('',*,*,#14794,.T.);
#21625=ORIENTED_EDGE('',*,*,#14795,.F.);
#21626=ORIENTED_EDGE('',*,*,#14796,.T.);
#21627=ORIENTED_EDGE('',*,*,#14797,.T.);
#21628=ORIENTED_EDGE('',*,*,#14798,.T.);
#21629=ORIENTED_EDGE('',*,*,#14799,.T.);
#21630=ORIENTED_EDGE('',*,*,#14792,.F.);
#21631=ORIENTED_EDGE('',*,*,#14800,.F.);
#21632=ORIENTED_EDGE('',*,*,#14797,.F.);
#21633=ORIENTED_EDGE('',*,*,#14801,.F.);
#21634=ORIENTED_EDGE('',*,*,#14802,.T.);
#21635=ORIENTED_EDGE('',*,*,#14803,.T.);
#21636=ORIENTED_EDGE('',*,*,#14804,.T.);
#21637=ORIENTED_EDGE('',*,*,#14805,.T.);
#21638=ORIENTED_EDGE('',*,*,#14803,.F.);
#21639=ORIENTED_EDGE('',*,*,#14806,.F.);
#21640=ORIENTED_EDGE('',*,*,#14807,.T.);
#21641=ORIENTED_EDGE('',*,*,#14808,.F.);
#21642=ORIENTED_EDGE('',*,*,#14809,.T.);
#21643=ORIENTED_EDGE('',*,*,#14810,.T.);
#21644=ORIENTED_EDGE('',*,*,#14811,.T.);
#21645=ORIENTED_EDGE('',*,*,#14812,.T.);
#21646=ORIENTED_EDGE('',*,*,#14805,.F.);
#21647=ORIENTED_EDGE('',*,*,#14813,.F.);
#21648=ORIENTED_EDGE('',*,*,#14810,.F.);
#21649=ORIENTED_EDGE('',*,*,#14814,.F.);
#21650=ORIENTED_EDGE('',*,*,#14815,.T.);
#21651=ORIENTED_EDGE('',*,*,#14816,.T.);
#21652=ORIENTED_EDGE('',*,*,#14817,.T.);
#21653=ORIENTED_EDGE('',*,*,#14818,.T.);
#21654=ORIENTED_EDGE('',*,*,#14816,.F.);
#21655=ORIENTED_EDGE('',*,*,#14819,.F.);
#21656=ORIENTED_EDGE('',*,*,#14820,.T.);
#21657=ORIENTED_EDGE('',*,*,#14821,.F.);
#21658=ORIENTED_EDGE('',*,*,#14822,.T.);
#21659=ORIENTED_EDGE('',*,*,#14823,.T.);
#21660=ORIENTED_EDGE('',*,*,#14824,.T.);
#21661=ORIENTED_EDGE('',*,*,#14825,.T.);
#21662=ORIENTED_EDGE('',*,*,#14818,.F.);
#21663=ORIENTED_EDGE('',*,*,#14826,.F.);
#21664=ORIENTED_EDGE('',*,*,#14823,.F.);
#21665=ORIENTED_EDGE('',*,*,#14827,.F.);
#21666=ORIENTED_EDGE('',*,*,#14828,.T.);
#21667=ORIENTED_EDGE('',*,*,#14829,.T.);
#21668=ORIENTED_EDGE('',*,*,#14830,.T.);
#21669=ORIENTED_EDGE('',*,*,#14831,.T.);
#21670=ORIENTED_EDGE('',*,*,#14829,.F.);
#21671=ORIENTED_EDGE('',*,*,#14832,.F.);
#21672=ORIENTED_EDGE('',*,*,#14833,.T.);
#21673=ORIENTED_EDGE('',*,*,#14834,.F.);
#21674=ORIENTED_EDGE('',*,*,#14835,.T.);
#21675=ORIENTED_EDGE('',*,*,#14836,.T.);
#21676=ORIENTED_EDGE('',*,*,#14837,.T.);
#21677=ORIENTED_EDGE('',*,*,#14838,.T.);
#21678=ORIENTED_EDGE('',*,*,#14831,.F.);
#21679=ORIENTED_EDGE('',*,*,#14839,.F.);
#21680=ORIENTED_EDGE('',*,*,#14836,.F.);
#21681=ORIENTED_EDGE('',*,*,#14840,.F.);
#21682=ORIENTED_EDGE('',*,*,#14552,.F.);
#21683=ORIENTED_EDGE('',*,*,#14841,.F.);
#21684=ORIENTED_EDGE('',*,*,#14842,.F.);
#21685=ORIENTED_EDGE('',*,*,#14843,.F.);
#21686=ORIENTED_EDGE('',*,*,#14844,.F.);
#21687=ORIENTED_EDGE('',*,*,#14845,.F.);
#21688=ORIENTED_EDGE('',*,*,#14846,.F.);
#21689=ORIENTED_EDGE('',*,*,#14547,.F.);
#21690=ORIENTED_EDGE('',*,*,#14847,.F.);
#21691=ORIENTED_EDGE('',*,*,#14842,.T.);
#21692=ORIENTED_EDGE('',*,*,#14848,.F.);
#21693=ORIENTED_EDGE('',*,*,#14849,.F.);
#21694=ORIENTED_EDGE('',*,*,#14565,.F.);
#21695=ORIENTED_EDGE('',*,*,#14850,.F.);
#21696=ORIENTED_EDGE('',*,*,#14851,.F.);
#21697=ORIENTED_EDGE('',*,*,#14852,.F.);
#21698=ORIENTED_EDGE('',*,*,#14853,.F.);
#21699=ORIENTED_EDGE('',*,*,#14854,.F.);
#21700=ORIENTED_EDGE('',*,*,#14855,.F.);
#21701=ORIENTED_EDGE('',*,*,#14560,.F.);
#21702=ORIENTED_EDGE('',*,*,#14856,.F.);
#21703=ORIENTED_EDGE('',*,*,#14851,.T.);
#21704=ORIENTED_EDGE('',*,*,#14857,.F.);
#21705=ORIENTED_EDGE('',*,*,#14858,.F.);
#21706=ORIENTED_EDGE('',*,*,#14578,.F.);
#21707=ORIENTED_EDGE('',*,*,#14859,.F.);
#21708=ORIENTED_EDGE('',*,*,#14860,.F.);
#21709=ORIENTED_EDGE('',*,*,#14861,.F.);
#21710=ORIENTED_EDGE('',*,*,#14862,.F.);
#21711=ORIENTED_EDGE('',*,*,#14863,.F.);
#21712=ORIENTED_EDGE('',*,*,#14864,.F.);
#21713=ORIENTED_EDGE('',*,*,#14573,.F.);
#21714=ORIENTED_EDGE('',*,*,#14865,.F.);
#21715=ORIENTED_EDGE('',*,*,#14860,.T.);
#21716=ORIENTED_EDGE('',*,*,#14866,.F.);
#21717=ORIENTED_EDGE('',*,*,#14867,.F.);
#21718=ORIENTED_EDGE('',*,*,#14591,.F.);
#21719=ORIENTED_EDGE('',*,*,#14868,.F.);
#21720=ORIENTED_EDGE('',*,*,#14869,.F.);
#21721=ORIENTED_EDGE('',*,*,#14870,.F.);
#21722=ORIENTED_EDGE('',*,*,#14871,.F.);
#21723=ORIENTED_EDGE('',*,*,#14872,.F.);
#21724=ORIENTED_EDGE('',*,*,#14873,.F.);
#21725=ORIENTED_EDGE('',*,*,#14586,.F.);
#21726=ORIENTED_EDGE('',*,*,#14874,.F.);
#21727=ORIENTED_EDGE('',*,*,#14869,.T.);
#21728=ORIENTED_EDGE('',*,*,#14875,.F.);
#21729=ORIENTED_EDGE('',*,*,#14876,.F.);
#21730=ORIENTED_EDGE('',*,*,#14604,.F.);
#21731=ORIENTED_EDGE('',*,*,#14877,.F.);
#21732=ORIENTED_EDGE('',*,*,#14878,.F.);
#21733=ORIENTED_EDGE('',*,*,#14879,.F.);
#21734=ORIENTED_EDGE('',*,*,#14880,.F.);
#21735=ORIENTED_EDGE('',*,*,#14881,.F.);
#21736=ORIENTED_EDGE('',*,*,#14882,.F.);
#21737=ORIENTED_EDGE('',*,*,#14599,.F.);
#21738=ORIENTED_EDGE('',*,*,#14883,.F.);
#21739=ORIENTED_EDGE('',*,*,#14878,.T.);
#21740=ORIENTED_EDGE('',*,*,#14884,.F.);
#21741=ORIENTED_EDGE('',*,*,#14885,.F.);
#21742=ORIENTED_EDGE('',*,*,#14617,.F.);
#21743=ORIENTED_EDGE('',*,*,#14886,.F.);
#21744=ORIENTED_EDGE('',*,*,#14887,.F.);
#21745=ORIENTED_EDGE('',*,*,#14888,.F.);
#21746=ORIENTED_EDGE('',*,*,#14889,.F.);
#21747=ORIENTED_EDGE('',*,*,#14890,.F.);
#21748=ORIENTED_EDGE('',*,*,#14891,.F.);
#21749=ORIENTED_EDGE('',*,*,#14612,.F.);
#21750=ORIENTED_EDGE('',*,*,#14892,.F.);
#21751=ORIENTED_EDGE('',*,*,#14887,.T.);
#21752=ORIENTED_EDGE('',*,*,#14893,.F.);
#21753=ORIENTED_EDGE('',*,*,#14894,.F.);
#21754=ORIENTED_EDGE('',*,*,#14630,.F.);
#21755=ORIENTED_EDGE('',*,*,#14895,.F.);
#21756=ORIENTED_EDGE('',*,*,#14896,.F.);
#21757=ORIENTED_EDGE('',*,*,#14897,.F.);
#21758=ORIENTED_EDGE('',*,*,#14898,.F.);
#21759=ORIENTED_EDGE('',*,*,#14899,.F.);
#21760=ORIENTED_EDGE('',*,*,#14900,.F.);
#21761=ORIENTED_EDGE('',*,*,#14625,.F.);
#21762=ORIENTED_EDGE('',*,*,#14901,.F.);
#21763=ORIENTED_EDGE('',*,*,#14896,.T.);
#21764=ORIENTED_EDGE('',*,*,#14902,.F.);
#21765=ORIENTED_EDGE('',*,*,#14903,.F.);
#21766=ORIENTED_EDGE('',*,*,#14643,.F.);
#21767=ORIENTED_EDGE('',*,*,#14904,.F.);
#21768=ORIENTED_EDGE('',*,*,#14905,.F.);
#21769=ORIENTED_EDGE('',*,*,#14906,.F.);
#21770=ORIENTED_EDGE('',*,*,#14907,.F.);
#21771=ORIENTED_EDGE('',*,*,#14908,.F.);
#21772=ORIENTED_EDGE('',*,*,#14909,.F.);
#21773=ORIENTED_EDGE('',*,*,#14638,.F.);
#21774=ORIENTED_EDGE('',*,*,#14910,.F.);
#21775=ORIENTED_EDGE('',*,*,#14905,.T.);
#21776=ORIENTED_EDGE('',*,*,#14911,.F.);
#21777=ORIENTED_EDGE('',*,*,#14912,.F.);
#21778=ORIENTED_EDGE('',*,*,#14656,.F.);
#21779=ORIENTED_EDGE('',*,*,#14913,.F.);
#21780=ORIENTED_EDGE('',*,*,#14914,.F.);
#21781=ORIENTED_EDGE('',*,*,#14915,.F.);
#21782=ORIENTED_EDGE('',*,*,#14916,.F.);
#21783=ORIENTED_EDGE('',*,*,#14917,.F.);
#21784=ORIENTED_EDGE('',*,*,#14918,.F.);
#21785=ORIENTED_EDGE('',*,*,#14651,.F.);
#21786=ORIENTED_EDGE('',*,*,#14919,.F.);
#21787=ORIENTED_EDGE('',*,*,#14914,.T.);
#21788=ORIENTED_EDGE('',*,*,#14920,.F.);
#21789=ORIENTED_EDGE('',*,*,#14921,.F.);
#21790=ORIENTED_EDGE('',*,*,#14669,.F.);
#21791=ORIENTED_EDGE('',*,*,#14922,.F.);
#21792=ORIENTED_EDGE('',*,*,#14923,.F.);
#21793=ORIENTED_EDGE('',*,*,#14924,.F.);
#21794=ORIENTED_EDGE('',*,*,#14925,.F.);
#21795=ORIENTED_EDGE('',*,*,#14926,.F.);
#21796=ORIENTED_EDGE('',*,*,#14927,.F.);
#21797=ORIENTED_EDGE('',*,*,#14664,.F.);
#21798=ORIENTED_EDGE('',*,*,#14928,.F.);
#21799=ORIENTED_EDGE('',*,*,#14923,.T.);
#21800=ORIENTED_EDGE('',*,*,#14929,.F.);
#21801=ORIENTED_EDGE('',*,*,#14930,.F.);
#21802=ORIENTED_EDGE('',*,*,#14682,.F.);
#21803=ORIENTED_EDGE('',*,*,#14931,.F.);
#21804=ORIENTED_EDGE('',*,*,#14932,.F.);
#21805=ORIENTED_EDGE('',*,*,#14933,.F.);
#21806=ORIENTED_EDGE('',*,*,#14934,.F.);
#21807=ORIENTED_EDGE('',*,*,#14935,.F.);
#21808=ORIENTED_EDGE('',*,*,#14936,.F.);
#21809=ORIENTED_EDGE('',*,*,#14677,.F.);
#21810=ORIENTED_EDGE('',*,*,#14937,.F.);
#21811=ORIENTED_EDGE('',*,*,#14932,.T.);
#21812=ORIENTED_EDGE('',*,*,#14938,.F.);
#21813=ORIENTED_EDGE('',*,*,#14939,.F.);
#21814=ORIENTED_EDGE('',*,*,#14695,.F.);
#21815=ORIENTED_EDGE('',*,*,#14940,.F.);
#21816=ORIENTED_EDGE('',*,*,#14941,.F.);
#21817=ORIENTED_EDGE('',*,*,#14942,.F.);
#21818=ORIENTED_EDGE('',*,*,#14943,.F.);
#21819=ORIENTED_EDGE('',*,*,#14944,.F.);
#21820=ORIENTED_EDGE('',*,*,#14945,.F.);
#21821=ORIENTED_EDGE('',*,*,#14690,.F.);
#21822=ORIENTED_EDGE('',*,*,#14946,.F.);
#21823=ORIENTED_EDGE('',*,*,#14941,.T.);
#21824=ORIENTED_EDGE('',*,*,#14947,.F.);
#21825=ORIENTED_EDGE('',*,*,#14948,.F.);
#21826=ORIENTED_EDGE('',*,*,#14708,.F.);
#21827=ORIENTED_EDGE('',*,*,#14949,.F.);
#21828=ORIENTED_EDGE('',*,*,#14950,.F.);
#21829=ORIENTED_EDGE('',*,*,#14951,.F.);
#21830=ORIENTED_EDGE('',*,*,#14952,.F.);
#21831=ORIENTED_EDGE('',*,*,#14953,.F.);
#21832=ORIENTED_EDGE('',*,*,#14954,.F.);
#21833=ORIENTED_EDGE('',*,*,#14703,.F.);
#21834=ORIENTED_EDGE('',*,*,#14955,.F.);
#21835=ORIENTED_EDGE('',*,*,#14950,.T.);
#21836=ORIENTED_EDGE('',*,*,#14956,.F.);
#21837=ORIENTED_EDGE('',*,*,#14957,.F.);
#21838=ORIENTED_EDGE('',*,*,#14721,.F.);
#21839=ORIENTED_EDGE('',*,*,#14958,.F.);
#21840=ORIENTED_EDGE('',*,*,#14959,.F.);
#21841=ORIENTED_EDGE('',*,*,#14960,.F.);
#21842=ORIENTED_EDGE('',*,*,#14961,.F.);
#21843=ORIENTED_EDGE('',*,*,#14962,.F.);
#21844=ORIENTED_EDGE('',*,*,#14963,.F.);
#21845=ORIENTED_EDGE('',*,*,#14716,.F.);
#21846=ORIENTED_EDGE('',*,*,#14964,.F.);
#21847=ORIENTED_EDGE('',*,*,#14959,.T.);
#21848=ORIENTED_EDGE('',*,*,#14965,.F.);
#21849=ORIENTED_EDGE('',*,*,#14966,.F.);
#21850=ORIENTED_EDGE('',*,*,#14734,.F.);
#21851=ORIENTED_EDGE('',*,*,#14967,.F.);
#21852=ORIENTED_EDGE('',*,*,#14968,.F.);
#21853=ORIENTED_EDGE('',*,*,#14969,.F.);
#21854=ORIENTED_EDGE('',*,*,#14970,.F.);
#21855=ORIENTED_EDGE('',*,*,#14971,.F.);
#21856=ORIENTED_EDGE('',*,*,#14972,.F.);
#21857=ORIENTED_EDGE('',*,*,#14729,.F.);
#21858=ORIENTED_EDGE('',*,*,#14973,.F.);
#21859=ORIENTED_EDGE('',*,*,#14968,.T.);
#21860=ORIENTED_EDGE('',*,*,#14974,.F.);
#21861=ORIENTED_EDGE('',*,*,#14975,.F.);
#21862=ORIENTED_EDGE('',*,*,#14747,.F.);
#21863=ORIENTED_EDGE('',*,*,#14976,.F.);
#21864=ORIENTED_EDGE('',*,*,#14977,.F.);
#21865=ORIENTED_EDGE('',*,*,#14978,.F.);
#21866=ORIENTED_EDGE('',*,*,#14979,.F.);
#21867=ORIENTED_EDGE('',*,*,#14980,.F.);
#21868=ORIENTED_EDGE('',*,*,#14981,.F.);
#21869=ORIENTED_EDGE('',*,*,#14742,.F.);
#21870=ORIENTED_EDGE('',*,*,#14982,.F.);
#21871=ORIENTED_EDGE('',*,*,#14977,.T.);
#21872=ORIENTED_EDGE('',*,*,#14983,.F.);
#21873=ORIENTED_EDGE('',*,*,#14984,.F.);
#21874=ORIENTED_EDGE('',*,*,#14760,.F.);
#21875=ORIENTED_EDGE('',*,*,#14985,.F.);
#21876=ORIENTED_EDGE('',*,*,#14986,.F.);
#21877=ORIENTED_EDGE('',*,*,#14987,.F.);
#21878=ORIENTED_EDGE('',*,*,#14988,.F.);
#21879=ORIENTED_EDGE('',*,*,#14989,.F.);
#21880=ORIENTED_EDGE('',*,*,#14990,.F.);
#21881=ORIENTED_EDGE('',*,*,#14755,.F.);
#21882=ORIENTED_EDGE('',*,*,#14991,.F.);
#21883=ORIENTED_EDGE('',*,*,#14986,.T.);
#21884=ORIENTED_EDGE('',*,*,#14992,.F.);
#21885=ORIENTED_EDGE('',*,*,#14993,.F.);
#21886=ORIENTED_EDGE('',*,*,#14773,.F.);
#21887=ORIENTED_EDGE('',*,*,#14994,.F.);
#21888=ORIENTED_EDGE('',*,*,#14995,.F.);
#21889=ORIENTED_EDGE('',*,*,#14996,.F.);
#21890=ORIENTED_EDGE('',*,*,#14997,.F.);
#21891=ORIENTED_EDGE('',*,*,#14998,.F.);
#21892=ORIENTED_EDGE('',*,*,#14999,.F.);
#21893=ORIENTED_EDGE('',*,*,#14768,.F.);
#21894=ORIENTED_EDGE('',*,*,#15000,.F.);
#21895=ORIENTED_EDGE('',*,*,#14995,.T.);
#21896=ORIENTED_EDGE('',*,*,#15001,.F.);
#21897=ORIENTED_EDGE('',*,*,#15002,.F.);
#21898=ORIENTED_EDGE('',*,*,#14786,.F.);
#21899=ORIENTED_EDGE('',*,*,#15003,.F.);
#21900=ORIENTED_EDGE('',*,*,#15004,.F.);
#21901=ORIENTED_EDGE('',*,*,#15005,.F.);
#21902=ORIENTED_EDGE('',*,*,#15006,.F.);
#21903=ORIENTED_EDGE('',*,*,#15007,.F.);
#21904=ORIENTED_EDGE('',*,*,#15008,.F.);
#21905=ORIENTED_EDGE('',*,*,#14781,.F.);
#21906=ORIENTED_EDGE('',*,*,#15009,.F.);
#21907=ORIENTED_EDGE('',*,*,#15004,.T.);
#21908=ORIENTED_EDGE('',*,*,#15010,.F.);
#21909=ORIENTED_EDGE('',*,*,#15011,.F.);
#21910=ORIENTED_EDGE('',*,*,#14799,.F.);
#21911=ORIENTED_EDGE('',*,*,#15012,.F.);
#21912=ORIENTED_EDGE('',*,*,#15013,.F.);
#21913=ORIENTED_EDGE('',*,*,#15014,.F.);
#21914=ORIENTED_EDGE('',*,*,#15015,.F.);
#21915=ORIENTED_EDGE('',*,*,#15016,.F.);
#21916=ORIENTED_EDGE('',*,*,#15017,.F.);
#21917=ORIENTED_EDGE('',*,*,#14794,.F.);
#21918=ORIENTED_EDGE('',*,*,#15018,.F.);
#21919=ORIENTED_EDGE('',*,*,#15013,.T.);
#21920=ORIENTED_EDGE('',*,*,#15019,.F.);
#21921=ORIENTED_EDGE('',*,*,#15020,.F.);
#21922=ORIENTED_EDGE('',*,*,#14812,.F.);
#21923=ORIENTED_EDGE('',*,*,#15021,.F.);
#21924=ORIENTED_EDGE('',*,*,#15022,.F.);
#21925=ORIENTED_EDGE('',*,*,#15023,.F.);
#21926=ORIENTED_EDGE('',*,*,#15024,.F.);
#21927=ORIENTED_EDGE('',*,*,#15025,.F.);
#21928=ORIENTED_EDGE('',*,*,#15026,.F.);
#21929=ORIENTED_EDGE('',*,*,#14807,.F.);
#21930=ORIENTED_EDGE('',*,*,#15027,.F.);
#21931=ORIENTED_EDGE('',*,*,#15022,.T.);
#21932=ORIENTED_EDGE('',*,*,#15028,.F.);
#21933=ORIENTED_EDGE('',*,*,#15029,.F.);
#21934=ORIENTED_EDGE('',*,*,#14825,.F.);
#21935=ORIENTED_EDGE('',*,*,#15030,.F.);
#21936=ORIENTED_EDGE('',*,*,#15031,.F.);
#21937=ORIENTED_EDGE('',*,*,#15032,.F.);
#21938=ORIENTED_EDGE('',*,*,#15033,.F.);
#21939=ORIENTED_EDGE('',*,*,#15034,.F.);
#21940=ORIENTED_EDGE('',*,*,#15035,.F.);
#21941=ORIENTED_EDGE('',*,*,#14820,.F.);
#21942=ORIENTED_EDGE('',*,*,#15036,.F.);
#21943=ORIENTED_EDGE('',*,*,#15031,.T.);
#21944=ORIENTED_EDGE('',*,*,#15037,.F.);
#21945=ORIENTED_EDGE('',*,*,#15038,.F.);
#21946=ORIENTED_EDGE('',*,*,#14838,.F.);
#21947=ORIENTED_EDGE('',*,*,#15039,.F.);
#21948=ORIENTED_EDGE('',*,*,#15040,.F.);
#21949=ORIENTED_EDGE('',*,*,#15041,.F.);
#21950=ORIENTED_EDGE('',*,*,#15042,.F.);
#21951=ORIENTED_EDGE('',*,*,#15043,.F.);
#21952=ORIENTED_EDGE('',*,*,#15044,.F.);
#21953=ORIENTED_EDGE('',*,*,#14833,.F.);
#21954=ORIENTED_EDGE('',*,*,#15045,.F.);
#21955=ORIENTED_EDGE('',*,*,#15040,.T.);
#21956=ORIENTED_EDGE('',*,*,#15046,.F.);
#21957=ORIENTED_EDGE('',*,*,#15047,.F.);
#21958=ORIENTED_EDGE('',*,*,#14844,.T.);
#21959=ORIENTED_EDGE('',*,*,#14546,.T.);
#21960=ORIENTED_EDGE('',*,*,#14542,.F.);
#21961=ORIENTED_EDGE('',*,*,#14554,.T.);
#21962=ORIENTED_EDGE('',*,*,#14549,.F.);
#21963=ORIENTED_EDGE('',*,*,#14843,.T.);
#21964=ORIENTED_EDGE('',*,*,#14847,.T.);
#21965=ORIENTED_EDGE('',*,*,#15048,.F.);
#21966=ORIENTED_EDGE('',*,*,#14853,.T.);
#21967=ORIENTED_EDGE('',*,*,#14559,.T.);
#21968=ORIENTED_EDGE('',*,*,#14555,.F.);
#21969=ORIENTED_EDGE('',*,*,#14567,.T.);
#21970=ORIENTED_EDGE('',*,*,#14562,.F.);
#21971=ORIENTED_EDGE('',*,*,#14852,.T.);
#21972=ORIENTED_EDGE('',*,*,#14856,.T.);
#21973=ORIENTED_EDGE('',*,*,#15049,.F.);
#21974=ORIENTED_EDGE('',*,*,#14862,.T.);
#21975=ORIENTED_EDGE('',*,*,#14572,.T.);
#21976=ORIENTED_EDGE('',*,*,#14568,.F.);
#21977=ORIENTED_EDGE('',*,*,#14580,.T.);
#21978=ORIENTED_EDGE('',*,*,#14575,.F.);
#21979=ORIENTED_EDGE('',*,*,#14861,.T.);
#21980=ORIENTED_EDGE('',*,*,#14865,.T.);
#21981=ORIENTED_EDGE('',*,*,#15050,.F.);
#21982=ORIENTED_EDGE('',*,*,#14871,.T.);
#21983=ORIENTED_EDGE('',*,*,#14585,.T.);
#21984=ORIENTED_EDGE('',*,*,#14581,.F.);
#21985=ORIENTED_EDGE('',*,*,#14593,.T.);
#21986=ORIENTED_EDGE('',*,*,#14588,.F.);
#21987=ORIENTED_EDGE('',*,*,#14870,.T.);
#21988=ORIENTED_EDGE('',*,*,#14874,.T.);
#21989=ORIENTED_EDGE('',*,*,#15051,.F.);
#21990=ORIENTED_EDGE('',*,*,#14880,.T.);
#21991=ORIENTED_EDGE('',*,*,#14598,.T.);
#21992=ORIENTED_EDGE('',*,*,#14594,.F.);
#21993=ORIENTED_EDGE('',*,*,#14606,.T.);
#21994=ORIENTED_EDGE('',*,*,#14601,.F.);
#21995=ORIENTED_EDGE('',*,*,#14879,.T.);
#21996=ORIENTED_EDGE('',*,*,#14883,.T.);
#21997=ORIENTED_EDGE('',*,*,#15052,.F.);
#21998=ORIENTED_EDGE('',*,*,#14889,.T.);
#21999=ORIENTED_EDGE('',*,*,#14611,.T.);
#22000=ORIENTED_EDGE('',*,*,#14607,.F.);
#22001=ORIENTED_EDGE('',*,*,#14619,.T.);
#22002=ORIENTED_EDGE('',*,*,#14614,.F.);
#22003=ORIENTED_EDGE('',*,*,#14888,.T.);
#22004=ORIENTED_EDGE('',*,*,#14892,.T.);
#22005=ORIENTED_EDGE('',*,*,#15053,.F.);
#22006=ORIENTED_EDGE('',*,*,#14898,.T.);
#22007=ORIENTED_EDGE('',*,*,#14624,.T.);
#22008=ORIENTED_EDGE('',*,*,#14620,.F.);
#22009=ORIENTED_EDGE('',*,*,#14632,.T.);
#22010=ORIENTED_EDGE('',*,*,#14627,.F.);
#22011=ORIENTED_EDGE('',*,*,#14897,.T.);
#22012=ORIENTED_EDGE('',*,*,#14901,.T.);
#22013=ORIENTED_EDGE('',*,*,#15054,.F.);
#22014=ORIENTED_EDGE('',*,*,#14907,.T.);
#22015=ORIENTED_EDGE('',*,*,#14637,.T.);
#22016=ORIENTED_EDGE('',*,*,#14633,.F.);
#22017=ORIENTED_EDGE('',*,*,#14645,.T.);
#22018=ORIENTED_EDGE('',*,*,#14640,.F.);
#22019=ORIENTED_EDGE('',*,*,#14906,.T.);
#22020=ORIENTED_EDGE('',*,*,#14910,.T.);
#22021=ORIENTED_EDGE('',*,*,#15055,.F.);
#22022=ORIENTED_EDGE('',*,*,#14916,.T.);
#22023=ORIENTED_EDGE('',*,*,#14650,.T.);
#22024=ORIENTED_EDGE('',*,*,#14646,.F.);
#22025=ORIENTED_EDGE('',*,*,#14658,.T.);
#22026=ORIENTED_EDGE('',*,*,#14653,.F.);
#22027=ORIENTED_EDGE('',*,*,#14915,.T.);
#22028=ORIENTED_EDGE('',*,*,#14919,.T.);
#22029=ORIENTED_EDGE('',*,*,#15056,.F.);
#22030=ORIENTED_EDGE('',*,*,#14925,.T.);
#22031=ORIENTED_EDGE('',*,*,#14663,.T.);
#22032=ORIENTED_EDGE('',*,*,#14659,.F.);
#22033=ORIENTED_EDGE('',*,*,#14671,.T.);
#22034=ORIENTED_EDGE('',*,*,#14666,.F.);
#22035=ORIENTED_EDGE('',*,*,#14924,.T.);
#22036=ORIENTED_EDGE('',*,*,#14928,.T.);
#22037=ORIENTED_EDGE('',*,*,#15057,.F.);
#22038=ORIENTED_EDGE('',*,*,#14934,.T.);
#22039=ORIENTED_EDGE('',*,*,#14676,.T.);
#22040=ORIENTED_EDGE('',*,*,#14672,.F.);
#22041=ORIENTED_EDGE('',*,*,#14684,.T.);
#22042=ORIENTED_EDGE('',*,*,#14679,.F.);
#22043=ORIENTED_EDGE('',*,*,#14933,.T.);
#22044=ORIENTED_EDGE('',*,*,#14937,.T.);
#22045=ORIENTED_EDGE('',*,*,#15058,.F.);
#22046=ORIENTED_EDGE('',*,*,#14943,.T.);
#22047=ORIENTED_EDGE('',*,*,#14689,.T.);
#22048=ORIENTED_EDGE('',*,*,#14685,.F.);
#22049=ORIENTED_EDGE('',*,*,#14697,.T.);
#22050=ORIENTED_EDGE('',*,*,#14692,.F.);
#22051=ORIENTED_EDGE('',*,*,#14942,.T.);
#22052=ORIENTED_EDGE('',*,*,#14946,.T.);
#22053=ORIENTED_EDGE('',*,*,#15059,.F.);
#22054=ORIENTED_EDGE('',*,*,#14952,.T.);
#22055=ORIENTED_EDGE('',*,*,#14702,.T.);
#22056=ORIENTED_EDGE('',*,*,#14698,.F.);
#22057=ORIENTED_EDGE('',*,*,#14710,.T.);
#22058=ORIENTED_EDGE('',*,*,#14705,.F.);
#22059=ORIENTED_EDGE('',*,*,#14951,.T.);
#22060=ORIENTED_EDGE('',*,*,#14955,.T.);
#22061=ORIENTED_EDGE('',*,*,#15060,.F.);
#22062=ORIENTED_EDGE('',*,*,#14961,.T.);
#22063=ORIENTED_EDGE('',*,*,#14715,.T.);
#22064=ORIENTED_EDGE('',*,*,#14711,.F.);
#22065=ORIENTED_EDGE('',*,*,#14723,.T.);
#22066=ORIENTED_EDGE('',*,*,#14718,.F.);
#22067=ORIENTED_EDGE('',*,*,#14960,.T.);
#22068=ORIENTED_EDGE('',*,*,#14964,.T.);
#22069=ORIENTED_EDGE('',*,*,#15061,.F.);
#22070=ORIENTED_EDGE('',*,*,#14970,.T.);
#22071=ORIENTED_EDGE('',*,*,#14728,.T.);
#22072=ORIENTED_EDGE('',*,*,#14724,.F.);
#22073=ORIENTED_EDGE('',*,*,#14736,.T.);
#22074=ORIENTED_EDGE('',*,*,#14731,.F.);
#22075=ORIENTED_EDGE('',*,*,#14969,.T.);
#22076=ORIENTED_EDGE('',*,*,#14973,.T.);
#22077=ORIENTED_EDGE('',*,*,#15062,.F.);
#22078=ORIENTED_EDGE('',*,*,#14979,.T.);
#22079=ORIENTED_EDGE('',*,*,#14741,.T.);
#22080=ORIENTED_EDGE('',*,*,#14737,.F.);
#22081=ORIENTED_EDGE('',*,*,#14749,.T.);
#22082=ORIENTED_EDGE('',*,*,#14744,.F.);
#22083=ORIENTED_EDGE('',*,*,#14978,.T.);
#22084=ORIENTED_EDGE('',*,*,#14982,.T.);
#22085=ORIENTED_EDGE('',*,*,#15063,.F.);
#22086=ORIENTED_EDGE('',*,*,#14988,.T.);
#22087=ORIENTED_EDGE('',*,*,#14754,.T.);
#22088=ORIENTED_EDGE('',*,*,#14750,.F.);
#22089=ORIENTED_EDGE('',*,*,#14762,.T.);
#22090=ORIENTED_EDGE('',*,*,#14757,.F.);
#22091=ORIENTED_EDGE('',*,*,#14987,.T.);
#22092=ORIENTED_EDGE('',*,*,#14991,.T.);
#22093=ORIENTED_EDGE('',*,*,#15064,.F.);
#22094=ORIENTED_EDGE('',*,*,#14997,.T.);
#22095=ORIENTED_EDGE('',*,*,#14767,.T.);
#22096=ORIENTED_EDGE('',*,*,#14763,.F.);
#22097=ORIENTED_EDGE('',*,*,#14775,.T.);
#22098=ORIENTED_EDGE('',*,*,#14770,.F.);
#22099=ORIENTED_EDGE('',*,*,#14996,.T.);
#22100=ORIENTED_EDGE('',*,*,#15000,.T.);
#22101=ORIENTED_EDGE('',*,*,#15065,.F.);
#22102=ORIENTED_EDGE('',*,*,#15006,.T.);
#22103=ORIENTED_EDGE('',*,*,#14780,.T.);
#22104=ORIENTED_EDGE('',*,*,#14776,.F.);
#22105=ORIENTED_EDGE('',*,*,#14788,.T.);
#22106=ORIENTED_EDGE('',*,*,#14783,.F.);
#22107=ORIENTED_EDGE('',*,*,#15005,.T.);
#22108=ORIENTED_EDGE('',*,*,#15009,.T.);
#22109=ORIENTED_EDGE('',*,*,#15066,.F.);
#22110=ORIENTED_EDGE('',*,*,#15015,.T.);
#22111=ORIENTED_EDGE('',*,*,#14793,.T.);
#22112=ORIENTED_EDGE('',*,*,#14789,.F.);
#22113=ORIENTED_EDGE('',*,*,#14801,.T.);
#22114=ORIENTED_EDGE('',*,*,#14796,.F.);
#22115=ORIENTED_EDGE('',*,*,#15014,.T.);
#22116=ORIENTED_EDGE('',*,*,#15018,.T.);
#22117=ORIENTED_EDGE('',*,*,#15067,.F.);
#22118=ORIENTED_EDGE('',*,*,#15024,.T.);
#22119=ORIENTED_EDGE('',*,*,#14806,.T.);
#22120=ORIENTED_EDGE('',*,*,#14802,.F.);
#22121=ORIENTED_EDGE('',*,*,#14814,.T.);
#22122=ORIENTED_EDGE('',*,*,#14809,.F.);
#22123=ORIENTED_EDGE('',*,*,#15023,.T.);
#22124=ORIENTED_EDGE('',*,*,#15027,.T.);
#22125=ORIENTED_EDGE('',*,*,#15068,.F.);
#22126=ORIENTED_EDGE('',*,*,#15033,.T.);
#22127=ORIENTED_EDGE('',*,*,#14819,.T.);
#22128=ORIENTED_EDGE('',*,*,#14815,.F.);
#22129=ORIENTED_EDGE('',*,*,#14827,.T.);
#22130=ORIENTED_EDGE('',*,*,#14822,.F.);
#22131=ORIENTED_EDGE('',*,*,#15032,.T.);
#22132=ORIENTED_EDGE('',*,*,#15036,.T.);
#22133=ORIENTED_EDGE('',*,*,#15069,.F.);
#22134=ORIENTED_EDGE('',*,*,#15042,.T.);
#22135=ORIENTED_EDGE('',*,*,#14832,.T.);
#22136=ORIENTED_EDGE('',*,*,#14828,.F.);
#22137=ORIENTED_EDGE('',*,*,#14840,.T.);
#22138=ORIENTED_EDGE('',*,*,#14835,.F.);
#22139=ORIENTED_EDGE('',*,*,#15041,.T.);
#22140=ORIENTED_EDGE('',*,*,#15045,.T.);
#22141=ORIENTED_EDGE('',*,*,#15070,.F.);
#22142=ORIENTED_EDGE('',*,*,#15071,.T.);
#22143=ORIENTED_EDGE('',*,*,#15072,.T.);
#22144=ORIENTED_EDGE('',*,*,#15073,.F.);
#22145=ORIENTED_EDGE('',*,*,#15074,.T.);
#22146=ORIENTED_EDGE('',*,*,#15075,.F.);
#22147=ORIENTED_EDGE('',*,*,#15076,.T.);
#22148=ORIENTED_EDGE('',*,*,#15077,.T.);
#22149=ORIENTED_EDGE('',*,*,#15078,.F.);
#22150=ORIENTED_EDGE('',*,*,#15079,.F.);
#22151=ORIENTED_EDGE('',*,*,#14846,.T.);
#22152=ORIENTED_EDGE('',*,*,#15080,.T.);
#22153=ORIENTED_EDGE('',*,*,#15081,.T.);
#22154=ORIENTED_EDGE('',*,*,#15082,.T.);
#22155=ORIENTED_EDGE('',*,*,#15083,.F.);
#22156=ORIENTED_EDGE('',*,*,#15084,.T.);
#22157=ORIENTED_EDGE('',*,*,#15085,.F.);
#22158=ORIENTED_EDGE('',*,*,#15086,.T.);
#22159=ORIENTED_EDGE('',*,*,#15087,.T.);
#22160=ORIENTED_EDGE('',*,*,#15088,.T.);
#22161=ORIENTED_EDGE('',*,*,#15046,.T.);
#22162=ORIENTED_EDGE('',*,*,#15039,.T.);
#22163=ORIENTED_EDGE('',*,*,#14837,.F.);
#22164=ORIENTED_EDGE('',*,*,#14839,.T.);
#22165=ORIENTED_EDGE('',*,*,#14830,.F.);
#22166=ORIENTED_EDGE('',*,*,#14834,.T.);
#22167=ORIENTED_EDGE('',*,*,#15044,.T.);
#22168=ORIENTED_EDGE('',*,*,#15089,.T.);
#22169=ORIENTED_EDGE('',*,*,#15037,.T.);
#22170=ORIENTED_EDGE('',*,*,#15030,.T.);
#22171=ORIENTED_EDGE('',*,*,#14824,.F.);
#22172=ORIENTED_EDGE('',*,*,#14826,.T.);
#22173=ORIENTED_EDGE('',*,*,#14817,.F.);
#22174=ORIENTED_EDGE('',*,*,#14821,.T.);
#22175=ORIENTED_EDGE('',*,*,#15035,.T.);
#22176=ORIENTED_EDGE('',*,*,#15090,.T.);
#22177=ORIENTED_EDGE('',*,*,#15028,.T.);
#22178=ORIENTED_EDGE('',*,*,#15021,.T.);
#22179=ORIENTED_EDGE('',*,*,#14811,.F.);
#22180=ORIENTED_EDGE('',*,*,#14813,.T.);
#22181=ORIENTED_EDGE('',*,*,#14804,.F.);
#22182=ORIENTED_EDGE('',*,*,#14808,.T.);
#22183=ORIENTED_EDGE('',*,*,#15026,.T.);
#22184=ORIENTED_EDGE('',*,*,#15091,.T.);
#22185=ORIENTED_EDGE('',*,*,#15019,.T.);
#22186=ORIENTED_EDGE('',*,*,#15012,.T.);
#22187=ORIENTED_EDGE('',*,*,#14798,.F.);
#22188=ORIENTED_EDGE('',*,*,#14800,.T.);
#22189=ORIENTED_EDGE('',*,*,#14791,.F.);
#22190=ORIENTED_EDGE('',*,*,#14795,.T.);
#22191=ORIENTED_EDGE('',*,*,#15017,.T.);
#22192=ORIENTED_EDGE('',*,*,#15092,.T.);
#22193=ORIENTED_EDGE('',*,*,#15010,.T.);
#22194=ORIENTED_EDGE('',*,*,#15003,.T.);
#22195=ORIENTED_EDGE('',*,*,#14785,.F.);
#22196=ORIENTED_EDGE('',*,*,#14787,.T.);
#22197=ORIENTED_EDGE('',*,*,#14778,.F.);
#22198=ORIENTED_EDGE('',*,*,#14782,.T.);
#22199=ORIENTED_EDGE('',*,*,#15008,.T.);
#22200=ORIENTED_EDGE('',*,*,#15093,.T.);
#22201=ORIENTED_EDGE('',*,*,#15001,.T.);
#22202=ORIENTED_EDGE('',*,*,#14994,.T.);
#22203=ORIENTED_EDGE('',*,*,#14772,.F.);
#22204=ORIENTED_EDGE('',*,*,#14774,.T.);
#22205=ORIENTED_EDGE('',*,*,#14765,.F.);
#22206=ORIENTED_EDGE('',*,*,#14769,.T.);
#22207=ORIENTED_EDGE('',*,*,#14999,.T.);
#22208=ORIENTED_EDGE('',*,*,#15094,.T.);
#22209=ORIENTED_EDGE('',*,*,#14992,.T.);
#22210=ORIENTED_EDGE('',*,*,#14985,.T.);
#22211=ORIENTED_EDGE('',*,*,#14759,.F.);
#22212=ORIENTED_EDGE('',*,*,#14761,.T.);
#22213=ORIENTED_EDGE('',*,*,#14752,.F.);
#22214=ORIENTED_EDGE('',*,*,#14756,.T.);
#22215=ORIENTED_EDGE('',*,*,#14990,.T.);
#22216=ORIENTED_EDGE('',*,*,#15095,.T.);
#22217=ORIENTED_EDGE('',*,*,#14983,.T.);
#22218=ORIENTED_EDGE('',*,*,#14976,.T.);
#22219=ORIENTED_EDGE('',*,*,#14746,.F.);
#22220=ORIENTED_EDGE('',*,*,#14748,.T.);
#22221=ORIENTED_EDGE('',*,*,#14739,.F.);
#22222=ORIENTED_EDGE('',*,*,#14743,.T.);
#22223=ORIENTED_EDGE('',*,*,#14981,.T.);
#22224=ORIENTED_EDGE('',*,*,#15096,.T.);
#22225=ORIENTED_EDGE('',*,*,#14974,.T.);
#22226=ORIENTED_EDGE('',*,*,#14967,.T.);
#22227=ORIENTED_EDGE('',*,*,#14733,.F.);
#22228=ORIENTED_EDGE('',*,*,#14735,.T.);
#22229=ORIENTED_EDGE('',*,*,#14726,.F.);
#22230=ORIENTED_EDGE('',*,*,#14730,.T.);
#22231=ORIENTED_EDGE('',*,*,#14972,.T.);
#22232=ORIENTED_EDGE('',*,*,#15097,.T.);
#22233=ORIENTED_EDGE('',*,*,#14965,.T.);
#22234=ORIENTED_EDGE('',*,*,#14958,.T.);
#22235=ORIENTED_EDGE('',*,*,#14720,.F.);
#22236=ORIENTED_EDGE('',*,*,#14722,.T.);
#22237=ORIENTED_EDGE('',*,*,#14713,.F.);
#22238=ORIENTED_EDGE('',*,*,#14717,.T.);
#22239=ORIENTED_EDGE('',*,*,#14963,.T.);
#22240=ORIENTED_EDGE('',*,*,#15098,.T.);
#22241=ORIENTED_EDGE('',*,*,#14956,.T.);
#22242=ORIENTED_EDGE('',*,*,#14949,.T.);
#22243=ORIENTED_EDGE('',*,*,#14707,.F.);
#22244=ORIENTED_EDGE('',*,*,#14709,.T.);
#22245=ORIENTED_EDGE('',*,*,#14700,.F.);
#22246=ORIENTED_EDGE('',*,*,#14704,.T.);
#22247=ORIENTED_EDGE('',*,*,#14954,.T.);
#22248=ORIENTED_EDGE('',*,*,#15099,.T.);
#22249=ORIENTED_EDGE('',*,*,#14947,.T.);
#22250=ORIENTED_EDGE('',*,*,#14940,.T.);
#22251=ORIENTED_EDGE('',*,*,#14694,.F.);
#22252=ORIENTED_EDGE('',*,*,#14696,.T.);
#22253=ORIENTED_EDGE('',*,*,#14687,.F.);
#22254=ORIENTED_EDGE('',*,*,#14691,.T.);
#22255=ORIENTED_EDGE('',*,*,#14945,.T.);
#22256=ORIENTED_EDGE('',*,*,#15100,.T.);
#22257=ORIENTED_EDGE('',*,*,#14938,.T.);
#22258=ORIENTED_EDGE('',*,*,#14931,.T.);
#22259=ORIENTED_EDGE('',*,*,#14681,.F.);
#22260=ORIENTED_EDGE('',*,*,#14683,.T.);
#22261=ORIENTED_EDGE('',*,*,#14674,.F.);
#22262=ORIENTED_EDGE('',*,*,#14678,.T.);
#22263=ORIENTED_EDGE('',*,*,#14936,.T.);
#22264=ORIENTED_EDGE('',*,*,#15101,.T.);
#22265=ORIENTED_EDGE('',*,*,#14929,.T.);
#22266=ORIENTED_EDGE('',*,*,#14922,.T.);
#22267=ORIENTED_EDGE('',*,*,#14668,.F.);
#22268=ORIENTED_EDGE('',*,*,#14670,.T.);
#22269=ORIENTED_EDGE('',*,*,#14661,.F.);
#22270=ORIENTED_EDGE('',*,*,#14665,.T.);
#22271=ORIENTED_EDGE('',*,*,#14927,.T.);
#22272=ORIENTED_EDGE('',*,*,#15102,.T.);
#22273=ORIENTED_EDGE('',*,*,#14920,.T.);
#22274=ORIENTED_EDGE('',*,*,#14913,.T.);
#22275=ORIENTED_EDGE('',*,*,#14655,.F.);
#22276=ORIENTED_EDGE('',*,*,#14657,.T.);
#22277=ORIENTED_EDGE('',*,*,#14648,.F.);
#22278=ORIENTED_EDGE('',*,*,#14652,.T.);
#22279=ORIENTED_EDGE('',*,*,#14918,.T.);
#22280=ORIENTED_EDGE('',*,*,#15103,.T.);
#22281=ORIENTED_EDGE('',*,*,#14911,.T.);
#22282=ORIENTED_EDGE('',*,*,#14904,.T.);
#22283=ORIENTED_EDGE('',*,*,#14642,.F.);
#22284=ORIENTED_EDGE('',*,*,#14644,.T.);
#22285=ORIENTED_EDGE('',*,*,#14635,.F.);
#22286=ORIENTED_EDGE('',*,*,#14639,.T.);
#22287=ORIENTED_EDGE('',*,*,#14909,.T.);
#22288=ORIENTED_EDGE('',*,*,#15104,.T.);
#22289=ORIENTED_EDGE('',*,*,#14902,.T.);
#22290=ORIENTED_EDGE('',*,*,#14895,.T.);
#22291=ORIENTED_EDGE('',*,*,#14629,.F.);
#22292=ORIENTED_EDGE('',*,*,#14631,.T.);
#22293=ORIENTED_EDGE('',*,*,#14622,.F.);
#22294=ORIENTED_EDGE('',*,*,#14626,.T.);
#22295=ORIENTED_EDGE('',*,*,#14900,.T.);
#22296=ORIENTED_EDGE('',*,*,#15105,.T.);
#22297=ORIENTED_EDGE('',*,*,#14893,.T.);
#22298=ORIENTED_EDGE('',*,*,#14886,.T.);
#22299=ORIENTED_EDGE('',*,*,#14616,.F.);
#22300=ORIENTED_EDGE('',*,*,#14618,.T.);
#22301=ORIENTED_EDGE('',*,*,#14609,.F.);
#22302=ORIENTED_EDGE('',*,*,#14613,.T.);
#22303=ORIENTED_EDGE('',*,*,#14891,.T.);
#22304=ORIENTED_EDGE('',*,*,#15106,.T.);
#22305=ORIENTED_EDGE('',*,*,#14884,.T.);
#22306=ORIENTED_EDGE('',*,*,#14877,.T.);
#22307=ORIENTED_EDGE('',*,*,#14603,.F.);
#22308=ORIENTED_EDGE('',*,*,#14605,.T.);
#22309=ORIENTED_EDGE('',*,*,#14596,.F.);
#22310=ORIENTED_EDGE('',*,*,#14600,.T.);
#22311=ORIENTED_EDGE('',*,*,#14882,.T.);
#22312=ORIENTED_EDGE('',*,*,#15107,.T.);
#22313=ORIENTED_EDGE('',*,*,#14875,.T.);
#22314=ORIENTED_EDGE('',*,*,#14868,.T.);
#22315=ORIENTED_EDGE('',*,*,#14590,.F.);
#22316=ORIENTED_EDGE('',*,*,#14592,.T.);
#22317=ORIENTED_EDGE('',*,*,#14583,.F.);
#22318=ORIENTED_EDGE('',*,*,#14587,.T.);
#22319=ORIENTED_EDGE('',*,*,#14873,.T.);
#22320=ORIENTED_EDGE('',*,*,#15108,.T.);
#22321=ORIENTED_EDGE('',*,*,#14866,.T.);
#22322=ORIENTED_EDGE('',*,*,#14859,.T.);
#22323=ORIENTED_EDGE('',*,*,#14577,.F.);
#22324=ORIENTED_EDGE('',*,*,#14579,.T.);
#22325=ORIENTED_EDGE('',*,*,#14570,.F.);
#22326=ORIENTED_EDGE('',*,*,#14574,.T.);
#22327=ORIENTED_EDGE('',*,*,#14864,.T.);
#22328=ORIENTED_EDGE('',*,*,#15109,.T.);
#22329=ORIENTED_EDGE('',*,*,#14857,.T.);
#22330=ORIENTED_EDGE('',*,*,#14850,.T.);
#22331=ORIENTED_EDGE('',*,*,#14564,.F.);
#22332=ORIENTED_EDGE('',*,*,#14566,.T.);
#22333=ORIENTED_EDGE('',*,*,#14557,.F.);
#22334=ORIENTED_EDGE('',*,*,#14561,.T.);
#22335=ORIENTED_EDGE('',*,*,#14855,.T.);
#22336=ORIENTED_EDGE('',*,*,#15110,.T.);
#22337=ORIENTED_EDGE('',*,*,#14848,.T.);
#22338=ORIENTED_EDGE('',*,*,#14841,.T.);
#22339=ORIENTED_EDGE('',*,*,#14551,.F.);
#22340=ORIENTED_EDGE('',*,*,#14553,.T.);
#22341=ORIENTED_EDGE('',*,*,#14544,.F.);
#22342=ORIENTED_EDGE('',*,*,#14548,.T.);
#22343=ORIENTED_EDGE('',*,*,#15111,.T.);
#22344=ORIENTED_EDGE('',*,*,#15047,.T.);
#22345=ORIENTED_EDGE('',*,*,#15088,.F.);
#22346=ORIENTED_EDGE('',*,*,#15112,.T.);
#22347=ORIENTED_EDGE('',*,*,#15070,.T.);
#22348=ORIENTED_EDGE('',*,*,#15038,.T.);
#22349=ORIENTED_EDGE('',*,*,#15089,.F.);
#22350=ORIENTED_EDGE('',*,*,#15043,.T.);
#22351=ORIENTED_EDGE('',*,*,#15069,.T.);
#22352=ORIENTED_EDGE('',*,*,#15029,.T.);
#22353=ORIENTED_EDGE('',*,*,#15090,.F.);
#22354=ORIENTED_EDGE('',*,*,#15034,.T.);
#22355=ORIENTED_EDGE('',*,*,#15068,.T.);
#22356=ORIENTED_EDGE('',*,*,#15020,.T.);
#22357=ORIENTED_EDGE('',*,*,#15091,.F.);
#22358=ORIENTED_EDGE('',*,*,#15025,.T.);
#22359=ORIENTED_EDGE('',*,*,#15067,.T.);
#22360=ORIENTED_EDGE('',*,*,#15011,.T.);
#22361=ORIENTED_EDGE('',*,*,#15092,.F.);
#22362=ORIENTED_EDGE('',*,*,#15016,.T.);
#22363=ORIENTED_EDGE('',*,*,#15066,.T.);
#22364=ORIENTED_EDGE('',*,*,#15002,.T.);
#22365=ORIENTED_EDGE('',*,*,#15093,.F.);
#22366=ORIENTED_EDGE('',*,*,#15007,.T.);
#22367=ORIENTED_EDGE('',*,*,#15065,.T.);
#22368=ORIENTED_EDGE('',*,*,#14993,.T.);
#22369=ORIENTED_EDGE('',*,*,#15094,.F.);
#22370=ORIENTED_EDGE('',*,*,#14998,.T.);
#22371=ORIENTED_EDGE('',*,*,#15064,.T.);
#22372=ORIENTED_EDGE('',*,*,#14984,.T.);
#22373=ORIENTED_EDGE('',*,*,#15095,.F.);
#22374=ORIENTED_EDGE('',*,*,#14989,.T.);
#22375=ORIENTED_EDGE('',*,*,#15063,.T.);
#22376=ORIENTED_EDGE('',*,*,#14975,.T.);
#22377=ORIENTED_EDGE('',*,*,#15096,.F.);
#22378=ORIENTED_EDGE('',*,*,#14980,.T.);
#22379=ORIENTED_EDGE('',*,*,#15062,.T.);
#22380=ORIENTED_EDGE('',*,*,#14966,.T.);
#22381=ORIENTED_EDGE('',*,*,#15097,.F.);
#22382=ORIENTED_EDGE('',*,*,#14971,.T.);
#22383=ORIENTED_EDGE('',*,*,#15061,.T.);
#22384=ORIENTED_EDGE('',*,*,#14957,.T.);
#22385=ORIENTED_EDGE('',*,*,#15098,.F.);
#22386=ORIENTED_EDGE('',*,*,#14962,.T.);
#22387=ORIENTED_EDGE('',*,*,#15060,.T.);
#22388=ORIENTED_EDGE('',*,*,#14948,.T.);
#22389=ORIENTED_EDGE('',*,*,#15099,.F.);
#22390=ORIENTED_EDGE('',*,*,#14953,.T.);
#22391=ORIENTED_EDGE('',*,*,#15059,.T.);
#22392=ORIENTED_EDGE('',*,*,#14939,.T.);
#22393=ORIENTED_EDGE('',*,*,#15100,.F.);
#22394=ORIENTED_EDGE('',*,*,#14944,.T.);
#22395=ORIENTED_EDGE('',*,*,#15058,.T.);
#22396=ORIENTED_EDGE('',*,*,#14930,.T.);
#22397=ORIENTED_EDGE('',*,*,#15101,.F.);
#22398=ORIENTED_EDGE('',*,*,#14935,.T.);
#22399=ORIENTED_EDGE('',*,*,#15057,.T.);
#22400=ORIENTED_EDGE('',*,*,#14921,.T.);
#22401=ORIENTED_EDGE('',*,*,#15102,.F.);
#22402=ORIENTED_EDGE('',*,*,#14926,.T.);
#22403=ORIENTED_EDGE('',*,*,#15056,.T.);
#22404=ORIENTED_EDGE('',*,*,#14912,.T.);
#22405=ORIENTED_EDGE('',*,*,#15103,.F.);
#22406=ORIENTED_EDGE('',*,*,#14917,.T.);
#22407=ORIENTED_EDGE('',*,*,#15055,.T.);
#22408=ORIENTED_EDGE('',*,*,#14903,.T.);
#22409=ORIENTED_EDGE('',*,*,#15104,.F.);
#22410=ORIENTED_EDGE('',*,*,#14908,.T.);
#22411=ORIENTED_EDGE('',*,*,#15054,.T.);
#22412=ORIENTED_EDGE('',*,*,#14894,.T.);
#22413=ORIENTED_EDGE('',*,*,#15105,.F.);
#22414=ORIENTED_EDGE('',*,*,#14899,.T.);
#22415=ORIENTED_EDGE('',*,*,#15053,.T.);
#22416=ORIENTED_EDGE('',*,*,#14885,.T.);
#22417=ORIENTED_EDGE('',*,*,#15106,.F.);
#22418=ORIENTED_EDGE('',*,*,#14890,.T.);
#22419=ORIENTED_EDGE('',*,*,#15052,.T.);
#22420=ORIENTED_EDGE('',*,*,#14876,.T.);
#22421=ORIENTED_EDGE('',*,*,#15107,.F.);
#22422=ORIENTED_EDGE('',*,*,#14881,.T.);
#22423=ORIENTED_EDGE('',*,*,#15051,.T.);
#22424=ORIENTED_EDGE('',*,*,#14867,.T.);
#22425=ORIENTED_EDGE('',*,*,#15108,.F.);
#22426=ORIENTED_EDGE('',*,*,#14872,.T.);
#22427=ORIENTED_EDGE('',*,*,#15050,.T.);
#22428=ORIENTED_EDGE('',*,*,#14858,.T.);
#22429=ORIENTED_EDGE('',*,*,#15109,.F.);
#22430=ORIENTED_EDGE('',*,*,#14863,.T.);
#22431=ORIENTED_EDGE('',*,*,#15049,.T.);
#22432=ORIENTED_EDGE('',*,*,#14849,.T.);
#22433=ORIENTED_EDGE('',*,*,#15110,.F.);
#22434=ORIENTED_EDGE('',*,*,#14854,.T.);
#22435=ORIENTED_EDGE('',*,*,#15048,.T.);
#22436=ORIENTED_EDGE('',*,*,#15073,.T.);
#22437=ORIENTED_EDGE('',*,*,#15113,.T.);
#22438=ORIENTED_EDGE('',*,*,#15085,.T.);
#22439=ORIENTED_EDGE('',*,*,#15114,.T.);
#22440=ORIENTED_EDGE('',*,*,#15113,.F.);
#22441=ORIENTED_EDGE('',*,*,#15072,.F.);
#22442=ORIENTED_EDGE('',*,*,#15115,.T.);
#22443=ORIENTED_EDGE('',*,*,#15086,.F.);
#22444=ORIENTED_EDGE('',*,*,#15075,.T.);
#22445=ORIENTED_EDGE('',*,*,#15116,.T.);
#22446=ORIENTED_EDGE('',*,*,#15083,.T.);
#22447=ORIENTED_EDGE('',*,*,#15117,.T.);
#22448=ORIENTED_EDGE('',*,*,#15114,.F.);
#22449=ORIENTED_EDGE('',*,*,#15084,.F.);
#22450=ORIENTED_EDGE('',*,*,#15116,.F.);
#22451=ORIENTED_EDGE('',*,*,#15074,.F.);
#22452=ORIENTED_EDGE('',*,*,#15117,.F.);
#22453=ORIENTED_EDGE('',*,*,#15082,.F.);
#22454=ORIENTED_EDGE('',*,*,#15118,.F.);
#22455=ORIENTED_EDGE('',*,*,#15076,.F.);
#22456=ORIENTED_EDGE('',*,*,#15071,.F.);
#22457=ORIENTED_EDGE('',*,*,#15112,.F.);
#22458=ORIENTED_EDGE('',*,*,#15087,.F.);
#22459=ORIENTED_EDGE('',*,*,#15115,.F.);
#22460=ORIENTED_EDGE('',*,*,#15077,.F.);
#22461=ORIENTED_EDGE('',*,*,#15118,.T.);
#22462=ORIENTED_EDGE('',*,*,#15081,.F.);
#22463=ORIENTED_EDGE('',*,*,#15119,.F.);
#22464=ORIENTED_EDGE('',*,*,#15111,.F.);
#22465=ORIENTED_EDGE('',*,*,#15120,.T.);
#22466=ORIENTED_EDGE('',*,*,#15079,.T.);
#22467=ORIENTED_EDGE('',*,*,#15120,.F.);
#22468=ORIENTED_EDGE('',*,*,#14845,.T.);
#22469=ORIENTED_EDGE('',*,*,#15078,.T.);
#22470=ORIENTED_EDGE('',*,*,#15119,.T.);
#22471=ORIENTED_EDGE('',*,*,#15080,.F.);
#23628=CYLINDRICAL_SURFACE('',#26660,0.5);
#23629=CYLINDRICAL_SURFACE('',#26664,0.5);
#23630=CYLINDRICAL_SURFACE('',#26667,21.4999999999992);
#23631=CYLINDRICAL_SURFACE('',#26670,0.5);
#23632=CYLINDRICAL_SURFACE('',#26674,0.5);
#23633=CYLINDRICAL_SURFACE('',#26677,21.4999999999992);
#23634=CYLINDRICAL_SURFACE('',#26680,0.5);
#23635=CYLINDRICAL_SURFACE('',#26684,0.5);
#23636=CYLINDRICAL_SURFACE('',#26687,21.4999999999992);
#23637=CYLINDRICAL_SURFACE('',#26690,0.5);
#23638=CYLINDRICAL_SURFACE('',#26694,0.5);
#23639=CYLINDRICAL_SURFACE('',#26697,21.4999999999992);
#23640=CYLINDRICAL_SURFACE('',#26700,0.5);
#23641=CYLINDRICAL_SURFACE('',#26704,0.5);
#23642=CYLINDRICAL_SURFACE('',#26707,21.4999999999992);
#23643=CYLINDRICAL_SURFACE('',#26710,0.5);
#23644=CYLINDRICAL_SURFACE('',#26714,0.5);
#23645=CYLINDRICAL_SURFACE('',#26717,21.4999999999992);
#23646=CYLINDRICAL_SURFACE('',#26720,0.5);
#23647=CYLINDRICAL_SURFACE('',#26724,0.5);
#23648=CYLINDRICAL_SURFACE('',#26727,21.4999999999992);
#23649=CYLINDRICAL_SURFACE('',#26730,0.5);
#23650=CYLINDRICAL_SURFACE('',#26734,0.5);
#23651=CYLINDRICAL_SURFACE('',#26737,21.4999999999992);
#23652=CYLINDRICAL_SURFACE('',#26740,0.5);
#23653=CYLINDRICAL_SURFACE('',#26744,0.5);
#23654=CYLINDRICAL_SURFACE('',#26747,21.4999999999992);
#23655=CYLINDRICAL_SURFACE('',#26750,0.5);
#23656=CYLINDRICAL_SURFACE('',#26754,0.5);
#23657=CYLINDRICAL_SURFACE('',#26757,21.4999999999992);
#23658=CYLINDRICAL_SURFACE('',#26760,0.5);
#23659=CYLINDRICAL_SURFACE('',#26764,0.5);
#23660=CYLINDRICAL_SURFACE('',#26767,21.4999999999992);
#23661=CYLINDRICAL_SURFACE('',#26770,0.5);
#23662=CYLINDRICAL_SURFACE('',#26774,0.5);
#23663=CYLINDRICAL_SURFACE('',#26777,21.4999999999992);
#23664=CYLINDRICAL_SURFACE('',#26780,0.5);
#23665=CYLINDRICAL_SURFACE('',#26784,0.5);
#23666=CYLINDRICAL_SURFACE('',#26787,21.4999999999992);
#23667=CYLINDRICAL_SURFACE('',#26790,0.5);
#23668=CYLINDRICAL_SURFACE('',#26794,0.5);
#23669=CYLINDRICAL_SURFACE('',#26797,21.4999999999992);
#23670=CYLINDRICAL_SURFACE('',#26800,0.5);
#23671=CYLINDRICAL_SURFACE('',#26804,0.5);
#23672=CYLINDRICAL_SURFACE('',#26807,21.4999999999992);
#23673=CYLINDRICAL_SURFACE('',#26810,0.5);
#23674=CYLINDRICAL_SURFACE('',#26814,0.5);
#23675=CYLINDRICAL_SURFACE('',#26817,21.4999999999992);
#23676=CYLINDRICAL_SURFACE('',#26820,0.5);
#23677=CYLINDRICAL_SURFACE('',#26824,0.5);
#23678=CYLINDRICAL_SURFACE('',#26827,21.4999999999992);
#23679=CYLINDRICAL_SURFACE('',#26830,0.5);
#23680=CYLINDRICAL_SURFACE('',#26834,0.5);
#23681=CYLINDRICAL_SURFACE('',#26837,21.4999999999992);
#23682=CYLINDRICAL_SURFACE('',#26840,0.5);
#23683=CYLINDRICAL_SURFACE('',#26844,0.5);
#23684=CYLINDRICAL_SURFACE('',#26847,21.4999999999992);
#23685=CYLINDRICAL_SURFACE('',#26850,0.5);
#23686=CYLINDRICAL_SURFACE('',#26854,0.5);
#23687=CYLINDRICAL_SURFACE('',#26857,21.4999999999992);
#23688=CYLINDRICAL_SURFACE('',#26860,0.5);
#23689=CYLINDRICAL_SURFACE('',#26864,0.5);
#23690=CYLINDRICAL_SURFACE('',#26867,21.4999999999992);
#23691=CYLINDRICAL_SURFACE('',#26870,0.5);
#23692=CYLINDRICAL_SURFACE('',#26874,0.5);
#23693=CYLINDRICAL_SURFACE('',#26877,21.4999999999992);
#23694=CYLINDRICAL_SURFACE('',#26880,0.5);
#23695=CYLINDRICAL_SURFACE('',#26884,0.5);
#23696=CYLINDRICAL_SURFACE('',#26887,21.4999999999992);
#23697=CYLINDRICAL_SURFACE('',#26971,26.);
#23698=CYLINDRICAL_SURFACE('',#26972,26.);
#23699=CYLINDRICAL_SURFACE('',#26973,26.);
#23700=CYLINDRICAL_SURFACE('',#26974,26.);
#23701=CYLINDRICAL_SURFACE('',#26975,26.);
#23702=CYLINDRICAL_SURFACE('',#26976,26.);
#23703=CYLINDRICAL_SURFACE('',#26977,26.);
#23704=CYLINDRICAL_SURFACE('',#26978,26.);
#23705=CYLINDRICAL_SURFACE('',#26979,26.);
#23706=CYLINDRICAL_SURFACE('',#26980,26.);
#23707=CYLINDRICAL_SURFACE('',#26981,26.);
#23708=CYLINDRICAL_SURFACE('',#26982,26.);
#23709=CYLINDRICAL_SURFACE('',#26983,26.);
#23710=CYLINDRICAL_SURFACE('',#26984,26.);
#23711=CYLINDRICAL_SURFACE('',#26985,26.);
#23712=CYLINDRICAL_SURFACE('',#26986,26.);
#23713=CYLINDRICAL_SURFACE('',#26987,26.);
#23714=CYLINDRICAL_SURFACE('',#26988,26.);
#23715=CYLINDRICAL_SURFACE('',#26989,26.);
#23716=CYLINDRICAL_SURFACE('',#26990,26.);
#23717=CYLINDRICAL_SURFACE('',#26991,26.);
#23718=CYLINDRICAL_SURFACE('',#26992,26.);
#23719=CYLINDRICAL_SURFACE('',#26993,26.);
#23720=CYLINDRICAL_SURFACE('',#26994,0.5);
#23721=CYLINDRICAL_SURFACE('',#26996,0.5);
#23722=CYLINDRICAL_SURFACE('',#26997,21.4999999999992);
#23723=CYLINDRICAL_SURFACE('',#26999,7.);
#23724=CYLINDRICAL_SURFACE('',#27000,26.);
#24811=ADVANCED_FACE('',(#2705),#23628,.F.);
#24812=ADVANCED_FACE('',(#2706),#1585,.F.);
#24813=ADVANCED_FACE('',(#2707),#23629,.F.);
#24814=ADVANCED_FACE('',(#2708),#23630,.T.);
#24815=ADVANCED_FACE('',(#2709),#23631,.F.);
#24816=ADVANCED_FACE('',(#2710),#1586,.F.);
#24817=ADVANCED_FACE('',(#2711),#23632,.F.);
#24818=ADVANCED_FACE('',(#2712),#23633,.T.);
#24819=ADVANCED_FACE('',(#2713),#23634,.F.);
#24820=ADVANCED_FACE('',(#2714),#1587,.F.);
#24821=ADVANCED_FACE('',(#2715),#23635,.F.);
#24822=ADVANCED_FACE('',(#2716),#23636,.T.);
#24823=ADVANCED_FACE('',(#2717),#23637,.F.);
#24824=ADVANCED_FACE('',(#2718),#1588,.F.);
#24825=ADVANCED_FACE('',(#2719),#23638,.F.);
#24826=ADVANCED_FACE('',(#2720),#23639,.T.);
#24827=ADVANCED_FACE('',(#2721),#23640,.F.);
#24828=ADVANCED_FACE('',(#2722),#1589,.F.);
#24829=ADVANCED_FACE('',(#2723),#23641,.F.);
#24830=ADVANCED_FACE('',(#2724),#23642,.T.);
#24831=ADVANCED_FACE('',(#2725),#23643,.F.);
#24832=ADVANCED_FACE('',(#2726),#1590,.F.);
#24833=ADVANCED_FACE('',(#2727),#23644,.F.);
#24834=ADVANCED_FACE('',(#2728),#23645,.T.);
#24835=ADVANCED_FACE('',(#2729),#23646,.F.);
#24836=ADVANCED_FACE('',(#2730),#1591,.F.);
#24837=ADVANCED_FACE('',(#2731),#23647,.F.);
#24838=ADVANCED_FACE('',(#2732),#23648,.T.);
#24839=ADVANCED_FACE('',(#2733),#23649,.F.);
#24840=ADVANCED_FACE('',(#2734),#1592,.F.);
#24841=ADVANCED_FACE('',(#2735),#23650,.F.);
#24842=ADVANCED_FACE('',(#2736),#23651,.T.);
#24843=ADVANCED_FACE('',(#2737),#23652,.F.);
#24844=ADVANCED_FACE('',(#2738),#1593,.F.);
#24845=ADVANCED_FACE('',(#2739),#23653,.F.);
#24846=ADVANCED_FACE('',(#2740),#23654,.T.);
#24847=ADVANCED_FACE('',(#2741),#23655,.F.);
#24848=ADVANCED_FACE('',(#2742),#1594,.F.);
#24849=ADVANCED_FACE('',(#2743),#23656,.F.);
#24850=ADVANCED_FACE('',(#2744),#23657,.T.);
#24851=ADVANCED_FACE('',(#2745),#23658,.F.);
#24852=ADVANCED_FACE('',(#2746),#1595,.F.);
#24853=ADVANCED_FACE('',(#2747),#23659,.F.);
#24854=ADVANCED_FACE('',(#2748),#23660,.T.);
#24855=ADVANCED_FACE('',(#2749),#23661,.F.);
#24856=ADVANCED_FACE('',(#2750),#1596,.F.);
#24857=ADVANCED_FACE('',(#2751),#23662,.F.);
#24858=ADVANCED_FACE('',(#2752),#23663,.T.);
#24859=ADVANCED_FACE('',(#2753),#23664,.F.);
#24860=ADVANCED_FACE('',(#2754),#1597,.F.);
#24861=ADVANCED_FACE('',(#2755),#23665,.F.);
#24862=ADVANCED_FACE('',(#2756),#23666,.T.);
#24863=ADVANCED_FACE('',(#2757),#23667,.F.);
#24864=ADVANCED_FACE('',(#2758),#1598,.F.);
#24865=ADVANCED_FACE('',(#2759),#23668,.F.);
#24866=ADVANCED_FACE('',(#2760),#23669,.T.);
#24867=ADVANCED_FACE('',(#2761),#23670,.F.);
#24868=ADVANCED_FACE('',(#2762),#1599,.F.);
#24869=ADVANCED_FACE('',(#2763),#23671,.F.);
#24870=ADVANCED_FACE('',(#2764),#23672,.T.);
#24871=ADVANCED_FACE('',(#2765),#23673,.F.);
#24872=ADVANCED_FACE('',(#2766),#1600,.F.);
#24873=ADVANCED_FACE('',(#2767),#23674,.F.);
#24874=ADVANCED_FACE('',(#2768),#23675,.T.);
#24875=ADVANCED_FACE('',(#2769),#23676,.F.);
#24876=ADVANCED_FACE('',(#2770),#1601,.F.);
#24877=ADVANCED_FACE('',(#2771),#23677,.F.);
#24878=ADVANCED_FACE('',(#2772),#23678,.T.);
#24879=ADVANCED_FACE('',(#2773),#23679,.F.);
#24880=ADVANCED_FACE('',(#2774),#1602,.F.);
#24881=ADVANCED_FACE('',(#2775),#23680,.F.);
#24882=ADVANCED_FACE('',(#2776),#23681,.T.);
#24883=ADVANCED_FACE('',(#2777),#23682,.F.);
#24884=ADVANCED_FACE('',(#2778),#1603,.F.);
#24885=ADVANCED_FACE('',(#2779),#23683,.F.);
#24886=ADVANCED_FACE('',(#2780),#23684,.T.);
#24887=ADVANCED_FACE('',(#2781),#23685,.F.);
#24888=ADVANCED_FACE('',(#2782),#1604,.F.);
#24889=ADVANCED_FACE('',(#2783),#23686,.F.);
#24890=ADVANCED_FACE('',(#2784),#23687,.T.);
#24891=ADVANCED_FACE('',(#2785),#23688,.F.);
#24892=ADVANCED_FACE('',(#2786),#1605,.F.);
#24893=ADVANCED_FACE('',(#2787),#23689,.F.);
#24894=ADVANCED_FACE('',(#2788),#23690,.T.);
#24895=ADVANCED_FACE('',(#2789),#23691,.F.);
#24896=ADVANCED_FACE('',(#2790),#1606,.F.);
#24897=ADVANCED_FACE('',(#2791),#23692,.F.);
#24898=ADVANCED_FACE('',(#2792),#23693,.T.);
#24899=ADVANCED_FACE('',(#2793),#23694,.F.);
#24900=ADVANCED_FACE('',(#2794),#1607,.F.);
#24901=ADVANCED_FACE('',(#2795),#23695,.F.);
#24902=ADVANCED_FACE('',(#2796),#23696,.T.);
#24903=ADVANCED_FACE('',(#2797),#1608,.F.);
#24904=ADVANCED_FACE('',(#2798),#1075,.F.);
#24905=ADVANCED_FACE('',(#2799),#1076,.F.);
#24906=ADVANCED_FACE('',(#2800),#1609,.F.);
#24907=ADVANCED_FACE('',(#2801),#1077,.F.);
#24908=ADVANCED_FACE('',(#2802),#1078,.F.);
#24909=ADVANCED_FACE('',(#2803),#1610,.F.);
#24910=ADVANCED_FACE('',(#2804),#1079,.F.);
#24911=ADVANCED_FACE('',(#2805),#1080,.F.);
#24912=ADVANCED_FACE('',(#2806),#1611,.F.);
#24913=ADVANCED_FACE('',(#2807),#1081,.F.);
#24914=ADVANCED_FACE('',(#2808),#1082,.F.);
#24915=ADVANCED_FACE('',(#2809),#1612,.F.);
#24916=ADVANCED_FACE('',(#2810),#1083,.F.);
#24917=ADVANCED_FACE('',(#2811),#1084,.F.);
#24918=ADVANCED_FACE('',(#2812),#1613,.F.);
#24919=ADVANCED_FACE('',(#2813),#1085,.F.);
#24920=ADVANCED_FACE('',(#2814),#1086,.F.);
#24921=ADVANCED_FACE('',(#2815),#1614,.F.);
#24922=ADVANCED_FACE('',(#2816),#1087,.F.);
#24923=ADVANCED_FACE('',(#2817),#1088,.F.);
#24924=ADVANCED_FACE('',(#2818),#1615,.F.);
#24925=ADVANCED_FACE('',(#2819),#1089,.F.);
#24926=ADVANCED_FACE('',(#2820),#1090,.F.);
#24927=ADVANCED_FACE('',(#2821),#1616,.F.);
#24928=ADVANCED_FACE('',(#2822),#1091,.F.);
#24929=ADVANCED_FACE('',(#2823),#1092,.F.);
#24930=ADVANCED_FACE('',(#2824),#1617,.F.);
#24931=ADVANCED_FACE('',(#2825),#1093,.F.);
#24932=ADVANCED_FACE('',(#2826),#1094,.F.);
#24933=ADVANCED_FACE('',(#2827),#1618,.F.);
#24934=ADVANCED_FACE('',(#2828),#1095,.F.);
#24935=ADVANCED_FACE('',(#2829),#1096,.F.);
#24936=ADVANCED_FACE('',(#2830),#1619,.F.);
#24937=ADVANCED_FACE('',(#2831),#1097,.F.);
#24938=ADVANCED_FACE('',(#2832),#1098,.F.);
#24939=ADVANCED_FACE('',(#2833),#1620,.F.);
#24940=ADVANCED_FACE('',(#2834),#1099,.F.);
#24941=ADVANCED_FACE('',(#2835),#1100,.F.);
#24942=ADVANCED_FACE('',(#2836),#1621,.F.);
#24943=ADVANCED_FACE('',(#2837),#1101,.F.);
#24944=ADVANCED_FACE('',(#2838),#1102,.F.);
#24945=ADVANCED_FACE('',(#2839),#1622,.F.);
#24946=ADVANCED_FACE('',(#2840),#1103,.F.);
#24947=ADVANCED_FACE('',(#2841),#1104,.F.);
#24948=ADVANCED_FACE('',(#2842),#1623,.F.);
#24949=ADVANCED_FACE('',(#2843),#1105,.F.);
#24950=ADVANCED_FACE('',(#2844),#1106,.F.);
#24951=ADVANCED_FACE('',(#2845),#1624,.F.);
#24952=ADVANCED_FACE('',(#2846),#1107,.F.);
#24953=ADVANCED_FACE('',(#2847),#1108,.F.);
#24954=ADVANCED_FACE('',(#2848),#1625,.F.);
#24955=ADVANCED_FACE('',(#2849),#1109,.F.);
#24956=ADVANCED_FACE('',(#2850),#1110,.F.);
#24957=ADVANCED_FACE('',(#2851),#1626,.F.);
#24958=ADVANCED_FACE('',(#2852),#1111,.F.);
#24959=ADVANCED_FACE('',(#2853),#1112,.F.);
#24960=ADVANCED_FACE('',(#2854),#1627,.F.);
#24961=ADVANCED_FACE('',(#2855),#1113,.F.);
#24962=ADVANCED_FACE('',(#2856),#1114,.F.);
#24963=ADVANCED_FACE('',(#2857),#1628,.F.);
#24964=ADVANCED_FACE('',(#2858),#1115,.F.);
#24965=ADVANCED_FACE('',(#2859),#1116,.F.);
#24966=ADVANCED_FACE('',(#2860),#1629,.F.);
#24967=ADVANCED_FACE('',(#2861),#1117,.F.);
#24968=ADVANCED_FACE('',(#2862),#1118,.F.);
#24969=ADVANCED_FACE('',(#2863),#1630,.F.);
#24970=ADVANCED_FACE('',(#2864),#1119,.F.);
#24971=ADVANCED_FACE('',(#2865),#1120,.F.);
#24972=ADVANCED_FACE('',(#2866,#1283),#1631,.F.);
#24973=ADVANCED_FACE('',(#2867,#1284),#1632,.T.);
#24974=ADVANCED_FACE('',(#2868),#23697,.T.);
#24975=ADVANCED_FACE('',(#2869),#23698,.T.);
#24976=ADVANCED_FACE('',(#2870),#23699,.T.);
#24977=ADVANCED_FACE('',(#2871),#23700,.T.);
#24978=ADVANCED_FACE('',(#2872),#23701,.T.);
#24979=ADVANCED_FACE('',(#2873),#23702,.T.);
#24980=ADVANCED_FACE('',(#2874),#23703,.T.);
#24981=ADVANCED_FACE('',(#2875),#23704,.T.);
#24982=ADVANCED_FACE('',(#2876),#23705,.T.);
#24983=ADVANCED_FACE('',(#2877),#23706,.T.);
#24984=ADVANCED_FACE('',(#2878),#23707,.T.);
#24985=ADVANCED_FACE('',(#2879),#23708,.T.);
#24986=ADVANCED_FACE('',(#2880),#23709,.T.);
#24987=ADVANCED_FACE('',(#2881),#23710,.T.);
#24988=ADVANCED_FACE('',(#2882),#23711,.T.);
#24989=ADVANCED_FACE('',(#2883),#23712,.T.);
#24990=ADVANCED_FACE('',(#2884),#23713,.T.);
#24991=ADVANCED_FACE('',(#2885),#23714,.T.);
#24992=ADVANCED_FACE('',(#2886),#23715,.T.);
#24993=ADVANCED_FACE('',(#2887),#23716,.T.);
#24994=ADVANCED_FACE('',(#2888),#23717,.T.);
#24995=ADVANCED_FACE('',(#2889),#23718,.T.);
#24996=ADVANCED_FACE('',(#2890),#23719,.T.);
#24997=ADVANCED_FACE('',(#2891),#23720,.F.);
#24998=ADVANCED_FACE('',(#2892),#1633,.F.);
#24999=ADVANCED_FACE('',(#2893),#23721,.F.);
#25000=ADVANCED_FACE('',(#2894),#23722,.T.);
#25001=ADVANCED_FACE('',(#2895),#1634,.F.);
#25002=ADVANCED_FACE('',(#2896),#1121,.F.);
#25003=ADVANCED_FACE('',(#2897),#1122,.F.);
#25004=ADVANCED_FACE('',(#2898),#23723,.F.);
#25005=ADVANCED_FACE('',(#2899),#23724,.T.);
#25156=CLOSED_SHELL('',(#24811,#24812,#24813,#24814,#24815,#24816,#24817,
#24818,#24819,#24820,#24821,#24822,#24823,#24824,#24825,#24826,#24827,#24828,
#24829,#24830,#24831,#24832,#24833,#24834,#24835,#24836,#24837,#24838,#24839,
#24840,#24841,#24842,#24843,#24844,#24845,#24846,#24847,#24848,#24849,#24850,
#24851,#24852,#24853,#24854,#24855,#24856,#24857,#24858,#24859,#24860,#24861,
#24862,#24863,#24864,#24865,#24866,#24867,#24868,#24869,#24870,#24871,#24872,
#24873,#24874,#24875,#24876,#24877,#24878,#24879,#24880,#24881,#24882,#24883,
#24884,#24885,#24886,#24887,#24888,#24889,#24890,#24891,#24892,#24893,#24894,
#24895,#24896,#24897,#24898,#24899,#24900,#24901,#24902,#24903,#24904,#24905,
#24906,#24907,#24908,#24909,#24910,#24911,#24912,#24913,#24914,#24915,#24916,
#24917,#24918,#24919,#24920,#24921,#24922,#24923,#24924,#24925,#24926,#24927,
#24928,#24929,#24930,#24931,#24932,#24933,#24934,#24935,#24936,#24937,#24938,
#24939,#24940,#24941,#24942,#24943,#24944,#24945,#24946,#24947,#24948,#24949,
#24950,#24951,#24952,#24953,#24954,#24955,#24956,#24957,#24958,#24959,#24960,
#24961,#24962,#24963,#24964,#24965,#24966,#24967,#24968,#24969,#24970,#24971,
#24972,#24973,#24974,#24975,#24976,#24977,#24978,#24979,#24980,#24981,#24982,
#24983,#24984,#24985,#24986,#24987,#24988,#24989,#24990,#24991,#24992,#24993,
#24994,#24995,#24996,#24997,#24998,#24999,#25000,#25001,#25002,#25003,#25004,
#25005));
#26659=AXIS2_PLACEMENT_3D('',#215380,#30631,#30632);
#26660=AXIS2_PLACEMENT_3D('',#215381,#30633,#30634);
#26661=AXIS2_PLACEMENT_3D('',#215384,#30635,#30636);
#26662=AXIS2_PLACEMENT_3D('',#215388,#30638,#30639);
#26663=AXIS2_PLACEMENT_3D('',#215390,#30641,#30642);
#26664=AXIS2_PLACEMENT_3D('',#215396,#30646,#30647);
#26665=AXIS2_PLACEMENT_3D('',#215399,#30648,#30649);
#26666=AXIS2_PLACEMENT_3D('',#215403,#30651,#30652);
#26667=AXIS2_PLACEMENT_3D('',#215405,#30654,#30655);
#26668=AXIS2_PLACEMENT_3D('',#215406,#30656,#30657);
#26669=AXIS2_PLACEMENT_3D('',#215407,#30658,#30659);
#26670=AXIS2_PLACEMENT_3D('',#215408,#30660,#30661);
#26671=AXIS2_PLACEMENT_3D('',#215411,#30662,#30663);
#26672=AXIS2_PLACEMENT_3D('',#215415,#30665,#30666);
#26673=AXIS2_PLACEMENT_3D('',#215417,#30668,#30669);
#26674=AXIS2_PLACEMENT_3D('',#215423,#30673,#30674);
#26675=AXIS2_PLACEMENT_3D('',#215426,#30675,#30676);
#26676=AXIS2_PLACEMENT_3D('',#215430,#30678,#30679);
#26677=AXIS2_PLACEMENT_3D('',#215432,#30681,#30682);
#26678=AXIS2_PLACEMENT_3D('',#215433,#30683,#30684);
#26679=AXIS2_PLACEMENT_3D('',#215434,#30685,#30686);
#26680=AXIS2_PLACEMENT_3D('',#215435,#30687,#30688);
#26681=AXIS2_PLACEMENT_3D('',#215438,#30689,#30690);
#26682=AXIS2_PLACEMENT_3D('',#215442,#30692,#30693);
#26683=AXIS2_PLACEMENT_3D('',#215444,#30695,#30696);
#26684=AXIS2_PLACEMENT_3D('',#215450,#30700,#30701);
#26685=AXIS2_PLACEMENT_3D('',#215453,#30702,#30703);
#26686=AXIS2_PLACEMENT_3D('',#215457,#30705,#30706);
#26687=AXIS2_PLACEMENT_3D('',#215459,#30708,#30709);
#26688=AXIS2_PLACEMENT_3D('',#215460,#30710,#30711);
#26689=AXIS2_PLACEMENT_3D('',#215461,#30712,#30713);
#26690=AXIS2_PLACEMENT_3D('',#215462,#30714,#30715);
#26691=AXIS2_PLACEMENT_3D('',#215465,#30716,#30717);
#26692=AXIS2_PLACEMENT_3D('',#215469,#30719,#30720);
#26693=AXIS2_PLACEMENT_3D('',#215471,#30722,#30723);
#26694=AXIS2_PLACEMENT_3D('',#215477,#30727,#30728);
#26695=AXIS2_PLACEMENT_3D('',#215480,#30729,#30730);
#26696=AXIS2_PLACEMENT_3D('',#215484,#30732,#30733);
#26697=AXIS2_PLACEMENT_3D('',#215486,#30735,#30736);
#26698=AXIS2_PLACEMENT_3D('',#215487,#30737,#30738);
#26699=AXIS2_PLACEMENT_3D('',#215488,#30739,#30740);
#26700=AXIS2_PLACEMENT_3D('',#215489,#30741,#30742);
#26701=AXIS2_PLACEMENT_3D('',#215492,#30743,#30744);
#26702=AXIS2_PLACEMENT_3D('',#215496,#30746,#30747);
#26703=AXIS2_PLACEMENT_3D('',#215498,#30749,#30750);
#26704=AXIS2_PLACEMENT_3D('',#215504,#30754,#30755);
#26705=AXIS2_PLACEMENT_3D('',#215507,#30756,#30757);
#26706=AXIS2_PLACEMENT_3D('',#215511,#30759,#30760);
#26707=AXIS2_PLACEMENT_3D('',#215513,#30762,#30763);
#26708=AXIS2_PLACEMENT_3D('',#215514,#30764,#30765);
#26709=AXIS2_PLACEMENT_3D('',#215515,#30766,#30767);
#26710=AXIS2_PLACEMENT_3D('',#215516,#30768,#30769);
#26711=AXIS2_PLACEMENT_3D('',#215519,#30770,#30771);
#26712=AXIS2_PLACEMENT_3D('',#215523,#30773,#30774);
#26713=AXIS2_PLACEMENT_3D('',#215525,#30776,#30777);
#26714=AXIS2_PLACEMENT_3D('',#215531,#30781,#30782);
#26715=AXIS2_PLACEMENT_3D('',#215534,#30783,#30784);
#26716=AXIS2_PLACEMENT_3D('',#215538,#30786,#30787);
#26717=AXIS2_PLACEMENT_3D('',#215540,#30789,#30790);
#26718=AXIS2_PLACEMENT_3D('',#215541,#30791,#30792);
#26719=AXIS2_PLACEMENT_3D('',#215542,#30793,#30794);
#26720=AXIS2_PLACEMENT_3D('',#215543,#30795,#30796);
#26721=AXIS2_PLACEMENT_3D('',#215546,#30797,#30798);
#26722=AXIS2_PLACEMENT_3D('',#215550,#30800,#30801);
#26723=AXIS2_PLACEMENT_3D('',#215552,#30803,#30804);
#26724=AXIS2_PLACEMENT_3D('',#215558,#30808,#30809);
#26725=AXIS2_PLACEMENT_3D('',#215561,#30810,#30811);
#26726=AXIS2_PLACEMENT_3D('',#215565,#30813,#30814);
#26727=AXIS2_PLACEMENT_3D('',#215567,#30816,#30817);
#26728=AXIS2_PLACEMENT_3D('',#215568,#30818,#30819);
#26729=AXIS2_PLACEMENT_3D('',#215569,#30820,#30821);
#26730=AXIS2_PLACEMENT_3D('',#215570,#30822,#30823);
#26731=AXIS2_PLACEMENT_3D('',#215573,#30824,#30825);
#26732=AXIS2_PLACEMENT_3D('',#215577,#30827,#30828);
#26733=AXIS2_PLACEMENT_3D('',#215579,#30830,#30831);
#26734=AXIS2_PLACEMENT_3D('',#215585,#30835,#30836);
#26735=AXIS2_PLACEMENT_3D('',#215588,#30837,#30838);
#26736=AXIS2_PLACEMENT_3D('',#215592,#30840,#30841);
#26737=AXIS2_PLACEMENT_3D('',#215594,#30843,#30844);
#26738=AXIS2_PLACEMENT_3D('',#215595,#30845,#30846);
#26739=AXIS2_PLACEMENT_3D('',#215596,#30847,#30848);
#26740=AXIS2_PLACEMENT_3D('',#215597,#30849,#30850);
#26741=AXIS2_PLACEMENT_3D('',#215600,#30851,#30852);
#26742=AXIS2_PLACEMENT_3D('',#215604,#30854,#30855);
#26743=AXIS2_PLACEMENT_3D('',#215606,#30857,#30858);
#26744=AXIS2_PLACEMENT_3D('',#215612,#30862,#30863);
#26745=AXIS2_PLACEMENT_3D('',#215615,#30864,#30865);
#26746=AXIS2_PLACEMENT_3D('',#215619,#30867,#30868);
#26747=AXIS2_PLACEMENT_3D('',#215621,#30870,#30871);
#26748=AXIS2_PLACEMENT_3D('',#215622,#30872,#30873);
#26749=AXIS2_PLACEMENT_3D('',#215623,#30874,#30875);
#26750=AXIS2_PLACEMENT_3D('',#215624,#30876,#30877);
#26751=AXIS2_PLACEMENT_3D('',#215627,#30878,#30879);
#26752=AXIS2_PLACEMENT_3D('',#215631,#30881,#30882);
#26753=AXIS2_PLACEMENT_3D('',#215633,#30884,#30885);
#26754=AXIS2_PLACEMENT_3D('',#215639,#30889,#30890);
#26755=AXIS2_PLACEMENT_3D('',#215642,#30891,#30892);
#26756=AXIS2_PLACEMENT_3D('',#215646,#30894,#30895);
#26757=AXIS2_PLACEMENT_3D('',#215648,#30897,#30898);
#26758=AXIS2_PLACEMENT_3D('',#215649,#30899,#30900);
#26759=AXIS2_PLACEMENT_3D('',#215650,#30901,#30902);
#26760=AXIS2_PLACEMENT_3D('',#215651,#30903,#30904);
#26761=AXIS2_PLACEMENT_3D('',#215654,#30905,#30906);
#26762=AXIS2_PLACEMENT_3D('',#215658,#30908,#30909);
#26763=AXIS2_PLACEMENT_3D('',#215660,#30911,#30912);
#26764=AXIS2_PLACEMENT_3D('',#215666,#30916,#30917);
#26765=AXIS2_PLACEMENT_3D('',#215669,#30918,#30919);
#26766=AXIS2_PLACEMENT_3D('',#215673,#30921,#30922);
#26767=AXIS2_PLACEMENT_3D('',#215675,#30924,#30925);
#26768=AXIS2_PLACEMENT_3D('',#215676,#30926,#30927);
#26769=AXIS2_PLACEMENT_3D('',#215677,#30928,#30929);
#26770=AXIS2_PLACEMENT_3D('',#215678,#30930,#30931);
#26771=AXIS2_PLACEMENT_3D('',#215681,#30932,#30933);
#26772=AXIS2_PLACEMENT_3D('',#215685,#30935,#30936);
#26773=AXIS2_PLACEMENT_3D('',#215687,#30938,#30939);
#26774=AXIS2_PLACEMENT_3D('',#215693,#30943,#30944);
#26775=AXIS2_PLACEMENT_3D('',#215696,#30945,#30946);
#26776=AXIS2_PLACEMENT_3D('',#215700,#30948,#30949);
#26777=AXIS2_PLACEMENT_3D('',#215702,#30951,#30952);
#26778=AXIS2_PLACEMENT_3D('',#215703,#30953,#30954);
#26779=AXIS2_PLACEMENT_3D('',#215704,#30955,#30956);
#26780=AXIS2_PLACEMENT_3D('',#215705,#30957,#30958);
#26781=AXIS2_PLACEMENT_3D('',#215708,#30959,#30960);
#26782=AXIS2_PLACEMENT_3D('',#215712,#30962,#30963);
#26783=AXIS2_PLACEMENT_3D('',#215714,#30965,#30966);
#26784=AXIS2_PLACEMENT_3D('',#215720,#30970,#30971);
#26785=AXIS2_PLACEMENT_3D('',#215723,#30972,#30973);
#26786=AXIS2_PLACEMENT_3D('',#215727,#30975,#30976);
#26787=AXIS2_PLACEMENT_3D('',#215729,#30978,#30979);
#26788=AXIS2_PLACEMENT_3D('',#215730,#30980,#30981);
#26789=AXIS2_PLACEMENT_3D('',#215731,#30982,#30983);
#26790=AXIS2_PLACEMENT_3D('',#215732,#30984,#30985);
#26791=AXIS2_PLACEMENT_3D('',#215735,#30986,#30987);
#26792=AXIS2_PLACEMENT_3D('',#215739,#30989,#30990);
#26793=AXIS2_PLACEMENT_3D('',#215741,#30992,#30993);
#26794=AXIS2_PLACEMENT_3D('',#215747,#30997,#30998);
#26795=AXIS2_PLACEMENT_3D('',#215750,#30999,#31000);
#26796=AXIS2_PLACEMENT_3D('',#215754,#31002,#31003);
#26797=AXIS2_PLACEMENT_3D('',#215756,#31005,#31006);
#26798=AXIS2_PLACEMENT_3D('',#215757,#31007,#31008);
#26799=AXIS2_PLACEMENT_3D('',#215758,#31009,#31010);
#26800=AXIS2_PLACEMENT_3D('',#215759,#31011,#31012);
#26801=AXIS2_PLACEMENT_3D('',#215762,#31013,#31014);
#26802=AXIS2_PLACEMENT_3D('',#215766,#31016,#31017);
#26803=AXIS2_PLACEMENT_3D('',#215768,#31019,#31020);
#26804=AXIS2_PLACEMENT_3D('',#215774,#31024,#31025);
#26805=AXIS2_PLACEMENT_3D('',#215777,#31026,#31027);
#26806=AXIS2_PLACEMENT_3D('',#215781,#31029,#31030);
#26807=AXIS2_PLACEMENT_3D('',#215783,#31032,#31033);
#26808=AXIS2_PLACEMENT_3D('',#215784,#31034,#31035);
#26809=AXIS2_PLACEMENT_3D('',#215785,#31036,#31037);
#26810=AXIS2_PLACEMENT_3D('',#215786,#31038,#31039);
#26811=AXIS2_PLACEMENT_3D('',#215789,#31040,#31041);
#26812=AXIS2_PLACEMENT_3D('',#215793,#31043,#31044);
#26813=AXIS2_PLACEMENT_3D('',#215795,#31046,#31047);
#26814=AXIS2_PLACEMENT_3D('',#215801,#31051,#31052);
#26815=AXIS2_PLACEMENT_3D('',#215804,#31053,#31054);
#26816=AXIS2_PLACEMENT_3D('',#215808,#31056,#31057);
#26817=AXIS2_PLACEMENT_3D('',#215810,#31059,#31060);
#26818=AXIS2_PLACEMENT_3D('',#215811,#31061,#31062);
#26819=AXIS2_PLACEMENT_3D('',#215812,#31063,#31064);
#26820=AXIS2_PLACEMENT_3D('',#215813,#31065,#31066);
#26821=AXIS2_PLACEMENT_3D('',#215816,#31067,#31068);
#26822=AXIS2_PLACEMENT_3D('',#215820,#31070,#31071);
#26823=AXIS2_PLACEMENT_3D('',#215822,#31073,#31074);
#26824=AXIS2_PLACEMENT_3D('',#215828,#31078,#31079);
#26825=AXIS2_PLACEMENT_3D('',#215831,#31080,#31081);
#26826=AXIS2_PLACEMENT_3D('',#215835,#31083,#31084);
#26827=AXIS2_PLACEMENT_3D('',#215837,#31086,#31087);
#26828=AXIS2_PLACEMENT_3D('',#215838,#31088,#31089);
#26829=AXIS2_PLACEMENT_3D('',#215839,#31090,#31091);
#26830=AXIS2_PLACEMENT_3D('',#215840,#31092,#31093);
#26831=AXIS2_PLACEMENT_3D('',#215843,#31094,#31095);
#26832=AXIS2_PLACEMENT_3D('',#215847,#31097,#31098);
#26833=AXIS2_PLACEMENT_3D('',#215849,#31100,#31101);
#26834=AXIS2_PLACEMENT_3D('',#215855,#31105,#31106);
#26835=AXIS2_PLACEMENT_3D('',#215858,#31107,#31108);
#26836=AXIS2_PLACEMENT_3D('',#215862,#31110,#31111);
#26837=AXIS2_PLACEMENT_3D('',#215864,#31113,#31114);
#26838=AXIS2_PLACEMENT_3D('',#215865,#31115,#31116);
#26839=AXIS2_PLACEMENT_3D('',#215866,#31117,#31118);
#26840=AXIS2_PLACEMENT_3D('',#215867,#31119,#31120);
#26841=AXIS2_PLACEMENT_3D('',#215870,#31121,#31122);
#26842=AXIS2_PLACEMENT_3D('',#215874,#31124,#31125);
#26843=AXIS2_PLACEMENT_3D('',#215876,#31127,#31128);
#26844=AXIS2_PLACEMENT_3D('',#215882,#31132,#31133);
#26845=AXIS2_PLACEMENT_3D('',#215885,#31134,#31135);
#26846=AXIS2_PLACEMENT_3D('',#215889,#31137,#31138);
#26847=AXIS2_PLACEMENT_3D('',#215891,#31140,#31141);
#26848=AXIS2_PLACEMENT_3D('',#215892,#31142,#31143);
#26849=AXIS2_PLACEMENT_3D('',#215893,#31144,#31145);
#26850=AXIS2_PLACEMENT_3D('',#215894,#31146,#31147);
#26851=AXIS2_PLACEMENT_3D('',#215897,#31148,#31149);
#26852=AXIS2_PLACEMENT_3D('',#215901,#31151,#31152);
#26853=AXIS2_PLACEMENT_3D('',#215903,#31154,#31155);
#26854=AXIS2_PLACEMENT_3D('',#215909,#31159,#31160);
#26855=AXIS2_PLACEMENT_3D('',#215912,#31161,#31162);
#26856=AXIS2_PLACEMENT_3D('',#215916,#31164,#31165);
#26857=AXIS2_PLACEMENT_3D('',#215918,#31167,#31168);
#26858=AXIS2_PLACEMENT_3D('',#215919,#31169,#31170);
#26859=AXIS2_PLACEMENT_3D('',#215920,#31171,#31172);
#26860=AXIS2_PLACEMENT_3D('',#215921,#31173,#31174);
#26861=AXIS2_PLACEMENT_3D('',#215924,#31175,#31176);
#26862=AXIS2_PLACEMENT_3D('',#215928,#31178,#31179);
#26863=AXIS2_PLACEMENT_3D('',#215930,#31181,#31182);
#26864=AXIS2_PLACEMENT_3D('',#215936,#31186,#31187);
#26865=AXIS2_PLACEMENT_3D('',#215939,#31188,#31189);
#26866=AXIS2_PLACEMENT_3D('',#215943,#31191,#31192);
#26867=AXIS2_PLACEMENT_3D('',#215945,#31194,#31195);
#26868=AXIS2_PLACEMENT_3D('',#215946,#31196,#31197);
#26869=AXIS2_PLACEMENT_3D('',#215947,#31198,#31199);
#26870=AXIS2_PLACEMENT_3D('',#215948,#31200,#31201);
#26871=AXIS2_PLACEMENT_3D('',#215951,#31202,#31203);
#26872=AXIS2_PLACEMENT_3D('',#215955,#31205,#31206);
#26873=AXIS2_PLACEMENT_3D('',#215957,#31208,#31209);
#26874=AXIS2_PLACEMENT_3D('',#215963,#31213,#31214);
#26875=AXIS2_PLACEMENT_3D('',#215966,#31215,#31216);
#26876=AXIS2_PLACEMENT_3D('',#215970,#31218,#31219);
#26877=AXIS2_PLACEMENT_3D('',#215972,#31221,#31222);
#26878=AXIS2_PLACEMENT_3D('',#215973,#31223,#31224);
#26879=AXIS2_PLACEMENT_3D('',#215974,#31225,#31226);
#26880=AXIS2_PLACEMENT_3D('',#215975,#31227,#31228);
#26881=AXIS2_PLACEMENT_3D('',#215978,#31229,#31230);
#26882=AXIS2_PLACEMENT_3D('',#215982,#31232,#31233);
#26883=AXIS2_PLACEMENT_3D('',#215984,#31235,#31236);
#26884=AXIS2_PLACEMENT_3D('',#215990,#31240,#31241);
#26885=AXIS2_PLACEMENT_3D('',#215993,#31242,#31243);
#26886=AXIS2_PLACEMENT_3D('',#215997,#31245,#31246);
#26887=AXIS2_PLACEMENT_3D('',#215999,#31248,#31249);
#26888=AXIS2_PLACEMENT_3D('',#216000,#31250,#31251);
#26889=AXIS2_PLACEMENT_3D('',#216001,#31252,#31253);
#26890=AXIS2_PLACEMENT_3D('',#216002,#31254,#31255);
#26891=AXIS2_PLACEMENT_3D('',#217654,#31261,#31262);
#26892=AXIS2_PLACEMENT_3D('',#219306,#31268,#31269);
#26893=AXIS2_PLACEMENT_3D('',#220958,#31275,#31276);
#26894=AXIS2_PLACEMENT_3D('',#222610,#31282,#31283);
#26895=AXIS2_PLACEMENT_3D('',#224262,#31289,#31290);
#26896=AXIS2_PLACEMENT_3D('',#225914,#31296,#31297);
#26897=AXIS2_PLACEMENT_3D('',#227566,#31303,#31304);
#26898=AXIS2_PLACEMENT_3D('',#229218,#31310,#31311);
#26899=AXIS2_PLACEMENT_3D('',#230870,#31317,#31318);
#26900=AXIS2_PLACEMENT_3D('',#232522,#31324,#31325);
#26901=AXIS2_PLACEMENT_3D('',#234174,#31331,#31332);
#26902=AXIS2_PLACEMENT_3D('',#235826,#31338,#31339);
#26903=AXIS2_PLACEMENT_3D('',#237478,#31345,#31346);
#26904=AXIS2_PLACEMENT_3D('',#239130,#31352,#31353);
#26905=AXIS2_PLACEMENT_3D('',#240782,#31359,#31360);
#26906=AXIS2_PLACEMENT_3D('',#242434,#31366,#31367);
#26907=AXIS2_PLACEMENT_3D('',#244086,#31373,#31374);
#26908=AXIS2_PLACEMENT_3D('',#245738,#31380,#31381);
#26909=AXIS2_PLACEMENT_3D('',#247390,#31387,#31388);
#26910=AXIS2_PLACEMENT_3D('',#249042,#31394,#31395);
#26911=AXIS2_PLACEMENT_3D('',#250694,#31401,#31402);
#26912=AXIS2_PLACEMENT_3D('',#252346,#31408,#31409);
#26913=AXIS2_PLACEMENT_3D('',#253998,#31415,#31416);
#26914=AXIS2_PLACEMENT_3D('',#253999,#31417,#31418);
#26915=AXIS2_PLACEMENT_3D('',#254000,#31419,#31420);
#26916=AXIS2_PLACEMENT_3D('',#254001,#31421,#31422);
#26917=AXIS2_PLACEMENT_3D('',#254002,#31423,#31424);
#26918=AXIS2_PLACEMENT_3D('',#254003,#31425,#31426);
#26919=AXIS2_PLACEMENT_3D('',#254004,#31427,#31428);
#26920=AXIS2_PLACEMENT_3D('',#254005,#31429,#31430);
#26921=AXIS2_PLACEMENT_3D('',#254006,#31431,#31432);
#26922=AXIS2_PLACEMENT_3D('',#254007,#31433,#31434);
#26923=AXIS2_PLACEMENT_3D('',#254008,#31435,#31436);
#26924=AXIS2_PLACEMENT_3D('',#254009,#31437,#31438);
#26925=AXIS2_PLACEMENT_3D('',#254010,#31439,#31440);
#26926=AXIS2_PLACEMENT_3D('',#254011,#31441,#31442);
#26927=AXIS2_PLACEMENT_3D('',#254012,#31443,#31444);
#26928=AXIS2_PLACEMENT_3D('',#254013,#31445,#31446);
#26929=AXIS2_PLACEMENT_3D('',#254014,#31447,#31448);
#26930=AXIS2_PLACEMENT_3D('',#254015,#31449,#31450);
#26931=AXIS2_PLACEMENT_3D('',#254016,#31451,#31452);
#26932=AXIS2_PLACEMENT_3D('',#254017,#31453,#31454);
#26933=AXIS2_PLACEMENT_3D('',#254018,#31455,#31456);
#26934=AXIS2_PLACEMENT_3D('',#254019,#31457,#31458);
#26935=AXIS2_PLACEMENT_3D('',#254020,#31459,#31460);
#26936=AXIS2_PLACEMENT_3D('',#254022,#31461,#31462);
#26937=AXIS2_PLACEMENT_3D('',#254232,#31464,#31465);
#26938=AXIS2_PLACEMENT_3D('',#254234,#31466,#31467);
#26939=AXIS2_PLACEMENT_3D('',#254236,#31468,#31469);
#26940=AXIS2_PLACEMENT_3D('',#254445,#31471,#31472);
#26941=AXIS2_PLACEMENT_3D('',#254447,#31473,#31474);
#26942=AXIS2_PLACEMENT_3D('',#254448,#31475,#31476);
#26943=AXIS2_PLACEMENT_3D('',#254450,#31477,#31478);
#26944=AXIS2_PLACEMENT_3D('',#254660,#31480,#31481);
#26945=AXIS2_PLACEMENT_3D('',#254662,#31482,#31483);
#26946=AXIS2_PLACEMENT_3D('',#254664,#31484,#31485);
#26947=AXIS2_PLACEMENT_3D('',#254873,#31487,#31488);
#26948=AXIS2_PLACEMENT_3D('',#254874,#31489,#31490);
#26949=AXIS2_PLACEMENT_3D('',#254875,#31491,#31492);
#26950=AXIS2_PLACEMENT_3D('',#254876,#31493,#31494);
#26951=AXIS2_PLACEMENT_3D('',#254877,#31495,#31496);
#26952=AXIS2_PLACEMENT_3D('',#254878,#31497,#31498);
#26953=AXIS2_PLACEMENT_3D('',#254879,#31499,#31500);
#26954=AXIS2_PLACEMENT_3D('',#254880,#31501,#31502);
#26955=AXIS2_PLACEMENT_3D('',#254881,#31503,#31504);
#26956=AXIS2_PLACEMENT_3D('',#254882,#31505,#31506);
#26957=AXIS2_PLACEMENT_3D('',#254883,#31507,#31508);
#26958=AXIS2_PLACEMENT_3D('',#254884,#31509,#31510);
#26959=AXIS2_PLACEMENT_3D('',#254885,#31511,#31512);
#26960=AXIS2_PLACEMENT_3D('',#254886,#31513,#31514);
#26961=AXIS2_PLACEMENT_3D('',#254887,#31515,#31516);
#26962=AXIS2_PLACEMENT_3D('',#254888,#31517,#31518);
#26963=AXIS2_PLACEMENT_3D('',#254889,#31519,#31520);
#26964=AXIS2_PLACEMENT_3D('',#254890,#31521,#31522);
#26965=AXIS2_PLACEMENT_3D('',#254891,#31523,#31524);
#26966=AXIS2_PLACEMENT_3D('',#254892,#31525,#31526);
#26967=AXIS2_PLACEMENT_3D('',#254893,#31527,#31528);
#26968=AXIS2_PLACEMENT_3D('',#254894,#31529,#31530);
#26969=AXIS2_PLACEMENT_3D('',#254895,#31531,#31532);
#26970=AXIS2_PLACEMENT_3D('',#254897,#31533,#31534);
#26971=AXIS2_PLACEMENT_3D('',#254898,#31535,#31536);
#26972=AXIS2_PLACEMENT_3D('',#254900,#31538,#31539);
#26973=AXIS2_PLACEMENT_3D('',#254901,#31540,#31541);
#26974=AXIS2_PLACEMENT_3D('',#254902,#31542,#31543);
#26975=AXIS2_PLACEMENT_3D('',#254903,#31544,#31545);
#26976=AXIS2_PLACEMENT_3D('',#254904,#31546,#31547);
#26977=AXIS2_PLACEMENT_3D('',#254905,#31548,#31549);
#26978=AXIS2_PLACEMENT_3D('',#254906,#31550,#31551);
#26979=AXIS2_PLACEMENT_3D('',#254907,#31552,#31553);
#26980=AXIS2_PLACEMENT_3D('',#254908,#31554,#31555);
#26981=AXIS2_PLACEMENT_3D('',#254909,#31556,#31557);
#26982=AXIS2_PLACEMENT_3D('',#254910,#31558,#31559);
#26983=AXIS2_PLACEMENT_3D('',#254911,#31560,#31561);
#26984=AXIS2_PLACEMENT_3D('',#254912,#31562,#31563);
#26985=AXIS2_PLACEMENT_3D('',#254913,#31564,#31565);
#26986=AXIS2_PLACEMENT_3D('',#254914,#31566,#31567);
#26987=AXIS2_PLACEMENT_3D('',#254915,#31568,#31569);
#26988=AXIS2_PLACEMENT_3D('',#254916,#31570,#31571);
#26989=AXIS2_PLACEMENT_3D('',#254917,#31572,#31573);
#26990=AXIS2_PLACEMENT_3D('',#254918,#31574,#31575);
#26991=AXIS2_PLACEMENT_3D('',#254919,#31576,#31577);
#26992=AXIS2_PLACEMENT_3D('',#254920,#31578,#31579);
#26993=AXIS2_PLACEMENT_3D('',#254921,#31580,#31581);
#26994=AXIS2_PLACEMENT_3D('',#254922,#31582,#31583);
#26995=AXIS2_PLACEMENT_3D('',#254925,#31586,#31587);
#26996=AXIS2_PLACEMENT_3D('',#254927,#31589,#31590);
#26997=AXIS2_PLACEMENT_3D('',#254930,#31593,#31594);
#26998=AXIS2_PLACEMENT_3D('',#254931,#31595,#31596);
#26999=AXIS2_PLACEMENT_3D('',#255754,#31599,#31600);
#27000=AXIS2_PLACEMENT_3D('',#255756,#31602,#31603);
#30631=DIRECTION('axis',(0.,0.,1.));
#30632=DIRECTION('refdir',(1.,0.,0.));
#30633=DIRECTION('center_axis',(0.,0.,1.));
#30634=DIRECTION('ref_axis',(-0.640971010199212,0.767565087848712,0.));
#30635=DIRECTION('center_axis',(0.,0.,-1.));
#30636=DIRECTION('ref_axis',(-0.640971010199212,0.767565087848712,0.));
#30637=DIRECTION('',(0.,0.,1.));
#30638=DIRECTION('center_axis',(0.,0.,1.));
#30639=DIRECTION('ref_axis',(-0.640971010199212,0.767565087848712,0.));
#30640=DIRECTION('',(0.,0.,-1.));
#30641=DIRECTION('center_axis',(0.0781910030252328,0.996938396815926,0.));
#30642=DIRECTION('ref_axis',(-0.996938396815926,0.0781910030252328,0.));
#30643=DIRECTION('',(-0.996938396815926,0.0781910030252328,0.));
#30644=DIRECTION('',(0.,0.,1.));
#30645=DIRECTION('',(0.996938396815926,-0.0781910030252328,0.));
#30646=DIRECTION('center_axis',(0.,0.,1.));
#30647=DIRECTION('ref_axis',(-0.817790915745045,-0.575515436912756,0.));
#30648=DIRECTION('center_axis',(0.,0.,-1.));
#30649=DIRECTION('ref_axis',(-0.817790915745045,-0.575515436912756,0.));
#30650=DIRECTION('',(0.,0.,1.));
#30651=DIRECTION('center_axis',(0.,0.,1.));
#30652=DIRECTION('ref_axis',(-0.817790915745045,-0.575515436912756,0.));
#30653=DIRECTION('',(0.,0.,-1.));
#30654=DIRECTION('center_axis',(0.,0.,1.));
#30655=DIRECTION('ref_axis',(0.983205865442321,-0.18249993468442,0.));
#30656=DIRECTION('center_axis',(0.,0.,1.));
#30657=DIRECTION('ref_axis',(0.983205865442321,-0.18249993468442,0.));
#30658=DIRECTION('center_axis',(0.,0.,-1.));
#30659=DIRECTION('ref_axis',(0.983205865442321,-0.18249993468442,0.));
#30660=DIRECTION('center_axis',(0.,0.,1.));
#30661=DIRECTION('ref_axis',(-0.420469989562984,0.907306446509064,0.));
#30662=DIRECTION('center_axis',(0.,0.,-1.));
#30663=DIRECTION('ref_axis',(-0.420469989562984,0.907306446509064,0.));
#30664=DIRECTION('',(0.,0.,1.));
#30665=DIRECTION('center_axis',(0.,0.,1.));
#30666=DIRECTION('ref_axis',(-0.420469989562984,0.907306446509064,0.));
#30667=DIRECTION('',(0.,0.,-1.));
#30668=DIRECTION('center_axis',(0.333553353095455,0.942731223965123,0.));
#30669=DIRECTION('ref_axis',(-0.942731223965123,0.333553353095455,0.));
#30670=DIRECTION('',(-0.942731223965123,0.333553353095455,0.));
#30671=DIRECTION('',(0.,0.,1.));
#30672=DIRECTION('',(0.942731223965123,-0.333553353095455,0.));
#30673=DIRECTION('center_axis',(0.,0.,1.));
#30674=DIRECTION('ref_axis',(-0.93887972184625,-0.344245360035407,0.));
#30675=DIRECTION('center_axis',(0.,0.,-1.));
#30676=DIRECTION('ref_axis',(-0.93887972184625,-0.344245360035407,0.));
#30677=DIRECTION('',(0.,0.,1.));
#30678=DIRECTION('center_axis',(0.,0.,1.));
#30679=DIRECTION('ref_axis',(-0.93887972184625,-0.344245360035407,0.));
#30680=DIRECTION('',(0.,0.,-1.));
#30681=DIRECTION('center_axis',(0.,0.,1.));
#30682=DIRECTION('ref_axis',(0.902469479163338,-0.430753803440728,0.));
#30683=DIRECTION('center_axis',(0.,0.,1.));
#30684=DIRECTION('ref_axis',(0.902469479163338,-0.430753803440728,0.));
#30685=DIRECTION('center_axis',(0.,0.,-1.));
#30686=DIRECTION('ref_axis',(0.902469479163338,-0.430753803440728,0.));
#30687=DIRECTION('center_axis',(0.,0.,1.));
#30688=DIRECTION('ref_axis',(-0.171314633997541,0.985216370234624,0.));
#30689=DIRECTION('center_axis',(0.,0.,-1.));
#30690=DIRECTION('ref_axis',(-0.171314633997541,0.985216370234624,0.));
#30691=DIRECTION('',(0.,0.,1.));
#30692=DIRECTION('center_axis',(0.,0.,1.));
#30693=DIRECTION('ref_axis',(-0.171314633997541,0.985216370234624,0.));
#30694=DIRECTION('',(0.,0.,-1.));
#30695=DIRECTION('center_axis',(0.5661845933752,0.824278476138107,0.));
#30696=DIRECTION('ref_axis',(-0.824278476138107,0.5661845933752,0.));
#30697=DIRECTION('',(-0.824278476138107,0.5661845933752,0.));
#30698=DIRECTION('',(0.,0.,1.));
#30699=DIRECTION('',(0.824278476138107,-0.5661845933752,0.));
#30700=DIRECTION('center_axis',(0.,0.,1.));
#30701=DIRECTION('ref_axis',(-0.995985426475728,-0.0895155307640121,0.));
#30702=DIRECTION('center_axis',(0.,0.,-1.));
#30703=DIRECTION('ref_axis',(-0.995985426475728,-0.0895155307640121,0.));
#30704=DIRECTION('',(0.,0.,1.));
#30705=DIRECTION('center_axis',(0.,0.,1.));
#30706=DIRECTION('ref_axis',(-0.995985426475728,-0.0895155307640121,0.));
#30707=DIRECTION('',(0.,0.,-1.));
#30708=DIRECTION('center_axis',(0.,0.,1.));
#30709=DIRECTION('ref_axis',(0.760231289280704,-0.649652512346868,0.));
#30710=DIRECTION('center_axis',(0.,0.,1.));
#30711=DIRECTION('ref_axis',(0.760231289280704,-0.649652512346868,0.));
#30712=DIRECTION('center_axis',(0.,0.,-1.));
#30713=DIRECTION('ref_axis',(0.760231289280704,-0.649652512346868,0.));
#30714=DIRECTION('center_axis',(0.,0.,1.));
#30715=DIRECTION('ref_axis',(0.0895155307640188,0.995985426475727,0.));
#30716=DIRECTION('center_axis',(0.,0.,-1.));
#30717=DIRECTION('ref_axis',(0.0895155307640188,0.995985426475727,0.));
#30718=DIRECTION('',(0.,0.,1.));
#30719=DIRECTION('center_axis',(0.,0.,1.));
#30720=DIRECTION('ref_axis',(0.0895155307640188,0.995985426475727,0.));
#30721=DIRECTION('',(0.,0.,-1.));
#30722=DIRECTION('center_axis',(0.760231289280706,0.649652512346866,0.));
#30723=DIRECTION('ref_axis',(-0.649652512346866,0.760231289280706,0.));
#30724=DIRECTION('',(-0.649652512346866,0.760231289280706,0.));
#30725=DIRECTION('',(0.,0.,1.));
#30726=DIRECTION('',(0.649652512346866,-0.760231289280706,0.));
#30727=DIRECTION('center_axis',(0.,0.,1.));
#30728=DIRECTION('ref_axis',(-0.985216370234624,0.171314633997541,0.));
#30729=DIRECTION('center_axis',(0.,0.,-1.));
#30730=DIRECTION('ref_axis',(-0.985216370234624,0.171314633997541,0.));
#30731=DIRECTION('',(0.,0.,1.));
#30732=DIRECTION('center_axis',(0.,0.,1.));
#30733=DIRECTION('ref_axis',(-0.985216370234624,0.171314633997541,0.));
#30734=DIRECTION('',(0.,0.,-1.));
#30735=DIRECTION('center_axis',(0.,0.,1.));
#30736=DIRECTION('ref_axis',(0.566184593375197,-0.824278476138108,0.));
#30737=DIRECTION('center_axis',(0.,0.,1.));
#30738=DIRECTION('ref_axis',(0.566184593375197,-0.824278476138108,0.));
#30739=DIRECTION('center_axis',(0.,0.,-1.));
#30740=DIRECTION('ref_axis',(0.566184593375197,-0.824278476138108,0.));
#30741=DIRECTION('center_axis',(0.,0.,1.));
#30742=DIRECTION('ref_axis',(0.344245360035407,0.938879721846251,0.));
#30743=DIRECTION('center_axis',(0.,0.,-1.));
#30744=DIRECTION('ref_axis',(0.344245360035407,0.938879721846251,0.));
#30745=DIRECTION('',(0.,0.,1.));
#30746=DIRECTION('center_axis',(0.,0.,1.));
#30747=DIRECTION('ref_axis',(0.344245360035407,0.938879721846251,0.));
#30748=DIRECTION('',(0.,0.,-1.));
#30749=DIRECTION('center_axis',(0.902469479163339,0.430753803440726,0.));
#30750=DIRECTION('ref_axis',(-0.430753803440726,0.902469479163339,0.));
#30751=DIRECTION('',(-0.430753803440726,0.902469479163339,0.));
#30752=DIRECTION('',(0.,0.,1.));
#30753=DIRECTION('',(0.430753803440726,-0.902469479163339,0.));
#30754=DIRECTION('center_axis',(0.,0.,1.));
#30755=DIRECTION('ref_axis',(-0.907306446509064,0.420469989562983,0.));
#30756=DIRECTION('center_axis',(0.,0.,-1.));
#30757=DIRECTION('ref_axis',(-0.907306446509064,0.420469989562983,0.));
#30758=DIRECTION('',(0.,0.,1.));
#30759=DIRECTION('center_axis',(0.,0.,1.));
#30760=DIRECTION('ref_axis',(-0.907306446509064,0.420469989562983,0.));
#30761=DIRECTION('',(0.,0.,-1.));
#30762=DIRECTION('center_axis',(0.,0.,1.));
#30763=DIRECTION('ref_axis',(0.333553353095452,-0.942731223965124,0.));
#30764=DIRECTION('center_axis',(0.,0.,1.));
#30765=DIRECTION('ref_axis',(0.333553353095452,-0.942731223965124,0.));
#30766=DIRECTION('center_axis',(0.,0.,-1.));
#30767=DIRECTION('ref_axis',(0.333553353095452,-0.942731223965124,0.));
#30768=DIRECTION('center_axis',(0.,0.,1.));
#30769=DIRECTION('ref_axis',(0.575515436912747,0.817790915745051,0.));
#30770=DIRECTION('center_axis',(0.,0.,-1.));
#30771=DIRECTION('ref_axis',(0.575515436912747,0.817790915745051,0.));
#30772=DIRECTION('',(0.,0.,1.));
#30773=DIRECTION('center_axis',(0.,0.,1.));
#30774=DIRECTION('ref_axis',(0.575515436912747,0.817790915745051,0.));
#30775=DIRECTION('',(0.,0.,-1.));
#30776=DIRECTION('center_axis',(0.983205865442321,0.182499934684417,0.));
#30777=DIRECTION('ref_axis',(-0.182499934684417,0.983205865442321,0.));
#30778=DIRECTION('',(-0.182499934684417,0.983205865442321,0.));
#30779=DIRECTION('',(0.,0.,1.));
#30780=DIRECTION('',(0.182499934684417,-0.983205865442321,0.));
#30781=DIRECTION('center_axis',(0.,0.,1.));
#30782=DIRECTION('ref_axis',(-0.767565087848714,0.64097101019921,0.));
#30783=DIRECTION('center_axis',(0.,0.,-1.));
#30784=DIRECTION('ref_axis',(-0.767565087848714,0.64097101019921,0.));
#30785=DIRECTION('',(0.,0.,1.));
#30786=DIRECTION('center_axis',(0.,0.,1.));
#30787=DIRECTION('ref_axis',(-0.767565087848714,0.64097101019921,0.));
#30788=DIRECTION('',(0.,0.,-1.));
#30789=DIRECTION('center_axis',(0.,0.,1.));
#30790=DIRECTION('ref_axis',(0.07819100302523,-0.996938396815926,0.));
#30791=DIRECTION('center_axis',(0.,0.,1.));
#30792=DIRECTION('ref_axis',(0.07819100302523,-0.996938396815926,0.));
#30793=DIRECTION('center_axis',(0.,0.,-1.));
#30794=DIRECTION('ref_axis',(0.07819100302523,-0.996938396815926,0.));
#30795=DIRECTION('center_axis',(0.,0.,1.));
#30796=DIRECTION('ref_axis',(0.767565087848712,0.640971010199212,0.));
#30797=DIRECTION('center_axis',(0.,0.,-1.));
#30798=DIRECTION('ref_axis',(0.767565087848712,0.640971010199212,0.));
#30799=DIRECTION('',(0.,0.,1.));
#30800=DIRECTION('center_axis',(0.,0.,1.));
#30801=DIRECTION('ref_axis',(0.767565087848712,0.640971010199212,0.));
#30802=DIRECTION('',(0.,0.,-1.));
#30803=DIRECTION('center_axis',(0.996938396815926,-0.0781910030252327,0.));
#30804=DIRECTION('ref_axis',(0.0781910030252327,0.996938396815926,0.));
#30805=DIRECTION('',(0.0781910030252327,0.996938396815926,0.));
#30806=DIRECTION('',(0.,0.,1.));
#30807=DIRECTION('',(-0.0781910030252327,-0.996938396815926,0.));
#30808=DIRECTION('center_axis',(0.,0.,1.));
#30809=DIRECTION('ref_axis',(-0.575515436912756,0.817790915745045,0.));
#30810=DIRECTION('center_axis',(0.,0.,-1.));
#30811=DIRECTION('ref_axis',(-0.575515436912756,0.817790915745045,0.));
#30812=DIRECTION('',(0.,0.,1.));
#30813=DIRECTION('center_axis',(0.,0.,1.));
#30814=DIRECTION('ref_axis',(-0.575515436912756,0.817790915745045,0.));
#30815=DIRECTION('',(0.,0.,-1.));
#30816=DIRECTION('center_axis',(0.,0.,1.));
#30817=DIRECTION('ref_axis',(-0.18249993468442,-0.983205865442321,0.));
#30818=DIRECTION('center_axis',(0.,0.,1.));
#30819=DIRECTION('ref_axis',(-0.18249993468442,-0.983205865442321,0.));
#30820=DIRECTION('center_axis',(0.,0.,-1.));
#30821=DIRECTION('ref_axis',(-0.18249993468442,-0.983205865442321,0.));
#30822=DIRECTION('center_axis',(0.,0.,1.));
#30823=DIRECTION('ref_axis',(0.907306446509064,0.420469989562984,0.));
#30824=DIRECTION('center_axis',(0.,0.,-1.));
#30825=DIRECTION('ref_axis',(0.907306446509064,0.420469989562984,0.));
#30826=DIRECTION('',(0.,0.,1.));
#30827=DIRECTION('center_axis',(0.,0.,1.));
#30828=DIRECTION('ref_axis',(0.907306446509064,0.420469989562984,0.));
#30829=DIRECTION('',(0.,0.,-1.));
#30830=DIRECTION('center_axis',(0.942731223965123,-0.333553353095455,0.));
#30831=DIRECTION('ref_axis',(0.333553353095455,0.942731223965123,0.));
#30832=DIRECTION('',(0.333553353095455,0.942731223965123,0.));
#30833=DIRECTION('',(0.,0.,1.));
#30834=DIRECTION('',(-0.333553353095455,-0.942731223965123,0.));
#30835=DIRECTION('center_axis',(0.,0.,1.));
#30836=DIRECTION('ref_axis',(-0.344245360035407,0.93887972184625,0.));
#30837=DIRECTION('center_axis',(0.,0.,-1.));
#30838=DIRECTION('ref_axis',(-0.344245360035407,0.93887972184625,0.));
#30839=DIRECTION('',(0.,0.,1.));
#30840=DIRECTION('center_axis',(0.,0.,1.));
#30841=DIRECTION('ref_axis',(-0.344245360035407,0.93887972184625,0.));
#30842=DIRECTION('',(0.,0.,-1.));
#30843=DIRECTION('center_axis',(0.,0.,1.));
#30844=DIRECTION('ref_axis',(-0.430753803440728,-0.902469479163338,0.));
#30845=DIRECTION('center_axis',(0.,0.,1.));
#30846=DIRECTION('ref_axis',(-0.430753803440728,-0.902469479163338,0.));
#30847=DIRECTION('center_axis',(0.,0.,-1.));
#30848=DIRECTION('ref_axis',(-0.430753803440728,-0.902469479163338,0.));
#30849=DIRECTION('center_axis',(0.,0.,1.));
#30850=DIRECTION('ref_axis',(0.985216370234623,0.171314633997547,0.));
#30851=DIRECTION('center_axis',(0.,0.,-1.));
#30852=DIRECTION('ref_axis',(0.985216370234623,0.171314633997547,0.));
#30853=DIRECTION('',(0.,0.,1.));
#30854=DIRECTION('center_axis',(0.,0.,1.));
#30855=DIRECTION('ref_axis',(0.985216370234623,0.171314633997547,0.));
#30856=DIRECTION('',(0.,0.,-1.));
#30857=DIRECTION('center_axis',(0.824278476138107,-0.5661845933752,0.));
#30858=DIRECTION('ref_axis',(0.5661845933752,0.824278476138107,0.));
#30859=DIRECTION('',(0.5661845933752,0.824278476138107,0.));
#30860=DIRECTION('',(0.,0.,1.));
#30861=DIRECTION('',(-0.5661845933752,-0.824278476138107,0.));
#30862=DIRECTION('center_axis',(0.,0.,1.));
#30863=DIRECTION('ref_axis',(-0.0895155307640188,0.995985426475727,0.));
#30864=DIRECTION('center_axis',(0.,0.,-1.));
#30865=DIRECTION('ref_axis',(-0.0895155307640188,0.995985426475727,0.));
#30866=DIRECTION('',(0.,0.,1.));
#30867=DIRECTION('center_axis',(0.,0.,1.));
#30868=DIRECTION('ref_axis',(-0.0895155307640188,0.995985426475727,0.));
#30869=DIRECTION('',(0.,0.,-1.));
#30870=DIRECTION('center_axis',(0.,0.,1.));
#30871=DIRECTION('ref_axis',(-0.649652512346869,-0.760231289280704,0.));
#30872=DIRECTION('center_axis',(0.,0.,1.));
#30873=DIRECTION('ref_axis',(-0.649652512346869,-0.760231289280704,0.));
#30874=DIRECTION('center_axis',(0.,0.,-1.));
#30875=DIRECTION('ref_axis',(-0.649652512346869,-0.760231289280704,0.));
#30876=DIRECTION('center_axis',(0.,0.,1.));
#30877=DIRECTION('ref_axis',(0.995985426475728,-0.0895155307640127,0.));
#30878=DIRECTION('center_axis',(0.,0.,-1.));
#30879=DIRECTION('ref_axis',(0.995985426475728,-0.0895155307640127,0.));
#30880=DIRECTION('',(0.,0.,1.));
#30881=DIRECTION('center_axis',(0.,0.,1.));
#30882=DIRECTION('ref_axis',(0.995985426475728,-0.0895155307640127,0.));
#30883=DIRECTION('',(0.,0.,-1.));
#30884=DIRECTION('center_axis',(0.649652512346867,-0.760231289280706,0.));
#30885=DIRECTION('ref_axis',(0.760231289280706,0.649652512346867,0.));
#30886=DIRECTION('',(0.760231289280706,0.649652512346867,0.));
#30887=DIRECTION('',(0.,0.,1.));
#30888=DIRECTION('',(-0.760231289280706,-0.649652512346867,0.));
#30889=DIRECTION('center_axis',(0.,0.,1.));
#30890=DIRECTION('ref_axis',(0.17131463399754,0.985216370234625,0.));
#30891=DIRECTION('center_axis',(0.,0.,-1.));
#30892=DIRECTION('ref_axis',(0.17131463399754,0.985216370234625,0.));
#30893=DIRECTION('',(0.,0.,1.));
#30894=DIRECTION('center_axis',(0.,0.,1.));
#30895=DIRECTION('ref_axis',(0.17131463399754,0.985216370234625,0.));
#30896=DIRECTION('',(0.,0.,-1.));
#30897=DIRECTION('center_axis',(0.,0.,1.));
#30898=DIRECTION('ref_axis',(-0.824278476138108,-0.566184593375198,0.));
#30899=DIRECTION('center_axis',(0.,0.,1.));
#30900=DIRECTION('ref_axis',(-0.824278476138108,-0.566184593375198,0.));
#30901=DIRECTION('center_axis',(0.,0.,-1.));
#30902=DIRECTION('ref_axis',(-0.824278476138108,-0.566184593375198,0.));
#30903=DIRECTION('center_axis',(0.,0.,1.));
#30904=DIRECTION('ref_axis',(0.93887972184625,-0.344245360035407,0.));
#30905=DIRECTION('center_axis',(0.,0.,-1.));
#30906=DIRECTION('ref_axis',(0.93887972184625,-0.344245360035407,0.));
#30907=DIRECTION('',(0.,0.,1.));
#30908=DIRECTION('center_axis',(0.,0.,1.));
#30909=DIRECTION('ref_axis',(0.93887972184625,-0.344245360035407,0.));
#30910=DIRECTION('',(0.,0.,-1.));
#30911=DIRECTION('center_axis',(0.430753803440726,-0.902469479163339,0.));
#30912=DIRECTION('ref_axis',(0.902469479163339,0.430753803440726,0.));
#30913=DIRECTION('',(0.902469479163339,0.430753803440726,0.));
#30914=DIRECTION('',(0.,0.,1.));
#30915=DIRECTION('',(-0.902469479163339,-0.430753803440726,0.));
#30916=DIRECTION('center_axis',(0.,0.,1.));
#30917=DIRECTION('ref_axis',(0.420469989562982,0.907306446509065,0.));
#30918=DIRECTION('center_axis',(0.,0.,-1.));
#30919=DIRECTION('ref_axis',(0.420469989562982,0.907306446509065,0.));
#30920=DIRECTION('',(0.,0.,1.));
#30921=DIRECTION('center_axis',(0.,0.,1.));
#30922=DIRECTION('ref_axis',(0.420469989562982,0.907306446509065,0.));
#30923=DIRECTION('',(0.,0.,-1.));
#30924=DIRECTION('center_axis',(0.,0.,1.));
#30925=DIRECTION('ref_axis',(-0.942731223965124,-0.333553353095452,0.));
#30926=DIRECTION('center_axis',(0.,0.,1.));
#30927=DIRECTION('ref_axis',(-0.942731223965124,-0.333553353095452,0.));
#30928=DIRECTION('center_axis',(0.,0.,-1.));
#30929=DIRECTION('ref_axis',(-0.942731223965124,-0.333553353095452,0.));
#30930=DIRECTION('center_axis',(0.,0.,1.));
#30931=DIRECTION('ref_axis',(0.817790915745051,-0.575515436912747,0.));
#30932=DIRECTION('center_axis',(0.,0.,-1.));
#30933=DIRECTION('ref_axis',(0.817790915745051,-0.575515436912747,0.));
#30934=DIRECTION('',(0.,0.,1.));
#30935=DIRECTION('center_axis',(0.,0.,1.));
#30936=DIRECTION('ref_axis',(0.817790915745051,-0.575515436912747,0.));
#30937=DIRECTION('',(0.,0.,-1.));
#30938=DIRECTION('center_axis',(0.182499934684417,-0.983205865442321,0.));
#30939=DIRECTION('ref_axis',(0.983205865442321,0.182499934684417,0.));
#30940=DIRECTION('',(0.983205865442321,0.182499934684417,0.));
#30941=DIRECTION('',(0.,0.,1.));
#30942=DIRECTION('',(-0.983205865442321,-0.182499934684417,0.));
#30943=DIRECTION('center_axis',(0.,0.,1.));
#30944=DIRECTION('ref_axis',(0.64097101019921,0.767565087848714,0.));
#30945=DIRECTION('center_axis',(0.,0.,-1.));
#30946=DIRECTION('ref_axis',(0.64097101019921,0.767565087848714,0.));
#30947=DIRECTION('',(0.,0.,1.));
#30948=DIRECTION('center_axis',(0.,0.,1.));
#30949=DIRECTION('ref_axis',(0.64097101019921,0.767565087848714,0.));
#30950=DIRECTION('',(0.,0.,-1.));
#30951=DIRECTION('center_axis',(0.,0.,1.));
#30952=DIRECTION('ref_axis',(-0.996938396815926,-0.07819100302523,0.));
#30953=DIRECTION('center_axis',(0.,0.,1.));
#30954=DIRECTION('ref_axis',(-0.996938396815926,-0.07819100302523,0.));
#30955=DIRECTION('center_axis',(0.,0.,-1.));
#30956=DIRECTION('ref_axis',(-0.996938396815926,-0.07819100302523,0.));
#30957=DIRECTION('center_axis',(0.,0.,1.));
#30958=DIRECTION('ref_axis',(0.640971010199219,-0.767565087848706,0.));
#30959=DIRECTION('center_axis',(0.,0.,-1.));
#30960=DIRECTION('ref_axis',(0.640971010199219,-0.767565087848706,0.));
#30961=DIRECTION('',(0.,0.,1.));
#30962=DIRECTION('center_axis',(0.,0.,1.));
#30963=DIRECTION('ref_axis',(0.640971010199219,-0.767565087848706,0.));
#30964=DIRECTION('',(0.,0.,-1.));
#30965=DIRECTION('center_axis',(-0.0781910030252323,-0.996938396815926,
0.));
#30966=DIRECTION('ref_axis',(0.996938396815926,-0.0781910030252323,0.));
#30967=DIRECTION('',(0.996938396815926,-0.0781910030252323,0.));
#30968=DIRECTION('',(0.,0.,1.));
#30969=DIRECTION('',(-0.996938396815926,0.0781910030252323,0.));
#30970=DIRECTION('center_axis',(0.,0.,1.));
#30971=DIRECTION('ref_axis',(0.817790915745049,0.57551543691275,0.));
#30972=DIRECTION('center_axis',(0.,0.,-1.));
#30973=DIRECTION('ref_axis',(0.817790915745049,0.57551543691275,0.));
#30974=DIRECTION('',(0.,0.,1.));
#30975=DIRECTION('center_axis',(0.,0.,1.));
#30976=DIRECTION('ref_axis',(0.817790915745049,0.57551543691275,0.));
#30977=DIRECTION('',(0.,0.,-1.));
#30978=DIRECTION('center_axis',(0.,0.,1.));
#30979=DIRECTION('ref_axis',(-0.983205865442321,0.18249993468442,0.));
#30980=DIRECTION('center_axis',(0.,0.,1.));
#30981=DIRECTION('ref_axis',(-0.983205865442321,0.18249993468442,0.));
#30982=DIRECTION('center_axis',(0.,0.,-1.));
#30983=DIRECTION('ref_axis',(-0.983205865442321,0.18249993468442,0.));
#30984=DIRECTION('center_axis',(0.,0.,1.));
#30985=DIRECTION('ref_axis',(0.420469989562984,-0.907306446509064,0.));
#30986=DIRECTION('center_axis',(0.,0.,-1.));
#30987=DIRECTION('ref_axis',(0.420469989562984,-0.907306446509064,0.));
#30988=DIRECTION('',(0.,0.,1.));
#30989=DIRECTION('center_axis',(0.,0.,1.));
#30990=DIRECTION('ref_axis',(0.420469989562984,-0.907306446509064,0.));
#30991=DIRECTION('',(0.,0.,-1.));
#30992=DIRECTION('center_axis',(-0.333553353095454,-0.942731223965123,0.));
#30993=DIRECTION('ref_axis',(0.942731223965123,-0.333553353095454,0.));
#30994=DIRECTION('',(0.942731223965123,-0.333553353095454,0.));
#30995=DIRECTION('',(0.,0.,1.));
#30996=DIRECTION('',(-0.942731223965123,0.333553353095454,0.));
#30997=DIRECTION('center_axis',(0.,0.,1.));
#30998=DIRECTION('ref_axis',(0.93887972184625,0.344245360035408,0.));
#30999=DIRECTION('center_axis',(0.,0.,-1.));
#31000=DIRECTION('ref_axis',(0.93887972184625,0.344245360035408,0.));
#31001=DIRECTION('',(0.,0.,1.));
#31002=DIRECTION('center_axis',(0.,0.,1.));
#31003=DIRECTION('ref_axis',(0.93887972184625,0.344245360035408,0.));
#31004=DIRECTION('',(0.,0.,-1.));
#31005=DIRECTION('center_axis',(0.,0.,1.));
#31006=DIRECTION('ref_axis',(-0.902469479163338,0.430753803440728,0.));
#31007=DIRECTION('center_axis',(0.,0.,1.));
#31008=DIRECTION('ref_axis',(-0.902469479163338,0.430753803440728,0.));
#31009=DIRECTION('center_axis',(0.,0.,-1.));
#31010=DIRECTION('ref_axis',(-0.902469479163338,0.430753803440728,0.));
#31011=DIRECTION('center_axis',(0.,0.,1.));
#31012=DIRECTION('ref_axis',(0.171314633997546,-0.985216370234624,0.));
#31013=DIRECTION('center_axis',(0.,0.,-1.));
#31014=DIRECTION('ref_axis',(0.171314633997546,-0.985216370234624,0.));
#31015=DIRECTION('',(0.,0.,1.));
#31016=DIRECTION('center_axis',(0.,0.,1.));
#31017=DIRECTION('ref_axis',(0.171314633997546,-0.985216370234624,0.));
#31018=DIRECTION('',(0.,0.,-1.));
#31019=DIRECTION('center_axis',(-0.5661845933752,-0.824278476138107,0.));
#31020=DIRECTION('ref_axis',(0.824278476138107,-0.5661845933752,0.));
#31021=DIRECTION('',(0.824278476138107,-0.5661845933752,0.));
#31022=DIRECTION('',(0.,0.,1.));
#31023=DIRECTION('',(-0.824278476138107,0.5661845933752,0.));
#31024=DIRECTION('center_axis',(0.,0.,1.));
#31025=DIRECTION('ref_axis',(0.995985426475728,0.0895155307640127,0.));
#31026=DIRECTION('center_axis',(0.,0.,-1.));
#31027=DIRECTION('ref_axis',(0.995985426475728,0.0895155307640127,0.));
#31028=DIRECTION('',(0.,0.,1.));
#31029=DIRECTION('center_axis',(0.,0.,1.));
#31030=DIRECTION('ref_axis',(0.995985426475728,0.0895155307640127,0.));
#31031=DIRECTION('',(0.,0.,-1.));
#31032=DIRECTION('center_axis',(0.,0.,1.));
#31033=DIRECTION('ref_axis',(-0.760231289280704,0.649652512346868,0.));
#31034=DIRECTION('center_axis',(0.,0.,1.));
#31035=DIRECTION('ref_axis',(-0.760231289280704,0.649652512346868,0.));
#31036=DIRECTION('center_axis',(0.,0.,-1.));
#31037=DIRECTION('ref_axis',(-0.760231289280704,0.649652512346868,0.));
#31038=DIRECTION('center_axis',(0.,0.,1.));
#31039=DIRECTION('ref_axis',(-0.0895155307640188,-0.995985426475727,0.));
#31040=DIRECTION('center_axis',(0.,0.,-1.));
#31041=DIRECTION('ref_axis',(-0.0895155307640188,-0.995985426475727,0.));
#31042=DIRECTION('',(0.,0.,1.));
#31043=DIRECTION('center_axis',(0.,0.,1.));
#31044=DIRECTION('ref_axis',(-0.0895155307640188,-0.995985426475727,0.));
#31045=DIRECTION('',(0.,0.,-1.));
#31046=DIRECTION('center_axis',(-0.760231289280706,-0.649652512346867,0.));
#31047=DIRECTION('ref_axis',(0.649652512346867,-0.760231289280706,0.));
#31048=DIRECTION('',(0.649652512346867,-0.760231289280706,0.));
#31049=DIRECTION('',(0.,0.,1.));
#31050=DIRECTION('',(-0.649652512346867,0.760231289280706,0.));
#31051=DIRECTION('center_axis',(0.,0.,1.));
#31052=DIRECTION('ref_axis',(0.985216370234623,-0.171314633997547,0.));
#31053=DIRECTION('center_axis',(0.,0.,-1.));
#31054=DIRECTION('ref_axis',(0.985216370234623,-0.171314633997547,0.));
#31055=DIRECTION('',(0.,0.,1.));
#31056=DIRECTION('center_axis',(0.,0.,1.));
#31057=DIRECTION('ref_axis',(0.985216370234623,-0.171314633997547,0.));
#31058=DIRECTION('',(0.,0.,-1.));
#31059=DIRECTION('center_axis',(0.,0.,1.));
#31060=DIRECTION('ref_axis',(-0.566184593375198,0.824278476138108,0.));
#31061=DIRECTION('center_axis',(0.,0.,1.));
#31062=DIRECTION('ref_axis',(-0.566184593375198,0.824278476138108,0.));
#31063=DIRECTION('center_axis',(0.,0.,-1.));
#31064=DIRECTION('ref_axis',(-0.566184593375198,0.824278476138108,0.));
#31065=DIRECTION('center_axis',(0.,0.,1.));
#31066=DIRECTION('ref_axis',(-0.34424536003541,-0.93887972184625,0.));
#31067=DIRECTION('center_axis',(0.,0.,-1.));
#31068=DIRECTION('ref_axis',(-0.34424536003541,-0.93887972184625,0.));
#31069=DIRECTION('',(0.,0.,1.));
#31070=DIRECTION('center_axis',(0.,0.,1.));
#31071=DIRECTION('ref_axis',(-0.34424536003541,-0.93887972184625,0.));
#31072=DIRECTION('',(0.,0.,-1.));
#31073=DIRECTION('center_axis',(-0.902469479163339,-0.430753803440726,0.));
#31074=DIRECTION('ref_axis',(0.430753803440726,-0.902469479163339,0.));
#31075=DIRECTION('',(0.430753803440726,-0.902469479163339,0.));
#31076=DIRECTION('',(0.,0.,1.));
#31077=DIRECTION('',(-0.430753803440726,0.902469479163339,0.));
#31078=DIRECTION('center_axis',(0.,0.,1.));
#31079=DIRECTION('ref_axis',(0.907306446509069,-0.420469989562973,0.));
#31080=DIRECTION('center_axis',(0.,0.,-1.));
#31081=DIRECTION('ref_axis',(0.907306446509069,-0.420469989562973,0.));
#31082=DIRECTION('',(0.,0.,1.));
#31083=DIRECTION('center_axis',(0.,0.,1.));
#31084=DIRECTION('ref_axis',(0.907306446509069,-0.420469989562973,0.));
#31085=DIRECTION('',(0.,0.,-1.));
#31086=DIRECTION('center_axis',(0.,0.,1.));
#31087=DIRECTION('ref_axis',(-0.333553353095452,0.942731223965124,0.));
#31088=DIRECTION('center_axis',(0.,0.,1.));
#31089=DIRECTION('ref_axis',(-0.333553353095452,0.942731223965124,0.));
#31090=DIRECTION('center_axis',(0.,0.,-1.));
#31091=DIRECTION('ref_axis',(-0.333553353095452,0.942731223965124,0.));
#31092=DIRECTION('center_axis',(0.,0.,1.));
#31093=DIRECTION('ref_axis',(-0.575515436912748,-0.817790915745051,0.));
#31094=DIRECTION('center_axis',(0.,0.,-1.));
#31095=DIRECTION('ref_axis',(-0.575515436912748,-0.817790915745051,0.));
#31096=DIRECTION('',(0.,0.,1.));
#31097=DIRECTION('center_axis',(0.,0.,1.));
#31098=DIRECTION('ref_axis',(-0.575515436912748,-0.817790915745051,0.));
#31099=DIRECTION('',(0.,0.,-1.));
#31100=DIRECTION('center_axis',(-0.983205865442321,-0.182499934684418,0.));
#31101=DIRECTION('ref_axis',(0.182499934684418,-0.983205865442321,0.));
#31102=DIRECTION('',(0.182499934684418,-0.983205865442321,0.));
#31103=DIRECTION('',(0.,0.,1.));
#31104=DIRECTION('',(-0.182499934684418,0.983205865442321,0.));
#31105=DIRECTION('center_axis',(0.,0.,1.));
#31106=DIRECTION('ref_axis',(0.767565087848708,-0.640971010199218,0.));
#31107=DIRECTION('center_axis',(0.,0.,-1.));
#31108=DIRECTION('ref_axis',(0.767565087848708,-0.640971010199218,0.));
#31109=DIRECTION('',(0.,0.,1.));
#31110=DIRECTION('center_axis',(0.,0.,1.));
#31111=DIRECTION('ref_axis',(0.767565087848708,-0.640971010199218,0.));
#31112=DIRECTION('',(0.,0.,-1.));
#31113=DIRECTION('center_axis',(0.,0.,1.));
#31114=DIRECTION('ref_axis',(-0.0781910030252301,0.996938396815926,0.));
#31115=DIRECTION('center_axis',(0.,0.,1.));
#31116=DIRECTION('ref_axis',(-0.0781910030252301,0.996938396815926,0.));
#31117=DIRECTION('center_axis',(0.,0.,-1.));
#31118=DIRECTION('ref_axis',(-0.0781910030252301,0.996938396815926,0.));
#31119=DIRECTION('center_axis',(0.,0.,1.));
#31120=DIRECTION('ref_axis',(-0.767565087848706,-0.640971010199219,0.));
#31121=DIRECTION('center_axis',(0.,0.,-1.));
#31122=DIRECTION('ref_axis',(-0.767565087848706,-0.640971010199219,0.));
#31123=DIRECTION('',(0.,0.,1.));
#31124=DIRECTION('center_axis',(0.,0.,1.));
#31125=DIRECTION('ref_axis',(-0.767565087848706,-0.640971010199219,0.));
#31126=DIRECTION('',(0.,0.,-1.));
#31127=DIRECTION('center_axis',(-0.996938396815926,0.0781910030252323,0.));
#31128=DIRECTION('ref_axis',(-0.0781910030252323,-0.996938396815926,0.));
#31129=DIRECTION('',(-0.0781910030252323,-0.996938396815926,0.));
#31130=DIRECTION('',(0.,0.,1.));
#31131=DIRECTION('',(0.0781910030252323,0.996938396815926,0.));
#31132=DIRECTION('center_axis',(0.,0.,1.));
#31133=DIRECTION('ref_axis',(0.57551543691275,-0.817790915745049,0.));
#31134=DIRECTION('center_axis',(0.,0.,-1.));
#31135=DIRECTION('ref_axis',(0.57551543691275,-0.817790915745049,0.));
#31136=DIRECTION('',(0.,0.,1.));
#31137=DIRECTION('center_axis',(0.,0.,1.));
#31138=DIRECTION('ref_axis',(0.57551543691275,-0.817790915745049,0.));
#31139=DIRECTION('',(0.,0.,-1.));
#31140=DIRECTION('center_axis',(0.,0.,1.));
#31141=DIRECTION('ref_axis',(0.18249993468442,0.983205865442321,0.));
#31142=DIRECTION('center_axis',(0.,0.,1.));
#31143=DIRECTION('ref_axis',(0.18249993468442,0.983205865442321,0.));
#31144=DIRECTION('center_axis',(0.,0.,-1.));
#31145=DIRECTION('ref_axis',(0.18249993468442,0.983205865442321,0.));
#31146=DIRECTION('center_axis',(0.,0.,1.));
#31147=DIRECTION('ref_axis',(-0.907306446509064,-0.420469989562983,0.));
#31148=DIRECTION('center_axis',(0.,0.,-1.));
#31149=DIRECTION('ref_axis',(-0.907306446509064,-0.420469989562983,0.));
#31150=DIRECTION('',(0.,0.,1.));
#31151=DIRECTION('center_axis',(0.,0.,1.));
#31152=DIRECTION('ref_axis',(-0.907306446509064,-0.420469989562983,0.));
#31153=DIRECTION('',(0.,0.,-1.));
#31154=DIRECTION('center_axis',(-0.942731223965123,0.333553353095454,0.));
#31155=DIRECTION('ref_axis',(-0.333553353095454,-0.942731223965123,0.));
#31156=DIRECTION('',(-0.333553353095454,-0.942731223965123,0.));
#31157=DIRECTION('',(0.,0.,1.));
#31158=DIRECTION('',(0.333553353095454,0.942731223965123,0.));
#31159=DIRECTION('center_axis',(0.,0.,1.));
#31160=DIRECTION('ref_axis',(0.344245360035413,-0.938879721846248,0.));
#31161=DIRECTION('center_axis',(0.,0.,-1.));
#31162=DIRECTION('ref_axis',(0.344245360035413,-0.938879721846248,0.));
#31163=DIRECTION('',(0.,0.,1.));
#31164=DIRECTION('center_axis',(0.,0.,1.));
#31165=DIRECTION('ref_axis',(0.344245360035413,-0.938879721846248,0.));
#31166=DIRECTION('',(0.,0.,-1.));
#31167=DIRECTION('center_axis',(0.,0.,1.));
#31168=DIRECTION('ref_axis',(0.430753803440728,0.902469479163338,0.));
#31169=DIRECTION('center_axis',(0.,0.,1.));
#31170=DIRECTION('ref_axis',(0.430753803440728,0.902469479163338,0.));
#31171=DIRECTION('center_axis',(0.,0.,-1.));
#31172=DIRECTION('ref_axis',(0.430753803440728,0.902469479163338,0.));
#31173=DIRECTION('center_axis',(0.,0.,1.));
#31174=DIRECTION('ref_axis',(-0.985216370234624,-0.171314633997546,0.));
#31175=DIRECTION('center_axis',(0.,0.,-1.));
#31176=DIRECTION('ref_axis',(-0.985216370234624,-0.171314633997546,0.));
#31177=DIRECTION('',(0.,0.,1.));
#31178=DIRECTION('center_axis',(0.,0.,1.));
#31179=DIRECTION('ref_axis',(-0.985216370234624,-0.171314633997546,0.));
#31180=DIRECTION('',(0.,0.,-1.));
#31181=DIRECTION('center_axis',(-0.824278476138107,0.5661845933752,0.));
#31182=DIRECTION('ref_axis',(-0.5661845933752,-0.824278476138107,0.));
#31183=DIRECTION('',(-0.5661845933752,-0.824278476138107,0.));
#31184=DIRECTION('',(0.,0.,1.));
#31185=DIRECTION('',(0.5661845933752,0.824278476138107,0.));
#31186=DIRECTION('center_axis',(0.,0.,1.));
#31187=DIRECTION('ref_axis',(0.0895155307640121,-0.995985426475728,0.));
#31188=DIRECTION('center_axis',(0.,0.,-1.));
#31189=DIRECTION('ref_axis',(0.0895155307640121,-0.995985426475728,0.));
#31190=DIRECTION('',(0.,0.,1.));
#31191=DIRECTION('center_axis',(0.,0.,1.));
#31192=DIRECTION('ref_axis',(0.0895155307640121,-0.995985426475728,0.));
#31193=DIRECTION('',(0.,0.,-1.));
#31194=DIRECTION('center_axis',(0.,0.,1.));
#31195=DIRECTION('ref_axis',(0.649652512346868,0.760231289280704,0.));
#31196=DIRECTION('center_axis',(0.,0.,1.));
#31197=DIRECTION('ref_axis',(0.649652512346868,0.760231289280704,0.));
#31198=DIRECTION('center_axis',(0.,0.,-1.));
#31199=DIRECTION('ref_axis',(0.649652512346868,0.760231289280704,0.));
#31200=DIRECTION('center_axis',(0.,0.,1.));
#31201=DIRECTION('ref_axis',(-0.995985426475728,0.0895155307640127,0.));
#31202=DIRECTION('center_axis',(0.,0.,-1.));
#31203=DIRECTION('ref_axis',(-0.995985426475728,0.0895155307640127,0.));
#31204=DIRECTION('',(0.,0.,1.));
#31205=DIRECTION('center_axis',(0.,0.,1.));
#31206=DIRECTION('ref_axis',(-0.995985426475728,0.0895155307640127,0.));
#31207=DIRECTION('',(0.,0.,-1.));
#31208=DIRECTION('center_axis',(-0.649652512346867,0.760231289280706,0.));
#31209=DIRECTION('ref_axis',(-0.760231289280706,-0.649652512346867,0.));
#31210=DIRECTION('',(-0.760231289280706,-0.649652512346867,0.));
#31211=DIRECTION('',(0.,0.,1.));
#31212=DIRECTION('',(0.760231289280706,0.649652512346867,0.));
#31213=DIRECTION('center_axis',(0.,0.,1.));
#31214=DIRECTION('ref_axis',(-0.171314633997547,-0.985216370234623,0.));
#31215=DIRECTION('center_axis',(0.,0.,-1.));
#31216=DIRECTION('ref_axis',(-0.171314633997547,-0.985216370234623,0.));
#31217=DIRECTION('',(0.,0.,1.));
#31218=DIRECTION('center_axis',(0.,0.,1.));
#31219=DIRECTION('ref_axis',(-0.171314633997547,-0.985216370234623,0.));
#31220=DIRECTION('',(0.,0.,-1.));
#31221=DIRECTION('center_axis',(0.,0.,1.));
#31222=DIRECTION('ref_axis',(0.824278476138108,0.566184593375198,0.));
#31223=DIRECTION('center_axis',(0.,0.,1.));
#31224=DIRECTION('ref_axis',(0.824278476138108,0.566184593375198,0.));
#31225=DIRECTION('center_axis',(0.,0.,-1.));
#31226=DIRECTION('ref_axis',(0.824278476138108,0.566184593375198,0.));
#31227=DIRECTION('center_axis',(0.,0.,1.));
#31228=DIRECTION('ref_axis',(-0.93887972184625,0.34424536003541,0.));
#31229=DIRECTION('center_axis',(0.,0.,-1.));
#31230=DIRECTION('ref_axis',(-0.93887972184625,0.34424536003541,0.));
#31231=DIRECTION('',(0.,0.,1.));
#31232=DIRECTION('center_axis',(0.,0.,1.));
#31233=DIRECTION('ref_axis',(-0.93887972184625,0.34424536003541,0.));
#31234=DIRECTION('',(0.,0.,-1.));
#31235=DIRECTION('center_axis',(-0.430753803440726,0.902469479163339,0.));
#31236=DIRECTION('ref_axis',(-0.902469479163339,-0.430753803440726,0.));
#31237=DIRECTION('',(-0.902469479163339,-0.430753803440726,0.));
#31238=DIRECTION('',(0.,0.,1.));
#31239=DIRECTION('',(0.902469479163339,0.430753803440726,0.));
#31240=DIRECTION('center_axis',(0.,0.,1.));
#31241=DIRECTION('ref_axis',(-0.420469989562974,-0.907306446509068,0.));
#31242=DIRECTION('center_axis',(0.,0.,-1.));
#31243=DIRECTION('ref_axis',(-0.420469989562974,-0.907306446509068,0.));
#31244=DIRECTION('',(0.,0.,1.));
#31245=DIRECTION('center_axis',(0.,0.,1.));
#31246=DIRECTION('ref_axis',(-0.420469989562974,-0.907306446509068,0.));
#31247=DIRECTION('',(0.,0.,-1.));
#31248=DIRECTION('center_axis',(0.,0.,1.));
#31249=DIRECTION('ref_axis',(0.942731223965124,0.333553353095452,0.));
#31250=DIRECTION('center_axis',(0.,0.,1.));
#31251=DIRECTION('ref_axis',(0.942731223965124,0.333553353095452,0.));
#31252=DIRECTION('center_axis',(0.,0.,-1.));
#31253=DIRECTION('ref_axis',(0.942731223965124,0.333553353095452,0.));
#31254=DIRECTION('center_axis',(-0.18249993468442,-0.983205865442321,0.));
#31255=DIRECTION('ref_axis',(0.983205865442321,-0.182499934684419,0.));
#31256=DIRECTION('',(-0.983205865442321,0.182499934684419,0.));
#31257=DIRECTION('',(0.,0.,1.));
#31258=DIRECTION('',(0.983205865442321,-0.182499934684419,0.));
#31259=DIRECTION('',(0.,0.,-1.));
#31260=DIRECTION('',(0.,0.,1.));
#31261=DIRECTION('center_axis',(-0.430753803440728,-0.902469479163338,0.));
#31262=DIRECTION('ref_axis',(0.902469479163338,-0.430753803440728,0.));
#31263=DIRECTION('',(-0.902469479163338,0.430753803440728,0.));
#31264=DIRECTION('',(0.,0.,1.));
#31265=DIRECTION('',(0.902469479163338,-0.430753803440728,0.));
#31266=DIRECTION('',(0.,0.,-1.));
#31267=DIRECTION('',(0.,0.,1.));
#31268=DIRECTION('center_axis',(-0.649652512346868,-0.760231289280705,0.));
#31269=DIRECTION('ref_axis',(0.760231289280705,-0.649652512346868,0.));
#31270=DIRECTION('',(-0.760231289280705,0.649652512346868,0.));
#31271=DIRECTION('',(0.,0.,1.));
#31272=DIRECTION('',(0.760231289280705,-0.649652512346868,0.));
#31273=DIRECTION('',(0.,0.,-1.));
#31274=DIRECTION('',(0.,0.,1.));
#31275=DIRECTION('center_axis',(-0.824278476138108,-0.566184593375198,0.));
#31276=DIRECTION('ref_axis',(0.566184593375198,-0.824278476138108,0.));
#31277=DIRECTION('',(-0.566184593375198,0.824278476138108,0.));
#31278=DIRECTION('',(0.,0.,1.));
#31279=DIRECTION('',(0.566184593375198,-0.824278476138108,0.));
#31280=DIRECTION('',(0.,0.,-1.));
#31281=DIRECTION('',(0.,0.,1.));
#31282=DIRECTION('center_axis',(-0.942731223965124,-0.333553353095453,0.));
#31283=DIRECTION('ref_axis',(0.333553353095453,-0.942731223965124,0.));
#31284=DIRECTION('',(-0.333553353095453,0.942731223965124,0.));
#31285=DIRECTION('',(0.,0.,1.));
#31286=DIRECTION('',(0.333553353095453,-0.942731223965124,0.));
#31287=DIRECTION('',(0.,0.,-1.));
#31288=DIRECTION('',(0.,0.,1.));
#31289=DIRECTION('center_axis',(-0.996938396815926,-0.0781910030252307,
0.));
#31290=DIRECTION('ref_axis',(0.0781910030252307,-0.996938396815926,0.));
#31291=DIRECTION('',(-0.0781910030252307,0.996938396815926,0.));
#31292=DIRECTION('',(0.,0.,1.));
#31293=DIRECTION('',(0.0781910030252307,-0.996938396815926,0.));
#31294=DIRECTION('',(0.,0.,-1.));
#31295=DIRECTION('',(0.,0.,1.));
#31296=DIRECTION('center_axis',(-0.983205865442321,0.182499934684419,0.));
#31297=DIRECTION('ref_axis',(-0.182499934684419,-0.983205865442321,0.));
#31298=DIRECTION('',(0.182499934684419,0.983205865442321,0.));
#31299=DIRECTION('',(0.,0.,1.));
#31300=DIRECTION('',(-0.182499934684419,-0.983205865442321,0.));
#31301=DIRECTION('',(0.,0.,-1.));
#31302=DIRECTION('',(0.,0.,1.));
#31303=DIRECTION('center_axis',(-0.902469479163338,0.430753803440728,0.));
#31304=DIRECTION('ref_axis',(-0.430753803440728,-0.902469479163338,0.));
#31305=DIRECTION('',(0.430753803440728,0.902469479163338,0.));
#31306=DIRECTION('',(0.,0.,1.));
#31307=DIRECTION('',(-0.430753803440728,-0.902469479163338,0.));
#31308=DIRECTION('',(0.,0.,-1.));
#31309=DIRECTION('',(0.,0.,1.));
#31310=DIRECTION('center_axis',(-0.760231289280705,0.649652512346868,0.));
#31311=DIRECTION('ref_axis',(-0.649652512346868,-0.760231289280705,0.));
#31312=DIRECTION('',(0.649652512346868,0.760231289280705,0.));
#31313=DIRECTION('',(0.,0.,1.));
#31314=DIRECTION('',(-0.649652512346868,-0.760231289280705,0.));
#31315=DIRECTION('',(0.,0.,-1.));
#31316=DIRECTION('',(0.,0.,1.));
#31317=DIRECTION('center_axis',(-0.566184593375199,0.824278476138108,0.));
#31318=DIRECTION('ref_axis',(-0.824278476138108,-0.566184593375198,0.));
#31319=DIRECTION('',(0.824278476138108,0.566184593375198,0.));
#31320=DIRECTION('',(0.,0.,1.));
#31321=DIRECTION('',(-0.824278476138108,-0.566184593375198,0.));
#31322=DIRECTION('',(0.,0.,-1.));
#31323=DIRECTION('',(0.,0.,1.));
#31324=DIRECTION('center_axis',(-0.333553353095453,0.942731223965124,0.));
#31325=DIRECTION('ref_axis',(-0.942731223965124,-0.333553353095453,0.));
#31326=DIRECTION('',(0.942731223965124,0.333553353095453,0.));
#31327=DIRECTION('',(0.,0.,1.));
#31328=DIRECTION('',(-0.942731223965124,-0.333553353095453,0.));
#31329=DIRECTION('',(0.,0.,-1.));
#31330=DIRECTION('',(0.,0.,1.));
#31331=DIRECTION('center_axis',(-0.0781910030252307,0.996938396815926,0.));
#31332=DIRECTION('ref_axis',(-0.996938396815926,-0.0781910030252307,0.));
#31333=DIRECTION('',(0.996938396815926,0.0781910030252307,0.));
#31334=DIRECTION('',(0.,0.,1.));
#31335=DIRECTION('',(-0.996938396815926,-0.0781910030252307,0.));
#31336=DIRECTION('',(0.,0.,-1.));
#31337=DIRECTION('',(0.,0.,1.));
#31338=DIRECTION('center_axis',(0.182499934684419,0.983205865442321,0.));
#31339=DIRECTION('ref_axis',(-0.983205865442321,0.182499934684419,0.));
#31340=DIRECTION('',(0.983205865442321,-0.182499934684419,0.));
#31341=DIRECTION('',(0.,0.,1.));
#31342=DIRECTION('',(-0.983205865442321,0.182499934684419,0.));
#31343=DIRECTION('',(0.,0.,-1.));
#31344=DIRECTION('',(0.,0.,1.));
#31345=DIRECTION('center_axis',(0.430753803440728,0.902469479163338,0.));
#31346=DIRECTION('ref_axis',(-0.902469479163338,0.430753803440727,0.));
#31347=DIRECTION('',(0.902469479163338,-0.430753803440727,0.));
#31348=DIRECTION('',(0.,0.,1.));
#31349=DIRECTION('',(-0.902469479163338,0.430753803440727,0.));
#31350=DIRECTION('',(0.,0.,-1.));
#31351=DIRECTION('',(0.,0.,1.));
#31352=DIRECTION('center_axis',(0.649652512346868,0.760231289280705,0.));
#31353=DIRECTION('ref_axis',(-0.760231289280705,0.649652512346868,0.));
#31354=DIRECTION('',(0.760231289280705,-0.649652512346868,0.));
#31355=DIRECTION('',(0.,0.,1.));
#31356=DIRECTION('',(-0.760231289280705,0.649652512346868,0.));
#31357=DIRECTION('',(0.,0.,-1.));
#31358=DIRECTION('',(0.,0.,1.));
#31359=DIRECTION('center_axis',(0.824278476138108,0.566184593375199,0.));
#31360=DIRECTION('ref_axis',(-0.566184593375199,0.824278476138108,0.));
#31361=DIRECTION('',(0.566184593375199,-0.824278476138108,0.));
#31362=DIRECTION('',(0.,0.,1.));
#31363=DIRECTION('',(-0.566184593375199,0.824278476138108,0.));
#31364=DIRECTION('',(0.,0.,-1.));
#31365=DIRECTION('',(0.,0.,1.));
#31366=DIRECTION('center_axis',(0.942731223965124,0.333553353095453,0.));
#31367=DIRECTION('ref_axis',(-0.333553353095453,0.942731223965124,0.));
#31368=DIRECTION('',(0.333553353095453,-0.942731223965124,0.));
#31369=DIRECTION('',(0.,0.,1.));
#31370=DIRECTION('',(-0.333553353095453,0.942731223965124,0.));
#31371=DIRECTION('',(0.,0.,-1.));
#31372=DIRECTION('',(0.,0.,1.));
#31373=DIRECTION('center_axis',(0.996938396815926,0.0781910030252308,0.));
#31374=DIRECTION('ref_axis',(-0.0781910030252308,0.996938396815926,0.));
#31375=DIRECTION('',(0.0781910030252308,-0.996938396815926,0.));
#31376=DIRECTION('',(0.,0.,1.));
#31377=DIRECTION('',(-0.0781910030252308,0.996938396815926,0.));
#31378=DIRECTION('',(0.,0.,-1.));
#31379=DIRECTION('',(0.,0.,1.));
#31380=DIRECTION('center_axis',(0.983205865442321,-0.182499934684419,0.));
#31381=DIRECTION('ref_axis',(0.182499934684419,0.983205865442321,0.));
#31382=DIRECTION('',(-0.182499934684419,-0.983205865442321,0.));
#31383=DIRECTION('',(0.,0.,1.));
#31384=DIRECTION('',(0.182499934684419,0.983205865442321,0.));
#31385=DIRECTION('',(0.,0.,-1.));
#31386=DIRECTION('',(0.,0.,1.));
#31387=DIRECTION('center_axis',(0.902469479163338,-0.430753803440727,0.));
#31388=DIRECTION('ref_axis',(0.430753803440727,0.902469479163338,0.));
#31389=DIRECTION('',(-0.430753803440727,-0.902469479163338,0.));
#31390=DIRECTION('',(0.,0.,1.));
#31391=DIRECTION('',(0.430753803440727,0.902469479163338,0.));
#31392=DIRECTION('',(0.,0.,-1.));
#31393=DIRECTION('',(0.,0.,1.));
#31394=DIRECTION('center_axis',(0.760231289280705,-0.649652512346868,0.));
#31395=DIRECTION('ref_axis',(0.649652512346868,0.760231289280705,0.));
#31396=DIRECTION('',(-0.649652512346868,-0.760231289280705,0.));
#31397=DIRECTION('',(0.,0.,1.));
#31398=DIRECTION('',(0.649652512346868,0.760231289280705,0.));
#31399=DIRECTION('',(0.,0.,-1.));
#31400=DIRECTION('',(0.,0.,1.));
#31401=DIRECTION('center_axis',(0.566184593375199,-0.824278476138108,0.));
#31402=DIRECTION('ref_axis',(0.824278476138108,0.566184593375199,0.));
#31403=DIRECTION('',(-0.824278476138108,-0.566184593375199,0.));
#31404=DIRECTION('',(0.,0.,1.));
#31405=DIRECTION('',(0.824278476138108,0.566184593375199,0.));
#31406=DIRECTION('',(0.,0.,-1.));
#31407=DIRECTION('',(0.,0.,1.));
#31408=DIRECTION('center_axis',(0.333553353095453,-0.942731223965124,0.));
#31409=DIRECTION('ref_axis',(0.942731223965124,0.333553353095453,0.));
#31410=DIRECTION('',(-0.942731223965124,-0.333553353095453,0.));
#31411=DIRECTION('',(0.,0.,1.));
#31412=DIRECTION('',(0.942731223965124,0.333553353095453,0.));
#31413=DIRECTION('',(0.,0.,-1.));
#31414=DIRECTION('',(0.,0.,1.));
#31415=DIRECTION('center_axis',(0.,0.,1.));
#31416=DIRECTION('ref_axis',(1.,0.,0.));
#31417=DIRECTION('center_axis',(0.,0.,1.));
#31418=DIRECTION('ref_axis',(1.,0.,0.));
#31419=DIRECTION('center_axis',(0.,0.,1.));
#31420=DIRECTION('ref_axis',(1.,0.,0.));
#31421=DIRECTION('center_axis',(0.,0.,1.));
#31422=DIRECTION('ref_axis',(1.,0.,0.));
#31423=DIRECTION('center_axis',(0.,0.,1.));
#31424=DIRECTION('ref_axis',(1.,0.,0.));
#31425=DIRECTION('center_axis',(0.,0.,1.));
#31426=DIRECTION('ref_axis',(1.,0.,0.));
#31427=DIRECTION('center_axis',(0.,0.,1.));
#31428=DIRECTION('ref_axis',(1.,0.,0.));
#31429=DIRECTION('center_axis',(0.,0.,1.));
#31430=DIRECTION('ref_axis',(1.,0.,0.));
#31431=DIRECTION('center_axis',(0.,0.,1.));
#31432=DIRECTION('ref_axis',(1.,0.,0.));
#31433=DIRECTION('center_axis',(0.,0.,1.));
#31434=DIRECTION('ref_axis',(1.,0.,0.));
#31435=DIRECTION('center_axis',(0.,0.,1.));
#31436=DIRECTION('ref_axis',(1.,0.,0.));
#31437=DIRECTION('center_axis',(0.,0.,1.));
#31438=DIRECTION('ref_axis',(1.,0.,0.));
#31439=DIRECTION('center_axis',(0.,0.,1.));
#31440=DIRECTION('ref_axis',(1.,0.,0.));
#31441=DIRECTION('center_axis',(0.,0.,1.));
#31442=DIRECTION('ref_axis',(1.,0.,0.));
#31443=DIRECTION('center_axis',(0.,0.,1.));
#31444=DIRECTION('ref_axis',(1.,0.,0.));
#31445=DIRECTION('center_axis',(0.,0.,1.));
#31446=DIRECTION('ref_axis',(1.,0.,0.));
#31447=DIRECTION('center_axis',(0.,0.,1.));
#31448=DIRECTION('ref_axis',(1.,0.,0.));
#31449=DIRECTION('center_axis',(0.,0.,1.));
#31450=DIRECTION('ref_axis',(1.,0.,0.));
#31451=DIRECTION('center_axis',(0.,0.,1.));
#31452=DIRECTION('ref_axis',(1.,0.,0.));
#31453=DIRECTION('center_axis',(0.,0.,1.));
#31454=DIRECTION('ref_axis',(1.,0.,0.));
#31455=DIRECTION('center_axis',(0.,0.,1.));
#31456=DIRECTION('ref_axis',(1.,0.,0.));
#31457=DIRECTION('center_axis',(0.,0.,1.));
#31458=DIRECTION('ref_axis',(1.,0.,0.));
#31459=DIRECTION('center_axis',(0.,0.,1.));
#31460=DIRECTION('ref_axis',(1.,0.,0.));
#31461=DIRECTION('center_axis',(0.,0.,1.));
#31462=DIRECTION('ref_axis',(1.,0.,0.));
#31463=DIRECTION('',(-0.983205865442321,-0.182499934684418,0.));
#31464=DIRECTION('center_axis',(0.,0.,-1.));
#31465=DIRECTION('ref_axis',(-0.817790915745051,0.575515436912748,0.));
#31466=DIRECTION('center_axis',(0.,0.,-1.));
#31467=DIRECTION('ref_axis',(0.996938396815926,0.0781910030252301,0.));
#31468=DIRECTION('center_axis',(0.,0.,-1.));
#31469=DIRECTION('ref_axis',(-0.640971010199219,-0.767565087848707,0.));
#31470=DIRECTION('',(0.996938396815926,0.0781910030252308,0.));
#31471=DIRECTION('center_axis',(0.,0.,1.));
#31472=DIRECTION('ref_axis',(1.,0.,0.));
#31473=DIRECTION('center_axis',(0.,0.,-1.));
#31474=DIRECTION('ref_axis',(1.,0.,0.));
#31475=DIRECTION('center_axis',(0.,0.,1.));
#31476=DIRECTION('ref_axis',(1.,0.,0.));
#31477=DIRECTION('center_axis',(0.,0.,1.));
#31478=DIRECTION('ref_axis',(1.,0.,0.));
#31479=DIRECTION('',(-0.996938396815926,-0.0781910030252308,0.));
#31480=DIRECTION('center_axis',(0.,0.,1.));
#31481=DIRECTION('ref_axis',(-0.640971010199219,-0.767565087848707,0.));
#31482=DIRECTION('center_axis',(0.,0.,1.));
#31483=DIRECTION('ref_axis',(0.996938396815926,0.0781910030252301,0.));
#31484=DIRECTION('center_axis',(0.,0.,1.));
#31485=DIRECTION('ref_axis',(-0.817790915745051,0.575515436912748,0.));
#31486=DIRECTION('',(0.983205865442321,0.182499934684418,0.));
#31487=DIRECTION('center_axis',(0.,0.,1.));
#31488=DIRECTION('ref_axis',(1.,0.,0.));
#31489=DIRECTION('center_axis',(0.,0.,1.));
#31490=DIRECTION('ref_axis',(1.,0.,0.));
#31491=DIRECTION('center_axis',(0.,0.,1.));
#31492=DIRECTION('ref_axis',(1.,0.,0.));
#31493=DIRECTION('center_axis',(0.,0.,1.));
#31494=DIRECTION('ref_axis',(1.,0.,0.));
#31495=DIRECTION('center_axis',(0.,0.,1.));
#31496=DIRECTION('ref_axis',(1.,0.,0.));
#31497=DIRECTION('center_axis',(0.,0.,1.));
#31498=DIRECTION('ref_axis',(1.,0.,0.));
#31499=DIRECTION('center_axis',(0.,0.,1.));
#31500=DIRECTION('ref_axis',(1.,0.,0.));
#31501=DIRECTION('center_axis',(0.,0.,1.));
#31502=DIRECTION('ref_axis',(1.,0.,0.));
#31503=DIRECTION('center_axis',(0.,0.,1.));
#31504=DIRECTION('ref_axis',(1.,0.,0.));
#31505=DIRECTION('center_axis',(0.,0.,1.));
#31506=DIRECTION('ref_axis',(1.,0.,0.));
#31507=DIRECTION('center_axis',(0.,0.,1.));
#31508=DIRECTION('ref_axis',(1.,0.,0.));
#31509=DIRECTION('center_axis',(0.,0.,1.));
#31510=DIRECTION('ref_axis',(1.,0.,0.));
#31511=DIRECTION('center_axis',(0.,0.,1.));
#31512=DIRECTION('ref_axis',(1.,0.,0.));
#31513=DIRECTION('center_axis',(0.,0.,1.));
#31514=DIRECTION('ref_axis',(1.,0.,0.));
#31515=DIRECTION('center_axis',(0.,0.,1.));
#31516=DIRECTION('ref_axis',(1.,0.,0.));
#31517=DIRECTION('center_axis',(0.,0.,1.));
#31518=DIRECTION('ref_axis',(1.,0.,0.));
#31519=DIRECTION('center_axis',(0.,0.,1.));
#31520=DIRECTION('ref_axis',(1.,0.,0.));
#31521=DIRECTION('center_axis',(0.,0.,1.));
#31522=DIRECTION('ref_axis',(1.,0.,0.));
#31523=DIRECTION('center_axis',(0.,0.,1.));
#31524=DIRECTION('ref_axis',(1.,0.,0.));
#31525=DIRECTION('center_axis',(0.,0.,1.));
#31526=DIRECTION('ref_axis',(1.,0.,0.));
#31527=DIRECTION('center_axis',(0.,0.,1.));
#31528=DIRECTION('ref_axis',(1.,0.,0.));
#31529=DIRECTION('center_axis',(0.,0.,1.));
#31530=DIRECTION('ref_axis',(1.,0.,0.));
#31531=DIRECTION('center_axis',(0.,0.,1.));
#31532=DIRECTION('ref_axis',(1.,0.,0.));
#31533=DIRECTION('center_axis',(0.,0.,-1.));
#31534=DIRECTION('ref_axis',(1.,0.,0.));
#31535=DIRECTION('center_axis',(0.,0.,1.));
#31536=DIRECTION('ref_axis',(1.,0.,0.));
#31537=DIRECTION('',(0.,0.,-1.));
#31538=DIRECTION('center_axis',(0.,0.,1.));
#31539=DIRECTION('ref_axis',(1.,0.,0.));
#31540=DIRECTION('center_axis',(0.,0.,1.));
#31541=DIRECTION('ref_axis',(1.,0.,0.));
#31542=DIRECTION('center_axis',(0.,0.,1.));
#31543=DIRECTION('ref_axis',(1.,0.,0.));
#31544=DIRECTION('center_axis',(0.,0.,1.));
#31545=DIRECTION('ref_axis',(1.,0.,0.));
#31546=DIRECTION('center_axis',(0.,0.,1.));
#31547=DIRECTION('ref_axis',(1.,0.,0.));
#31548=DIRECTION('center_axis',(0.,0.,1.));
#31549=DIRECTION('ref_axis',(1.,0.,0.));
#31550=DIRECTION('center_axis',(0.,0.,1.));
#31551=DIRECTION('ref_axis',(1.,0.,0.));
#31552=DIRECTION('center_axis',(0.,0.,1.));
#31553=DIRECTION('ref_axis',(1.,0.,0.));
#31554=DIRECTION('center_axis',(0.,0.,1.));
#31555=DIRECTION('ref_axis',(1.,0.,0.));
#31556=DIRECTION('center_axis',(0.,0.,1.));
#31557=DIRECTION('ref_axis',(1.,0.,0.));
#31558=DIRECTION('center_axis',(0.,0.,1.));
#31559=DIRECTION('ref_axis',(-1.,-1.22464679914735E-16,0.));
#31560=DIRECTION('center_axis',(0.,0.,1.));
#31561=DIRECTION('ref_axis',(1.,0.,0.));
#31562=DIRECTION('center_axis',(0.,0.,1.));
#31563=DIRECTION('ref_axis',(1.,0.,0.));
#31564=DIRECTION('center_axis',(0.,0.,1.));
#31565=DIRECTION('ref_axis',(1.,0.,0.));
#31566=DIRECTION('center_axis',(0.,0.,1.));
#31567=DIRECTION('ref_axis',(1.,0.,0.));
#31568=DIRECTION('center_axis',(0.,0.,1.));
#31569=DIRECTION('ref_axis',(1.,0.,0.));
#31570=DIRECTION('center_axis',(0.,0.,1.));
#31571=DIRECTION('ref_axis',(1.,0.,0.));
#31572=DIRECTION('center_axis',(0.,0.,1.));
#31573=DIRECTION('ref_axis',(1.,0.,0.));
#31574=DIRECTION('center_axis',(0.,0.,1.));
#31575=DIRECTION('ref_axis',(1.,0.,0.));
#31576=DIRECTION('center_axis',(0.,0.,1.));
#31577=DIRECTION('ref_axis',(1.,0.,0.));
#31578=DIRECTION('center_axis',(0.,0.,1.));
#31579=DIRECTION('ref_axis',(1.,0.,0.));
#31580=DIRECTION('center_axis',(0.,0.,1.));
#31581=DIRECTION('ref_axis',(1.,0.,0.));
#31582=DIRECTION('center_axis',(0.,0.,1.));
#31583=DIRECTION('ref_axis',(-0.817790915745051,0.575515436912748,0.));
#31584=DIRECTION('',(0.,0.,1.));
#31585=DIRECTION('',(0.,0.,-1.));
#31586=DIRECTION('center_axis',(-0.182499934684418,0.983205865442321,0.));
#31587=DIRECTION('ref_axis',(-0.983205865442321,-0.182499934684418,0.));
#31588=DIRECTION('',(0.,0.,1.));
#31589=DIRECTION('center_axis',(0.,0.,1.));
#31590=DIRECTION('ref_axis',(-0.640971010199219,-0.767565087848707,0.));
#31591=DIRECTION('',(0.,0.,1.));
#31592=DIRECTION('',(0.,0.,-1.));
#31593=DIRECTION('center_axis',(0.,0.,1.));
#31594=DIRECTION('ref_axis',(0.996938396815926,0.0781910030252301,0.));
#31595=DIRECTION('center_axis',(0.0781910030252308,-0.996938396815926,0.));
#31596=DIRECTION('ref_axis',(0.996938396815926,0.0781910030252308,0.));
#31597=DIRECTION('',(0.,0.,1.));
#31598=DIRECTION('',(0.,0.,1.));
#31599=DIRECTION('center_axis',(0.,0.,1.));
#31600=DIRECTION('ref_axis',(1.,0.,0.));
#31601=DIRECTION('',(0.,0.,-1.));
#31602=DIRECTION('center_axis',(0.,0.,1.));
#31603=DIRECTION('ref_axis',(1.,0.,0.));
#215380=CARTESIAN_POINT('',(0.,0.,0.));
#215381=CARTESIAN_POINT('Origin',(21.88788407408,-2.2182269405164,0.));
#215382=CARTESIAN_POINT('',(21.3904321633055,-2.1678126918683,0.));
#215383=CARTESIAN_POINT('',(21.9269795755927,-1.71975774210843,0.));
#215384=CARTESIAN_POINT('Origin',(21.88788407408,-2.2182269405164,0.));
#215385=CARTESIAN_POINT('',(21.9269795755927,-1.71975774210843,12.));
#215386=CARTESIAN_POINT('',(21.9269795755927,-1.71975774210843,0.));
#215387=CARTESIAN_POINT('',(21.3904321633055,-2.1678126918683,12.));
#215388=CARTESIAN_POINT('Origin',(21.88788407408,-2.2182269405164,12.));
#215389=CARTESIAN_POINT('',(21.3904321633055,-2.1678126918683,0.));
#215390=CARTESIAN_POINT('Origin',(22.4835757167854,-1.76341220531181,0.));
#215391=CARTESIAN_POINT('',(22.4835757167854,-1.76341220531181,0.));
#215392=CARTESIAN_POINT('',(11.2417878583927,-0.881706102655892,0.));
#215393=CARTESIAN_POINT('',(22.4835757167854,-1.76341220531181,12.));
#215394=CARTESIAN_POINT('',(22.4835757167854,-1.76341220531181,0.));
#215395=CARTESIAN_POINT('',(11.2417878583927,-0.881706102655892,12.));
#215396=CARTESIAN_POINT('Origin',(21.7161918885402,-3.52235856495314,0.));
#215397=CARTESIAN_POINT('',(21.624941921198,-4.0139614976743,0.));
#215398=CARTESIAN_POINT('',(21.2226420728916,-3.4423049612042,0.));
#215399=CARTESIAN_POINT('Origin',(21.7161918885402,-3.52235856495314,0.));
#215400=CARTESIAN_POINT('',(21.2226420728916,-3.4423049612042,12.));
#215401=CARTESIAN_POINT('',(21.2226420728916,-3.4423049612042,0.));
#215402=CARTESIAN_POINT('',(21.624941921198,-4.0139614976743,12.));
#215403=CARTESIAN_POINT('Origin',(21.7161918885402,-3.52235856495314,12.));
#215404=CARTESIAN_POINT('',(21.624941921198,-4.0139614976743,0.));
#215405=CARTESIAN_POINT('Origin',(7.6920903736728E-13,-1.31973449697531E-13,
0.));
#215406=CARTESIAN_POINT('Origin',(7.6920903736728E-13,-1.31973449697531E-13,
12.));
#215407=CARTESIAN_POINT('Origin',(7.6920903736728E-13,-1.31973449697531E-13,
0.));
#215408=CARTESIAN_POINT('Origin',(20.56795313141,-7.80764394578304,0.));
#215409=CARTESIAN_POINT('',(20.1004996511507,-7.63019749246979,0.));
#215410=CARTESIAN_POINT('',(20.7347298079577,-7.33627833380047,0.));
#215411=CARTESIAN_POINT('Origin',(20.56795313141,-7.80764394578304,0.));
#215412=CARTESIAN_POINT('',(20.7347298079577,-7.33627833380047,12.));
#215413=CARTESIAN_POINT('',(20.7347298079577,-7.33627833380047,0.));
#215414=CARTESIAN_POINT('',(20.1004996511507,-7.63019749246979,12.));
#215415=CARTESIAN_POINT('Origin',(20.56795313141,-7.80764394578304,12.));
#215416=CARTESIAN_POINT('',(20.1004996511507,-7.63019749246979,0.));
#215417=CARTESIAN_POINT('Origin',(21.2610617890679,-7.52250298901266,0.));
#215418=CARTESIAN_POINT('',(21.2610617890679,-7.52250298901266,0.));
#215419=CARTESIAN_POINT('',(10.6305308945339,-3.76125149450632,0.));
#215420=CARTESIAN_POINT('',(21.2610617890679,-7.52250298901266,12.));
#215421=CARTESIAN_POINT('',(21.2610617890679,-7.52250298901266,0.));
#215422=CARTESIAN_POINT('',(10.6305308945339,-3.76125149450632,12.));
#215423=CARTESIAN_POINT('Origin',(20.0645771135003,-9.02290115519382,0.));
#215424=CARTESIAN_POINT('',(19.84920021178,-9.47413589477549,0.));
#215425=CARTESIAN_POINT('',(19.6085639972844,-8.81783521984851,0.));
#215426=CARTESIAN_POINT('Origin',(20.0645771135003,-9.02290115519382,0.));
#215427=CARTESIAN_POINT('',(19.6085639972844,-8.81783521984851,12.));
#215428=CARTESIAN_POINT('',(19.6085639972844,-8.81783521984851,0.));
#215429=CARTESIAN_POINT('',(19.84920021178,-9.47413589477549,12.));
#215430=CARTESIAN_POINT('Origin',(20.0645771135003,-9.02290115519382,12.));
#215431=CARTESIAN_POINT('',(19.84920021178,-9.47413589477549,0.));
#215432=CARTESIAN_POINT('Origin',(7.08841632778409E-13,-3.26562511982935E-13,
0.));
#215433=CARTESIAN_POINT('Origin',(7.08841632778409E-13,-3.26562511982935E-13,
12.));
#215434=CARTESIAN_POINT('Origin',(7.08841632778409E-13,-3.26562511982935E-13,
0.));
#215435=CARTESIAN_POINT('Origin',(17.846350172984,-12.8649829188862,0.));
#215436=CARTESIAN_POINT('',(17.4407513054162,-12.572596943457,0.));
#215437=CARTESIAN_POINT('',(18.1294424696716,-12.4528436808172,0.));
#215438=CARTESIAN_POINT('Origin',(17.846350172984,-12.8649829188862,0.));
#215439=CARTESIAN_POINT('',(18.1294424696716,-12.4528436808172,12.));
#215440=CARTESIAN_POINT('',(18.1294424696716,-12.4528436808172,0.));
#215441=CARTESIAN_POINT('',(17.4407513054162,-12.572596943457,12.));
#215442=CARTESIAN_POINT('Origin',(17.846350172984,-12.8649829188862,12.));
#215443=CARTESIAN_POINT('',(17.4407513054162,-12.572596943457,0.));
#215444=CARTESIAN_POINT('Origin',(18.5896416359912,-12.7689476255363,0.));
#215445=CARTESIAN_POINT('',(18.5896416359912,-12.7689476255363,0.));
#215446=CARTESIAN_POINT('',(9.29482081799561,-6.38447381276812,0.));
#215447=CARTESIAN_POINT('',(18.5896416359912,-12.7689476255363,12.));
#215448=CARTESIAN_POINT('',(18.5896416359912,-12.7689476255363,0.));
#215449=CARTESIAN_POINT('',(9.29482081799561,-6.38447381276812,12.));
#215450=CARTESIAN_POINT('Origin',(17.0455945664569,-13.9085479427572,0.));
#215451=CARTESIAN_POINT('',(16.7207683102834,-14.2886635873976,0.));
#215452=CARTESIAN_POINT('',(16.6581946899465,-13.5924445804218,0.));
#215453=CARTESIAN_POINT('Origin',(17.0455945664569,-13.9085479427572,0.));
#215454=CARTESIAN_POINT('',(16.6581946899465,-13.5924445804218,12.));
#215455=CARTESIAN_POINT('',(16.6581946899465,-13.5924445804218,0.));
#215456=CARTESIAN_POINT('',(16.7207683102834,-14.2886635873976,12.));
#215457=CARTESIAN_POINT('Origin',(17.0455945664569,-13.9085479427572,12.));
#215458=CARTESIAN_POINT('',(16.7207683102834,-14.2886635873976,0.));
#215459=CARTESIAN_POINT('Origin',(6.00167842331873E-13,-4.9889687874677E-13,
0.));
#215460=CARTESIAN_POINT('Origin',(6.00167842331873E-13,-4.9889687874677E-13,
12.));
#215461=CARTESIAN_POINT('Origin',(6.00167842331873E-13,-4.9889687874677E-13,
0.));
#215462=CARTESIAN_POINT('Origin',(13.9085479427572,-17.0455945664569,0.));
#215463=CARTESIAN_POINT('',(13.5924445804218,-16.6581946899465,0.));
#215464=CARTESIAN_POINT('',(14.2886635873976,-16.7207683102834,0.));
#215465=CARTESIAN_POINT('Origin',(13.9085479427572,-17.0455945664569,0.));
#215466=CARTESIAN_POINT('',(14.2886635873976,-16.7207683102834,12.));
#215467=CARTESIAN_POINT('',(14.2886635873976,-16.7207683102834,0.));
#215468=CARTESIAN_POINT('',(13.5924445804218,-16.6581946899465,12.));
#215469=CARTESIAN_POINT('Origin',(13.9085479427572,-17.0455945664569,12.));
#215470=CARTESIAN_POINT('',(13.5924445804218,-16.6581946899465,0.));
#215471=CARTESIAN_POINT('Origin',(14.6513681262571,-17.1452095830633,0.));
#215472=CARTESIAN_POINT('',(14.6513681262571,-17.1452095830633,0.));
#215473=CARTESIAN_POINT('',(7.32568406312854,-8.57260479153162,0.));
#215474=CARTESIAN_POINT('',(14.6513681262571,-17.1452095830633,12.));
#215475=CARTESIAN_POINT('',(14.6513681262571,-17.1452095830633,0.));
#215476=CARTESIAN_POINT('',(7.32568406312854,-8.57260479153162,12.));
#215477=CARTESIAN_POINT('Origin',(12.8649829188862,-17.846350172984,0.));
#215478=CARTESIAN_POINT('',(12.4528436808172,-18.1294424696716,0.));
#215479=CARTESIAN_POINT('',(12.572596943457,-17.4407513054162,0.));
#215480=CARTESIAN_POINT('Origin',(12.8649829188862,-17.846350172984,0.));
#215481=CARTESIAN_POINT('',(12.572596943457,-17.4407513054162,12.));
#215482=CARTESIAN_POINT('',(12.572596943457,-17.4407513054162,0.));
#215483=CARTESIAN_POINT('',(12.4528436808172,-18.1294424696716,12.));
#215484=CARTESIAN_POINT('Origin',(12.8649829188862,-17.846350172984,12.));
#215485=CARTESIAN_POINT('',(12.4528436808172,-18.1294424696716,0.));
#215486=CARTESIAN_POINT('Origin',(4.50593605254674E-13,-6.37232247690087E-13,
0.));
#215487=CARTESIAN_POINT('Origin',(4.50593605254674E-13,-6.37232247690087E-13,
12.));
#215488=CARTESIAN_POINT('Origin',(4.50593605254674E-13,-6.37232247690087E-13,
0.));
#215489=CARTESIAN_POINT('Origin',(9.02290115519381,-20.0645771135004,0.));
#215490=CARTESIAN_POINT('',(8.81783521984849,-19.6085639972844,0.));
#215491=CARTESIAN_POINT('',(9.47413589477548,-19.84920021178,0.));
#215492=CARTESIAN_POINT('Origin',(9.02290115519381,-20.0645771135004,0.));
#215493=CARTESIAN_POINT('',(9.47413589477548,-19.84920021178,12.));
#215494=CARTESIAN_POINT('',(9.47413589477547,-19.84920021178,0.));
#215495=CARTESIAN_POINT('',(8.81783521984849,-19.6085639972844,12.));
#215496=CARTESIAN_POINT('Origin',(9.02290115519381,-20.0645771135004,12.));
#215497=CARTESIAN_POINT('',(8.81783521984849,-19.6085639972844,0.));
#215498=CARTESIAN_POINT('Origin',(9.71462809124915,-20.353053841303,0.));
#215499=CARTESIAN_POINT('',(9.71462809124915,-20.353053841303,0.));
#215500=CARTESIAN_POINT('',(4.85731404562459,-10.1765269206515,0.));
#215501=CARTESIAN_POINT('',(9.71462809124915,-20.353053841303,12.));
#215502=CARTESIAN_POINT('',(9.71462809124915,-20.353053841303,0.));
#215503=CARTESIAN_POINT('',(4.85731404562459,-10.1765269206515,12.));
#215504=CARTESIAN_POINT('Origin',(7.80764394578302,-20.56795313141,0.));
#215505=CARTESIAN_POINT('',(7.33627833380045,-20.7347298079577,0.));
#215506=CARTESIAN_POINT('',(7.63019749246977,-20.1004996511507,0.));
#215507=CARTESIAN_POINT('Origin',(7.80764394578302,-20.56795313141,0.));
#215508=CARTESIAN_POINT('',(7.63019749246977,-20.1004996511507,12.));
#215509=CARTESIAN_POINT('',(7.63019749246977,-20.1004996511507,0.));
#215510=CARTESIAN_POINT('',(7.33627833380045,-20.7347298079577,12.));
#215511=CARTESIAN_POINT('Origin',(7.80764394578302,-20.56795313141,12.));
#215512=CARTESIAN_POINT('',(7.33627833380045,-20.7347298079577,0.));
#215513=CARTESIAN_POINT('Origin',(2.70312158620511E-13,-7.32141292029404E-13,
0.));
#215514=CARTESIAN_POINT('Origin',(2.70312158620511E-13,-7.32141292029404E-13,
12.));
#215515=CARTESIAN_POINT('Origin',(2.70312158620511E-13,-7.32141292029404E-13,
0.));
#215516=CARTESIAN_POINT('Origin',(3.52235856495312,-21.7161918885403,0.));
#215517=CARTESIAN_POINT('',(3.44230496120418,-21.2226420728916,0.));
#215518=CARTESIAN_POINT('',(4.01396149767428,-21.624941921198,0.));
#215519=CARTESIAN_POINT('Origin',(3.52235856495312,-21.7161918885403,0.));
#215520=CARTESIAN_POINT('',(4.01396149767428,-21.624941921198,12.));
#215521=CARTESIAN_POINT('',(4.01396149767428,-21.624941921198,0.));
#215522=CARTESIAN_POINT('',(3.44230496120418,-21.2226420728916,12.));
#215523=CARTESIAN_POINT('Origin',(3.52235856495312,-21.7161918885403,12.));
#215524=CARTESIAN_POINT('',(3.44230496120418,-21.2226420728916,0.));
#215525=CARTESIAN_POINT('Origin',(4.11585220600461,-22.1738711152697,0.));
#215526=CARTESIAN_POINT('',(4.11585220600461,-22.1738711152697,0.));
#215527=CARTESIAN_POINT('',(2.05792610300232,-11.0869355576349,0.));
#215528=CARTESIAN_POINT('',(4.11585220600461,-22.1738711152697,12.));
#215529=CARTESIAN_POINT('',(4.11585220600461,-22.1738711152697,0.));
#215530=CARTESIAN_POINT('',(2.05792610300232,-11.0869355576349,12.));
#215531=CARTESIAN_POINT('Origin',(2.21822694051637,-21.8878840740801,0.));
#215532=CARTESIAN_POINT('',(1.71975774210841,-21.9269795755927,0.));
#215533=CARTESIAN_POINT('',(2.16781269186827,-21.3904321633055,0.));
#215534=CARTESIAN_POINT('Origin',(2.21822694051637,-21.8878840740801,0.));
#215535=CARTESIAN_POINT('',(2.16781269186827,-21.3904321633055,12.));
#215536=CARTESIAN_POINT('',(2.16781269186827,-21.3904321633055,0.));
#215537=CARTESIAN_POINT('',(1.71975774210841,-21.9269795755927,12.));
#215538=CARTESIAN_POINT('Origin',(2.21822694051637,-21.8878840740801,12.));
#215539=CARTESIAN_POINT('',(1.71975774210841,-21.9269795755927,0.));
#215540=CARTESIAN_POINT('Origin',(7.16093850883225E-14,-7.7715611723761E-13,
0.));
#215541=CARTESIAN_POINT('Origin',(7.16093850883225E-14,-7.7715611723761E-13,
12.));
#215542=CARTESIAN_POINT('Origin',(7.16093850883225E-14,-7.7715611723761E-13,
0.));
#215543=CARTESIAN_POINT('Origin',(-2.21822694051639,-21.88788407408,0.));
#215544=CARTESIAN_POINT('',(-2.16781269186829,-21.3904321633055,0.));
#215545=CARTESIAN_POINT('',(-1.71975774210843,-21.9269795755927,0.));
#215546=CARTESIAN_POINT('Origin',(-2.21822694051639,-21.88788407408,0.));
#215547=CARTESIAN_POINT('',(-1.71975774210843,-21.9269795755927,12.));
#215548=CARTESIAN_POINT('',(-1.71975774210843,-21.9269795755927,0.));
#215549=CARTESIAN_POINT('',(-2.16781269186829,-21.3904321633055,12.));
#215550=CARTESIAN_POINT('Origin',(-2.21822694051639,-21.88788407408,12.));
#215551=CARTESIAN_POINT('',(-2.16781269186829,-21.3904321633055,0.));
#215552=CARTESIAN_POINT('Origin',(-1.76341220531181,-22.4835757167854,0.));
#215553=CARTESIAN_POINT('',(-1.76341220531181,-22.4835757167854,0.));
#215554=CARTESIAN_POINT('',(-0.881706102655891,-11.2417878583927,0.));
#215555=CARTESIAN_POINT('',(-1.76341220531181,-22.4835757167854,12.));
#215556=CARTESIAN_POINT('',(-1.76341220531181,-22.4835757167854,0.));
#215557=CARTESIAN_POINT('',(-0.881706102655891,-11.2417878583927,12.));
#215558=CARTESIAN_POINT('Origin',(-3.52235856495314,-21.7161918885402,0.));
#215559=CARTESIAN_POINT('',(-4.0139614976743,-21.624941921198,0.));
#215560=CARTESIAN_POINT('',(-3.4423049612042,-21.2226420728916,0.));
#215561=CARTESIAN_POINT('Origin',(-3.52235856495314,-21.7161918885402,0.));
#215562=CARTESIAN_POINT('',(-3.4423049612042,-21.2226420728916,12.));
#215563=CARTESIAN_POINT('',(-3.4423049612042,-21.2226420728916,0.));
#215564=CARTESIAN_POINT('',(-4.0139614976743,-21.624941921198,12.));
#215565=CARTESIAN_POINT('Origin',(-3.52235856495314,-21.7161918885402,12.));
#215566=CARTESIAN_POINT('',(-4.0139614976743,-21.624941921198,0.));
#215567=CARTESIAN_POINT('Origin',(-1.31973449697531E-13,-7.6920903736728E-13,
0.));
#215568=CARTESIAN_POINT('Origin',(-1.31973449697531E-13,-7.6920903736728E-13,
12.));
#215569=CARTESIAN_POINT('Origin',(-1.31973449697531E-13,-7.6920903736728E-13,
0.));
#215570=CARTESIAN_POINT('Origin',(-7.80764394578304,-20.56795313141,0.));
#215571=CARTESIAN_POINT('',(-7.63019749246979,-20.1004996511507,0.));
#215572=CARTESIAN_POINT('',(-7.33627833380047,-20.7347298079577,0.));
#215573=CARTESIAN_POINT('Origin',(-7.80764394578304,-20.56795313141,0.));
#215574=CARTESIAN_POINT('',(-7.33627833380047,-20.7347298079577,12.));
#215575=CARTESIAN_POINT('',(-7.33627833380047,-20.7347298079577,0.));
#215576=CARTESIAN_POINT('',(-7.63019749246979,-20.1004996511507,12.));
#215577=CARTESIAN_POINT('Origin',(-7.80764394578304,-20.56795313141,12.));
#215578=CARTESIAN_POINT('',(-7.63019749246979,-20.1004996511507,0.));
#215579=CARTESIAN_POINT('Origin',(-7.52250298901266,-21.2610617890679,0.));
#215580=CARTESIAN_POINT('',(-7.52250298901266,-21.2610617890679,0.));
#215581=CARTESIAN_POINT('',(-3.76125149450632,-10.6305308945339,0.));
#215582=CARTESIAN_POINT('',(-7.52250298901266,-21.2610617890679,12.));
#215583=CARTESIAN_POINT('',(-7.52250298901266,-21.2610617890679,0.));
#215584=CARTESIAN_POINT('',(-3.76125149450632,-10.6305308945339,12.));
#215585=CARTESIAN_POINT('Origin',(-9.02290115519382,-20.0645771135003,0.));
#215586=CARTESIAN_POINT('',(-9.47413589477549,-19.84920021178,0.));
#215587=CARTESIAN_POINT('',(-8.81783521984851,-19.6085639972844,0.));
#215588=CARTESIAN_POINT('Origin',(-9.02290115519382,-20.0645771135003,0.));
#215589=CARTESIAN_POINT('',(-8.81783521984851,-19.6085639972844,12.));
#215590=CARTESIAN_POINT('',(-8.81783521984851,-19.6085639972844,0.));
#215591=CARTESIAN_POINT('',(-9.47413589477549,-19.84920021178,12.));
#215592=CARTESIAN_POINT('Origin',(-9.02290115519382,-20.0645771135003,12.));
#215593=CARTESIAN_POINT('',(-9.47413589477549,-19.84920021178,0.));
#215594=CARTESIAN_POINT('Origin',(-3.26562511982935E-13,-7.08841632778409E-13,
0.));
#215595=CARTESIAN_POINT('Origin',(-3.26562511982935E-13,-7.08841632778409E-13,
12.));
#215596=CARTESIAN_POINT('Origin',(-3.26562511982935E-13,-7.08841632778409E-13,
0.));
#215597=CARTESIAN_POINT('Origin',(-12.8649829188863,-17.846350172984,0.));
#215598=CARTESIAN_POINT('',(-12.572596943457,-17.4407513054161,0.));
#215599=CARTESIAN_POINT('',(-12.4528436808172,-18.1294424696716,0.));
#215600=CARTESIAN_POINT('Origin',(-12.8649829188863,-17.846350172984,0.));
#215601=CARTESIAN_POINT('',(-12.4528436808172,-18.1294424696716,12.));
#215602=CARTESIAN_POINT('',(-12.4528436808172,-18.1294424696716,0.));
#215603=CARTESIAN_POINT('',(-12.572596943457,-17.4407513054161,12.));
#215604=CARTESIAN_POINT('Origin',(-12.8649829188863,-17.846350172984,12.));
#215605=CARTESIAN_POINT('',(-12.572596943457,-17.4407513054161,0.));
#215606=CARTESIAN_POINT('Origin',(-12.7689476255363,-18.5896416359912,0.));
#215607=CARTESIAN_POINT('',(-12.7689476255363,-18.5896416359912,0.));
#215608=CARTESIAN_POINT('',(-6.38447381276812,-9.29482081799561,0.));
#215609=CARTESIAN_POINT('',(-12.7689476255363,-18.5896416359912,12.));
#215610=CARTESIAN_POINT('',(-12.7689476255363,-18.5896416359912,0.));
#215611=CARTESIAN_POINT('',(-6.38447381276812,-9.29482081799561,12.));
#215612=CARTESIAN_POINT('Origin',(-13.9085479427572,-17.0455945664569,0.));
#215613=CARTESIAN_POINT('',(-14.2886635873976,-16.7207683102834,0.));
#215614=CARTESIAN_POINT('',(-13.5924445804218,-16.6581946899465,0.));
#215615=CARTESIAN_POINT('Origin',(-13.9085479427572,-17.0455945664569,0.));
#215616=CARTESIAN_POINT('',(-13.5924445804218,-16.6581946899465,12.));
#215617=CARTESIAN_POINT('',(-13.5924445804218,-16.6581946899465,0.));
#215618=CARTESIAN_POINT('',(-14.2886635873976,-16.7207683102834,12.));
#215619=CARTESIAN_POINT('Origin',(-13.9085479427572,-17.0455945664569,12.));
#215620=CARTESIAN_POINT('',(-14.2886635873976,-16.7207683102834,0.));
#215621=CARTESIAN_POINT('Origin',(-4.9889687874677E-13,-6.00167842331873E-13,
0.));
#215622=CARTESIAN_POINT('Origin',(-4.9889687874677E-13,-6.00167842331873E-13,
12.));
#215623=CARTESIAN_POINT('Origin',(-4.9889687874677E-13,-6.00167842331873E-13,
0.));
#215624=CARTESIAN_POINT('Origin',(-17.0455945664569,-13.9085479427572,0.));
#215625=CARTESIAN_POINT('',(-16.6581946899465,-13.5924445804218,0.));
#215626=CARTESIAN_POINT('',(-16.7207683102834,-14.2886635873976,0.));
#215627=CARTESIAN_POINT('Origin',(-17.0455945664569,-13.9085479427572,0.));
#215628=CARTESIAN_POINT('',(-16.7207683102834,-14.2886635873976,12.));
#215629=CARTESIAN_POINT('',(-16.7207683102834,-14.2886635873976,0.));
#215630=CARTESIAN_POINT('',(-16.6581946899465,-13.5924445804218,12.));
#215631=CARTESIAN_POINT('Origin',(-17.0455945664569,-13.9085479427572,12.));
#215632=CARTESIAN_POINT('',(-16.6581946899465,-13.5924445804218,0.));
#215633=CARTESIAN_POINT('Origin',(-17.1452095830633,-14.6513681262571,0.));
#215634=CARTESIAN_POINT('',(-17.1452095830633,-14.6513681262571,0.));
#215635=CARTESIAN_POINT('',(-8.57260479153162,-7.32568406312855,0.));
#215636=CARTESIAN_POINT('',(-17.1452095830633,-14.6513681262571,12.));
#215637=CARTESIAN_POINT('',(-17.1452095830633,-14.6513681262571,0.));
#215638=CARTESIAN_POINT('',(-8.57260479153162,-7.32568406312855,12.));
#215639=CARTESIAN_POINT('Origin',(-17.846350172984,-12.8649829188862,0.));
#215640=CARTESIAN_POINT('',(-18.1294424696716,-12.4528436808172,0.));
#215641=CARTESIAN_POINT('',(-17.4407513054162,-12.572596943457,0.));
#215642=CARTESIAN_POINT('Origin',(-17.846350172984,-12.8649829188862,0.));
#215643=CARTESIAN_POINT('',(-17.4407513054162,-12.572596943457,12.));
#215644=CARTESIAN_POINT('',(-17.4407513054162,-12.572596943457,0.));
#215645=CARTESIAN_POINT('',(-18.1294424696716,-12.4528436808172,12.));
#215646=CARTESIAN_POINT('Origin',(-17.846350172984,-12.8649829188862,12.));
#215647=CARTESIAN_POINT('',(-18.1294424696716,-12.4528436808172,0.));
#215648=CARTESIAN_POINT('Origin',(-6.37232247690086E-13,-4.50593605254675E-13,
0.));
#215649=CARTESIAN_POINT('Origin',(-6.37232247690086E-13,-4.50593605254675E-13,
12.));
#215650=CARTESIAN_POINT('Origin',(-6.37232247690086E-13,-4.50593605254675E-13,
0.));
#215651=CARTESIAN_POINT('Origin',(-20.0645771135004,-9.0229011551938,0.));
#215652=CARTESIAN_POINT('',(-19.6085639972844,-8.81783521984849,0.));
#215653=CARTESIAN_POINT('',(-19.84920021178,-9.47413589477548,0.));
#215654=CARTESIAN_POINT('Origin',(-20.0645771135004,-9.0229011551938,0.));
#215655=CARTESIAN_POINT('',(-19.84920021178,-9.47413589477548,12.));
#215656=CARTESIAN_POINT('',(-19.84920021178,-9.47413589477547,0.));
#215657=CARTESIAN_POINT('',(-19.6085639972844,-8.81783521984849,12.));
#215658=CARTESIAN_POINT('Origin',(-20.0645771135004,-9.0229011551938,12.));
#215659=CARTESIAN_POINT('',(-19.6085639972844,-8.81783521984849,0.));
#215660=CARTESIAN_POINT('Origin',(-20.353053841303,-9.71462809124915,0.));
#215661=CARTESIAN_POINT('',(-20.353053841303,-9.71462809124915,0.));
#215662=CARTESIAN_POINT('',(-10.1765269206515,-4.85731404562459,0.));
#215663=CARTESIAN_POINT('',(-20.353053841303,-9.71462809124915,12.));
#215664=CARTESIAN_POINT('',(-20.353053841303,-9.71462809124915,0.));
#215665=CARTESIAN_POINT('',(-10.1765269206515,-4.85731404562459,12.));
#215666=CARTESIAN_POINT('Origin',(-20.56795313141,-7.80764394578302,0.));
#215667=CARTESIAN_POINT('',(-20.7347298079577,-7.33627833380045,0.));
#215668=CARTESIAN_POINT('',(-20.1004996511507,-7.63019749246977,0.));
#215669=CARTESIAN_POINT('Origin',(-20.56795313141,-7.80764394578302,0.));
#215670=CARTESIAN_POINT('',(-20.1004996511507,-7.63019749246977,12.));
#215671=CARTESIAN_POINT('',(-20.1004996511507,-7.63019749246977,0.));
#215672=CARTESIAN_POINT('',(-20.7347298079577,-7.33627833380045,12.));
#215673=CARTESIAN_POINT('Origin',(-20.56795313141,-7.80764394578302,12.));
#215674=CARTESIAN_POINT('',(-20.7347298079577,-7.33627833380045,0.));
#215675=CARTESIAN_POINT('Origin',(-7.32141292029404E-13,-2.70312158620511E-13,
0.));
#215676=CARTESIAN_POINT('Origin',(-7.32141292029404E-13,-2.70312158620511E-13,
12.));
#215677=CARTESIAN_POINT('Origin',(-7.32141292029404E-13,-2.70312158620511E-13,
0.));
#215678=CARTESIAN_POINT('Origin',(-21.7161918885403,-3.52235856495312,0.));
#215679=CARTESIAN_POINT('',(-21.2226420728916,-3.44230496120418,0.));
#215680=CARTESIAN_POINT('',(-21.624941921198,-4.01396149767428,0.));
#215681=CARTESIAN_POINT('Origin',(-21.7161918885403,-3.52235856495312,0.));
#215682=CARTESIAN_POINT('',(-21.624941921198,-4.01396149767428,12.));
#215683=CARTESIAN_POINT('',(-21.624941921198,-4.01396149767428,0.));
#215684=CARTESIAN_POINT('',(-21.2226420728916,-3.44230496120418,12.));
#215685=CARTESIAN_POINT('Origin',(-21.7161918885403,-3.52235856495312,12.));
#215686=CARTESIAN_POINT('',(-21.2226420728916,-3.44230496120418,0.));
#215687=CARTESIAN_POINT('Origin',(-22.1738711152697,-4.11585220600461,0.));
#215688=CARTESIAN_POINT('',(-22.1738711152697,-4.11585220600461,0.));
#215689=CARTESIAN_POINT('',(-11.0869355576349,-2.05792610300232,0.));
#215690=CARTESIAN_POINT('',(-22.1738711152697,-4.11585220600461,12.));
#215691=CARTESIAN_POINT('',(-22.1738711152697,-4.11585220600461,0.));
#215692=CARTESIAN_POINT('',(-11.0869355576349,-2.05792610300232,12.));
#215693=CARTESIAN_POINT('Origin',(-21.8878840740801,-2.21822694051637,0.));
#215694=CARTESIAN_POINT('',(-21.9269795755927,-1.71975774210841,0.));
#215695=CARTESIAN_POINT('',(-21.3904321633055,-2.16781269186828,0.));
#215696=CARTESIAN_POINT('Origin',(-21.8878840740801,-2.21822694051637,0.));
#215697=CARTESIAN_POINT('',(-21.3904321633055,-2.16781269186828,12.));
#215698=CARTESIAN_POINT('',(-21.3904321633055,-2.16781269186827,0.));
#215699=CARTESIAN_POINT('',(-21.9269795755927,-1.71975774210841,12.));
#215700=CARTESIAN_POINT('Origin',(-21.8878840740801,-2.21822694051637,12.));
#215701=CARTESIAN_POINT('',(-21.9269795755927,-1.71975774210841,0.));
#215702=CARTESIAN_POINT('Origin',(-7.7715611723761E-13,-7.16093850883225E-14,
0.));
#215703=CARTESIAN_POINT('Origin',(-7.7715611723761E-13,-7.16093850883225E-14,
12.));
#215704=CARTESIAN_POINT('Origin',(-7.7715611723761E-13,-7.16093850883225E-14,
0.));
#215705=CARTESIAN_POINT('Origin',(-21.8878840740801,2.21822694051638,0.));
#215706=CARTESIAN_POINT('',(-21.3904321633055,2.16781269186828,0.));
#215707=CARTESIAN_POINT('',(-21.9269795755927,1.71975774210842,0.));
#215708=CARTESIAN_POINT('Origin',(-21.8878840740801,2.21822694051638,0.));
#215709=CARTESIAN_POINT('',(-21.9269795755927,1.71975774210842,12.));
#215710=CARTESIAN_POINT('',(-21.9269795755927,1.71975774210842,0.));
#215711=CARTESIAN_POINT('',(-21.3904321633055,2.16781269186828,12.));
#215712=CARTESIAN_POINT('Origin',(-21.8878840740801,2.21822694051638,12.));
#215713=CARTESIAN_POINT('',(-21.3904321633055,2.16781269186828,0.));
#215714=CARTESIAN_POINT('Origin',(-22.4835757167854,1.7634122053118,0.));
#215715=CARTESIAN_POINT('',(-22.4835757167854,1.7634122053118,0.));
#215716=CARTESIAN_POINT('',(-11.2417878583927,0.881706102655883,0.));
#215717=CARTESIAN_POINT('',(-22.4835757167854,1.7634122053118,12.));
#215718=CARTESIAN_POINT('',(-22.4835757167854,1.7634122053118,0.));
#215719=CARTESIAN_POINT('',(-11.2417878583927,0.881706102655883,12.));
#215720=CARTESIAN_POINT('Origin',(-21.7161918885402,3.52235856495312,0.));
#215721=CARTESIAN_POINT('',(-21.624941921198,4.01396149767429,0.));
#215722=CARTESIAN_POINT('',(-21.2226420728916,3.44230496120419,0.));
#215723=CARTESIAN_POINT('Origin',(-21.7161918885402,3.52235856495312,0.));
#215724=CARTESIAN_POINT('',(-21.2226420728916,3.44230496120419,12.));
#215725=CARTESIAN_POINT('',(-21.2226420728916,3.44230496120419,0.));
#215726=CARTESIAN_POINT('',(-21.624941921198,4.01396149767429,12.));
#215727=CARTESIAN_POINT('Origin',(-21.7161918885402,3.52235856495312,12.));
#215728=CARTESIAN_POINT('',(-21.624941921198,4.01396149767429,0.));
#215729=CARTESIAN_POINT('Origin',(-7.6920903736728E-13,1.31973449697531E-13,
0.));
#215730=CARTESIAN_POINT('Origin',(-7.6920903736728E-13,1.31973449697531E-13,
12.));
#215731=CARTESIAN_POINT('Origin',(-7.6920903736728E-13,1.31973449697531E-13,
0.));
#215732=CARTESIAN_POINT('Origin',(-20.56795313141,7.80764394578303,0.));
#215733=CARTESIAN_POINT('',(-20.1004996511507,7.63019749246978,0.));
#215734=CARTESIAN_POINT('',(-20.7347298079577,7.33627833380047,0.));
#215735=CARTESIAN_POINT('Origin',(-20.56795313141,7.80764394578303,0.));
#215736=CARTESIAN_POINT('',(-20.7347298079577,7.33627833380047,12.));
#215737=CARTESIAN_POINT('',(-20.7347298079577,7.33627833380047,0.));
#215738=CARTESIAN_POINT('',(-20.1004996511507,7.63019749246978,12.));
#215739=CARTESIAN_POINT('Origin',(-20.56795313141,7.80764394578303,12.));
#215740=CARTESIAN_POINT('',(-20.1004996511507,7.63019749246978,0.));
#215741=CARTESIAN_POINT('Origin',(-21.2610617890679,7.52250298901265,0.));
#215742=CARTESIAN_POINT('',(-21.2610617890679,7.52250298901265,0.));
#215743=CARTESIAN_POINT('',(-10.6305308945339,3.76125149450631,0.));
#215744=CARTESIAN_POINT('',(-21.2610617890679,7.52250298901265,12.));
#215745=CARTESIAN_POINT('',(-21.2610617890679,7.52250298901265,0.));
#215746=CARTESIAN_POINT('',(-10.6305308945339,3.76125149450631,12.));
#215747=CARTESIAN_POINT('Origin',(-20.0645771135003,9.02290115519382,0.));
#215748=CARTESIAN_POINT('',(-19.84920021178,9.47413589477549,0.));
#215749=CARTESIAN_POINT('',(-19.6085639972844,8.81783521984851,0.));
#215750=CARTESIAN_POINT('Origin',(-20.0645771135003,9.02290115519382,0.));
#215751=CARTESIAN_POINT('',(-19.6085639972844,8.81783521984851,12.));
#215752=CARTESIAN_POINT('',(-19.6085639972844,8.81783521984851,0.));
#215753=CARTESIAN_POINT('',(-19.84920021178,9.47413589477549,12.));
#215754=CARTESIAN_POINT('Origin',(-20.0645771135003,9.02290115519382,12.));
#215755=CARTESIAN_POINT('',(-19.84920021178,9.47413589477549,0.));
#215756=CARTESIAN_POINT('Origin',(-7.08841632778408E-13,3.26562511982935E-13,
0.));
#215757=CARTESIAN_POINT('Origin',(-7.08841632778408E-13,3.26562511982935E-13,
12.));
#215758=CARTESIAN_POINT('Origin',(-7.08841632778408E-13,3.26562511982935E-13,
0.));
#215759=CARTESIAN_POINT('Origin',(-17.846350172984,12.8649829188862,0.));
#215760=CARTESIAN_POINT('',(-17.4407513054162,12.572596943457,0.));
#215761=CARTESIAN_POINT('',(-18.1294424696716,12.4528436808172,0.));
#215762=CARTESIAN_POINT('Origin',(-17.846350172984,12.8649829188862,0.));
#215763=CARTESIAN_POINT('',(-18.1294424696716,12.4528436808172,12.));
#215764=CARTESIAN_POINT('',(-18.1294424696716,12.4528436808172,0.));
#215765=CARTESIAN_POINT('',(-17.4407513054162,12.572596943457,12.));
#215766=CARTESIAN_POINT('Origin',(-17.846350172984,12.8649829188862,12.));
#215767=CARTESIAN_POINT('',(-17.4407513054162,12.572596943457,0.));
#215768=CARTESIAN_POINT('Origin',(-18.5896416359912,12.7689476255363,0.));
#215769=CARTESIAN_POINT('',(-18.5896416359912,12.7689476255363,0.));
#215770=CARTESIAN_POINT('',(-9.29482081799561,6.38447381276812,0.));
#215771=CARTESIAN_POINT('',(-18.5896416359912,12.7689476255363,12.));
#215772=CARTESIAN_POINT('',(-18.5896416359912,12.7689476255363,0.));
#215773=CARTESIAN_POINT('',(-9.29482081799561,6.38447381276812,12.));
#215774=CARTESIAN_POINT('Origin',(-17.0455945664569,13.9085479427572,0.));
#215775=CARTESIAN_POINT('',(-16.7207683102834,14.2886635873976,0.));
#215776=CARTESIAN_POINT('',(-16.6581946899465,13.5924445804218,0.));
#215777=CARTESIAN_POINT('Origin',(-17.0455945664569,13.9085479427572,0.));
#215778=CARTESIAN_POINT('',(-16.6581946899465,13.5924445804218,12.));
#215779=CARTESIAN_POINT('',(-16.6581946899465,13.5924445804218,0.));
#215780=CARTESIAN_POINT('',(-16.7207683102834,14.2886635873976,12.));
#215781=CARTESIAN_POINT('Origin',(-17.0455945664569,13.9085479427572,12.));
#215782=CARTESIAN_POINT('',(-16.7207683102834,14.2886635873976,0.));
#215783=CARTESIAN_POINT('Origin',(-6.00167842331873E-13,4.9889687874677E-13,
0.));
#215784=CARTESIAN_POINT('Origin',(-6.00167842331873E-13,4.9889687874677E-13,
12.));
#215785=CARTESIAN_POINT('Origin',(-6.00167842331873E-13,4.9889687874677E-13,
0.));
#215786=CARTESIAN_POINT('Origin',(-13.9085479427572,17.0455945664569,0.));
#215787=CARTESIAN_POINT('',(-13.5924445804218,16.6581946899465,0.));
#215788=CARTESIAN_POINT('',(-14.2886635873976,16.7207683102834,0.));
#215789=CARTESIAN_POINT('Origin',(-13.9085479427572,17.0455945664569,0.));
#215790=CARTESIAN_POINT('',(-14.2886635873976,16.7207683102834,12.));
#215791=CARTESIAN_POINT('',(-14.2886635873976,16.7207683102834,0.));
#215792=CARTESIAN_POINT('',(-13.5924445804218,16.6581946899465,12.));
#215793=CARTESIAN_POINT('Origin',(-13.9085479427572,17.0455945664569,12.));
#215794=CARTESIAN_POINT('',(-13.5924445804218,16.6581946899465,0.));
#215795=CARTESIAN_POINT('Origin',(-14.6513681262571,17.1452095830633,0.));
#215796=CARTESIAN_POINT('',(-14.6513681262571,17.1452095830633,0.));
#215797=CARTESIAN_POINT('',(-7.32568406312854,8.57260479153162,0.));
#215798=CARTESIAN_POINT('',(-14.6513681262571,17.1452095830633,12.));
#215799=CARTESIAN_POINT('',(-14.6513681262571,17.1452095830633,0.));
#215800=CARTESIAN_POINT('',(-7.32568406312854,8.57260479153162,12.));
#215801=CARTESIAN_POINT('Origin',(-12.8649829188862,17.846350172984,0.));
#215802=CARTESIAN_POINT('',(-12.4528436808172,18.1294424696716,0.));
#215803=CARTESIAN_POINT('',(-12.572596943457,17.4407513054162,0.));
#215804=CARTESIAN_POINT('Origin',(-12.8649829188862,17.846350172984,0.));
#215805=CARTESIAN_POINT('',(-12.572596943457,17.4407513054162,12.));
#215806=CARTESIAN_POINT('',(-12.572596943457,17.4407513054162,0.));
#215807=CARTESIAN_POINT('',(-12.4528436808172,18.1294424696716,12.));
#215808=CARTESIAN_POINT('Origin',(-12.8649829188862,17.846350172984,12.));
#215809=CARTESIAN_POINT('',(-12.4528436808172,18.1294424696716,0.));
#215810=CARTESIAN_POINT('Origin',(-4.50593605254675E-13,6.37232247690086E-13,
0.));
#215811=CARTESIAN_POINT('Origin',(-4.50593605254675E-13,6.37232247690086E-13,
12.));
#215812=CARTESIAN_POINT('Origin',(-4.50593605254675E-13,6.37232247690086E-13,
0.));
#215813=CARTESIAN_POINT('Origin',(-9.02290115519381,20.0645771135003,0.));
#215814=CARTESIAN_POINT('',(-8.8178352198485,19.6085639972844,0.));
#215815=CARTESIAN_POINT('',(-9.47413589477548,19.84920021178,0.));
#215816=CARTESIAN_POINT('Origin',(-9.02290115519381,20.0645771135003,0.));
#215817=CARTESIAN_POINT('',(-9.47413589477548,19.84920021178,12.));
#215818=CARTESIAN_POINT('',(-9.47413589477548,19.84920021178,0.));
#215819=CARTESIAN_POINT('',(-8.8178352198485,19.6085639972844,12.));
#215820=CARTESIAN_POINT('Origin',(-9.02290115519381,20.0645771135003,12.));
#215821=CARTESIAN_POINT('',(-8.8178352198485,19.6085639972844,0.));
#215822=CARTESIAN_POINT('Origin',(-9.71462809124916,20.353053841303,0.));
#215823=CARTESIAN_POINT('',(-9.71462809124916,20.353053841303,0.));
#215824=CARTESIAN_POINT('',(-4.85731404562459,10.1765269206515,0.));
#215825=CARTESIAN_POINT('',(-9.71462809124916,20.353053841303,12.));
#215826=CARTESIAN_POINT('',(-9.71462809124916,20.353053841303,0.));
#215827=CARTESIAN_POINT('',(-4.85731404562459,10.1765269206515,12.));
#215828=CARTESIAN_POINT('Origin',(-7.80764394578302,20.56795313141,0.));
#215829=CARTESIAN_POINT('',(-7.33627833380046,20.7347298079577,0.));
#215830=CARTESIAN_POINT('',(-7.63019749246977,20.1004996511507,0.));
#215831=CARTESIAN_POINT('Origin',(-7.80764394578302,20.56795313141,0.));
#215832=CARTESIAN_POINT('',(-7.63019749246977,20.1004996511507,12.));
#215833=CARTESIAN_POINT('',(-7.63019749246977,20.1004996511507,0.));
#215834=CARTESIAN_POINT('',(-7.33627833380046,20.7347298079577,12.));
#215835=CARTESIAN_POINT('Origin',(-7.80764394578302,20.56795313141,12.));
#215836=CARTESIAN_POINT('',(-7.33627833380046,20.7347298079577,0.));
#215837=CARTESIAN_POINT('Origin',(-2.70312158620511E-13,7.32141292029404E-13,
0.));
#215838=CARTESIAN_POINT('Origin',(-2.70312158620511E-13,7.32141292029404E-13,
12.));
#215839=CARTESIAN_POINT('Origin',(-2.70312158620511E-13,7.32141292029404E-13,
0.));
#215840=CARTESIAN_POINT('Origin',(-3.52235856495312,21.7161918885402,0.));
#215841=CARTESIAN_POINT('',(-3.44230496120418,21.2226420728916,0.));
#215842=CARTESIAN_POINT('',(-4.01396149767428,21.624941921198,0.));
#215843=CARTESIAN_POINT('Origin',(-3.52235856495312,21.7161918885402,0.));
#215844=CARTESIAN_POINT('',(-4.01396149767428,21.624941921198,12.));
#215845=CARTESIAN_POINT('',(-4.01396149767428,21.624941921198,0.));
#215846=CARTESIAN_POINT('',(-3.44230496120418,21.2226420728916,12.));
#215847=CARTESIAN_POINT('Origin',(-3.52235856495312,21.7161918885402,12.));
#215848=CARTESIAN_POINT('',(-3.44230496120418,21.2226420728916,0.));
#215849=CARTESIAN_POINT('Origin',(-4.11585220600461,22.1738711152697,0.));
#215850=CARTESIAN_POINT('',(-4.11585220600461,22.1738711152697,0.));
#215851=CARTESIAN_POINT('',(-2.05792610300232,11.0869355576349,0.));
#215852=CARTESIAN_POINT('',(-4.11585220600461,22.1738711152697,12.));
#215853=CARTESIAN_POINT('',(-4.11585220600461,22.1738711152697,0.));
#215854=CARTESIAN_POINT('',(-2.05792610300232,11.0869355576349,12.));
#215855=CARTESIAN_POINT('Origin',(-2.21822694051637,21.8878840740801,0.));
#215856=CARTESIAN_POINT('',(-1.71975774210841,21.9269795755927,0.));
#215857=CARTESIAN_POINT('',(-2.16781269186828,21.3904321633055,0.));
#215858=CARTESIAN_POINT('Origin',(-2.21822694051637,21.8878840740801,0.));
#215859=CARTESIAN_POINT('',(-2.16781269186828,21.3904321633055,12.));
#215860=CARTESIAN_POINT('',(-2.16781269186828,21.3904321633055,0.));
#215861=CARTESIAN_POINT('',(-1.71975774210841,21.9269795755927,12.));
#215862=CARTESIAN_POINT('Origin',(-2.21822694051637,21.8878840740801,12.));
#215863=CARTESIAN_POINT('',(-1.71975774210841,21.9269795755927,0.));
#215864=CARTESIAN_POINT('Origin',(-7.16093850883226E-14,7.7715611723761E-13,
0.));
#215865=CARTESIAN_POINT('Origin',(-7.16093850883226E-14,7.7715611723761E-13,
12.));
#215866=CARTESIAN_POINT('Origin',(-7.16093850883226E-14,7.7715611723761E-13,
0.));
#215867=CARTESIAN_POINT('Origin',(2.21822694051638,21.8878840740801,0.));
#215868=CARTESIAN_POINT('',(2.16781269186828,21.3904321633055,0.));
#215869=CARTESIAN_POINT('',(1.71975774210842,21.9269795755927,0.));
#215870=CARTESIAN_POINT('Origin',(2.21822694051638,21.8878840740801,0.));
#215871=CARTESIAN_POINT('',(1.71975774210842,21.9269795755927,12.));
#215872=CARTESIAN_POINT('',(1.71975774210842,21.9269795755927,0.));
#215873=CARTESIAN_POINT('',(2.16781269186828,21.3904321633055,12.));
#215874=CARTESIAN_POINT('Origin',(2.21822694051638,21.8878840740801,12.));
#215875=CARTESIAN_POINT('',(2.16781269186828,21.3904321633055,0.));
#215876=CARTESIAN_POINT('Origin',(1.7634122053118,22.4835757167854,0.));
#215877=CARTESIAN_POINT('',(1.7634122053118,22.4835757167854,0.));
#215878=CARTESIAN_POINT('',(0.881706102655883,11.2417878583927,0.));
#215879=CARTESIAN_POINT('',(1.7634122053118,22.4835757167854,12.));
#215880=CARTESIAN_POINT('',(1.7634122053118,22.4835757167854,0.));
#215881=CARTESIAN_POINT('',(0.881706102655883,11.2417878583927,12.));
#215882=CARTESIAN_POINT('Origin',(3.52235856495312,21.7161918885402,0.));
#215883=CARTESIAN_POINT('',(4.01396149767429,21.624941921198,0.));
#215884=CARTESIAN_POINT('',(3.44230496120419,21.2226420728916,0.));
#215885=CARTESIAN_POINT('Origin',(3.52235856495312,21.7161918885402,0.));
#215886=CARTESIAN_POINT('',(3.44230496120419,21.2226420728916,12.));
#215887=CARTESIAN_POINT('',(3.44230496120419,21.2226420728916,0.));
#215888=CARTESIAN_POINT('',(4.01396149767429,21.624941921198,12.));
#215889=CARTESIAN_POINT('Origin',(3.52235856495312,21.7161918885402,12.));
#215890=CARTESIAN_POINT('',(4.01396149767429,21.624941921198,0.));
#215891=CARTESIAN_POINT('Origin',(1.31973449697531E-13,7.6920903736728E-13,
0.));
#215892=CARTESIAN_POINT('Origin',(1.31973449697531E-13,7.6920903736728E-13,
12.));
#215893=CARTESIAN_POINT('Origin',(1.31973449697531E-13,7.6920903736728E-13,
0.));
#215894=CARTESIAN_POINT('Origin',(7.80764394578303,20.56795313141,0.));
#215895=CARTESIAN_POINT('',(7.63019749246978,20.1004996511507,0.));
#215896=CARTESIAN_POINT('',(7.33627833380047,20.7347298079577,0.));
#215897=CARTESIAN_POINT('Origin',(7.80764394578303,20.56795313141,0.));
#215898=CARTESIAN_POINT('',(7.33627833380047,20.7347298079577,12.));
#215899=CARTESIAN_POINT('',(7.33627833380046,20.7347298079577,0.));
#215900=CARTESIAN_POINT('',(7.63019749246978,20.1004996511507,12.));
#215901=CARTESIAN_POINT('Origin',(7.80764394578303,20.56795313141,12.));
#215902=CARTESIAN_POINT('',(7.63019749246978,20.1004996511507,0.));
#215903=CARTESIAN_POINT('Origin',(7.52250298901265,21.2610617890679,0.));
#215904=CARTESIAN_POINT('',(7.52250298901265,21.2610617890679,0.));
#215905=CARTESIAN_POINT('',(3.76125149450631,10.6305308945339,0.));
#215906=CARTESIAN_POINT('',(7.52250298901265,21.2610617890679,12.));
#215907=CARTESIAN_POINT('',(7.52250298901265,21.2610617890679,0.));
#215908=CARTESIAN_POINT('',(3.76125149450631,10.6305308945339,12.));
#215909=CARTESIAN_POINT('Origin',(9.02290115519382,20.0645771135003,0.));
#215910=CARTESIAN_POINT('',(9.47413589477549,19.84920021178,0.));
#215911=CARTESIAN_POINT('',(8.8178352198485,19.6085639972844,0.));
#215912=CARTESIAN_POINT('Origin',(9.02290115519382,20.0645771135003,0.));
#215913=CARTESIAN_POINT('',(8.8178352198485,19.6085639972844,12.));
#215914=CARTESIAN_POINT('',(8.8178352198485,19.6085639972844,0.));
#215915=CARTESIAN_POINT('',(9.47413589477549,19.84920021178,12.));
#215916=CARTESIAN_POINT('Origin',(9.02290115519382,20.0645771135003,12.));
#215917=CARTESIAN_POINT('',(9.47413589477549,19.84920021178,0.));
#215918=CARTESIAN_POINT('Origin',(3.26562511982935E-13,7.08841632778409E-13,
0.));
#215919=CARTESIAN_POINT('Origin',(3.26562511982935E-13,7.08841632778409E-13,
12.));
#215920=CARTESIAN_POINT('Origin',(3.26562511982935E-13,7.08841632778409E-13,
0.));
#215921=CARTESIAN_POINT('Origin',(12.8649829188862,17.846350172984,0.));
#215922=CARTESIAN_POINT('',(12.572596943457,17.4407513054162,0.));
#215923=CARTESIAN_POINT('',(12.4528436808172,18.1294424696716,0.));
#215924=CARTESIAN_POINT('Origin',(12.8649829188862,17.846350172984,0.));
#215925=CARTESIAN_POINT('',(12.4528436808172,18.1294424696716,12.));
#215926=CARTESIAN_POINT('',(12.4528436808172,18.1294424696716,0.));
#215927=CARTESIAN_POINT('',(12.572596943457,17.4407513054162,12.));
#215928=CARTESIAN_POINT('Origin',(12.8649829188862,17.846350172984,12.));
#215929=CARTESIAN_POINT('',(12.572596943457,17.4407513054162,0.));
#215930=CARTESIAN_POINT('Origin',(12.7689476255363,18.5896416359912,0.));
#215931=CARTESIAN_POINT('',(12.7689476255363,18.5896416359912,0.));
#215932=CARTESIAN_POINT('',(6.38447381276812,9.29482081799561,0.));
#215933=CARTESIAN_POINT('',(12.7689476255363,18.5896416359912,12.));
#215934=CARTESIAN_POINT('',(12.7689476255363,18.5896416359912,0.));
#215935=CARTESIAN_POINT('',(6.38447381276812,9.29482081799561,12.));
#215936=CARTESIAN_POINT('Origin',(13.9085479427572,17.0455945664569,0.));
#215937=CARTESIAN_POINT('',(14.2886635873976,16.7207683102834,0.));
#215938=CARTESIAN_POINT('',(13.5924445804218,16.6581946899465,0.));
#215939=CARTESIAN_POINT('Origin',(13.9085479427572,17.0455945664569,0.));
#215940=CARTESIAN_POINT('',(13.5924445804218,16.6581946899465,12.));
#215941=CARTESIAN_POINT('',(13.5924445804218,16.6581946899465,0.));
#215942=CARTESIAN_POINT('',(14.2886635873976,16.7207683102834,12.));
#215943=CARTESIAN_POINT('Origin',(13.9085479427572,17.0455945664569,12.));
#215944=CARTESIAN_POINT('',(14.2886635873976,16.7207683102834,0.));
#215945=CARTESIAN_POINT('Origin',(4.9889687874677E-13,6.00167842331873E-13,
0.));
#215946=CARTESIAN_POINT('Origin',(4.9889687874677E-13,6.00167842331873E-13,
12.));
#215947=CARTESIAN_POINT('Origin',(4.9889687874677E-13,6.00167842331873E-13,
0.));
#215948=CARTESIAN_POINT('Origin',(17.0455945664569,13.9085479427572,0.));
#215949=CARTESIAN_POINT('',(16.6581946899465,13.5924445804218,0.));
#215950=CARTESIAN_POINT('',(16.7207683102834,14.2886635873976,0.));
#215951=CARTESIAN_POINT('Origin',(17.0455945664569,13.9085479427572,0.));
#215952=CARTESIAN_POINT('',(16.7207683102834,14.2886635873976,12.));
#215953=CARTESIAN_POINT('',(16.7207683102834,14.2886635873976,0.));
#215954=CARTESIAN_POINT('',(16.6581946899465,13.5924445804218,12.));
#215955=CARTESIAN_POINT('Origin',(17.0455945664569,13.9085479427572,12.));
#215956=CARTESIAN_POINT('',(16.6581946899465,13.5924445804218,0.));
#215957=CARTESIAN_POINT('Origin',(17.1452095830633,14.6513681262571,0.));
#215958=CARTESIAN_POINT('',(17.1452095830633,14.6513681262571,0.));
#215959=CARTESIAN_POINT('',(8.57260479153162,7.32568406312855,0.));
#215960=CARTESIAN_POINT('',(17.1452095830633,14.6513681262571,12.));
#215961=CARTESIAN_POINT('',(17.1452095830633,14.6513681262571,0.));
#215962=CARTESIAN_POINT('',(8.57260479153162,7.32568406312855,12.));
#215963=CARTESIAN_POINT('Origin',(17.846350172984,12.8649829188862,0.));
#215964=CARTESIAN_POINT('',(18.1294424696716,12.4528436808172,0.));
#215965=CARTESIAN_POINT('',(17.4407513054162,12.572596943457,0.));
#215966=CARTESIAN_POINT('Origin',(17.846350172984,12.8649829188862,0.));
#215967=CARTESIAN_POINT('',(17.4407513054162,12.572596943457,12.));
#215968=CARTESIAN_POINT('',(17.4407513054162,12.572596943457,0.));
#215969=CARTESIAN_POINT('',(18.1294424696716,12.4528436808172,12.));
#215970=CARTESIAN_POINT('Origin',(17.846350172984,12.8649829188862,12.));
#215971=CARTESIAN_POINT('',(18.1294424696716,12.4528436808172,0.));
#215972=CARTESIAN_POINT('Origin',(6.37232247690086E-13,4.50593605254675E-13,
0.));
#215973=CARTESIAN_POINT('Origin',(6.37232247690086E-13,4.50593605254675E-13,
12.));
#215974=CARTESIAN_POINT('Origin',(6.37232247690086E-13,4.50593605254675E-13,
0.));
#215975=CARTESIAN_POINT('Origin',(20.0645771135003,9.02290115519381,0.));
#215976=CARTESIAN_POINT('',(19.6085639972844,8.8178352198485,0.));
#215977=CARTESIAN_POINT('',(19.84920021178,9.47413589477548,0.));
#215978=CARTESIAN_POINT('Origin',(20.0645771135003,9.02290115519381,0.));
#215979=CARTESIAN_POINT('',(19.84920021178,9.47413589477548,12.));
#215980=CARTESIAN_POINT('',(19.84920021178,9.47413589477548,0.));
#215981=CARTESIAN_POINT('',(19.6085639972844,8.8178352198485,12.));
#215982=CARTESIAN_POINT('Origin',(20.0645771135003,9.02290115519381,12.));
#215983=CARTESIAN_POINT('',(19.6085639972844,8.8178352198485,0.));
#215984=CARTESIAN_POINT('Origin',(20.353053841303,9.71462809124916,0.));
#215985=CARTESIAN_POINT('',(20.353053841303,9.71462809124916,0.));
#215986=CARTESIAN_POINT('',(10.1765269206515,4.85731404562459,0.));
#215987=CARTESIAN_POINT('',(20.353053841303,9.71462809124916,12.));
#215988=CARTESIAN_POINT('',(20.353053841303,9.71462809124916,0.));
#215989=CARTESIAN_POINT('',(10.1765269206515,4.85731404562459,12.));
#215990=CARTESIAN_POINT('Origin',(20.56795313141,7.80764394578302,0.));
#215991=CARTESIAN_POINT('',(20.7347298079577,7.33627833380046,0.));
#215992=CARTESIAN_POINT('',(20.1004996511507,7.63019749246977,0.));
#215993=CARTESIAN_POINT('Origin',(20.56795313141,7.80764394578302,0.));
#215994=CARTESIAN_POINT('',(20.1004996511507,7.63019749246977,12.));
#215995=CARTESIAN_POINT('',(20.1004996511507,7.63019749246977,0.));
#215996=CARTESIAN_POINT('',(20.7347298079577,7.33627833380046,12.));
#215997=CARTESIAN_POINT('Origin',(20.56795313141,7.80764394578302,12.));
#215998=CARTESIAN_POINT('',(20.7347298079577,7.33627833380046,0.));
#215999=CARTESIAN_POINT('Origin',(7.32141292029404E-13,2.70312158620511E-13,
0.));
#216000=CARTESIAN_POINT('Origin',(7.32141292029404E-13,2.70312158620511E-13,
12.));
#216001=CARTESIAN_POINT('Origin',(7.32141292029404E-13,2.70312158620511E-13,
0.));
#216002=CARTESIAN_POINT('Origin',(21.1389261070099,-3.92374859571502,0.));
#216003=CARTESIAN_POINT('',(22.1738711152697,-4.11585220600463,12.));
#216004=CARTESIAN_POINT('',(10.5694630535049,-1.96187429785751,12.));
#216005=CARTESIAN_POINT('',(22.1738711152697,-4.11585220600463,0.));
#216006=CARTESIAN_POINT('',(22.1738711152697,-4.11585220600463,0.));
#216007=CARTESIAN_POINT('',(10.5694630535049,-1.96187429785751,0.));
#216008=CARTESIAN_POINT('Ctrl Pts',(25.991588367311,-0.661312440730916,
0.));
#216009=CARTESIAN_POINT('Ctrl Pts',(25.991588367311,-0.661312440730916,
12.));
#216010=CARTESIAN_POINT('Ctrl Pts',(25.9865613464773,-0.66402831318764,
0.));
#216011=CARTESIAN_POINT('Ctrl Pts',(25.9865613464773,-0.66402831318764,
12.));
#216012=CARTESIAN_POINT('Ctrl Pts',(25.9765104298071,-0.669451306780839,
0.));
#216013=CARTESIAN_POINT('Ctrl Pts',(25.9765104298071,-0.669451306780839,
12.));
#216014=CARTESIAN_POINT('Ctrl Pts',(25.9614434297919,-0.67755954320974,
0.));
#216015=CARTESIAN_POINT('Ctrl Pts',(25.9614434297919,-0.67755954320974,
12.));
#216016=CARTESIAN_POINT('Ctrl Pts',(25.9413728471909,-0.688318015057744,
0.));
#216017=CARTESIAN_POINT('Ctrl Pts',(25.9413728471909,-0.688318015057744,
12.));
#216018=CARTESIAN_POINT('Ctrl Pts',(25.9163158909426,-0.701678575228769,
0.));
#216019=CARTESIAN_POINT('Ctrl Pts',(25.9163158909426,-0.701678575228769,
12.));
#216020=CARTESIAN_POINT('Ctrl Pts',(25.8912902614969,-0.714951588527653,
0.));
#216021=CARTESIAN_POINT('Ctrl Pts',(25.8912902614969,-0.714951588527653,
12.));
#216022=CARTESIAN_POINT('Ctrl Pts',(25.8662960624185,-0.728137036482349,
0.));
#216023=CARTESIAN_POINT('Ctrl Pts',(25.8662960624185,-0.728137036482349,
12.));
#216024=CARTESIAN_POINT('Ctrl Pts',(25.8413334619054,-0.74123490266382,
0.));
#216025=CARTESIAN_POINT('Ctrl Pts',(25.8413334619054,-0.74123490266382,
12.));
#216026=CARTESIAN_POINT('Ctrl Pts',(25.8164027059984,-0.754245175609537,
0.));
#216027=CARTESIAN_POINT('Ctrl Pts',(25.8164027059984,-0.754245175609537,
12.));
#216028=CARTESIAN_POINT('Ctrl Pts',(25.7915041383376,-0.767167852651183,
0.));
#216029=CARTESIAN_POINT('Ctrl Pts',(25.7915041383376,-0.767167852651183,
12.));
#216030=CARTESIAN_POINT('Ctrl Pts',(25.7666381946955,-0.780002940291977,
0.));
#216031=CARTESIAN_POINT('Ctrl Pts',(25.7666381946955,-0.780002940291977,
12.));
#216032=CARTESIAN_POINT('Ctrl Pts',(25.7418053757746,-0.79275045161614,
0.));
#216033=CARTESIAN_POINT('Ctrl Pts',(25.7418053757746,-0.79275045161614,
12.));
#216034=CARTESIAN_POINT('Ctrl Pts',(25.7170062262525,-0.805410404554366,
0.));
#216035=CARTESIAN_POINT('Ctrl Pts',(25.7170062262525,-0.805410404554366,
12.));
#216036=CARTESIAN_POINT('Ctrl Pts',(25.6922413110194,-0.817982819787478,
0.));
#216037=CARTESIAN_POINT('Ctrl Pts',(25.6922413110194,-0.817982819787478,
12.));
#216038=CARTESIAN_POINT('Ctrl Pts',(25.6675111931952,-0.830467718864221,
0.));
#216039=CARTESIAN_POINT('Ctrl Pts',(25.6675111931952,-0.830467718864221,
12.));
#216040=CARTESIAN_POINT('Ctrl Pts',(25.6428164100055,-0.842865122120773,
0.));
#216041=CARTESIAN_POINT('Ctrl Pts',(25.6428164100055,-0.842865122120773,
12.));
#216042=CARTESIAN_POINT('Ctrl Pts',(25.6181574536049,-0.855175047036563,
0.));
#216043=CARTESIAN_POINT('Ctrl Pts',(25.6181574536049,-0.855175047036563,
12.));
#216044=CARTESIAN_POINT('Ctrl Pts',(25.5935347843585,-0.867397509338443,
0.));
#216045=CARTESIAN_POINT('Ctrl Pts',(25.5935347843585,-0.867397509338443,
12.));
#216046=CARTESIAN_POINT('Ctrl Pts',(25.5689488408156,-0.879532523834308,
0.));
#216047=CARTESIAN_POINT('Ctrl Pts',(25.5689488408156,-0.879532523834308,
12.));
#216048=CARTESIAN_POINT('Ctrl Pts',(25.5444000508211,-0.891580105349052,
0.));
#216049=CARTESIAN_POINT('Ctrl Pts',(25.5444000508211,-0.891580105349052,
12.));
#216050=CARTESIAN_POINT('Ctrl Pts',(25.5198888424194,-0.903540269651121,
0.));
#216051=CARTESIAN_POINT('Ctrl Pts',(25.5198888424194,-0.903540269651121,
12.));
#216052=CARTESIAN_POINT('Ctrl Pts',(25.4954156541795,-0.915413034335626,
0.));
#216053=CARTESIAN_POINT('Ctrl Pts',(25.4954156541795,-0.915413034335626,
12.));
#216054=CARTESIAN_POINT('Ctrl Pts',(25.4709809475009,-0.927198419886108,
0.));
#216055=CARTESIAN_POINT('Ctrl Pts',(25.4709809475009,-0.927198419886108,
12.));
#216056=CARTESIAN_POINT('Ctrl Pts',(25.4465852044849,-0.938896449496205,
0.));
#216057=CARTESIAN_POINT('Ctrl Pts',(25.4465852044849,-0.938896449496205,
12.));
#216058=CARTESIAN_POINT('Ctrl Pts',(25.4222289223167,-0.950507148597483,
0.));
#216059=CARTESIAN_POINT('Ctrl Pts',(25.4222289223167,-0.950507148597483,
12.));
#216060=CARTESIAN_POINT('Ctrl Pts',(25.3979126089163,-0.962030544503156,
0.));
#216061=CARTESIAN_POINT('Ctrl Pts',(25.3979126089163,-0.962030544503156,
12.));
#216062=CARTESIAN_POINT('Ctrl Pts',(25.3736367778845,-0.973466666000178,
0.));
#216063=CARTESIAN_POINT('Ctrl Pts',(25.3736367778845,-0.973466666000178,
12.));
#216064=CARTESIAN_POINT('Ctrl Pts',(25.3494019441441,-0.984815543003986,
0.));
#216065=CARTESIAN_POINT('Ctrl Pts',(25.3494019441441,-0.984815543003986,
12.));
#216066=CARTESIAN_POINT('Ctrl Pts',(25.3252086182968,-0.996077206120637,
0.));
#216067=CARTESIAN_POINT('Ctrl Pts',(25.3252086182968,-0.996077206120637,
12.));
#216068=CARTESIAN_POINT('Ctrl Pts',(25.3010573055547,-1.00725168656897,
0.));
#216069=CARTESIAN_POINT('Ctrl Pts',(25.3010573055547,-1.00725168656897,
12.));
#216070=CARTESIAN_POINT('Ctrl Pts',(25.276948508726,-1.01833901642238,0.));
#216071=CARTESIAN_POINT('Ctrl Pts',(25.276948508726,-1.01833901642238,12.));
#216072=CARTESIAN_POINT('Ctrl Pts',(25.2528827300422,-1.02933922876807,
0.));
#216073=CARTESIAN_POINT('Ctrl Pts',(25.2528827300422,-1.02933922876807,
12.));
#216074=CARTESIAN_POINT('Ctrl Pts',(25.2288604735086,-1.04025235791508,
0.));
#216075=CARTESIAN_POINT('Ctrl Pts',(25.2288604735086,-1.04025235791508,
12.));
#216076=CARTESIAN_POINT('Ctrl Pts',(25.2048822469028,-1.05107843957933,
0.));
#216077=CARTESIAN_POINT('Ctrl Pts',(25.2048822469028,-1.05107843957933,
12.));
#216078=CARTESIAN_POINT('Ctrl Pts',(25.1809485642192,-1.06181751111769,
0.));
#216079=CARTESIAN_POINT('Ctrl Pts',(25.1809485642192,-1.06181751111769,
12.));
#216080=CARTESIAN_POINT('Ctrl Pts',(25.157059946931,-1.07246961165477,0.));
#216081=CARTESIAN_POINT('Ctrl Pts',(25.157059946931,-1.07246961165477,12.));
#216082=CARTESIAN_POINT('Ctrl Pts',(25.1332169227413,-1.08303478197189,
0.));
#216083=CARTESIAN_POINT('Ctrl Pts',(25.1332169227413,-1.08303478197189,
12.));
#216084=CARTESIAN_POINT('Ctrl Pts',(25.1094200248446,-1.09351306445309,
0.));
#216085=CARTESIAN_POINT('Ctrl Pts',(25.1094200248446,-1.09351306445309,
12.));
#216086=CARTESIAN_POINT('Ctrl Pts',(25.0856697909679,-1.10390450301747,
0.));
#216087=CARTESIAN_POINT('Ctrl Pts',(25.0856697909679,-1.10390450301747,
12.));
#216088=CARTESIAN_POINT('Ctrl Pts',(25.0619667625336,-1.11420914306891,
0.));
#216089=CARTESIAN_POINT('Ctrl Pts',(25.0619667625336,-1.11420914306891,
12.));
#216090=CARTESIAN_POINT('Ctrl Pts',(25.0383114836899,-1.12442703144453,
0.));
#216091=CARTESIAN_POINT('Ctrl Pts',(25.0383114836899,-1.12442703144453,
12.));
#216092=CARTESIAN_POINT('Ctrl Pts',(25.0147045006195,-1.13455821638531,
0.));
#216093=CARTESIAN_POINT('Ctrl Pts',(25.0147045006195,-1.13455821638531,
12.));
#216094=CARTESIAN_POINT('Ctrl Pts',(24.9911463621433,-1.14460274758202,
0.));
#216095=CARTESIAN_POINT('Ctrl Pts',(24.9911463621433,-1.14460274758202,
12.));
#216096=CARTESIAN_POINT('Ctrl Pts',(24.9676376201502,-1.15456067621891,
0.));
#216097=CARTESIAN_POINT('Ctrl Pts',(24.9676376201502,-1.15456067621891,
12.));
#216098=CARTESIAN_POINT('Ctrl Pts',(24.9441788300932,-1.16443205502851,
0.));
#216099=CARTESIAN_POINT('Ctrl Pts',(24.9441788300932,-1.16443205502851,
12.));
#216100=CARTESIAN_POINT('Ctrl Pts',(24.9207705514448,-1.17421693835042,
0.));
#216101=CARTESIAN_POINT('Ctrl Pts',(24.9207705514448,-1.17421693835042,
12.));
#216102=CARTESIAN_POINT('Ctrl Pts',(24.8974133481829,-1.18391538220104,
0.));
#216103=CARTESIAN_POINT('Ctrl Pts',(24.8974133481829,-1.18391538220104,
12.));
#216104=CARTESIAN_POINT('Ctrl Pts',(24.8741077892075,-1.19352744434066,
0.));
#216105=CARTESIAN_POINT('Ctrl Pts',(24.8741077892075,-1.19352744434066,
12.));
#216106=CARTESIAN_POINT('Ctrl Pts',(24.8508544481974,-1.20305318426021,
0.));
#216107=CARTESIAN_POINT('Ctrl Pts',(24.8508544481974,-1.20305318426021,
12.));
#216108=CARTESIAN_POINT('Ctrl Pts',(24.8276539035092,-1.21249266318209,
0.));
#216109=CARTESIAN_POINT('Ctrl Pts',(24.8276539035092,-1.21249266318209,
12.));
#216110=CARTESIAN_POINT('Ctrl Pts',(24.8045067380536,-1.22184594406529,
0.));
#216111=CARTESIAN_POINT('Ctrl Pts',(24.8045067380536,-1.22184594406529,
12.));
#216112=CARTESIAN_POINT('Ctrl Pts',(24.7814135391799,-1.23111309161845,
0.));
#216113=CARTESIAN_POINT('Ctrl Pts',(24.7814135391799,-1.23111309161845,
12.));
#216114=CARTESIAN_POINT('Ctrl Pts',(24.7583748985438,-1.2402941723199,0.));
#216115=CARTESIAN_POINT('Ctrl Pts',(24.7583748985438,-1.2402941723199,12.));
#216116=CARTESIAN_POINT('Ctrl Pts',(24.7353914120011,-1.24938925444327,
0.));
#216117=CARTESIAN_POINT('Ctrl Pts',(24.7353914120011,-1.24938925444327,
12.));
#216118=CARTESIAN_POINT('Ctrl Pts',(24.7124636797894,-1.25839840807419,
0.));
#216119=CARTESIAN_POINT('Ctrl Pts',(24.7124636797894,-1.25839840807419,
12.));
#216120=CARTESIAN_POINT('Ctrl Pts',(24.6895923066836,-1.26732170513501,
0.));
#216121=CARTESIAN_POINT('Ctrl Pts',(24.6895923066836,-1.26732170513501,
12.));
#216122=CARTESIAN_POINT('Ctrl Pts',(24.6667779021559,-1.27615921941643,
0.));
#216123=CARTESIAN_POINT('Ctrl Pts',(24.6667779021559,-1.27615921941643,
12.));
#216124=CARTESIAN_POINT('Ctrl Pts',(24.6440210805278,-1.28491102661515,
0.));
#216125=CARTESIAN_POINT('Ctrl Pts',(24.6440210805278,-1.28491102661515,
12.));
#216126=CARTESIAN_POINT('Ctrl Pts',(24.6213224611229,-1.29357720438108,
0.));
#216127=CARTESIAN_POINT('Ctrl Pts',(24.6213224611229,-1.29357720438108,
12.));
#216128=CARTESIAN_POINT('Ctrl Pts',(24.5986826684027,-1.30215783236363,
0.));
#216129=CARTESIAN_POINT('Ctrl Pts',(24.5986826684027,-1.30215783236363,
12.));
#216130=CARTESIAN_POINT('Ctrl Pts',(24.5761023320183,-1.31065299222023,
0.));
#216131=CARTESIAN_POINT('Ctrl Pts',(24.5761023320183,-1.31065299222023,
12.));
#216132=CARTESIAN_POINT('Ctrl Pts',(24.5535820868674,-1.31906276763669,
0.));
#216133=CARTESIAN_POINT('Ctrl Pts',(24.5535820868674,-1.31906276763669,
12.));
#216134=CARTESIAN_POINT('Ctrl Pts',(24.5311225731435,-1.32738724435327,
0.));
#216135=CARTESIAN_POINT('Ctrl Pts',(24.5311225731435,-1.32738724435327,
12.));
#216136=CARTESIAN_POINT('Ctrl Pts',(24.5087244363856,-1.33562651019687,
0.));
#216137=CARTESIAN_POINT('Ctrl Pts',(24.5087244363856,-1.33562651019687,
12.));
#216138=CARTESIAN_POINT('Ctrl Pts',(24.4863883275134,-1.34378065512339,
0.));
#216139=CARTESIAN_POINT('Ctrl Pts',(24.4863883275134,-1.34378065512339,
12.));
#216140=CARTESIAN_POINT('Ctrl Pts',(24.4641149028892,-1.35184977125649,
0.));
#216141=CARTESIAN_POINT('Ctrl Pts',(24.4641149028892,-1.35184977125649,
12.));
#216142=CARTESIAN_POINT('Ctrl Pts',(24.4419048244523,-1.35983395290629,
0.));
#216143=CARTESIAN_POINT('Ctrl Pts',(24.4419048244523,-1.35983395290629,
12.));
#216144=CARTESIAN_POINT('Ctrl Pts',(24.4197587598337,-1.36773329659958,
0.));
#216145=CARTESIAN_POINT('Ctrl Pts',(24.4197587598337,-1.36773329659958,
12.));
#216146=CARTESIAN_POINT('Ctrl Pts',(24.3976773824732,-1.37554790111611,
0.));
#216147=CARTESIAN_POINT('Ctrl Pts',(24.3976773824732,-1.37554790111611,
12.));
#216148=CARTESIAN_POINT('Ctrl Pts',(24.3756613717299,-1.38327786753,0.));
#216149=CARTESIAN_POINT('Ctrl Pts',(24.3756613717299,-1.38327786753,12.));
#216150=CARTESIAN_POINT('Ctrl Pts',(24.3537114129875,-1.3909232992639,0.));
#216151=CARTESIAN_POINT('Ctrl Pts',(24.3537114129875,-1.3909232992639,12.));
#216152=CARTESIAN_POINT('Ctrl Pts',(24.3318281977643,-1.39848430212808,
0.));
#216153=CARTESIAN_POINT('Ctrl Pts',(24.3318281977643,-1.39848430212808,
12.));
#216154=CARTESIAN_POINT('Ctrl Pts',(24.3100124238311,-1.40596098434339,
0.));
#216155=CARTESIAN_POINT('Ctrl Pts',(24.3100124238311,-1.40596098434339,
12.));
#216156=CARTESIAN_POINT('Ctrl Pts',(24.288264795321,-1.41335345657684,0.));
#216157=CARTESIAN_POINT('Ctrl Pts',(24.288264795321,-1.41335345657684,12.));
#216158=CARTESIAN_POINT('Ctrl Pts',(24.2665860228356,-1.42066183198254,
0.));
#216159=CARTESIAN_POINT('Ctrl Pts',(24.2665860228356,-1.42066183198254,
12.));
#216160=CARTESIAN_POINT('Ctrl Pts',(24.2449768235488,-1.42788622624855,
0.));
#216161=CARTESIAN_POINT('Ctrl Pts',(24.2449768235488,-1.42788622624855,
12.));
#216162=CARTESIAN_POINT('Ctrl Pts',(24.2234379212984,-1.4350267576551,0.));
#216163=CARTESIAN_POINT('Ctrl Pts',(24.2234379212984,-1.4350267576551,12.));
#216164=CARTESIAN_POINT('Ctrl Pts',(24.201970046722,-1.44208354711083,0.));
#216165=CARTESIAN_POINT('Ctrl Pts',(24.201970046722,-1.44208354711083,12.));
#216166=CARTESIAN_POINT('Ctrl Pts',(24.1805739374038,-1.44905671818729,
0.));
#216167=CARTESIAN_POINT('Ctrl Pts',(24.1805739374038,-1.44905671818729,
12.));
#216168=CARTESIAN_POINT('Ctrl Pts',(24.1592503380107,-1.45594639716319,
0.));
#216169=CARTESIAN_POINT('Ctrl Pts',(24.1592503380107,-1.45594639716319,
12.));
#216170=CARTESIAN_POINT('Ctrl Pts',(24.1380000004272,-1.46275271307399,
0.));
#216171=CARTESIAN_POINT('Ctrl Pts',(24.1380000004272,-1.46275271307399,
12.));
#216172=CARTESIAN_POINT('Ctrl Pts',(24.1168236838824,-1.46947579776993,
0.));
#216173=CARTESIAN_POINT('Ctrl Pts',(24.1168236838824,-1.46947579776993,
12.));
#216174=CARTESIAN_POINT('Ctrl Pts',(24.0957221550778,-1.47611578597743,
0.));
#216175=CARTESIAN_POINT('Ctrl Pts',(24.0957221550778,-1.47611578597743,
12.));
#216176=CARTESIAN_POINT('Ctrl Pts',(24.0746961883528,-1.48267281533684,
0.));
#216177=CARTESIAN_POINT('Ctrl Pts',(24.0746961883528,-1.48267281533684,
12.));
#216178=CARTESIAN_POINT('Ctrl Pts',(24.0537465658429,-1.48914702644889,
0.));
#216179=CARTESIAN_POINT('Ctrl Pts',(24.0537465658429,-1.48914702644889,
12.));
#216180=CARTESIAN_POINT('Ctrl Pts',(24.0328740776331,-1.49553856292802,
0.));
#216181=CARTESIAN_POINT('Ctrl Pts',(24.0328740776331,-1.49553856292802,
12.));
#216182=CARTESIAN_POINT('Ctrl Pts',(24.0120795219086,-1.501847571461,0.));
#216183=CARTESIAN_POINT('Ctrl Pts',(24.0120795219086,-1.501847571461,12.));
#216184=CARTESIAN_POINT('Ctrl Pts',(23.9913637050927,-1.50807420187695,
0.));
#216185=CARTESIAN_POINT('Ctrl Pts',(23.9913637050927,-1.50807420187695,
12.));
#216186=CARTESIAN_POINT('Ctrl Pts',(23.970727442014,-1.51421860720616,0.));
#216187=CARTESIAN_POINT('Ctrl Pts',(23.970727442014,-1.51421860720616,12.));
#216188=CARTESIAN_POINT('Ctrl Pts',(23.9501715561033,-1.52028094372793,
0.));
#216189=CARTESIAN_POINT('Ctrl Pts',(23.9501715561033,-1.52028094372793,
12.));
#216190=CARTESIAN_POINT('Ctrl Pts',(23.9296968795757,-1.52626137103033,
0.));
#216191=CARTESIAN_POINT('Ctrl Pts',(23.9296968795757,-1.52626137103033,
12.));
#216192=CARTESIAN_POINT('Ctrl Pts',(23.9093042536119,-1.53216005207464,
0.));
#216193=CARTESIAN_POINT('Ctrl Pts',(23.9093042536119,-1.53216005207464,
12.));
#216194=CARTESIAN_POINT('Ctrl Pts',(23.8889945285318,-1.53797715326759,
0.));
#216195=CARTESIAN_POINT('Ctrl Pts',(23.8889945285318,-1.53797715326759,
12.));
#216196=CARTESIAN_POINT('Ctrl Pts',(23.8687685639642,-1.54371284453992,
0.));
#216197=CARTESIAN_POINT('Ctrl Pts',(23.8687685639642,-1.54371284453992,
12.));
#216198=CARTESIAN_POINT('Ctrl Pts',(23.8486272290705,-1.54936729940542,
0.));
#216199=CARTESIAN_POINT('Ctrl Pts',(23.8486272290705,-1.54936729940542,
12.));
#216200=CARTESIAN_POINT('Ctrl Pts',(23.8285714027636,-1.55494069502636,
0.));
#216201=CARTESIAN_POINT('Ctrl Pts',(23.8285714027636,-1.55494069502636,
12.));
#216202=CARTESIAN_POINT('Ctrl Pts',(23.8086019739194,-1.56043321228635,
0.));
#216203=CARTESIAN_POINT('Ctrl Pts',(23.8086019739194,-1.56043321228635,
12.));
#216204=CARTESIAN_POINT('Ctrl Pts',(23.7887198415878,-1.56584503586844,
0.));
#216205=CARTESIAN_POINT('Ctrl Pts',(23.7887198415878,-1.56584503586844,
12.));
#216206=CARTESIAN_POINT('Ctrl Pts',(23.7689259151862,-1.57117635434409,
0.));
#216207=CARTESIAN_POINT('Ctrl Pts',(23.7689259151862,-1.57117635434409,
12.));
#216208=CARTESIAN_POINT('Ctrl Pts',(23.749221114736,-1.57642736025247,0.));
#216209=CARTESIAN_POINT('Ctrl Pts',(23.749221114736,-1.57642736025247,12.));
#216210=CARTESIAN_POINT('Ctrl Pts',(23.72960637113,-1.58159825017359,0.));
#216211=CARTESIAN_POINT('Ctrl Pts',(23.72960637113,-1.58159825017359,12.));
#216212=CARTESIAN_POINT('Ctrl Pts',(23.710082626383,-1.58668922481222,0.));
#216213=CARTESIAN_POINT('Ctrl Pts',(23.710082626383,-1.58668922481222,12.));
#216214=CARTESIAN_POINT('Ctrl Pts',(23.6906508338833,-1.59170048908634,
0.));
#216215=CARTESIAN_POINT('Ctrl Pts',(23.6906508338833,-1.59170048908634,
12.));
#216216=CARTESIAN_POINT('Ctrl Pts',(23.671311958631,-1.59663225222464,0.));
#216217=CARTESIAN_POINT('Ctrl Pts',(23.671311958631,-1.59663225222464,12.));
#216218=CARTESIAN_POINT('Ctrl Pts',(23.6520669774876,-1.60148472786596,
0.));
#216219=CARTESIAN_POINT('Ctrl Pts',(23.6520669774876,-1.60148472786596,
12.));
#216220=CARTESIAN_POINT('Ctrl Pts',(23.6329168794929,-1.60625813414674,
0.));
#216221=CARTESIAN_POINT('Ctrl Pts',(23.6329168794929,-1.60625813414674,
12.));
#216222=CARTESIAN_POINT('Ctrl Pts',(23.6138626661653,-1.61095269379779,
0.));
#216223=CARTESIAN_POINT('Ctrl Pts',(23.6138626661653,-1.61095269379779,
12.));
#216224=CARTESIAN_POINT('Ctrl Pts',(23.5949053517997,-1.61556863424699,
0.));
#216225=CARTESIAN_POINT('Ctrl Pts',(23.5949053517997,-1.61556863424699,
12.));
#216226=CARTESIAN_POINT('Ctrl Pts',(23.57604596376,-1.62010618772867,0.));
#216227=CARTESIAN_POINT('Ctrl Pts',(23.57604596376,-1.62010618772867,12.));
#216228=CARTESIAN_POINT('Ctrl Pts',(23.5572855427601,-1.62456559140066,
0.));
#216229=CARTESIAN_POINT('Ctrl Pts',(23.5572855427601,-1.62456559140066,
12.));
#216230=CARTESIAN_POINT('Ctrl Pts',(23.538625143226,-1.62894708745224,0.));
#216231=CARTESIAN_POINT('Ctrl Pts',(23.538625143226,-1.62894708745224,12.));
#216232=CARTESIAN_POINT('Ctrl Pts',(23.5200658336612,-1.63325092321727,
0.));
#216233=CARTESIAN_POINT('Ctrl Pts',(23.5200658336612,-1.63325092321727,
12.));
#216234=CARTESIAN_POINT('Ctrl Pts',(23.5016086970003,-1.63747735129475,
0.));
#216235=CARTESIAN_POINT('Ctrl Pts',(23.5016086970003,-1.63747735129475,
12.));
#216236=CARTESIAN_POINT('Ctrl Pts',(23.4832548309645,-1.64162662967529,
0.));
#216237=CARTESIAN_POINT('Ctrl Pts',(23.4832548309645,-1.64162662967529,
12.));
#216238=CARTESIAN_POINT('Ctrl Pts',(23.4650053483932,-1.64569902187612,
0.));
#216239=CARTESIAN_POINT('Ctrl Pts',(23.4650053483932,-1.64569902187612,
12.));
#216240=CARTESIAN_POINT('Ctrl Pts',(23.4468613776574,-1.64969479707341,
0.));
#216241=CARTESIAN_POINT('Ctrl Pts',(23.4468613776574,-1.64969479707341,
12.));
#216242=CARTESIAN_POINT('Ctrl Pts',(23.4288240631043,-1.6536142302373,0.));
#216243=CARTESIAN_POINT('Ctrl Pts',(23.4288240631043,-1.6536142302373,12.));
#216244=CARTESIAN_POINT('Ctrl Pts',(23.4108945654805,-1.65745760227506,
0.));
#216245=CARTESIAN_POINT('Ctrl Pts',(23.4108945654805,-1.65745760227506,
12.));
#216246=CARTESIAN_POINT('Ctrl Pts',(23.3930740623619,-1.66122520018012,
0.));
#216247=CARTESIAN_POINT('Ctrl Pts',(23.3930740623619,-1.66122520018012,
12.));
#216248=CARTESIAN_POINT('Ctrl Pts',(23.3753637485545,-1.66491731718878,
0.));
#216249=CARTESIAN_POINT('Ctrl Pts',(23.3753637485545,-1.66491731718878,
12.));
#216250=CARTESIAN_POINT('Ctrl Pts',(23.3577648365744,-1.66853425293997,
0.));
#216251=CARTESIAN_POINT('Ctrl Pts',(23.3577648365744,-1.66853425293997,
12.));
#216252=CARTESIAN_POINT('Ctrl Pts',(23.3402785571865,-1.67207631363923,
0.));
#216253=CARTESIAN_POINT('Ctrl Pts',(23.3402785571865,-1.67207631363923,
12.));
#216254=CARTESIAN_POINT('Ctrl Pts',(23.3229061599144,-1.67554381222995,
0.));
#216255=CARTESIAN_POINT('Ctrl Pts',(23.3229061599144,-1.67554381222995,
12.));
#216256=CARTESIAN_POINT('Ctrl Pts',(23.3056489135611,-1.67893706857118,
0.));
#216257=CARTESIAN_POINT('Ctrl Pts',(23.3056489135611,-1.67893706857118,
12.));
#216258=CARTESIAN_POINT('Ctrl Pts',(23.2885081066951,-1.68225640962169,
0.));
#216259=CARTESIAN_POINT('Ctrl Pts',(23.2885081066951,-1.68225640962169,
12.));
#216260=CARTESIAN_POINT('Ctrl Pts',(23.2714850482246,-1.68550216963259,
0.));
#216261=CARTESIAN_POINT('Ctrl Pts',(23.2714850482246,-1.68550216963259,
12.));
#216262=CARTESIAN_POINT('Ctrl Pts',(23.2545810680537,-1.68867469034897,
0.));
#216263=CARTESIAN_POINT('Ctrl Pts',(23.2545810680537,-1.68867469034897,
12.));
#216264=CARTESIAN_POINT('Ctrl Pts',(23.2377975177013,-1.69177432121712,
0.));
#216265=CARTESIAN_POINT('Ctrl Pts',(23.2377975177013,-1.69177432121712,
12.));
#216266=CARTESIAN_POINT('Ctrl Pts',(23.2211357709374,-1.69480141959954,
0.));
#216267=CARTESIAN_POINT('Ctrl Pts',(23.2211357709374,-1.69480141959954,
12.));
#216268=CARTESIAN_POINT('Ctrl Pts',(23.2045972243767,-1.69775635099444,
0.));
#216269=CARTESIAN_POINT('Ctrl Pts',(23.2045972243767,-1.69775635099444,
12.));
#216270=CARTESIAN_POINT('Ctrl Pts',(23.1881832981851,-1.70063948927011,
0.));
#216271=CARTESIAN_POINT('Ctrl Pts',(23.1881832981851,-1.70063948927011,
12.));
#216272=CARTESIAN_POINT('Ctrl Pts',(23.1718954368751,-1.70345121691278,
0.));
#216273=CARTESIAN_POINT('Ctrl Pts',(23.1718954368751,-1.70345121691278,
12.));
#216274=CARTESIAN_POINT('Ctrl Pts',(23.1557351100614,-1.70619192527853,
0.));
#216275=CARTESIAN_POINT('Ctrl Pts',(23.1557351100614,-1.70619192527853,
12.));
#216276=CARTESIAN_POINT('Ctrl Pts',(23.1397038132356,-1.70886201485453,
0.));
#216277=CARTESIAN_POINT('Ctrl Pts',(23.1397038132356,-1.70886201485453,
12.));
#216278=CARTESIAN_POINT('Ctrl Pts',(23.1238030684925,-1.71146189552175,
0.));
#216279=CARTESIAN_POINT('Ctrl Pts',(23.1238030684925,-1.71146189552175,
12.));
#216280=CARTESIAN_POINT('Ctrl Pts',(23.1080344254286,-1.71399198684705,
0.));
#216281=CARTESIAN_POINT('Ctrl Pts',(23.1080344254286,-1.71399198684705,
12.));
#216282=CARTESIAN_POINT('Ctrl Pts',(23.0923994621213,-1.71645271839298,
0.));
#216283=CARTESIAN_POINT('Ctrl Pts',(23.0923994621213,-1.71645271839298,
12.));
#216284=CARTESIAN_POINT('Ctrl Pts',(23.0768997860708,-1.71884453003028,
0.));
#216285=CARTESIAN_POINT('Ctrl Pts',(23.0768997860708,-1.71884453003028,
12.));
#216286=CARTESIAN_POINT('Ctrl Pts',(23.0615370351562,-1.72116787225993,
0.));
#216287=CARTESIAN_POINT('Ctrl Pts',(23.0615370351562,-1.72116787225993,
12.));
#216288=CARTESIAN_POINT('Ctrl Pts',(23.0463128785531,-1.72342320653748,
0.));
#216289=CARTESIAN_POINT('Ctrl Pts',(23.0463128785531,-1.72342320653748,
12.));
#216290=CARTESIAN_POINT('Ctrl Pts',(23.0312290178883,-1.72561100564047,
0.));
#216291=CARTESIAN_POINT('Ctrl Pts',(23.0312290178883,-1.72561100564047,
12.));
#216292=CARTESIAN_POINT('Ctrl Pts',(23.0162871884168,-1.7277317540471,0.));
#216293=CARTESIAN_POINT('Ctrl Pts',(23.0162871884168,-1.7277317540471,12.));
#216294=CARTESIAN_POINT('Ctrl Pts',(23.001489160189,-1.72978594832137,0.));
#216295=CARTESIAN_POINT('Ctrl Pts',(23.001489160189,-1.72978594832137,12.));
#216296=CARTESIAN_POINT('Ctrl Pts',(22.9868367391978,-1.73177409750192,
0.));
#216297=CARTESIAN_POINT('Ctrl Pts',(22.9868367391978,-1.73177409750192,
12.));
#216298=CARTESIAN_POINT('Ctrl Pts',(22.9723317685688,-1.73369672350816,
0.));
#216299=CARTESIAN_POINT('Ctrl Pts',(22.9723317685688,-1.73369672350816,
12.));
#216300=CARTESIAN_POINT('Ctrl Pts',(22.9579761301063,-1.73555436162771,
0.));
#216301=CARTESIAN_POINT('Ctrl Pts',(22.9579761301063,-1.73555436162771,
12.));
#216302=CARTESIAN_POINT('Ctrl Pts',(22.9437717457826,-1.7373475610004,0.));
#216303=CARTESIAN_POINT('Ctrl Pts',(22.9437717457826,-1.7373475610004,12.));
#216304=CARTESIAN_POINT('Ctrl Pts',(22.9297205792586,-1.73907688511667,
0.));
#216305=CARTESIAN_POINT('Ctrl Pts',(22.9297205792586,-1.73907688511667,
12.));
#216306=CARTESIAN_POINT('Ctrl Pts',(22.9158246373363,-1.7407429123106,0.));
#216307=CARTESIAN_POINT('Ctrl Pts',(22.9158246373363,-1.7407429123106,12.));
#216308=CARTESIAN_POINT('Ctrl Pts',(22.9020859716141,-1.74234623630081,
0.));
#216309=CARTESIAN_POINT('Ctrl Pts',(22.9020859716141,-1.74234623630081,
12.));
#216310=CARTESIAN_POINT('Ctrl Pts',(22.888506680335,-1.74388746677704,0.));
#216311=CARTESIAN_POINT('Ctrl Pts',(22.888506680335,-1.74388746677704,12.));
#216312=CARTESIAN_POINT('Ctrl Pts',(22.8750889101696,-1.74536722998202,
0.));
#216313=CARTESIAN_POINT('Ctrl Pts',(22.8750889101696,-1.74536722998202,
12.));
#216314=CARTESIAN_POINT('Ctrl Pts',(22.8618348580235,-1.74678616930666,
0.));
#216315=CARTESIAN_POINT('Ctrl Pts',(22.8618348580235,-1.74678616930666,
12.));
#216316=CARTESIAN_POINT('Ctrl Pts',(22.8487467728076,-1.74814494588494,
0.));
#216317=CARTESIAN_POINT('Ctrl Pts',(22.8487467728076,-1.74814494588494,
12.));
#216318=CARTESIAN_POINT('Ctrl Pts',(22.8358269579853,-1.74944423940117,
0.));
#216319=CARTESIAN_POINT('Ctrl Pts',(22.8358269579853,-1.74944423940117,
12.));
#216320=CARTESIAN_POINT('Ctrl Pts',(22.8230777741284,-1.75068474890884,
0.));
#216321=CARTESIAN_POINT('Ctrl Pts',(22.8230777741284,-1.75068474890884,
12.));
#216322=CARTESIAN_POINT('Ctrl Pts',(22.8105016414713,-1.75186719365593,
0.));
#216323=CARTESIAN_POINT('Ctrl Pts',(22.8105016414713,-1.75186719365593,
12.));
#216324=CARTESIAN_POINT('Ctrl Pts',(22.7981010424314,-1.75299231391468,
0.));
#216325=CARTESIAN_POINT('Ctrl Pts',(22.7981010424314,-1.75299231391468,
12.));
#216326=CARTESIAN_POINT('Ctrl Pts',(22.7858785242361,-1.75406087182937,
0.));
#216327=CARTESIAN_POINT('Ctrl Pts',(22.7858785242361,-1.75406087182937,
12.));
#216328=CARTESIAN_POINT('Ctrl Pts',(22.7738367016118,-1.75507365227133,
0.));
#216329=CARTESIAN_POINT('Ctrl Pts',(22.7738367016118,-1.75507365227133,
12.));
#216330=CARTESIAN_POINT('Ctrl Pts',(22.7619782595013,-1.75603146371642,
0.));
#216331=CARTESIAN_POINT('Ctrl Pts',(22.7619782595013,-1.75603146371642,
12.));
#216332=CARTESIAN_POINT('Ctrl Pts',(22.750305955645,-1.75693513908908,0.));
#216333=CARTESIAN_POINT('Ctrl Pts',(22.750305955645,-1.75693513908908,12.));
#216334=CARTESIAN_POINT('Ctrl Pts',(22.7388226235559,-1.75778553673245,
0.));
#216335=CARTESIAN_POINT('Ctrl Pts',(22.7388226235559,-1.75778553673245,
12.));
#216336=CARTESIAN_POINT('Ctrl Pts',(22.72753117773,-1.75858354204634,0.));
#216337=CARTESIAN_POINT('Ctrl Pts',(22.72753117773,-1.75858354204634,12.));
#216338=CARTESIAN_POINT('Ctrl Pts',(22.7164346186006,-1.75933006905926,
0.));
#216339=CARTESIAN_POINT('Ctrl Pts',(22.7164346186006,-1.75933006905926,
12.));
#216340=CARTESIAN_POINT('Ctrl Pts',(22.7055360375485,-1.76002606202402,
0.));
#216341=CARTESIAN_POINT('Ctrl Pts',(22.7055360375485,-1.76002606202402,
12.));
#216342=CARTESIAN_POINT('Ctrl Pts',(22.6948386219851,-1.76067249704888,
0.));
#216343=CARTESIAN_POINT('Ctrl Pts',(22.6948386219851,-1.76067249704888,
12.));
#216344=CARTESIAN_POINT('Ctrl Pts',(22.684345658525,-1.76127038310615,0.));
#216345=CARTESIAN_POINT('Ctrl Pts',(22.684345658525,-1.76127038310615,12.));
#216346=CARTESIAN_POINT('Ctrl Pts',(22.67406053567,-1.76182076289527,0.));
#216347=CARTESIAN_POINT('Ctrl Pts',(22.67406053567,-1.76182076289527,12.));
#216348=CARTESIAN_POINT('Ctrl Pts',(22.6639867471753,-1.7623247139257,0.));
#216349=CARTESIAN_POINT('Ctrl Pts',(22.6639867471753,-1.7623247139257,12.));
#216350=CARTESIAN_POINT('Ctrl Pts',(22.6541278938409,-1.76278334912562,
0.));
#216351=CARTESIAN_POINT('Ctrl Pts',(22.6541278938409,-1.76278334912562,
12.));
#216352=CARTESIAN_POINT('Ctrl Pts',(22.6444876940423,-1.76319782013917,
0.));
#216353=CARTESIAN_POINT('Ctrl Pts',(22.6444876940423,-1.76319782013917,
12.));
#216354=CARTESIAN_POINT('Ctrl Pts',(22.6350699979359,-1.76356932176274,
0.));
#216355=CARTESIAN_POINT('Ctrl Pts',(22.6350699979359,-1.76356932176274,
12.));
#216356=CARTESIAN_POINT('Ctrl Pts',(22.6258787994848,-1.76389909571404,
0.));
#216357=CARTESIAN_POINT('Ctrl Pts',(22.6258787994848,-1.76389909571404,
12.));
#216358=CARTESIAN_POINT('Ctrl Pts',(22.6169182517694,-1.76418843543741,
0.));
#216359=CARTESIAN_POINT('Ctrl Pts',(22.6169182517694,-1.76418843543741,
12.));
#216360=CARTESIAN_POINT('Ctrl Pts',(22.6081926681343,-1.76443868648017,
0.));
#216361=CARTESIAN_POINT('Ctrl Pts',(22.6081926681343,-1.76443868648017,
12.));
#216362=CARTESIAN_POINT('Ctrl Pts',(22.5997065145638,-1.76465124413558,
0.));
#216363=CARTESIAN_POINT('Ctrl Pts',(22.5997065145638,-1.76465124413558,
12.));
#216364=CARTESIAN_POINT('Ctrl Pts',(22.5914644078105,-1.76482755288412,
0.));
#216365=CARTESIAN_POINT('Ctrl Pts',(22.5914644078105,-1.76482755288412,
12.));
#216366=CARTESIAN_POINT('Ctrl Pts',(22.5834711038022,-1.76496910283089,
0.));
#216367=CARTESIAN_POINT('Ctrl Pts',(22.5834711038022,-1.76496910283089,
12.));
#216368=CARTESIAN_POINT('Ctrl Pts',(22.5757315316353,-1.76507744026747,
0.));
#216369=CARTESIAN_POINT('Ctrl Pts',(22.5757315316353,-1.76507744026747,
12.));
#216370=CARTESIAN_POINT('Ctrl Pts',(22.5682508499873,-1.76515418518832,
0.));
#216371=CARTESIAN_POINT('Ctrl Pts',(22.5682508499873,-1.76515418518832,
12.));
#216372=CARTESIAN_POINT('Ctrl Pts',(22.5610344912501,-1.76520104500451,
0.));
#216373=CARTESIAN_POINT('Ctrl Pts',(22.5610344912501,-1.76520104500451,
12.));
#216374=CARTESIAN_POINT('Ctrl Pts',(22.5540882235837,-1.76521983384064,
0.));
#216375=CARTESIAN_POINT('Ctrl Pts',(22.5540882235837,-1.76521983384064,
12.));
#216376=CARTESIAN_POINT('Ctrl Pts',(22.5474180954006,-1.76521245524048,
0.));
#216377=CARTESIAN_POINT('Ctrl Pts',(22.5474180954006,-1.76521245524048,
12.));
#216378=CARTESIAN_POINT('Ctrl Pts',(22.5410303590892,-1.76518087841494,
0.));
#216379=CARTESIAN_POINT('Ctrl Pts',(22.5410303590892,-1.76518087841494,
12.));
#216380=CARTESIAN_POINT('Ctrl Pts',(22.5349313983571,-1.76512711563255,
0.));
#216381=CARTESIAN_POINT('Ctrl Pts',(22.5349313983571,-1.76512711563255,
12.));
#216382=CARTESIAN_POINT('Ctrl Pts',(22.529127665298,-1.7650532026276,0.));
#216383=CARTESIAN_POINT('Ctrl Pts',(22.529127665298,-1.7650532026276,12.));
#216384=CARTESIAN_POINT('Ctrl Pts',(22.5236259635515,-1.76496128643376,
0.));
#216385=CARTESIAN_POINT('Ctrl Pts',(22.5236259635515,-1.76496128643376,
12.));
#216386=CARTESIAN_POINT('Ctrl Pts',(22.5184336670207,-1.76485369319896,
0.));
#216387=CARTESIAN_POINT('Ctrl Pts',(22.5184336670207,-1.76485369319896,
12.));
#216388=CARTESIAN_POINT('Ctrl Pts',(22.5135590569554,-1.7647330328115,0.));
#216389=CARTESIAN_POINT('Ctrl Pts',(22.5135590569554,-1.7647330328115,12.));
#216390=CARTESIAN_POINT('Ctrl Pts',(22.5090112700212,-1.76460218257314,
0.));
#216391=CARTESIAN_POINT('Ctrl Pts',(22.5090112700212,-1.76460218257314,
12.));
#216392=CARTESIAN_POINT('Ctrl Pts',(22.5047996391978,-1.76446408210366,
0.));
#216393=CARTESIAN_POINT('Ctrl Pts',(22.5047996391978,-1.76446408210366,
12.));
#216394=CARTESIAN_POINT('Ctrl Pts',(22.5009332677316,-1.76432160068739,
0.));
#216395=CARTESIAN_POINT('Ctrl Pts',(22.5009332677316,-1.76432160068739,
12.));
#216396=CARTESIAN_POINT('Ctrl Pts',(22.4974203063191,-1.76417731243484,
0.));
#216397=CARTESIAN_POINT('Ctrl Pts',(22.4974203063191,-1.76417731243484,
12.));
#216398=CARTESIAN_POINT('Ctrl Pts',(22.4942693792449,-1.76403393880317,
0.));
#216399=CARTESIAN_POINT('Ctrl Pts',(22.4942693792449,-1.76403393880317,
12.));
#216400=CARTESIAN_POINT('Ctrl Pts',(22.4914909094908,-1.76389475965715,
0.));
#216401=CARTESIAN_POINT('Ctrl Pts',(22.4914909094908,-1.76389475965715,
12.));
#216402=CARTESIAN_POINT('Ctrl Pts',(22.4890991659479,-1.76376424879469,
0.));
#216403=CARTESIAN_POINT('Ctrl Pts',(22.4890991659479,-1.76376424879469,
12.));
#216404=CARTESIAN_POINT('Ctrl Pts',(22.4871115206572,-1.76364784232927,
0.));
#216405=CARTESIAN_POINT('Ctrl Pts',(22.4871115206572,-1.76364784232927,
12.));
#216406=CARTESIAN_POINT('Ctrl Pts',(22.4855446605991,-1.7635507604555,0.));
#216407=CARTESIAN_POINT('Ctrl Pts',(22.4855446605991,-1.7635507604555,12.));
#216408=CARTESIAN_POINT('Ctrl Pts',(22.4844112933125,-1.76347698284863,
0.));
#216409=CARTESIAN_POINT('Ctrl Pts',(22.4844112933125,-1.76347698284863,
12.));
#216410=CARTESIAN_POINT('Ctrl Pts',(22.4838562517064,-1.7634381343466,0.));
#216411=CARTESIAN_POINT('Ctrl Pts',(22.4838562517064,-1.7634381343466,12.));
#216412=CARTESIAN_POINT('Ctrl Pts',(22.4836387052228,-1.76342064263638,
0.));
#216413=CARTESIAN_POINT('Ctrl Pts',(22.4836387052228,-1.76342064263638,
12.));
#216414=CARTESIAN_POINT('Ctrl Pts',(22.4835819929788,-1.76341415538792,
0.));
#216415=CARTESIAN_POINT('Ctrl Pts',(22.4835819929788,-1.76341415538792,
12.));
#216416=CARTESIAN_POINT('Ctrl Pts',(22.4835757167854,-1.76341220531181,
0.));
#216417=CARTESIAN_POINT('Ctrl Pts',(22.4835757167854,-1.76341220531181,
12.));
#216418=CARTESIAN_POINT('',(25.991588367311,-0.661312440730916,0.));
#216419=CARTESIAN_POINT('Ctrl Pts',(25.991588367311,-0.661312440730916,
0.));
#216420=CARTESIAN_POINT('Ctrl Pts',(25.9865613464773,-0.66402831318764,
0.));
#216421=CARTESIAN_POINT('Ctrl Pts',(25.9765104298071,-0.669451306780839,
0.));
#216422=CARTESIAN_POINT('Ctrl Pts',(25.9614434297919,-0.67755954320974,
0.));
#216423=CARTESIAN_POINT('Ctrl Pts',(25.9413728471909,-0.688318015057744,
0.));
#216424=CARTESIAN_POINT('Ctrl Pts',(25.9163158909426,-0.701678575228769,
0.));
#216425=CARTESIAN_POINT('Ctrl Pts',(25.8912902614969,-0.714951588527653,
0.));
#216426=CARTESIAN_POINT('Ctrl Pts',(25.8662960624185,-0.728137036482349,
0.));
#216427=CARTESIAN_POINT('Ctrl Pts',(25.8413334619054,-0.74123490266382,
0.));
#216428=CARTESIAN_POINT('Ctrl Pts',(25.8164027059984,-0.754245175609537,
0.));
#216429=CARTESIAN_POINT('Ctrl Pts',(25.7915041383376,-0.767167852651183,
0.));
#216430=CARTESIAN_POINT('Ctrl Pts',(25.7666381946955,-0.780002940291977,
0.));
#216431=CARTESIAN_POINT('Ctrl Pts',(25.7418053757746,-0.79275045161614,
0.));
#216432=CARTESIAN_POINT('Ctrl Pts',(25.7170062262525,-0.805410404554366,
0.));
#216433=CARTESIAN_POINT('Ctrl Pts',(25.6922413110194,-0.817982819787478,
0.));
#216434=CARTESIAN_POINT('Ctrl Pts',(25.6675111931952,-0.830467718864221,
0.));
#216435=CARTESIAN_POINT('Ctrl Pts',(25.6428164100055,-0.842865122120773,
0.));
#216436=CARTESIAN_POINT('Ctrl Pts',(25.6181574536049,-0.855175047036563,
0.));
#216437=CARTESIAN_POINT('Ctrl Pts',(25.5935347843585,-0.867397509338443,
0.));
#216438=CARTESIAN_POINT('Ctrl Pts',(25.5689488408156,-0.879532523834308,
0.));
#216439=CARTESIAN_POINT('Ctrl Pts',(25.5444000508211,-0.891580105349052,
0.));
#216440=CARTESIAN_POINT('Ctrl Pts',(25.5198888424194,-0.903540269651121,
0.));
#216441=CARTESIAN_POINT('Ctrl Pts',(25.4954156541795,-0.915413034335626,
0.));
#216442=CARTESIAN_POINT('Ctrl Pts',(25.4709809475009,-0.927198419886108,
0.));
#216443=CARTESIAN_POINT('Ctrl Pts',(25.4465852044849,-0.938896449496205,
0.));
#216444=CARTESIAN_POINT('Ctrl Pts',(25.4222289223167,-0.950507148597483,
0.));
#216445=CARTESIAN_POINT('Ctrl Pts',(25.3979126089163,-0.962030544503156,
0.));
#216446=CARTESIAN_POINT('Ctrl Pts',(25.3736367778845,-0.973466666000178,
0.));
#216447=CARTESIAN_POINT('Ctrl Pts',(25.3494019441441,-0.984815543003986,
0.));
#216448=CARTESIAN_POINT('Ctrl Pts',(25.3252086182968,-0.996077206120637,
0.));
#216449=CARTESIAN_POINT('Ctrl Pts',(25.3010573055547,-1.00725168656897,
0.));
#216450=CARTESIAN_POINT('Ctrl Pts',(25.276948508726,-1.01833901642238,0.));
#216451=CARTESIAN_POINT('Ctrl Pts',(25.2528827300422,-1.02933922876807,
0.));
#216452=CARTESIAN_POINT('Ctrl Pts',(25.2288604735086,-1.04025235791508,
0.));
#216453=CARTESIAN_POINT('Ctrl Pts',(25.2048822469028,-1.05107843957933,
0.));
#216454=CARTESIAN_POINT('Ctrl Pts',(25.1809485642192,-1.06181751111769,
0.));
#216455=CARTESIAN_POINT('Ctrl Pts',(25.157059946931,-1.07246961165477,0.));
#216456=CARTESIAN_POINT('Ctrl Pts',(25.1332169227413,-1.08303478197189,
0.));
#216457=CARTESIAN_POINT('Ctrl Pts',(25.1094200248446,-1.09351306445309,
0.));
#216458=CARTESIAN_POINT('Ctrl Pts',(25.0856697909679,-1.10390450301747,
0.));
#216459=CARTESIAN_POINT('Ctrl Pts',(25.0619667625336,-1.11420914306891,
0.));
#216460=CARTESIAN_POINT('Ctrl Pts',(25.0383114836899,-1.12442703144453,
0.));
#216461=CARTESIAN_POINT('Ctrl Pts',(25.0147045006195,-1.13455821638531,
0.));
#216462=CARTESIAN_POINT('Ctrl Pts',(24.9911463621433,-1.14460274758202,
0.));
#216463=CARTESIAN_POINT('Ctrl Pts',(24.9676376201502,-1.15456067621891,
0.));
#216464=CARTESIAN_POINT('Ctrl Pts',(24.9441788300932,-1.16443205502851,
0.));
#216465=CARTESIAN_POINT('Ctrl Pts',(24.9207705514448,-1.17421693835042,
0.));
#216466=CARTESIAN_POINT('Ctrl Pts',(24.8974133481829,-1.18391538220104,
0.));
#216467=CARTESIAN_POINT('Ctrl Pts',(24.8741077892075,-1.19352744434066,
0.));
#216468=CARTESIAN_POINT('Ctrl Pts',(24.8508544481974,-1.20305318426021,
0.));
#216469=CARTESIAN_POINT('Ctrl Pts',(24.8276539035092,-1.21249266318209,
0.));
#216470=CARTESIAN_POINT('Ctrl Pts',(24.8045067380536,-1.22184594406529,
0.));
#216471=CARTESIAN_POINT('Ctrl Pts',(24.7814135391799,-1.23111309161845,
0.));
#216472=CARTESIAN_POINT('Ctrl Pts',(24.7583748985438,-1.2402941723199,0.));
#216473=CARTESIAN_POINT('Ctrl Pts',(24.7353914120011,-1.24938925444327,
0.));
#216474=CARTESIAN_POINT('Ctrl Pts',(24.7124636797894,-1.25839840807419,
0.));
#216475=CARTESIAN_POINT('Ctrl Pts',(24.6895923066836,-1.26732170513501,
0.));
#216476=CARTESIAN_POINT('Ctrl Pts',(24.6667779021559,-1.27615921941643,
0.));
#216477=CARTESIAN_POINT('Ctrl Pts',(24.6440210805278,-1.28491102661515,
0.));
#216478=CARTESIAN_POINT('Ctrl Pts',(24.6213224611229,-1.29357720438108,
0.));
#216479=CARTESIAN_POINT('Ctrl Pts',(24.5986826684027,-1.30215783236363,
0.));
#216480=CARTESIAN_POINT('Ctrl Pts',(24.5761023320183,-1.31065299222023,
0.));
#216481=CARTESIAN_POINT('Ctrl Pts',(24.5535820868674,-1.31906276763669,
0.));
#216482=CARTESIAN_POINT('Ctrl Pts',(24.5311225731435,-1.32738724435327,
0.));
#216483=CARTESIAN_POINT('Ctrl Pts',(24.5087244363856,-1.33562651019687,
0.));
#216484=CARTESIAN_POINT('Ctrl Pts',(24.4863883275134,-1.34378065512339,
0.));
#216485=CARTESIAN_POINT('Ctrl Pts',(24.4641149028892,-1.35184977125649,
0.));
#216486=CARTESIAN_POINT('Ctrl Pts',(24.4419048244523,-1.35983395290629,
0.));
#216487=CARTESIAN_POINT('Ctrl Pts',(24.4197587598337,-1.36773329659958,
0.));
#216488=CARTESIAN_POINT('Ctrl Pts',(24.3976773824732,-1.37554790111611,
0.));
#216489=CARTESIAN_POINT('Ctrl Pts',(24.3756613717299,-1.38327786753,0.));
#216490=CARTESIAN_POINT('Ctrl Pts',(24.3537114129875,-1.3909232992639,0.));
#216491=CARTESIAN_POINT('Ctrl Pts',(24.3318281977643,-1.39848430212808,
0.));
#216492=CARTESIAN_POINT('Ctrl Pts',(24.3100124238311,-1.40596098434339,
0.));
#216493=CARTESIAN_POINT('Ctrl Pts',(24.288264795321,-1.41335345657684,0.));
#216494=CARTESIAN_POINT('Ctrl Pts',(24.2665860228356,-1.42066183198254,
0.));
#216495=CARTESIAN_POINT('Ctrl Pts',(24.2449768235488,-1.42788622624855,
0.));
#216496=CARTESIAN_POINT('Ctrl Pts',(24.2234379212984,-1.4350267576551,0.));
#216497=CARTESIAN_POINT('Ctrl Pts',(24.201970046722,-1.44208354711083,0.));
#216498=CARTESIAN_POINT('Ctrl Pts',(24.1805739374038,-1.44905671818729,
0.));
#216499=CARTESIAN_POINT('Ctrl Pts',(24.1592503380107,-1.45594639716319,
0.));
#216500=CARTESIAN_POINT('Ctrl Pts',(24.1380000004272,-1.46275271307399,
0.));
#216501=CARTESIAN_POINT('Ctrl Pts',(24.1168236838824,-1.46947579776993,
0.));
#216502=CARTESIAN_POINT('Ctrl Pts',(24.0957221550778,-1.47611578597743,
0.));
#216503=CARTESIAN_POINT('Ctrl Pts',(24.0746961883528,-1.48267281533684,
0.));
#216504=CARTESIAN_POINT('Ctrl Pts',(24.0537465658429,-1.48914702644889,
0.));
#216505=CARTESIAN_POINT('Ctrl Pts',(24.0328740776331,-1.49553856292802,
0.));
#216506=CARTESIAN_POINT('Ctrl Pts',(24.0120795219086,-1.501847571461,0.));
#216507=CARTESIAN_POINT('Ctrl Pts',(23.9913637050927,-1.50807420187695,
0.));
#216508=CARTESIAN_POINT('Ctrl Pts',(23.970727442014,-1.51421860720616,0.));
#216509=CARTESIAN_POINT('Ctrl Pts',(23.9501715561033,-1.52028094372793,
0.));
#216510=CARTESIAN_POINT('Ctrl Pts',(23.9296968795757,-1.52626137103033,
0.));
#216511=CARTESIAN_POINT('Ctrl Pts',(23.9093042536119,-1.53216005207464,
0.));
#216512=CARTESIAN_POINT('Ctrl Pts',(23.8889945285318,-1.53797715326759,
0.));
#216513=CARTESIAN_POINT('Ctrl Pts',(23.8687685639642,-1.54371284453992,
0.));
#216514=CARTESIAN_POINT('Ctrl Pts',(23.8486272290705,-1.54936729940542,
0.));
#216515=CARTESIAN_POINT('Ctrl Pts',(23.8285714027636,-1.55494069502636,
0.));
#216516=CARTESIAN_POINT('Ctrl Pts',(23.8086019739194,-1.56043321228635,
0.));
#216517=CARTESIAN_POINT('Ctrl Pts',(23.7887198415878,-1.56584503586844,
0.));
#216518=CARTESIAN_POINT('Ctrl Pts',(23.7689259151862,-1.57117635434409,
0.));
#216519=CARTESIAN_POINT('Ctrl Pts',(23.749221114736,-1.57642736025247,0.));
#216520=CARTESIAN_POINT('Ctrl Pts',(23.72960637113,-1.58159825017359,0.));
#216521=CARTESIAN_POINT('Ctrl Pts',(23.710082626383,-1.58668922481222,0.));
#216522=CARTESIAN_POINT('Ctrl Pts',(23.6906508338833,-1.59170048908634,
0.));
#216523=CARTESIAN_POINT('Ctrl Pts',(23.671311958631,-1.59663225222464,0.));
#216524=CARTESIAN_POINT('Ctrl Pts',(23.6520669774876,-1.60148472786596,
0.));
#216525=CARTESIAN_POINT('Ctrl Pts',(23.6329168794929,-1.60625813414674,
0.));
#216526=CARTESIAN_POINT('Ctrl Pts',(23.6138626661653,-1.61095269379779,
0.));
#216527=CARTESIAN_POINT('Ctrl Pts',(23.5949053517997,-1.61556863424699,
0.));
#216528=CARTESIAN_POINT('Ctrl Pts',(23.57604596376,-1.62010618772867,0.));
#216529=CARTESIAN_POINT('Ctrl Pts',(23.5572855427601,-1.62456559140066,
0.));
#216530=CARTESIAN_POINT('Ctrl Pts',(23.538625143226,-1.62894708745224,0.));
#216531=CARTESIAN_POINT('Ctrl Pts',(23.5200658336612,-1.63325092321727,
0.));
#216532=CARTESIAN_POINT('Ctrl Pts',(23.5016086970003,-1.63747735129475,
0.));
#216533=CARTESIAN_POINT('Ctrl Pts',(23.4832548309645,-1.64162662967529,
0.));
#216534=CARTESIAN_POINT('Ctrl Pts',(23.4650053483932,-1.64569902187612,
0.));
#216535=CARTESIAN_POINT('Ctrl Pts',(23.4468613776574,-1.64969479707341,
0.));
#216536=CARTESIAN_POINT('Ctrl Pts',(23.4288240631043,-1.6536142302373,0.));
#216537=CARTESIAN_POINT('Ctrl Pts',(23.4108945654805,-1.65745760227506,
0.));
#216538=CARTESIAN_POINT('Ctrl Pts',(23.3930740623619,-1.66122520018012,
0.));
#216539=CARTESIAN_POINT('Ctrl Pts',(23.3753637485545,-1.66491731718878,
0.));
#216540=CARTESIAN_POINT('Ctrl Pts',(23.3577648365744,-1.66853425293997,
0.));
#216541=CARTESIAN_POINT('Ctrl Pts',(23.3402785571865,-1.67207631363923,
0.));
#216542=CARTESIAN_POINT('Ctrl Pts',(23.3229061599144,-1.67554381222995,
0.));
#216543=CARTESIAN_POINT('Ctrl Pts',(23.3056489135611,-1.67893706857118,
0.));
#216544=CARTESIAN_POINT('Ctrl Pts',(23.2885081066951,-1.68225640962169,
0.));
#216545=CARTESIAN_POINT('Ctrl Pts',(23.2714850482246,-1.68550216963259,
0.));
#216546=CARTESIAN_POINT('Ctrl Pts',(23.2545810680537,-1.68867469034897,
0.));
#216547=CARTESIAN_POINT('Ctrl Pts',(23.2377975177013,-1.69177432121712,
0.));
#216548=CARTESIAN_POINT('Ctrl Pts',(23.2211357709374,-1.69480141959954,
0.));
#216549=CARTESIAN_POINT('Ctrl Pts',(23.2045972243767,-1.69775635099444,
0.));
#216550=CARTESIAN_POINT('Ctrl Pts',(23.1881832981851,-1.70063948927011,
0.));
#216551=CARTESIAN_POINT('Ctrl Pts',(23.1718954368751,-1.70345121691278,
0.));
#216552=CARTESIAN_POINT('Ctrl Pts',(23.1557351100614,-1.70619192527853,
0.));
#216553=CARTESIAN_POINT('Ctrl Pts',(23.1397038132356,-1.70886201485453,
0.));
#216554=CARTESIAN_POINT('Ctrl Pts',(23.1238030684925,-1.71146189552175,
0.));
#216555=CARTESIAN_POINT('Ctrl Pts',(23.1080344254286,-1.71399198684705,
0.));
#216556=CARTESIAN_POINT('Ctrl Pts',(23.0923994621213,-1.71645271839298,
0.));
#216557=CARTESIAN_POINT('Ctrl Pts',(23.0768997860708,-1.71884453003028,
0.));
#216558=CARTESIAN_POINT('Ctrl Pts',(23.0615370351562,-1.72116787225993,
0.));
#216559=CARTESIAN_POINT('Ctrl Pts',(23.0463128785531,-1.72342320653748,
0.));
#216560=CARTESIAN_POINT('Ctrl Pts',(23.0312290178883,-1.72561100564047,
0.));
#216561=CARTESIAN_POINT('Ctrl Pts',(23.0162871884168,-1.7277317540471,0.));
#216562=CARTESIAN_POINT('Ctrl Pts',(23.001489160189,-1.72978594832137,0.));
#216563=CARTESIAN_POINT('Ctrl Pts',(22.9868367391978,-1.73177409750192,
0.));
#216564=CARTESIAN_POINT('Ctrl Pts',(22.9723317685688,-1.73369672350816,
0.));
#216565=CARTESIAN_POINT('Ctrl Pts',(22.9579761301063,-1.73555436162771,
0.));
#216566=CARTESIAN_POINT('Ctrl Pts',(22.9437717457826,-1.7373475610004,0.));
#216567=CARTESIAN_POINT('Ctrl Pts',(22.9297205792586,-1.73907688511667,
0.));
#216568=CARTESIAN_POINT('Ctrl Pts',(22.9158246373363,-1.7407429123106,0.));
#216569=CARTESIAN_POINT('Ctrl Pts',(22.9020859716141,-1.74234623630081,
0.));
#216570=CARTESIAN_POINT('Ctrl Pts',(22.888506680335,-1.74388746677704,0.));
#216571=CARTESIAN_POINT('Ctrl Pts',(22.8750889101696,-1.74536722998202,
0.));
#216572=CARTESIAN_POINT('Ctrl Pts',(22.8618348580235,-1.74678616930666,
0.));
#216573=CARTESIAN_POINT('Ctrl Pts',(22.8487467728076,-1.74814494588494,
0.));
#216574=CARTESIAN_POINT('Ctrl Pts',(22.8358269579853,-1.74944423940117,
0.));
#216575=CARTESIAN_POINT('Ctrl Pts',(22.8230777741284,-1.75068474890884,
0.));
#216576=CARTESIAN_POINT('Ctrl Pts',(22.8105016414713,-1.75186719365593,
0.));
#216577=CARTESIAN_POINT('Ctrl Pts',(22.7981010424314,-1.75299231391468,
0.));
#216578=CARTESIAN_POINT('Ctrl Pts',(22.7858785242361,-1.75406087182937,
0.));
#216579=CARTESIAN_POINT('Ctrl Pts',(22.7738367016118,-1.75507365227133,
0.));
#216580=CARTESIAN_POINT('Ctrl Pts',(22.7619782595013,-1.75603146371642,
0.));
#216581=CARTESIAN_POINT('Ctrl Pts',(22.750305955645,-1.75693513908908,0.));
#216582=CARTESIAN_POINT('Ctrl Pts',(22.7388226235559,-1.75778553673245,
0.));
#216583=CARTESIAN_POINT('Ctrl Pts',(22.72753117773,-1.75858354204634,0.));
#216584=CARTESIAN_POINT('Ctrl Pts',(22.7164346186006,-1.75933006905926,
0.));
#216585=CARTESIAN_POINT('Ctrl Pts',(22.7055360375485,-1.76002606202402,
0.));
#216586=CARTESIAN_POINT('Ctrl Pts',(22.6948386219851,-1.76067249704888,
0.));
#216587=CARTESIAN_POINT('Ctrl Pts',(22.684345658525,-1.76127038310615,0.));
#216588=CARTESIAN_POINT('Ctrl Pts',(22.67406053567,-1.76182076289527,0.));
#216589=CARTESIAN_POINT('Ctrl Pts',(22.6639867471753,-1.7623247139257,0.));
#216590=CARTESIAN_POINT('Ctrl Pts',(22.6541278938409,-1.76278334912562,
0.));
#216591=CARTESIAN_POINT('Ctrl Pts',(22.6444876940423,-1.76319782013917,
0.));
#216592=CARTESIAN_POINT('Ctrl Pts',(22.6350699979359,-1.76356932176274,
0.));
#216593=CARTESIAN_POINT('Ctrl Pts',(22.6258787994848,-1.76389909571404,
0.));
#216594=CARTESIAN_POINT('Ctrl Pts',(22.6169182517694,-1.76418843543741,
0.));
#216595=CARTESIAN_POINT('Ctrl Pts',(22.6081926681343,-1.76443868648017,
0.));
#216596=CARTESIAN_POINT('Ctrl Pts',(22.5997065145638,-1.76465124413558,
0.));
#216597=CARTESIAN_POINT('Ctrl Pts',(22.5914644078105,-1.76482755288412,
0.));
#216598=CARTESIAN_POINT('Ctrl Pts',(22.5834711038022,-1.76496910283089,
0.));
#216599=CARTESIAN_POINT('Ctrl Pts',(22.5757315316353,-1.76507744026747,
0.));
#216600=CARTESIAN_POINT('Ctrl Pts',(22.5682508499873,-1.76515418518832,
0.));
#216601=CARTESIAN_POINT('Ctrl Pts',(22.5610344912501,-1.76520104500451,
0.));
#216602=CARTESIAN_POINT('Ctrl Pts',(22.5540882235837,-1.76521983384064,
0.));
#216603=CARTESIAN_POINT('Ctrl Pts',(22.5474180954006,-1.76521245524048,
0.));
#216604=CARTESIAN_POINT('Ctrl Pts',(22.5410303590892,-1.76518087841494,
0.));
#216605=CARTESIAN_POINT('Ctrl Pts',(22.5349313983571,-1.76512711563255,
0.));
#216606=CARTESIAN_POINT('Ctrl Pts',(22.529127665298,-1.7650532026276,0.));
#216607=CARTESIAN_POINT('Ctrl Pts',(22.5236259635515,-1.76496128643376,
0.));
#216608=CARTESIAN_POINT('Ctrl Pts',(22.5184336670207,-1.76485369319896,
0.));
#216609=CARTESIAN_POINT('Ctrl Pts',(22.5135590569554,-1.7647330328115,0.));
#216610=CARTESIAN_POINT('Ctrl Pts',(22.5090112700212,-1.76460218257314,
0.));
#216611=CARTESIAN_POINT('Ctrl Pts',(22.5047996391978,-1.76446408210366,
0.));
#216612=CARTESIAN_POINT('Ctrl Pts',(22.5009332677316,-1.76432160068739,
0.));
#216613=CARTESIAN_POINT('Ctrl Pts',(22.4974203063191,-1.76417731243484,
0.));
#216614=CARTESIAN_POINT('Ctrl Pts',(22.4942693792449,-1.76403393880317,
0.));
#216615=CARTESIAN_POINT('Ctrl Pts',(22.4914909094908,-1.76389475965715,
0.));
#216616=CARTESIAN_POINT('Ctrl Pts',(22.4890991659479,-1.76376424879469,
0.));
#216617=CARTESIAN_POINT('Ctrl Pts',(22.4871115206572,-1.76364784232927,
0.));
#216618=CARTESIAN_POINT('Ctrl Pts',(22.4855446605991,-1.7635507604555,0.));
#216619=CARTESIAN_POINT('Ctrl Pts',(22.4844112933125,-1.76347698284863,
0.));
#216620=CARTESIAN_POINT('Ctrl Pts',(22.4838562517064,-1.7634381343466,0.));
#216621=CARTESIAN_POINT('Ctrl Pts',(22.4836387052228,-1.76342064263638,
0.));
#216622=CARTESIAN_POINT('Ctrl Pts',(22.4835819929788,-1.76341415538792,
0.));
#216623=CARTESIAN_POINT('Ctrl Pts',(22.4835757167854,-1.76341220531181,
0.));
#216624=CARTESIAN_POINT('',(25.991588367311,-0.661312440730916,12.));
#216625=CARTESIAN_POINT('',(25.991588367311,-0.661312440730916,0.));
#216626=CARTESIAN_POINT('Ctrl Pts',(22.4835757167854,-1.76341220531181,
12.));
#216627=CARTESIAN_POINT('Ctrl Pts',(22.4835819929788,-1.76341415538792,
12.));
#216628=CARTESIAN_POINT('Ctrl Pts',(22.4836387052228,-1.76342064263638,
12.));
#216629=CARTESIAN_POINT('Ctrl Pts',(22.4838562517064,-1.7634381343466,12.));
#216630=CARTESIAN_POINT('Ctrl Pts',(22.4844112933125,-1.76347698284863,
12.));
#216631=CARTESIAN_POINT('Ctrl Pts',(22.4855446605991,-1.7635507604555,12.));
#216632=CARTESIAN_POINT('Ctrl Pts',(22.4871115206572,-1.76364784232927,
12.));
#216633=CARTESIAN_POINT('Ctrl Pts',(22.4890991659479,-1.76376424879469,
12.));
#216634=CARTESIAN_POINT('Ctrl Pts',(22.4914909094908,-1.76389475965715,
12.));
#216635=CARTESIAN_POINT('Ctrl Pts',(22.4942693792449,-1.76403393880317,
12.));
#216636=CARTESIAN_POINT('Ctrl Pts',(22.4974203063191,-1.76417731243484,
12.));
#216637=CARTESIAN_POINT('Ctrl Pts',(22.5009332677316,-1.76432160068739,
12.));
#216638=CARTESIAN_POINT('Ctrl Pts',(22.5047996391978,-1.76446408210366,
12.));
#216639=CARTESIAN_POINT('Ctrl Pts',(22.5090112700212,-1.76460218257314,
12.));
#216640=CARTESIAN_POINT('Ctrl Pts',(22.5135590569554,-1.7647330328115,12.));
#216641=CARTESIAN_POINT('Ctrl Pts',(22.5184336670207,-1.76485369319896,
12.));
#216642=CARTESIAN_POINT('Ctrl Pts',(22.5236259635515,-1.76496128643376,
12.));
#216643=CARTESIAN_POINT('Ctrl Pts',(22.529127665298,-1.7650532026276,12.));
#216644=CARTESIAN_POINT('Ctrl Pts',(22.5349313983571,-1.76512711563255,
12.));
#216645=CARTESIAN_POINT('Ctrl Pts',(22.5410303590892,-1.76518087841494,
12.));
#216646=CARTESIAN_POINT('Ctrl Pts',(22.5474180954006,-1.76521245524048,
12.));
#216647=CARTESIAN_POINT('Ctrl Pts',(22.5540882235837,-1.76521983384064,
12.));
#216648=CARTESIAN_POINT('Ctrl Pts',(22.5610344912501,-1.76520104500451,
12.));
#216649=CARTESIAN_POINT('Ctrl Pts',(22.5682508499873,-1.76515418518832,
12.));
#216650=CARTESIAN_POINT('Ctrl Pts',(22.5757315316353,-1.76507744026747,
12.));
#216651=CARTESIAN_POINT('Ctrl Pts',(22.5834711038022,-1.76496910283089,
12.));
#216652=CARTESIAN_POINT('Ctrl Pts',(22.5914644078105,-1.76482755288412,
12.));
#216653=CARTESIAN_POINT('Ctrl Pts',(22.5997065145638,-1.76465124413558,
12.));
#216654=CARTESIAN_POINT('Ctrl Pts',(22.6081926681343,-1.76443868648017,
12.));
#216655=CARTESIAN_POINT('Ctrl Pts',(22.6169182517694,-1.76418843543741,
12.));
#216656=CARTESIAN_POINT('Ctrl Pts',(22.6258787994848,-1.76389909571404,
12.));
#216657=CARTESIAN_POINT('Ctrl Pts',(22.6350699979359,-1.76356932176274,
12.));
#216658=CARTESIAN_POINT('Ctrl Pts',(22.6444876940423,-1.76319782013917,
12.));
#216659=CARTESIAN_POINT('Ctrl Pts',(22.6541278938409,-1.76278334912562,
12.));
#216660=CARTESIAN_POINT('Ctrl Pts',(22.6639867471753,-1.7623247139257,12.));
#216661=CARTESIAN_POINT('Ctrl Pts',(22.67406053567,-1.76182076289527,12.));
#216662=CARTESIAN_POINT('Ctrl Pts',(22.684345658525,-1.76127038310615,12.));
#216663=CARTESIAN_POINT('Ctrl Pts',(22.6948386219851,-1.76067249704888,
12.));
#216664=CARTESIAN_POINT('Ctrl Pts',(22.7055360375485,-1.76002606202402,
12.));
#216665=CARTESIAN_POINT('Ctrl Pts',(22.7164346186006,-1.75933006905926,
12.));
#216666=CARTESIAN_POINT('Ctrl Pts',(22.72753117773,-1.75858354204634,12.));
#216667=CARTESIAN_POINT('Ctrl Pts',(22.7388226235559,-1.75778553673245,
12.));
#216668=CARTESIAN_POINT('Ctrl Pts',(22.750305955645,-1.75693513908908,12.));
#216669=CARTESIAN_POINT('Ctrl Pts',(22.7619782595013,-1.75603146371642,
12.));
#216670=CARTESIAN_POINT('Ctrl Pts',(22.7738367016118,-1.75507365227133,
12.));
#216671=CARTESIAN_POINT('Ctrl Pts',(22.7858785242361,-1.75406087182937,
12.));
#216672=CARTESIAN_POINT('Ctrl Pts',(22.7981010424314,-1.75299231391468,
12.));
#216673=CARTESIAN_POINT('Ctrl Pts',(22.8105016414713,-1.75186719365593,
12.));
#216674=CARTESIAN_POINT('Ctrl Pts',(22.8230777741284,-1.75068474890884,
12.));
#216675=CARTESIAN_POINT('Ctrl Pts',(22.8358269579853,-1.74944423940117,
12.));
#216676=CARTESIAN_POINT('Ctrl Pts',(22.8487467728076,-1.74814494588494,
12.));
#216677=CARTESIAN_POINT('Ctrl Pts',(22.8618348580235,-1.74678616930666,
12.));
#216678=CARTESIAN_POINT('Ctrl Pts',(22.8750889101696,-1.74536722998202,
12.));
#216679=CARTESIAN_POINT('Ctrl Pts',(22.888506680335,-1.74388746677704,12.));
#216680=CARTESIAN_POINT('Ctrl Pts',(22.9020859716141,-1.74234623630081,
12.));
#216681=CARTESIAN_POINT('Ctrl Pts',(22.9158246373363,-1.7407429123106,12.));
#216682=CARTESIAN_POINT('Ctrl Pts',(22.9297205792586,-1.73907688511667,
12.));
#216683=CARTESIAN_POINT('Ctrl Pts',(22.9437717457826,-1.7373475610004,12.));
#216684=CARTESIAN_POINT('Ctrl Pts',(22.9579761301063,-1.73555436162771,
12.));
#216685=CARTESIAN_POINT('Ctrl Pts',(22.9723317685688,-1.73369672350816,
12.));
#216686=CARTESIAN_POINT('Ctrl Pts',(22.9868367391978,-1.73177409750192,
12.));
#216687=CARTESIAN_POINT('Ctrl Pts',(23.001489160189,-1.72978594832137,12.));
#216688=CARTESIAN_POINT('Ctrl Pts',(23.0162871884168,-1.7277317540471,12.));
#216689=CARTESIAN_POINT('Ctrl Pts',(23.0312290178883,-1.72561100564047,
12.));
#216690=CARTESIAN_POINT('Ctrl Pts',(23.0463128785531,-1.72342320653748,
12.));
#216691=CARTESIAN_POINT('Ctrl Pts',(23.0615370351562,-1.72116787225993,
12.));
#216692=CARTESIAN_POINT('Ctrl Pts',(23.0768997860708,-1.71884453003028,
12.));
#216693=CARTESIAN_POINT('Ctrl Pts',(23.0923994621213,-1.71645271839298,
12.));
#216694=CARTESIAN_POINT('Ctrl Pts',(23.1080344254286,-1.71399198684705,
12.));
#216695=CARTESIAN_POINT('Ctrl Pts',(23.1238030684925,-1.71146189552175,
12.));
#216696=CARTESIAN_POINT('Ctrl Pts',(23.1397038132356,-1.70886201485453,
12.));
#216697=CARTESIAN_POINT('Ctrl Pts',(23.1557351100614,-1.70619192527853,
12.));
#216698=CARTESIAN_POINT('Ctrl Pts',(23.1718954368751,-1.70345121691278,
12.));
#216699=CARTESIAN_POINT('Ctrl Pts',(23.1881832981851,-1.70063948927011,
12.));
#216700=CARTESIAN_POINT('Ctrl Pts',(23.2045972243767,-1.69775635099444,
12.));
#216701=CARTESIAN_POINT('Ctrl Pts',(23.2211357709374,-1.69480141959954,
12.));
#216702=CARTESIAN_POINT('Ctrl Pts',(23.2377975177013,-1.69177432121712,
12.));
#216703=CARTESIAN_POINT('Ctrl Pts',(23.2545810680537,-1.68867469034897,
12.));
#216704=CARTESIAN_POINT('Ctrl Pts',(23.2714850482246,-1.68550216963259,
12.));
#216705=CARTESIAN_POINT('Ctrl Pts',(23.2885081066951,-1.68225640962169,
12.));
#216706=CARTESIAN_POINT('Ctrl Pts',(23.3056489135611,-1.67893706857118,
12.));
#216707=CARTESIAN_POINT('Ctrl Pts',(23.3229061599144,-1.67554381222995,
12.));
#216708=CARTESIAN_POINT('Ctrl Pts',(23.3402785571865,-1.67207631363923,
12.));
#216709=CARTESIAN_POINT('Ctrl Pts',(23.3577648365744,-1.66853425293997,
12.));
#216710=CARTESIAN_POINT('Ctrl Pts',(23.3753637485545,-1.66491731718878,
12.));
#216711=CARTESIAN_POINT('Ctrl Pts',(23.3930740623619,-1.66122520018012,
12.));
#216712=CARTESIAN_POINT('Ctrl Pts',(23.4108945654805,-1.65745760227506,
12.));
#216713=CARTESIAN_POINT('Ctrl Pts',(23.4288240631043,-1.6536142302373,12.));
#216714=CARTESIAN_POINT('Ctrl Pts',(23.4468613776574,-1.64969479707341,
12.));
#216715=CARTESIAN_POINT('Ctrl Pts',(23.4650053483932,-1.64569902187612,
12.));
#216716=CARTESIAN_POINT('Ctrl Pts',(23.4832548309645,-1.64162662967529,
12.));
#216717=CARTESIAN_POINT('Ctrl Pts',(23.5016086970003,-1.63747735129475,
12.));
#216718=CARTESIAN_POINT('Ctrl Pts',(23.5200658336612,-1.63325092321727,
12.));
#216719=CARTESIAN_POINT('Ctrl Pts',(23.538625143226,-1.62894708745224,12.));
#216720=CARTESIAN_POINT('Ctrl Pts',(23.5572855427601,-1.62456559140066,
12.));
#216721=CARTESIAN_POINT('Ctrl Pts',(23.57604596376,-1.62010618772867,12.));
#216722=CARTESIAN_POINT('Ctrl Pts',(23.5949053517997,-1.61556863424699,
12.));
#216723=CARTESIAN_POINT('Ctrl Pts',(23.6138626661653,-1.61095269379779,
12.));
#216724=CARTESIAN_POINT('Ctrl Pts',(23.6329168794929,-1.60625813414674,
12.));
#216725=CARTESIAN_POINT('Ctrl Pts',(23.6520669774876,-1.60148472786596,
12.));
#216726=CARTESIAN_POINT('Ctrl Pts',(23.671311958631,-1.59663225222464,12.));
#216727=CARTESIAN_POINT('Ctrl Pts',(23.6906508338833,-1.59170048908634,
12.));
#216728=CARTESIAN_POINT('Ctrl Pts',(23.710082626383,-1.58668922481222,12.));
#216729=CARTESIAN_POINT('Ctrl Pts',(23.72960637113,-1.58159825017359,12.));
#216730=CARTESIAN_POINT('Ctrl Pts',(23.749221114736,-1.57642736025247,12.));
#216731=CARTESIAN_POINT('Ctrl Pts',(23.7689259151862,-1.57117635434409,
12.));
#216732=CARTESIAN_POINT('Ctrl Pts',(23.7887198415878,-1.56584503586844,
12.));
#216733=CARTESIAN_POINT('Ctrl Pts',(23.8086019739194,-1.56043321228635,
12.));
#216734=CARTESIAN_POINT('Ctrl Pts',(23.8285714027636,-1.55494069502636,
12.));
#216735=CARTESIAN_POINT('Ctrl Pts',(23.8486272290705,-1.54936729940542,
12.));
#216736=CARTESIAN_POINT('Ctrl Pts',(23.8687685639642,-1.54371284453992,
12.));
#216737=CARTESIAN_POINT('Ctrl Pts',(23.8889945285318,-1.53797715326759,
12.));
#216738=CARTESIAN_POINT('Ctrl Pts',(23.9093042536119,-1.53216005207464,
12.));
#216739=CARTESIAN_POINT('Ctrl Pts',(23.9296968795757,-1.52626137103033,
12.));
#216740=CARTESIAN_POINT('Ctrl Pts',(23.9501715561033,-1.52028094372793,
12.));
#216741=CARTESIAN_POINT('Ctrl Pts',(23.970727442014,-1.51421860720616,12.));
#216742=CARTESIAN_POINT('Ctrl Pts',(23.9913637050927,-1.50807420187695,
12.));
#216743=CARTESIAN_POINT('Ctrl Pts',(24.0120795219086,-1.501847571461,12.));
#216744=CARTESIAN_POINT('Ctrl Pts',(24.0328740776331,-1.49553856292802,
12.));
#216745=CARTESIAN_POINT('Ctrl Pts',(24.0537465658429,-1.48914702644889,
12.));
#216746=CARTESIAN_POINT('Ctrl Pts',(24.0746961883528,-1.48267281533684,
12.));
#216747=CARTESIAN_POINT('Ctrl Pts',(24.0957221550778,-1.47611578597743,
12.));
#216748=CARTESIAN_POINT('Ctrl Pts',(24.1168236838824,-1.46947579776993,
12.));
#216749=CARTESIAN_POINT('Ctrl Pts',(24.1380000004272,-1.46275271307399,
12.));
#216750=CARTESIAN_POINT('Ctrl Pts',(24.1592503380107,-1.45594639716319,
12.));
#216751=CARTESIAN_POINT('Ctrl Pts',(24.1805739374038,-1.44905671818729,
12.));
#216752=CARTESIAN_POINT('Ctrl Pts',(24.201970046722,-1.44208354711083,12.));
#216753=CARTESIAN_POINT('Ctrl Pts',(24.2234379212984,-1.4350267576551,12.));
#216754=CARTESIAN_POINT('Ctrl Pts',(24.2449768235488,-1.42788622624855,
12.));
#216755=CARTESIAN_POINT('Ctrl Pts',(24.2665860228356,-1.42066183198254,
12.));
#216756=CARTESIAN_POINT('Ctrl Pts',(24.288264795321,-1.41335345657684,12.));
#216757=CARTESIAN_POINT('Ctrl Pts',(24.3100124238311,-1.40596098434339,
12.));
#216758=CARTESIAN_POINT('Ctrl Pts',(24.3318281977643,-1.39848430212808,
12.));
#216759=CARTESIAN_POINT('Ctrl Pts',(24.3537114129875,-1.3909232992639,12.));
#216760=CARTESIAN_POINT('Ctrl Pts',(24.3756613717299,-1.38327786753,12.));
#216761=CARTESIAN_POINT('Ctrl Pts',(24.3976773824732,-1.37554790111611,
12.));
#216762=CARTESIAN_POINT('Ctrl Pts',(24.4197587598337,-1.36773329659958,
12.));
#216763=CARTESIAN_POINT('Ctrl Pts',(24.4419048244523,-1.35983395290629,
12.));
#216764=CARTESIAN_POINT('Ctrl Pts',(24.4641149028892,-1.35184977125649,
12.));
#216765=CARTESIAN_POINT('Ctrl Pts',(24.4863883275134,-1.34378065512339,
12.));
#216766=CARTESIAN_POINT('Ctrl Pts',(24.5087244363856,-1.33562651019687,
12.));
#216767=CARTESIAN_POINT('Ctrl Pts',(24.5311225731435,-1.32738724435327,
12.));
#216768=CARTESIAN_POINT('Ctrl Pts',(24.5535820868674,-1.31906276763669,
12.));
#216769=CARTESIAN_POINT('Ctrl Pts',(24.5761023320183,-1.31065299222023,
12.));
#216770=CARTESIAN_POINT('Ctrl Pts',(24.5986826684027,-1.30215783236363,
12.));
#216771=CARTESIAN_POINT('Ctrl Pts',(24.6213224611229,-1.29357720438108,
12.));
#216772=CARTESIAN_POINT('Ctrl Pts',(24.6440210805278,-1.28491102661515,
12.));
#216773=CARTESIAN_POINT('Ctrl Pts',(24.6667779021559,-1.27615921941643,
12.));
#216774=CARTESIAN_POINT('Ctrl Pts',(24.6895923066836,-1.26732170513501,
12.));
#216775=CARTESIAN_POINT('Ctrl Pts',(24.7124636797894,-1.25839840807419,
12.));
#216776=CARTESIAN_POINT('Ctrl Pts',(24.7353914120011,-1.24938925444327,
12.));
#216777=CARTESIAN_POINT('Ctrl Pts',(24.7583748985438,-1.2402941723199,12.));
#216778=CARTESIAN_POINT('Ctrl Pts',(24.7814135391799,-1.23111309161845,
12.));
#216779=CARTESIAN_POINT('Ctrl Pts',(24.8045067380536,-1.22184594406529,
12.));
#216780=CARTESIAN_POINT('Ctrl Pts',(24.8276539035092,-1.21249266318209,
12.));
#216781=CARTESIAN_POINT('Ctrl Pts',(24.8508544481974,-1.20305318426021,
12.));
#216782=CARTESIAN_POINT('Ctrl Pts',(24.8741077892075,-1.19352744434066,
12.));
#216783=CARTESIAN_POINT('Ctrl Pts',(24.8974133481829,-1.18391538220104,
12.));
#216784=CARTESIAN_POINT('Ctrl Pts',(24.9207705514448,-1.17421693835042,
12.));
#216785=CARTESIAN_POINT('Ctrl Pts',(24.9441788300932,-1.16443205502851,
12.));
#216786=CARTESIAN_POINT('Ctrl Pts',(24.9676376201502,-1.15456067621891,
12.));
#216787=CARTESIAN_POINT('Ctrl Pts',(24.9911463621433,-1.14460274758202,
12.));
#216788=CARTESIAN_POINT('Ctrl Pts',(25.0147045006195,-1.13455821638531,
12.));
#216789=CARTESIAN_POINT('Ctrl Pts',(25.0383114836899,-1.12442703144453,
12.));
#216790=CARTESIAN_POINT('Ctrl Pts',(25.0619667625336,-1.11420914306891,
12.));
#216791=CARTESIAN_POINT('Ctrl Pts',(25.0856697909679,-1.10390450301747,
12.));
#216792=CARTESIAN_POINT('Ctrl Pts',(25.1094200248446,-1.09351306445309,
12.));
#216793=CARTESIAN_POINT('Ctrl Pts',(25.1332169227413,-1.08303478197189,
12.));
#216794=CARTESIAN_POINT('Ctrl Pts',(25.157059946931,-1.07246961165477,12.));
#216795=CARTESIAN_POINT('Ctrl Pts',(25.1809485642192,-1.06181751111769,
12.));
#216796=CARTESIAN_POINT('Ctrl Pts',(25.2048822469028,-1.05107843957933,
12.));
#216797=CARTESIAN_POINT('Ctrl Pts',(25.2288604735086,-1.04025235791508,
12.));
#216798=CARTESIAN_POINT('Ctrl Pts',(25.2528827300422,-1.02933922876807,
12.));
#216799=CARTESIAN_POINT('Ctrl Pts',(25.276948508726,-1.01833901642238,12.));
#216800=CARTESIAN_POINT('Ctrl Pts',(25.3010573055547,-1.00725168656897,
12.));
#216801=CARTESIAN_POINT('Ctrl Pts',(25.3252086182968,-0.996077206120637,
12.));
#216802=CARTESIAN_POINT('Ctrl Pts',(25.3494019441441,-0.984815543003986,
12.));
#216803=CARTESIAN_POINT('Ctrl Pts',(25.3736367778845,-0.973466666000178,
12.));
#216804=CARTESIAN_POINT('Ctrl Pts',(25.3979126089163,-0.962030544503156,
12.));
#216805=CARTESIAN_POINT('Ctrl Pts',(25.4222289223167,-0.950507148597483,
12.));
#216806=CARTESIAN_POINT('Ctrl Pts',(25.4465852044849,-0.938896449496205,
12.));
#216807=CARTESIAN_POINT('Ctrl Pts',(25.4709809475009,-0.927198419886108,
12.));
#216808=CARTESIAN_POINT('Ctrl Pts',(25.4954156541795,-0.915413034335626,
12.));
#216809=CARTESIAN_POINT('Ctrl Pts',(25.5198888424194,-0.903540269651121,
12.));
#216810=CARTESIAN_POINT('Ctrl Pts',(25.5444000508211,-0.891580105349052,
12.));
#216811=CARTESIAN_POINT('Ctrl Pts',(25.5689488408156,-0.879532523834308,
12.));
#216812=CARTESIAN_POINT('Ctrl Pts',(25.5935347843585,-0.867397509338443,
12.));
#216813=CARTESIAN_POINT('Ctrl Pts',(25.6181574536049,-0.855175047036563,
12.));
#216814=CARTESIAN_POINT('Ctrl Pts',(25.6428164100055,-0.842865122120773,
12.));
#216815=CARTESIAN_POINT('Ctrl Pts',(25.6675111931952,-0.830467718864221,
12.));
#216816=CARTESIAN_POINT('Ctrl Pts',(25.6922413110194,-0.817982819787478,
12.));
#216817=CARTESIAN_POINT('Ctrl Pts',(25.7170062262525,-0.805410404554366,
12.));
#216818=CARTESIAN_POINT('Ctrl Pts',(25.7418053757746,-0.79275045161614,
12.));
#216819=CARTESIAN_POINT('Ctrl Pts',(25.7666381946955,-0.780002940291977,
12.));
#216820=CARTESIAN_POINT('Ctrl Pts',(25.7915041383376,-0.767167852651183,
12.));
#216821=CARTESIAN_POINT('Ctrl Pts',(25.8164027059984,-0.754245175609537,
12.));
#216822=CARTESIAN_POINT('Ctrl Pts',(25.8413334619054,-0.74123490266382,
12.));
#216823=CARTESIAN_POINT('Ctrl Pts',(25.8662960624185,-0.728137036482349,
12.));
#216824=CARTESIAN_POINT('Ctrl Pts',(25.8912902614969,-0.714951588527653,
12.));
#216825=CARTESIAN_POINT('Ctrl Pts',(25.9163158909426,-0.701678575228769,
12.));
#216826=CARTESIAN_POINT('Ctrl Pts',(25.9413728471909,-0.688318015057744,
12.));
#216827=CARTESIAN_POINT('Ctrl Pts',(25.9614434297919,-0.67755954320974,
12.));
#216828=CARTESIAN_POINT('Ctrl Pts',(25.9765104298071,-0.669451306780839,
12.));
#216829=CARTESIAN_POINT('Ctrl Pts',(25.9865613464773,-0.66402831318764,
12.));
#216830=CARTESIAN_POINT('Ctrl Pts',(25.991588367311,-0.661312440730916,
12.));
#216831=CARTESIAN_POINT('Ctrl Pts',(22.1738711152697,-4.11585220600463,
0.));
#216832=CARTESIAN_POINT('Ctrl Pts',(22.1738711152697,-4.11585220600463,
12.));
#216833=CARTESIAN_POINT('Ctrl Pts',(22.173877682324,-4.11585194677443,0.));
#216834=CARTESIAN_POINT('Ctrl Pts',(22.173877682324,-4.11585194677443,12.));
#216835=CARTESIAN_POINT('Ctrl Pts',(22.1739341411687,-4.11586035878288,
0.));
#216836=CARTESIAN_POINT('Ctrl Pts',(22.1739341411687,-4.11586035878288,
12.));
#216837=CARTESIAN_POINT('Ctrl Pts',(22.1741488021234,-4.11589976826168,
0.));
#216838=CARTESIAN_POINT('Ctrl Pts',(22.1741488021234,-4.11589976826168,
12.));
#216839=CARTESIAN_POINT('Ctrl Pts',(22.1746949858775,-4.11600589882846,
0.));
#216840=CARTESIAN_POINT('Ctrl Pts',(22.1746949858775,-4.11600589882846,
12.));
#216841=CARTESIAN_POINT('Ctrl Pts',(22.1758088296598,-4.1162279721707,0.));
#216842=CARTESIAN_POINT('Ctrl Pts',(22.1758088296598,-4.1162279721707,12.));
#216843=CARTESIAN_POINT('Ctrl Pts',(22.177347426894,-4.11653973150519,0.));
#216844=CARTESIAN_POINT('Ctrl Pts',(22.177347426894,-4.11653973150519,12.));
#216845=CARTESIAN_POINT('Ctrl Pts',(22.179297473024,-4.11694173195005,0.));
#216846=CARTESIAN_POINT('Ctrl Pts',(22.179297473024,-4.11694173195005,12.));
#216847=CARTESIAN_POINT('Ctrl Pts',(22.1816414985788,-4.11743469691757,
0.));
#216848=CARTESIAN_POINT('Ctrl Pts',(22.1816414985788,-4.11743469691757,
12.));
#216849=CARTESIAN_POINT('Ctrl Pts',(22.1843613164855,-4.11801938107481,
0.));
#216850=CARTESIAN_POINT('Ctrl Pts',(22.1843613164855,-4.11801938107481,
12.));
#216851=CARTESIAN_POINT('Ctrl Pts',(22.1874419861496,-4.11869641271775,
0.));
#216852=CARTESIAN_POINT('Ctrl Pts',(22.1874419861496,-4.11869641271775,
12.));
#216853=CARTESIAN_POINT('Ctrl Pts',(22.1908725908525,-4.11946626228637,
0.));
#216854=CARTESIAN_POINT('Ctrl Pts',(22.1908725908525,-4.11946626228637,
12.));
#216855=CARTESIAN_POINT('Ctrl Pts',(22.1946440958098,-4.12032932637738,
0.));
#216856=CARTESIAN_POINT('Ctrl Pts',(22.1946440958098,-4.12032932637738,
12.));
#216857=CARTESIAN_POINT('Ctrl Pts',(22.1987479618246,-4.12128598183523,
0.));
#216858=CARTESIAN_POINT('Ctrl Pts',(22.1987479618246,-4.12128598183523,
12.));
#216859=CARTESIAN_POINT('Ctrl Pts',(22.2031746532106,-4.12233664408228,
0.));
#216860=CARTESIAN_POINT('Ctrl Pts',(22.2031746532106,-4.12233664408228,
12.));
#216861=CARTESIAN_POINT('Ctrl Pts',(22.2079143941719,-4.12348173702024,
0.));
#216862=CARTESIAN_POINT('Ctrl Pts',(22.2079143941719,-4.12348173702024,
12.));
#216863=CARTESIAN_POINT('Ctrl Pts',(22.2129576146671,-4.12472167516608,
0.));
#216864=CARTESIAN_POINT('Ctrl Pts',(22.2129576146671,-4.12472167516608,
12.));
#216865=CARTESIAN_POINT('Ctrl Pts',(22.2182956401341,-4.12605683613308,
0.));
#216866=CARTESIAN_POINT('Ctrl Pts',(22.2182956401341,-4.12605683613308,
12.));
#216867=CARTESIAN_POINT('Ctrl Pts',(22.2239207458781,-4.12748755830105,
0.));
#216868=CARTESIAN_POINT('Ctrl Pts',(22.2239207458781,-4.12748755830105,
12.));
#216869=CARTESIAN_POINT('Ctrl Pts',(22.2298258043947,-4.1290141546338,0.));
#216870=CARTESIAN_POINT('Ctrl Pts',(22.2298258043947,-4.1290141546338,12.));
#216871=CARTESIAN_POINT('Ctrl Pts',(22.2360040565533,-4.13063692157499,
0.));
#216872=CARTESIAN_POINT('Ctrl Pts',(22.2360040565533,-4.13063692157499,
12.));
#216873=CARTESIAN_POINT('Ctrl Pts',(22.2424488153523,-4.13235615060161,
0.));
#216874=CARTESIAN_POINT('Ctrl Pts',(22.2424488153523,-4.13235615060161,
12.));
#216875=CARTESIAN_POINT('Ctrl Pts',(22.249153531779,-4.13417212558811,0.));
#216876=CARTESIAN_POINT('Ctrl Pts',(22.249153531779,-4.13417212558811,12.));
#216877=CARTESIAN_POINT('Ctrl Pts',(22.2561118708421,-4.13608511977227,
0.));
#216878=CARTESIAN_POINT('Ctrl Pts',(22.2561118708421,-4.13608511977227,
12.));
#216879=CARTESIAN_POINT('Ctrl Pts',(22.2633177913972,-4.13809539255423,
0.));
#216880=CARTESIAN_POINT('Ctrl Pts',(22.2633177913972,-4.13809539255423,
12.));
#216881=CARTESIAN_POINT('Ctrl Pts',(22.2707656042457,-4.14020318715992,
0.));
#216882=CARTESIAN_POINT('Ctrl Pts',(22.2707656042457,-4.14020318715992,
12.));
#216883=CARTESIAN_POINT('Ctrl Pts',(22.2784499072027,-4.14240873321985,
0.));
#216884=CARTESIAN_POINT('Ctrl Pts',(22.2784499072027,-4.14240873321985,
12.));
#216885=CARTESIAN_POINT('Ctrl Pts',(22.2863655389166,-4.14471224859297,
0.));
#216886=CARTESIAN_POINT('Ctrl Pts',(22.2863655389166,-4.14471224859297,
12.));
#216887=CARTESIAN_POINT('Ctrl Pts',(22.2945075198467,-4.14711394168557,
0.));
#216888=CARTESIAN_POINT('Ctrl Pts',(22.2945075198467,-4.14711394168557,
12.));
#216889=CARTESIAN_POINT('Ctrl Pts',(22.3028710166933,-4.14961401285523,
0.));
#216890=CARTESIAN_POINT('Ctrl Pts',(22.3028710166933,-4.14961401285523,
12.));
#216891=CARTESIAN_POINT('Ctrl Pts',(22.3114513545185,-4.15221265396991,
0.));
#216892=CARTESIAN_POINT('Ctrl Pts',(22.3114513545185,-4.15221265396991,
12.));
#216893=CARTESIAN_POINT('Ctrl Pts',(22.3202440186979,-4.15491004835282,
0.));
#216894=CARTESIAN_POINT('Ctrl Pts',(22.3202440186979,-4.15491004835282,
12.));
#216895=CARTESIAN_POINT('Ctrl Pts',(22.3292446628959,-4.15770637047891,
0.));
#216896=CARTESIAN_POINT('Ctrl Pts',(22.3292446628959,-4.15770637047891,
12.));
#216897=CARTESIAN_POINT('Ctrl Pts',(22.3384491078602,-4.16060178604165,
0.));
#216898=CARTESIAN_POINT('Ctrl Pts',(22.3384491078602,-4.16060178604165,
12.));
#216899=CARTESIAN_POINT('Ctrl Pts',(22.3478533253889,-4.16359645263189,
0.));
#216900=CARTESIAN_POINT('Ctrl Pts',(22.3478533253889,-4.16359645263189,
12.));
#216901=CARTESIAN_POINT('Ctrl Pts',(22.3574534257396,-4.16669052026601,
0.));
#216902=CARTESIAN_POINT('Ctrl Pts',(22.3574534257396,-4.16669052026601,
12.));
#216903=CARTESIAN_POINT('Ctrl Pts',(22.3672456427599,-4.16988413199458,
0.));
#216904=CARTESIAN_POINT('Ctrl Pts',(22.3672456427599,-4.16988413199458,
12.));
#216905=CARTESIAN_POINT('Ctrl Pts',(22.3772263228617,-4.17317742436146,
0.));
#216906=CARTESIAN_POINT('Ctrl Pts',(22.3772263228617,-4.17317742436146,
12.));
#216907=CARTESIAN_POINT('Ctrl Pts',(22.3873919231334,-4.17657052752826,
0.));
#216908=CARTESIAN_POINT('Ctrl Pts',(22.3873919231334,-4.17657052752826,
12.));
#216909=CARTESIAN_POINT('Ctrl Pts',(22.3977390078075,-4.18006356544883,
0.));
#216910=CARTESIAN_POINT('Ctrl Pts',(22.3977390078075,-4.18006356544883,
12.));
#216911=CARTESIAN_POINT('Ctrl Pts',(22.4082642454453,-4.18365665600852,
0.));
#216912=CARTESIAN_POINT('Ctrl Pts',(22.4082642454453,-4.18365665600852,
12.));
#216913=CARTESIAN_POINT('Ctrl Pts',(22.4189644056115,-4.18734991117722,
0.));
#216914=CARTESIAN_POINT('Ctrl Pts',(22.4189644056115,-4.18734991117722,
12.));
#216915=CARTESIAN_POINT('Ctrl Pts',(22.4298363535421,-4.19114343726943,
0.));
#216916=CARTESIAN_POINT('Ctrl Pts',(22.4298363535421,-4.19114343726943,
12.));
#216917=CARTESIAN_POINT('Ctrl Pts',(22.4408770448917,-4.19503733518862,
0.));
#216918=CARTESIAN_POINT('Ctrl Pts',(22.4408770448917,-4.19503733518862,
12.));
#216919=CARTESIAN_POINT('Ctrl Pts',(22.4520835205419,-4.19903170066356,
0.));
#216920=CARTESIAN_POINT('Ctrl Pts',(22.4520835205419,-4.19903170066356,
12.));
#216921=CARTESIAN_POINT('Ctrl Pts',(22.4634529011433,-4.20312662448172,
0.));
#216922=CARTESIAN_POINT('Ctrl Pts',(22.4634529011433,-4.20312662448172,
12.));
#216923=CARTESIAN_POINT('Ctrl Pts',(22.4749823839915,-4.20732219265649,
0.));
#216924=CARTESIAN_POINT('Ctrl Pts',(22.4749823839915,-4.20732219265649,
12.));
#216925=CARTESIAN_POINT('Ctrl Pts',(22.4866692403147,-4.21161848657429,
0.));
#216926=CARTESIAN_POINT('Ctrl Pts',(22.4866692403147,-4.21161848657429,
12.));
#216927=CARTESIAN_POINT('Ctrl Pts',(22.4985108124229,-4.21601558313909,
0.));
#216928=CARTESIAN_POINT('Ctrl Pts',(22.4985108124229,-4.21601558313909,
12.));
#216929=CARTESIAN_POINT('Ctrl Pts',(22.5105045108882,-4.22051355490198,
0.));
#216930=CARTESIAN_POINT('Ctrl Pts',(22.5105045108882,-4.22051355490198,
12.));
#216931=CARTESIAN_POINT('Ctrl Pts',(22.5226478117885,-4.22511247020041,
0.));
#216932=CARTESIAN_POINT('Ctrl Pts',(22.5226478117885,-4.22511247020041,
12.));
#216933=CARTESIAN_POINT('Ctrl Pts',(22.5349382540587,-4.22981239330733,
0.));
#216934=CARTESIAN_POINT('Ctrl Pts',(22.5349382540587,-4.22981239330733,
12.));
#216935=CARTESIAN_POINT('Ctrl Pts',(22.5473734368086,-4.23461338456714,
0.));
#216936=CARTESIAN_POINT('Ctrl Pts',(22.5473734368086,-4.23461338456714,
12.));
#216937=CARTESIAN_POINT('Ctrl Pts',(22.559951016643,-4.23951550052527,0.));
#216938=CARTESIAN_POINT('Ctrl Pts',(22.559951016643,-4.23951550052527,12.));
#216939=CARTESIAN_POINT('Ctrl Pts',(22.5726687049922,-4.2445187940486,0.));
#216940=CARTESIAN_POINT('Ctrl Pts',(22.5726687049922,-4.2445187940486,12.));
#216941=CARTESIAN_POINT('Ctrl Pts',(22.5855242662479,-4.24962331444186,
0.));
#216942=CARTESIAN_POINT('Ctrl Pts',(22.5855242662479,-4.24962331444186,
12.));
#216943=CARTESIAN_POINT('Ctrl Pts',(22.5985155158637,-4.25482910755486,
0.));
#216944=CARTESIAN_POINT('Ctrl Pts',(22.5985155158637,-4.25482910755486,
12.));
#216945=CARTESIAN_POINT('Ctrl Pts',(22.611640318482,-4.26013621588304,0.));
#216946=CARTESIAN_POINT('Ctrl Pts',(22.611640318482,-4.26013621588304,12.));
#216947=CARTESIAN_POINT('Ctrl Pts',(22.6248965859975,-4.26554467865572,
0.));
#216948=CARTESIAN_POINT('Ctrl Pts',(22.6248965859975,-4.26554467865572,
12.));
#216949=CARTESIAN_POINT('Ctrl Pts',(22.6382822758171,-4.27105453193,0.));
#216950=CARTESIAN_POINT('Ctrl Pts',(22.6382822758171,-4.27105453193,12.));
#216951=CARTESIAN_POINT('Ctrl Pts',(22.6517953893303,-4.27666580869118,
0.));
#216952=CARTESIAN_POINT('Ctrl Pts',(22.6517953893303,-4.27666580869118,
12.));
#216953=CARTESIAN_POINT('Ctrl Pts',(22.665433970311,-4.2823785389406,0.));
#216954=CARTESIAN_POINT('Ctrl Pts',(22.665433970311,-4.2823785389406,12.));
#216955=CARTESIAN_POINT('Ctrl Pts',(22.6791961033536,-4.28819274977767,
0.));
#216956=CARTESIAN_POINT('Ctrl Pts',(22.6791961033536,-4.28819274977767,
12.));
#216957=CARTESIAN_POINT('Ctrl Pts',(22.6930799122545,-4.29410846547062,
0.));
#216958=CARTESIAN_POINT('Ctrl Pts',(22.6930799122545,-4.29410846547062,
12.));
#216959=CARTESIAN_POINT('Ctrl Pts',(22.707083558756,-4.30012570754067,0.));
#216960=CARTESIAN_POINT('Ctrl Pts',(22.707083558756,-4.30012570754067,12.));
#216961=CARTESIAN_POINT('Ctrl Pts',(22.7212052413384,-4.30624449484075,
0.));
#216962=CARTESIAN_POINT('Ctrl Pts',(22.7212052413384,-4.30624449484075,
12.));
#216963=CARTESIAN_POINT('Ctrl Pts',(22.7354431939926,-4.31246484362551,
0.));
#216964=CARTESIAN_POINT('Ctrl Pts',(22.7354431939926,-4.31246484362551,
12.));
#216965=CARTESIAN_POINT('Ctrl Pts',(22.7497956849852,-4.31878676761231,
0.));
#216966=CARTESIAN_POINT('Ctrl Pts',(22.7497956849852,-4.31878676761231,
12.));
#216967=CARTESIAN_POINT('Ctrl Pts',(22.764261015648,-4.32521027803748,0.));
#216968=CARTESIAN_POINT('Ctrl Pts',(22.764261015648,-4.32521027803748,12.));
#216969=CARTESIAN_POINT('Ctrl Pts',(22.7788375194081,-4.33173538373183,
0.));
#216970=CARTESIAN_POINT('Ctrl Pts',(22.7788375194081,-4.33173538373183,
12.));
#216971=CARTESIAN_POINT('Ctrl Pts',(22.7935235607807,-4.33836209118444,
0.));
#216972=CARTESIAN_POINT('Ctrl Pts',(22.7935235607807,-4.33836209118444,
12.));
#216973=CARTESIAN_POINT('Ctrl Pts',(22.808317534379,-4.34509040460066,0.));
#216974=CARTESIAN_POINT('Ctrl Pts',(22.808317534379,-4.34509040460066,12.));
#216975=CARTESIAN_POINT('Ctrl Pts',(22.8232178638873,-4.35192032594802,
0.));
#216976=CARTESIAN_POINT('Ctrl Pts',(22.8232178638873,-4.35192032594802,
12.));
#216977=CARTESIAN_POINT('Ctrl Pts',(22.838223001118,-4.3588518550056,0.));
#216978=CARTESIAN_POINT('Ctrl Pts',(22.838223001118,-4.3588518550056,12.));
#216979=CARTESIAN_POINT('Ctrl Pts',(22.8533314252419,-4.36588498943011,
0.));
#216980=CARTESIAN_POINT('Ctrl Pts',(22.8533314252419,-4.36588498943011,
12.));
#216981=CARTESIAN_POINT('Ctrl Pts',(22.8685416419725,-4.37301972480753,
0.));
#216982=CARTESIAN_POINT('Ctrl Pts',(22.8685416419725,-4.37301972480753,
12.));
#216983=CARTESIAN_POINT('Ctrl Pts',(22.8838521827702,-4.38025605470091,
0.));
#216984=CARTESIAN_POINT('Ctrl Pts',(22.8838521827702,-4.38025605470091,
12.));
#216985=CARTESIAN_POINT('Ctrl Pts',(22.8992616040108,-4.38759397068393,
0.));
#216986=CARTESIAN_POINT('Ctrl Pts',(22.8992616040108,-4.38759397068393,
12.));
#216987=CARTESIAN_POINT('Ctrl Pts',(22.9147684862425,-4.39503346238455,
0.));
#216988=CARTESIAN_POINT('Ctrl Pts',(22.9147684862425,-4.39503346238455,
12.));
#216989=CARTESIAN_POINT('Ctrl Pts',(22.9303714335549,-4.40257451754309,
0.));
#216990=CARTESIAN_POINT('Ctrl Pts',(22.9303714335549,-4.40257451754309,
12.));
#216991=CARTESIAN_POINT('Ctrl Pts',(22.9460690729092,-4.41021712205549,
0.));
#216992=CARTESIAN_POINT('Ctrl Pts',(22.9460690729092,-4.41021712205549,
12.));
#216993=CARTESIAN_POINT('Ctrl Pts',(22.9618600534866,-4.41796126001311,
0.));
#216994=CARTESIAN_POINT('Ctrl Pts',(22.9618600534866,-4.41796126001311,
12.));
#216995=CARTESIAN_POINT('Ctrl Pts',(22.9777430460021,-4.42580691372772,
0.));
#216996=CARTESIAN_POINT('Ctrl Pts',(22.9777430460021,-4.42580691372772,
12.));
#216997=CARTESIAN_POINT('Ctrl Pts',(22.9937167421009,-4.43375406376906,
0.));
#216998=CARTESIAN_POINT('Ctrl Pts',(22.9937167421009,-4.43375406376906,
12.));
#216999=CARTESIAN_POINT('Ctrl Pts',(23.0097798538399,-4.44180268901667,
0.));
#217000=CARTESIAN_POINT('Ctrl Pts',(23.0097798538399,-4.44180268901667,
12.));
#217001=CARTESIAN_POINT('Ctrl Pts',(23.0259311131395,-4.44995276669699,
0.));
#217002=CARTESIAN_POINT('Ctrl Pts',(23.0259311131395,-4.44995276669699,
12.));
#217003=CARTESIAN_POINT('Ctrl Pts',(23.0421692712466,-4.45820427241678,
0.));
#217004=CARTESIAN_POINT('Ctrl Pts',(23.0421692712466,-4.45820427241678,
12.));
#217005=CARTESIAN_POINT('Ctrl Pts',(23.0584930981723,-4.46655718018206,
0.));
#217006=CARTESIAN_POINT('Ctrl Pts',(23.0584930981723,-4.46655718018206,
12.));
#217007=CARTESIAN_POINT('Ctrl Pts',(23.0749013821867,-4.47501146242822,
0.));
#217008=CARTESIAN_POINT('Ctrl Pts',(23.0749013821867,-4.47501146242822,
12.));
#217009=CARTESIAN_POINT('Ctrl Pts',(23.0913929293909,-4.48356709006757,
0.));
#217010=CARTESIAN_POINT('Ctrl Pts',(23.0913929293909,-4.48356709006757,
12.));
#217011=CARTESIAN_POINT('Ctrl Pts',(23.1079665632629,-4.49222403252202,
0.));
#217012=CARTESIAN_POINT('Ctrl Pts',(23.1079665632629,-4.49222403252202,
12.));
#217013=CARTESIAN_POINT('Ctrl Pts',(23.1246211242117,-4.5009822577518,0.));
#217014=CARTESIAN_POINT('Ctrl Pts',(23.1246211242117,-4.5009822577518,12.));
#217015=CARTESIAN_POINT('Ctrl Pts',(23.1413554691136,-4.50984173227088,
0.));
#217016=CARTESIAN_POINT('Ctrl Pts',(23.1413554691136,-4.50984173227088,
12.));
#217017=CARTESIAN_POINT('Ctrl Pts',(23.1581684708778,-4.51880242116786,
0.));
#217018=CARTESIAN_POINT('Ctrl Pts',(23.1581684708778,-4.51880242116786,
12.));
#217019=CARTESIAN_POINT('Ctrl Pts',(23.1750590180923,-4.52786428815049,
0.));
#217020=CARTESIAN_POINT('Ctrl Pts',(23.1750590180923,-4.52786428815049,
12.));
#217021=CARTESIAN_POINT('Ctrl Pts',(23.1920260146474,-4.53702729557586,
0.));
#217022=CARTESIAN_POINT('Ctrl Pts',(23.1920260146474,-4.53702729557586,
12.));
#217023=CARTESIAN_POINT('Ctrl Pts',(23.2090683793627,-4.54629140447543,
0.));
#217024=CARTESIAN_POINT('Ctrl Pts',(23.2090683793627,-4.54629140447543,
12.));
#217025=CARTESIAN_POINT('Ctrl Pts',(23.2261850456054,-4.55565657456957,
0.));
#217026=CARTESIAN_POINT('Ctrl Pts',(23.2261850456054,-4.55565657456957,
12.));
#217027=CARTESIAN_POINT('Ctrl Pts',(23.2433749609117,-4.56512276427812,
0.));
#217028=CARTESIAN_POINT('Ctrl Pts',(23.2433749609117,-4.56512276427812,
12.));
#217029=CARTESIAN_POINT('Ctrl Pts',(23.2606370866853,-4.57468993076071,
0.));
#217030=CARTESIAN_POINT('Ctrl Pts',(23.2606370866853,-4.57468993076071,
12.));
#217031=CARTESIAN_POINT('Ctrl Pts',(23.2779703978868,-4.58435802994675,
0.));
#217032=CARTESIAN_POINT('Ctrl Pts',(23.2779703978868,-4.58435802994675,
12.));
#217033=CARTESIAN_POINT('Ctrl Pts',(23.295373882719,-4.59412701655751,0.));
#217034=CARTESIAN_POINT('Ctrl Pts',(23.295373882719,-4.59412701655751,12.));
#217035=CARTESIAN_POINT('Ctrl Pts',(23.3128465423119,-4.60399684412176,
0.));
#217036=CARTESIAN_POINT('Ctrl Pts',(23.3128465423119,-4.60399684412176,
12.));
#217037=CARTESIAN_POINT('Ctrl Pts',(23.3303873903947,-4.6139674649785,0.));
#217038=CARTESIAN_POINT('Ctrl Pts',(23.3303873903947,-4.6139674649785,12.));
#217039=CARTESIAN_POINT('Ctrl Pts',(23.3479954530281,-4.62403883030825,
0.));
#217040=CARTESIAN_POINT('Ctrl Pts',(23.3479954530281,-4.62403883030825,
12.));
#217041=CARTESIAN_POINT('Ctrl Pts',(23.3656697683496,-4.63421089016556,
0.));
#217042=CARTESIAN_POINT('Ctrl Pts',(23.3656697683496,-4.63421089016556,
12.));
#217043=CARTESIAN_POINT('Ctrl Pts',(23.383409386307,-4.64448359349936,0.));
#217044=CARTESIAN_POINT('Ctrl Pts',(23.383409386307,-4.64448359349936,12.));
#217045=CARTESIAN_POINT('Ctrl Pts',(23.4012133683957,-4.65485688816923,
0.));
#217046=CARTESIAN_POINT('Ctrl Pts',(23.4012133683957,-4.65485688816923,
12.));
#217047=CARTESIAN_POINT('Ctrl Pts',(23.4190807873798,-4.66533072094664,
0.));
#217048=CARTESIAN_POINT('Ctrl Pts',(23.4190807873798,-4.66533072094664,
12.));
#217049=CARTESIAN_POINT('Ctrl Pts',(23.4370107270444,-4.67590503753051,
0.));
#217050=CARTESIAN_POINT('Ctrl Pts',(23.4370107270444,-4.67590503753051,
12.));
#217051=CARTESIAN_POINT('Ctrl Pts',(23.4550022819852,-4.68657978258298,
0.));
#217052=CARTESIAN_POINT('Ctrl Pts',(23.4550022819852,-4.68657978258298,
12.));
#217053=CARTESIAN_POINT('Ctrl Pts',(23.4730545573849,-4.69735489975024,
0.));
#217054=CARTESIAN_POINT('Ctrl Pts',(23.4730545573849,-4.69735489975024,
12.));
#217055=CARTESIAN_POINT('Ctrl Pts',(23.491166668789,-4.70823033167821,0.));
#217056=CARTESIAN_POINT('Ctrl Pts',(23.491166668789,-4.70823033167821,12.));
#217057=CARTESIAN_POINT('Ctrl Pts',(23.5093377418784,-4.71920602001905,
0.));
#217058=CARTESIAN_POINT('Ctrl Pts',(23.5093377418784,-4.71920602001905,
12.));
#217059=CARTESIAN_POINT('Ctrl Pts',(23.5275669122378,-4.73028190543032,
0.));
#217060=CARTESIAN_POINT('Ctrl Pts',(23.5275669122378,-4.73028190543032,
12.));
#217061=CARTESIAN_POINT('Ctrl Pts',(23.5458533251715,-4.74145792760699,
0.));
#217062=CARTESIAN_POINT('Ctrl Pts',(23.5458533251715,-4.74145792760699,
12.));
#217063=CARTESIAN_POINT('Ctrl Pts',(23.564196135517,-4.75273402530616,0.));
#217064=CARTESIAN_POINT('Ctrl Pts',(23.564196135517,-4.75273402530616,12.));
#217065=CARTESIAN_POINT('Ctrl Pts',(23.5825945074535,-4.76411013636252,
0.));
#217066=CARTESIAN_POINT('Ctrl Pts',(23.5825945074535,-4.76411013636252,
12.));
#217067=CARTESIAN_POINT('Ctrl Pts',(23.6010476143099,-4.77558619769876,
0.));
#217068=CARTESIAN_POINT('Ctrl Pts',(23.6010476143099,-4.77558619769876,
12.));
#217069=CARTESIAN_POINT('Ctrl Pts',(23.6195546383625,-4.78716214532105,
0.));
#217070=CARTESIAN_POINT('Ctrl Pts',(23.6195546383625,-4.78716214532105,
12.));
#217071=CARTESIAN_POINT('Ctrl Pts',(23.6381147706581,-4.79883791433231,
0.));
#217072=CARTESIAN_POINT('Ctrl Pts',(23.6381147706581,-4.79883791433231,
12.));
#217073=CARTESIAN_POINT('Ctrl Pts',(23.6567272108631,-4.81061343896443,
0.));
#217074=CARTESIAN_POINT('Ctrl Pts',(23.6567272108631,-4.81061343896443,
12.));
#217075=CARTESIAN_POINT('Ctrl Pts',(23.6753911671023,-4.82248865259571,
0.));
#217076=CARTESIAN_POINT('Ctrl Pts',(23.6753911671023,-4.82248865259571,
12.));
#217077=CARTESIAN_POINT('Ctrl Pts',(23.6941058557971,-4.83446348776268,
0.));
#217078=CARTESIAN_POINT('Ctrl Pts',(23.6941058557971,-4.83446348776268,
12.));
#217079=CARTESIAN_POINT('Ctrl Pts',(23.7128705015014,-4.84653787616424,
0.));
#217080=CARTESIAN_POINT('Ctrl Pts',(23.7128705015014,-4.84653787616424,
12.));
#217081=CARTESIAN_POINT('Ctrl Pts',(23.7316843367308,-4.85871174865493,
0.));
#217082=CARTESIAN_POINT('Ctrl Pts',(23.7316843367308,-4.85871174865493,
12.));
#217083=CARTESIAN_POINT('Ctrl Pts',(23.7505466018239,-4.87098503527144,
0.));
#217084=CARTESIAN_POINT('Ctrl Pts',(23.7505466018239,-4.87098503527144,
12.));
#217085=CARTESIAN_POINT('Ctrl Pts',(23.7694565448044,-4.88335766525566,
0.));
#217086=CARTESIAN_POINT('Ctrl Pts',(23.7694565448044,-4.88335766525566,
12.));
#217087=CARTESIAN_POINT('Ctrl Pts',(23.7884134212381,-4.89582956706772,
0.));
#217088=CARTESIAN_POINT('Ctrl Pts',(23.7884134212381,-4.89582956706772,
12.));
#217089=CARTESIAN_POINT('Ctrl Pts',(23.8074164940897,-4.90840066839348,
0.));
#217090=CARTESIAN_POINT('Ctrl Pts',(23.8074164940897,-4.90840066839348,
12.));
#217091=CARTESIAN_POINT('Ctrl Pts',(23.8264650335721,-4.92107089613978,
0.));
#217092=CARTESIAN_POINT('Ctrl Pts',(23.8264650335721,-4.92107089613978,
12.));
#217093=CARTESIAN_POINT('Ctrl Pts',(23.8455583170062,-4.93384017643443,
0.));
#217094=CARTESIAN_POINT('Ctrl Pts',(23.8455583170062,-4.93384017643443,
12.));
#217095=CARTESIAN_POINT('Ctrl Pts',(23.8646956287172,-4.94670843465869,
0.));
#217096=CARTESIAN_POINT('Ctrl Pts',(23.8646956287172,-4.94670843465869,
12.));
#217097=CARTESIAN_POINT('Ctrl Pts',(23.883876259922,-4.95967559546566,0.));
#217098=CARTESIAN_POINT('Ctrl Pts',(23.883876259922,-4.95967559546566,12.));
#217099=CARTESIAN_POINT('Ctrl Pts',(23.9030995086164,-4.9727415827923,0.));
#217100=CARTESIAN_POINT('Ctrl Pts',(23.9030995086164,-4.9727415827923,12.));
#217101=CARTESIAN_POINT('Ctrl Pts',(23.9223646794591,-4.98590631986534,
0.));
#217102=CARTESIAN_POINT('Ctrl Pts',(23.9223646794591,-4.98590631986534,
12.));
#217103=CARTESIAN_POINT('Ctrl Pts',(23.9416710836528,-4.9991697291931,0.));
#217104=CARTESIAN_POINT('Ctrl Pts',(23.9416710836528,-4.9991697291931,12.));
#217105=CARTESIAN_POINT('Ctrl Pts',(23.9610180388271,-5.01253173257459,
0.));
#217106=CARTESIAN_POINT('Ctrl Pts',(23.9610180388271,-5.01253173257459,
12.));
#217107=CARTESIAN_POINT('Ctrl Pts',(23.9804048689228,-5.02599225112462,
0.));
#217108=CARTESIAN_POINT('Ctrl Pts',(23.9804048689228,-5.02599225112462,
12.));
#217109=CARTESIAN_POINT('Ctrl Pts',(23.9998309040747,-5.03955120528528,
0.));
#217110=CARTESIAN_POINT('Ctrl Pts',(23.9998309040747,-5.03955120528528,
12.));
#217111=CARTESIAN_POINT('Ctrl Pts',(24.0192954804896,-5.05320851483069,
0.));
#217112=CARTESIAN_POINT('Ctrl Pts',(24.0192954804896,-5.05320851483069,
12.));
#217113=CARTESIAN_POINT('Ctrl Pts',(24.0387979403268,-5.0669640988664,0.));
#217114=CARTESIAN_POINT('Ctrl Pts',(24.0387979403268,-5.0669640988664,12.));
#217115=CARTESIAN_POINT('Ctrl Pts',(24.0583376315636,-5.08081787581271,
0.));
#217116=CARTESIAN_POINT('Ctrl Pts',(24.0583376315636,-5.08081787581271,
12.));
#217117=CARTESIAN_POINT('Ctrl Pts',(24.0779139079264,-5.09476976342618,
0.));
#217118=CARTESIAN_POINT('Ctrl Pts',(24.0779139079264,-5.09476976342618,
12.));
#217119=CARTESIAN_POINT('Ctrl Pts',(24.0975261288444,-5.10881967883126,
0.));
#217120=CARTESIAN_POINT('Ctrl Pts',(24.0975261288444,-5.10881967883126,
12.));
#217121=CARTESIAN_POINT('Ctrl Pts',(24.117173659394,-5.12296753853858,0.));
#217122=CARTESIAN_POINT('Ctrl Pts',(24.117173659394,-5.12296753853858,12.));
#217123=CARTESIAN_POINT('Ctrl Pts',(24.1368558702443,-5.13721325845746,
0.));
#217124=CARTESIAN_POINT('Ctrl Pts',(24.1368558702443,-5.13721325845746,
12.));
#217125=CARTESIAN_POINT('Ctrl Pts',(24.1565721375971,-5.1515567539008,0.));
#217126=CARTESIAN_POINT('Ctrl Pts',(24.1565721375971,-5.1515567539008,12.));
#217127=CARTESIAN_POINT('Ctrl Pts',(24.1763218431344,-5.16599793957987,
0.));
#217128=CARTESIAN_POINT('Ctrl Pts',(24.1763218431344,-5.16599793957987,
12.));
#217129=CARTESIAN_POINT('Ctrl Pts',(24.1961043738755,-5.180536729614,0.));
#217130=CARTESIAN_POINT('Ctrl Pts',(24.1961043738755,-5.180536729614,12.));
#217131=CARTESIAN_POINT('Ctrl Pts',(24.2159191220171,-5.19517303753648,
0.));
#217132=CARTESIAN_POINT('Ctrl Pts',(24.2159191220171,-5.19517303753648,
12.));
#217133=CARTESIAN_POINT('Ctrl Pts',(24.2357654847766,-5.20990677629177,
0.));
#217134=CARTESIAN_POINT('Ctrl Pts',(24.2357654847766,-5.20990677629177,
12.));
#217135=CARTESIAN_POINT('Ctrl Pts',(24.2556428642294,-5.22473785822443,
0.));
#217136=CARTESIAN_POINT('Ctrl Pts',(24.2556428642294,-5.22473785822443,
12.));
#217137=CARTESIAN_POINT('Ctrl Pts',(24.2755506671525,-5.2396661950629,0.));
#217138=CARTESIAN_POINT('Ctrl Pts',(24.2755506671525,-5.2396661950629,12.));
#217139=CARTESIAN_POINT('Ctrl Pts',(24.2954883048447,-5.25469169788858,
0.));
#217140=CARTESIAN_POINT('Ctrl Pts',(24.2954883048447,-5.25469169788858,
12.));
#217141=CARTESIAN_POINT('Ctrl Pts',(24.3154551932221,-5.269814277188,0.));
#217142=CARTESIAN_POINT('Ctrl Pts',(24.3154551932221,-5.269814277188,12.));
#217143=CARTESIAN_POINT('Ctrl Pts',(24.3354507529414,-5.28503384290649,
0.));
#217144=CARTESIAN_POINT('Ctrl Pts',(24.3354507529414,-5.28503384290649,
12.));
#217145=CARTESIAN_POINT('Ctrl Pts',(24.3554744095075,-5.30035030449065,
0.));
#217146=CARTESIAN_POINT('Ctrl Pts',(24.3554744095075,-5.30035030449065,
12.));
#217147=CARTESIAN_POINT('Ctrl Pts',(24.3755255933917,-5.31576357092527,
0.));
#217148=CARTESIAN_POINT('Ctrl Pts',(24.3755255933917,-5.31576357092527,
12.));
#217149=CARTESIAN_POINT('Ctrl Pts',(24.3956037401293,-5.33127355076035,
0.));
#217150=CARTESIAN_POINT('Ctrl Pts',(24.3956037401293,-5.33127355076035,
12.));
#217151=CARTESIAN_POINT('Ctrl Pts',(24.4157082904614,-5.34688015213538,
0.));
#217152=CARTESIAN_POINT('Ctrl Pts',(24.4157082904614,-5.34688015213538,
12.));
#217153=CARTESIAN_POINT('Ctrl Pts',(24.435838689915,-5.36258328273628,0.));
#217154=CARTESIAN_POINT('Ctrl Pts',(24.435838689915,-5.36258328273628,12.));
#217155=CARTESIAN_POINT('Ctrl Pts',(24.4559943883157,-5.37838284973696,
0.));
#217156=CARTESIAN_POINT('Ctrl Pts',(24.4559943883157,-5.37838284973696,
12.));
#217157=CARTESIAN_POINT('Ctrl Pts',(24.4761748393321,-5.39427875973825,
0.));
#217158=CARTESIAN_POINT('Ctrl Pts',(24.4761748393321,-5.39427875973825,
12.));
#217159=CARTESIAN_POINT('Ctrl Pts',(24.496379499983,-5.41027091869242,0.));
#217160=CARTESIAN_POINT('Ctrl Pts',(24.496379499983,-5.41027091869242,12.));
#217161=CARTESIAN_POINT('Ctrl Pts',(24.5166078302108,-5.4263592318342,0.));
#217162=CARTESIAN_POINT('Ctrl Pts',(24.5166078302108,-5.4263592318342,12.));
#217163=CARTESIAN_POINT('Ctrl Pts',(24.5368592922863,-5.44254360356881,
0.));
#217164=CARTESIAN_POINT('Ctrl Pts',(24.5368592922863,-5.44254360356881,
12.));
#217165=CARTESIAN_POINT('Ctrl Pts',(24.5571333514842,-5.45882393762263,
0.));
#217166=CARTESIAN_POINT('Ctrl Pts',(24.5571333514842,-5.45882393762263,
12.));
#217167=CARTESIAN_POINT('Ctrl Pts',(24.5774294770329,-5.4752001372442,0.));
#217168=CARTESIAN_POINT('Ctrl Pts',(24.5774294770329,-5.4752001372442,12.));
#217169=CARTESIAN_POINT('Ctrl Pts',(24.5977471429364,-5.49167210537248,
0.));
#217170=CARTESIAN_POINT('Ctrl Pts',(24.5977471429364,-5.49167210537248,
12.));
#217171=CARTESIAN_POINT('Ctrl Pts',(24.6180858289179,-5.50823974481963,
0.));
#217172=CARTESIAN_POINT('Ctrl Pts',(24.6180858289179,-5.50823974481963,
12.));
#217173=CARTESIAN_POINT('Ctrl Pts',(24.6384450211467,-5.52490295840993,
0.));
#217174=CARTESIAN_POINT('Ctrl Pts',(24.6384450211467,-5.52490295840993,
12.));
#217175=CARTESIAN_POINT('Ctrl Pts',(24.6588242134738,-5.54166164919584,
0.));
#217176=CARTESIAN_POINT('Ctrl Pts',(24.6588242134738,-5.54166164919584,
12.));
#217177=CARTESIAN_POINT('Ctrl Pts',(24.6792229061794,-5.55851572025377,
0.));
#217178=CARTESIAN_POINT('Ctrl Pts',(24.6792229061794,-5.55851572025377,
12.));
#217179=CARTESIAN_POINT('Ctrl Pts',(24.6996406035517,-5.57546507427756,
0.));
#217180=CARTESIAN_POINT('Ctrl Pts',(24.6996406035517,-5.57546507427756,
12.));
#217181=CARTESIAN_POINT('Ctrl Pts',(24.7200768119088,-5.59250961323988,
0.));
#217182=CARTESIAN_POINT('Ctrl Pts',(24.7200768119088,-5.59250961323988,
12.));
#217183=CARTESIAN_POINT('Ctrl Pts',(24.7405310372739,-5.60964923798492,
0.));
#217184=CARTESIAN_POINT('Ctrl Pts',(24.7405310372739,-5.60964923798492,
12.));
#217185=CARTESIAN_POINT('Ctrl Pts',(24.7610027835697,-5.62688384790924,
0.));
#217186=CARTESIAN_POINT('Ctrl Pts',(24.7610027835697,-5.62688384790924,
12.));
#217187=CARTESIAN_POINT('Ctrl Pts',(24.781491549672,-5.64421334042262,0.));
#217188=CARTESIAN_POINT('Ctrl Pts',(24.781491549672,-5.64421334042262,12.));
#217189=CARTESIAN_POINT('Ctrl Pts',(24.8019968304605,-5.66163761114922,
0.));
#217190=CARTESIAN_POINT('Ctrl Pts',(24.8019968304605,-5.66163761114922,
12.));
#217191=CARTESIAN_POINT('Ctrl Pts',(24.8225181223845,-5.67915655496543,
0.));
#217192=CARTESIAN_POINT('Ctrl Pts',(24.8225181223845,-5.67915655496543,
12.));
#217193=CARTESIAN_POINT('Ctrl Pts',(24.8430549277621,-5.69677006679445,
0.));
#217194=CARTESIAN_POINT('Ctrl Pts',(24.8430549277621,-5.69677006679445,
12.));
#217195=CARTESIAN_POINT('Ctrl Pts',(24.8636067597669,-5.71447804252028,
0.));
#217196=CARTESIAN_POINT('Ctrl Pts',(24.8636067597669,-5.71447804252028,
12.));
#217197=CARTESIAN_POINT('Ctrl Pts',(24.884173146722,-5.73228037976928,0.));
#217198=CARTESIAN_POINT('Ctrl Pts',(24.884173146722,-5.73228037976928,12.));
#217199=CARTESIAN_POINT('Ctrl Pts',(24.904753637648,-5.75017697890805,0.));
#217200=CARTESIAN_POINT('Ctrl Pts',(24.904753637648,-5.75017697890805,12.));
#217201=CARTESIAN_POINT('Ctrl Pts',(24.9253478043656,-5.76816774342221,
0.));
#217202=CARTESIAN_POINT('Ctrl Pts',(24.9253478043656,-5.76816774342221,
12.));
#217203=CARTESIAN_POINT('Ctrl Pts',(24.945955229334,-5.78625257775682,0.));
#217204=CARTESIAN_POINT('Ctrl Pts',(24.945955229334,-5.78625257775682,12.));
#217205=CARTESIAN_POINT('Ctrl Pts',(24.9665754954496,-5.80443138549727,
0.));
#217206=CARTESIAN_POINT('Ctrl Pts',(24.9665754954496,-5.80443138549727,
12.));
#217207=CARTESIAN_POINT('Ctrl Pts',(24.9872081752734,-5.822704067442,0.));
#217208=CARTESIAN_POINT('Ctrl Pts',(24.9872081752734,-5.822704067442,12.));
#217209=CARTESIAN_POINT('Ctrl Pts',(25.0078528200564,-5.84107051963072,
0.));
#217210=CARTESIAN_POINT('Ctrl Pts',(25.0078528200564,-5.84107051963072,
12.));
#217211=CARTESIAN_POINT('Ctrl Pts',(25.0285089498899,-5.85953063156827,
0.));
#217212=CARTESIAN_POINT('Ctrl Pts',(25.0285089498899,-5.85953063156827,
12.));
#217213=CARTESIAN_POINT('Ctrl Pts',(25.049176040591,-5.87808428385367,0.));
#217214=CARTESIAN_POINT('Ctrl Pts',(25.049176040591,-5.87808428385367,12.));
#217215=CARTESIAN_POINT('Ctrl Pts',(25.0698535426514,-5.89673135155515,
0.));
#217216=CARTESIAN_POINT('Ctrl Pts',(25.0698535426514,-5.89673135155515,
12.));
#217217=CARTESIAN_POINT('Ctrl Pts',(25.0905409050773,-5.91547170844448,
0.));
#217218=CARTESIAN_POINT('Ctrl Pts',(25.0905409050773,-5.91547170844448,
12.));
#217219=CARTESIAN_POINT('Ctrl Pts',(25.1112375971106,-5.93430523086836,
0.));
#217220=CARTESIAN_POINT('Ctrl Pts',(25.1112375971106,-5.93430523086836,
12.));
#217221=CARTESIAN_POINT('Ctrl Pts',(25.1319431317237,-5.95323180187379,
0.));
#217222=CARTESIAN_POINT('Ctrl Pts',(25.1319431317237,-5.95323180187379,
12.));
#217223=CARTESIAN_POINT('Ctrl Pts',(25.1526570863092,-5.97225131495618,
0.));
#217224=CARTESIAN_POINT('Ctrl Pts',(25.1526570863092,-5.97225131495618,
12.));
#217225=CARTESIAN_POINT('Ctrl Pts',(25.1733791296259,-5.99136367859755,
0.));
#217226=CARTESIAN_POINT('Ctrl Pts',(25.1733791296259,-5.99136367859755,
12.));
#217227=CARTESIAN_POINT('Ctrl Pts',(25.1941090269819,-6.01056881804614,
0.));
#217228=CARTESIAN_POINT('Ctrl Pts',(25.1941090269819,-6.01056881804614,
12.));
#217229=CARTESIAN_POINT('Ctrl Pts',(25.21484662016,-6.02986667389998,0.));
#217230=CARTESIAN_POINT('Ctrl Pts',(25.21484662016,-6.02986667389998,12.));
#217231=CARTESIAN_POINT('Ctrl Pts',(25.2355918139032,-6.04925720151219,
0.));
#217232=CARTESIAN_POINT('Ctrl Pts',(25.2355918139032,-6.04925720151219,
12.));
#217233=CARTESIAN_POINT('Ctrl Pts',(25.2521940105705,-6.06484373634547,
0.));
#217234=CARTESIAN_POINT('Ctrl Pts',(25.2521940105705,-6.06484373634547,
12.));
#217235=CARTESIAN_POINT('Ctrl Pts',(25.2646490489922,-6.07657531787491,
0.));
#217236=CARTESIAN_POINT('Ctrl Pts',(25.2646490489922,-6.07657531787491,
12.));
#217237=CARTESIAN_POINT('Ctrl Pts',(25.2729539149517,-6.08441489609794,
0.));
#217238=CARTESIAN_POINT('Ctrl Pts',(25.2729539149517,-6.08441489609794,
12.));
#217239=CARTESIAN_POINT('Ctrl Pts',(25.2771067246846,-6.088339316177,0.));
#217240=CARTESIAN_POINT('Ctrl Pts',(25.2771067246846,-6.088339316177,12.));
#217241=CARTESIAN_POINT('',(25.2771067246846,-6.088339316177,0.));
#217242=CARTESIAN_POINT('Ctrl Pts',(22.1738711152697,-4.11585220600463,
0.));
#217243=CARTESIAN_POINT('Ctrl Pts',(22.173877682324,-4.11585194677443,0.));
#217244=CARTESIAN_POINT('Ctrl Pts',(22.1739341411687,-4.11586035878288,
0.));
#217245=CARTESIAN_POINT('Ctrl Pts',(22.1741488021234,-4.11589976826168,
0.));
#217246=CARTESIAN_POINT('Ctrl Pts',(22.1746949858775,-4.11600589882846,
0.));
#217247=CARTESIAN_POINT('Ctrl Pts',(22.1758088296598,-4.1162279721707,0.));
#217248=CARTESIAN_POINT('Ctrl Pts',(22.177347426894,-4.11653973150519,0.));
#217249=CARTESIAN_POINT('Ctrl Pts',(22.179297473024,-4.11694173195005,0.));
#217250=CARTESIAN_POINT('Ctrl Pts',(22.1816414985788,-4.11743469691757,
0.));
#217251=CARTESIAN_POINT('Ctrl Pts',(22.1843613164855,-4.11801938107481,
0.));
#217252=CARTESIAN_POINT('Ctrl Pts',(22.1874419861496,-4.11869641271775,
0.));
#217253=CARTESIAN_POINT('Ctrl Pts',(22.1908725908525,-4.11946626228637,
0.));
#217254=CARTESIAN_POINT('Ctrl Pts',(22.1946440958098,-4.12032932637738,
0.));
#217255=CARTESIAN_POINT('Ctrl Pts',(22.1987479618246,-4.12128598183523,
0.));
#217256=CARTESIAN_POINT('Ctrl Pts',(22.2031746532106,-4.12233664408228,
0.));
#217257=CARTESIAN_POINT('Ctrl Pts',(22.2079143941719,-4.12348173702024,
0.));
#217258=CARTESIAN_POINT('Ctrl Pts',(22.2129576146671,-4.12472167516608,
0.));
#217259=CARTESIAN_POINT('Ctrl Pts',(22.2182956401341,-4.12605683613308,
0.));
#217260=CARTESIAN_POINT('Ctrl Pts',(22.2239207458781,-4.12748755830105,
0.));
#217261=CARTESIAN_POINT('Ctrl Pts',(22.2298258043947,-4.1290141546338,0.));
#217262=CARTESIAN_POINT('Ctrl Pts',(22.2360040565533,-4.13063692157499,
0.));
#217263=CARTESIAN_POINT('Ctrl Pts',(22.2424488153523,-4.13235615060161,
0.));
#217264=CARTESIAN_POINT('Ctrl Pts',(22.249153531779,-4.13417212558811,0.));
#217265=CARTESIAN_POINT('Ctrl Pts',(22.2561118708421,-4.13608511977227,
0.));
#217266=CARTESIAN_POINT('Ctrl Pts',(22.2633177913972,-4.13809539255423,
0.));
#217267=CARTESIAN_POINT('Ctrl Pts',(22.2707656042457,-4.14020318715992,
0.));
#217268=CARTESIAN_POINT('Ctrl Pts',(22.2784499072027,-4.14240873321985,
0.));
#217269=CARTESIAN_POINT('Ctrl Pts',(22.2863655389166,-4.14471224859297,
0.));
#217270=CARTESIAN_POINT('Ctrl Pts',(22.2945075198467,-4.14711394168557,
0.));
#217271=CARTESIAN_POINT('Ctrl Pts',(22.3028710166933,-4.14961401285523,
0.));
#217272=CARTESIAN_POINT('Ctrl Pts',(22.3114513545185,-4.15221265396991,
0.));
#217273=CARTESIAN_POINT('Ctrl Pts',(22.3202440186979,-4.15491004835282,
0.));
#217274=CARTESIAN_POINT('Ctrl Pts',(22.3292446628959,-4.15770637047891,
0.));
#217275=CARTESIAN_POINT('Ctrl Pts',(22.3384491078602,-4.16060178604165,
0.));
#217276=CARTESIAN_POINT('Ctrl Pts',(22.3478533253889,-4.16359645263189,
0.));
#217277=CARTESIAN_POINT('Ctrl Pts',(22.3574534257396,-4.16669052026601,
0.));
#217278=CARTESIAN_POINT('Ctrl Pts',(22.3672456427599,-4.16988413199458,
0.));
#217279=CARTESIAN_POINT('Ctrl Pts',(22.3772263228617,-4.17317742436146,
0.));
#217280=CARTESIAN_POINT('Ctrl Pts',(22.3873919231334,-4.17657052752826,
0.));
#217281=CARTESIAN_POINT('Ctrl Pts',(22.3977390078075,-4.18006356544883,
0.));
#217282=CARTESIAN_POINT('Ctrl Pts',(22.4082642454453,-4.18365665600852,
0.));
#217283=CARTESIAN_POINT('Ctrl Pts',(22.4189644056115,-4.18734991117722,
0.));
#217284=CARTESIAN_POINT('Ctrl Pts',(22.4298363535421,-4.19114343726943,
0.));
#217285=CARTESIAN_POINT('Ctrl Pts',(22.4408770448917,-4.19503733518862,
0.));
#217286=CARTESIAN_POINT('Ctrl Pts',(22.4520835205419,-4.19903170066356,
0.));
#217287=CARTESIAN_POINT('Ctrl Pts',(22.4634529011433,-4.20312662448172,
0.));
#217288=CARTESIAN_POINT('Ctrl Pts',(22.4749823839915,-4.20732219265649,
0.));
#217289=CARTESIAN_POINT('Ctrl Pts',(22.4866692403147,-4.21161848657429,
0.));
#217290=CARTESIAN_POINT('Ctrl Pts',(22.4985108124229,-4.21601558313909,
0.));
#217291=CARTESIAN_POINT('Ctrl Pts',(22.5105045108882,-4.22051355490198,
0.));
#217292=CARTESIAN_POINT('Ctrl Pts',(22.5226478117885,-4.22511247020041,
0.));
#217293=CARTESIAN_POINT('Ctrl Pts',(22.5349382540587,-4.22981239330733,
0.));
#217294=CARTESIAN_POINT('Ctrl Pts',(22.5473734368086,-4.23461338456714,
0.));
#217295=CARTESIAN_POINT('Ctrl Pts',(22.559951016643,-4.23951550052527,0.));
#217296=CARTESIAN_POINT('Ctrl Pts',(22.5726687049922,-4.2445187940486,0.));
#217297=CARTESIAN_POINT('Ctrl Pts',(22.5855242662479,-4.24962331444186,
0.));
#217298=CARTESIAN_POINT('Ctrl Pts',(22.5985155158637,-4.25482910755486,
0.));
#217299=CARTESIAN_POINT('Ctrl Pts',(22.611640318482,-4.26013621588304,0.));
#217300=CARTESIAN_POINT('Ctrl Pts',(22.6248965859975,-4.26554467865572,
0.));
#217301=CARTESIAN_POINT('Ctrl Pts',(22.6382822758171,-4.27105453193,0.));
#217302=CARTESIAN_POINT('Ctrl Pts',(22.6517953893303,-4.27666580869118,
0.));
#217303=CARTESIAN_POINT('Ctrl Pts',(22.665433970311,-4.2823785389406,0.));
#217304=CARTESIAN_POINT('Ctrl Pts',(22.6791961033536,-4.28819274977767,
0.));
#217305=CARTESIAN_POINT('Ctrl Pts',(22.6930799122545,-4.29410846547062,
0.));
#217306=CARTESIAN_POINT('Ctrl Pts',(22.707083558756,-4.30012570754067,0.));
#217307=CARTESIAN_POINT('Ctrl Pts',(22.7212052413384,-4.30624449484075,
0.));
#217308=CARTESIAN_POINT('Ctrl Pts',(22.7354431939926,-4.31246484362551,
0.));
#217309=CARTESIAN_POINT('Ctrl Pts',(22.7497956849852,-4.31878676761231,
0.));
#217310=CARTESIAN_POINT('Ctrl Pts',(22.764261015648,-4.32521027803748,0.));
#217311=CARTESIAN_POINT('Ctrl Pts',(22.7788375194081,-4.33173538373183,
0.));
#217312=CARTESIAN_POINT('Ctrl Pts',(22.7935235607807,-4.33836209118444,
0.));
#217313=CARTESIAN_POINT('Ctrl Pts',(22.808317534379,-4.34509040460066,0.));
#217314=CARTESIAN_POINT('Ctrl Pts',(22.8232178638873,-4.35192032594802,
0.));
#217315=CARTESIAN_POINT('Ctrl Pts',(22.838223001118,-4.3588518550056,0.));
#217316=CARTESIAN_POINT('Ctrl Pts',(22.8533314252419,-4.36588498943011,
0.));
#217317=CARTESIAN_POINT('Ctrl Pts',(22.8685416419725,-4.37301972480753,
0.));
#217318=CARTESIAN_POINT('Ctrl Pts',(22.8838521827702,-4.38025605470091,
0.));
#217319=CARTESIAN_POINT('Ctrl Pts',(22.8992616040108,-4.38759397068393,
0.));
#217320=CARTESIAN_POINT('Ctrl Pts',(22.9147684862425,-4.39503346238455,
0.));
#217321=CARTESIAN_POINT('Ctrl Pts',(22.9303714335549,-4.40257451754309,
0.));
#217322=CARTESIAN_POINT('Ctrl Pts',(22.9460690729092,-4.41021712205549,
0.));
#217323=CARTESIAN_POINT('Ctrl Pts',(22.9618600534866,-4.41796126001311,
0.));
#217324=CARTESIAN_POINT('Ctrl Pts',(22.9777430460021,-4.42580691372772,
0.));
#217325=CARTESIAN_POINT('Ctrl Pts',(22.9937167421009,-4.43375406376906,
0.));
#217326=CARTESIAN_POINT('Ctrl Pts',(23.0097798538399,-4.44180268901667,
0.));
#217327=CARTESIAN_POINT('Ctrl Pts',(23.0259311131395,-4.44995276669699,
0.));
#217328=CARTESIAN_POINT('Ctrl Pts',(23.0421692712466,-4.45820427241678,
0.));
#217329=CARTESIAN_POINT('Ctrl Pts',(23.0584930981723,-4.46655718018206,
0.));
#217330=CARTESIAN_POINT('Ctrl Pts',(23.0749013821867,-4.47501146242822,
0.));
#217331=CARTESIAN_POINT('Ctrl Pts',(23.0913929293909,-4.48356709006757,
0.));
#217332=CARTESIAN_POINT('Ctrl Pts',(23.1079665632629,-4.49222403252202,
0.));
#217333=CARTESIAN_POINT('Ctrl Pts',(23.1246211242117,-4.5009822577518,0.));
#217334=CARTESIAN_POINT('Ctrl Pts',(23.1413554691136,-4.50984173227088,
0.));
#217335=CARTESIAN_POINT('Ctrl Pts',(23.1581684708778,-4.51880242116786,
0.));
#217336=CARTESIAN_POINT('Ctrl Pts',(23.1750590180923,-4.52786428815049,
0.));
#217337=CARTESIAN_POINT('Ctrl Pts',(23.1920260146474,-4.53702729557586,
0.));
#217338=CARTESIAN_POINT('Ctrl Pts',(23.2090683793627,-4.54629140447543,
0.));
#217339=CARTESIAN_POINT('Ctrl Pts',(23.2261850456054,-4.55565657456957,
0.));
#217340=CARTESIAN_POINT('Ctrl Pts',(23.2433749609117,-4.56512276427812,
0.));
#217341=CARTESIAN_POINT('Ctrl Pts',(23.2606370866853,-4.57468993076071,
0.));
#217342=CARTESIAN_POINT('Ctrl Pts',(23.2779703978868,-4.58435802994675,
0.));
#217343=CARTESIAN_POINT('Ctrl Pts',(23.295373882719,-4.59412701655751,0.));
#217344=CARTESIAN_POINT('Ctrl Pts',(23.3128465423119,-4.60399684412176,
0.));
#217345=CARTESIAN_POINT('Ctrl Pts',(23.3303873903947,-4.6139674649785,0.));
#217346=CARTESIAN_POINT('Ctrl Pts',(23.3479954530281,-4.62403883030825,
0.));
#217347=CARTESIAN_POINT('Ctrl Pts',(23.3656697683496,-4.63421089016556,
0.));
#217348=CARTESIAN_POINT('Ctrl Pts',(23.383409386307,-4.64448359349936,0.));
#217349=CARTESIAN_POINT('Ctrl Pts',(23.4012133683957,-4.65485688816923,
0.));
#217350=CARTESIAN_POINT('Ctrl Pts',(23.4190807873798,-4.66533072094664,
0.));
#217351=CARTESIAN_POINT('Ctrl Pts',(23.4370107270444,-4.67590503753051,
0.));
#217352=CARTESIAN_POINT('Ctrl Pts',(23.4550022819852,-4.68657978258298,
0.));
#217353=CARTESIAN_POINT('Ctrl Pts',(23.4730545573849,-4.69735489975024,
0.));
#217354=CARTESIAN_POINT('Ctrl Pts',(23.491166668789,-4.70823033167821,0.));
#217355=CARTESIAN_POINT('Ctrl Pts',(23.5093377418784,-4.71920602001905,
0.));
#217356=CARTESIAN_POINT('Ctrl Pts',(23.5275669122378,-4.73028190543032,
0.));
#217357=CARTESIAN_POINT('Ctrl Pts',(23.5458533251715,-4.74145792760699,
0.));
#217358=CARTESIAN_POINT('Ctrl Pts',(23.564196135517,-4.75273402530616,0.));
#217359=CARTESIAN_POINT('Ctrl Pts',(23.5825945074535,-4.76411013636252,
0.));
#217360=CARTESIAN_POINT('Ctrl Pts',(23.6010476143099,-4.77558619769876,
0.));
#217361=CARTESIAN_POINT('Ctrl Pts',(23.6195546383625,-4.78716214532105,
0.));
#217362=CARTESIAN_POINT('Ctrl Pts',(23.6381147706581,-4.79883791433231,
0.));
#217363=CARTESIAN_POINT('Ctrl Pts',(23.6567272108631,-4.81061343896443,
0.));
#217364=CARTESIAN_POINT('Ctrl Pts',(23.6753911671023,-4.82248865259571,
0.));
#217365=CARTESIAN_POINT('Ctrl Pts',(23.6941058557971,-4.83446348776268,
0.));
#217366=CARTESIAN_POINT('Ctrl Pts',(23.7128705015014,-4.84653787616424,
0.));
#217367=CARTESIAN_POINT('Ctrl Pts',(23.7316843367308,-4.85871174865493,
0.));
#217368=CARTESIAN_POINT('Ctrl Pts',(23.7505466018239,-4.87098503527144,
0.));
#217369=CARTESIAN_POINT('Ctrl Pts',(23.7694565448044,-4.88335766525566,
0.));
#217370=CARTESIAN_POINT('Ctrl Pts',(23.7884134212381,-4.89582956706772,
0.));
#217371=CARTESIAN_POINT('Ctrl Pts',(23.8074164940897,-4.90840066839348,
0.));
#217372=CARTESIAN_POINT('Ctrl Pts',(23.8264650335721,-4.92107089613978,
0.));
#217373=CARTESIAN_POINT('Ctrl Pts',(23.8455583170062,-4.93384017643443,
0.));
#217374=CARTESIAN_POINT('Ctrl Pts',(23.8646956287172,-4.94670843465869,
0.));
#217375=CARTESIAN_POINT('Ctrl Pts',(23.883876259922,-4.95967559546566,0.));
#217376=CARTESIAN_POINT('Ctrl Pts',(23.9030995086164,-4.9727415827923,0.));
#217377=CARTESIAN_POINT('Ctrl Pts',(23.9223646794591,-4.98590631986534,
0.));
#217378=CARTESIAN_POINT('Ctrl Pts',(23.9416710836528,-4.9991697291931,0.));
#217379=CARTESIAN_POINT('Ctrl Pts',(23.9610180388271,-5.01253173257459,
0.));
#217380=CARTESIAN_POINT('Ctrl Pts',(23.9804048689228,-5.02599225112462,
0.));
#217381=CARTESIAN_POINT('Ctrl Pts',(23.9998309040747,-5.03955120528528,
0.));
#217382=CARTESIAN_POINT('Ctrl Pts',(24.0192954804896,-5.05320851483069,
0.));
#217383=CARTESIAN_POINT('Ctrl Pts',(24.0387979403268,-5.0669640988664,0.));
#217384=CARTESIAN_POINT('Ctrl Pts',(24.0583376315636,-5.08081787581271,
0.));
#217385=CARTESIAN_POINT('Ctrl Pts',(24.0779139079264,-5.09476976342618,
0.));
#217386=CARTESIAN_POINT('Ctrl Pts',(24.0975261288444,-5.10881967883126,
0.));
#217387=CARTESIAN_POINT('Ctrl Pts',(24.117173659394,-5.12296753853858,0.));
#217388=CARTESIAN_POINT('Ctrl Pts',(24.1368558702443,-5.13721325845746,
0.));
#217389=CARTESIAN_POINT('Ctrl Pts',(24.1565721375971,-5.1515567539008,0.));
#217390=CARTESIAN_POINT('Ctrl Pts',(24.1763218431344,-5.16599793957987,
0.));
#217391=CARTESIAN_POINT('Ctrl Pts',(24.1961043738755,-5.180536729614,0.));
#217392=CARTESIAN_POINT('Ctrl Pts',(24.2159191220171,-5.19517303753648,
0.));
#217393=CARTESIAN_POINT('Ctrl Pts',(24.2357654847766,-5.20990677629177,
0.));
#217394=CARTESIAN_POINT('Ctrl Pts',(24.2556428642294,-5.22473785822443,
0.));
#217395=CARTESIAN_POINT('Ctrl Pts',(24.2755506671525,-5.2396661950629,0.));
#217396=CARTESIAN_POINT('Ctrl Pts',(24.2954883048447,-5.25469169788858,
0.));
#217397=CARTESIAN_POINT('Ctrl Pts',(24.3154551932221,-5.269814277188,0.));
#217398=CARTESIAN_POINT('Ctrl Pts',(24.3354507529414,-5.28503384290649,
0.));
#217399=CARTESIAN_POINT('Ctrl Pts',(24.3554744095075,-5.30035030449065,
0.));
#217400=CARTESIAN_POINT('Ctrl Pts',(24.3755255933917,-5.31576357092527,
0.));
#217401=CARTESIAN_POINT('Ctrl Pts',(24.3956037401293,-5.33127355076035,
0.));
#217402=CARTESIAN_POINT('Ctrl Pts',(24.4157082904614,-5.34688015213538,
0.));
#217403=CARTESIAN_POINT('Ctrl Pts',(24.435838689915,-5.36258328273628,0.));
#217404=CARTESIAN_POINT('Ctrl Pts',(24.4559943883157,-5.37838284973696,
0.));
#217405=CARTESIAN_POINT('Ctrl Pts',(24.4761748393321,-5.39427875973825,
0.));
#217406=CARTESIAN_POINT('Ctrl Pts',(24.496379499983,-5.41027091869242,0.));
#217407=CARTESIAN_POINT('Ctrl Pts',(24.5166078302108,-5.4263592318342,0.));
#217408=CARTESIAN_POINT('Ctrl Pts',(24.5368592922863,-5.44254360356881,
0.));
#217409=CARTESIAN_POINT('Ctrl Pts',(24.5571333514842,-5.45882393762263,
0.));
#217410=CARTESIAN_POINT('Ctrl Pts',(24.5774294770329,-5.4752001372442,0.));
#217411=CARTESIAN_POINT('Ctrl Pts',(24.5977471429364,-5.49167210537248,
0.));
#217412=CARTESIAN_POINT('Ctrl Pts',(24.6180858289179,-5.50823974481963,
0.));
#217413=CARTESIAN_POINT('Ctrl Pts',(24.6384450211467,-5.52490295840993,
0.));
#217414=CARTESIAN_POINT('Ctrl Pts',(24.6588242134738,-5.54166164919584,
0.));
#217415=CARTESIAN_POINT('Ctrl Pts',(24.6792229061794,-5.55851572025377,
0.));
#217416=CARTESIAN_POINT('Ctrl Pts',(24.6996406035517,-5.57546507427756,
0.));
#217417=CARTESIAN_POINT('Ctrl Pts',(24.7200768119088,-5.59250961323988,
0.));
#217418=CARTESIAN_POINT('Ctrl Pts',(24.7405310372739,-5.60964923798492,
0.));
#217419=CARTESIAN_POINT('Ctrl Pts',(24.7610027835697,-5.62688384790924,
0.));
#217420=CARTESIAN_POINT('Ctrl Pts',(24.781491549672,-5.64421334042262,0.));
#217421=CARTESIAN_POINT('Ctrl Pts',(24.8019968304605,-5.66163761114922,
0.));
#217422=CARTESIAN_POINT('Ctrl Pts',(24.8225181223845,-5.67915655496543,
0.));
#217423=CARTESIAN_POINT('Ctrl Pts',(24.8430549277621,-5.69677006679445,
0.));
#217424=CARTESIAN_POINT('Ctrl Pts',(24.8636067597669,-5.71447804252028,
0.));
#217425=CARTESIAN_POINT('Ctrl Pts',(24.884173146722,-5.73228037976928,0.));
#217426=CARTESIAN_POINT('Ctrl Pts',(24.904753637648,-5.75017697890805,0.));
#217427=CARTESIAN_POINT('Ctrl Pts',(24.9253478043656,-5.76816774342221,
0.));
#217428=CARTESIAN_POINT('Ctrl Pts',(24.945955229334,-5.78625257775682,0.));
#217429=CARTESIAN_POINT('Ctrl Pts',(24.9665754954496,-5.80443138549727,
0.));
#217430=CARTESIAN_POINT('Ctrl Pts',(24.9872081752734,-5.822704067442,0.));
#217431=CARTESIAN_POINT('Ctrl Pts',(25.0078528200564,-5.84107051963072,
0.));
#217432=CARTESIAN_POINT('Ctrl Pts',(25.0285089498899,-5.85953063156827,
0.));
#217433=CARTESIAN_POINT('Ctrl Pts',(25.049176040591,-5.87808428385367,0.));
#217434=CARTESIAN_POINT('Ctrl Pts',(25.0698535426514,-5.89673135155515,
0.));
#217435=CARTESIAN_POINT('Ctrl Pts',(25.0905409050773,-5.91547170844448,
0.));
#217436=CARTESIAN_POINT('Ctrl Pts',(25.1112375971106,-5.93430523086836,
0.));
#217437=CARTESIAN_POINT('Ctrl Pts',(25.1319431317237,-5.95323180187379,
0.));
#217438=CARTESIAN_POINT('Ctrl Pts',(25.1526570863092,-5.97225131495618,
0.));
#217439=CARTESIAN_POINT('Ctrl Pts',(25.1733791296259,-5.99136367859755,
0.));
#217440=CARTESIAN_POINT('Ctrl Pts',(25.1941090269819,-6.01056881804614,
0.));
#217441=CARTESIAN_POINT('Ctrl Pts',(25.21484662016,-6.02986667389998,0.));
#217442=CARTESIAN_POINT('Ctrl Pts',(25.2355918139032,-6.04925720151219,
0.));
#217443=CARTESIAN_POINT('Ctrl Pts',(25.2521940105705,-6.06484373634547,
0.));
#217444=CARTESIAN_POINT('Ctrl Pts',(25.2646490489922,-6.07657531787491,
0.));
#217445=CARTESIAN_POINT('Ctrl Pts',(25.2729539149517,-6.08441489609794,
0.));
#217446=CARTESIAN_POINT('Ctrl Pts',(25.2771067246846,-6.088339316177,0.));
#217447=CARTESIAN_POINT('',(25.2771067246846,-6.088339316177,12.));
#217448=CARTESIAN_POINT('Ctrl Pts',(25.2771067246846,-6.088339316177,12.));
#217449=CARTESIAN_POINT('Ctrl Pts',(25.2729539149517,-6.08441489609794,
12.));
#217450=CARTESIAN_POINT('Ctrl Pts',(25.2646490489922,-6.07657531787491,
12.));
#217451=CARTESIAN_POINT('Ctrl Pts',(25.2521940105705,-6.06484373634547,
12.));
#217452=CARTESIAN_POINT('Ctrl Pts',(25.2355918139032,-6.04925720151219,
12.));
#217453=CARTESIAN_POINT('Ctrl Pts',(25.21484662016,-6.02986667389998,12.));
#217454=CARTESIAN_POINT('Ctrl Pts',(25.1941090269819,-6.01056881804614,
12.));
#217455=CARTESIAN_POINT('Ctrl Pts',(25.1733791296259,-5.99136367859755,
12.));
#217456=CARTESIAN_POINT('Ctrl Pts',(25.1526570863092,-5.97225131495618,
12.));
#217457=CARTESIAN_POINT('Ctrl Pts',(25.1319431317237,-5.95323180187379,
12.));
#217458=CARTESIAN_POINT('Ctrl Pts',(25.1112375971106,-5.93430523086836,
12.));
#217459=CARTESIAN_POINT('Ctrl Pts',(25.0905409050773,-5.91547170844448,
12.));
#217460=CARTESIAN_POINT('Ctrl Pts',(25.0698535426514,-5.89673135155515,
12.));
#217461=CARTESIAN_POINT('Ctrl Pts',(25.049176040591,-5.87808428385367,12.));
#217462=CARTESIAN_POINT('Ctrl Pts',(25.0285089498899,-5.85953063156827,
12.));
#217463=CARTESIAN_POINT('Ctrl Pts',(25.0078528200564,-5.84107051963072,
12.));
#217464=CARTESIAN_POINT('Ctrl Pts',(24.9872081752734,-5.822704067442,12.));
#217465=CARTESIAN_POINT('Ctrl Pts',(24.9665754954496,-5.80443138549727,
12.));
#217466=CARTESIAN_POINT('Ctrl Pts',(24.945955229334,-5.78625257775682,12.));
#217467=CARTESIAN_POINT('Ctrl Pts',(24.9253478043656,-5.76816774342221,
12.));
#217468=CARTESIAN_POINT('Ctrl Pts',(24.904753637648,-5.75017697890805,12.));
#217469=CARTESIAN_POINT('Ctrl Pts',(24.884173146722,-5.73228037976928,12.));
#217470=CARTESIAN_POINT('Ctrl Pts',(24.8636067597669,-5.71447804252028,
12.));
#217471=CARTESIAN_POINT('Ctrl Pts',(24.8430549277621,-5.69677006679445,
12.));
#217472=CARTESIAN_POINT('Ctrl Pts',(24.8225181223845,-5.67915655496543,
12.));
#217473=CARTESIAN_POINT('Ctrl Pts',(24.8019968304605,-5.66163761114922,
12.));
#217474=CARTESIAN_POINT('Ctrl Pts',(24.781491549672,-5.64421334042262,12.));
#217475=CARTESIAN_POINT('Ctrl Pts',(24.7610027835697,-5.62688384790924,
12.));
#217476=CARTESIAN_POINT('Ctrl Pts',(24.7405310372739,-5.60964923798492,
12.));
#217477=CARTESIAN_POINT('Ctrl Pts',(24.7200768119088,-5.59250961323988,
12.));
#217478=CARTESIAN_POINT('Ctrl Pts',(24.6996406035517,-5.57546507427756,
12.));
#217479=CARTESIAN_POINT('Ctrl Pts',(24.6792229061794,-5.55851572025377,
12.));
#217480=CARTESIAN_POINT('Ctrl Pts',(24.6588242134738,-5.54166164919584,
12.));
#217481=CARTESIAN_POINT('Ctrl Pts',(24.6384450211467,-5.52490295840993,
12.));
#217482=CARTESIAN_POINT('Ctrl Pts',(24.6180858289179,-5.50823974481963,
12.));
#217483=CARTESIAN_POINT('Ctrl Pts',(24.5977471429364,-5.49167210537248,
12.));
#217484=CARTESIAN_POINT('Ctrl Pts',(24.5774294770329,-5.4752001372442,12.));
#217485=CARTESIAN_POINT('Ctrl Pts',(24.5571333514842,-5.45882393762263,
12.));
#217486=CARTESIAN_POINT('Ctrl Pts',(24.5368592922863,-5.44254360356881,
12.));
#217487=CARTESIAN_POINT('Ctrl Pts',(24.5166078302108,-5.4263592318342,12.));
#217488=CARTESIAN_POINT('Ctrl Pts',(24.496379499983,-5.41027091869242,12.));
#217489=CARTESIAN_POINT('Ctrl Pts',(24.4761748393321,-5.39427875973825,
12.));
#217490=CARTESIAN_POINT('Ctrl Pts',(24.4559943883157,-5.37838284973696,
12.));
#217491=CARTESIAN_POINT('Ctrl Pts',(24.435838689915,-5.36258328273628,12.));
#217492=CARTESIAN_POINT('Ctrl Pts',(24.4157082904614,-5.34688015213538,
12.));
#217493=CARTESIAN_POINT('Ctrl Pts',(24.3956037401293,-5.33127355076035,
12.));
#217494=CARTESIAN_POINT('Ctrl Pts',(24.3755255933917,-5.31576357092527,
12.));
#217495=CARTESIAN_POINT('Ctrl Pts',(24.3554744095075,-5.30035030449065,
12.));
#217496=CARTESIAN_POINT('Ctrl Pts',(24.3354507529414,-5.28503384290649,
12.));
#217497=CARTESIAN_POINT('Ctrl Pts',(24.3154551932221,-5.269814277188,12.));
#217498=CARTESIAN_POINT('Ctrl Pts',(24.2954883048447,-5.25469169788858,
12.));
#217499=CARTESIAN_POINT('Ctrl Pts',(24.2755506671525,-5.2396661950629,12.));
#217500=CARTESIAN_POINT('Ctrl Pts',(24.2556428642294,-5.22473785822443,
12.));
#217501=CARTESIAN_POINT('Ctrl Pts',(24.2357654847766,-5.20990677629177,
12.));
#217502=CARTESIAN_POINT('Ctrl Pts',(24.2159191220171,-5.19517303753648,
12.));
#217503=CARTESIAN_POINT('Ctrl Pts',(24.1961043738755,-5.180536729614,12.));
#217504=CARTESIAN_POINT('Ctrl Pts',(24.1763218431344,-5.16599793957987,
12.));
#217505=CARTESIAN_POINT('Ctrl Pts',(24.1565721375971,-5.1515567539008,12.));
#217506=CARTESIAN_POINT('Ctrl Pts',(24.1368558702443,-5.13721325845746,
12.));
#217507=CARTESIAN_POINT('Ctrl Pts',(24.117173659394,-5.12296753853858,12.));
#217508=CARTESIAN_POINT('Ctrl Pts',(24.0975261288444,-5.10881967883126,
12.));
#217509=CARTESIAN_POINT('Ctrl Pts',(24.0779139079264,-5.09476976342618,
12.));
#217510=CARTESIAN_POINT('Ctrl Pts',(24.0583376315636,-5.08081787581271,
12.));
#217511=CARTESIAN_POINT('Ctrl Pts',(24.0387979403268,-5.0669640988664,12.));
#217512=CARTESIAN_POINT('Ctrl Pts',(24.0192954804896,-5.05320851483069,
12.));
#217513=CARTESIAN_POINT('Ctrl Pts',(23.9998309040747,-5.03955120528528,
12.));
#217514=CARTESIAN_POINT('Ctrl Pts',(23.9804048689228,-5.02599225112462,
12.));
#217515=CARTESIAN_POINT('Ctrl Pts',(23.9610180388271,-5.01253173257459,
12.));
#217516=CARTESIAN_POINT('Ctrl Pts',(23.9416710836528,-4.9991697291931,12.));
#217517=CARTESIAN_POINT('Ctrl Pts',(23.9223646794591,-4.98590631986534,
12.));
#217518=CARTESIAN_POINT('Ctrl Pts',(23.9030995086164,-4.9727415827923,12.));
#217519=CARTESIAN_POINT('Ctrl Pts',(23.883876259922,-4.95967559546566,12.));
#217520=CARTESIAN_POINT('Ctrl Pts',(23.8646956287172,-4.94670843465869,
12.));
#217521=CARTESIAN_POINT('Ctrl Pts',(23.8455583170062,-4.93384017643443,
12.));
#217522=CARTESIAN_POINT('Ctrl Pts',(23.8264650335721,-4.92107089613978,
12.));
#217523=CARTESIAN_POINT('Ctrl Pts',(23.8074164940897,-4.90840066839348,
12.));
#217524=CARTESIAN_POINT('Ctrl Pts',(23.7884134212381,-4.89582956706772,
12.));
#217525=CARTESIAN_POINT('Ctrl Pts',(23.7694565448044,-4.88335766525566,
12.));
#217526=CARTESIAN_POINT('Ctrl Pts',(23.7505466018239,-4.87098503527144,
12.));
#217527=CARTESIAN_POINT('Ctrl Pts',(23.7316843367308,-4.85871174865493,
12.));
#217528=CARTESIAN_POINT('Ctrl Pts',(23.7128705015014,-4.84653787616424,
12.));
#217529=CARTESIAN_POINT('Ctrl Pts',(23.6941058557971,-4.83446348776268,
12.));
#217530=CARTESIAN_POINT('Ctrl Pts',(23.6753911671023,-4.82248865259571,
12.));
#217531=CARTESIAN_POINT('Ctrl Pts',(23.6567272108631,-4.81061343896443,
12.));
#217532=CARTESIAN_POINT('Ctrl Pts',(23.6381147706581,-4.79883791433231,
12.));
#217533=CARTESIAN_POINT('Ctrl Pts',(23.6195546383625,-4.78716214532105,
12.));
#217534=CARTESIAN_POINT('Ctrl Pts',(23.6010476143099,-4.77558619769876,
12.));
#217535=CARTESIAN_POINT('Ctrl Pts',(23.5825945074535,-4.76411013636252,
12.));
#217536=CARTESIAN_POINT('Ctrl Pts',(23.564196135517,-4.75273402530616,12.));
#217537=CARTESIAN_POINT('Ctrl Pts',(23.5458533251715,-4.74145792760699,
12.));
#217538=CARTESIAN_POINT('Ctrl Pts',(23.5275669122378,-4.73028190543032,
12.));
#217539=CARTESIAN_POINT('Ctrl Pts',(23.5093377418784,-4.71920602001905,
12.));
#217540=CARTESIAN_POINT('Ctrl Pts',(23.491166668789,-4.70823033167821,12.));
#217541=CARTESIAN_POINT('Ctrl Pts',(23.4730545573849,-4.69735489975024,
12.));
#217542=CARTESIAN_POINT('Ctrl Pts',(23.4550022819852,-4.68657978258298,
12.));
#217543=CARTESIAN_POINT('Ctrl Pts',(23.4370107270444,-4.67590503753051,
12.));
#217544=CARTESIAN_POINT('Ctrl Pts',(23.4190807873798,-4.66533072094664,
12.));
#217545=CARTESIAN_POINT('Ctrl Pts',(23.4012133683957,-4.65485688816923,
12.));
#217546=CARTESIAN_POINT('Ctrl Pts',(23.383409386307,-4.64448359349936,12.));
#217547=CARTESIAN_POINT('Ctrl Pts',(23.3656697683496,-4.63421089016556,
12.));
#217548=CARTESIAN_POINT('Ctrl Pts',(23.3479954530281,-4.62403883030825,
12.));
#217549=CARTESIAN_POINT('Ctrl Pts',(23.3303873903947,-4.6139674649785,12.));
#217550=CARTESIAN_POINT('Ctrl Pts',(23.3128465423119,-4.60399684412176,
12.));
#217551=CARTESIAN_POINT('Ctrl Pts',(23.295373882719,-4.59412701655751,12.));
#217552=CARTESIAN_POINT('Ctrl Pts',(23.2779703978868,-4.58435802994675,
12.));
#217553=CARTESIAN_POINT('Ctrl Pts',(23.2606370866853,-4.57468993076071,
12.));
#217554=CARTESIAN_POINT('Ctrl Pts',(23.2433749609117,-4.56512276427812,
12.));
#217555=CARTESIAN_POINT('Ctrl Pts',(23.2261850456054,-4.55565657456957,
12.));
#217556=CARTESIAN_POINT('Ctrl Pts',(23.2090683793627,-4.54629140447543,
12.));
#217557=CARTESIAN_POINT('Ctrl Pts',(23.1920260146474,-4.53702729557586,
12.));
#217558=CARTESIAN_POINT('Ctrl Pts',(23.1750590180923,-4.52786428815049,
12.));
#217559=CARTESIAN_POINT('Ctrl Pts',(23.1581684708778,-4.51880242116786,
12.));
#217560=CARTESIAN_POINT('Ctrl Pts',(23.1413554691136,-4.50984173227088,
12.));
#217561=CARTESIAN_POINT('Ctrl Pts',(23.1246211242117,-4.5009822577518,12.));
#217562=CARTESIAN_POINT('Ctrl Pts',(23.1079665632629,-4.49222403252202,
12.));
#217563=CARTESIAN_POINT('Ctrl Pts',(23.0913929293909,-4.48356709006757,
12.));
#217564=CARTESIAN_POINT('Ctrl Pts',(23.0749013821867,-4.47501146242822,
12.));
#217565=CARTESIAN_POINT('Ctrl Pts',(23.0584930981723,-4.46655718018206,
12.));
#217566=CARTESIAN_POINT('Ctrl Pts',(23.0421692712466,-4.45820427241678,
12.));
#217567=CARTESIAN_POINT('Ctrl Pts',(23.0259311131395,-4.44995276669699,
12.));
#217568=CARTESIAN_POINT('Ctrl Pts',(23.0097798538399,-4.44180268901667,
12.));
#217569=CARTESIAN_POINT('Ctrl Pts',(22.9937167421009,-4.43375406376906,
12.));
#217570=CARTESIAN_POINT('Ctrl Pts',(22.9777430460021,-4.42580691372772,
12.));
#217571=CARTESIAN_POINT('Ctrl Pts',(22.9618600534866,-4.41796126001311,
12.));
#217572=CARTESIAN_POINT('Ctrl Pts',(22.9460690729092,-4.41021712205549,
12.));
#217573=CARTESIAN_POINT('Ctrl Pts',(22.9303714335549,-4.40257451754309,
12.));
#217574=CARTESIAN_POINT('Ctrl Pts',(22.9147684862425,-4.39503346238455,
12.));
#217575=CARTESIAN_POINT('Ctrl Pts',(22.8992616040108,-4.38759397068393,
12.));
#217576=CARTESIAN_POINT('Ctrl Pts',(22.8838521827702,-4.38025605470091,
12.));
#217577=CARTESIAN_POINT('Ctrl Pts',(22.8685416419725,-4.37301972480753,
12.));
#217578=CARTESIAN_POINT('Ctrl Pts',(22.8533314252419,-4.36588498943011,
12.));
#217579=CARTESIAN_POINT('Ctrl Pts',(22.838223001118,-4.3588518550056,12.));
#217580=CARTESIAN_POINT('Ctrl Pts',(22.8232178638873,-4.35192032594802,
12.));
#217581=CARTESIAN_POINT('Ctrl Pts',(22.808317534379,-4.34509040460066,12.));
#217582=CARTESIAN_POINT('Ctrl Pts',(22.7935235607807,-4.33836209118444,
12.));
#217583=CARTESIAN_POINT('Ctrl Pts',(22.7788375194081,-4.33173538373183,
12.));
#217584=CARTESIAN_POINT('Ctrl Pts',(22.764261015648,-4.32521027803748,12.));
#217585=CARTESIAN_POINT('Ctrl Pts',(22.7497956849852,-4.31878676761231,
12.));
#217586=CARTESIAN_POINT('Ctrl Pts',(22.7354431939926,-4.31246484362551,
12.));
#217587=CARTESIAN_POINT('Ctrl Pts',(22.7212052413384,-4.30624449484075,
12.));
#217588=CARTESIAN_POINT('Ctrl Pts',(22.707083558756,-4.30012570754067,12.));
#217589=CARTESIAN_POINT('Ctrl Pts',(22.6930799122545,-4.29410846547062,
12.));
#217590=CARTESIAN_POINT('Ctrl Pts',(22.6791961033536,-4.28819274977767,
12.));
#217591=CARTESIAN_POINT('Ctrl Pts',(22.665433970311,-4.2823785389406,12.));
#217592=CARTESIAN_POINT('Ctrl Pts',(22.6517953893303,-4.27666580869118,
12.));
#217593=CARTESIAN_POINT('Ctrl Pts',(22.6382822758171,-4.27105453193,12.));
#217594=CARTESIAN_POINT('Ctrl Pts',(22.6248965859975,-4.26554467865572,
12.));
#217595=CARTESIAN_POINT('Ctrl Pts',(22.611640318482,-4.26013621588304,12.));
#217596=CARTESIAN_POINT('Ctrl Pts',(22.5985155158637,-4.25482910755486,
12.));
#217597=CARTESIAN_POINT('Ctrl Pts',(22.5855242662479,-4.24962331444186,
12.));
#217598=CARTESIAN_POINT('Ctrl Pts',(22.5726687049922,-4.2445187940486,12.));
#217599=CARTESIAN_POINT('Ctrl Pts',(22.559951016643,-4.23951550052527,12.));
#217600=CARTESIAN_POINT('Ctrl Pts',(22.5473734368086,-4.23461338456714,
12.));
#217601=CARTESIAN_POINT('Ctrl Pts',(22.5349382540587,-4.22981239330733,
12.));
#217602=CARTESIAN_POINT('Ctrl Pts',(22.5226478117885,-4.22511247020041,
12.));
#217603=CARTESIAN_POINT('Ctrl Pts',(22.5105045108882,-4.22051355490198,
12.));
#217604=CARTESIAN_POINT('Ctrl Pts',(22.4985108124229,-4.21601558313909,
12.));
#217605=CARTESIAN_POINT('Ctrl Pts',(22.4866692403147,-4.21161848657429,
12.));
#217606=CARTESIAN_POINT('Ctrl Pts',(22.4749823839915,-4.20732219265649,
12.));
#217607=CARTESIAN_POINT('Ctrl Pts',(22.4634529011433,-4.20312662448172,
12.));
#217608=CARTESIAN_POINT('Ctrl Pts',(22.4520835205419,-4.19903170066356,
12.));
#217609=CARTESIAN_POINT('Ctrl Pts',(22.4408770448917,-4.19503733518862,
12.));
#217610=CARTESIAN_POINT('Ctrl Pts',(22.4298363535421,-4.19114343726943,
12.));
#217611=CARTESIAN_POINT('Ctrl Pts',(22.4189644056115,-4.18734991117722,
12.));
#217612=CARTESIAN_POINT('Ctrl Pts',(22.4082642454453,-4.18365665600852,
12.));
#217613=CARTESIAN_POINT('Ctrl Pts',(22.3977390078075,-4.18006356544883,
12.));
#217614=CARTESIAN_POINT('Ctrl Pts',(22.3873919231334,-4.17657052752826,
12.));
#217615=CARTESIAN_POINT('Ctrl Pts',(22.3772263228617,-4.17317742436146,
12.));
#217616=CARTESIAN_POINT('Ctrl Pts',(22.3672456427599,-4.16988413199458,
12.));
#217617=CARTESIAN_POINT('Ctrl Pts',(22.3574534257396,-4.16669052026601,
12.));
#217618=CARTESIAN_POINT('Ctrl Pts',(22.3478533253889,-4.16359645263189,
12.));
#217619=CARTESIAN_POINT('Ctrl Pts',(22.3384491078602,-4.16060178604165,
12.));
#217620=CARTESIAN_POINT('Ctrl Pts',(22.3292446628959,-4.15770637047891,
12.));
#217621=CARTESIAN_POINT('Ctrl Pts',(22.3202440186979,-4.15491004835282,
12.));
#217622=CARTESIAN_POINT('Ctrl Pts',(22.3114513545185,-4.15221265396991,
12.));
#217623=CARTESIAN_POINT('Ctrl Pts',(22.3028710166933,-4.14961401285523,
12.));
#217624=CARTESIAN_POINT('Ctrl Pts',(22.2945075198467,-4.14711394168557,
12.));
#217625=CARTESIAN_POINT('Ctrl Pts',(22.2863655389166,-4.14471224859297,
12.));
#217626=CARTESIAN_POINT('Ctrl Pts',(22.2784499072027,-4.14240873321985,
12.));
#217627=CARTESIAN_POINT('Ctrl Pts',(22.2707656042457,-4.14020318715992,
12.));
#217628=CARTESIAN_POINT('Ctrl Pts',(22.2633177913972,-4.13809539255423,
12.));
#217629=CARTESIAN_POINT('Ctrl Pts',(22.2561118708421,-4.13608511977227,
12.));
#217630=CARTESIAN_POINT('Ctrl Pts',(22.249153531779,-4.13417212558811,12.));
#217631=CARTESIAN_POINT('Ctrl Pts',(22.2424488153523,-4.13235615060161,
12.));
#217632=CARTESIAN_POINT('Ctrl Pts',(22.2360040565533,-4.13063692157499,
12.));
#217633=CARTESIAN_POINT('Ctrl Pts',(22.2298258043947,-4.1290141546338,12.));
#217634=CARTESIAN_POINT('Ctrl Pts',(22.2239207458781,-4.12748755830105,
12.));
#217635=CARTESIAN_POINT('Ctrl Pts',(22.2182956401341,-4.12605683613308,
12.));
#217636=CARTESIAN_POINT('Ctrl Pts',(22.2129576146671,-4.12472167516608,
12.));
#217637=CARTESIAN_POINT('Ctrl Pts',(22.2079143941719,-4.12348173702024,
12.));
#217638=CARTESIAN_POINT('Ctrl Pts',(22.2031746532106,-4.12233664408228,
12.));
#217639=CARTESIAN_POINT('Ctrl Pts',(22.1987479618246,-4.12128598183523,
12.));
#217640=CARTESIAN_POINT('Ctrl Pts',(22.1946440958098,-4.12032932637738,
12.));
#217641=CARTESIAN_POINT('Ctrl Pts',(22.1908725908525,-4.11946626228637,
12.));
#217642=CARTESIAN_POINT('Ctrl Pts',(22.1874419861496,-4.11869641271775,
12.));
#217643=CARTESIAN_POINT('Ctrl Pts',(22.1843613164855,-4.11801938107481,
12.));
#217644=CARTESIAN_POINT('Ctrl Pts',(22.1816414985788,-4.11743469691757,
12.));
#217645=CARTESIAN_POINT('Ctrl Pts',(22.179297473024,-4.11694173195005,12.));
#217646=CARTESIAN_POINT('Ctrl Pts',(22.177347426894,-4.11653973150519,12.));
#217647=CARTESIAN_POINT('Ctrl Pts',(22.1758088296598,-4.1162279721707,12.));
#217648=CARTESIAN_POINT('Ctrl Pts',(22.1746949858775,-4.11600589882846,
12.));
#217649=CARTESIAN_POINT('Ctrl Pts',(22.1741488021234,-4.11589976826168,
12.));
#217650=CARTESIAN_POINT('Ctrl Pts',(22.1739341411687,-4.11586035878288,
12.));
#217651=CARTESIAN_POINT('Ctrl Pts',(22.173877682324,-4.11585194677443,12.));
#217652=CARTESIAN_POINT('Ctrl Pts',(22.1738711152697,-4.11585220600463,
12.));
#217653=CARTESIAN_POINT('',(25.2771067246846,-6.088339316177,0.));
#217654=CARTESIAN_POINT('Origin',(19.4030938020118,-9.26120677397565,0.));
#217655=CARTESIAN_POINT('',(20.353053841303,-9.71462809124917,12.));
#217656=CARTESIAN_POINT('',(9.70154690100589,-4.63060338698782,12.));
#217657=CARTESIAN_POINT('',(20.353053841303,-9.71462809124917,0.));
#217658=CARTESIAN_POINT('',(20.353053841303,-9.71462809124917,0.));
#217659=CARTESIAN_POINT('',(9.70154690100589,-4.63060338698782,0.));
#217660=CARTESIAN_POINT('Ctrl Pts',(24.9347862158358,-7.36589684767345,
0.));
#217661=CARTESIAN_POINT('Ctrl Pts',(24.9347862158358,-7.36589684767345,
12.));
#217662=CARTESIAN_POINT('Ctrl Pts',(24.9292275670674,-7.36721909028843,
0.));
#217663=CARTESIAN_POINT('Ctrl Pts',(24.9292275670674,-7.36721909028843,
12.));
#217664=CARTESIAN_POINT('Ctrl Pts',(24.9181155530543,-7.36985593120091,
0.));
#217665=CARTESIAN_POINT('Ctrl Pts',(24.9181155530543,-7.36985593120091,
12.));
#217666=CARTESIAN_POINT('Ctrl Pts',(24.901463382605,-7.37378825961676,0.));
#217667=CARTESIAN_POINT('Ctrl Pts',(24.901463382605,-7.37378825961676,12.));
#217668=CARTESIAN_POINT('Ctrl Pts',(24.8792921911115,-7.3789854964027,0.));
#217669=CARTESIAN_POINT('Ctrl Pts',(24.8792921911115,-7.3789854964027,12.));
#217670=CARTESIAN_POINT('Ctrl Pts',(24.8516310625176,-7.38540558903621,
0.));
#217671=CARTESIAN_POINT('Ctrl Pts',(24.8516310625176,-7.38540558903621,
12.));
#217672=CARTESIAN_POINT('Ctrl Pts',(24.8240228520893,-7.39174922585809,
0.));
#217673=CARTESIAN_POINT('Ctrl Pts',(24.8240228520893,-7.39174922585809,
12.));
#217674=CARTESIAN_POINT('Ctrl Pts',(24.7964676646431,-7.39801641583013,
0.));
#217675=CARTESIAN_POINT('Ctrl Pts',(24.7964676646431,-7.39801641583013,
12.));
#217676=CARTESIAN_POINT('Ctrl Pts',(24.7689656668983,-7.40420718661603,
0.));
#217677=CARTESIAN_POINT('Ctrl Pts',(24.7689656668983,-7.40420718661603,
12.));
#217678=CARTESIAN_POINT('Ctrl Pts',(24.7415170994784,-7.41032159082382,
0.));
#217679=CARTESIAN_POINT('Ctrl Pts',(24.7415170994784,-7.41032159082382,
12.));
#217680=CARTESIAN_POINT('Ctrl Pts',(24.7141222950051,-7.41635971481674,
0.));
#217681=CARTESIAN_POINT('Ctrl Pts',(24.7141222950051,-7.41635971481674,
12.));
#217682=CARTESIAN_POINT('Ctrl Pts',(24.6867816727192,-7.42232167766266,
0.));
#217683=CARTESIAN_POINT('Ctrl Pts',(24.6867816727192,-7.42232167766266,
12.));
#217684=CARTESIAN_POINT('Ctrl Pts',(24.6594957128756,-7.42820762159126,
0.));
#217685=CARTESIAN_POINT('Ctrl Pts',(24.6594957128756,-7.42820762159126,
12.));
#217686=CARTESIAN_POINT('Ctrl Pts',(24.6322649369517,-7.43401770489524,
0.));
#217687=CARTESIAN_POINT('Ctrl Pts',(24.6322649369517,-7.43401770489524,
12.));
#217688=CARTESIAN_POINT('Ctrl Pts',(24.6050898852368,-7.43975209375504,
0.));
#217689=CARTESIAN_POINT('Ctrl Pts',(24.6050898852368,-7.43975209375504,
12.));
#217690=CARTESIAN_POINT('Ctrl Pts',(24.577971096086,-7.44541095473135,0.));
#217691=CARTESIAN_POINT('Ctrl Pts',(24.577971096086,-7.44541095473135,12.));
#217692=CARTESIAN_POINT('Ctrl Pts',(24.5509090831559,-7.4509944465116,0.));
#217693=CARTESIAN_POINT('Ctrl Pts',(24.5509090831559,-7.4509944465116,12.));
#217694=CARTESIAN_POINT('Ctrl Pts',(24.5239043173072,-7.45650271335862,
0.));
#217695=CARTESIAN_POINT('Ctrl Pts',(24.5239043173072,-7.45650271335862,
12.));
#217696=CARTESIAN_POINT('Ctrl Pts',(24.4969572391483,-7.46193588961464,
0.));
#217697=CARTESIAN_POINT('Ctrl Pts',(24.4969572391483,-7.46193588961464,
12.));
#217698=CARTESIAN_POINT('Ctrl Pts',(24.4700682684524,-7.46729410308787,
0.));
#217699=CARTESIAN_POINT('Ctrl Pts',(24.4700682684524,-7.46729410308787,
12.));
#217700=CARTESIAN_POINT('Ctrl Pts',(24.443237814649,-7.47257747883246,0.));
#217701=CARTESIAN_POINT('Ctrl Pts',(24.443237814649,-7.47257747883246,12.));
#217702=CARTESIAN_POINT('Ctrl Pts',(24.4164662871163,-7.47778614286565,
0.));
#217703=CARTESIAN_POINT('Ctrl Pts',(24.4164662871163,-7.47778614286565,
12.));
#217704=CARTESIAN_POINT('Ctrl Pts',(24.3897541049254,-7.48292022569301,
0.));
#217705=CARTESIAN_POINT('Ctrl Pts',(24.3897541049254,-7.48292022569301,
12.));
#217706=CARTESIAN_POINT('Ctrl Pts',(24.3631017084524,-7.48797986651909,
0.));
#217707=CARTESIAN_POINT('Ctrl Pts',(24.3631017084524,-7.48797986651909,
12.));
#217708=CARTESIAN_POINT('Ctrl Pts',(24.3365095573685,-7.49296521252421,
0.));
#217709=CARTESIAN_POINT('Ctrl Pts',(24.3365095573685,-7.49296521252421,
12.));
#217710=CARTESIAN_POINT('Ctrl Pts',(24.3099781253355,-7.49787641695439,
0.));
#217711=CARTESIAN_POINT('Ctrl Pts',(24.3099781253355,-7.49787641695439,
12.));
#217712=CARTESIAN_POINT('Ctrl Pts',(24.2835078958973,-7.50271363765152,
0.));
#217713=CARTESIAN_POINT('Ctrl Pts',(24.2835078958973,-7.50271363765152,
12.));
#217714=CARTESIAN_POINT('Ctrl Pts',(24.2570993577034,-7.50747703535134,
0.));
#217715=CARTESIAN_POINT('Ctrl Pts',(24.2570993577034,-7.50747703535134,
12.));
#217716=CARTESIAN_POINT('Ctrl Pts',(24.2307530003887,-7.51216677222181,
0.));
#217717=CARTESIAN_POINT('Ctrl Pts',(24.2307530003887,-7.51216677222181,
12.));
#217718=CARTESIAN_POINT('Ctrl Pts',(24.2044693092349,-7.51678300997949,
0.));
#217719=CARTESIAN_POINT('Ctrl Pts',(24.2044693092349,-7.51678300997949,
12.));
#217720=CARTESIAN_POINT('Ctrl Pts',(24.1782487641594,-7.52132590953802,
0.));
#217721=CARTESIAN_POINT('Ctrl Pts',(24.1782487641594,-7.52132590953802,
12.));
#217722=CARTESIAN_POINT('Ctrl Pts',(24.1520918425364,-7.52579563201424,
0.));
#217723=CARTESIAN_POINT('Ctrl Pts',(24.1520918425364,-7.52579563201424,
12.));
#217724=CARTESIAN_POINT('Ctrl Pts',(24.1259990209207,-7.53019233935502,
0.));
#217725=CARTESIAN_POINT('Ctrl Pts',(24.1259990209207,-7.53019233935502,
12.));
#217726=CARTESIAN_POINT('Ctrl Pts',(24.0999707772642,-7.53451619514649,
0.));
#217727=CARTESIAN_POINT('Ctrl Pts',(24.0999707772642,-7.53451619514649,
12.));
#217728=CARTESIAN_POINT('Ctrl Pts',(24.0740075927985,-7.53876736531014,
0.));
#217729=CARTESIAN_POINT('Ctrl Pts',(24.0740075927985,-7.53876736531014,
12.));
#217730=CARTESIAN_POINT('Ctrl Pts',(24.0481099543353,-7.54294601896145,
0.));
#217731=CARTESIAN_POINT('Ctrl Pts',(24.0481099543353,-7.54294601896145,
12.));
#217732=CARTESIAN_POINT('Ctrl Pts',(24.022278355453,-7.5470523288591,0.));
#217733=CARTESIAN_POINT('Ctrl Pts',(24.022278355453,-7.5470523288591,12.));
#217734=CARTESIAN_POINT('Ctrl Pts',(23.9965132953185,-7.55108647097441,
0.));
#217735=CARTESIAN_POINT('Ctrl Pts',(23.9965132953185,-7.55108647097441,
12.));
#217736=CARTESIAN_POINT('Ctrl Pts',(23.9708152779884,-7.55504862424812,
0.));
#217737=CARTESIAN_POINT('Ctrl Pts',(23.9708152779884,-7.55504862424812,
12.));
#217738=CARTESIAN_POINT('Ctrl Pts',(23.9451848115,-7.55893897027683,0.));
#217739=CARTESIAN_POINT('Ctrl Pts',(23.9451848115,-7.55893897027683,12.));
#217740=CARTESIAN_POINT('Ctrl Pts',(23.9196224070759,-7.56275769304773,
0.));
#217741=CARTESIAN_POINT('Ctrl Pts',(23.9196224070759,-7.56275769304773,
12.));
#217742=CARTESIAN_POINT('Ctrl Pts',(23.8941285782003,-7.56650497863792,
0.));
#217743=CARTESIAN_POINT('Ctrl Pts',(23.8941285782003,-7.56650497863792,
12.));
#217744=CARTESIAN_POINT('Ctrl Pts',(23.8687038399597,-7.57018101500711,
0.));
#217745=CARTESIAN_POINT('Ctrl Pts',(23.8687038399597,-7.57018101500711,
12.));
#217746=CARTESIAN_POINT('Ctrl Pts',(23.8433487096134,-7.57378599219817,
0.));
#217747=CARTESIAN_POINT('Ctrl Pts',(23.8433487096134,-7.57378599219817,
12.));
#217748=CARTESIAN_POINT('Ctrl Pts',(23.8180637069977,-7.57732010249066,
0.));
#217749=CARTESIAN_POINT('Ctrl Pts',(23.8180637069977,-7.57732010249066,
12.));
#217750=CARTESIAN_POINT('Ctrl Pts',(23.7928493549908,-7.58078354058212,
0.));
#217751=CARTESIAN_POINT('Ctrl Pts',(23.7928493549908,-7.58078354058212,
12.));
#217752=CARTESIAN_POINT('Ctrl Pts',(23.7677061799376,-7.58417650376272,
0.));
#217753=CARTESIAN_POINT('Ctrl Pts',(23.7677061799376,-7.58417650376272,
12.));
#217754=CARTESIAN_POINT('Ctrl Pts',(23.7426347121006,-7.58749919210832,
0.));
#217755=CARTESIAN_POINT('Ctrl Pts',(23.7426347121006,-7.58749919210832,
12.));
#217756=CARTESIAN_POINT('Ctrl Pts',(23.7176354860457,-7.59075180865327,
0.));
#217757=CARTESIAN_POINT('Ctrl Pts',(23.7176354860457,-7.59075180865327,
12.));
#217758=CARTESIAN_POINT('Ctrl Pts',(23.6927090405067,-7.59393455934042,
0.));
#217759=CARTESIAN_POINT('Ctrl Pts',(23.6927090405067,-7.59393455934042,
12.));
#217760=CARTESIAN_POINT('Ctrl Pts',(23.6678559182876,-7.59704765299572,
0.));
#217761=CARTESIAN_POINT('Ctrl Pts',(23.6678559182876,-7.59704765299572,
12.));
#217762=CARTESIAN_POINT('Ctrl Pts',(23.6430766661419,-7.6000913013013,0.));
#217763=CARTESIAN_POINT('Ctrl Pts',(23.6430766661419,-7.6000913013013,12.));
#217764=CARTESIAN_POINT('Ctrl Pts',(23.6183718346576,-7.60306571877806,
0.));
#217765=CARTESIAN_POINT('Ctrl Pts',(23.6183718346576,-7.60306571877806,
12.));
#217766=CARTESIAN_POINT('Ctrl Pts',(23.5937419781244,-7.60597112277094,
0.));
#217767=CARTESIAN_POINT('Ctrl Pts',(23.5937419781244,-7.60597112277094,
12.));
#217768=CARTESIAN_POINT('Ctrl Pts',(23.5691876544243,-7.608807733446,0.));
#217769=CARTESIAN_POINT('Ctrl Pts',(23.5691876544243,-7.608807733446,12.));
#217770=CARTESIAN_POINT('Ctrl Pts',(23.5447094252028,-7.61157577385372,
0.));
#217771=CARTESIAN_POINT('Ctrl Pts',(23.5447094252028,-7.61157577385372,
12.));
#217772=CARTESIAN_POINT('Ctrl Pts',(23.5203078560128,-7.61427546999299,
0.));
#217773=CARTESIAN_POINT('Ctrl Pts',(23.5203078560128,-7.61427546999299,
12.));
#217774=CARTESIAN_POINT('Ctrl Pts',(23.4959835164608,-7.61690705088319,
0.));
#217775=CARTESIAN_POINT('Ctrl Pts',(23.4959835164608,-7.61690705088319,
12.));
#217776=CARTESIAN_POINT('Ctrl Pts',(23.4717369803438,-7.61947074863978,
0.));
#217777=CARTESIAN_POINT('Ctrl Pts',(23.4717369803438,-7.61947074863978,
12.));
#217778=CARTESIAN_POINT('Ctrl Pts',(23.4475688257854,-7.62196679855957,
0.));
#217779=CARTESIAN_POINT('Ctrl Pts',(23.4475688257854,-7.62196679855957,
12.));
#217780=CARTESIAN_POINT('Ctrl Pts',(23.4234796353544,-7.62439543920055,
0.));
#217781=CARTESIAN_POINT('Ctrl Pts',(23.4234796353544,-7.62439543920055,
12.));
#217782=CARTESIAN_POINT('Ctrl Pts',(23.3994699961122,-7.62675691240335,
0.));
#217783=CARTESIAN_POINT('Ctrl Pts',(23.3994699961122,-7.62675691240335,
12.));
#217784=CARTESIAN_POINT('Ctrl Pts',(23.3755404996638,-7.62905146332598,
0.));
#217785=CARTESIAN_POINT('Ctrl Pts',(23.3755404996638,-7.62905146332598,
12.));
#217786=CARTESIAN_POINT('Ctrl Pts',(23.3516917421973,-7.63127934048139,
0.));
#217787=CARTESIAN_POINT('Ctrl Pts',(23.3516917421973,-7.63127934048139,
12.));
#217788=CARTESIAN_POINT('Ctrl Pts',(23.3279243245241,-7.63344079578163,
0.));
#217789=CARTESIAN_POINT('Ctrl Pts',(23.3279243245241,-7.63344079578163,
12.));
#217790=CARTESIAN_POINT('Ctrl Pts',(23.3042388521021,-7.63553608458784,
0.));
#217791=CARTESIAN_POINT('Ctrl Pts',(23.3042388521021,-7.63553608458784,
12.));
#217792=CARTESIAN_POINT('Ctrl Pts',(23.2806359350853,-7.63756546576375,
0.));
#217793=CARTESIAN_POINT('Ctrl Pts',(23.2806359350853,-7.63756546576375,
12.));
#217794=CARTESIAN_POINT('Ctrl Pts',(23.2571161884487,-7.63952920172837,
0.));
#217795=CARTESIAN_POINT('Ctrl Pts',(23.2571161884487,-7.63952920172837,
12.));
#217796=CARTESIAN_POINT('Ctrl Pts',(23.2336802320912,-7.64142755851508,
0.));
#217797=CARTESIAN_POINT('Ctrl Pts',(23.2336802320912,-7.64142755851508,
12.));
#217798=CARTESIAN_POINT('Ctrl Pts',(23.2103286909399,-7.64326080583684,
0.));
#217799=CARTESIAN_POINT('Ctrl Pts',(23.2103286909399,-7.64326080583684,
12.));
#217800=CARTESIAN_POINT('Ctrl Pts',(23.1870621950452,-7.64502921715483,
0.));
#217801=CARTESIAN_POINT('Ctrl Pts',(23.1870621950452,-7.64502921715483,
12.));
#217802=CARTESIAN_POINT('Ctrl Pts',(23.1638813796691,-7.64673306975797,
0.));
#217803=CARTESIAN_POINT('Ctrl Pts',(23.1638813796691,-7.64673306975797,
12.));
#217804=CARTESIAN_POINT('Ctrl Pts',(23.1407868853815,-7.64837264482929,
0.));
#217805=CARTESIAN_POINT('Ctrl Pts',(23.1407868853815,-7.64837264482929,
12.));
#217806=CARTESIAN_POINT('Ctrl Pts',(23.1177793581674,-7.64994822749845,
0.));
#217807=CARTESIAN_POINT('Ctrl Pts',(23.1177793581674,-7.64994822749845,
12.));
#217808=CARTESIAN_POINT('Ctrl Pts',(23.0948594495246,-7.65146010690465,
0.));
#217809=CARTESIAN_POINT('Ctrl Pts',(23.0948594495246,-7.65146010690465,
12.));
#217810=CARTESIAN_POINT('Ctrl Pts',(23.072027816555,-7.65290857626357,0.));
#217811=CARTESIAN_POINT('Ctrl Pts',(23.072027816555,-7.65290857626357,12.));
#217812=CARTESIAN_POINT('Ctrl Pts',(23.049285122053,-7.65429393293955,0.));
#217813=CARTESIAN_POINT('Ctrl Pts',(23.049285122053,-7.65429393293955,12.));
#217814=CARTESIAN_POINT('Ctrl Pts',(23.0266320345792,-7.65561647852555,
0.));
#217815=CARTESIAN_POINT('Ctrl Pts',(23.0266320345792,-7.65561647852555,
12.));
#217816=CARTESIAN_POINT('Ctrl Pts',(23.004069228582,-7.6568765189133,0.));
#217817=CARTESIAN_POINT('Ctrl Pts',(23.004069228582,-7.6568765189133,12.));
#217818=CARTESIAN_POINT('Ctrl Pts',(22.9815973845301,-7.65807436436453,
0.));
#217819=CARTESIAN_POINT('Ctrl Pts',(22.9815973845301,-7.65807436436453,
12.));
#217820=CARTESIAN_POINT('Ctrl Pts',(22.9592171890332,-7.65921032958912,
0.));
#217821=CARTESIAN_POINT('Ctrl Pts',(22.9592171890332,-7.65921032958912,
12.));
#217822=CARTESIAN_POINT('Ctrl Pts',(22.9369293349592,-7.66028473382777,
0.));
#217823=CARTESIAN_POINT('Ctrl Pts',(22.9369293349592,-7.66028473382777,
12.));
#217824=CARTESIAN_POINT('Ctrl Pts',(22.9147345215418,-7.661297900941,0.));
#217825=CARTESIAN_POINT('Ctrl Pts',(22.9147345215418,-7.661297900941,12.));
#217826=CARTESIAN_POINT('Ctrl Pts',(22.8926334544879,-7.66225015950148,
0.));
#217827=CARTESIAN_POINT('Ctrl Pts',(22.8926334544879,-7.66225015950148,
12.));
#217828=CARTESIAN_POINT('Ctrl Pts',(22.870626846128,-7.66314184287334,0.));
#217829=CARTESIAN_POINT('Ctrl Pts',(22.870626846128,-7.66314184287334,12.));
#217830=CARTESIAN_POINT('Ctrl Pts',(22.8487154155569,-7.66397328929805,
0.));
#217831=CARTESIAN_POINT('Ctrl Pts',(22.8487154155569,-7.66397328929805,
12.));
#217832=CARTESIAN_POINT('Ctrl Pts',(22.8268998887678,-7.66474484198553,
0.));
#217833=CARTESIAN_POINT('Ctrl Pts',(22.8268998887678,-7.66474484198553,
12.));
#217834=CARTESIAN_POINT('Ctrl Pts',(22.8051809987833,-7.66545684920988,
0.));
#217835=CARTESIAN_POINT('Ctrl Pts',(22.8051809987833,-7.66545684920988,
12.));
#217836=CARTESIAN_POINT('Ctrl Pts',(22.7835594857697,-7.66610966441259,
0.));
#217837=CARTESIAN_POINT('Ctrl Pts',(22.7835594857697,-7.66610966441259,
12.));
#217838=CARTESIAN_POINT('Ctrl Pts',(22.7620360971839,-7.66670364630273,
0.));
#217839=CARTESIAN_POINT('Ctrl Pts',(22.7620360971839,-7.66670364630273,
12.));
#217840=CARTESIAN_POINT('Ctrl Pts',(22.7406115879508,-7.66723915895413,
0.));
#217841=CARTESIAN_POINT('Ctrl Pts',(22.7406115879508,-7.66723915895413,
12.));
#217842=CARTESIAN_POINT('Ctrl Pts',(22.7192867206242,-7.6677165719101,0.));
#217843=CARTESIAN_POINT('Ctrl Pts',(22.7192867206242,-7.6677165719101,12.));
#217844=CARTESIAN_POINT('Ctrl Pts',(22.6980622655446,-7.66813626029277,
0.));
#217845=CARTESIAN_POINT('Ctrl Pts',(22.6980622655446,-7.66813626029277,
12.));
#217846=CARTESIAN_POINT('Ctrl Pts',(22.6769390009889,-7.66849860491763,
0.));
#217847=CARTESIAN_POINT('Ctrl Pts',(22.6769390009889,-7.66849860491763,
12.));
#217848=CARTESIAN_POINT('Ctrl Pts',(22.6559177133133,-7.66880399241354,
0.));
#217849=CARTESIAN_POINT('Ctrl Pts',(22.6559177133133,-7.66880399241354,
12.));
#217850=CARTESIAN_POINT('Ctrl Pts',(22.6349991971547,-7.66905281533745,
0.));
#217851=CARTESIAN_POINT('Ctrl Pts',(22.6349991971547,-7.66905281533745,
12.));
#217852=CARTESIAN_POINT('Ctrl Pts',(22.6141842556248,-7.66924547229435,
0.));
#217853=CARTESIAN_POINT('Ctrl Pts',(22.6141842556248,-7.66924547229435,
12.));
#217854=CARTESIAN_POINT('Ctrl Pts',(22.5934737004955,-7.66938236806241,
0.));
#217855=CARTESIAN_POINT('Ctrl Pts',(22.5934737004955,-7.66938236806241,
12.));
#217856=CARTESIAN_POINT('Ctrl Pts',(22.5728683523828,-7.66946391372299,
0.));
#217857=CARTESIAN_POINT('Ctrl Pts',(22.5728683523828,-7.66946391372299,
12.));
#217858=CARTESIAN_POINT('Ctrl Pts',(22.5523690409109,-7.66949052679672,
0.));
#217859=CARTESIAN_POINT('Ctrl Pts',(22.5523690409109,-7.66949052679672,
12.));
#217860=CARTESIAN_POINT('Ctrl Pts',(22.5319766049191,-7.66946263138116,
0.));
#217861=CARTESIAN_POINT('Ctrl Pts',(22.5319766049191,-7.66946263138116,
12.));
#217862=CARTESIAN_POINT('Ctrl Pts',(22.5116918927023,-7.66938065829083,
0.));
#217863=CARTESIAN_POINT('Ctrl Pts',(22.5116918927023,-7.66938065829083,
12.));
#217864=CARTESIAN_POINT('Ctrl Pts',(22.4915157622308,-7.66924504520302,
0.));
#217865=CARTESIAN_POINT('Ctrl Pts',(22.4915157622308,-7.66924504520302,
12.));
#217866=CARTESIAN_POINT('Ctrl Pts',(22.47144908137,-7.66905623680836,0.));
#217867=CARTESIAN_POINT('Ctrl Pts',(22.47144908137,-7.66905623680836,12.));
#217868=CARTESIAN_POINT('Ctrl Pts',(22.4514927280862,-7.6688146849666,0.));
#217869=CARTESIAN_POINT('Ctrl Pts',(22.4514927280862,-7.6688146849666,12.));
#217870=CARTESIAN_POINT('Ctrl Pts',(22.4316475906616,-7.66852084886746,
0.));
#217871=CARTESIAN_POINT('Ctrl Pts',(22.4316475906616,-7.66852084886746,
12.));
#217872=CARTESIAN_POINT('Ctrl Pts',(22.411914567977,-7.66817519519682,0.));
#217873=CARTESIAN_POINT('Ctrl Pts',(22.411914567977,-7.66817519519682,12.));
#217874=CARTESIAN_POINT('Ctrl Pts',(22.3922945697782,-7.6677781983082,0.));
#217875=CARTESIAN_POINT('Ctrl Pts',(22.3922945697782,-7.6677781983082,12.));
#217876=CARTESIAN_POINT('Ctrl Pts',(22.3727885169361,-7.66733034039887,
0.));
#217877=CARTESIAN_POINT('Ctrl Pts',(22.3727885169361,-7.66733034039887,
12.));
#217878=CARTESIAN_POINT('Ctrl Pts',(22.3533973417013,-7.66683211169134,
0.));
#217879=CARTESIAN_POINT('Ctrl Pts',(22.3533973417013,-7.66683211169134,
12.));
#217880=CARTESIAN_POINT('Ctrl Pts',(22.3341219879454,-7.66628401061906,
0.));
#217881=CARTESIAN_POINT('Ctrl Pts',(22.3341219879454,-7.66628401061906,
12.));
#217882=CARTESIAN_POINT('Ctrl Pts',(22.3149634114823,-7.66568654402442,
0.));
#217883=CARTESIAN_POINT('Ctrl Pts',(22.3149634114823,-7.66568654402442,
12.));
#217884=CARTESIAN_POINT('Ctrl Pts',(22.2959225803925,-7.66504022736263,
0.));
#217885=CARTESIAN_POINT('Ctrl Pts',(22.2959225803925,-7.66504022736263,
12.));
#217886=CARTESIAN_POINT('Ctrl Pts',(22.2770004753332,-7.66434558490973,
0.));
#217887=CARTESIAN_POINT('Ctrl Pts',(22.2770004753332,-7.66434558490973,
12.));
#217888=CARTESIAN_POINT('Ctrl Pts',(22.2581980898487,-7.66360314997662,
0.));
#217889=CARTESIAN_POINT('Ctrl Pts',(22.2581980898487,-7.66360314997662,
12.));
#217890=CARTESIAN_POINT('Ctrl Pts',(22.239516430656,-7.66281346512546,0.));
#217891=CARTESIAN_POINT('Ctrl Pts',(22.239516430656,-7.66281346512546,12.));
#217892=CARTESIAN_POINT('Ctrl Pts',(22.2209565180098,-7.66197708240436,
0.));
#217893=CARTESIAN_POINT('Ctrl Pts',(22.2209565180098,-7.66197708240436,
12.));
#217894=CARTESIAN_POINT('Ctrl Pts',(22.2025193860972,-7.66109456359292,
0.));
#217895=CARTESIAN_POINT('Ctrl Pts',(22.2025193860972,-7.66109456359292,
12.));
#217896=CARTESIAN_POINT('Ctrl Pts',(22.1842060834092,-7.66016648045008,
0.));
#217897=CARTESIAN_POINT('Ctrl Pts',(22.1842060834092,-7.66016648045008,
12.));
#217898=CARTESIAN_POINT('Ctrl Pts',(22.1660176731174,-7.65919341496926,
0.));
#217899=CARTESIAN_POINT('Ctrl Pts',(22.1660176731174,-7.65919341496926,
12.));
#217900=CARTESIAN_POINT('Ctrl Pts',(22.1479552334206,-7.65817595963351,
0.));
#217901=CARTESIAN_POINT('Ctrl Pts',(22.1479552334206,-7.65817595963351,
12.));
#217902=CARTESIAN_POINT('Ctrl Pts',(22.1300198579671,-7.65711471769407,
0.));
#217903=CARTESIAN_POINT('Ctrl Pts',(22.1300198579671,-7.65711471769407,
12.));
#217904=CARTESIAN_POINT('Ctrl Pts',(22.1122126563327,-7.65601030346819,
0.));
#217905=CARTESIAN_POINT('Ctrl Pts',(22.1122126563327,-7.65601030346819,
12.));
#217906=CARTESIAN_POINT('Ctrl Pts',(22.094534754469,-7.65486334263651,0.));
#217907=CARTESIAN_POINT('Ctrl Pts',(22.094534754469,-7.65486334263651,12.));
#217908=CARTESIAN_POINT('Ctrl Pts',(22.0769872951596,-7.65367447254945,
0.));
#217909=CARTESIAN_POINT('Ctrl Pts',(22.0769872951596,-7.65367447254945,
12.));
#217910=CARTESIAN_POINT('Ctrl Pts',(22.0595714384432,-7.65244434253104,
0.));
#217911=CARTESIAN_POINT('Ctrl Pts',(22.0595714384432,-7.65244434253104,
12.));
#217912=CARTESIAN_POINT('Ctrl Pts',(22.0422883621176,-7.65117361421347,
0.));
#217913=CARTESIAN_POINT('Ctrl Pts',(22.0422883621176,-7.65117361421347,
12.));
#217914=CARTESIAN_POINT('Ctrl Pts',(22.0251392623209,-7.64986296190157,
0.));
#217915=CARTESIAN_POINT('Ctrl Pts',(22.0251392623209,-7.64986296190157,
12.));
#217916=CARTESIAN_POINT('Ctrl Pts',(22.0081253540773,-7.64851307293346,
0.));
#217917=CARTESIAN_POINT('Ctrl Pts',(22.0081253540773,-7.64851307293346,
12.));
#217918=CARTESIAN_POINT('Ctrl Pts',(21.9912478718542,-7.64712464805258,
0.));
#217919=CARTESIAN_POINT('Ctrl Pts',(21.9912478718542,-7.64712464805258,
12.));
#217920=CARTESIAN_POINT('Ctrl Pts',(21.97450807008,-7.64569840177359,0.));
#217921=CARTESIAN_POINT('Ctrl Pts',(21.97450807008,-7.64569840177359,12.));
#217922=CARTESIAN_POINT('Ctrl Pts',(21.9579072237653,-7.64423506279154,
0.));
#217923=CARTESIAN_POINT('Ctrl Pts',(21.9579072237653,-7.64423506279154,
12.));
#217924=CARTESIAN_POINT('Ctrl Pts',(21.9414466292074,-7.64273537442707,
0.));
#217925=CARTESIAN_POINT('Ctrl Pts',(21.9414466292074,-7.64273537442707,
12.));
#217926=CARTESIAN_POINT('Ctrl Pts',(21.9251276046546,-7.6412000950654,0.));
#217927=CARTESIAN_POINT('Ctrl Pts',(21.9251276046546,-7.6412000950654,12.));
#217928=CARTESIAN_POINT('Ctrl Pts',(21.9089514909873,-7.63962999860917,
0.));
#217929=CARTESIAN_POINT('Ctrl Pts',(21.9089514909873,-7.63962999860917,
12.));
#217930=CARTESIAN_POINT('Ctrl Pts',(21.8929196523511,-7.63802587492008,
0.));
#217931=CARTESIAN_POINT('Ctrl Pts',(21.8929196523511,-7.63802587492008,
12.));
#217932=CARTESIAN_POINT('Ctrl Pts',(21.8770334769492,-7.63638853033368,
0.));
#217933=CARTESIAN_POINT('Ctrl Pts',(21.8770334769492,-7.63638853033368,
12.));
#217934=CARTESIAN_POINT('Ctrl Pts',(21.8612943779086,-7.63471878821204,
0.));
#217935=CARTESIAN_POINT('Ctrl Pts',(21.8612943779086,-7.63471878821204,
12.));
#217936=CARTESIAN_POINT('Ctrl Pts',(21.8457037941084,-7.63301748948936,
0.));
#217937=CARTESIAN_POINT('Ctrl Pts',(21.8457037941084,-7.63301748948936,
12.));
#217938=CARTESIAN_POINT('Ctrl Pts',(21.8302631910197,-7.6312854932304,0.));
#217939=CARTESIAN_POINT('Ctrl Pts',(21.8302631910197,-7.6312854932304,12.));
#217940=CARTESIAN_POINT('Ctrl Pts',(21.8149740615093,-7.62952367718151,
0.));
#217941=CARTESIAN_POINT('Ctrl Pts',(21.8149740615093,-7.62952367718151,
12.));
#217942=CARTESIAN_POINT('Ctrl Pts',(21.7998379268583,-7.62773293842409,
0.));
#217943=CARTESIAN_POINT('Ctrl Pts',(21.7998379268583,-7.62773293842409,
12.));
#217944=CARTESIAN_POINT('Ctrl Pts',(21.7848563378022,-7.62591419404521,
0.));
#217945=CARTESIAN_POINT('Ctrl Pts',(21.7848563378022,-7.62591419404521,
12.));
#217946=CARTESIAN_POINT('Ctrl Pts',(21.7700308755583,-7.62406838181164,
0.));
#217947=CARTESIAN_POINT('Ctrl Pts',(21.7700308755583,-7.62406838181164,
12.));
#217948=CARTESIAN_POINT('Ctrl Pts',(21.7553631528329,-7.62219646084226,
0.));
#217949=CARTESIAN_POINT('Ctrl Pts',(21.7553631528329,-7.62219646084226,
12.));
#217950=CARTESIAN_POINT('Ctrl Pts',(21.7408548148657,-7.62029941230855,
0.));
#217951=CARTESIAN_POINT('Ctrl Pts',(21.7408548148657,-7.62029941230855,
12.));
#217952=CARTESIAN_POINT('Ctrl Pts',(21.7265075407977,-7.61837824030542,
0.));
#217953=CARTESIAN_POINT('Ctrl Pts',(21.7265075407977,-7.61837824030542,
12.));
#217954=CARTESIAN_POINT('Ctrl Pts',(21.7123230449835,-7.61643397270425,
0.));
#217955=CARTESIAN_POINT('Ctrl Pts',(21.7123230449835,-7.61643397270425,
12.));
#217956=CARTESIAN_POINT('Ctrl Pts',(21.6983030783321,-7.61446766202787,
0.));
#217957=CARTESIAN_POINT('Ctrl Pts',(21.6983030783321,-7.61446766202787,
12.));
#217958=CARTESIAN_POINT('Ctrl Pts',(21.6844494295813,-7.61248038630265,
0.));
#217959=CARTESIAN_POINT('Ctrl Pts',(21.6844494295813,-7.61248038630265,
12.));
#217960=CARTESIAN_POINT('Ctrl Pts',(21.6707639267573,-7.6104732500095,0.));
#217961=CARTESIAN_POINT('Ctrl Pts',(21.6707639267573,-7.6104732500095,12.));
#217962=CARTESIAN_POINT('Ctrl Pts',(21.6572484388079,-7.60844738512872,
0.));
#217963=CARTESIAN_POINT('Ctrl Pts',(21.6572484388079,-7.60844738512872,
12.));
#217964=CARTESIAN_POINT('Ctrl Pts',(21.6439048771743,-7.60640395216359,
0.));
#217965=CARTESIAN_POINT('Ctrl Pts',(21.6439048771743,-7.60640395216359,
12.));
#217966=CARTESIAN_POINT('Ctrl Pts',(21.6307351973823,-7.604344141183,0.));
#217967=CARTESIAN_POINT('Ctrl Pts',(21.6307351973823,-7.604344141183,12.));
#217968=CARTESIAN_POINT('Ctrl Pts',(21.6177414005991,-7.60226917285432,
0.));
#217969=CARTESIAN_POINT('Ctrl Pts',(21.6177414005991,-7.60226917285432,
12.));
#217970=CARTESIAN_POINT('Ctrl Pts',(21.6049255358842,-7.60018029988238,
0.));
#217971=CARTESIAN_POINT('Ctrl Pts',(21.6049255358842,-7.60018029988238,
12.));
#217972=CARTESIAN_POINT('Ctrl Pts',(21.5922897024466,-7.59807880846193,
0.));
#217973=CARTESIAN_POINT('Ctrl Pts',(21.5922897024466,-7.59807880846193,
12.));
#217974=CARTESIAN_POINT('Ctrl Pts',(21.5798360518978,-7.59596601973589,
0.));
#217975=CARTESIAN_POINT('Ctrl Pts',(21.5798360518978,-7.59596601973589,
12.));
#217976=CARTESIAN_POINT('Ctrl Pts',(21.5675667904728,-7.5938432912493,0.));
#217977=CARTESIAN_POINT('Ctrl Pts',(21.5675667904728,-7.5938432912493,12.));
#217978=CARTESIAN_POINT('Ctrl Pts',(21.5554841813465,-7.59171201844793,
0.));
#217979=CARTESIAN_POINT('Ctrl Pts',(21.5554841813465,-7.59171201844793,
12.));
#217980=CARTESIAN_POINT('Ctrl Pts',(21.5435905470113,-7.58957363620026,
0.));
#217981=CARTESIAN_POINT('Ctrl Pts',(21.5435905470113,-7.58957363620026,
12.));
#217982=CARTESIAN_POINT('Ctrl Pts',(21.5318882716735,-7.58742962034834,
0.));
#217983=CARTESIAN_POINT('Ctrl Pts',(21.5318882716735,-7.58742962034834,
12.));
#217984=CARTESIAN_POINT('Ctrl Pts',(21.5203798035294,-7.58528148919114,
0.));
#217985=CARTESIAN_POINT('Ctrl Pts',(21.5203798035294,-7.58528148919114,
12.));
#217986=CARTESIAN_POINT('Ctrl Pts',(21.5090676573866,-7.58313080519159,
0.));
#217987=CARTESIAN_POINT('Ctrl Pts',(21.5090676573866,-7.58313080519159,
12.));
#217988=CARTESIAN_POINT('Ctrl Pts',(21.4979544192739,-7.5809791779073,0.));
#217989=CARTESIAN_POINT('Ctrl Pts',(21.4979544192739,-7.5809791779073,12.));
#217990=CARTESIAN_POINT('Ctrl Pts',(21.4870427508193,-7.57882826679131,
0.));
#217991=CARTESIAN_POINT('Ctrl Pts',(21.4870427508193,-7.57882826679131,
12.));
#217992=CARTESIAN_POINT('Ctrl Pts',(21.4763353936766,-7.57667978403003,
0.));
#217993=CARTESIAN_POINT('Ctrl Pts',(21.4763353936766,-7.57667978403003,
12.));
#217994=CARTESIAN_POINT('Ctrl Pts',(21.4658351740135,-7.57453549743435,
0.));
#217995=CARTESIAN_POINT('Ctrl Pts',(21.4658351740135,-7.57453549743435,
12.));
#217996=CARTESIAN_POINT('Ctrl Pts',(21.4555450053147,-7.57239723223521,
0.));
#217997=CARTESIAN_POINT('Ctrl Pts',(21.4555450053147,-7.57239723223521,
12.));
#217998=CARTESIAN_POINT('Ctrl Pts',(21.445467890751,-7.5702668726117,0.));
#217999=CARTESIAN_POINT('Ctrl Pts',(21.445467890751,-7.5702668726117,12.));
#218000=CARTESIAN_POINT('Ctrl Pts',(21.435606926151,-7.56814636360842,0.));
#218001=CARTESIAN_POINT('Ctrl Pts',(21.435606926151,-7.56814636360842,12.));
#218002=CARTESIAN_POINT('Ctrl Pts',(21.4259653015732,-7.56603771218706,
0.));
#218003=CARTESIAN_POINT('Ctrl Pts',(21.4259653015732,-7.56603771218706,
12.));
#218004=CARTESIAN_POINT('Ctrl Pts',(21.4165463106252,-7.56394299313683,
0.));
#218005=CARTESIAN_POINT('Ctrl Pts',(21.4165463106252,-7.56394299313683,
12.));
#218006=CARTESIAN_POINT('Ctrl Pts',(21.4073533630364,-7.56186435703622,
0.));
#218007=CARTESIAN_POINT('Ctrl Pts',(21.4073533630364,-7.56186435703622,
12.));
#218008=CARTESIAN_POINT('Ctrl Pts',(21.3983899952988,-7.55980403700615,
0.));
#218009=CARTESIAN_POINT('Ctrl Pts',(21.3983899952988,-7.55980403700615,
12.));
#218010=CARTESIAN_POINT('Ctrl Pts',(21.3896598842119,-7.55776435731422,
0.));
#218011=CARTESIAN_POINT('Ctrl Pts',(21.3896598842119,-7.55776435731422,
12.));
#218012=CARTESIAN_POINT('Ctrl Pts',(21.3811668478933,-7.55574773403508,
0.));
#218013=CARTESIAN_POINT('Ctrl Pts',(21.3811668478933,-7.55574773403508,
12.));
#218014=CARTESIAN_POINT('Ctrl Pts',(21.3729148390244,-7.55375667080032,
0.));
#218015=CARTESIAN_POINT('Ctrl Pts',(21.3729148390244,-7.55375667080032,
12.));
#218016=CARTESIAN_POINT('Ctrl Pts',(21.3649079431864,-7.55179375777442,
0.));
#218017=CARTESIAN_POINT('Ctrl Pts',(21.3649079431864,-7.55179375777442,
12.));
#218018=CARTESIAN_POINT('Ctrl Pts',(21.3571503685853,-7.54986166521307,
0.));
#218019=CARTESIAN_POINT('Ctrl Pts',(21.3571503685853,-7.54986166521307,
12.));
#218020=CARTESIAN_POINT('Ctrl Pts',(21.349646476153,-7.54796316246327,0.));
#218021=CARTESIAN_POINT('Ctrl Pts',(21.349646476153,-7.54796316246327,12.));
#218022=CARTESIAN_POINT('Ctrl Pts',(21.3424008295038,-7.54610114948351,
0.));
#218023=CARTESIAN_POINT('Ctrl Pts',(21.3424008295038,-7.54610114948351,
12.));
#218024=CARTESIAN_POINT('Ctrl Pts',(21.3354182340149,-7.54427868151269,
0.));
#218025=CARTESIAN_POINT('Ctrl Pts',(21.3354182340149,-7.54427868151269,
12.));
#218026=CARTESIAN_POINT('Ctrl Pts',(21.328703791771,-7.54249900377032,0.));
#218027=CARTESIAN_POINT('Ctrl Pts',(21.328703791771,-7.54249900377032,12.));
#218028=CARTESIAN_POINT('Ctrl Pts',(21.3222628524165,-7.5407655203828,0.));
#218029=CARTESIAN_POINT('Ctrl Pts',(21.3222628524165,-7.5407655203828,12.));
#218030=CARTESIAN_POINT('Ctrl Pts',(21.3161009456256,-7.53908175169899,
0.));
#218031=CARTESIAN_POINT('Ctrl Pts',(21.3161009456256,-7.53908175169899,
12.));
#218032=CARTESIAN_POINT('Ctrl Pts',(21.3102237167729,-7.5374512936462,0.));
#218033=CARTESIAN_POINT('Ctrl Pts',(21.3102237167729,-7.5374512936462,12.));
#218034=CARTESIAN_POINT('Ctrl Pts',(21.3046368712156,-7.53587778251743,
0.));
#218035=CARTESIAN_POINT('Ctrl Pts',(21.3046368712156,-7.53587778251743,
12.));
#218036=CARTESIAN_POINT('Ctrl Pts',(21.2993464250717,-7.53436505309949,
0.));
#218037=CARTESIAN_POINT('Ctrl Pts',(21.2993464250717,-7.53436505309949,
12.));
#218038=CARTESIAN_POINT('Ctrl Pts',(21.2943588989331,-7.53291726078527,
0.));
#218039=CARTESIAN_POINT('Ctrl Pts',(21.2943588989331,-7.53291726078527,
12.));
#218040=CARTESIAN_POINT('Ctrl Pts',(21.2896816163843,-7.53153906987847,
0.));
#218041=CARTESIAN_POINT('Ctrl Pts',(21.2896816163843,-7.53153906987847,
12.));
#218042=CARTESIAN_POINT('Ctrl Pts',(21.2853226580658,-7.53023562438221,
0.));
#218043=CARTESIAN_POINT('Ctrl Pts',(21.2853226580658,-7.53023562438221,
12.));
#218044=CARTESIAN_POINT('Ctrl Pts',(21.2812902781143,-7.52901217930407,
0.));
#218045=CARTESIAN_POINT('Ctrl Pts',(21.2812902781143,-7.52901217930407,
12.));
#218046=CARTESIAN_POINT('Ctrl Pts',(21.2775925269651,-7.52787386225344,
0.));
#218047=CARTESIAN_POINT('Ctrl Pts',(21.2775925269651,-7.52787386225344,
12.));
#218048=CARTESIAN_POINT('Ctrl Pts',(21.2742366113578,-7.52682526918561,
0.));
#218049=CARTESIAN_POINT('Ctrl Pts',(21.2742366113578,-7.52682526918561,
12.));
#218050=CARTESIAN_POINT('Ctrl Pts',(21.2712301573465,-7.52587126095544,
0.));
#218051=CARTESIAN_POINT('Ctrl Pts',(21.2712301573465,-7.52587126095544,
12.));
#218052=CARTESIAN_POINT('Ctrl Pts',(21.2685823838672,-7.52501770333522,
0.));
#218053=CARTESIAN_POINT('Ctrl Pts',(21.2685823838672,-7.52501770333522,
12.));
#218054=CARTESIAN_POINT('Ctrl Pts',(21.266305915706,-7.52427261074264,0.));
#218055=CARTESIAN_POINT('Ctrl Pts',(21.266305915706,-7.52427261074264,12.));
#218056=CARTESIAN_POINT('Ctrl Pts',(21.2644161259965,-7.52364573027521,
0.));
#218057=CARTESIAN_POINT('Ctrl Pts',(21.2644161259965,-7.52364573027521,
12.));
#218058=CARTESIAN_POINT('Ctrl Pts',(21.262927782038,-7.52314642316203,0.));
#218059=CARTESIAN_POINT('Ctrl Pts',(21.262927782038,-7.52314642316203,12.));
#218060=CARTESIAN_POINT('Ctrl Pts',(21.261852128355,-7.52278182242728,0.));
#218061=CARTESIAN_POINT('Ctrl Pts',(21.261852128355,-7.52278182242728,12.));
#218062=CARTESIAN_POINT('Ctrl Pts',(21.2613260540651,-7.52260064231736,
0.));
#218063=CARTESIAN_POINT('Ctrl Pts',(21.2613260540651,-7.52260064231736,
12.));
#218064=CARTESIAN_POINT('Ctrl Pts',(21.261120447486,-7.52252744144958,0.));
#218065=CARTESIAN_POINT('Ctrl Pts',(21.261120447486,-7.52252744144958,12.));
#218066=CARTESIAN_POINT('Ctrl Pts',(21.2610673466883,-7.52250649703992,
0.));
#218067=CARTESIAN_POINT('Ctrl Pts',(21.2610673466883,-7.52250649703992,
12.));
#218068=CARTESIAN_POINT('Ctrl Pts',(21.2610617890679,-7.52250298901266,
0.));
#218069=CARTESIAN_POINT('Ctrl Pts',(21.2610617890679,-7.52250298901266,
12.));
#218070=CARTESIAN_POINT('',(24.9347862158358,-7.36589684767345,0.));
#218071=CARTESIAN_POINT('Ctrl Pts',(24.9347862158358,-7.36589684767345,
0.));
#218072=CARTESIAN_POINT('Ctrl Pts',(24.9292275670674,-7.36721909028843,
0.));
#218073=CARTESIAN_POINT('Ctrl Pts',(24.9181155530543,-7.36985593120091,
0.));
#218074=CARTESIAN_POINT('Ctrl Pts',(24.901463382605,-7.37378825961676,0.));
#218075=CARTESIAN_POINT('Ctrl Pts',(24.8792921911115,-7.3789854964027,0.));
#218076=CARTESIAN_POINT('Ctrl Pts',(24.8516310625176,-7.38540558903621,
0.));
#218077=CARTESIAN_POINT('Ctrl Pts',(24.8240228520893,-7.39174922585809,
0.));
#218078=CARTESIAN_POINT('Ctrl Pts',(24.7964676646431,-7.39801641583013,
0.));
#218079=CARTESIAN_POINT('Ctrl Pts',(24.7689656668983,-7.40420718661603,
0.));
#218080=CARTESIAN_POINT('Ctrl Pts',(24.7415170994784,-7.41032159082382,
0.));
#218081=CARTESIAN_POINT('Ctrl Pts',(24.7141222950051,-7.41635971481674,
0.));
#218082=CARTESIAN_POINT('Ctrl Pts',(24.6867816727192,-7.42232167766266,
0.));
#218083=CARTESIAN_POINT('Ctrl Pts',(24.6594957128756,-7.42820762159126,
0.));
#218084=CARTESIAN_POINT('Ctrl Pts',(24.6322649369517,-7.43401770489524,
0.));
#218085=CARTESIAN_POINT('Ctrl Pts',(24.6050898852368,-7.43975209375504,
0.));
#218086=CARTESIAN_POINT('Ctrl Pts',(24.577971096086,-7.44541095473135,0.));
#218087=CARTESIAN_POINT('Ctrl Pts',(24.5509090831559,-7.4509944465116,0.));
#218088=CARTESIAN_POINT('Ctrl Pts',(24.5239043173072,-7.45650271335862,
0.));
#218089=CARTESIAN_POINT('Ctrl Pts',(24.4969572391483,-7.46193588961464,
0.));
#218090=CARTESIAN_POINT('Ctrl Pts',(24.4700682684524,-7.46729410308787,
0.));
#218091=CARTESIAN_POINT('Ctrl Pts',(24.443237814649,-7.47257747883246,0.));
#218092=CARTESIAN_POINT('Ctrl Pts',(24.4164662871163,-7.47778614286565,
0.));
#218093=CARTESIAN_POINT('Ctrl Pts',(24.3897541049254,-7.48292022569301,
0.));
#218094=CARTESIAN_POINT('Ctrl Pts',(24.3631017084524,-7.48797986651909,
0.));
#218095=CARTESIAN_POINT('Ctrl Pts',(24.3365095573685,-7.49296521252421,
0.));
#218096=CARTESIAN_POINT('Ctrl Pts',(24.3099781253355,-7.49787641695439,
0.));
#218097=CARTESIAN_POINT('Ctrl Pts',(24.2835078958973,-7.50271363765152,
0.));
#218098=CARTESIAN_POINT('Ctrl Pts',(24.2570993577034,-7.50747703535134,
0.));
#218099=CARTESIAN_POINT('Ctrl Pts',(24.2307530003887,-7.51216677222181,
0.));
#218100=CARTESIAN_POINT('Ctrl Pts',(24.2044693092349,-7.51678300997949,
0.));
#218101=CARTESIAN_POINT('Ctrl Pts',(24.1782487641594,-7.52132590953802,
0.));
#218102=CARTESIAN_POINT('Ctrl Pts',(24.1520918425364,-7.52579563201424,
0.));
#218103=CARTESIAN_POINT('Ctrl Pts',(24.1259990209207,-7.53019233935502,
0.));
#218104=CARTESIAN_POINT('Ctrl Pts',(24.0999707772642,-7.53451619514649,
0.));
#218105=CARTESIAN_POINT('Ctrl Pts',(24.0740075927985,-7.53876736531014,
0.));
#218106=CARTESIAN_POINT('Ctrl Pts',(24.0481099543353,-7.54294601896145,
0.));
#218107=CARTESIAN_POINT('Ctrl Pts',(24.022278355453,-7.5470523288591,0.));
#218108=CARTESIAN_POINT('Ctrl Pts',(23.9965132953185,-7.55108647097441,
0.));
#218109=CARTESIAN_POINT('Ctrl Pts',(23.9708152779884,-7.55504862424812,
0.));
#218110=CARTESIAN_POINT('Ctrl Pts',(23.9451848115,-7.55893897027683,0.));
#218111=CARTESIAN_POINT('Ctrl Pts',(23.9196224070759,-7.56275769304773,
0.));
#218112=CARTESIAN_POINT('Ctrl Pts',(23.8941285782003,-7.56650497863792,
0.));
#218113=CARTESIAN_POINT('Ctrl Pts',(23.8687038399597,-7.57018101500711,
0.));
#218114=CARTESIAN_POINT('Ctrl Pts',(23.8433487096134,-7.57378599219817,
0.));
#218115=CARTESIAN_POINT('Ctrl Pts',(23.8180637069977,-7.57732010249066,
0.));
#218116=CARTESIAN_POINT('Ctrl Pts',(23.7928493549908,-7.58078354058212,
0.));
#218117=CARTESIAN_POINT('Ctrl Pts',(23.7677061799376,-7.58417650376272,
0.));
#218118=CARTESIAN_POINT('Ctrl Pts',(23.7426347121006,-7.58749919210832,
0.));
#218119=CARTESIAN_POINT('Ctrl Pts',(23.7176354860457,-7.59075180865327,
0.));
#218120=CARTESIAN_POINT('Ctrl Pts',(23.6927090405067,-7.59393455934042,
0.));
#218121=CARTESIAN_POINT('Ctrl Pts',(23.6678559182876,-7.59704765299572,
0.));
#218122=CARTESIAN_POINT('Ctrl Pts',(23.6430766661419,-7.6000913013013,0.));
#218123=CARTESIAN_POINT('Ctrl Pts',(23.6183718346576,-7.60306571877806,
0.));
#218124=CARTESIAN_POINT('Ctrl Pts',(23.5937419781244,-7.60597112277094,
0.));
#218125=CARTESIAN_POINT('Ctrl Pts',(23.5691876544243,-7.608807733446,0.));
#218126=CARTESIAN_POINT('Ctrl Pts',(23.5447094252028,-7.61157577385372,
0.));
#218127=CARTESIAN_POINT('Ctrl Pts',(23.5203078560128,-7.61427546999299,
0.));
#218128=CARTESIAN_POINT('Ctrl Pts',(23.4959835164608,-7.61690705088319,
0.));
#218129=CARTESIAN_POINT('Ctrl Pts',(23.4717369803438,-7.61947074863978,
0.));
#218130=CARTESIAN_POINT('Ctrl Pts',(23.4475688257854,-7.62196679855957,
0.));
#218131=CARTESIAN_POINT('Ctrl Pts',(23.4234796353544,-7.62439543920055,
0.));
#218132=CARTESIAN_POINT('Ctrl Pts',(23.3994699961122,-7.62675691240335,
0.));
#218133=CARTESIAN_POINT('Ctrl Pts',(23.3755404996638,-7.62905146332598,
0.));
#218134=CARTESIAN_POINT('Ctrl Pts',(23.3516917421973,-7.63127934048139,
0.));
#218135=CARTESIAN_POINT('Ctrl Pts',(23.3279243245241,-7.63344079578163,
0.));
#218136=CARTESIAN_POINT('Ctrl Pts',(23.3042388521021,-7.63553608458784,
0.));
#218137=CARTESIAN_POINT('Ctrl Pts',(23.2806359350853,-7.63756546576375,
0.));
#218138=CARTESIAN_POINT('Ctrl Pts',(23.2571161884487,-7.63952920172837,
0.));
#218139=CARTESIAN_POINT('Ctrl Pts',(23.2336802320912,-7.64142755851508,
0.));
#218140=CARTESIAN_POINT('Ctrl Pts',(23.2103286909399,-7.64326080583684,
0.));
#218141=CARTESIAN_POINT('Ctrl Pts',(23.1870621950452,-7.64502921715483,
0.));
#218142=CARTESIAN_POINT('Ctrl Pts',(23.1638813796691,-7.64673306975797,
0.));
#218143=CARTESIAN_POINT('Ctrl Pts',(23.1407868853815,-7.64837264482929,
0.));
#218144=CARTESIAN_POINT('Ctrl Pts',(23.1177793581674,-7.64994822749845,
0.));
#218145=CARTESIAN_POINT('Ctrl Pts',(23.0948594495246,-7.65146010690465,
0.));
#218146=CARTESIAN_POINT('Ctrl Pts',(23.072027816555,-7.65290857626357,0.));
#218147=CARTESIAN_POINT('Ctrl Pts',(23.049285122053,-7.65429393293955,0.));
#218148=CARTESIAN_POINT('Ctrl Pts',(23.0266320345792,-7.65561647852555,
0.));
#218149=CARTESIAN_POINT('Ctrl Pts',(23.004069228582,-7.6568765189133,0.));
#218150=CARTESIAN_POINT('Ctrl Pts',(22.9815973845301,-7.65807436436453,
0.));
#218151=CARTESIAN_POINT('Ctrl Pts',(22.9592171890332,-7.65921032958912,
0.));
#218152=CARTESIAN_POINT('Ctrl Pts',(22.9369293349592,-7.66028473382777,
0.));
#218153=CARTESIAN_POINT('Ctrl Pts',(22.9147345215418,-7.661297900941,0.));
#218154=CARTESIAN_POINT('Ctrl Pts',(22.8926334544879,-7.66225015950148,
0.));
#218155=CARTESIAN_POINT('Ctrl Pts',(22.870626846128,-7.66314184287334,0.));
#218156=CARTESIAN_POINT('Ctrl Pts',(22.8487154155569,-7.66397328929805,
0.));
#218157=CARTESIAN_POINT('Ctrl Pts',(22.8268998887678,-7.66474484198553,
0.));
#218158=CARTESIAN_POINT('Ctrl Pts',(22.8051809987833,-7.66545684920988,
0.));
#218159=CARTESIAN_POINT('Ctrl Pts',(22.7835594857697,-7.66610966441259,
0.));
#218160=CARTESIAN_POINT('Ctrl Pts',(22.7620360971839,-7.66670364630273,
0.));
#218161=CARTESIAN_POINT('Ctrl Pts',(22.7406115879508,-7.66723915895413,
0.));
#218162=CARTESIAN_POINT('Ctrl Pts',(22.7192867206242,-7.6677165719101,0.));
#218163=CARTESIAN_POINT('Ctrl Pts',(22.6980622655446,-7.66813626029277,
0.));
#218164=CARTESIAN_POINT('Ctrl Pts',(22.6769390009889,-7.66849860491763,
0.));
#218165=CARTESIAN_POINT('Ctrl Pts',(22.6559177133133,-7.66880399241354,
0.));
#218166=CARTESIAN_POINT('Ctrl Pts',(22.6349991971547,-7.66905281533745,
0.));
#218167=CARTESIAN_POINT('Ctrl Pts',(22.6141842556248,-7.66924547229435,
0.));
#218168=CARTESIAN_POINT('Ctrl Pts',(22.5934737004955,-7.66938236806241,
0.));
#218169=CARTESIAN_POINT('Ctrl Pts',(22.5728683523828,-7.66946391372299,
0.));
#218170=CARTESIAN_POINT('Ctrl Pts',(22.5523690409109,-7.66949052679672,
0.));
#218171=CARTESIAN_POINT('Ctrl Pts',(22.5319766049191,-7.66946263138116,
0.));
#218172=CARTESIAN_POINT('Ctrl Pts',(22.5116918927023,-7.66938065829083,
0.));
#218173=CARTESIAN_POINT('Ctrl Pts',(22.4915157622308,-7.66924504520302,
0.));
#218174=CARTESIAN_POINT('Ctrl Pts',(22.47144908137,-7.66905623680836,0.));
#218175=CARTESIAN_POINT('Ctrl Pts',(22.4514927280862,-7.6688146849666,0.));
#218176=CARTESIAN_POINT('Ctrl Pts',(22.4316475906616,-7.66852084886746,
0.));
#218177=CARTESIAN_POINT('Ctrl Pts',(22.411914567977,-7.66817519519682,0.));
#218178=CARTESIAN_POINT('Ctrl Pts',(22.3922945697782,-7.6677781983082,0.));
#218179=CARTESIAN_POINT('Ctrl Pts',(22.3727885169361,-7.66733034039887,
0.));
#218180=CARTESIAN_POINT('Ctrl Pts',(22.3533973417013,-7.66683211169134,
0.));
#218181=CARTESIAN_POINT('Ctrl Pts',(22.3341219879454,-7.66628401061906,
0.));
#218182=CARTESIAN_POINT('Ctrl Pts',(22.3149634114823,-7.66568654402442,
0.));
#218183=CARTESIAN_POINT('Ctrl Pts',(22.2959225803925,-7.66504022736263,
0.));
#218184=CARTESIAN_POINT('Ctrl Pts',(22.2770004753332,-7.66434558490973,
0.));
#218185=CARTESIAN_POINT('Ctrl Pts',(22.2581980898487,-7.66360314997662,
0.));
#218186=CARTESIAN_POINT('Ctrl Pts',(22.239516430656,-7.66281346512546,0.));
#218187=CARTESIAN_POINT('Ctrl Pts',(22.2209565180098,-7.66197708240436,
0.));
#218188=CARTESIAN_POINT('Ctrl Pts',(22.2025193860972,-7.66109456359292,
0.));
#218189=CARTESIAN_POINT('Ctrl Pts',(22.1842060834092,-7.66016648045008,
0.));
#218190=CARTESIAN_POINT('Ctrl Pts',(22.1660176731174,-7.65919341496926,
0.));
#218191=CARTESIAN_POINT('Ctrl Pts',(22.1479552334206,-7.65817595963351,
0.));
#218192=CARTESIAN_POINT('Ctrl Pts',(22.1300198579671,-7.65711471769407,
0.));
#218193=CARTESIAN_POINT('Ctrl Pts',(22.1122126563327,-7.65601030346819,
0.));
#218194=CARTESIAN_POINT('Ctrl Pts',(22.094534754469,-7.65486334263651,0.));
#218195=CARTESIAN_POINT('Ctrl Pts',(22.0769872951596,-7.65367447254945,
0.));
#218196=CARTESIAN_POINT('Ctrl Pts',(22.0595714384432,-7.65244434253104,
0.));
#218197=CARTESIAN_POINT('Ctrl Pts',(22.0422883621176,-7.65117361421347,
0.));
#218198=CARTESIAN_POINT('Ctrl Pts',(22.0251392623209,-7.64986296190157,
0.));
#218199=CARTESIAN_POINT('Ctrl Pts',(22.0081253540773,-7.64851307293346,
0.));
#218200=CARTESIAN_POINT('Ctrl Pts',(21.9912478718542,-7.64712464805258,
0.));
#218201=CARTESIAN_POINT('Ctrl Pts',(21.97450807008,-7.64569840177359,0.));
#218202=CARTESIAN_POINT('Ctrl Pts',(21.9579072237653,-7.64423506279154,
0.));
#218203=CARTESIAN_POINT('Ctrl Pts',(21.9414466292074,-7.64273537442707,
0.));
#218204=CARTESIAN_POINT('Ctrl Pts',(21.9251276046546,-7.6412000950654,0.));
#218205=CARTESIAN_POINT('Ctrl Pts',(21.9089514909873,-7.63962999860917,
0.));
#218206=CARTESIAN_POINT('Ctrl Pts',(21.8929196523511,-7.63802587492008,
0.));
#218207=CARTESIAN_POINT('Ctrl Pts',(21.8770334769492,-7.63638853033368,
0.));
#218208=CARTESIAN_POINT('Ctrl Pts',(21.8612943779086,-7.63471878821204,
0.));
#218209=CARTESIAN_POINT('Ctrl Pts',(21.8457037941084,-7.63301748948936,
0.));
#218210=CARTESIAN_POINT('Ctrl Pts',(21.8302631910197,-7.6312854932304,0.));
#218211=CARTESIAN_POINT('Ctrl Pts',(21.8149740615093,-7.62952367718151,
0.));
#218212=CARTESIAN_POINT('Ctrl Pts',(21.7998379268583,-7.62773293842409,
0.));
#218213=CARTESIAN_POINT('Ctrl Pts',(21.7848563378022,-7.62591419404521,
0.));
#218214=CARTESIAN_POINT('Ctrl Pts',(21.7700308755583,-7.62406838181164,
0.));
#218215=CARTESIAN_POINT('Ctrl Pts',(21.7553631528329,-7.62219646084226,
0.));
#218216=CARTESIAN_POINT('Ctrl Pts',(21.7408548148657,-7.62029941230855,
0.));
#218217=CARTESIAN_POINT('Ctrl Pts',(21.7265075407977,-7.61837824030542,
0.));
#218218=CARTESIAN_POINT('Ctrl Pts',(21.7123230449835,-7.61643397270425,
0.));
#218219=CARTESIAN_POINT('Ctrl Pts',(21.6983030783321,-7.61446766202787,
0.));
#218220=CARTESIAN_POINT('Ctrl Pts',(21.6844494295813,-7.61248038630265,
0.));
#218221=CARTESIAN_POINT('Ctrl Pts',(21.6707639267573,-7.6104732500095,0.));
#218222=CARTESIAN_POINT('Ctrl Pts',(21.6572484388079,-7.60844738512872,
0.));
#218223=CARTESIAN_POINT('Ctrl Pts',(21.6439048771743,-7.60640395216359,
0.));
#218224=CARTESIAN_POINT('Ctrl Pts',(21.6307351973823,-7.604344141183,0.));
#218225=CARTESIAN_POINT('Ctrl Pts',(21.6177414005991,-7.60226917285432,
0.));
#218226=CARTESIAN_POINT('Ctrl Pts',(21.6049255358842,-7.60018029988238,
0.));
#218227=CARTESIAN_POINT('Ctrl Pts',(21.5922897024466,-7.59807880846193,
0.));
#218228=CARTESIAN_POINT('Ctrl Pts',(21.5798360518978,-7.59596601973589,
0.));
#218229=CARTESIAN_POINT('Ctrl Pts',(21.5675667904728,-7.5938432912493,0.));
#218230=CARTESIAN_POINT('Ctrl Pts',(21.5554841813465,-7.59171201844793,
0.));
#218231=CARTESIAN_POINT('Ctrl Pts',(21.5435905470113,-7.58957363620026,
0.));
#218232=CARTESIAN_POINT('Ctrl Pts',(21.5318882716735,-7.58742962034834,
0.));
#218233=CARTESIAN_POINT('Ctrl Pts',(21.5203798035294,-7.58528148919114,
0.));
#218234=CARTESIAN_POINT('Ctrl Pts',(21.5090676573866,-7.58313080519159,
0.));
#218235=CARTESIAN_POINT('Ctrl Pts',(21.4979544192739,-7.5809791779073,0.));
#218236=CARTESIAN_POINT('Ctrl Pts',(21.4870427508193,-7.57882826679131,
0.));
#218237=CARTESIAN_POINT('Ctrl Pts',(21.4763353936766,-7.57667978403003,
0.));
#218238=CARTESIAN_POINT('Ctrl Pts',(21.4658351740135,-7.57453549743435,
0.));
#218239=CARTESIAN_POINT('Ctrl Pts',(21.4555450053147,-7.57239723223521,
0.));
#218240=CARTESIAN_POINT('Ctrl Pts',(21.445467890751,-7.5702668726117,0.));
#218241=CARTESIAN_POINT('Ctrl Pts',(21.435606926151,-7.56814636360842,0.));
#218242=CARTESIAN_POINT('Ctrl Pts',(21.4259653015732,-7.56603771218706,
0.));
#218243=CARTESIAN_POINT('Ctrl Pts',(21.4165463106252,-7.56394299313683,
0.));
#218244=CARTESIAN_POINT('Ctrl Pts',(21.4073533630364,-7.56186435703622,
0.));
#218245=CARTESIAN_POINT('Ctrl Pts',(21.3983899952988,-7.55980403700615,
0.));
#218246=CARTESIAN_POINT('Ctrl Pts',(21.3896598842119,-7.55776435731422,
0.));
#218247=CARTESIAN_POINT('Ctrl Pts',(21.3811668478933,-7.55574773403508,
0.));
#218248=CARTESIAN_POINT('Ctrl Pts',(21.3729148390244,-7.55375667080032,
0.));
#218249=CARTESIAN_POINT('Ctrl Pts',(21.3649079431864,-7.55179375777442,
0.));
#218250=CARTESIAN_POINT('Ctrl Pts',(21.3571503685853,-7.54986166521307,
0.));
#218251=CARTESIAN_POINT('Ctrl Pts',(21.349646476153,-7.54796316246327,0.));
#218252=CARTESIAN_POINT('Ctrl Pts',(21.3424008295038,-7.54610114948351,
0.));
#218253=CARTESIAN_POINT('Ctrl Pts',(21.3354182340149,-7.54427868151269,
0.));
#218254=CARTESIAN_POINT('Ctrl Pts',(21.328703791771,-7.54249900377032,0.));
#218255=CARTESIAN_POINT('Ctrl Pts',(21.3222628524165,-7.5407655203828,0.));
#218256=CARTESIAN_POINT('Ctrl Pts',(21.3161009456256,-7.53908175169899,
0.));
#218257=CARTESIAN_POINT('Ctrl Pts',(21.3102237167729,-7.5374512936462,0.));
#218258=CARTESIAN_POINT('Ctrl Pts',(21.3046368712156,-7.53587778251743,
0.));
#218259=CARTESIAN_POINT('Ctrl Pts',(21.2993464250717,-7.53436505309949,
0.));
#218260=CARTESIAN_POINT('Ctrl Pts',(21.2943588989331,-7.53291726078527,
0.));
#218261=CARTESIAN_POINT('Ctrl Pts',(21.2896816163843,-7.53153906987847,
0.));
#218262=CARTESIAN_POINT('Ctrl Pts',(21.2853226580658,-7.53023562438221,
0.));
#218263=CARTESIAN_POINT('Ctrl Pts',(21.2812902781143,-7.52901217930407,
0.));
#218264=CARTESIAN_POINT('Ctrl Pts',(21.2775925269651,-7.52787386225344,
0.));
#218265=CARTESIAN_POINT('Ctrl Pts',(21.2742366113578,-7.52682526918561,
0.));
#218266=CARTESIAN_POINT('Ctrl Pts',(21.2712301573465,-7.52587126095544,
0.));
#218267=CARTESIAN_POINT('Ctrl Pts',(21.2685823838672,-7.52501770333522,
0.));
#218268=CARTESIAN_POINT('Ctrl Pts',(21.266305915706,-7.52427261074264,0.));
#218269=CARTESIAN_POINT('Ctrl Pts',(21.2644161259965,-7.52364573027521,
0.));
#218270=CARTESIAN_POINT('Ctrl Pts',(21.262927782038,-7.52314642316203,0.));
#218271=CARTESIAN_POINT('Ctrl Pts',(21.261852128355,-7.52278182242728,0.));
#218272=CARTESIAN_POINT('Ctrl Pts',(21.2613260540651,-7.52260064231736,
0.));
#218273=CARTESIAN_POINT('Ctrl Pts',(21.261120447486,-7.52252744144958,0.));
#218274=CARTESIAN_POINT('Ctrl Pts',(21.2610673466883,-7.52250649703992,
0.));
#218275=CARTESIAN_POINT('Ctrl Pts',(21.2610617890679,-7.52250298901266,
0.));
#218276=CARTESIAN_POINT('',(24.9347862158358,-7.36589684767345,12.));
#218277=CARTESIAN_POINT('',(24.9347862158358,-7.36589684767345,0.));
#218278=CARTESIAN_POINT('Ctrl Pts',(21.2610617890679,-7.52250298901266,
12.));
#218279=CARTESIAN_POINT('Ctrl Pts',(21.2610673466883,-7.52250649703992,
12.));
#218280=CARTESIAN_POINT('Ctrl Pts',(21.261120447486,-7.52252744144958,12.));
#218281=CARTESIAN_POINT('Ctrl Pts',(21.2613260540651,-7.52260064231736,
12.));
#218282=CARTESIAN_POINT('Ctrl Pts',(21.261852128355,-7.52278182242728,12.));
#218283=CARTESIAN_POINT('Ctrl Pts',(21.262927782038,-7.52314642316203,12.));
#218284=CARTESIAN_POINT('Ctrl Pts',(21.2644161259965,-7.52364573027521,
12.));
#218285=CARTESIAN_POINT('Ctrl Pts',(21.266305915706,-7.52427261074264,12.));
#218286=CARTESIAN_POINT('Ctrl Pts',(21.2685823838672,-7.52501770333522,
12.));
#218287=CARTESIAN_POINT('Ctrl Pts',(21.2712301573465,-7.52587126095544,
12.));
#218288=CARTESIAN_POINT('Ctrl Pts',(21.2742366113578,-7.52682526918561,
12.));
#218289=CARTESIAN_POINT('Ctrl Pts',(21.2775925269651,-7.52787386225344,
12.));
#218290=CARTESIAN_POINT('Ctrl Pts',(21.2812902781143,-7.52901217930407,
12.));
#218291=CARTESIAN_POINT('Ctrl Pts',(21.2853226580658,-7.53023562438221,
12.));
#218292=CARTESIAN_POINT('Ctrl Pts',(21.2896816163843,-7.53153906987847,
12.));
#218293=CARTESIAN_POINT('Ctrl Pts',(21.2943588989331,-7.53291726078527,
12.));
#218294=CARTESIAN_POINT('Ctrl Pts',(21.2993464250717,-7.53436505309949,
12.));
#218295=CARTESIAN_POINT('Ctrl Pts',(21.3046368712156,-7.53587778251743,
12.));
#218296=CARTESIAN_POINT('Ctrl Pts',(21.3102237167729,-7.5374512936462,12.));
#218297=CARTESIAN_POINT('Ctrl Pts',(21.3161009456256,-7.53908175169899,
12.));
#218298=CARTESIAN_POINT('Ctrl Pts',(21.3222628524165,-7.5407655203828,12.));
#218299=CARTESIAN_POINT('Ctrl Pts',(21.328703791771,-7.54249900377032,12.));
#218300=CARTESIAN_POINT('Ctrl Pts',(21.3354182340149,-7.54427868151269,
12.));
#218301=CARTESIAN_POINT('Ctrl Pts',(21.3424008295038,-7.54610114948351,
12.));
#218302=CARTESIAN_POINT('Ctrl Pts',(21.349646476153,-7.54796316246327,12.));
#218303=CARTESIAN_POINT('Ctrl Pts',(21.3571503685853,-7.54986166521307,
12.));
#218304=CARTESIAN_POINT('Ctrl Pts',(21.3649079431864,-7.55179375777442,
12.));
#218305=CARTESIAN_POINT('Ctrl Pts',(21.3729148390244,-7.55375667080032,
12.));
#218306=CARTESIAN_POINT('Ctrl Pts',(21.3811668478933,-7.55574773403508,
12.));
#218307=CARTESIAN_POINT('Ctrl Pts',(21.3896598842119,-7.55776435731422,
12.));
#218308=CARTESIAN_POINT('Ctrl Pts',(21.3983899952988,-7.55980403700615,
12.));
#218309=CARTESIAN_POINT('Ctrl Pts',(21.4073533630364,-7.56186435703622,
12.));
#218310=CARTESIAN_POINT('Ctrl Pts',(21.4165463106252,-7.56394299313683,
12.));
#218311=CARTESIAN_POINT('Ctrl Pts',(21.4259653015732,-7.56603771218706,
12.));
#218312=CARTESIAN_POINT('Ctrl Pts',(21.435606926151,-7.56814636360842,12.));
#218313=CARTESIAN_POINT('Ctrl Pts',(21.445467890751,-7.5702668726117,12.));
#218314=CARTESIAN_POINT('Ctrl Pts',(21.4555450053147,-7.57239723223521,
12.));
#218315=CARTESIAN_POINT('Ctrl Pts',(21.4658351740135,-7.57453549743435,
12.));
#218316=CARTESIAN_POINT('Ctrl Pts',(21.4763353936766,-7.57667978403003,
12.));
#218317=CARTESIAN_POINT('Ctrl Pts',(21.4870427508193,-7.57882826679131,
12.));
#218318=CARTESIAN_POINT('Ctrl Pts',(21.4979544192739,-7.5809791779073,12.));
#218319=CARTESIAN_POINT('Ctrl Pts',(21.5090676573866,-7.58313080519159,
12.));
#218320=CARTESIAN_POINT('Ctrl Pts',(21.5203798035294,-7.58528148919114,
12.));
#218321=CARTESIAN_POINT('Ctrl Pts',(21.5318882716735,-7.58742962034834,
12.));
#218322=CARTESIAN_POINT('Ctrl Pts',(21.5435905470113,-7.58957363620026,
12.));
#218323=CARTESIAN_POINT('Ctrl Pts',(21.5554841813465,-7.59171201844793,
12.));
#218324=CARTESIAN_POINT('Ctrl Pts',(21.5675667904728,-7.5938432912493,12.));
#218325=CARTESIAN_POINT('Ctrl Pts',(21.5798360518978,-7.59596601973589,
12.));
#218326=CARTESIAN_POINT('Ctrl Pts',(21.5922897024466,-7.59807880846193,
12.));
#218327=CARTESIAN_POINT('Ctrl Pts',(21.6049255358842,-7.60018029988238,
12.));
#218328=CARTESIAN_POINT('Ctrl Pts',(21.6177414005991,-7.60226917285432,
12.));
#218329=CARTESIAN_POINT('Ctrl Pts',(21.6307351973823,-7.604344141183,12.));
#218330=CARTESIAN_POINT('Ctrl Pts',(21.6439048771743,-7.60640395216359,
12.));
#218331=CARTESIAN_POINT('Ctrl Pts',(21.6572484388079,-7.60844738512872,
12.));
#218332=CARTESIAN_POINT('Ctrl Pts',(21.6707639267573,-7.6104732500095,12.));
#218333=CARTESIAN_POINT('Ctrl Pts',(21.6844494295813,-7.61248038630265,
12.));
#218334=CARTESIAN_POINT('Ctrl Pts',(21.6983030783321,-7.61446766202787,
12.));
#218335=CARTESIAN_POINT('Ctrl Pts',(21.7123230449835,-7.61643397270425,
12.));
#218336=CARTESIAN_POINT('Ctrl Pts',(21.7265075407977,-7.61837824030542,
12.));
#218337=CARTESIAN_POINT('Ctrl Pts',(21.7408548148657,-7.62029941230855,
12.));
#218338=CARTESIAN_POINT('Ctrl Pts',(21.7553631528329,-7.62219646084226,
12.));
#218339=CARTESIAN_POINT('Ctrl Pts',(21.7700308755583,-7.62406838181164,
12.));
#218340=CARTESIAN_POINT('Ctrl Pts',(21.7848563378022,-7.62591419404521,
12.));
#218341=CARTESIAN_POINT('Ctrl Pts',(21.7998379268583,-7.62773293842409,
12.));
#218342=CARTESIAN_POINT('Ctrl Pts',(21.8149740615093,-7.62952367718151,
12.));
#218343=CARTESIAN_POINT('Ctrl Pts',(21.8302631910197,-7.6312854932304,12.));
#218344=CARTESIAN_POINT('Ctrl Pts',(21.8457037941084,-7.63301748948936,
12.));
#218345=CARTESIAN_POINT('Ctrl Pts',(21.8612943779086,-7.63471878821204,
12.));
#218346=CARTESIAN_POINT('Ctrl Pts',(21.8770334769492,-7.63638853033368,
12.));
#218347=CARTESIAN_POINT('Ctrl Pts',(21.8929196523511,-7.63802587492008,
12.));
#218348=CARTESIAN_POINT('Ctrl Pts',(21.9089514909873,-7.63962999860917,
12.));
#218349=CARTESIAN_POINT('Ctrl Pts',(21.9251276046546,-7.6412000950654,12.));
#218350=CARTESIAN_POINT('Ctrl Pts',(21.9414466292074,-7.64273537442707,
12.));
#218351=CARTESIAN_POINT('Ctrl Pts',(21.9579072237653,-7.64423506279154,
12.));
#218352=CARTESIAN_POINT('Ctrl Pts',(21.97450807008,-7.64569840177359,12.));
#218353=CARTESIAN_POINT('Ctrl Pts',(21.9912478718542,-7.64712464805258,
12.));
#218354=CARTESIAN_POINT('Ctrl Pts',(22.0081253540773,-7.64851307293346,
12.));
#218355=CARTESIAN_POINT('Ctrl Pts',(22.0251392623209,-7.64986296190157,
12.));
#218356=CARTESIAN_POINT('Ctrl Pts',(22.0422883621176,-7.65117361421347,
12.));
#218357=CARTESIAN_POINT('Ctrl Pts',(22.0595714384432,-7.65244434253104,
12.));
#218358=CARTESIAN_POINT('Ctrl Pts',(22.0769872951596,-7.65367447254945,
12.));
#218359=CARTESIAN_POINT('Ctrl Pts',(22.094534754469,-7.65486334263651,12.));
#218360=CARTESIAN_POINT('Ctrl Pts',(22.1122126563327,-7.65601030346819,
12.));
#218361=CARTESIAN_POINT('Ctrl Pts',(22.1300198579671,-7.65711471769407,
12.));
#218362=CARTESIAN_POINT('Ctrl Pts',(22.1479552334206,-7.65817595963351,
12.));
#218363=CARTESIAN_POINT('Ctrl Pts',(22.1660176731174,-7.65919341496926,
12.));
#218364=CARTESIAN_POINT('Ctrl Pts',(22.1842060834092,-7.66016648045008,
12.));
#218365=CARTESIAN_POINT('Ctrl Pts',(22.2025193860972,-7.66109456359292,
12.));
#218366=CARTESIAN_POINT('Ctrl Pts',(22.2209565180098,-7.66197708240436,
12.));
#218367=CARTESIAN_POINT('Ctrl Pts',(22.239516430656,-7.66281346512546,12.));
#218368=CARTESIAN_POINT('Ctrl Pts',(22.2581980898487,-7.66360314997662,
12.));
#218369=CARTESIAN_POINT('Ctrl Pts',(22.2770004753332,-7.66434558490973,
12.));
#218370=CARTESIAN_POINT('Ctrl Pts',(22.2959225803925,-7.66504022736263,
12.));
#218371=CARTESIAN_POINT('Ctrl Pts',(22.3149634114823,-7.66568654402442,
12.));
#218372=CARTESIAN_POINT('Ctrl Pts',(22.3341219879454,-7.66628401061906,
12.));
#218373=CARTESIAN_POINT('Ctrl Pts',(22.3533973417013,-7.66683211169134,
12.));
#218374=CARTESIAN_POINT('Ctrl Pts',(22.3727885169361,-7.66733034039887,
12.));
#218375=CARTESIAN_POINT('Ctrl Pts',(22.3922945697782,-7.6677781983082,12.));
#218376=CARTESIAN_POINT('Ctrl Pts',(22.411914567977,-7.66817519519682,12.));
#218377=CARTESIAN_POINT('Ctrl Pts',(22.4316475906616,-7.66852084886746,
12.));
#218378=CARTESIAN_POINT('Ctrl Pts',(22.4514927280862,-7.6688146849666,12.));
#218379=CARTESIAN_POINT('Ctrl Pts',(22.47144908137,-7.66905623680836,12.));
#218380=CARTESIAN_POINT('Ctrl Pts',(22.4915157622308,-7.66924504520302,
12.));
#218381=CARTESIAN_POINT('Ctrl Pts',(22.5116918927023,-7.66938065829083,
12.));
#218382=CARTESIAN_POINT('Ctrl Pts',(22.5319766049191,-7.66946263138116,
12.));
#218383=CARTESIAN_POINT('Ctrl Pts',(22.5523690409109,-7.66949052679672,
12.));
#218384=CARTESIAN_POINT('Ctrl Pts',(22.5728683523828,-7.66946391372299,
12.));
#218385=CARTESIAN_POINT('Ctrl Pts',(22.5934737004955,-7.66938236806241,
12.));
#218386=CARTESIAN_POINT('Ctrl Pts',(22.6141842556248,-7.66924547229435,
12.));
#218387=CARTESIAN_POINT('Ctrl Pts',(22.6349991971547,-7.66905281533745,
12.));
#218388=CARTESIAN_POINT('Ctrl Pts',(22.6559177133133,-7.66880399241354,
12.));
#218389=CARTESIAN_POINT('Ctrl Pts',(22.6769390009889,-7.66849860491763,
12.));
#218390=CARTESIAN_POINT('Ctrl Pts',(22.6980622655446,-7.66813626029277,
12.));
#218391=CARTESIAN_POINT('Ctrl Pts',(22.7192867206242,-7.6677165719101,12.));
#218392=CARTESIAN_POINT('Ctrl Pts',(22.7406115879508,-7.66723915895413,
12.));
#218393=CARTESIAN_POINT('Ctrl Pts',(22.7620360971839,-7.66670364630273,
12.));
#218394=CARTESIAN_POINT('Ctrl Pts',(22.7835594857697,-7.66610966441259,
12.));
#218395=CARTESIAN_POINT('Ctrl Pts',(22.8051809987833,-7.66545684920988,
12.));
#218396=CARTESIAN_POINT('Ctrl Pts',(22.8268998887678,-7.66474484198553,
12.));
#218397=CARTESIAN_POINT('Ctrl Pts',(22.8487154155569,-7.66397328929805,
12.));
#218398=CARTESIAN_POINT('Ctrl Pts',(22.870626846128,-7.66314184287334,12.));
#218399=CARTESIAN_POINT('Ctrl Pts',(22.8926334544879,-7.66225015950148,
12.));
#218400=CARTESIAN_POINT('Ctrl Pts',(22.9147345215418,-7.661297900941,12.));
#218401=CARTESIAN_POINT('Ctrl Pts',(22.9369293349592,-7.66028473382777,
12.));
#218402=CARTESIAN_POINT('Ctrl Pts',(22.9592171890332,-7.65921032958912,
12.));
#218403=CARTESIAN_POINT('Ctrl Pts',(22.9815973845301,-7.65807436436453,
12.));
#218404=CARTESIAN_POINT('Ctrl Pts',(23.004069228582,-7.6568765189133,12.));
#218405=CARTESIAN_POINT('Ctrl Pts',(23.0266320345792,-7.65561647852555,
12.));
#218406=CARTESIAN_POINT('Ctrl Pts',(23.049285122053,-7.65429393293955,12.));
#218407=CARTESIAN_POINT('Ctrl Pts',(23.072027816555,-7.65290857626357,12.));
#218408=CARTESIAN_POINT('Ctrl Pts',(23.0948594495246,-7.65146010690465,
12.));
#218409=CARTESIAN_POINT('Ctrl Pts',(23.1177793581674,-7.64994822749845,
12.));
#218410=CARTESIAN_POINT('Ctrl Pts',(23.1407868853815,-7.64837264482929,
12.));
#218411=CARTESIAN_POINT('Ctrl Pts',(23.1638813796691,-7.64673306975797,
12.));
#218412=CARTESIAN_POINT('Ctrl Pts',(23.1870621950452,-7.64502921715483,
12.));
#218413=CARTESIAN_POINT('Ctrl Pts',(23.2103286909399,-7.64326080583684,
12.));
#218414=CARTESIAN_POINT('Ctrl Pts',(23.2336802320912,-7.64142755851508,
12.));
#218415=CARTESIAN_POINT('Ctrl Pts',(23.2571161884487,-7.63952920172837,
12.));
#218416=CARTESIAN_POINT('Ctrl Pts',(23.2806359350853,-7.63756546576375,
12.));
#218417=CARTESIAN_POINT('Ctrl Pts',(23.3042388521021,-7.63553608458784,
12.));
#218418=CARTESIAN_POINT('Ctrl Pts',(23.3279243245241,-7.63344079578163,
12.));
#218419=CARTESIAN_POINT('Ctrl Pts',(23.3516917421973,-7.63127934048139,
12.));
#218420=CARTESIAN_POINT('Ctrl Pts',(23.3755404996638,-7.62905146332598,
12.));
#218421=CARTESIAN_POINT('Ctrl Pts',(23.3994699961122,-7.62675691240335,
12.));
#218422=CARTESIAN_POINT('Ctrl Pts',(23.4234796353544,-7.62439543920055,
12.));
#218423=CARTESIAN_POINT('Ctrl Pts',(23.4475688257854,-7.62196679855957,
12.));
#218424=CARTESIAN_POINT('Ctrl Pts',(23.4717369803438,-7.61947074863978,
12.));
#218425=CARTESIAN_POINT('Ctrl Pts',(23.4959835164608,-7.61690705088319,
12.));
#218426=CARTESIAN_POINT('Ctrl Pts',(23.5203078560128,-7.61427546999299,
12.));
#218427=CARTESIAN_POINT('Ctrl Pts',(23.5447094252028,-7.61157577385372,
12.));
#218428=CARTESIAN_POINT('Ctrl Pts',(23.5691876544243,-7.608807733446,12.));
#218429=CARTESIAN_POINT('Ctrl Pts',(23.5937419781244,-7.60597112277094,
12.));
#218430=CARTESIAN_POINT('Ctrl Pts',(23.6183718346576,-7.60306571877806,
12.));
#218431=CARTESIAN_POINT('Ctrl Pts',(23.6430766661419,-7.6000913013013,12.));
#218432=CARTESIAN_POINT('Ctrl Pts',(23.6678559182876,-7.59704765299572,
12.));
#218433=CARTESIAN_POINT('Ctrl Pts',(23.6927090405067,-7.59393455934042,
12.));
#218434=CARTESIAN_POINT('Ctrl Pts',(23.7176354860457,-7.59075180865327,
12.));
#218435=CARTESIAN_POINT('Ctrl Pts',(23.7426347121006,-7.58749919210832,
12.));
#218436=CARTESIAN_POINT('Ctrl Pts',(23.7677061799376,-7.58417650376272,
12.));
#218437=CARTESIAN_POINT('Ctrl Pts',(23.7928493549908,-7.58078354058212,
12.));
#218438=CARTESIAN_POINT('Ctrl Pts',(23.8180637069977,-7.57732010249066,
12.));
#218439=CARTESIAN_POINT('Ctrl Pts',(23.8433487096134,-7.57378599219817,
12.));
#218440=CARTESIAN_POINT('Ctrl Pts',(23.8687038399597,-7.57018101500711,
12.));
#218441=CARTESIAN_POINT('Ctrl Pts',(23.8941285782003,-7.56650497863792,
12.));
#218442=CARTESIAN_POINT('Ctrl Pts',(23.9196224070759,-7.56275769304773,
12.));
#218443=CARTESIAN_POINT('Ctrl Pts',(23.9451848115,-7.55893897027683,12.));
#218444=CARTESIAN_POINT('Ctrl Pts',(23.9708152779884,-7.55504862424812,
12.));
#218445=CARTESIAN_POINT('Ctrl Pts',(23.9965132953185,-7.55108647097441,
12.));
#218446=CARTESIAN_POINT('Ctrl Pts',(24.022278355453,-7.5470523288591,12.));
#218447=CARTESIAN_POINT('Ctrl Pts',(24.0481099543353,-7.54294601896145,
12.));
#218448=CARTESIAN_POINT('Ctrl Pts',(24.0740075927985,-7.53876736531014,
12.));
#218449=CARTESIAN_POINT('Ctrl Pts',(24.0999707772642,-7.53451619514649,
12.));
#218450=CARTESIAN_POINT('Ctrl Pts',(24.1259990209207,-7.53019233935502,
12.));
#218451=CARTESIAN_POINT('Ctrl Pts',(24.1520918425364,-7.52579563201424,
12.));
#218452=CARTESIAN_POINT('Ctrl Pts',(24.1782487641594,-7.52132590953802,
12.));
#218453=CARTESIAN_POINT('Ctrl Pts',(24.2044693092349,-7.51678300997949,
12.));
#218454=CARTESIAN_POINT('Ctrl Pts',(24.2307530003887,-7.51216677222181,
12.));
#218455=CARTESIAN_POINT('Ctrl Pts',(24.2570993577034,-7.50747703535134,
12.));
#218456=CARTESIAN_POINT('Ctrl Pts',(24.2835078958973,-7.50271363765152,
12.));
#218457=CARTESIAN_POINT('Ctrl Pts',(24.3099781253355,-7.49787641695439,
12.));
#218458=CARTESIAN_POINT('Ctrl Pts',(24.3365095573685,-7.49296521252421,
12.));
#218459=CARTESIAN_POINT('Ctrl Pts',(24.3631017084524,-7.48797986651909,
12.));
#218460=CARTESIAN_POINT('Ctrl Pts',(24.3897541049254,-7.48292022569301,
12.));
#218461=CARTESIAN_POINT('Ctrl Pts',(24.4164662871163,-7.47778614286565,
12.));
#218462=CARTESIAN_POINT('Ctrl Pts',(24.443237814649,-7.47257747883246,12.));
#218463=CARTESIAN_POINT('Ctrl Pts',(24.4700682684524,-7.46729410308787,
12.));
#218464=CARTESIAN_POINT('Ctrl Pts',(24.4969572391483,-7.46193588961464,
12.));
#218465=CARTESIAN_POINT('Ctrl Pts',(24.5239043173072,-7.45650271335862,
12.));
#218466=CARTESIAN_POINT('Ctrl Pts',(24.5509090831559,-7.4509944465116,12.));
#218467=CARTESIAN_POINT('Ctrl Pts',(24.577971096086,-7.44541095473135,12.));
#218468=CARTESIAN_POINT('Ctrl Pts',(24.6050898852368,-7.43975209375504,
12.));
#218469=CARTESIAN_POINT('Ctrl Pts',(24.6322649369517,-7.43401770489524,
12.));
#218470=CARTESIAN_POINT('Ctrl Pts',(24.6594957128756,-7.42820762159126,
12.));
#218471=CARTESIAN_POINT('Ctrl Pts',(24.6867816727192,-7.42232167766266,
12.));
#218472=CARTESIAN_POINT('Ctrl Pts',(24.7141222950051,-7.41635971481674,
12.));
#218473=CARTESIAN_POINT('Ctrl Pts',(24.7415170994784,-7.41032159082382,
12.));
#218474=CARTESIAN_POINT('Ctrl Pts',(24.7689656668983,-7.40420718661603,
12.));
#218475=CARTESIAN_POINT('Ctrl Pts',(24.7964676646431,-7.39801641583013,
12.));
#218476=CARTESIAN_POINT('Ctrl Pts',(24.8240228520893,-7.39174922585809,
12.));
#218477=CARTESIAN_POINT('Ctrl Pts',(24.8516310625176,-7.38540558903621,
12.));
#218478=CARTESIAN_POINT('Ctrl Pts',(24.8792921911115,-7.3789854964027,12.));
#218479=CARTESIAN_POINT('Ctrl Pts',(24.901463382605,-7.37378825961676,12.));
#218480=CARTESIAN_POINT('Ctrl Pts',(24.9181155530543,-7.36985593120091,
12.));
#218481=CARTESIAN_POINT('Ctrl Pts',(24.9292275670674,-7.36721909028843,
12.));
#218482=CARTESIAN_POINT('Ctrl Pts',(24.9347862158358,-7.36589684767345,
12.));
#218483=CARTESIAN_POINT('Ctrl Pts',(20.353053841303,-9.71462809124917,0.));
#218484=CARTESIAN_POINT('Ctrl Pts',(20.353053841303,-9.71462809124917,12.));
#218485=CARTESIAN_POINT('Ctrl Pts',(20.353060251684,-9.71462954053074,0.));
#218486=CARTESIAN_POINT('Ctrl Pts',(20.353060251684,-9.71462954053074,12.));
#218487=CARTESIAN_POINT('Ctrl Pts',(20.3531126095522,-9.71465227853122,
0.));
#218488=CARTESIAN_POINT('Ctrl Pts',(20.3531126095522,-9.71465227853122,
12.));
#218489=CARTESIAN_POINT('Ctrl Pts',(20.3533097561886,-9.71474590350792,
0.));
#218490=CARTESIAN_POINT('Ctrl Pts',(20.3533097561886,-9.71474590350792,
12.));
#218491=CARTESIAN_POINT('Ctrl Pts',(20.3538098605706,-9.71498978052101,
0.));
#218492=CARTESIAN_POINT('Ctrl Pts',(20.3538098605706,-9.71498978052101,
12.));
#218493=CARTESIAN_POINT('Ctrl Pts',(20.3548282742361,-9.71549257088175,
0.));
#218494=CARTESIAN_POINT('Ctrl Pts',(20.3548282742361,-9.71549257088175,
12.));
#218495=CARTESIAN_POINT('Ctrl Pts',(20.3562337557875,-9.71619192554147,
0.));
#218496=CARTESIAN_POINT('Ctrl Pts',(20.3562337557875,-9.71619192554147,
12.));
#218497=CARTESIAN_POINT('Ctrl Pts',(20.3580133103357,-9.71708493723062,
0.));
#218498=CARTESIAN_POINT('Ctrl Pts',(20.3580133103357,-9.71708493723062,
12.));
#218499=CARTESIAN_POINT('Ctrl Pts',(20.3601498764344,-9.71816778327999,
0.));
#218500=CARTESIAN_POINT('Ctrl Pts',(20.3601498764344,-9.71816778327999,
12.));
#218501=CARTESIAN_POINT('Ctrl Pts',(20.362625691398,-9.71943648548115,0.));
#218502=CARTESIAN_POINT('Ctrl Pts',(20.362625691398,-9.71943648548115,12.));
#218503=CARTESIAN_POINT('Ctrl Pts',(20.3654261611055,-9.72088778381102,
0.));
#218504=CARTESIAN_POINT('Ctrl Pts',(20.3654261611055,-9.72088778381102,
12.));
#218505=CARTESIAN_POINT('Ctrl Pts',(20.3685406190576,-9.72251930722504,
0.));
#218506=CARTESIAN_POINT('Ctrl Pts',(20.3685406190576,-9.72251930722504,
12.));
#218507=CARTESIAN_POINT('Ctrl Pts',(20.371960235676,-9.72432910043193,0.));
#218508=CARTESIAN_POINT('Ctrl Pts',(20.371960235676,-9.72432910043193,12.));
#218509=CARTESIAN_POINT('Ctrl Pts',(20.3756766651952,-9.72631531732871,
0.));
#218510=CARTESIAN_POINT('Ctrl Pts',(20.3756766651952,-9.72631531732871,
12.));
#218511=CARTESIAN_POINT('Ctrl Pts',(20.3796805893304,-9.72847589116533,
0.));
#218512=CARTESIAN_POINT('Ctrl Pts',(20.3796805893304,-9.72847589116533,
12.));
#218513=CARTESIAN_POINT('Ctrl Pts',(20.3839624556742,-9.73080870123726,
0.));
#218514=CARTESIAN_POINT('Ctrl Pts',(20.3839624556742,-9.73080870123726,
12.));
#218515=CARTESIAN_POINT('Ctrl Pts',(20.3885129129912,-9.73331167102812,
0.));
#218516=CARTESIAN_POINT('Ctrl Pts',(20.3885129129912,-9.73331167102812,
12.));
#218517=CARTESIAN_POINT('Ctrl Pts',(20.3933234845646,-9.7359829201425,0.));
#218518=CARTESIAN_POINT('Ctrl Pts',(20.3933234845646,-9.7359829201425,12.));
#218519=CARTESIAN_POINT('Ctrl Pts',(20.3983866213331,-9.73882077613206,
0.));
#218520=CARTESIAN_POINT('Ctrl Pts',(20.3983866213331,-9.73882077613206,
12.));
#218521=CARTESIAN_POINT('Ctrl Pts',(20.4036953576549,-9.74182369656273,
0.));
#218522=CARTESIAN_POINT('Ctrl Pts',(20.4036953576549,-9.74182369656273,
12.));
#218523=CARTESIAN_POINT('Ctrl Pts',(20.4092430879861,-9.74499021838537,
0.));
#218524=CARTESIAN_POINT('Ctrl Pts',(20.4092430879861,-9.74499021838537,
12.));
#218525=CARTESIAN_POINT('Ctrl Pts',(20.4150232777393,-9.74831889242175,
0.));
#218526=CARTESIAN_POINT('Ctrl Pts',(20.4150232777393,-9.74831889242175,
12.));
#218527=CARTESIAN_POINT('Ctrl Pts',(20.4210295275818,-9.75180829786433,
0.));
#218528=CARTESIAN_POINT('Ctrl Pts',(20.4210295275818,-9.75180829786433,
12.));
#218529=CARTESIAN_POINT('Ctrl Pts',(20.4272556476629,-9.75545705902416,
0.));
#218530=CARTESIAN_POINT('Ctrl Pts',(20.4272556476629,-9.75545705902416,
12.));
#218531=CARTESIAN_POINT('Ctrl Pts',(20.4336957355474,-9.7592638628993,0.));
#218532=CARTESIAN_POINT('Ctrl Pts',(20.4336957355474,-9.7592638628993,12.));
#218533=CARTESIAN_POINT('Ctrl Pts',(20.4403442329401,-9.76322747195502,
0.));
#218534=CARTESIAN_POINT('Ctrl Pts',(20.4403442329401,-9.76322747195502,
12.));
#218535=CARTESIAN_POINT('Ctrl Pts',(20.447195862298,-9.76734670980897,0.));
#218536=CARTESIAN_POINT('Ctrl Pts',(20.447195862298,-9.76734670980897,12.));
#218537=CARTESIAN_POINT('Ctrl Pts',(20.4542455817527,-9.7716204510407,0.));
#218538=CARTESIAN_POINT('Ctrl Pts',(20.4542455817527,-9.7716204510407,12.));
#218539=CARTESIAN_POINT('Ctrl Pts',(20.4614885274973,-9.77604760815523,
0.));
#218540=CARTESIAN_POINT('Ctrl Pts',(20.4614885274973,-9.77604760815523,
12.));
#218541=CARTESIAN_POINT('Ctrl Pts',(20.4689199790668,-9.78062712373313,
0.));
#218542=CARTESIAN_POINT('Ctrl Pts',(20.4689199790668,-9.78062712373313,
12.));
#218543=CARTESIAN_POINT('Ctrl Pts',(20.4765353711585,-9.78535797314162,
0.));
#218544=CARTESIAN_POINT('Ctrl Pts',(20.4765353711585,-9.78535797314162,
12.));
#218545=CARTESIAN_POINT('Ctrl Pts',(20.4843302955329,-9.7902391649866,0.));
#218546=CARTESIAN_POINT('Ctrl Pts',(20.4843302955329,-9.7902391649866,12.));
#218547=CARTESIAN_POINT('Ctrl Pts',(20.4923005087945,-9.79526974288344,
0.));
#218548=CARTESIAN_POINT('Ctrl Pts',(20.4923005087945,-9.79526974288344,
12.));
#218549=CARTESIAN_POINT('Ctrl Pts',(20.500441931211,-9.80044878520968,0.));
#218550=CARTESIAN_POINT('Ctrl Pts',(20.500441931211,-9.80044878520968,12.));
#218551=CARTESIAN_POINT('Ctrl Pts',(20.5087506310507,-9.80577540161103,
0.));
#218552=CARTESIAN_POINT('Ctrl Pts',(20.5087506310507,-9.80577540161103,
12.));
#218553=CARTESIAN_POINT('Ctrl Pts',(20.5172228122839,-9.81124873025278,
0.));
#218554=CARTESIAN_POINT('Ctrl Pts',(20.5172228122839,-9.81124873025278,
12.));
#218555=CARTESIAN_POINT('Ctrl Pts',(20.5258548000625,-9.81686793455918,
0.));
#218556=CARTESIAN_POINT('Ctrl Pts',(20.5258548000625,-9.81686793455918,
12.));
#218557=CARTESIAN_POINT('Ctrl Pts',(20.534643029951,-9.82263220080328,0.));
#218558=CARTESIAN_POINT('Ctrl Pts',(20.534643029951,-9.82263220080328,12.));
#218559=CARTESIAN_POINT('Ctrl Pts',(20.5435840460717,-9.82854073773858,
0.));
#218560=CARTESIAN_POINT('Ctrl Pts',(20.5435840460717,-9.82854073773858,
12.));
#218561=CARTESIAN_POINT('Ctrl Pts',(20.5526744976461,-9.83459277585321,
0.));
#218562=CARTESIAN_POINT('Ctrl Pts',(20.5526744976461,-9.83459277585321,
12.));
#218563=CARTESIAN_POINT('Ctrl Pts',(20.5619111362406,-9.84078756677589,
0.));
#218564=CARTESIAN_POINT('Ctrl Pts',(20.5619111362406,-9.84078756677589,
12.));
#218565=CARTESIAN_POINT('Ctrl Pts',(20.5712908125145,-9.84712438256308,
0.));
#218566=CARTESIAN_POINT('Ctrl Pts',(20.5712908125145,-9.84712438256308,
12.));
#218567=CARTESIAN_POINT('Ctrl Pts',(20.580810471002,-9.85360251457004,0.));
#218568=CARTESIAN_POINT('Ctrl Pts',(20.580810471002,-9.85360251457004,12.));
#218569=CARTESIAN_POINT('Ctrl Pts',(20.5904671449754,-9.8602212723275,0.));
#218570=CARTESIAN_POINT('Ctrl Pts',(20.5904671449754,-9.8602212723275,12.));
#218571=CARTESIAN_POINT('Ctrl Pts',(20.6002579513696,-9.86697998242612,
0.));
#218572=CARTESIAN_POINT('Ctrl Pts',(20.6002579513696,-9.86697998242612,
12.));
#218573=CARTESIAN_POINT('Ctrl Pts',(20.6101800854491,-9.87387798732944,
0.));
#218574=CARTESIAN_POINT('Ctrl Pts',(20.6101800854491,-9.87387798732944,
12.));
#218575=CARTESIAN_POINT('Ctrl Pts',(20.6202308177472,-9.88091464472669,
0.));
#218576=CARTESIAN_POINT('Ctrl Pts',(20.6202308177472,-9.88091464472669,
12.));
#218577=CARTESIAN_POINT('Ctrl Pts',(20.6304074914086,-9.88808932697305,
0.));
#218578=CARTESIAN_POINT('Ctrl Pts',(20.6304074914086,-9.88808932697305,
12.));
#218579=CARTESIAN_POINT('Ctrl Pts',(20.6407075193977,-9.89540142049124,
0.));
#218580=CARTESIAN_POINT('Ctrl Pts',(20.6407075193977,-9.89540142049124,
12.));
#218581=CARTESIAN_POINT('Ctrl Pts',(20.6511283817415,-9.90285032516696,
0.));
#218582=CARTESIAN_POINT('Ctrl Pts',(20.6511283817415,-9.90285032516696,
12.));
#218583=CARTESIAN_POINT('Ctrl Pts',(20.6616676228315,-9.91043545377005,
0.));
#218584=CARTESIAN_POINT('Ctrl Pts',(20.6616676228315,-9.91043545377005,
12.));
#218585=CARTESIAN_POINT('Ctrl Pts',(20.6723228488261,-9.91815623141285,
0.));
#218586=CARTESIAN_POINT('Ctrl Pts',(20.6723228488261,-9.91815623141285,
12.));
#218587=CARTESIAN_POINT('Ctrl Pts',(20.6830917250255,-9.92601209498751,
0.));
#218588=CARTESIAN_POINT('Ctrl Pts',(20.6830917250255,-9.92601209498751,
12.));
#218589=CARTESIAN_POINT('Ctrl Pts',(20.6939719732485,-9.93400249259737,
0.));
#218590=CARTESIAN_POINT('Ctrl Pts',(20.6939719732485,-9.93400249259737,
12.));
#218591=CARTESIAN_POINT('Ctrl Pts',(20.7049613692237,-9.94212688298251,
0.));
#218592=CARTESIAN_POINT('Ctrl Pts',(20.7049613692237,-9.94212688298251,
12.));
#218593=CARTESIAN_POINT('Ctrl Pts',(20.716057740758,-9.95038473514962,0.));
#218594=CARTESIAN_POINT('Ctrl Pts',(20.716057740758,-9.95038473514962,12.));
#218595=CARTESIAN_POINT('Ctrl Pts',(20.7272589658752,-9.95877552798403,
0.));
#218596=CARTESIAN_POINT('Ctrl Pts',(20.7272589658752,-9.95877552798403,
12.));
#218597=CARTESIAN_POINT('Ctrl Pts',(20.7385629709795,-9.96729874986199,
0.));
#218598=CARTESIAN_POINT('Ctrl Pts',(20.7385629709795,-9.96729874986199,
12.));
#218599=CARTESIAN_POINT('Ctrl Pts',(20.7499677289625,-9.97595389823461,
0.));
#218600=CARTESIAN_POINT('Ctrl Pts',(20.7499677289625,-9.97595389823461,
12.));
#218601=CARTESIAN_POINT('Ctrl Pts',(20.7614712574989,-9.98474047926846,
0.));
#218602=CARTESIAN_POINT('Ctrl Pts',(20.7614712574989,-9.98474047926846,
12.));
#218603=CARTESIAN_POINT('Ctrl Pts',(20.7730716175417,-9.99365800754638,
0.));
#218604=CARTESIAN_POINT('Ctrl Pts',(20.7730716175417,-9.99365800754638,
12.));
#218605=CARTESIAN_POINT('Ctrl Pts',(20.7847669117568,-10.0027060057389,
0.));
#218606=CARTESIAN_POINT('Ctrl Pts',(20.7847669117568,-10.0027060057389,
12.));
#218607=CARTESIAN_POINT('Ctrl Pts',(20.7965552829907,-10.0118840042786,
0.));
#218608=CARTESIAN_POINT('Ctrl Pts',(20.7965552829907,-10.0118840042786,
12.));
#218609=CARTESIAN_POINT('Ctrl Pts',(20.8084349126885,-10.0211915410095,
0.));
#218610=CARTESIAN_POINT('Ctrl Pts',(20.8084349126885,-10.0211915410095,
12.));
#218611=CARTESIAN_POINT('Ctrl Pts',(20.8204040196599,-10.0306281609435,
0.));
#218612=CARTESIAN_POINT('Ctrl Pts',(20.8204040196599,-10.0306281609435,
12.));
#218613=CARTESIAN_POINT('Ctrl Pts',(20.8324608588906,-10.0401934160234,
0.));
#218614=CARTESIAN_POINT('Ctrl Pts',(20.8324608588906,-10.0401934160234,
12.));
#218615=CARTESIAN_POINT('Ctrl Pts',(20.8446037203402,-10.0498868648733,
0.));
#218616=CARTESIAN_POINT('Ctrl Pts',(20.8446037203402,-10.0498868648733,
12.));
#218617=CARTESIAN_POINT('Ctrl Pts',(20.856830927732,-10.0597080725375,0.));
#218618=CARTESIAN_POINT('Ctrl Pts',(20.856830927732,-10.0597080725375,12.));
#218619=CARTESIAN_POINT('Ctrl Pts',(20.8691408373705,-10.0696566102219,
0.));
#218620=CARTESIAN_POINT('Ctrl Pts',(20.8691408373705,-10.0696566102219,
12.));
#218621=CARTESIAN_POINT('Ctrl Pts',(20.8815318371844,-10.0797320551154,
0.));
#218622=CARTESIAN_POINT('Ctrl Pts',(20.8815318371844,-10.0797320551154,
12.));
#218623=CARTESIAN_POINT('Ctrl Pts',(20.8940023457371,-10.0899339901916,
0.));
#218624=CARTESIAN_POINT('Ctrl Pts',(20.8940023457371,-10.0899339901916,
12.));
#218625=CARTESIAN_POINT('Ctrl Pts',(20.9065508112556,-10.1002620040076,
0.));
#218626=CARTESIAN_POINT('Ctrl Pts',(20.9065508112556,-10.1002620040076,
12.));
#218627=CARTESIAN_POINT('Ctrl Pts',(20.9191757106266,-10.1107156904836,
0.));
#218628=CARTESIAN_POINT('Ctrl Pts',(20.9191757106266,-10.1107156904836,
12.));
#218629=CARTESIAN_POINT('Ctrl Pts',(20.931875548473,-10.1212946487057,0.));
#218630=CARTESIAN_POINT('Ctrl Pts',(20.931875548473,-10.1212946487057,12.));
#218631=CARTESIAN_POINT('Ctrl Pts',(20.944648856393,-10.1319984827909,0.));
#218632=CARTESIAN_POINT('Ctrl Pts',(20.944648856393,-10.1319984827909,12.));
#218633=CARTESIAN_POINT('Ctrl Pts',(20.9574941921591,-10.1428268017257,
0.));
#218634=CARTESIAN_POINT('Ctrl Pts',(20.9574941921591,-10.1428268017257,
12.));
#218635=CARTESIAN_POINT('Ctrl Pts',(20.970410138937,-10.1537792192065,0.));
#218636=CARTESIAN_POINT('Ctrl Pts',(20.970410138937,-10.1537792192065,12.));
#218637=CARTESIAN_POINT('Ctrl Pts',(20.9833953044736,-10.1648553534567,
0.));
#218638=CARTESIAN_POINT('Ctrl Pts',(20.9833953044736,-10.1648553534567,
12.));
#218639=CARTESIAN_POINT('Ctrl Pts',(20.9964483203685,-10.1760548270765,
0.));
#218640=CARTESIAN_POINT('Ctrl Pts',(20.9964483203685,-10.1760548270765,
12.));
#218641=CARTESIAN_POINT('Ctrl Pts',(21.0095678414486,-10.1873772669358,
0.));
#218642=CARTESIAN_POINT('Ctrl Pts',(21.0095678414486,-10.1873772669358,
12.));
#218643=CARTESIAN_POINT('Ctrl Pts',(21.0227525451107,-10.1988223040425,
0.));
#218644=CARTESIAN_POINT('Ctrl Pts',(21.0227525451107,-10.1988223040425,
12.));
#218645=CARTESIAN_POINT('Ctrl Pts',(21.0360011306814,-10.2103895734124,
0.));
#218646=CARTESIAN_POINT('Ctrl Pts',(21.0360011306814,-10.2103895734124,
12.));
#218647=CARTESIAN_POINT('Ctrl Pts',(21.0493123187483,-10.2220787139157,
0.));
#218648=CARTESIAN_POINT('Ctrl Pts',(21.0493123187483,-10.2220787139157,
12.));
#218649=CARTESIAN_POINT('Ctrl Pts',(21.0626848505665,-10.233889368157,0.));
#218650=CARTESIAN_POINT('Ctrl Pts',(21.0626848505665,-10.233889368157,12.));
#218651=CARTESIAN_POINT('Ctrl Pts',(21.0761174875448,-10.2458211823915,
0.));
#218652=CARTESIAN_POINT('Ctrl Pts',(21.0761174875448,-10.2458211823915,
12.));
#218653=CARTESIAN_POINT('Ctrl Pts',(21.0896090107066,-10.2578738064183,
0.));
#218654=CARTESIAN_POINT('Ctrl Pts',(21.0896090107066,-10.2578738064183,
12.));
#218655=CARTESIAN_POINT('Ctrl Pts',(21.1031582201625,-10.2700468934743,
0.));
#218656=CARTESIAN_POINT('Ctrl Pts',(21.1031582201625,-10.2700468934743,
12.));
#218657=CARTESIAN_POINT('Ctrl Pts',(21.1167639345623,-10.2823401001067,
0.));
#218658=CARTESIAN_POINT('Ctrl Pts',(21.1167639345623,-10.2823401001067,
12.));
#218659=CARTESIAN_POINT('Ctrl Pts',(21.130424990599,-10.2947530860714,0.));
#218660=CARTESIAN_POINT('Ctrl Pts',(21.130424990599,-10.2947530860714,12.));
#218661=CARTESIAN_POINT('Ctrl Pts',(21.1441402425831,-10.307285514268,0.));
#218662=CARTESIAN_POINT('Ctrl Pts',(21.1441402425831,-10.307285514268,12.));
#218663=CARTESIAN_POINT('Ctrl Pts',(21.1579085619959,-10.3199370506541,
0.));
#218664=CARTESIAN_POINT('Ctrl Pts',(21.1579085619959,-10.3199370506541,
12.));
#218665=CARTESIAN_POINT('Ctrl Pts',(21.1717288370512,-10.3327073641574,
0.));
#218666=CARTESIAN_POINT('Ctrl Pts',(21.1717288370512,-10.3327073641574,
12.));
#218667=CARTESIAN_POINT('Ctrl Pts',(21.1855999722427,-10.3455961265706,
0.));
#218668=CARTESIAN_POINT('Ctrl Pts',(21.1855999722427,-10.3455961265706,
12.));
#218669=CARTESIAN_POINT('Ctrl Pts',(21.1995208879205,-10.3586030124595,
0.));
#218670=CARTESIAN_POINT('Ctrl Pts',(21.1995208879205,-10.3586030124595,
12.));
#218671=CARTESIAN_POINT('Ctrl Pts',(21.2134905199359,-10.3717276991137,
0.));
#218672=CARTESIAN_POINT('Ctrl Pts',(21.2134905199359,-10.3717276991137,
12.));
#218673=CARTESIAN_POINT('Ctrl Pts',(21.2275078192708,-10.384969866479,0.));
#218674=CARTESIAN_POINT('Ctrl Pts',(21.2275078192708,-10.384969866479,12.));
#218675=CARTESIAN_POINT('Ctrl Pts',(21.2415717516713,-10.3983291970846,
0.));
#218676=CARTESIAN_POINT('Ctrl Pts',(21.2415717516713,-10.3983291970846,
12.));
#218677=CARTESIAN_POINT('Ctrl Pts',(21.2556812972741,-10.4118053759584,
0.));
#218678=CARTESIAN_POINT('Ctrl Pts',(21.2556812972741,-10.4118053759584,
12.));
#218679=CARTESIAN_POINT('Ctrl Pts',(21.2698354502391,-10.4253980905394,
0.));
#218680=CARTESIAN_POINT('Ctrl Pts',(21.2698354502391,-10.4253980905394,
12.));
#218681=CARTESIAN_POINT('Ctrl Pts',(21.2840332184471,-10.4391070306385,
0.));
#218682=CARTESIAN_POINT('Ctrl Pts',(21.2840332184471,-10.4391070306385,
12.));
#218683=CARTESIAN_POINT('Ctrl Pts',(21.2982736231924,-10.452931888387,0.));
#218684=CARTESIAN_POINT('Ctrl Pts',(21.2982736231924,-10.452931888387,12.));
#218685=CARTESIAN_POINT('Ctrl Pts',(21.312555698873,-10.4668723581768,0.));
#218686=CARTESIAN_POINT('Ctrl Pts',(21.312555698873,-10.4668723581768,12.));
#218687=CARTESIAN_POINT('Ctrl Pts',(21.3268784926823,-10.4809281365933,
0.));
#218688=CARTESIAN_POINT('Ctrl Pts',(21.3268784926823,-10.4809281365933,
12.));
#218689=CARTESIAN_POINT('Ctrl Pts',(21.3412410642912,-10.4950989223341,
0.));
#218690=CARTESIAN_POINT('Ctrl Pts',(21.3412410642912,-10.4950989223341,
12.));
#218691=CARTESIAN_POINT('Ctrl Pts',(21.3556424855822,-10.509384416169,0.));
#218692=CARTESIAN_POINT('Ctrl Pts',(21.3556424855822,-10.509384416169,12.));
#218693=CARTESIAN_POINT('Ctrl Pts',(21.3700818403942,-10.523784320906,0.));
#218694=CARTESIAN_POINT('Ctrl Pts',(21.3700818403942,-10.523784320906,12.));
#218695=CARTESIAN_POINT('Ctrl Pts',(21.3845582242604,-10.5382983413422,
0.));
#218696=CARTESIAN_POINT('Ctrl Pts',(21.3845582242604,-10.5382983413422,
12.));
#218697=CARTESIAN_POINT('Ctrl Pts',(21.3990707441495,-10.5529261842107,
0.));
#218698=CARTESIAN_POINT('Ctrl Pts',(21.3990707441495,-10.5529261842107,
12.));
#218699=CARTESIAN_POINT('Ctrl Pts',(21.4136185181974,-10.5676675581106,
0.));
#218700=CARTESIAN_POINT('Ctrl Pts',(21.4136185181974,-10.5676675581106,
12.));
#218701=CARTESIAN_POINT('Ctrl Pts',(21.4282006754624,-10.582522173457,0.));
#218702=CARTESIAN_POINT('Ctrl Pts',(21.4282006754624,-10.582522173457,12.));
#218703=CARTESIAN_POINT('Ctrl Pts',(21.4428163557137,-10.597489742462,0.));
#218704=CARTESIAN_POINT('Ctrl Pts',(21.4428163557137,-10.597489742462,12.));
#218705=CARTESIAN_POINT('Ctrl Pts',(21.4574647092093,-10.612569979096,0.));
#218706=CARTESIAN_POINT('Ctrl Pts',(21.4574647092093,-10.612569979096,12.));
#218707=CARTESIAN_POINT('Ctrl Pts',(21.4721448964766,-10.6277625990457,
0.));
#218708=CARTESIAN_POINT('Ctrl Pts',(21.4721448964766,-10.6277625990457,
12.));
#218709=CARTESIAN_POINT('Ctrl Pts',(21.4868560880893,-10.6430673196609,
0.));
#218710=CARTESIAN_POINT('Ctrl Pts',(21.4868560880893,-10.6430673196609,
12.));
#218711=CARTESIAN_POINT('Ctrl Pts',(21.5015974644454,-10.6584838598941,
0.));
#218712=CARTESIAN_POINT('Ctrl Pts',(21.5015974644454,-10.6584838598941,
12.));
#218713=CARTESIAN_POINT('Ctrl Pts',(21.5163682155805,-10.6740119402835,
0.));
#218714=CARTESIAN_POINT('Ctrl Pts',(21.5163682155805,-10.6740119402835,
12.));
#218715=CARTESIAN_POINT('Ctrl Pts',(21.531167540981,-10.689651282929,0.));
#218716=CARTESIAN_POINT('Ctrl Pts',(21.531167540981,-10.689651282929,12.));
#218717=CARTESIAN_POINT('Ctrl Pts',(21.5459946493955,-10.7054016114571,
0.));
#218718=CARTESIAN_POINT('Ctrl Pts',(21.5459946493955,-10.7054016114571,
12.));
#218719=CARTESIAN_POINT('Ctrl Pts',(21.5608487586467,-10.7212626509816,
0.));
#218720=CARTESIAN_POINT('Ctrl Pts',(21.5608487586467,-10.7212626509816,
12.));
#218721=CARTESIAN_POINT('Ctrl Pts',(21.5757290954372,-10.7372341280468,
0.));
#218722=CARTESIAN_POINT('Ctrl Pts',(21.5757290954372,-10.7372341280468,
12.));
#218723=CARTESIAN_POINT('Ctrl Pts',(21.5906348951745,-10.7533157705943,
0.));
#218724=CARTESIAN_POINT('Ctrl Pts',(21.5906348951745,-10.7533157705943,
12.));
#218725=CARTESIAN_POINT('Ctrl Pts',(21.6055654018179,-10.7695073079554,
0.));
#218726=CARTESIAN_POINT('Ctrl Pts',(21.6055654018179,-10.7695073079554,
12.));
#218727=CARTESIAN_POINT('Ctrl Pts',(21.6205198677176,-10.7858084708262,
0.));
#218728=CARTESIAN_POINT('Ctrl Pts',(21.6205198677176,-10.7858084708262,
12.));
#218729=CARTESIAN_POINT('Ctrl Pts',(21.6354975534557,-10.802218991237,0.));
#218730=CARTESIAN_POINT('Ctrl Pts',(21.6354975534557,-10.802218991237,12.));
#218731=CARTESIAN_POINT('Ctrl Pts',(21.6504977276864,-10.8187386025135,
0.));
#218732=CARTESIAN_POINT('Ctrl Pts',(21.6504977276864,-10.8187386025135,
12.));
#218733=CARTESIAN_POINT('Ctrl Pts',(21.6655196669727,-10.835367039227,0.));
#218734=CARTESIAN_POINT('Ctrl Pts',(21.6655196669727,-10.835367039227,12.));
#218735=CARTESIAN_POINT('Ctrl Pts',(21.6805626556461,-10.8521040371832,
0.));
#218736=CARTESIAN_POINT('Ctrl Pts',(21.6805626556461,-10.8521040371832,
12.));
#218737=CARTESIAN_POINT('Ctrl Pts',(21.6956259856667,-10.8689493334093,
0.));
#218738=CARTESIAN_POINT('Ctrl Pts',(21.6956259856667,-10.8689493334093,
12.));
#218739=CARTESIAN_POINT('Ctrl Pts',(21.7107089564822,-10.8859026661292,
0.));
#218740=CARTESIAN_POINT('Ctrl Pts',(21.7107089564822,-10.8859026661292,
12.));
#218741=CARTESIAN_POINT('Ctrl Pts',(21.7258108748874,-10.9029637747341,
0.));
#218742=CARTESIAN_POINT('Ctrl Pts',(21.7258108748874,-10.9029637747341,
12.));
#218743=CARTESIAN_POINT('Ctrl Pts',(21.74093105488,-10.9201323997386,0.));
#218744=CARTESIAN_POINT('Ctrl Pts',(21.74093105488,-10.9201323997386,12.));
#218745=CARTESIAN_POINT('Ctrl Pts',(21.7560688175252,-10.9374082827446,
0.));
#218746=CARTESIAN_POINT('Ctrl Pts',(21.7560688175252,-10.9374082827446,
12.));
#218747=CARTESIAN_POINT('Ctrl Pts',(21.7712234908468,-10.9547911664457,
0.));
#218748=CARTESIAN_POINT('Ctrl Pts',(21.7712234908468,-10.9547911664457,
12.));
#218749=CARTESIAN_POINT('Ctrl Pts',(21.7863944097143,-10.9722807946157,
0.));
#218750=CARTESIAN_POINT('Ctrl Pts',(21.7863944097143,-10.9722807946157,
12.));
#218751=CARTESIAN_POINT('Ctrl Pts',(21.8015809157302,-10.9898769120913,
0.));
#218752=CARTESIAN_POINT('Ctrl Pts',(21.8015809157302,-10.9898769120913,
12.));
#218753=CARTESIAN_POINT('Ctrl Pts',(21.8167823571168,-11.0075792647477,
0.));
#218754=CARTESIAN_POINT('Ctrl Pts',(21.8167823571168,-11.0075792647477,
12.));
#218755=CARTESIAN_POINT('Ctrl Pts',(21.8319980886033,-11.0253875994598,
0.));
#218756=CARTESIAN_POINT('Ctrl Pts',(21.8319980886033,-11.0253875994598,
12.));
#218757=CARTESIAN_POINT('Ctrl Pts',(21.8472274713103,-11.0433016640808,
0.));
#218758=CARTESIAN_POINT('Ctrl Pts',(21.8472274713103,-11.0433016640808,
12.));
#218759=CARTESIAN_POINT('Ctrl Pts',(21.8624698726319,-11.0613212074364,
0.));
#218760=CARTESIAN_POINT('Ctrl Pts',(21.8624698726319,-11.0613212074364,
12.));
#218761=CARTESIAN_POINT('Ctrl Pts',(21.8777246661191,-11.0794459793058,
0.));
#218762=CARTESIAN_POINT('Ctrl Pts',(21.8777246661191,-11.0794459793058,
12.));
#218763=CARTESIAN_POINT('Ctrl Pts',(21.8929912313608,-11.0976757303944,
0.));
#218764=CARTESIAN_POINT('Ctrl Pts',(21.8929912313608,-11.0976757303944,
12.));
#218765=CARTESIAN_POINT('Ctrl Pts',(21.9082689538687,-11.1160102123024,
0.));
#218766=CARTESIAN_POINT('Ctrl Pts',(21.9082689538687,-11.1160102123024,
12.));
#218767=CARTESIAN_POINT('Ctrl Pts',(21.9235572249518,-11.134449177474,0.));
#218768=CARTESIAN_POINT('Ctrl Pts',(21.9235572249518,-11.134449177474,12.));
#218769=CARTESIAN_POINT('Ctrl Pts',(21.9388554416437,-11.1529923792002,
0.));
#218770=CARTESIAN_POINT('Ctrl Pts',(21.9388554416437,-11.1529923792002,
12.));
#218771=CARTESIAN_POINT('Ctrl Pts',(21.9541630066504,-11.1716395716375,
0.));
#218772=CARTESIAN_POINT('Ctrl Pts',(21.9541630066504,-11.1716395716375,
12.));
#218773=CARTESIAN_POINT('Ctrl Pts',(21.9694793282913,-11.190390509811,0.));
#218774=CARTESIAN_POINT('Ctrl Pts',(21.9694793282913,-11.190390509811,12.));
#218775=CARTESIAN_POINT('Ctrl Pts',(21.9848038204439,-11.2092449496125,
0.));
#218776=CARTESIAN_POINT('Ctrl Pts',(21.9848038204439,-11.2092449496125,
12.));
#218777=CARTESIAN_POINT('Ctrl Pts',(22.0001359024839,-11.2282026477897,
0.));
#218778=CARTESIAN_POINT('Ctrl Pts',(22.0001359024839,-11.2282026477897,
12.));
#218779=CARTESIAN_POINT('Ctrl Pts',(22.0154749992364,-11.2472633619276,
0.));
#218780=CARTESIAN_POINT('Ctrl Pts',(22.0154749992364,-11.2472633619276,
12.));
#218781=CARTESIAN_POINT('Ctrl Pts',(22.0308205408351,-11.2664268504207,
0.));
#218782=CARTESIAN_POINT('Ctrl Pts',(22.0308205408351,-11.2664268504207,
12.));
#218783=CARTESIAN_POINT('Ctrl Pts',(22.046171962566,-11.2856928724374,0.));
#218784=CARTESIAN_POINT('Ctrl Pts',(22.046171962566,-11.2856928724374,12.));
#218785=CARTESIAN_POINT('Ctrl Pts',(22.0615287047179,-11.3050611878771,
0.));
#218786=CARTESIAN_POINT('Ctrl Pts',(22.0615287047179,-11.3050611878771,
12.));
#218787=CARTESIAN_POINT('Ctrl Pts',(22.0768902124267,-11.3245315573168,
0.));
#218788=CARTESIAN_POINT('Ctrl Pts',(22.0768902124267,-11.3245315573168,
12.));
#218789=CARTESIAN_POINT('Ctrl Pts',(22.0922559355293,-11.3441037419553,
0.));
#218790=CARTESIAN_POINT('Ctrl Pts',(22.0922559355293,-11.3441037419553,
12.));
#218791=CARTESIAN_POINT('Ctrl Pts',(22.1076253283978,-11.3637775035367,
0.));
#218792=CARTESIAN_POINT('Ctrl Pts',(22.1076253283978,-11.3637775035367,
12.));
#218793=CARTESIAN_POINT('Ctrl Pts',(22.1229978500185,-11.3835526044256,
0.));
#218794=CARTESIAN_POINT('Ctrl Pts',(22.1229978500185,-11.3835526044256,
12.));
#218795=CARTESIAN_POINT('Ctrl Pts',(22.1383729640963,-11.4034288076909,
0.));
#218796=CARTESIAN_POINT('Ctrl Pts',(22.1383729640963,-11.4034288076909,
12.));
#218797=CARTESIAN_POINT('Ctrl Pts',(22.1537501391486,-11.4234058771742,
0.));
#218798=CARTESIAN_POINT('Ctrl Pts',(22.1537501391486,-11.4234058771742,
12.));
#218799=CARTESIAN_POINT('Ctrl Pts',(22.1691288486096,-11.443483577557,0.));
#218800=CARTESIAN_POINT('Ctrl Pts',(22.1691288486096,-11.443483577557,12.));
#218801=CARTESIAN_POINT('Ctrl Pts',(22.1845085709169,-11.463661674411,0.));
#218802=CARTESIAN_POINT('Ctrl Pts',(22.1845085709169,-11.463661674411,12.));
#218803=CARTESIAN_POINT('Ctrl Pts',(22.1998887896435,-11.4839399342589,
0.));
#218804=CARTESIAN_POINT('Ctrl Pts',(22.1998887896435,-11.4839399342589,
12.));
#218805=CARTESIAN_POINT('Ctrl Pts',(22.215268993102,-11.504318124424,0.));
#218806=CARTESIAN_POINT('Ctrl Pts',(22.215268993102,-11.504318124424,12.));
#218807=CARTESIAN_POINT('Ctrl Pts',(22.2306486738899,-11.5247960128476,
0.));
#218808=CARTESIAN_POINT('Ctrl Pts',(22.2306486738899,-11.5247960128476,
12.));
#218809=CARTESIAN_POINT('Ctrl Pts',(22.2460273284653,-11.545373367912,0.));
#218810=CARTESIAN_POINT('Ctrl Pts',(22.2460273284653,-11.545373367912,12.));
#218811=CARTESIAN_POINT('Ctrl Pts',(22.2614044566898,-11.5660499582403,
0.));
#218812=CARTESIAN_POINT('Ctrl Pts',(22.2614044566898,-11.5660499582403,
12.));
#218813=CARTESIAN_POINT('Ctrl Pts',(22.2767795614349,-11.5868255525189,
0.));
#218814=CARTESIAN_POINT('Ctrl Pts',(22.2767795614349,-11.5868255525189,
12.));
#218815=CARTESIAN_POINT('Ctrl Pts',(22.2921521480357,-11.6076999192359,
0.));
#218816=CARTESIAN_POINT('Ctrl Pts',(22.2921521480357,-11.6076999192359,
12.));
#218817=CARTESIAN_POINT('Ctrl Pts',(22.3075217249049,-11.6286728270011,
0.));
#218818=CARTESIAN_POINT('Ctrl Pts',(22.3075217249049,-11.6286728270011,
12.));
#218819=CARTESIAN_POINT('Ctrl Pts',(22.3228878043976,-11.6497440449858,
0.));
#218820=CARTESIAN_POINT('Ctrl Pts',(22.3228878043976,-11.6497440449858,
12.));
#218821=CARTESIAN_POINT('Ctrl Pts',(22.3382499035618,-11.6709133432986,
0.));
#218822=CARTESIAN_POINT('Ctrl Pts',(22.3382499035618,-11.6709133432986,
12.));
#218823=CARTESIAN_POINT('Ctrl Pts',(22.3536075450028,-11.6921804934056,
0.));
#218824=CARTESIAN_POINT('Ctrl Pts',(22.3536075450028,-11.6921804934056,
12.));
#218825=CARTESIAN_POINT('Ctrl Pts',(22.3689602575492,-11.7135452684532,
0.));
#218826=CARTESIAN_POINT('Ctrl Pts',(22.3689602575492,-11.7135452684532,
12.));
#218827=CARTESIAN_POINT('Ctrl Pts',(22.3843075773905,-11.7350074437961,
0.));
#218828=CARTESIAN_POINT('Ctrl Pts',(22.3843075773905,-11.7350074437961,
12.));
#218829=CARTESIAN_POINT('Ctrl Pts',(22.39964904692,-11.7565667964765,0.));
#218830=CARTESIAN_POINT('Ctrl Pts',(22.39964904692,-11.7565667964765,12.));
#218831=CARTESIAN_POINT('Ctrl Pts',(22.4149842125018,-11.7782231042041,
0.));
#218832=CARTESIAN_POINT('Ctrl Pts',(22.4149842125018,-11.7782231042041,
12.));
#218833=CARTESIAN_POINT('Ctrl Pts',(22.4303126226468,-11.7999761445175,
0.));
#218834=CARTESIAN_POINT('Ctrl Pts',(22.4303126226468,-11.7999761445175,
12.));
#218835=CARTESIAN_POINT('Ctrl Pts',(22.4456338258738,-11.8218256937889,
0.));
#218836=CARTESIAN_POINT('Ctrl Pts',(22.4456338258738,-11.8218256937889,
12.));
#218837=CARTESIAN_POINT('Ctrl Pts',(22.4609473690469,-11.8437715264487,
0.));
#218838=CARTESIAN_POINT('Ctrl Pts',(22.4609473690469,-11.8437715264487,
12.));
#218839=CARTESIAN_POINT('Ctrl Pts',(22.4762527946694,-11.8658134137018,
0.));
#218840=CARTESIAN_POINT('Ctrl Pts',(22.4762527946694,-11.8658134137018,
12.));
#218841=CARTESIAN_POINT('Ctrl Pts',(22.4915496418472,-11.8879511239941,
0.));
#218842=CARTESIAN_POINT('Ctrl Pts',(22.4915496418472,-11.8879511239941,
12.));
#218843=CARTESIAN_POINT('Ctrl Pts',(22.5068374513958,-11.9101844254555,
0.));
#218844=CARTESIAN_POINT('Ctrl Pts',(22.5068374513958,-11.9101844254555,
12.));
#218845=CARTESIAN_POINT('Ctrl Pts',(22.5221157697869,-11.9325130877801,
0.));
#218846=CARTESIAN_POINT('Ctrl Pts',(22.5221157697869,-11.9325130877801,
12.));
#218847=CARTESIAN_POINT('Ctrl Pts',(22.5373841537299,-11.9549368843996,
0.));
#218848=CARTESIAN_POINT('Ctrl Pts',(22.5373841537299,-11.9549368843996,
12.));
#218849=CARTESIAN_POINT('Ctrl Pts',(22.5526421741159,-11.9774555943496,
0.));
#218850=CARTESIAN_POINT('Ctrl Pts',(22.5526421741159,-11.9774555943496,
12.));
#218851=CARTESIAN_POINT('Ctrl Pts',(22.5678894211194,-12.0000690046697,
0.));
#218852=CARTESIAN_POINT('Ctrl Pts',(22.5678894211194,-12.0000690046697,
12.));
#218853=CARTESIAN_POINT('Ctrl Pts',(22.5831255061306,-12.0227769113132,
0.));
#218854=CARTESIAN_POINT('Ctrl Pts',(22.5831255061306,-12.0227769113132,
12.));
#218855=CARTESIAN_POINT('Ctrl Pts',(22.5983500505675,-12.0455791139135,
0.));
#218856=CARTESIAN_POINT('Ctrl Pts',(22.5983500505675,-12.0455791139135,
12.));
#218857=CARTESIAN_POINT('Ctrl Pts',(22.613562676493,-12.0684754113869,0.));
#218858=CARTESIAN_POINT('Ctrl Pts',(22.613562676493,-12.0684754113869,12.));
#218859=CARTESIAN_POINT('Ctrl Pts',(22.628762996708,-12.0914655972828,0.));
#218860=CARTESIAN_POINT('Ctrl Pts',(22.628762996708,-12.0914655972828,12.));
#218861=CARTESIAN_POINT('Ctrl Pts',(22.6439506046611,-12.1145494550384,
0.));
#218862=CARTESIAN_POINT('Ctrl Pts',(22.6439506046611,-12.1145494550384,
12.));
#218863=CARTESIAN_POINT('Ctrl Pts',(22.6591250653942,-12.1377267537141,
0.));
#218864=CARTESIAN_POINT('Ctrl Pts',(22.6591250653942,-12.1377267537141,
12.));
#218865=CARTESIAN_POINT('Ctrl Pts',(22.6742859034891,-12.1609972423089,
0.));
#218866=CARTESIAN_POINT('Ctrl Pts',(22.6742859034891,-12.1609972423089,
12.));
#218867=CARTESIAN_POINT('Ctrl Pts',(22.6894326204959,-12.1843606579246,
0.));
#218868=CARTESIAN_POINT('Ctrl Pts',(22.6894326204959,-12.1843606579246,
12.));
#218869=CARTESIAN_POINT('Ctrl Pts',(22.7045647168659,-12.2078167360267,
0.));
#218870=CARTESIAN_POINT('Ctrl Pts',(22.7045647168659,-12.2078167360267,
12.));
#218871=CARTESIAN_POINT('Ctrl Pts',(22.7196817119299,-12.2313652198047,
0.));
#218872=CARTESIAN_POINT('Ctrl Pts',(22.7196817119299,-12.2313652198047,
12.));
#218873=CARTESIAN_POINT('Ctrl Pts',(22.7347831655251,-12.2550058702389,
0.));
#218874=CARTESIAN_POINT('Ctrl Pts',(22.7347831655251,-12.2550058702389,
12.));
#218875=CARTESIAN_POINT('Ctrl Pts',(22.7498686970096,-12.2787384750747,
0.));
#218876=CARTESIAN_POINT('Ctrl Pts',(22.7498686970096,-12.2787384750747,
12.));
#218877=CARTESIAN_POINT('Ctrl Pts',(22.7649380101154,-12.3025628601812,
0.));
#218878=CARTESIAN_POINT('Ctrl Pts',(22.7649380101154,-12.3025628601812,
12.));
#218879=CARTESIAN_POINT('Ctrl Pts',(22.7799908974947,-12.3264788926108,
0.));
#218880=CARTESIAN_POINT('Ctrl Pts',(22.7799908974947,-12.3264788926108,
12.));
#218881=CARTESIAN_POINT('Ctrl Pts',(22.7950272216959,-12.3504864740361,
0.));
#218882=CARTESIAN_POINT('Ctrl Pts',(22.7950272216959,-12.3504864740361,
12.));
#218883=CARTESIAN_POINT('Ctrl Pts',(22.8100469022632,-12.3745855366772,
0.));
#218884=CARTESIAN_POINT('Ctrl Pts',(22.8100469022632,-12.3745855366772,
12.));
#218885=CARTESIAN_POINT('Ctrl Pts',(22.8220493007353,-12.393937937903,0.));
#218886=CARTESIAN_POINT('Ctrl Pts',(22.8220493007353,-12.393937937903,12.));
#218887=CARTESIAN_POINT('Ctrl Pts',(22.8310435872852,-12.4084933766366,
0.));
#218888=CARTESIAN_POINT('Ctrl Pts',(22.8310435872852,-12.4084933766366,
12.));
#218889=CARTESIAN_POINT('Ctrl Pts',(22.8370364396497,-12.4182152851867,
0.));
#218890=CARTESIAN_POINT('Ctrl Pts',(22.8370364396497,-12.4182152851867,
12.));
#218891=CARTESIAN_POINT('Ctrl Pts',(22.8400320311648,-12.4230808101438,
0.));
#218892=CARTESIAN_POINT('Ctrl Pts',(22.8400320311648,-12.4230808101438,
12.));
#218893=CARTESIAN_POINT('',(22.8400320311648,-12.4230808101438,0.));
#218894=CARTESIAN_POINT('Ctrl Pts',(20.353053841303,-9.71462809124917,0.));
#218895=CARTESIAN_POINT('Ctrl Pts',(20.353060251684,-9.71462954053074,0.));
#218896=CARTESIAN_POINT('Ctrl Pts',(20.3531126095522,-9.71465227853122,
0.));
#218897=CARTESIAN_POINT('Ctrl Pts',(20.3533097561886,-9.71474590350792,
0.));
#218898=CARTESIAN_POINT('Ctrl Pts',(20.3538098605706,-9.71498978052101,
0.));
#218899=CARTESIAN_POINT('Ctrl Pts',(20.3548282742361,-9.71549257088175,
0.));
#218900=CARTESIAN_POINT('Ctrl Pts',(20.3562337557875,-9.71619192554147,
0.));
#218901=CARTESIAN_POINT('Ctrl Pts',(20.3580133103357,-9.71708493723062,
0.));
#218902=CARTESIAN_POINT('Ctrl Pts',(20.3601498764344,-9.71816778327999,
0.));
#218903=CARTESIAN_POINT('Ctrl Pts',(20.362625691398,-9.71943648548115,0.));
#218904=CARTESIAN_POINT('Ctrl Pts',(20.3654261611055,-9.72088778381102,
0.));
#218905=CARTESIAN_POINT('Ctrl Pts',(20.3685406190576,-9.72251930722504,
0.));
#218906=CARTESIAN_POINT('Ctrl Pts',(20.371960235676,-9.72432910043193,0.));
#218907=CARTESIAN_POINT('Ctrl Pts',(20.3756766651952,-9.72631531732871,
0.));
#218908=CARTESIAN_POINT('Ctrl Pts',(20.3796805893304,-9.72847589116533,
0.));
#218909=CARTESIAN_POINT('Ctrl Pts',(20.3839624556742,-9.73080870123726,
0.));
#218910=CARTESIAN_POINT('Ctrl Pts',(20.3885129129912,-9.73331167102812,
0.));
#218911=CARTESIAN_POINT('Ctrl Pts',(20.3933234845646,-9.7359829201425,0.));
#218912=CARTESIAN_POINT('Ctrl Pts',(20.3983866213331,-9.73882077613206,
0.));
#218913=CARTESIAN_POINT('Ctrl Pts',(20.4036953576549,-9.74182369656273,
0.));
#218914=CARTESIAN_POINT('Ctrl Pts',(20.4092430879861,-9.74499021838537,
0.));
#218915=CARTESIAN_POINT('Ctrl Pts',(20.4150232777393,-9.74831889242175,
0.));
#218916=CARTESIAN_POINT('Ctrl Pts',(20.4210295275818,-9.75180829786433,
0.));
#218917=CARTESIAN_POINT('Ctrl Pts',(20.4272556476629,-9.75545705902416,
0.));
#218918=CARTESIAN_POINT('Ctrl Pts',(20.4336957355474,-9.7592638628993,0.));
#218919=CARTESIAN_POINT('Ctrl Pts',(20.4403442329401,-9.76322747195502,
0.));
#218920=CARTESIAN_POINT('Ctrl Pts',(20.447195862298,-9.76734670980897,0.));
#218921=CARTESIAN_POINT('Ctrl Pts',(20.4542455817527,-9.7716204510407,0.));
#218922=CARTESIAN_POINT('Ctrl Pts',(20.4614885274973,-9.77604760815523,
0.));
#218923=CARTESIAN_POINT('Ctrl Pts',(20.4689199790668,-9.78062712373313,
0.));
#218924=CARTESIAN_POINT('Ctrl Pts',(20.4765353711585,-9.78535797314162,
0.));
#218925=CARTESIAN_POINT('Ctrl Pts',(20.4843302955329,-9.7902391649866,0.));
#218926=CARTESIAN_POINT('Ctrl Pts',(20.4923005087945,-9.79526974288344,
0.));
#218927=CARTESIAN_POINT('Ctrl Pts',(20.500441931211,-9.80044878520968,0.));
#218928=CARTESIAN_POINT('Ctrl Pts',(20.5087506310507,-9.80577540161103,
0.));
#218929=CARTESIAN_POINT('Ctrl Pts',(20.5172228122839,-9.81124873025278,
0.));
#218930=CARTESIAN_POINT('Ctrl Pts',(20.5258548000625,-9.81686793455918,
0.));
#218931=CARTESIAN_POINT('Ctrl Pts',(20.534643029951,-9.82263220080328,0.));
#218932=CARTESIAN_POINT('Ctrl Pts',(20.5435840460717,-9.82854073773858,
0.));
#218933=CARTESIAN_POINT('Ctrl Pts',(20.5526744976461,-9.83459277585321,
0.));
#218934=CARTESIAN_POINT('Ctrl Pts',(20.5619111362406,-9.84078756677589,
0.));
#218935=CARTESIAN_POINT('Ctrl Pts',(20.5712908125145,-9.84712438256308,
0.));
#218936=CARTESIAN_POINT('Ctrl Pts',(20.580810471002,-9.85360251457004,0.));
#218937=CARTESIAN_POINT('Ctrl Pts',(20.5904671449754,-9.8602212723275,0.));
#218938=CARTESIAN_POINT('Ctrl Pts',(20.6002579513696,-9.86697998242612,
0.));
#218939=CARTESIAN_POINT('Ctrl Pts',(20.6101800854491,-9.87387798732944,
0.));
#218940=CARTESIAN_POINT('Ctrl Pts',(20.6202308177472,-9.88091464472669,
0.));
#218941=CARTESIAN_POINT('Ctrl Pts',(20.6304074914086,-9.88808932697305,
0.));
#218942=CARTESIAN_POINT('Ctrl Pts',(20.6407075193977,-9.89540142049124,
0.));
#218943=CARTESIAN_POINT('Ctrl Pts',(20.6511283817415,-9.90285032516696,
0.));
#218944=CARTESIAN_POINT('Ctrl Pts',(20.6616676228315,-9.91043545377005,
0.));
#218945=CARTESIAN_POINT('Ctrl Pts',(20.6723228488261,-9.91815623141285,
0.));
#218946=CARTESIAN_POINT('Ctrl Pts',(20.6830917250255,-9.92601209498751,
0.));
#218947=CARTESIAN_POINT('Ctrl Pts',(20.6939719732485,-9.93400249259737,
0.));
#218948=CARTESIAN_POINT('Ctrl Pts',(20.7049613692237,-9.94212688298251,
0.));
#218949=CARTESIAN_POINT('Ctrl Pts',(20.716057740758,-9.95038473514962,0.));
#218950=CARTESIAN_POINT('Ctrl Pts',(20.7272589658752,-9.95877552798403,
0.));
#218951=CARTESIAN_POINT('Ctrl Pts',(20.7385629709795,-9.96729874986199,
0.));
#218952=CARTESIAN_POINT('Ctrl Pts',(20.7499677289625,-9.97595389823461,
0.));
#218953=CARTESIAN_POINT('Ctrl Pts',(20.7614712574989,-9.98474047926846,
0.));
#218954=CARTESIAN_POINT('Ctrl Pts',(20.7730716175417,-9.99365800754638,
0.));
#218955=CARTESIAN_POINT('Ctrl Pts',(20.7847669117568,-10.0027060057389,
0.));
#218956=CARTESIAN_POINT('Ctrl Pts',(20.7965552829907,-10.0118840042786,
0.));
#218957=CARTESIAN_POINT('Ctrl Pts',(20.8084349126885,-10.0211915410095,
0.));
#218958=CARTESIAN_POINT('Ctrl Pts',(20.8204040196599,-10.0306281609435,
0.));
#218959=CARTESIAN_POINT('Ctrl Pts',(20.8324608588906,-10.0401934160234,
0.));
#218960=CARTESIAN_POINT('Ctrl Pts',(20.8446037203402,-10.0498868648733,
0.));
#218961=CARTESIAN_POINT('Ctrl Pts',(20.856830927732,-10.0597080725375,0.));
#218962=CARTESIAN_POINT('Ctrl Pts',(20.8691408373705,-10.0696566102219,
0.));
#218963=CARTESIAN_POINT('Ctrl Pts',(20.8815318371844,-10.0797320551154,
0.));
#218964=CARTESIAN_POINT('Ctrl Pts',(20.8940023457371,-10.0899339901916,
0.));
#218965=CARTESIAN_POINT('Ctrl Pts',(20.9065508112556,-10.1002620040076,
0.));
#218966=CARTESIAN_POINT('Ctrl Pts',(20.9191757106266,-10.1107156904836,
0.));
#218967=CARTESIAN_POINT('Ctrl Pts',(20.931875548473,-10.1212946487057,0.));
#218968=CARTESIAN_POINT('Ctrl Pts',(20.944648856393,-10.1319984827909,0.));
#218969=CARTESIAN_POINT('Ctrl Pts',(20.9574941921591,-10.1428268017257,
0.));
#218970=CARTESIAN_POINT('Ctrl Pts',(20.970410138937,-10.1537792192065,0.));
#218971=CARTESIAN_POINT('Ctrl Pts',(20.9833953044736,-10.1648553534567,
0.));
#218972=CARTESIAN_POINT('Ctrl Pts',(20.9964483203685,-10.1760548270765,
0.));
#218973=CARTESIAN_POINT('Ctrl Pts',(21.0095678414486,-10.1873772669358,
0.));
#218974=CARTESIAN_POINT('Ctrl Pts',(21.0227525451107,-10.1988223040425,
0.));
#218975=CARTESIAN_POINT('Ctrl Pts',(21.0360011306814,-10.2103895734124,
0.));
#218976=CARTESIAN_POINT('Ctrl Pts',(21.0493123187483,-10.2220787139157,
0.));
#218977=CARTESIAN_POINT('Ctrl Pts',(21.0626848505665,-10.233889368157,0.));
#218978=CARTESIAN_POINT('Ctrl Pts',(21.0761174875448,-10.2458211823915,
0.));
#218979=CARTESIAN_POINT('Ctrl Pts',(21.0896090107066,-10.2578738064183,
0.));
#218980=CARTESIAN_POINT('Ctrl Pts',(21.1031582201625,-10.2700468934743,
0.));
#218981=CARTESIAN_POINT('Ctrl Pts',(21.1167639345623,-10.2823401001067,
0.));
#218982=CARTESIAN_POINT('Ctrl Pts',(21.130424990599,-10.2947530860714,0.));
#218983=CARTESIAN_POINT('Ctrl Pts',(21.1441402425831,-10.307285514268,0.));
#218984=CARTESIAN_POINT('Ctrl Pts',(21.1579085619959,-10.3199370506541,
0.));
#218985=CARTESIAN_POINT('Ctrl Pts',(21.1717288370512,-10.3327073641574,
0.));
#218986=CARTESIAN_POINT('Ctrl Pts',(21.1855999722427,-10.3455961265706,
0.));
#218987=CARTESIAN_POINT('Ctrl Pts',(21.1995208879205,-10.3586030124595,
0.));
#218988=CARTESIAN_POINT('Ctrl Pts',(21.2134905199359,-10.3717276991137,
0.));
#218989=CARTESIAN_POINT('Ctrl Pts',(21.2275078192708,-10.384969866479,0.));
#218990=CARTESIAN_POINT('Ctrl Pts',(21.2415717516713,-10.3983291970846,
0.));
#218991=CARTESIAN_POINT('Ctrl Pts',(21.2556812972741,-10.4118053759584,
0.));
#218992=CARTESIAN_POINT('Ctrl Pts',(21.2698354502391,-10.4253980905394,
0.));
#218993=CARTESIAN_POINT('Ctrl Pts',(21.2840332184471,-10.4391070306385,
0.));
#218994=CARTESIAN_POINT('Ctrl Pts',(21.2982736231924,-10.452931888387,0.));
#218995=CARTESIAN_POINT('Ctrl Pts',(21.312555698873,-10.4668723581768,0.));
#218996=CARTESIAN_POINT('Ctrl Pts',(21.3268784926823,-10.4809281365933,
0.));
#218997=CARTESIAN_POINT('Ctrl Pts',(21.3412410642912,-10.4950989223341,
0.));
#218998=CARTESIAN_POINT('Ctrl Pts',(21.3556424855822,-10.509384416169,0.));
#218999=CARTESIAN_POINT('Ctrl Pts',(21.3700818403942,-10.523784320906,0.));
#219000=CARTESIAN_POINT('Ctrl Pts',(21.3845582242604,-10.5382983413422,
0.));
#219001=CARTESIAN_POINT('Ctrl Pts',(21.3990707441495,-10.5529261842107,
0.));
#219002=CARTESIAN_POINT('Ctrl Pts',(21.4136185181974,-10.5676675581106,
0.));
#219003=CARTESIAN_POINT('Ctrl Pts',(21.4282006754624,-10.582522173457,0.));
#219004=CARTESIAN_POINT('Ctrl Pts',(21.4428163557137,-10.597489742462,0.));
#219005=CARTESIAN_POINT('Ctrl Pts',(21.4574647092093,-10.612569979096,0.));
#219006=CARTESIAN_POINT('Ctrl Pts',(21.4721448964766,-10.6277625990457,
0.));
#219007=CARTESIAN_POINT('Ctrl Pts',(21.4868560880893,-10.6430673196609,
0.));
#219008=CARTESIAN_POINT('Ctrl Pts',(21.5015974644454,-10.6584838598941,
0.));
#219009=CARTESIAN_POINT('Ctrl Pts',(21.5163682155805,-10.6740119402835,
0.));
#219010=CARTESIAN_POINT('Ctrl Pts',(21.531167540981,-10.689651282929,0.));
#219011=CARTESIAN_POINT('Ctrl Pts',(21.5459946493955,-10.7054016114571,
0.));
#219012=CARTESIAN_POINT('Ctrl Pts',(21.5608487586467,-10.7212626509816,
0.));
#219013=CARTESIAN_POINT('Ctrl Pts',(21.5757290954372,-10.7372341280468,
0.));
#219014=CARTESIAN_POINT('Ctrl Pts',(21.5906348951745,-10.7533157705943,
0.));
#219015=CARTESIAN_POINT('Ctrl Pts',(21.6055654018179,-10.7695073079554,
0.));
#219016=CARTESIAN_POINT('Ctrl Pts',(21.6205198677176,-10.7858084708262,
0.));
#219017=CARTESIAN_POINT('Ctrl Pts',(21.6354975534557,-10.802218991237,0.));
#219018=CARTESIAN_POINT('Ctrl Pts',(21.6504977276864,-10.8187386025135,
0.));
#219019=CARTESIAN_POINT('Ctrl Pts',(21.6655196669727,-10.835367039227,0.));
#219020=CARTESIAN_POINT('Ctrl Pts',(21.6805626556461,-10.8521040371832,
0.));
#219021=CARTESIAN_POINT('Ctrl Pts',(21.6956259856667,-10.8689493334093,
0.));
#219022=CARTESIAN_POINT('Ctrl Pts',(21.7107089564822,-10.8859026661292,
0.));
#219023=CARTESIAN_POINT('Ctrl Pts',(21.7258108748874,-10.9029637747341,
0.));
#219024=CARTESIAN_POINT('Ctrl Pts',(21.74093105488,-10.9201323997386,0.));
#219025=CARTESIAN_POINT('Ctrl Pts',(21.7560688175252,-10.9374082827446,
0.));
#219026=CARTESIAN_POINT('Ctrl Pts',(21.7712234908468,-10.9547911664457,
0.));
#219027=CARTESIAN_POINT('Ctrl Pts',(21.7863944097143,-10.9722807946157,
0.));
#219028=CARTESIAN_POINT('Ctrl Pts',(21.8015809157302,-10.9898769120913,
0.));
#219029=CARTESIAN_POINT('Ctrl Pts',(21.8167823571168,-11.0075792647477,
0.));
#219030=CARTESIAN_POINT('Ctrl Pts',(21.8319980886033,-11.0253875994598,
0.));
#219031=CARTESIAN_POINT('Ctrl Pts',(21.8472274713103,-11.0433016640808,
0.));
#219032=CARTESIAN_POINT('Ctrl Pts',(21.8624698726319,-11.0613212074364,
0.));
#219033=CARTESIAN_POINT('Ctrl Pts',(21.8777246661191,-11.0794459793058,
0.));
#219034=CARTESIAN_POINT('Ctrl Pts',(21.8929912313608,-11.0976757303944,
0.));
#219035=CARTESIAN_POINT('Ctrl Pts',(21.9082689538687,-11.1160102123024,
0.));
#219036=CARTESIAN_POINT('Ctrl Pts',(21.9235572249518,-11.134449177474,0.));
#219037=CARTESIAN_POINT('Ctrl Pts',(21.9388554416437,-11.1529923792002,
0.));
#219038=CARTESIAN_POINT('Ctrl Pts',(21.9541630066504,-11.1716395716375,
0.));
#219039=CARTESIAN_POINT('Ctrl Pts',(21.9694793282913,-11.190390509811,0.));
#219040=CARTESIAN_POINT('Ctrl Pts',(21.9848038204439,-11.2092449496125,
0.));
#219041=CARTESIAN_POINT('Ctrl Pts',(22.0001359024839,-11.2282026477897,
0.));
#219042=CARTESIAN_POINT('Ctrl Pts',(22.0154749992364,-11.2472633619276,
0.));
#219043=CARTESIAN_POINT('Ctrl Pts',(22.0308205408351,-11.2664268504207,
0.));
#219044=CARTESIAN_POINT('Ctrl Pts',(22.046171962566,-11.2856928724374,0.));
#219045=CARTESIAN_POINT('Ctrl Pts',(22.0615287047179,-11.3050611878771,
0.));
#219046=CARTESIAN_POINT('Ctrl Pts',(22.0768902124267,-11.3245315573168,
0.));
#219047=CARTESIAN_POINT('Ctrl Pts',(22.0922559355293,-11.3441037419553,
0.));
#219048=CARTESIAN_POINT('Ctrl Pts',(22.1076253283978,-11.3637775035367,
0.));
#219049=CARTESIAN_POINT('Ctrl Pts',(22.1229978500185,-11.3835526044256,
0.));
#219050=CARTESIAN_POINT('Ctrl Pts',(22.1383729640963,-11.4034288076909,
0.));
#219051=CARTESIAN_POINT('Ctrl Pts',(22.1537501391486,-11.4234058771742,
0.));
#219052=CARTESIAN_POINT('Ctrl Pts',(22.1691288486096,-11.443483577557,0.));
#219053=CARTESIAN_POINT('Ctrl Pts',(22.1845085709169,-11.463661674411,0.));
#219054=CARTESIAN_POINT('Ctrl Pts',(22.1998887896435,-11.4839399342589,
0.));
#219055=CARTESIAN_POINT('Ctrl Pts',(22.215268993102,-11.504318124424,0.));
#219056=CARTESIAN_POINT('Ctrl Pts',(22.2306486738899,-11.5247960128476,
0.));
#219057=CARTESIAN_POINT('Ctrl Pts',(22.2460273284653,-11.545373367912,0.));
#219058=CARTESIAN_POINT('Ctrl Pts',(22.2614044566898,-11.5660499582403,
0.));
#219059=CARTESIAN_POINT('Ctrl Pts',(22.2767795614349,-11.5868255525189,
0.));
#219060=CARTESIAN_POINT('Ctrl Pts',(22.2921521480357,-11.6076999192359,
0.));
#219061=CARTESIAN_POINT('Ctrl Pts',(22.3075217249049,-11.6286728270011,
0.));
#219062=CARTESIAN_POINT('Ctrl Pts',(22.3228878043976,-11.6497440449858,
0.));
#219063=CARTESIAN_POINT('Ctrl Pts',(22.3382499035618,-11.6709133432986,
0.));
#219064=CARTESIAN_POINT('Ctrl Pts',(22.3536075450028,-11.6921804934056,
0.));
#219065=CARTESIAN_POINT('Ctrl Pts',(22.3689602575492,-11.7135452684532,
0.));
#219066=CARTESIAN_POINT('Ctrl Pts',(22.3843075773905,-11.7350074437961,
0.));
#219067=CARTESIAN_POINT('Ctrl Pts',(22.39964904692,-11.7565667964765,0.));
#219068=CARTESIAN_POINT('Ctrl Pts',(22.4149842125018,-11.7782231042041,
0.));
#219069=CARTESIAN_POINT('Ctrl Pts',(22.4303126226468,-11.7999761445175,
0.));
#219070=CARTESIAN_POINT('Ctrl Pts',(22.4456338258738,-11.8218256937889,
0.));
#219071=CARTESIAN_POINT('Ctrl Pts',(22.4609473690469,-11.8437715264487,
0.));
#219072=CARTESIAN_POINT('Ctrl Pts',(22.4762527946694,-11.8658134137018,
0.));
#219073=CARTESIAN_POINT('Ctrl Pts',(22.4915496418472,-11.8879511239941,
0.));
#219074=CARTESIAN_POINT('Ctrl Pts',(22.5068374513958,-11.9101844254555,
0.));
#219075=CARTESIAN_POINT('Ctrl Pts',(22.5221157697869,-11.9325130877801,
0.));
#219076=CARTESIAN_POINT('Ctrl Pts',(22.5373841537299,-11.9549368843996,
0.));
#219077=CARTESIAN_POINT('Ctrl Pts',(22.5526421741159,-11.9774555943496,
0.));
#219078=CARTESIAN_POINT('Ctrl Pts',(22.5678894211194,-12.0000690046697,
0.));
#219079=CARTESIAN_POINT('Ctrl Pts',(22.5831255061306,-12.0227769113132,
0.));
#219080=CARTESIAN_POINT('Ctrl Pts',(22.5983500505675,-12.0455791139135,
0.));
#219081=CARTESIAN_POINT('Ctrl Pts',(22.613562676493,-12.0684754113869,0.));
#219082=CARTESIAN_POINT('Ctrl Pts',(22.628762996708,-12.0914655972828,0.));
#219083=CARTESIAN_POINT('Ctrl Pts',(22.6439506046611,-12.1145494550384,
0.));
#219084=CARTESIAN_POINT('Ctrl Pts',(22.6591250653942,-12.1377267537141,
0.));
#219085=CARTESIAN_POINT('Ctrl Pts',(22.6742859034891,-12.1609972423089,
0.));
#219086=CARTESIAN_POINT('Ctrl Pts',(22.6894326204959,-12.1843606579246,
0.));
#219087=CARTESIAN_POINT('Ctrl Pts',(22.7045647168659,-12.2078167360267,
0.));
#219088=CARTESIAN_POINT('Ctrl Pts',(22.7196817119299,-12.2313652198047,
0.));
#219089=CARTESIAN_POINT('Ctrl Pts',(22.7347831655251,-12.2550058702389,
0.));
#219090=CARTESIAN_POINT('Ctrl Pts',(22.7498686970096,-12.2787384750747,
0.));
#219091=CARTESIAN_POINT('Ctrl Pts',(22.7649380101154,-12.3025628601812,
0.));
#219092=CARTESIAN_POINT('Ctrl Pts',(22.7799908974947,-12.3264788926108,
0.));
#219093=CARTESIAN_POINT('Ctrl Pts',(22.7950272216959,-12.3504864740361,
0.));
#219094=CARTESIAN_POINT('Ctrl Pts',(22.8100469022632,-12.3745855366772,
0.));
#219095=CARTESIAN_POINT('Ctrl Pts',(22.8220493007353,-12.393937937903,0.));
#219096=CARTESIAN_POINT('Ctrl Pts',(22.8310435872852,-12.4084933766366,
0.));
#219097=CARTESIAN_POINT('Ctrl Pts',(22.8370364396497,-12.4182152851867,
0.));
#219098=CARTESIAN_POINT('Ctrl Pts',(22.8400320311648,-12.4230808101438,
0.));
#219099=CARTESIAN_POINT('',(22.8400320311648,-12.4230808101438,12.));
#219100=CARTESIAN_POINT('Ctrl Pts',(22.8400320311648,-12.4230808101438,
12.));
#219101=CARTESIAN_POINT('Ctrl Pts',(22.8370364396497,-12.4182152851867,
12.));
#219102=CARTESIAN_POINT('Ctrl Pts',(22.8310435872852,-12.4084933766366,
12.));
#219103=CARTESIAN_POINT('Ctrl Pts',(22.8220493007353,-12.393937937903,12.));
#219104=CARTESIAN_POINT('Ctrl Pts',(22.8100469022632,-12.3745855366772,
12.));
#219105=CARTESIAN_POINT('Ctrl Pts',(22.7950272216959,-12.3504864740361,
12.));
#219106=CARTESIAN_POINT('Ctrl Pts',(22.7799908974947,-12.3264788926108,
12.));
#219107=CARTESIAN_POINT('Ctrl Pts',(22.7649380101154,-12.3025628601812,
12.));
#219108=CARTESIAN_POINT('Ctrl Pts',(22.7498686970096,-12.2787384750747,
12.));
#219109=CARTESIAN_POINT('Ctrl Pts',(22.7347831655251,-12.2550058702389,
12.));
#219110=CARTESIAN_POINT('Ctrl Pts',(22.7196817119299,-12.2313652198047,
12.));
#219111=CARTESIAN_POINT('Ctrl Pts',(22.7045647168659,-12.2078167360267,
12.));
#219112=CARTESIAN_POINT('Ctrl Pts',(22.6894326204959,-12.1843606579246,
12.));
#219113=CARTESIAN_POINT('Ctrl Pts',(22.6742859034891,-12.1609972423089,
12.));
#219114=CARTESIAN_POINT('Ctrl Pts',(22.6591250653942,-12.1377267537141,
12.));
#219115=CARTESIAN_POINT('Ctrl Pts',(22.6439506046611,-12.1145494550384,
12.));
#219116=CARTESIAN_POINT('Ctrl Pts',(22.628762996708,-12.0914655972828,12.));
#219117=CARTESIAN_POINT('Ctrl Pts',(22.613562676493,-12.0684754113869,12.));
#219118=CARTESIAN_POINT('Ctrl Pts',(22.5983500505675,-12.0455791139135,
12.));
#219119=CARTESIAN_POINT('Ctrl Pts',(22.5831255061306,-12.0227769113132,
12.));
#219120=CARTESIAN_POINT('Ctrl Pts',(22.5678894211194,-12.0000690046697,
12.));
#219121=CARTESIAN_POINT('Ctrl Pts',(22.5526421741159,-11.9774555943496,
12.));
#219122=CARTESIAN_POINT('Ctrl Pts',(22.5373841537299,-11.9549368843996,
12.));
#219123=CARTESIAN_POINT('Ctrl Pts',(22.5221157697869,-11.9325130877801,
12.));
#219124=CARTESIAN_POINT('Ctrl Pts',(22.5068374513958,-11.9101844254555,
12.));
#219125=CARTESIAN_POINT('Ctrl Pts',(22.4915496418472,-11.8879511239941,
12.));
#219126=CARTESIAN_POINT('Ctrl Pts',(22.4762527946694,-11.8658134137018,
12.));
#219127=CARTESIAN_POINT('Ctrl Pts',(22.4609473690469,-11.8437715264487,
12.));
#219128=CARTESIAN_POINT('Ctrl Pts',(22.4456338258738,-11.8218256937889,
12.));
#219129=CARTESIAN_POINT('Ctrl Pts',(22.4303126226468,-11.7999761445175,
12.));
#219130=CARTESIAN_POINT('Ctrl Pts',(22.4149842125018,-11.7782231042041,
12.));
#219131=CARTESIAN_POINT('Ctrl Pts',(22.39964904692,-11.7565667964765,12.));
#219132=CARTESIAN_POINT('Ctrl Pts',(22.3843075773905,-11.7350074437961,
12.));
#219133=CARTESIAN_POINT('Ctrl Pts',(22.3689602575492,-11.7135452684532,
12.));
#219134=CARTESIAN_POINT('Ctrl Pts',(22.3536075450028,-11.6921804934056,
12.));
#219135=CARTESIAN_POINT('Ctrl Pts',(22.3382499035618,-11.6709133432986,
12.));
#219136=CARTESIAN_POINT('Ctrl Pts',(22.3228878043976,-11.6497440449858,
12.));
#219137=CARTESIAN_POINT('Ctrl Pts',(22.3075217249049,-11.6286728270011,
12.));
#219138=CARTESIAN_POINT('Ctrl Pts',(22.2921521480357,-11.6076999192359,
12.));
#219139=CARTESIAN_POINT('Ctrl Pts',(22.2767795614349,-11.5868255525189,
12.));
#219140=CARTESIAN_POINT('Ctrl Pts',(22.2614044566898,-11.5660499582403,
12.));
#219141=CARTESIAN_POINT('Ctrl Pts',(22.2460273284653,-11.545373367912,12.));
#219142=CARTESIAN_POINT('Ctrl Pts',(22.2306486738899,-11.5247960128476,
12.));
#219143=CARTESIAN_POINT('Ctrl Pts',(22.215268993102,-11.504318124424,12.));
#219144=CARTESIAN_POINT('Ctrl Pts',(22.1998887896435,-11.4839399342589,
12.));
#219145=CARTESIAN_POINT('Ctrl Pts',(22.1845085709169,-11.463661674411,12.));
#219146=CARTESIAN_POINT('Ctrl Pts',(22.1691288486096,-11.443483577557,12.));
#219147=CARTESIAN_POINT('Ctrl Pts',(22.1537501391486,-11.4234058771742,
12.));
#219148=CARTESIAN_POINT('Ctrl Pts',(22.1383729640963,-11.4034288076909,
12.));
#219149=CARTESIAN_POINT('Ctrl Pts',(22.1229978500185,-11.3835526044256,
12.));
#219150=CARTESIAN_POINT('Ctrl Pts',(22.1076253283978,-11.3637775035367,
12.));
#219151=CARTESIAN_POINT('Ctrl Pts',(22.0922559355293,-11.3441037419553,
12.));
#219152=CARTESIAN_POINT('Ctrl Pts',(22.0768902124267,-11.3245315573168,
12.));
#219153=CARTESIAN_POINT('Ctrl Pts',(22.0615287047179,-11.3050611878771,
12.));
#219154=CARTESIAN_POINT('Ctrl Pts',(22.046171962566,-11.2856928724374,12.));
#219155=CARTESIAN_POINT('Ctrl Pts',(22.0308205408351,-11.2664268504207,
12.));
#219156=CARTESIAN_POINT('Ctrl Pts',(22.0154749992364,-11.2472633619276,
12.));
#219157=CARTESIAN_POINT('Ctrl Pts',(22.0001359024839,-11.2282026477897,
12.));
#219158=CARTESIAN_POINT('Ctrl Pts',(21.9848038204439,-11.2092449496125,
12.));
#219159=CARTESIAN_POINT('Ctrl Pts',(21.9694793282913,-11.190390509811,12.));
#219160=CARTESIAN_POINT('Ctrl Pts',(21.9541630066504,-11.1716395716375,
12.));
#219161=CARTESIAN_POINT('Ctrl Pts',(21.9388554416437,-11.1529923792002,
12.));
#219162=CARTESIAN_POINT('Ctrl Pts',(21.9235572249518,-11.134449177474,12.));
#219163=CARTESIAN_POINT('Ctrl Pts',(21.9082689538687,-11.1160102123024,
12.));
#219164=CARTESIAN_POINT('Ctrl Pts',(21.8929912313608,-11.0976757303944,
12.));
#219165=CARTESIAN_POINT('Ctrl Pts',(21.8777246661191,-11.0794459793058,
12.));
#219166=CARTESIAN_POINT('Ctrl Pts',(21.8624698726319,-11.0613212074364,
12.));
#219167=CARTESIAN_POINT('Ctrl Pts',(21.8472274713103,-11.0433016640808,
12.));
#219168=CARTESIAN_POINT('Ctrl Pts',(21.8319980886033,-11.0253875994598,
12.));
#219169=CARTESIAN_POINT('Ctrl Pts',(21.8167823571168,-11.0075792647477,
12.));
#219170=CARTESIAN_POINT('Ctrl Pts',(21.8015809157302,-10.9898769120913,
12.));
#219171=CARTESIAN_POINT('Ctrl Pts',(21.7863944097143,-10.9722807946157,
12.));
#219172=CARTESIAN_POINT('Ctrl Pts',(21.7712234908468,-10.9547911664457,
12.));
#219173=CARTESIAN_POINT('Ctrl Pts',(21.7560688175252,-10.9374082827446,
12.));
#219174=CARTESIAN_POINT('Ctrl Pts',(21.74093105488,-10.9201323997386,12.));
#219175=CARTESIAN_POINT('Ctrl Pts',(21.7258108748874,-10.9029637747341,
12.));
#219176=CARTESIAN_POINT('Ctrl Pts',(21.7107089564822,-10.8859026661292,
12.));
#219177=CARTESIAN_POINT('Ctrl Pts',(21.6956259856667,-10.8689493334093,
12.));
#219178=CARTESIAN_POINT('Ctrl Pts',(21.6805626556461,-10.8521040371832,
12.));
#219179=CARTESIAN_POINT('Ctrl Pts',(21.6655196669727,-10.835367039227,12.));
#219180=CARTESIAN_POINT('Ctrl Pts',(21.6504977276864,-10.8187386025135,
12.));
#219181=CARTESIAN_POINT('Ctrl Pts',(21.6354975534557,-10.802218991237,12.));
#219182=CARTESIAN_POINT('Ctrl Pts',(21.6205198677176,-10.7858084708262,
12.));
#219183=CARTESIAN_POINT('Ctrl Pts',(21.6055654018179,-10.7695073079554,
12.));
#219184=CARTESIAN_POINT('Ctrl Pts',(21.5906348951745,-10.7533157705943,
12.));
#219185=CARTESIAN_POINT('Ctrl Pts',(21.5757290954372,-10.7372341280468,
12.));
#219186=CARTESIAN_POINT('Ctrl Pts',(21.5608487586467,-10.7212626509816,
12.));
#219187=CARTESIAN_POINT('Ctrl Pts',(21.5459946493955,-10.7054016114571,
12.));
#219188=CARTESIAN_POINT('Ctrl Pts',(21.531167540981,-10.689651282929,12.));
#219189=CARTESIAN_POINT('Ctrl Pts',(21.5163682155805,-10.6740119402835,
12.));
#219190=CARTESIAN_POINT('Ctrl Pts',(21.5015974644454,-10.6584838598941,
12.));
#219191=CARTESIAN_POINT('Ctrl Pts',(21.4868560880893,-10.6430673196609,
12.));
#219192=CARTESIAN_POINT('Ctrl Pts',(21.4721448964766,-10.6277625990457,
12.));
#219193=CARTESIAN_POINT('Ctrl Pts',(21.4574647092093,-10.612569979096,12.));
#219194=CARTESIAN_POINT('Ctrl Pts',(21.4428163557137,-10.597489742462,12.));
#219195=CARTESIAN_POINT('Ctrl Pts',(21.4282006754624,-10.582522173457,12.));
#219196=CARTESIAN_POINT('Ctrl Pts',(21.4136185181974,-10.5676675581106,
12.));
#219197=CARTESIAN_POINT('Ctrl Pts',(21.3990707441495,-10.5529261842107,
12.));
#219198=CARTESIAN_POINT('Ctrl Pts',(21.3845582242604,-10.5382983413422,
12.));
#219199=CARTESIAN_POINT('Ctrl Pts',(21.3700818403942,-10.523784320906,12.));
#219200=CARTESIAN_POINT('Ctrl Pts',(21.3556424855822,-10.509384416169,12.));
#219201=CARTESIAN_POINT('Ctrl Pts',(21.3412410642912,-10.4950989223341,
12.));
#219202=CARTESIAN_POINT('Ctrl Pts',(21.3268784926823,-10.4809281365933,
12.));
#219203=CARTESIAN_POINT('Ctrl Pts',(21.312555698873,-10.4668723581768,12.));
#219204=CARTESIAN_POINT('Ctrl Pts',(21.2982736231924,-10.452931888387,12.));
#219205=CARTESIAN_POINT('Ctrl Pts',(21.2840332184471,-10.4391070306385,
12.));
#219206=CARTESIAN_POINT('Ctrl Pts',(21.2698354502391,-10.4253980905394,
12.));
#219207=CARTESIAN_POINT('Ctrl Pts',(21.2556812972741,-10.4118053759584,
12.));
#219208=CARTESIAN_POINT('Ctrl Pts',(21.2415717516713,-10.3983291970846,
12.));
#219209=CARTESIAN_POINT('Ctrl Pts',(21.2275078192708,-10.384969866479,12.));
#219210=CARTESIAN_POINT('Ctrl Pts',(21.2134905199359,-10.3717276991137,
12.));
#219211=CARTESIAN_POINT('Ctrl Pts',(21.1995208879205,-10.3586030124595,
12.));
#219212=CARTESIAN_POINT('Ctrl Pts',(21.1855999722427,-10.3455961265706,
12.));
#219213=CARTESIAN_POINT('Ctrl Pts',(21.1717288370512,-10.3327073641574,
12.));
#219214=CARTESIAN_POINT('Ctrl Pts',(21.1579085619959,-10.3199370506541,
12.));
#219215=CARTESIAN_POINT('Ctrl Pts',(21.1441402425831,-10.307285514268,12.));
#219216=CARTESIAN_POINT('Ctrl Pts',(21.130424990599,-10.2947530860714,12.));
#219217=CARTESIAN_POINT('Ctrl Pts',(21.1167639345623,-10.2823401001067,
12.));
#219218=CARTESIAN_POINT('Ctrl Pts',(21.1031582201625,-10.2700468934743,
12.));
#219219=CARTESIAN_POINT('Ctrl Pts',(21.0896090107066,-10.2578738064183,
12.));
#219220=CARTESIAN_POINT('Ctrl Pts',(21.0761174875448,-10.2458211823915,
12.));
#219221=CARTESIAN_POINT('Ctrl Pts',(21.0626848505665,-10.233889368157,12.));
#219222=CARTESIAN_POINT('Ctrl Pts',(21.0493123187483,-10.2220787139157,
12.));
#219223=CARTESIAN_POINT('Ctrl Pts',(21.0360011306814,-10.2103895734124,
12.));
#219224=CARTESIAN_POINT('Ctrl Pts',(21.0227525451107,-10.1988223040425,
12.));
#219225=CARTESIAN_POINT('Ctrl Pts',(21.0095678414486,-10.1873772669358,
12.));
#219226=CARTESIAN_POINT('Ctrl Pts',(20.9964483203685,-10.1760548270765,
12.));
#219227=CARTESIAN_POINT('Ctrl Pts',(20.9833953044736,-10.1648553534567,
12.));
#219228=CARTESIAN_POINT('Ctrl Pts',(20.970410138937,-10.1537792192065,12.));
#219229=CARTESIAN_POINT('Ctrl Pts',(20.9574941921591,-10.1428268017257,
12.));
#219230=CARTESIAN_POINT('Ctrl Pts',(20.944648856393,-10.1319984827909,12.));
#219231=CARTESIAN_POINT('Ctrl Pts',(20.931875548473,-10.1212946487057,12.));
#219232=CARTESIAN_POINT('Ctrl Pts',(20.9191757106266,-10.1107156904836,
12.));
#219233=CARTESIAN_POINT('Ctrl Pts',(20.9065508112556,-10.1002620040076,
12.));
#219234=CARTESIAN_POINT('Ctrl Pts',(20.8940023457371,-10.0899339901916,
12.));
#219235=CARTESIAN_POINT('Ctrl Pts',(20.8815318371844,-10.0797320551154,
12.));
#219236=CARTESIAN_POINT('Ctrl Pts',(20.8691408373705,-10.0696566102219,
12.));
#219237=CARTESIAN_POINT('Ctrl Pts',(20.856830927732,-10.0597080725375,12.));
#219238=CARTESIAN_POINT('Ctrl Pts',(20.8446037203402,-10.0498868648733,
12.));
#219239=CARTESIAN_POINT('Ctrl Pts',(20.8324608588906,-10.0401934160234,
12.));
#219240=CARTESIAN_POINT('Ctrl Pts',(20.8204040196599,-10.0306281609435,
12.));
#219241=CARTESIAN_POINT('Ctrl Pts',(20.8084349126885,-10.0211915410095,
12.));
#219242=CARTESIAN_POINT('Ctrl Pts',(20.7965552829907,-10.0118840042786,
12.));
#219243=CARTESIAN_POINT('Ctrl Pts',(20.7847669117568,-10.0027060057389,
12.));
#219244=CARTESIAN_POINT('Ctrl Pts',(20.7730716175417,-9.99365800754638,
12.));
#219245=CARTESIAN_POINT('Ctrl Pts',(20.7614712574989,-9.98474047926846,
12.));
#219246=CARTESIAN_POINT('Ctrl Pts',(20.7499677289625,-9.97595389823461,
12.));
#219247=CARTESIAN_POINT('Ctrl Pts',(20.7385629709795,-9.96729874986199,
12.));
#219248=CARTESIAN_POINT('Ctrl Pts',(20.7272589658752,-9.95877552798403,
12.));
#219249=CARTESIAN_POINT('Ctrl Pts',(20.716057740758,-9.95038473514962,12.));
#219250=CARTESIAN_POINT('Ctrl Pts',(20.7049613692237,-9.94212688298251,
12.));
#219251=CARTESIAN_POINT('Ctrl Pts',(20.6939719732485,-9.93400249259737,
12.));
#219252=CARTESIAN_POINT('Ctrl Pts',(20.6830917250255,-9.92601209498751,
12.));
#219253=CARTESIAN_POINT('Ctrl Pts',(20.6723228488261,-9.91815623141285,
12.));
#219254=CARTESIAN_POINT('Ctrl Pts',(20.6616676228315,-9.91043545377005,
12.));
#219255=CARTESIAN_POINT('Ctrl Pts',(20.6511283817415,-9.90285032516696,
12.));
#219256=CARTESIAN_POINT('Ctrl Pts',(20.6407075193977,-9.89540142049124,
12.));
#219257=CARTESIAN_POINT('Ctrl Pts',(20.6304074914086,-9.88808932697305,
12.));
#219258=CARTESIAN_POINT('Ctrl Pts',(20.6202308177472,-9.88091464472669,
12.));
#219259=CARTESIAN_POINT('Ctrl Pts',(20.6101800854491,-9.87387798732944,
12.));
#219260=CARTESIAN_POINT('Ctrl Pts',(20.6002579513696,-9.86697998242612,
12.));
#219261=CARTESIAN_POINT('Ctrl Pts',(20.5904671449754,-9.8602212723275,12.));
#219262=CARTESIAN_POINT('Ctrl Pts',(20.580810471002,-9.85360251457004,12.));
#219263=CARTESIAN_POINT('Ctrl Pts',(20.5712908125145,-9.84712438256308,
12.));
#219264=CARTESIAN_POINT('Ctrl Pts',(20.5619111362406,-9.84078756677589,
12.));
#219265=CARTESIAN_POINT('Ctrl Pts',(20.5526744976461,-9.83459277585321,
12.));
#219266=CARTESIAN_POINT('Ctrl Pts',(20.5435840460717,-9.82854073773858,
12.));
#219267=CARTESIAN_POINT('Ctrl Pts',(20.534643029951,-9.82263220080328,12.));
#219268=CARTESIAN_POINT('Ctrl Pts',(20.5258548000625,-9.81686793455918,
12.));
#219269=CARTESIAN_POINT('Ctrl Pts',(20.5172228122839,-9.81124873025278,
12.));
#219270=CARTESIAN_POINT('Ctrl Pts',(20.5087506310507,-9.80577540161103,
12.));
#219271=CARTESIAN_POINT('Ctrl Pts',(20.500441931211,-9.80044878520968,12.));
#219272=CARTESIAN_POINT('Ctrl Pts',(20.4923005087945,-9.79526974288344,
12.));
#219273=CARTESIAN_POINT('Ctrl Pts',(20.4843302955329,-9.7902391649866,12.));
#219274=CARTESIAN_POINT('Ctrl Pts',(20.4765353711585,-9.78535797314162,
12.));
#219275=CARTESIAN_POINT('Ctrl Pts',(20.4689199790668,-9.78062712373313,
12.));
#219276=CARTESIAN_POINT('Ctrl Pts',(20.4614885274973,-9.77604760815523,
12.));
#219277=CARTESIAN_POINT('Ctrl Pts',(20.4542455817527,-9.7716204510407,12.));
#219278=CARTESIAN_POINT('Ctrl Pts',(20.447195862298,-9.76734670980897,12.));
#219279=CARTESIAN_POINT('Ctrl Pts',(20.4403442329401,-9.76322747195502,
12.));
#219280=CARTESIAN_POINT('Ctrl Pts',(20.4336957355474,-9.7592638628993,12.));
#219281=CARTESIAN_POINT('Ctrl Pts',(20.4272556476629,-9.75545705902416,
12.));
#219282=CARTESIAN_POINT('Ctrl Pts',(20.4210295275818,-9.75180829786433,
12.));
#219283=CARTESIAN_POINT('Ctrl Pts',(20.4150232777393,-9.74831889242175,
12.));
#219284=CARTESIAN_POINT('Ctrl Pts',(20.4092430879861,-9.74499021838537,
12.));
#219285=CARTESIAN_POINT('Ctrl Pts',(20.4036953576549,-9.74182369656273,
12.));
#219286=CARTESIAN_POINT('Ctrl Pts',(20.3983866213331,-9.73882077613206,
12.));
#219287=CARTESIAN_POINT('Ctrl Pts',(20.3933234845646,-9.7359829201425,12.));
#219288=CARTESIAN_POINT('Ctrl Pts',(20.3885129129912,-9.73331167102812,
12.));
#219289=CARTESIAN_POINT('Ctrl Pts',(20.3839624556742,-9.73080870123726,
12.));
#219290=CARTESIAN_POINT('Ctrl Pts',(20.3796805893304,-9.72847589116533,
12.));
#219291=CARTESIAN_POINT('Ctrl Pts',(20.3756766651952,-9.72631531732871,
12.));
#219292=CARTESIAN_POINT('Ctrl Pts',(20.371960235676,-9.72432910043193,12.));
#219293=CARTESIAN_POINT('Ctrl Pts',(20.3685406190576,-9.72251930722504,
12.));
#219294=CARTESIAN_POINT('Ctrl Pts',(20.3654261611055,-9.72088778381102,
12.));
#219295=CARTESIAN_POINT('Ctrl Pts',(20.362625691398,-9.71943648548115,12.));
#219296=CARTESIAN_POINT('Ctrl Pts',(20.3601498764344,-9.71816778327999,
12.));
#219297=CARTESIAN_POINT('Ctrl Pts',(20.3580133103357,-9.71708493723062,
12.));
#219298=CARTESIAN_POINT('Ctrl Pts',(20.3562337557875,-9.71619192554147,
12.));
#219299=CARTESIAN_POINT('Ctrl Pts',(20.3548282742361,-9.71549257088175,
12.));
#219300=CARTESIAN_POINT('Ctrl Pts',(20.3538098605706,-9.71498978052101,
12.));
#219301=CARTESIAN_POINT('Ctrl Pts',(20.3533097561886,-9.71474590350792,
12.));
#219302=CARTESIAN_POINT('Ctrl Pts',(20.3531126095522,-9.71465227853122,
12.));
#219303=CARTESIAN_POINT('Ctrl Pts',(20.353060251684,-9.71462954053074,12.));
#219304=CARTESIAN_POINT('Ctrl Pts',(20.353053841303,-9.71462809124917,12.));
#219305=CARTESIAN_POINT('',(22.8400320311648,-12.4230808101438,0.));
#219306=CARTESIAN_POINT('Origin',(16.3449727195351,-13.9675290154577,0.));
#219307=CARTESIAN_POINT('',(17.1452095830632,-14.6513681262571,12.));
#219308=CARTESIAN_POINT('',(8.17248635976757,-6.98376450772884,12.));
#219309=CARTESIAN_POINT('',(17.1452095830632,-14.6513681262571,0.));
#219310=CARTESIAN_POINT('',(17.1452095830632,-14.6513681262571,0.));
#219311=CARTESIAN_POINT('',(8.17248635976757,-6.98376450772884,0.));
#219312=CARTESIAN_POINT('Ctrl Pts',(22.1787195904339,-13.5685075571671,
0.));
#219313=CARTESIAN_POINT('Ctrl Pts',(22.1787195904339,-13.5685075571671,
12.));
#219314=CARTESIAN_POINT('Ctrl Pts',(22.1730081264583,-13.5683460612913,
0.));
#219315=CARTESIAN_POINT('Ctrl Pts',(22.1730081264583,-13.5683460612913,
12.));
#219316=CARTESIAN_POINT('Ctrl Pts',(22.1615922804939,-13.5680170531724,
0.));
#219317=CARTESIAN_POINT('Ctrl Pts',(22.1615922804939,-13.5680170531724,
12.));
#219318=CARTESIAN_POINT('Ctrl Pts',(22.1444897575076,-13.5675054918922,
0.));
#219319=CARTESIAN_POINT('Ctrl Pts',(22.1444897575076,-13.5675054918922,
12.));
#219320=CARTESIAN_POINT('Ctrl Pts',(22.1217288871823,-13.5667873105179,
0.));
#219321=CARTESIAN_POINT('Ctrl Pts',(22.1217288871823,-13.5667873105179,
12.));
#219322=CARTESIAN_POINT('Ctrl Pts',(22.0933486464442,-13.5658294169106,
0.));
#219323=CARTESIAN_POINT('Ctrl Pts',(22.0933486464442,-13.5658294169106,
12.));
#219324=CARTESIAN_POINT('Ctrl Pts',(22.0650393089492,-13.5648113688895,
0.));
#219325=CARTESIAN_POINT('Ctrl Pts',(22.0650393089492,-13.5648113688895,
12.));
#219326=CARTESIAN_POINT('Ctrl Pts',(22.0368009736227,-13.5637332022393,
0.));
#219327=CARTESIAN_POINT('Ctrl Pts',(22.0368009736227,-13.5637332022393,
12.));
#219328=CARTESIAN_POINT('Ctrl Pts',(22.0086337943431,-13.5625949868313,
0.));
#219329=CARTESIAN_POINT('Ctrl Pts',(22.0086337943431,-13.5625949868313,
12.));
#219330=CARTESIAN_POINT('Ctrl Pts',(21.9805379899192,-13.5613968357589,
0.));
#219331=CARTESIAN_POINT('Ctrl Pts',(21.9805379899192,-13.5613968357589,
12.));
#219332=CARTESIAN_POINT('Ctrl Pts',(21.9525138592862,-13.5601389185315,
0.));
#219333=CARTESIAN_POINT('Ctrl Pts',(21.9525138592862,-13.5601389185315,
12.));
#219334=CARTESIAN_POINT('Ctrl Pts',(21.9245617765827,-13.5588214586672,
0.));
#219335=CARTESIAN_POINT('Ctrl Pts',(21.9245617765827,-13.5588214586672,
12.));
#219336=CARTESIAN_POINT('Ctrl Pts',(21.8966821688876,-13.5574447178485,
0.));
#219337=CARTESIAN_POINT('Ctrl Pts',(21.8966821688876,-13.5574447178485,
12.));
#219338=CARTESIAN_POINT('Ctrl Pts',(21.8688754989401,-13.5560089839426,
0.));
#219339=CARTESIAN_POINT('Ctrl Pts',(21.8688754989401,-13.5560089839426,
12.));
#219340=CARTESIAN_POINT('Ctrl Pts',(21.841142245609,-13.5545145573048,0.));
#219341=CARTESIAN_POINT('Ctrl Pts',(21.841142245609,-13.5545145573048,12.));
#219342=CARTESIAN_POINT('Ctrl Pts',(21.8134828857963,-13.5529617381569,
0.));
#219343=CARTESIAN_POINT('Ctrl Pts',(21.8134828857963,-13.5529617381569,
12.));
#219344=CARTESIAN_POINT('Ctrl Pts',(21.7858978745848,-13.5513508127232,
0.));
#219345=CARTESIAN_POINT('Ctrl Pts',(21.7858978745848,-13.5513508127232,
12.));
#219346=CARTESIAN_POINT('Ctrl Pts',(21.7583876294532,-13.5496820422186,
0.));
#219347=CARTESIAN_POINT('Ctrl Pts',(21.7583876294532,-13.5496820422186,
12.));
#219348=CARTESIAN_POINT('Ctrl Pts',(21.730952541226,-13.5479556704457,0.));
#219349=CARTESIAN_POINT('Ctrl Pts',(21.730952541226,-13.5479556704457,12.));
#219350=CARTESIAN_POINT('Ctrl Pts',(21.7035929822939,-13.546171929503,0.));
#219351=CARTESIAN_POINT('Ctrl Pts',(21.7035929822939,-13.546171929503,12.));
#219352=CARTESIAN_POINT('Ctrl Pts',(21.676309315769,-13.5443310461516,0.));
#219353=CARTESIAN_POINT('Ctrl Pts',(21.676309315769,-13.5443310461516,12.));
#219354=CARTESIAN_POINT('Ctrl Pts',(21.6491019044647,-13.5424332480698,
0.));
#219355=CARTESIAN_POINT('Ctrl Pts',(21.6491019044647,-13.5424332480698,
12.));
#219356=CARTESIAN_POINT('Ctrl Pts',(21.6219711193951,-13.5404787697798,
0.));
#219357=CARTESIAN_POINT('Ctrl Pts',(21.6219711193951,-13.5404787697798,
12.));
#219358=CARTESIAN_POINT('Ctrl Pts',(21.5949173499022,-13.5384678597206,
0.));
#219359=CARTESIAN_POINT('Ctrl Pts',(21.5949173499022,-13.5384678597206,
12.));
#219360=CARTESIAN_POINT('Ctrl Pts',(21.5679410019011,-13.5364007790292,
0.));
#219361=CARTESIAN_POINT('Ctrl Pts',(21.5679410019011,-13.5364007790292,
12.));
#219362=CARTESIAN_POINT('Ctrl Pts',(21.5410424932511,-13.5342777983225,
0.));
#219363=CARTESIAN_POINT('Ctrl Pts',(21.5410424932511,-13.5342777983225,
12.));
#219364=CARTESIAN_POINT('Ctrl Pts',(21.5142222501671,-13.5320991952145,
0.));
#219365=CARTESIAN_POINT('Ctrl Pts',(21.5142222501671,-13.5320991952145,
12.));
#219366=CARTESIAN_POINT('Ctrl Pts',(21.487480703047,-13.5298652514357,0.));
#219367=CARTESIAN_POINT('Ctrl Pts',(21.487480703047,-13.5298652514357,12.));
#219368=CARTESIAN_POINT('Ctrl Pts',(21.4608182828695,-13.5275762503553,
0.));
#219369=CARTESIAN_POINT('Ctrl Pts',(21.4608182828695,-13.5275762503553,
12.));
#219370=CARTESIAN_POINT('Ctrl Pts',(21.4342354165254,-13.5252324737795,
0.));
#219371=CARTESIAN_POINT('Ctrl Pts',(21.4342354165254,-13.5252324737795,
12.));
#219372=CARTESIAN_POINT('Ctrl Pts',(21.4077325259318,-13.5228342013508,
0.));
#219373=CARTESIAN_POINT('Ctrl Pts',(21.4077325259318,-13.5228342013508,
12.));
#219374=CARTESIAN_POINT('Ctrl Pts',(21.3813100304967,-13.5203817122497,
0.));
#219375=CARTESIAN_POINT('Ctrl Pts',(21.3813100304967,-13.5203817122497,
12.));
#219376=CARTESIAN_POINT('Ctrl Pts',(21.3549683486219,-13.5178752862461,
0.));
#219377=CARTESIAN_POINT('Ctrl Pts',(21.3549683486219,-13.5178752862461,
12.));
#219378=CARTESIAN_POINT('Ctrl Pts',(21.328707899634,-13.5153152050554,0.));
#219379=CARTESIAN_POINT('Ctrl Pts',(21.328707899634,-13.5153152050554,12.));
#219380=CARTESIAN_POINT('Ctrl Pts',(21.3025291054236,-13.5127017534972,
0.));
#219381=CARTESIAN_POINT('Ctrl Pts',(21.3025291054236,-13.5127017534972,
12.));
#219382=CARTESIAN_POINT('Ctrl Pts',(21.2764323924442,-13.5100352209207,
0.));
#219383=CARTESIAN_POINT('Ctrl Pts',(21.2764323924442,-13.5100352209207,
12.));
#219384=CARTESIAN_POINT('Ctrl Pts',(21.2504181927429,-13.5073159019454,
0.));
#219385=CARTESIAN_POINT('Ctrl Pts',(21.2504181927429,-13.5073159019454,
12.));
#219386=CARTESIAN_POINT('Ctrl Pts',(21.224486942933,-13.5045440957404,0.));
#219387=CARTESIAN_POINT('Ctrl Pts',(21.224486942933,-13.5045440957404,12.));
#219388=CARTESIAN_POINT('Ctrl Pts',(21.1986390835825,-13.5017201056088,
0.));
#219389=CARTESIAN_POINT('Ctrl Pts',(21.1986390835825,-13.5017201056088,
12.));
#219390=CARTESIAN_POINT('Ctrl Pts',(21.1728750584173,-13.4988442384491,
0.));
#219391=CARTESIAN_POINT('Ctrl Pts',(21.1728750584173,-13.4988442384491,
12.));
#219392=CARTESIAN_POINT('Ctrl Pts',(21.1471953136209,-13.4959168042934,
0.));
#219393=CARTESIAN_POINT('Ctrl Pts',(21.1471953136209,-13.4959168042934,
12.));
#219394=CARTESIAN_POINT('Ctrl Pts',(21.1216002970209,-13.4929381157778,
0.));
#219395=CARTESIAN_POINT('Ctrl Pts',(21.1216002970209,-13.4929381157778,
12.));
#219396=CARTESIAN_POINT('Ctrl Pts',(21.0960904575048,-13.4899084877718,
0.));
#219397=CARTESIAN_POINT('Ctrl Pts',(21.0960904575048,-13.4899084877718,
12.));
#219398=CARTESIAN_POINT('Ctrl Pts',(21.0706662455202,-13.4868282377192,
0.));
#219399=CARTESIAN_POINT('Ctrl Pts',(21.0706662455202,-13.4868282377192,
12.));
#219400=CARTESIAN_POINT('Ctrl Pts',(21.0453281134247,-13.4836976858912,
0.));
#219401=CARTESIAN_POINT('Ctrl Pts',(21.0453281134247,-13.4836976858912,
12.));
#219402=CARTESIAN_POINT('Ctrl Pts',(21.0200765158885,-13.4805171556822,
0.));
#219403=CARTESIAN_POINT('Ctrl Pts',(21.0200765158885,-13.4805171556822,
12.));
#219404=CARTESIAN_POINT('Ctrl Pts',(20.9949119102592,-13.4772869738879,
0.));
#219405=CARTESIAN_POINT('Ctrl Pts',(20.9949119102592,-13.4772869738879,
12.));
#219406=CARTESIAN_POINT('Ctrl Pts',(20.9698347569476,-13.4740074710087,
0.));
#219407=CARTESIAN_POINT('Ctrl Pts',(20.9698347569476,-13.4740074710087,
12.));
#219408=CARTESIAN_POINT('Ctrl Pts',(20.9448455197557,-13.4706789815166,
0.));
#219409=CARTESIAN_POINT('Ctrl Pts',(20.9448455197557,-13.4706789815166,
12.));
#219410=CARTESIAN_POINT('Ctrl Pts',(20.9199446657584,-13.4673018437718,
0.));
#219411=CARTESIAN_POINT('Ctrl Pts',(20.9199446657584,-13.4673018437718,
12.));
#219412=CARTESIAN_POINT('Ctrl Pts',(20.8951326652158,-13.4638763999725,
0.));
#219413=CARTESIAN_POINT('Ctrl Pts',(20.8951326652158,-13.4638763999725,
12.));
#219414=CARTESIAN_POINT('Ctrl Pts',(20.8704099914641,-13.4604029960983,
0.));
#219415=CARTESIAN_POINT('Ctrl Pts',(20.8704099914641,-13.4604029960983,
12.));
#219416=CARTESIAN_POINT('Ctrl Pts',(20.8457771208082,-13.4568819818631,
0.));
#219417=CARTESIAN_POINT('Ctrl Pts',(20.8457771208082,-13.4568819818631,
12.));
#219418=CARTESIAN_POINT('Ctrl Pts',(20.821234532398,-13.4533137106667,0.));
#219419=CARTESIAN_POINT('Ctrl Pts',(20.821234532398,-13.4533137106667,12.));
#219420=CARTESIAN_POINT('Ctrl Pts',(20.7967827081227,-13.4496985395637,
0.));
#219421=CARTESIAN_POINT('Ctrl Pts',(20.7967827081227,-13.4496985395637,
12.));
#219422=CARTESIAN_POINT('Ctrl Pts',(20.7724221327608,-13.4460368293688,
0.));
#219423=CARTESIAN_POINT('Ctrl Pts',(20.7724221327608,-13.4460368293688,
12.));
#219424=CARTESIAN_POINT('Ctrl Pts',(20.7481532941013,-13.4423289447561,
0.));
#219425=CARTESIAN_POINT('Ctrl Pts',(20.7481532941013,-13.4423289447561,
12.));
#219426=CARTESIAN_POINT('Ctrl Pts',(20.7239766830675,-13.4385752543663,
0.));
#219427=CARTESIAN_POINT('Ctrl Pts',(20.7239766830675,-13.4385752543663,
12.));
#219428=CARTESIAN_POINT('Ctrl Pts',(20.6998927938288,-13.4347761309154,
0.));
#219429=CARTESIAN_POINT('Ctrl Pts',(20.6998927938288,-13.4347761309154,
12.));
#219430=CARTESIAN_POINT('Ctrl Pts',(20.6759021239103,-13.4309319513119,
0.));
#219431=CARTESIAN_POINT('Ctrl Pts',(20.6759021239103,-13.4309319513119,
12.));
#219432=CARTESIAN_POINT('Ctrl Pts',(20.6520051742869,-13.4270430967651,
0.));
#219433=CARTESIAN_POINT('Ctrl Pts',(20.6520051742869,-13.4270430967651,
12.));
#219434=CARTESIAN_POINT('Ctrl Pts',(20.6282024494237,-13.4231099528179,
0.));
#219435=CARTESIAN_POINT('Ctrl Pts',(20.6282024494237,-13.4231099528179,
12.));
#219436=CARTESIAN_POINT('Ctrl Pts',(20.6044944573153,-13.4191329093933,
0.));
#219437=CARTESIAN_POINT('Ctrl Pts',(20.6044944573153,-13.4191329093933,
12.));
#219438=CARTESIAN_POINT('Ctrl Pts',(20.5808817095155,-13.4151123608411,
0.));
#219439=CARTESIAN_POINT('Ctrl Pts',(20.5808817095155,-13.4151123608411,
12.));
#219440=CARTESIAN_POINT('Ctrl Pts',(20.5573647211639,-13.4110487059912,
0.));
#219441=CARTESIAN_POINT('Ctrl Pts',(20.5573647211639,-13.4110487059912,
12.));
#219442=CARTESIAN_POINT('Ctrl Pts',(20.5339440109956,-13.4069423482076,
0.));
#219443=CARTESIAN_POINT('Ctrl Pts',(20.5339440109956,-13.4069423482076,
12.));
#219444=CARTESIAN_POINT('Ctrl Pts',(20.5106201013753,-13.4027936954529,
0.));
#219445=CARTESIAN_POINT('Ctrl Pts',(20.5106201013753,-13.4027936954529,
12.));
#219446=CARTESIAN_POINT('Ctrl Pts',(20.487393518404,-13.3986031603716,0.));
#219447=CARTESIAN_POINT('Ctrl Pts',(20.487393518404,-13.3986031603716,12.));
#219448=CARTESIAN_POINT('Ctrl Pts',(20.4642647920038,-13.3943711603739,
0.));
#219449=CARTESIAN_POINT('Ctrl Pts',(20.4642647920038,-13.3943711603739,
12.));
#219450=CARTESIAN_POINT('Ctrl Pts',(20.4412344560008,-13.3900981177255,
0.));
#219451=CARTESIAN_POINT('Ctrl Pts',(20.4412344560008,-13.3900981177255,
12.));
#219452=CARTESIAN_POINT('Ctrl Pts',(20.4183030482002,-13.3857844596387,
0.));
#219453=CARTESIAN_POINT('Ctrl Pts',(20.4183030482002,-13.3857844596387,
12.));
#219454=CARTESIAN_POINT('Ctrl Pts',(20.3954711104502,-13.3814306183719,
0.));
#219455=CARTESIAN_POINT('Ctrl Pts',(20.3954711104502,-13.3814306183719,
12.));
#219456=CARTESIAN_POINT('Ctrl Pts',(20.3727391887184,-13.3770370313188,
0.));
#219457=CARTESIAN_POINT('Ctrl Pts',(20.3727391887184,-13.3770370313188,
12.));
#219458=CARTESIAN_POINT('Ctrl Pts',(20.3501078331814,-13.3726041410867,
0.));
#219459=CARTESIAN_POINT('Ctrl Pts',(20.3501078331814,-13.3726041410867,
12.));
#219460=CARTESIAN_POINT('Ctrl Pts',(20.3275775983029,-13.3681323955826,
0.));
#219461=CARTESIAN_POINT('Ctrl Pts',(20.3275775983029,-13.3681323955826,
12.));
#219462=CARTESIAN_POINT('Ctrl Pts',(20.3051490429048,-13.3636222481016,
0.));
#219463=CARTESIAN_POINT('Ctrl Pts',(20.3051490429048,-13.3636222481016,
12.));
#219464=CARTESIAN_POINT('Ctrl Pts',(20.2828227302339,-13.3590741574195,
0.));
#219465=CARTESIAN_POINT('Ctrl Pts',(20.2828227302339,-13.3590741574195,
12.));
#219466=CARTESIAN_POINT('Ctrl Pts',(20.2605992280122,-13.3544885878889,
0.));
#219467=CARTESIAN_POINT('Ctrl Pts',(20.2605992280122,-13.3544885878889,
12.));
#219468=CARTESIAN_POINT('Ctrl Pts',(20.2384791085359,-13.3498660095386,
0.));
#219469=CARTESIAN_POINT('Ctrl Pts',(20.2384791085359,-13.3498660095386,
12.));
#219470=CARTESIAN_POINT('Ctrl Pts',(20.216462948786,-13.3452068981766,0.));
#219471=CARTESIAN_POINT('Ctrl Pts',(20.216462948786,-13.3452068981766,12.));
#219472=CARTESIAN_POINT('Ctrl Pts',(20.1945513305235,-13.3405117354971,
0.));
#219473=CARTESIAN_POINT('Ctrl Pts',(20.1945513305235,-13.3405117354971,
12.));
#219474=CARTESIAN_POINT('Ctrl Pts',(20.1727448403817,-13.3357810091903,
0.));
#219475=CARTESIAN_POINT('Ctrl Pts',(20.1727448403817,-13.3357810091903,
12.));
#219476=CARTESIAN_POINT('Ctrl Pts',(20.1510440699474,-13.3310152130564,
0.));
#219477=CARTESIAN_POINT('Ctrl Pts',(20.1510440699474,-13.3310152130564,
12.));
#219478=CARTESIAN_POINT('Ctrl Pts',(20.1294496158402,-13.3262148471226,
0.));
#219479=CARTESIAN_POINT('Ctrl Pts',(20.1294496158402,-13.3262148471226,
12.));
#219480=CARTESIAN_POINT('Ctrl Pts',(20.1079620798375,-13.3213804177587,
0.));
#219481=CARTESIAN_POINT('Ctrl Pts',(20.1079620798375,-13.3213804177587,
12.));
#219482=CARTESIAN_POINT('Ctrl Pts',(20.0865820689882,-13.3165124377963,
0.));
#219483=CARTESIAN_POINT('Ctrl Pts',(20.0865820689882,-13.3165124377963,
12.));
#219484=CARTESIAN_POINT('Ctrl Pts',(20.0653101957188,-13.3116114266515,
0.));
#219485=CARTESIAN_POINT('Ctrl Pts',(20.0653101957188,-13.3116114266515,
12.));
#219486=CARTESIAN_POINT('Ctrl Pts',(20.0441470779345,-13.3066779104515,
0.));
#219487=CARTESIAN_POINT('Ctrl Pts',(20.0441470779345,-13.3066779104515,
12.));
#219488=CARTESIAN_POINT('Ctrl Pts',(20.0230933391038,-13.3017124221637,
0.));
#219489=CARTESIAN_POINT('Ctrl Pts',(20.0230933391038,-13.3017124221637,
12.));
#219490=CARTESIAN_POINT('Ctrl Pts',(20.0021496083738,-13.2967155017306,
0.));
#219491=CARTESIAN_POINT('Ctrl Pts',(20.0021496083738,-13.2967155017306,
12.));
#219492=CARTESIAN_POINT('Ctrl Pts',(19.981316520717,-13.2916876962094,0.));
#219493=CARTESIAN_POINT('Ctrl Pts',(19.981316520717,-13.2916876962094,12.));
#219494=CARTESIAN_POINT('Ctrl Pts',(19.9605947170586,-13.286629559915,0.));
#219495=CARTESIAN_POINT('Ctrl Pts',(19.9605947170586,-13.286629559915,12.));
#219496=CARTESIAN_POINT('Ctrl Pts',(19.9399848444019,-13.2815416545663,
0.));
#219497=CARTESIAN_POINT('Ctrl Pts',(19.9399848444019,-13.2815416545663,
12.));
#219498=CARTESIAN_POINT('Ctrl Pts',(19.9194875559422,-13.2764245494357,
0.));
#219499=CARTESIAN_POINT('Ctrl Pts',(19.9194875559422,-13.2764245494357,
12.));
#219500=CARTESIAN_POINT('Ctrl Pts',(19.8991035111745,-13.271278821502,0.));
#219501=CARTESIAN_POINT('Ctrl Pts',(19.8991035111745,-13.271278821502,12.));
#219502=CARTESIAN_POINT('Ctrl Pts',(19.8788333760577,-13.2661050556132,
0.));
#219503=CARTESIAN_POINT('Ctrl Pts',(19.8788333760577,-13.2661050556132,
12.));
#219504=CARTESIAN_POINT('Ctrl Pts',(19.8586778231715,-13.2609038446529,
0.));
#219505=CARTESIAN_POINT('Ctrl Pts',(19.8586778231715,-13.2609038446529,
12.));
#219506=CARTESIAN_POINT('Ctrl Pts',(19.8386375318634,-13.2556757897086,
0.));
#219507=CARTESIAN_POINT('Ctrl Pts',(19.8386375318634,-13.2556757897086,
12.));
#219508=CARTESIAN_POINT('Ctrl Pts',(19.8187131883917,-13.2504215002457,
0.));
#219509=CARTESIAN_POINT('Ctrl Pts',(19.8187131883917,-13.2504215002457,
12.));
#219510=CARTESIAN_POINT('Ctrl Pts',(19.7989054860495,-13.2451415942805,
0.));
#219511=CARTESIAN_POINT('Ctrl Pts',(19.7989054860495,-13.2451415942805,
12.));
#219512=CARTESIAN_POINT('Ctrl Pts',(19.7792151253289,-13.2398366985675,
0.));
#219513=CARTESIAN_POINT('Ctrl Pts',(19.7792151253289,-13.2398366985675,
12.));
#219514=CARTESIAN_POINT('Ctrl Pts',(19.7596428141168,-13.2345074487963,
0.));
#219515=CARTESIAN_POINT('Ctrl Pts',(19.7596428141168,-13.2345074487963,
12.));
#219516=CARTESIAN_POINT('Ctrl Pts',(19.7401892678697,-13.2291544897899,
0.));
#219517=CARTESIAN_POINT('Ctrl Pts',(19.7401892678697,-13.2291544897899,
12.));
#219518=CARTESIAN_POINT('Ctrl Pts',(19.7208552097868,-13.2237784757065,
0.));
#219519=CARTESIAN_POINT('Ctrl Pts',(19.7208552097868,-13.2237784757065,
12.));
#219520=CARTESIAN_POINT('Ctrl Pts',(19.7016413709685,-13.2183800702436,
0.));
#219521=CARTESIAN_POINT('Ctrl Pts',(19.7016413709685,-13.2183800702436,
12.));
#219522=CARTESIAN_POINT('Ctrl Pts',(19.6825484905823,-13.2129599468485,
0.));
#219523=CARTESIAN_POINT('Ctrl Pts',(19.6825484905823,-13.2129599468485,
12.));
#219524=CARTESIAN_POINT('Ctrl Pts',(19.6635773160936,-13.2075187889529,
0.));
#219525=CARTESIAN_POINT('Ctrl Pts',(19.6635773160936,-13.2075187889529,
12.));
#219526=CARTESIAN_POINT('Ctrl Pts',(19.6447286034772,-13.2020572902065,
0.));
#219527=CARTESIAN_POINT('Ctrl Pts',(19.6447286034772,-13.2020572902065,
12.));
#219528=CARTESIAN_POINT('Ctrl Pts',(19.6260031174244,-13.1965761547151,
0.));
#219529=CARTESIAN_POINT('Ctrl Pts',(19.6260031174244,-13.1965761547151,
12.));
#219530=CARTESIAN_POINT('Ctrl Pts',(19.6074016315414,-13.1910760972814,
0.));
#219531=CARTESIAN_POINT('Ctrl Pts',(19.6074016315414,-13.1910760972814,
12.));
#219532=CARTESIAN_POINT('Ctrl Pts',(19.5889249285338,-13.1855578436471,
0.));
#219533=CARTESIAN_POINT('Ctrl Pts',(19.5889249285338,-13.1855578436471,
12.));
#219534=CARTESIAN_POINT('Ctrl Pts',(19.5705738004667,-13.1800221307673,
0.));
#219535=CARTESIAN_POINT('Ctrl Pts',(19.5705738004667,-13.1800221307673,
12.));
#219536=CARTESIAN_POINT('Ctrl Pts',(19.5523490490244,-13.1744697070911,
0.));
#219537=CARTESIAN_POINT('Ctrl Pts',(19.5523490490244,-13.1744697070911,
12.));
#219538=CARTESIAN_POINT('Ctrl Pts',(19.5342514857562,-13.168901332843,0.));
#219539=CARTESIAN_POINT('Ctrl Pts',(19.5342514857562,-13.168901332843,12.));
#219540=CARTESIAN_POINT('Ctrl Pts',(19.5162819323213,-13.1633177803101,
0.));
#219541=CARTESIAN_POINT('Ctrl Pts',(19.5162819323213,-13.1633177803101,
12.));
#219542=CARTESIAN_POINT('Ctrl Pts',(19.4984412207082,-13.1577198341245,
0.));
#219543=CARTESIAN_POINT('Ctrl Pts',(19.4984412207082,-13.1577198341245,
12.));
#219544=CARTESIAN_POINT('Ctrl Pts',(19.4807301935268,-13.1521082915853,
0.));
#219545=CARTESIAN_POINT('Ctrl Pts',(19.4807301935268,-13.1521082915853,
12.));
#219546=CARTESIAN_POINT('Ctrl Pts',(19.4631497043258,-13.1464839629971,
0.));
#219547=CARTESIAN_POINT('Ctrl Pts',(19.4631497043258,-13.1464839629971,
12.));
#219548=CARTESIAN_POINT('Ctrl Pts',(19.4457006178876,-13.1408476720061,
0.));
#219549=CARTESIAN_POINT('Ctrl Pts',(19.4457006178876,-13.1408476720061,
12.));
#219550=CARTESIAN_POINT('Ctrl Pts',(19.4283838105262,-13.1352002559438,
0.));
#219551=CARTESIAN_POINT('Ctrl Pts',(19.4283838105262,-13.1352002559438,
12.));
#219552=CARTESIAN_POINT('Ctrl Pts',(19.4112001703557,-13.1295425661634,
0.));
#219553=CARTESIAN_POINT('Ctrl Pts',(19.4112001703557,-13.1295425661634,
12.));
#219554=CARTESIAN_POINT('Ctrl Pts',(19.3941505976263,-13.1238754684177,
0.));
#219555=CARTESIAN_POINT('Ctrl Pts',(19.3941505976263,-13.1238754684177,
12.));
#219556=CARTESIAN_POINT('Ctrl Pts',(19.3772360051091,-13.118199843271,0.));
#219557=CARTESIAN_POINT('Ctrl Pts',(19.3772360051091,-13.118199843271,12.));
#219558=CARTESIAN_POINT('Ctrl Pts',(19.3604573184515,-13.1125165865022,
0.));
#219559=CARTESIAN_POINT('Ctrl Pts',(19.3604573184515,-13.1125165865022,
12.));
#219560=CARTESIAN_POINT('Ctrl Pts',(19.3438154765395,-13.1068266095186,
0.));
#219561=CARTESIAN_POINT('Ctrl Pts',(19.3438154765395,-13.1068266095186,
12.));
#219562=CARTESIAN_POINT('Ctrl Pts',(19.3273114318269,-13.1011308397591,
0.));
#219563=CARTESIAN_POINT('Ctrl Pts',(19.3273114318269,-13.1011308397591,
12.));
#219564=CARTESIAN_POINT('Ctrl Pts',(19.310946150736,-13.0954302211479,0.));
#219565=CARTESIAN_POINT('Ctrl Pts',(19.310946150736,-13.0954302211479,12.));
#219566=CARTESIAN_POINT('Ctrl Pts',(19.2947206141247,-13.0897257145969,
0.));
#219567=CARTESIAN_POINT('Ctrl Pts',(19.2947206141247,-13.0897257145969,
12.));
#219568=CARTESIAN_POINT('Ctrl Pts',(19.2786358177198,-13.0840182984949,
0.));
#219569=CARTESIAN_POINT('Ctrl Pts',(19.2786358177198,-13.0840182984949,
12.));
#219570=CARTESIAN_POINT('Ctrl Pts',(19.2626927725596,-13.0783089692118,
0.));
#219571=CARTESIAN_POINT('Ctrl Pts',(19.2626927725596,-13.0783089692118,
12.));
#219572=CARTESIAN_POINT('Ctrl Pts',(19.2468925053989,-13.0725987415859,
0.));
#219573=CARTESIAN_POINT('Ctrl Pts',(19.2468925053989,-13.0725987415859,
12.));
#219574=CARTESIAN_POINT('Ctrl Pts',(19.2312360592033,-13.0668886494795,
0.));
#219575=CARTESIAN_POINT('Ctrl Pts',(19.2312360592033,-13.0668886494795,
12.));
#219576=CARTESIAN_POINT('Ctrl Pts',(19.2157244937142,-13.0611797463915,
0.));
#219577=CARTESIAN_POINT('Ctrl Pts',(19.2157244937142,-13.0611797463915,
12.));
#219578=CARTESIAN_POINT('Ctrl Pts',(19.2003588859772,-13.0554731060538,
0.));
#219579=CARTESIAN_POINT('Ctrl Pts',(19.2003588859772,-13.0554731060538,
12.));
#219580=CARTESIAN_POINT('Ctrl Pts',(19.1851403308825,-13.0497698230441,
0.));
#219581=CARTESIAN_POINT('Ctrl Pts',(19.1851403308825,-13.0497698230441,
12.));
#219582=CARTESIAN_POINT('Ctrl Pts',(19.1700699416622,-13.0440710133772,
0.));
#219583=CARTESIAN_POINT('Ctrl Pts',(19.1700699416622,-13.0440710133772,
12.));
#219584=CARTESIAN_POINT('Ctrl Pts',(19.155148850523,-13.0383778152068,0.));
#219585=CARTESIAN_POINT('Ctrl Pts',(19.155148850523,-13.0383778152068,12.));
#219586=CARTESIAN_POINT('Ctrl Pts',(19.1403782093386,-13.0326913895838,
0.));
#219587=CARTESIAN_POINT('Ctrl Pts',(19.1403782093386,-13.0326913895838,
12.));
#219588=CARTESIAN_POINT('Ctrl Pts',(19.1257591903099,-13.0270129211976,
0.));
#219589=CARTESIAN_POINT('Ctrl Pts',(19.1257591903099,-13.0270129211976,
12.));
#219590=CARTESIAN_POINT('Ctrl Pts',(19.111292986631,-13.0213436191328,0.));
#219591=CARTESIAN_POINT('Ctrl Pts',(19.111292986631,-13.0213436191328,12.));
#219592=CARTESIAN_POINT('Ctrl Pts',(19.0969808131228,-13.0156847176097,
0.));
#219593=CARTESIAN_POINT('Ctrl Pts',(19.0969808131228,-13.0156847176097,
12.));
#219594=CARTESIAN_POINT('Ctrl Pts',(19.0828239070484,-13.0100374768788,
0.));
#219595=CARTESIAN_POINT('Ctrl Pts',(19.0828239070484,-13.0100374768788,
12.));
#219596=CARTESIAN_POINT('Ctrl Pts',(19.0688235289437,-13.0044031841382,
0.));
#219597=CARTESIAN_POINT('Ctrl Pts',(19.0688235289437,-13.0044031841382,
12.));
#219598=CARTESIAN_POINT('Ctrl Pts',(19.0549809634354,-12.9987831544502,
0.));
#219599=CARTESIAN_POINT('Ctrl Pts',(19.0549809634354,-12.9987831544502,
12.));
#219600=CARTESIAN_POINT('Ctrl Pts',(19.0412975200398,-12.9931787316514,
0.));
#219601=CARTESIAN_POINT('Ctrl Pts',(19.0412975200398,-12.9931787316514,
12.));
#219602=CARTESIAN_POINT('Ctrl Pts',(19.0277745339908,-12.9875912893003,
0.));
#219603=CARTESIAN_POINT('Ctrl Pts',(19.0277745339908,-12.9875912893003,
12.));
#219604=CARTESIAN_POINT('Ctrl Pts',(19.014413367335,-12.9820222318716,0.));
#219605=CARTESIAN_POINT('Ctrl Pts',(19.014413367335,-12.9820222318716,12.));
#219606=CARTESIAN_POINT('Ctrl Pts',(19.0012154099792,-12.9764729959206,
0.));
#219607=CARTESIAN_POINT('Ctrl Pts',(19.0012154099792,-12.9764729959206,
12.));
#219608=CARTESIAN_POINT('Ctrl Pts',(18.9881820807585,-12.9709450512747,
0.));
#219609=CARTESIAN_POINT('Ctrl Pts',(18.9881820807585,-12.9709450512747,
12.));
#219610=CARTESIAN_POINT('Ctrl Pts',(18.9753148284473,-12.9654399021868,
0.));
#219611=CARTESIAN_POINT('Ctrl Pts',(18.9753148284473,-12.9654399021868,
12.));
#219612=CARTESIAN_POINT('Ctrl Pts',(18.9626151329226,-12.9599590886318,
0.));
#219613=CARTESIAN_POINT('Ctrl Pts',(18.9626151329226,-12.9599590886318,
12.));
#219614=CARTESIAN_POINT('Ctrl Pts',(18.9500845064714,-12.9545041877377,
0.));
#219615=CARTESIAN_POINT('Ctrl Pts',(18.9500845064714,-12.9545041877377,
12.));
#219616=CARTESIAN_POINT('Ctrl Pts',(18.9377244950435,-12.9490768151821,
0.));
#219617=CARTESIAN_POINT('Ctrl Pts',(18.9377244950435,-12.9490768151821,
12.));
#219618=CARTESIAN_POINT('Ctrl Pts',(18.9255366795196,-12.9436786266106,
0.));
#219619=CARTESIAN_POINT('Ctrl Pts',(18.9255366795196,-12.9436786266106,
12.));
#219620=CARTESIAN_POINT('Ctrl Pts',(18.9135226769466,-12.9383113190375,
0.));
#219621=CARTESIAN_POINT('Ctrl Pts',(18.9135226769466,-12.9383113190375,
12.));
#219622=CARTESIAN_POINT('Ctrl Pts',(18.9016841423402,-12.9329766328184,
0.));
#219623=CARTESIAN_POINT('Ctrl Pts',(18.9016841423402,-12.9329766328184,
12.));
#219624=CARTESIAN_POINT('Ctrl Pts',(18.8900227704888,-12.9276763536372,
0.));
#219625=CARTESIAN_POINT('Ctrl Pts',(18.8900227704888,-12.9276763536372,
12.));
#219626=CARTESIAN_POINT('Ctrl Pts',(18.8785402977528,-12.9224123144982,
0.));
#219627=CARTESIAN_POINT('Ctrl Pts',(18.8785402977528,-12.9224123144982,
12.));
#219628=CARTESIAN_POINT('Ctrl Pts',(18.8672385038328,-12.9171863977047,
0.));
#219629=CARTESIAN_POINT('Ctrl Pts',(18.8672385038328,-12.9171863977047,
12.));
#219630=CARTESIAN_POINT('Ctrl Pts',(18.8561192136201,-12.9120005369066,
0.));
#219631=CARTESIAN_POINT('Ctrl Pts',(18.8561192136201,-12.9120005369066,
12.));
#219632=CARTESIAN_POINT('Ctrl Pts',(18.8451842990986,-12.9068567191856,
0.));
#219633=CARTESIAN_POINT('Ctrl Pts',(18.8451842990986,-12.9068567191856,
12.));
#219634=CARTESIAN_POINT('Ctrl Pts',(18.834435681259,-12.9017569871738,0.));
#219635=CARTESIAN_POINT('Ctrl Pts',(18.834435681259,-12.9017569871738,12.));
#219636=CARTESIAN_POINT('Ctrl Pts',(18.8238753319124,-12.8967034410752,
0.));
#219637=CARTESIAN_POINT('Ctrl Pts',(18.8238753319124,-12.8967034410752,
12.));
#219638=CARTESIAN_POINT('Ctrl Pts',(18.8135052757815,-12.8916982409931,
0.));
#219639=CARTESIAN_POINT('Ctrl Pts',(18.8135052757815,-12.8916982409931,
12.));
#219640=CARTESIAN_POINT('Ctrl Pts',(18.8033275941939,-12.8867436109543,
0.));
#219641=CARTESIAN_POINT('Ctrl Pts',(18.8033275941939,-12.8867436109543,
12.));
#219642=CARTESIAN_POINT('Ctrl Pts',(18.7933444285867,-12.8818418427474,
0.));
#219643=CARTESIAN_POINT('Ctrl Pts',(18.7933444285867,-12.8818418427474,
12.));
#219644=CARTESIAN_POINT('Ctrl Pts',(18.7835579840481,-12.8769952998097,
0.));
#219645=CARTESIAN_POINT('Ctrl Pts',(18.7835579840481,-12.8769952998097,
12.));
#219646=CARTESIAN_POINT('Ctrl Pts',(18.7739705329028,-12.8722064211814,
0.));
#219647=CARTESIAN_POINT('Ctrl Pts',(18.7739705329028,-12.8722064211814,
12.));
#219648=CARTESIAN_POINT('Ctrl Pts',(18.7645844169568,-12.8674777239656,
0.));
#219649=CARTESIAN_POINT('Ctrl Pts',(18.7645844169568,-12.8674777239656,
12.));
#219650=CARTESIAN_POINT('Ctrl Pts',(18.7554020493888,-12.8628118054172,
0.));
#219651=CARTESIAN_POINT('Ctrl Pts',(18.7554020493888,-12.8628118054172,
12.));
#219652=CARTESIAN_POINT('Ctrl Pts',(18.7464259171248,-12.8582113455644,
0.));
#219653=CARTESIAN_POINT('Ctrl Pts',(18.7464259171248,-12.8582113455644,
12.));
#219654=CARTESIAN_POINT('Ctrl Pts',(18.7376585820851,-12.8536791086315,
0.));
#219655=CARTESIAN_POINT('Ctrl Pts',(18.7376585820851,-12.8536791086315,
12.));
#219656=CARTESIAN_POINT('Ctrl Pts',(18.7291026886552,-12.849217951159,0.));
#219657=CARTESIAN_POINT('Ctrl Pts',(18.7291026886552,-12.849217951159,12.));
#219658=CARTESIAN_POINT('Ctrl Pts',(18.7207609737701,-12.8448308329494,
0.));
#219659=CARTESIAN_POINT('Ctrl Pts',(18.7207609737701,-12.8448308329494,
12.));
#219660=CARTESIAN_POINT('Ctrl Pts',(18.7126362754446,-12.8405208263432,
0.));
#219661=CARTESIAN_POINT('Ctrl Pts',(18.7126362754446,-12.8405208263432,
12.));
#219662=CARTESIAN_POINT('Ctrl Pts',(18.7047315436296,-12.8362911280362,
0.));
#219663=CARTESIAN_POINT('Ctrl Pts',(18.7047315436296,-12.8362911280362,
12.));
#219664=CARTESIAN_POINT('Ctrl Pts',(18.6970498410173,-12.832145059979,0.));
#219665=CARTESIAN_POINT('Ctrl Pts',(18.6970498410173,-12.832145059979,12.));
#219666=CARTESIAN_POINT('Ctrl Pts',(18.6895943376172,-12.8280860635231,
0.));
#219667=CARTESIAN_POINT('Ctrl Pts',(18.6895943376172,-12.8280860635231,
12.));
#219668=CARTESIAN_POINT('Ctrl Pts',(18.6823683094139,-12.8241176980016,
0.));
#219669=CARTESIAN_POINT('Ctrl Pts',(18.6823683094139,-12.8241176980016,
12.));
#219670=CARTESIAN_POINT('Ctrl Pts',(18.6753751301091,-12.8202436318473,
0.));
#219671=CARTESIAN_POINT('Ctrl Pts',(18.6753751301091,-12.8202436318473,
12.));
#219672=CARTESIAN_POINT('Ctrl Pts',(18.6686182952798,-12.8164676687361,
0.));
#219673=CARTESIAN_POINT('Ctrl Pts',(18.6686182952798,-12.8164676687361,
12.));
#219674=CARTESIAN_POINT('Ctrl Pts',(18.6621014624746,-12.8127937909632,
0.));
#219675=CARTESIAN_POINT('Ctrl Pts',(18.6621014624746,-12.8127937909632,
12.));
#219676=CARTESIAN_POINT('Ctrl Pts',(18.6558284825772,-12.8092261933858,
0.));
#219677=CARTESIAN_POINT('Ctrl Pts',(18.6558284825772,-12.8092261933858,
12.));
#219678=CARTESIAN_POINT('Ctrl Pts',(18.6498034438986,-12.805769331162,0.));
#219679=CARTESIAN_POINT('Ctrl Pts',(18.6498034438986,-12.805769331162,12.));
#219680=CARTESIAN_POINT('Ctrl Pts',(18.6440306327457,-12.8024278770153,
0.));
#219681=CARTESIAN_POINT('Ctrl Pts',(18.6440306327457,-12.8024278770153,
12.));
#219682=CARTESIAN_POINT('Ctrl Pts',(18.63851447924,-12.7992066625264,0.));
#219683=CARTESIAN_POINT('Ctrl Pts',(18.63851447924,-12.7992066625264,12.));
#219684=CARTESIAN_POINT('Ctrl Pts',(18.6332595057005,-12.7961106222251,
0.));
#219685=CARTESIAN_POINT('Ctrl Pts',(18.6332595057005,-12.7961106222251,
12.));
#219686=CARTESIAN_POINT('Ctrl Pts',(18.6282702819371,-12.7931447451556,
0.));
#219687=CARTESIAN_POINT('Ctrl Pts',(18.6282702819371,-12.7931447451556,
12.));
#219688=CARTESIAN_POINT('Ctrl Pts',(18.6235516265575,-12.7903142925234,
0.));
#219689=CARTESIAN_POINT('Ctrl Pts',(18.6235516265575,-12.7903142925234,
12.));
#219690=CARTESIAN_POINT('Ctrl Pts',(18.6191087624752,-12.7876249657834,
0.));
#219691=CARTESIAN_POINT('Ctrl Pts',(18.6191087624752,-12.7876249657834,
12.));
#219692=CARTESIAN_POINT('Ctrl Pts',(18.6149475565189,-12.78508316579,0.));
#219693=CARTESIAN_POINT('Ctrl Pts',(18.6149475565189,-12.78508316579,12.));
#219694=CARTESIAN_POINT('Ctrl Pts',(18.611074482622,-12.7826959526924,0.));
#219695=CARTESIAN_POINT('Ctrl Pts',(18.611074482622,-12.7826959526924,12.));
#219696=CARTESIAN_POINT('Ctrl Pts',(18.6074961535723,-12.7804705387658,
0.));
#219697=CARTESIAN_POINT('Ctrl Pts',(18.6074961535723,-12.7804705387658,
12.));
#219698=CARTESIAN_POINT('Ctrl Pts',(18.6042190183703,-12.7784139605067,
0.));
#219699=CARTESIAN_POINT('Ctrl Pts',(18.6042190183703,-12.7784139605067,
12.));
#219700=CARTESIAN_POINT('Ctrl Pts',(18.6012488486708,-12.7765325225082,
0.));
#219701=CARTESIAN_POINT('Ctrl Pts',(18.6012488486708,-12.7765325225082,
12.));
#219702=CARTESIAN_POINT('Ctrl Pts',(18.5985917525949,-12.7748328937639,
0.));
#219703=CARTESIAN_POINT('Ctrl Pts',(18.5985917525949,-12.7748328937639,
12.));
#219704=CARTESIAN_POINT('Ctrl Pts',(18.5962551167772,-12.7733231262107,
0.));
#219705=CARTESIAN_POINT('Ctrl Pts',(18.5962551167772,-12.7733231262107,
12.));
#219706=CARTESIAN_POINT('Ctrl Pts',(18.5942490615409,-12.7720142287169,
0.));
#219707=CARTESIAN_POINT('Ctrl Pts',(18.5942490615409,-12.7720142287169,
12.));
#219708=CARTESIAN_POINT('Ctrl Pts',(18.5925859134582,-12.7709195951153,
0.));
#219709=CARTESIAN_POINT('Ctrl Pts',(18.5925859134582,-12.7709195951153,
12.));
#219710=CARTESIAN_POINT('Ctrl Pts',(18.5912775137806,-12.7700520897174,
0.));
#219711=CARTESIAN_POINT('Ctrl Pts',(18.5912775137806,-12.7700520897174,
12.));
#219712=CARTESIAN_POINT('Ctrl Pts',(18.590332877722,-12.7694215127923,0.));
#219713=CARTESIAN_POINT('Ctrl Pts',(18.590332877722,-12.7694215127923,12.));
#219714=CARTESIAN_POINT('Ctrl Pts',(18.589871621842,-12.7691103481996,0.));
#219715=CARTESIAN_POINT('Ctrl Pts',(18.589871621842,-12.7691103481996,12.));
#219716=CARTESIAN_POINT('Ctrl Pts',(18.5896919669158,-12.7689864266924,
0.));
#219717=CARTESIAN_POINT('Ctrl Pts',(18.5896919669158,-12.7689864266924,
12.));
#219718=CARTESIAN_POINT('Ctrl Pts',(18.5896460962961,-12.7689524524484,
0.));
#219719=CARTESIAN_POINT('Ctrl Pts',(18.5896460962961,-12.7689524524484,
12.));
#219720=CARTESIAN_POINT('Ctrl Pts',(18.5896416359912,-12.7689476255363,
0.));
#219721=CARTESIAN_POINT('Ctrl Pts',(18.5896416359912,-12.7689476255363,
12.));
#219722=CARTESIAN_POINT('',(22.1787195904339,-13.5685075571671,0.));
#219723=CARTESIAN_POINT('Ctrl Pts',(22.1787195904339,-13.5685075571671,
0.));
#219724=CARTESIAN_POINT('Ctrl Pts',(22.1730081264583,-13.5683460612913,
0.));
#219725=CARTESIAN_POINT('Ctrl Pts',(22.1615922804939,-13.5680170531724,
0.));
#219726=CARTESIAN_POINT('Ctrl Pts',(22.1444897575076,-13.5675054918922,
0.));
#219727=CARTESIAN_POINT('Ctrl Pts',(22.1217288871823,-13.5667873105179,
0.));
#219728=CARTESIAN_POINT('Ctrl Pts',(22.0933486464442,-13.5658294169106,
0.));
#219729=CARTESIAN_POINT('Ctrl Pts',(22.0650393089492,-13.5648113688895,
0.));
#219730=CARTESIAN_POINT('Ctrl Pts',(22.0368009736227,-13.5637332022393,
0.));
#219731=CARTESIAN_POINT('Ctrl Pts',(22.0086337943431,-13.5625949868313,
0.));
#219732=CARTESIAN_POINT('Ctrl Pts',(21.9805379899192,-13.5613968357589,
0.));
#219733=CARTESIAN_POINT('Ctrl Pts',(21.9525138592862,-13.5601389185315,
0.));
#219734=CARTESIAN_POINT('Ctrl Pts',(21.9245617765827,-13.5588214586672,
0.));
#219735=CARTESIAN_POINT('Ctrl Pts',(21.8966821688876,-13.5574447178485,
0.));
#219736=CARTESIAN_POINT('Ctrl Pts',(21.8688754989401,-13.5560089839426,
0.));
#219737=CARTESIAN_POINT('Ctrl Pts',(21.841142245609,-13.5545145573048,0.));
#219738=CARTESIAN_POINT('Ctrl Pts',(21.8134828857963,-13.5529617381569,
0.));
#219739=CARTESIAN_POINT('Ctrl Pts',(21.7858978745848,-13.5513508127232,
0.));
#219740=CARTESIAN_POINT('Ctrl Pts',(21.7583876294532,-13.5496820422186,
0.));
#219741=CARTESIAN_POINT('Ctrl Pts',(21.730952541226,-13.5479556704457,0.));
#219742=CARTESIAN_POINT('Ctrl Pts',(21.7035929822939,-13.546171929503,0.));
#219743=CARTESIAN_POINT('Ctrl Pts',(21.676309315769,-13.5443310461516,0.));
#219744=CARTESIAN_POINT('Ctrl Pts',(21.6491019044647,-13.5424332480698,
0.));
#219745=CARTESIAN_POINT('Ctrl Pts',(21.6219711193951,-13.5404787697798,
0.));
#219746=CARTESIAN_POINT('Ctrl Pts',(21.5949173499022,-13.5384678597206,
0.));
#219747=CARTESIAN_POINT('Ctrl Pts',(21.5679410019011,-13.5364007790292,
0.));
#219748=CARTESIAN_POINT('Ctrl Pts',(21.5410424932511,-13.5342777983225,
0.));
#219749=CARTESIAN_POINT('Ctrl Pts',(21.5142222501671,-13.5320991952145,
0.));
#219750=CARTESIAN_POINT('Ctrl Pts',(21.487480703047,-13.5298652514357,0.));
#219751=CARTESIAN_POINT('Ctrl Pts',(21.4608182828695,-13.5275762503553,
0.));
#219752=CARTESIAN_POINT('Ctrl Pts',(21.4342354165254,-13.5252324737795,
0.));
#219753=CARTESIAN_POINT('Ctrl Pts',(21.4077325259318,-13.5228342013508,
0.));
#219754=CARTESIAN_POINT('Ctrl Pts',(21.3813100304967,-13.5203817122497,
0.));
#219755=CARTESIAN_POINT('Ctrl Pts',(21.3549683486219,-13.5178752862461,
0.));
#219756=CARTESIAN_POINT('Ctrl Pts',(21.328707899634,-13.5153152050554,0.));
#219757=CARTESIAN_POINT('Ctrl Pts',(21.3025291054236,-13.5127017534972,
0.));
#219758=CARTESIAN_POINT('Ctrl Pts',(21.2764323924442,-13.5100352209207,
0.));
#219759=CARTESIAN_POINT('Ctrl Pts',(21.2504181927429,-13.5073159019454,
0.));
#219760=CARTESIAN_POINT('Ctrl Pts',(21.224486942933,-13.5045440957404,0.));
#219761=CARTESIAN_POINT('Ctrl Pts',(21.1986390835825,-13.5017201056088,
0.));
#219762=CARTESIAN_POINT('Ctrl Pts',(21.1728750584173,-13.4988442384491,
0.));
#219763=CARTESIAN_POINT('Ctrl Pts',(21.1471953136209,-13.4959168042934,
0.));
#219764=CARTESIAN_POINT('Ctrl Pts',(21.1216002970209,-13.4929381157778,
0.));
#219765=CARTESIAN_POINT('Ctrl Pts',(21.0960904575048,-13.4899084877718,
0.));
#219766=CARTESIAN_POINT('Ctrl Pts',(21.0706662455202,-13.4868282377192,
0.));
#219767=CARTESIAN_POINT('Ctrl Pts',(21.0453281134247,-13.4836976858912,
0.));
#219768=CARTESIAN_POINT('Ctrl Pts',(21.0200765158885,-13.4805171556822,
0.));
#219769=CARTESIAN_POINT('Ctrl Pts',(20.9949119102592,-13.4772869738879,
0.));
#219770=CARTESIAN_POINT('Ctrl Pts',(20.9698347569476,-13.4740074710087,
0.));
#219771=CARTESIAN_POINT('Ctrl Pts',(20.9448455197557,-13.4706789815166,
0.));
#219772=CARTESIAN_POINT('Ctrl Pts',(20.9199446657584,-13.4673018437718,
0.));
#219773=CARTESIAN_POINT('Ctrl Pts',(20.8951326652158,-13.4638763999725,
0.));
#219774=CARTESIAN_POINT('Ctrl Pts',(20.8704099914641,-13.4604029960983,
0.));
#219775=CARTESIAN_POINT('Ctrl Pts',(20.8457771208082,-13.4568819818631,
0.));
#219776=CARTESIAN_POINT('Ctrl Pts',(20.821234532398,-13.4533137106667,0.));
#219777=CARTESIAN_POINT('Ctrl Pts',(20.7967827081227,-13.4496985395637,
0.));
#219778=CARTESIAN_POINT('Ctrl Pts',(20.7724221327608,-13.4460368293688,
0.));
#219779=CARTESIAN_POINT('Ctrl Pts',(20.7481532941013,-13.4423289447561,
0.));
#219780=CARTESIAN_POINT('Ctrl Pts',(20.7239766830675,-13.4385752543663,
0.));
#219781=CARTESIAN_POINT('Ctrl Pts',(20.6998927938288,-13.4347761309154,
0.));
#219782=CARTESIAN_POINT('Ctrl Pts',(20.6759021239103,-13.4309319513119,
0.));
#219783=CARTESIAN_POINT('Ctrl Pts',(20.6520051742869,-13.4270430967651,
0.));
#219784=CARTESIAN_POINT('Ctrl Pts',(20.6282024494237,-13.4231099528179,
0.));
#219785=CARTESIAN_POINT('Ctrl Pts',(20.6044944573153,-13.4191329093933,
0.));
#219786=CARTESIAN_POINT('Ctrl Pts',(20.5808817095155,-13.4151123608411,
0.));
#219787=CARTESIAN_POINT('Ctrl Pts',(20.5573647211639,-13.4110487059912,
0.));
#219788=CARTESIAN_POINT('Ctrl Pts',(20.5339440109956,-13.4069423482076,
0.));
#219789=CARTESIAN_POINT('Ctrl Pts',(20.5106201013753,-13.4027936954529,
0.));
#219790=CARTESIAN_POINT('Ctrl Pts',(20.487393518404,-13.3986031603716,0.));
#219791=CARTESIAN_POINT('Ctrl Pts',(20.4642647920038,-13.3943711603739,
0.));
#219792=CARTESIAN_POINT('Ctrl Pts',(20.4412344560008,-13.3900981177255,
0.));
#219793=CARTESIAN_POINT('Ctrl Pts',(20.4183030482002,-13.3857844596387,
0.));
#219794=CARTESIAN_POINT('Ctrl Pts',(20.3954711104502,-13.3814306183719,
0.));
#219795=CARTESIAN_POINT('Ctrl Pts',(20.3727391887184,-13.3770370313188,
0.));
#219796=CARTESIAN_POINT('Ctrl Pts',(20.3501078331814,-13.3726041410867,
0.));
#219797=CARTESIAN_POINT('Ctrl Pts',(20.3275775983029,-13.3681323955826,
0.));
#219798=CARTESIAN_POINT('Ctrl Pts',(20.3051490429048,-13.3636222481016,
0.));
#219799=CARTESIAN_POINT('Ctrl Pts',(20.2828227302339,-13.3590741574195,
0.));
#219800=CARTESIAN_POINT('Ctrl Pts',(20.2605992280122,-13.3544885878889,
0.));
#219801=CARTESIAN_POINT('Ctrl Pts',(20.2384791085359,-13.3498660095386,
0.));
#219802=CARTESIAN_POINT('Ctrl Pts',(20.216462948786,-13.3452068981766,0.));
#219803=CARTESIAN_POINT('Ctrl Pts',(20.1945513305235,-13.3405117354971,
0.));
#219804=CARTESIAN_POINT('Ctrl Pts',(20.1727448403817,-13.3357810091903,
0.));
#219805=CARTESIAN_POINT('Ctrl Pts',(20.1510440699474,-13.3310152130564,
0.));
#219806=CARTESIAN_POINT('Ctrl Pts',(20.1294496158402,-13.3262148471226,
0.));
#219807=CARTESIAN_POINT('Ctrl Pts',(20.1079620798375,-13.3213804177587,
0.));
#219808=CARTESIAN_POINT('Ctrl Pts',(20.0865820689882,-13.3165124377963,
0.));
#219809=CARTESIAN_POINT('Ctrl Pts',(20.0653101957188,-13.3116114266515,
0.));
#219810=CARTESIAN_POINT('Ctrl Pts',(20.0441470779345,-13.3066779104515,
0.));
#219811=CARTESIAN_POINT('Ctrl Pts',(20.0230933391038,-13.3017124221637,
0.));
#219812=CARTESIAN_POINT('Ctrl Pts',(20.0021496083738,-13.2967155017306,
0.));
#219813=CARTESIAN_POINT('Ctrl Pts',(19.981316520717,-13.2916876962094,0.));
#219814=CARTESIAN_POINT('Ctrl Pts',(19.9605947170586,-13.286629559915,0.));
#219815=CARTESIAN_POINT('Ctrl Pts',(19.9399848444019,-13.2815416545663,
0.));
#219816=CARTESIAN_POINT('Ctrl Pts',(19.9194875559422,-13.2764245494357,
0.));
#219817=CARTESIAN_POINT('Ctrl Pts',(19.8991035111745,-13.271278821502,0.));
#219818=CARTESIAN_POINT('Ctrl Pts',(19.8788333760577,-13.2661050556132,
0.));
#219819=CARTESIAN_POINT('Ctrl Pts',(19.8586778231715,-13.2609038446529,
0.));
#219820=CARTESIAN_POINT('Ctrl Pts',(19.8386375318634,-13.2556757897086,
0.));
#219821=CARTESIAN_POINT('Ctrl Pts',(19.8187131883917,-13.2504215002457,
0.));
#219822=CARTESIAN_POINT('Ctrl Pts',(19.7989054860495,-13.2451415942805,
0.));
#219823=CARTESIAN_POINT('Ctrl Pts',(19.7792151253289,-13.2398366985675,
0.));
#219824=CARTESIAN_POINT('Ctrl Pts',(19.7596428141168,-13.2345074487963,
0.));
#219825=CARTESIAN_POINT('Ctrl Pts',(19.7401892678697,-13.2291544897899,
0.));
#219826=CARTESIAN_POINT('Ctrl Pts',(19.7208552097868,-13.2237784757065,
0.));
#219827=CARTESIAN_POINT('Ctrl Pts',(19.7016413709685,-13.2183800702436,
0.));
#219828=CARTESIAN_POINT('Ctrl Pts',(19.6825484905823,-13.2129599468485,
0.));
#219829=CARTESIAN_POINT('Ctrl Pts',(19.6635773160936,-13.2075187889529,
0.));
#219830=CARTESIAN_POINT('Ctrl Pts',(19.6447286034772,-13.2020572902065,
0.));
#219831=CARTESIAN_POINT('Ctrl Pts',(19.6260031174244,-13.1965761547151,
0.));
#219832=CARTESIAN_POINT('Ctrl Pts',(19.6074016315414,-13.1910760972814,
0.));
#219833=CARTESIAN_POINT('Ctrl Pts',(19.5889249285338,-13.1855578436471,
0.));
#219834=CARTESIAN_POINT('Ctrl Pts',(19.5705738004667,-13.1800221307673,
0.));
#219835=CARTESIAN_POINT('Ctrl Pts',(19.5523490490244,-13.1744697070911,
0.));
#219836=CARTESIAN_POINT('Ctrl Pts',(19.5342514857562,-13.168901332843,0.));
#219837=CARTESIAN_POINT('Ctrl Pts',(19.5162819323213,-13.1633177803101,
0.));
#219838=CARTESIAN_POINT('Ctrl Pts',(19.4984412207082,-13.1577198341245,
0.));
#219839=CARTESIAN_POINT('Ctrl Pts',(19.4807301935268,-13.1521082915853,
0.));
#219840=CARTESIAN_POINT('Ctrl Pts',(19.4631497043258,-13.1464839629971,
0.));
#219841=CARTESIAN_POINT('Ctrl Pts',(19.4457006178876,-13.1408476720061,
0.));
#219842=CARTESIAN_POINT('Ctrl Pts',(19.4283838105262,-13.1352002559438,
0.));
#219843=CARTESIAN_POINT('Ctrl Pts',(19.4112001703557,-13.1295425661634,
0.));
#219844=CARTESIAN_POINT('Ctrl Pts',(19.3941505976263,-13.1238754684177,
0.));
#219845=CARTESIAN_POINT('Ctrl Pts',(19.3772360051091,-13.118199843271,0.));
#219846=CARTESIAN_POINT('Ctrl Pts',(19.3604573184515,-13.1125165865022,
0.));
#219847=CARTESIAN_POINT('Ctrl Pts',(19.3438154765395,-13.1068266095186,
0.));
#219848=CARTESIAN_POINT('Ctrl Pts',(19.3273114318269,-13.1011308397591,
0.));
#219849=CARTESIAN_POINT('Ctrl Pts',(19.310946150736,-13.0954302211479,0.));
#219850=CARTESIAN_POINT('Ctrl Pts',(19.2947206141247,-13.0897257145969,
0.));
#219851=CARTESIAN_POINT('Ctrl Pts',(19.2786358177198,-13.0840182984949,
0.));
#219852=CARTESIAN_POINT('Ctrl Pts',(19.2626927725596,-13.0783089692118,
0.));
#219853=CARTESIAN_POINT('Ctrl Pts',(19.2468925053989,-13.0725987415859,
0.));
#219854=CARTESIAN_POINT('Ctrl Pts',(19.2312360592033,-13.0668886494795,
0.));
#219855=CARTESIAN_POINT('Ctrl Pts',(19.2157244937142,-13.0611797463915,
0.));
#219856=CARTESIAN_POINT('Ctrl Pts',(19.2003588859772,-13.0554731060538,
0.));
#219857=CARTESIAN_POINT('Ctrl Pts',(19.1851403308825,-13.0497698230441,
0.));
#219858=CARTESIAN_POINT('Ctrl Pts',(19.1700699416622,-13.0440710133772,
0.));
#219859=CARTESIAN_POINT('Ctrl Pts',(19.155148850523,-13.0383778152068,0.));
#219860=CARTESIAN_POINT('Ctrl Pts',(19.1403782093386,-13.0326913895838,
0.));
#219861=CARTESIAN_POINT('Ctrl Pts',(19.1257591903099,-13.0270129211976,
0.));
#219862=CARTESIAN_POINT('Ctrl Pts',(19.111292986631,-13.0213436191328,0.));
#219863=CARTESIAN_POINT('Ctrl Pts',(19.0969808131228,-13.0156847176097,
0.));
#219864=CARTESIAN_POINT('Ctrl Pts',(19.0828239070484,-13.0100374768788,
0.));
#219865=CARTESIAN_POINT('Ctrl Pts',(19.0688235289437,-13.0044031841382,
0.));
#219866=CARTESIAN_POINT('Ctrl Pts',(19.0549809634354,-12.9987831544502,
0.));
#219867=CARTESIAN_POINT('Ctrl Pts',(19.0412975200398,-12.9931787316514,
0.));
#219868=CARTESIAN_POINT('Ctrl Pts',(19.0277745339908,-12.9875912893003,
0.));
#219869=CARTESIAN_POINT('Ctrl Pts',(19.014413367335,-12.9820222318716,0.));
#219870=CARTESIAN_POINT('Ctrl Pts',(19.0012154099792,-12.9764729959206,
0.));
#219871=CARTESIAN_POINT('Ctrl Pts',(18.9881820807585,-12.9709450512747,
0.));
#219872=CARTESIAN_POINT('Ctrl Pts',(18.9753148284473,-12.9654399021868,
0.));
#219873=CARTESIAN_POINT('Ctrl Pts',(18.9626151329226,-12.9599590886318,
0.));
#219874=CARTESIAN_POINT('Ctrl Pts',(18.9500845064714,-12.9545041877377,
0.));
#219875=CARTESIAN_POINT('Ctrl Pts',(18.9377244950435,-12.9490768151821,
0.));
#219876=CARTESIAN_POINT('Ctrl Pts',(18.9255366795196,-12.9436786266106,
0.));
#219877=CARTESIAN_POINT('Ctrl Pts',(18.9135226769466,-12.9383113190375,
0.));
#219878=CARTESIAN_POINT('Ctrl Pts',(18.9016841423402,-12.9329766328184,
0.));
#219879=CARTESIAN_POINT('Ctrl Pts',(18.8900227704888,-12.9276763536372,
0.));
#219880=CARTESIAN_POINT('Ctrl Pts',(18.8785402977528,-12.9224123144982,
0.));
#219881=CARTESIAN_POINT('Ctrl Pts',(18.8672385038328,-12.9171863977047,
0.));
#219882=CARTESIAN_POINT('Ctrl Pts',(18.8561192136201,-12.9120005369066,
0.));
#219883=CARTESIAN_POINT('Ctrl Pts',(18.8451842990986,-12.9068567191856,
0.));
#219884=CARTESIAN_POINT('Ctrl Pts',(18.834435681259,-12.9017569871738,0.));
#219885=CARTESIAN_POINT('Ctrl Pts',(18.8238753319124,-12.8967034410752,
0.));
#219886=CARTESIAN_POINT('Ctrl Pts',(18.8135052757815,-12.8916982409931,
0.));
#219887=CARTESIAN_POINT('Ctrl Pts',(18.8033275941939,-12.8867436109543,
0.));
#219888=CARTESIAN_POINT('Ctrl Pts',(18.7933444285867,-12.8818418427474,
0.));
#219889=CARTESIAN_POINT('Ctrl Pts',(18.7835579840481,-12.8769952998097,
0.));
#219890=CARTESIAN_POINT('Ctrl Pts',(18.7739705329028,-12.8722064211814,
0.));
#219891=CARTESIAN_POINT('Ctrl Pts',(18.7645844169568,-12.8674777239656,
0.));
#219892=CARTESIAN_POINT('Ctrl Pts',(18.7554020493888,-12.8628118054172,
0.));
#219893=CARTESIAN_POINT('Ctrl Pts',(18.7464259171248,-12.8582113455644,
0.));
#219894=CARTESIAN_POINT('Ctrl Pts',(18.7376585820851,-12.8536791086315,
0.));
#219895=CARTESIAN_POINT('Ctrl Pts',(18.7291026886552,-12.849217951159,0.));
#219896=CARTESIAN_POINT('Ctrl Pts',(18.7207609737701,-12.8448308329494,
0.));
#219897=CARTESIAN_POINT('Ctrl Pts',(18.7126362754446,-12.8405208263432,
0.));
#219898=CARTESIAN_POINT('Ctrl Pts',(18.7047315436296,-12.8362911280362,
0.));
#219899=CARTESIAN_POINT('Ctrl Pts',(18.6970498410173,-12.832145059979,0.));
#219900=CARTESIAN_POINT('Ctrl Pts',(18.6895943376172,-12.8280860635231,
0.));
#219901=CARTESIAN_POINT('Ctrl Pts',(18.6823683094139,-12.8241176980016,
0.));
#219902=CARTESIAN_POINT('Ctrl Pts',(18.6753751301091,-12.8202436318473,
0.));
#219903=CARTESIAN_POINT('Ctrl Pts',(18.6686182952798,-12.8164676687361,
0.));
#219904=CARTESIAN_POINT('Ctrl Pts',(18.6621014624746,-12.8127937909632,
0.));
#219905=CARTESIAN_POINT('Ctrl Pts',(18.6558284825772,-12.8092261933858,
0.));
#219906=CARTESIAN_POINT('Ctrl Pts',(18.6498034438986,-12.805769331162,0.));
#219907=CARTESIAN_POINT('Ctrl Pts',(18.6440306327457,-12.8024278770153,
0.));
#219908=CARTESIAN_POINT('Ctrl Pts',(18.63851447924,-12.7992066625264,0.));
#219909=CARTESIAN_POINT('Ctrl Pts',(18.6332595057005,-12.7961106222251,
0.));
#219910=CARTESIAN_POINT('Ctrl Pts',(18.6282702819371,-12.7931447451556,
0.));
#219911=CARTESIAN_POINT('Ctrl Pts',(18.6235516265575,-12.7903142925234,
0.));
#219912=CARTESIAN_POINT('Ctrl Pts',(18.6191087624752,-12.7876249657834,
0.));
#219913=CARTESIAN_POINT('Ctrl Pts',(18.6149475565189,-12.78508316579,0.));
#219914=CARTESIAN_POINT('Ctrl Pts',(18.611074482622,-12.7826959526924,0.));
#219915=CARTESIAN_POINT('Ctrl Pts',(18.6074961535723,-12.7804705387658,
0.));
#219916=CARTESIAN_POINT('Ctrl Pts',(18.6042190183703,-12.7784139605067,
0.));
#219917=CARTESIAN_POINT('Ctrl Pts',(18.6012488486708,-12.7765325225082,
0.));
#219918=CARTESIAN_POINT('Ctrl Pts',(18.5985917525949,-12.7748328937639,
0.));
#219919=CARTESIAN_POINT('Ctrl Pts',(18.5962551167772,-12.7733231262107,
0.));
#219920=CARTESIAN_POINT('Ctrl Pts',(18.5942490615409,-12.7720142287169,
0.));
#219921=CARTESIAN_POINT('Ctrl Pts',(18.5925859134582,-12.7709195951153,
0.));
#219922=CARTESIAN_POINT('Ctrl Pts',(18.5912775137806,-12.7700520897174,
0.));
#219923=CARTESIAN_POINT('Ctrl Pts',(18.590332877722,-12.7694215127923,0.));
#219924=CARTESIAN_POINT('Ctrl Pts',(18.589871621842,-12.7691103481996,0.));
#219925=CARTESIAN_POINT('Ctrl Pts',(18.5896919669158,-12.7689864266924,
0.));
#219926=CARTESIAN_POINT('Ctrl Pts',(18.5896460962961,-12.7689524524484,
0.));
#219927=CARTESIAN_POINT('Ctrl Pts',(18.5896416359912,-12.7689476255363,
0.));
#219928=CARTESIAN_POINT('',(22.1787195904339,-13.5685075571671,12.));
#219929=CARTESIAN_POINT('',(22.1787195904339,-13.5685075571671,0.));
#219930=CARTESIAN_POINT('Ctrl Pts',(18.5896416359912,-12.7689476255363,
12.));
#219931=CARTESIAN_POINT('Ctrl Pts',(18.5896460962961,-12.7689524524484,
12.));
#219932=CARTESIAN_POINT('Ctrl Pts',(18.5896919669158,-12.7689864266924,
12.));
#219933=CARTESIAN_POINT('Ctrl Pts',(18.589871621842,-12.7691103481996,12.));
#219934=CARTESIAN_POINT('Ctrl Pts',(18.590332877722,-12.7694215127923,12.));
#219935=CARTESIAN_POINT('Ctrl Pts',(18.5912775137806,-12.7700520897174,
12.));
#219936=CARTESIAN_POINT('Ctrl Pts',(18.5925859134582,-12.7709195951153,
12.));
#219937=CARTESIAN_POINT('Ctrl Pts',(18.5942490615409,-12.7720142287169,
12.));
#219938=CARTESIAN_POINT('Ctrl Pts',(18.5962551167772,-12.7733231262107,
12.));
#219939=CARTESIAN_POINT('Ctrl Pts',(18.5985917525949,-12.7748328937639,
12.));
#219940=CARTESIAN_POINT('Ctrl Pts',(18.6012488486708,-12.7765325225082,
12.));
#219941=CARTESIAN_POINT('Ctrl Pts',(18.6042190183703,-12.7784139605067,
12.));
#219942=CARTESIAN_POINT('Ctrl Pts',(18.6074961535723,-12.7804705387658,
12.));
#219943=CARTESIAN_POINT('Ctrl Pts',(18.611074482622,-12.7826959526924,12.));
#219944=CARTESIAN_POINT('Ctrl Pts',(18.6149475565189,-12.78508316579,12.));
#219945=CARTESIAN_POINT('Ctrl Pts',(18.6191087624752,-12.7876249657834,
12.));
#219946=CARTESIAN_POINT('Ctrl Pts',(18.6235516265575,-12.7903142925234,
12.));
#219947=CARTESIAN_POINT('Ctrl Pts',(18.6282702819371,-12.7931447451556,
12.));
#219948=CARTESIAN_POINT('Ctrl Pts',(18.6332595057005,-12.7961106222251,
12.));
#219949=CARTESIAN_POINT('Ctrl Pts',(18.63851447924,-12.7992066625264,12.));
#219950=CARTESIAN_POINT('Ctrl Pts',(18.6440306327457,-12.8024278770153,
12.));
#219951=CARTESIAN_POINT('Ctrl Pts',(18.6498034438986,-12.805769331162,12.));
#219952=CARTESIAN_POINT('Ctrl Pts',(18.6558284825772,-12.8092261933858,
12.));
#219953=CARTESIAN_POINT('Ctrl Pts',(18.6621014624746,-12.8127937909632,
12.));
#219954=CARTESIAN_POINT('Ctrl Pts',(18.6686182952798,-12.8164676687361,
12.));
#219955=CARTESIAN_POINT('Ctrl Pts',(18.6753751301091,-12.8202436318473,
12.));
#219956=CARTESIAN_POINT('Ctrl Pts',(18.6823683094139,-12.8241176980016,
12.));
#219957=CARTESIAN_POINT('Ctrl Pts',(18.6895943376172,-12.8280860635231,
12.));
#219958=CARTESIAN_POINT('Ctrl Pts',(18.6970498410173,-12.832145059979,12.));
#219959=CARTESIAN_POINT('Ctrl Pts',(18.7047315436296,-12.8362911280362,
12.));
#219960=CARTESIAN_POINT('Ctrl Pts',(18.7126362754446,-12.8405208263432,
12.));
#219961=CARTESIAN_POINT('Ctrl Pts',(18.7207609737701,-12.8448308329494,
12.));
#219962=CARTESIAN_POINT('Ctrl Pts',(18.7291026886552,-12.849217951159,12.));
#219963=CARTESIAN_POINT('Ctrl Pts',(18.7376585820851,-12.8536791086315,
12.));
#219964=CARTESIAN_POINT('Ctrl Pts',(18.7464259171248,-12.8582113455644,
12.));
#219965=CARTESIAN_POINT('Ctrl Pts',(18.7554020493888,-12.8628118054172,
12.));
#219966=CARTESIAN_POINT('Ctrl Pts',(18.7645844169568,-12.8674777239656,
12.));
#219967=CARTESIAN_POINT('Ctrl Pts',(18.7739705329028,-12.8722064211814,
12.));
#219968=CARTESIAN_POINT('Ctrl Pts',(18.7835579840481,-12.8769952998097,
12.));
#219969=CARTESIAN_POINT('Ctrl Pts',(18.7933444285867,-12.8818418427474,
12.));
#219970=CARTESIAN_POINT('Ctrl Pts',(18.8033275941939,-12.8867436109543,
12.));
#219971=CARTESIAN_POINT('Ctrl Pts',(18.8135052757815,-12.8916982409931,
12.));
#219972=CARTESIAN_POINT('Ctrl Pts',(18.8238753319124,-12.8967034410752,
12.));
#219973=CARTESIAN_POINT('Ctrl Pts',(18.834435681259,-12.9017569871738,12.));
#219974=CARTESIAN_POINT('Ctrl Pts',(18.8451842990986,-12.9068567191856,
12.));
#219975=CARTESIAN_POINT('Ctrl Pts',(18.8561192136201,-12.9120005369066,
12.));
#219976=CARTESIAN_POINT('Ctrl Pts',(18.8672385038328,-12.9171863977047,
12.));
#219977=CARTESIAN_POINT('Ctrl Pts',(18.8785402977528,-12.9224123144982,
12.));
#219978=CARTESIAN_POINT('Ctrl Pts',(18.8900227704888,-12.9276763536372,
12.));
#219979=CARTESIAN_POINT('Ctrl Pts',(18.9016841423402,-12.9329766328184,
12.));
#219980=CARTESIAN_POINT('Ctrl Pts',(18.9135226769466,-12.9383113190375,
12.));
#219981=CARTESIAN_POINT('Ctrl Pts',(18.9255366795196,-12.9436786266106,
12.));
#219982=CARTESIAN_POINT('Ctrl Pts',(18.9377244950435,-12.9490768151821,
12.));
#219983=CARTESIAN_POINT('Ctrl Pts',(18.9500845064714,-12.9545041877377,
12.));
#219984=CARTESIAN_POINT('Ctrl Pts',(18.9626151329226,-12.9599590886318,
12.));
#219985=CARTESIAN_POINT('Ctrl Pts',(18.9753148284473,-12.9654399021868,
12.));
#219986=CARTESIAN_POINT('Ctrl Pts',(18.9881820807585,-12.9709450512747,
12.));
#219987=CARTESIAN_POINT('Ctrl Pts',(19.0012154099792,-12.9764729959206,
12.));
#219988=CARTESIAN_POINT('Ctrl Pts',(19.014413367335,-12.9820222318716,12.));
#219989=CARTESIAN_POINT('Ctrl Pts',(19.0277745339908,-12.9875912893003,
12.));
#219990=CARTESIAN_POINT('Ctrl Pts',(19.0412975200398,-12.9931787316514,
12.));
#219991=CARTESIAN_POINT('Ctrl Pts',(19.0549809634354,-12.9987831544502,
12.));
#219992=CARTESIAN_POINT('Ctrl Pts',(19.0688235289437,-13.0044031841382,
12.));
#219993=CARTESIAN_POINT('Ctrl Pts',(19.0828239070484,-13.0100374768788,
12.));
#219994=CARTESIAN_POINT('Ctrl Pts',(19.0969808131228,-13.0156847176097,
12.));
#219995=CARTESIAN_POINT('Ctrl Pts',(19.111292986631,-13.0213436191328,12.));
#219996=CARTESIAN_POINT('Ctrl Pts',(19.1257591903099,-13.0270129211976,
12.));
#219997=CARTESIAN_POINT('Ctrl Pts',(19.1403782093386,-13.0326913895838,
12.));
#219998=CARTESIAN_POINT('Ctrl Pts',(19.155148850523,-13.0383778152068,12.));
#219999=CARTESIAN_POINT('Ctrl Pts',(19.1700699416622,-13.0440710133772,
12.));
#220000=CARTESIAN_POINT('Ctrl Pts',(19.1851403308825,-13.0497698230441,
12.));
#220001=CARTESIAN_POINT('Ctrl Pts',(19.2003588859772,-13.0554731060538,
12.));
#220002=CARTESIAN_POINT('Ctrl Pts',(19.2157244937142,-13.0611797463915,
12.));
#220003=CARTESIAN_POINT('Ctrl Pts',(19.2312360592033,-13.0668886494795,
12.));
#220004=CARTESIAN_POINT('Ctrl Pts',(19.2468925053989,-13.0725987415859,
12.));
#220005=CARTESIAN_POINT('Ctrl Pts',(19.2626927725596,-13.0783089692118,
12.));
#220006=CARTESIAN_POINT('Ctrl Pts',(19.2786358177198,-13.0840182984949,
12.));
#220007=CARTESIAN_POINT('Ctrl Pts',(19.2947206141247,-13.0897257145969,
12.));
#220008=CARTESIAN_POINT('Ctrl Pts',(19.310946150736,-13.0954302211479,12.));
#220009=CARTESIAN_POINT('Ctrl Pts',(19.3273114318269,-13.1011308397591,
12.));
#220010=CARTESIAN_POINT('Ctrl Pts',(19.3438154765395,-13.1068266095186,
12.));
#220011=CARTESIAN_POINT('Ctrl Pts',(19.3604573184515,-13.1125165865022,
12.));
#220012=CARTESIAN_POINT('Ctrl Pts',(19.3772360051091,-13.118199843271,12.));
#220013=CARTESIAN_POINT('Ctrl Pts',(19.3941505976263,-13.1238754684177,
12.));
#220014=CARTESIAN_POINT('Ctrl Pts',(19.4112001703557,-13.1295425661634,
12.));
#220015=CARTESIAN_POINT('Ctrl Pts',(19.4283838105262,-13.1352002559438,
12.));
#220016=CARTESIAN_POINT('Ctrl Pts',(19.4457006178876,-13.1408476720061,
12.));
#220017=CARTESIAN_POINT('Ctrl Pts',(19.4631497043258,-13.1464839629971,
12.));
#220018=CARTESIAN_POINT('Ctrl Pts',(19.4807301935268,-13.1521082915853,
12.));
#220019=CARTESIAN_POINT('Ctrl Pts',(19.4984412207082,-13.1577198341245,
12.));
#220020=CARTESIAN_POINT('Ctrl Pts',(19.5162819323213,-13.1633177803101,
12.));
#220021=CARTESIAN_POINT('Ctrl Pts',(19.5342514857562,-13.168901332843,12.));
#220022=CARTESIAN_POINT('Ctrl Pts',(19.5523490490244,-13.1744697070911,
12.));
#220023=CARTESIAN_POINT('Ctrl Pts',(19.5705738004667,-13.1800221307673,
12.));
#220024=CARTESIAN_POINT('Ctrl Pts',(19.5889249285338,-13.1855578436471,
12.));
#220025=CARTESIAN_POINT('Ctrl Pts',(19.6074016315414,-13.1910760972814,
12.));
#220026=CARTESIAN_POINT('Ctrl Pts',(19.6260031174244,-13.1965761547151,
12.));
#220027=CARTESIAN_POINT('Ctrl Pts',(19.6447286034772,-13.2020572902065,
12.));
#220028=CARTESIAN_POINT('Ctrl Pts',(19.6635773160936,-13.2075187889529,
12.));
#220029=CARTESIAN_POINT('Ctrl Pts',(19.6825484905823,-13.2129599468485,
12.));
#220030=CARTESIAN_POINT('Ctrl Pts',(19.7016413709685,-13.2183800702436,
12.));
#220031=CARTESIAN_POINT('Ctrl Pts',(19.7208552097868,-13.2237784757065,
12.));
#220032=CARTESIAN_POINT('Ctrl Pts',(19.7401892678697,-13.2291544897899,
12.));
#220033=CARTESIAN_POINT('Ctrl Pts',(19.7596428141168,-13.2345074487963,
12.));
#220034=CARTESIAN_POINT('Ctrl Pts',(19.7792151253289,-13.2398366985675,
12.));
#220035=CARTESIAN_POINT('Ctrl Pts',(19.7989054860495,-13.2451415942805,
12.));
#220036=CARTESIAN_POINT('Ctrl Pts',(19.8187131883917,-13.2504215002457,
12.));
#220037=CARTESIAN_POINT('Ctrl Pts',(19.8386375318634,-13.2556757897086,
12.));
#220038=CARTESIAN_POINT('Ctrl Pts',(19.8586778231715,-13.2609038446529,
12.));
#220039=CARTESIAN_POINT('Ctrl Pts',(19.8788333760577,-13.2661050556132,
12.));
#220040=CARTESIAN_POINT('Ctrl Pts',(19.8991035111745,-13.271278821502,12.));
#220041=CARTESIAN_POINT('Ctrl Pts',(19.9194875559422,-13.2764245494357,
12.));
#220042=CARTESIAN_POINT('Ctrl Pts',(19.9399848444019,-13.2815416545663,
12.));
#220043=CARTESIAN_POINT('Ctrl Pts',(19.9605947170586,-13.286629559915,12.));
#220044=CARTESIAN_POINT('Ctrl Pts',(19.981316520717,-13.2916876962094,12.));
#220045=CARTESIAN_POINT('Ctrl Pts',(20.0021496083738,-13.2967155017306,
12.));
#220046=CARTESIAN_POINT('Ctrl Pts',(20.0230933391038,-13.3017124221637,
12.));
#220047=CARTESIAN_POINT('Ctrl Pts',(20.0441470779345,-13.3066779104515,
12.));
#220048=CARTESIAN_POINT('Ctrl Pts',(20.0653101957188,-13.3116114266515,
12.));
#220049=CARTESIAN_POINT('Ctrl Pts',(20.0865820689882,-13.3165124377963,
12.));
#220050=CARTESIAN_POINT('Ctrl Pts',(20.1079620798375,-13.3213804177587,
12.));
#220051=CARTESIAN_POINT('Ctrl Pts',(20.1294496158402,-13.3262148471226,
12.));
#220052=CARTESIAN_POINT('Ctrl Pts',(20.1510440699474,-13.3310152130564,
12.));
#220053=CARTESIAN_POINT('Ctrl Pts',(20.1727448403817,-13.3357810091903,
12.));
#220054=CARTESIAN_POINT('Ctrl Pts',(20.1945513305235,-13.3405117354971,
12.));
#220055=CARTESIAN_POINT('Ctrl Pts',(20.216462948786,-13.3452068981766,12.));
#220056=CARTESIAN_POINT('Ctrl Pts',(20.2384791085359,-13.3498660095386,
12.));
#220057=CARTESIAN_POINT('Ctrl Pts',(20.2605992280122,-13.3544885878889,
12.));
#220058=CARTESIAN_POINT('Ctrl Pts',(20.2828227302339,-13.3590741574195,
12.));
#220059=CARTESIAN_POINT('Ctrl Pts',(20.3051490429048,-13.3636222481016,
12.));
#220060=CARTESIAN_POINT('Ctrl Pts',(20.3275775983029,-13.3681323955826,
12.));
#220061=CARTESIAN_POINT('Ctrl Pts',(20.3501078331814,-13.3726041410867,
12.));
#220062=CARTESIAN_POINT('Ctrl Pts',(20.3727391887184,-13.3770370313188,
12.));
#220063=CARTESIAN_POINT('Ctrl Pts',(20.3954711104502,-13.3814306183719,
12.));
#220064=CARTESIAN_POINT('Ctrl Pts',(20.4183030482002,-13.3857844596387,
12.));
#220065=CARTESIAN_POINT('Ctrl Pts',(20.4412344560008,-13.3900981177255,
12.));
#220066=CARTESIAN_POINT('Ctrl Pts',(20.4642647920038,-13.3943711603739,
12.));
#220067=CARTESIAN_POINT('Ctrl Pts',(20.487393518404,-13.3986031603716,12.));
#220068=CARTESIAN_POINT('Ctrl Pts',(20.5106201013753,-13.4027936954529,
12.));
#220069=CARTESIAN_POINT('Ctrl Pts',(20.5339440109956,-13.4069423482076,
12.));
#220070=CARTESIAN_POINT('Ctrl Pts',(20.5573647211639,-13.4110487059912,
12.));
#220071=CARTESIAN_POINT('Ctrl Pts',(20.5808817095155,-13.4151123608411,
12.));
#220072=CARTESIAN_POINT('Ctrl Pts',(20.6044944573153,-13.4191329093933,
12.));
#220073=CARTESIAN_POINT('Ctrl Pts',(20.6282024494237,-13.4231099528179,
12.));
#220074=CARTESIAN_POINT('Ctrl Pts',(20.6520051742869,-13.4270430967651,
12.));
#220075=CARTESIAN_POINT('Ctrl Pts',(20.6759021239103,-13.4309319513119,
12.));
#220076=CARTESIAN_POINT('Ctrl Pts',(20.6998927938288,-13.4347761309154,
12.));
#220077=CARTESIAN_POINT('Ctrl Pts',(20.7239766830675,-13.4385752543663,
12.));
#220078=CARTESIAN_POINT('Ctrl Pts',(20.7481532941013,-13.4423289447561,
12.));
#220079=CARTESIAN_POINT('Ctrl Pts',(20.7724221327608,-13.4460368293688,
12.));
#220080=CARTESIAN_POINT('Ctrl Pts',(20.7967827081227,-13.4496985395637,
12.));
#220081=CARTESIAN_POINT('Ctrl Pts',(20.821234532398,-13.4533137106667,12.));
#220082=CARTESIAN_POINT('Ctrl Pts',(20.8457771208082,-13.4568819818631,
12.));
#220083=CARTESIAN_POINT('Ctrl Pts',(20.8704099914641,-13.4604029960983,
12.));
#220084=CARTESIAN_POINT('Ctrl Pts',(20.8951326652158,-13.4638763999725,
12.));
#220085=CARTESIAN_POINT('Ctrl Pts',(20.9199446657584,-13.4673018437718,
12.));
#220086=CARTESIAN_POINT('Ctrl Pts',(20.9448455197557,-13.4706789815166,
12.));
#220087=CARTESIAN_POINT('Ctrl Pts',(20.9698347569476,-13.4740074710087,
12.));
#220088=CARTESIAN_POINT('Ctrl Pts',(20.9949119102592,-13.4772869738879,
12.));
#220089=CARTESIAN_POINT('Ctrl Pts',(21.0200765158885,-13.4805171556822,
12.));
#220090=CARTESIAN_POINT('Ctrl Pts',(21.0453281134247,-13.4836976858912,
12.));
#220091=CARTESIAN_POINT('Ctrl Pts',(21.0706662455202,-13.4868282377192,
12.));
#220092=CARTESIAN_POINT('Ctrl Pts',(21.0960904575048,-13.4899084877718,
12.));
#220093=CARTESIAN_POINT('Ctrl Pts',(21.1216002970209,-13.4929381157778,
12.));
#220094=CARTESIAN_POINT('Ctrl Pts',(21.1471953136209,-13.4959168042934,
12.));
#220095=CARTESIAN_POINT('Ctrl Pts',(21.1728750584173,-13.4988442384491,
12.));
#220096=CARTESIAN_POINT('Ctrl Pts',(21.1986390835825,-13.5017201056088,
12.));
#220097=CARTESIAN_POINT('Ctrl Pts',(21.224486942933,-13.5045440957404,12.));
#220098=CARTESIAN_POINT('Ctrl Pts',(21.2504181927429,-13.5073159019454,
12.));
#220099=CARTESIAN_POINT('Ctrl Pts',(21.2764323924442,-13.5100352209207,
12.));
#220100=CARTESIAN_POINT('Ctrl Pts',(21.3025291054236,-13.5127017534972,
12.));
#220101=CARTESIAN_POINT('Ctrl Pts',(21.328707899634,-13.5153152050554,12.));
#220102=CARTESIAN_POINT('Ctrl Pts',(21.3549683486219,-13.5178752862461,
12.));
#220103=CARTESIAN_POINT('Ctrl Pts',(21.3813100304967,-13.5203817122497,
12.));
#220104=CARTESIAN_POINT('Ctrl Pts',(21.4077325259318,-13.5228342013508,
12.));
#220105=CARTESIAN_POINT('Ctrl Pts',(21.4342354165254,-13.5252324737795,
12.));
#220106=CARTESIAN_POINT('Ctrl Pts',(21.4608182828695,-13.5275762503553,
12.));
#220107=CARTESIAN_POINT('Ctrl Pts',(21.487480703047,-13.5298652514357,12.));
#220108=CARTESIAN_POINT('Ctrl Pts',(21.5142222501671,-13.5320991952145,
12.));
#220109=CARTESIAN_POINT('Ctrl Pts',(21.5410424932511,-13.5342777983225,
12.));
#220110=CARTESIAN_POINT('Ctrl Pts',(21.5679410019011,-13.5364007790292,
12.));
#220111=CARTESIAN_POINT('Ctrl Pts',(21.5949173499022,-13.5384678597206,
12.));
#220112=CARTESIAN_POINT('Ctrl Pts',(21.6219711193951,-13.5404787697798,
12.));
#220113=CARTESIAN_POINT('Ctrl Pts',(21.6491019044647,-13.5424332480698,
12.));
#220114=CARTESIAN_POINT('Ctrl Pts',(21.676309315769,-13.5443310461516,12.));
#220115=CARTESIAN_POINT('Ctrl Pts',(21.7035929822939,-13.546171929503,12.));
#220116=CARTESIAN_POINT('Ctrl Pts',(21.730952541226,-13.5479556704457,12.));
#220117=CARTESIAN_POINT('Ctrl Pts',(21.7583876294532,-13.5496820422186,
12.));
#220118=CARTESIAN_POINT('Ctrl Pts',(21.7858978745848,-13.5513508127232,
12.));
#220119=CARTESIAN_POINT('Ctrl Pts',(21.8134828857963,-13.5529617381569,
12.));
#220120=CARTESIAN_POINT('Ctrl Pts',(21.841142245609,-13.5545145573048,12.));
#220121=CARTESIAN_POINT('Ctrl Pts',(21.8688754989401,-13.5560089839426,
12.));
#220122=CARTESIAN_POINT('Ctrl Pts',(21.8966821688876,-13.5574447178485,
12.));
#220123=CARTESIAN_POINT('Ctrl Pts',(21.9245617765827,-13.5588214586672,
12.));
#220124=CARTESIAN_POINT('Ctrl Pts',(21.9525138592862,-13.5601389185315,
12.));
#220125=CARTESIAN_POINT('Ctrl Pts',(21.9805379899192,-13.5613968357589,
12.));
#220126=CARTESIAN_POINT('Ctrl Pts',(22.0086337943431,-13.5625949868313,
12.));
#220127=CARTESIAN_POINT('Ctrl Pts',(22.0368009736227,-13.5637332022393,
12.));
#220128=CARTESIAN_POINT('Ctrl Pts',(22.0650393089492,-13.5648113688895,
12.));
#220129=CARTESIAN_POINT('Ctrl Pts',(22.0933486464442,-13.5658294169106,
12.));
#220130=CARTESIAN_POINT('Ctrl Pts',(22.1217288871823,-13.5667873105179,
12.));
#220131=CARTESIAN_POINT('Ctrl Pts',(22.1444897575076,-13.5675054918922,
12.));
#220132=CARTESIAN_POINT('Ctrl Pts',(22.1615922804939,-13.5680170531724,
12.));
#220133=CARTESIAN_POINT('Ctrl Pts',(22.1730081264583,-13.5683460612913,
12.));
#220134=CARTESIAN_POINT('Ctrl Pts',(22.1787195904339,-13.5685075571671,
12.));
#220135=CARTESIAN_POINT('Ctrl Pts',(17.1452095830632,-14.6513681262571,
0.));
#220136=CARTESIAN_POINT('Ctrl Pts',(17.1452095830632,-14.6513681262571,
12.));
#220137=CARTESIAN_POINT('Ctrl Pts',(17.1452153999142,-14.6513711852843,
0.));
#220138=CARTESIAN_POINT('Ctrl Pts',(17.1452153999142,-14.6513711852843,
12.));
#220139=CARTESIAN_POINT('Ctrl Pts',(17.1452600887037,-14.6514066997196,
0.));
#220140=CARTESIAN_POINT('Ctrl Pts',(17.1452600887037,-14.6514066997196,
12.));
#220141=CARTESIAN_POINT('Ctrl Pts',(17.1454262858043,-14.6515481598068,
0.));
#220142=CARTESIAN_POINT('Ctrl Pts',(17.1454262858043,-14.6515481598068,
12.));
#220143=CARTESIAN_POINT('Ctrl Pts',(17.1458462295271,-14.6519131634508,
0.));
#220144=CARTESIAN_POINT('Ctrl Pts',(17.1458462295271,-14.6519131634508,
12.));
#220145=CARTESIAN_POINT('Ctrl Pts',(17.1466998098673,-14.6526624064978,
0.));
#220146=CARTESIAN_POINT('Ctrl Pts',(17.1466998098673,-14.6526624064978,
12.));
#220147=CARTESIAN_POINT('Ctrl Pts',(17.147876394491,-14.6537016966184,0.));
#220148=CARTESIAN_POINT('Ctrl Pts',(17.147876394491,-14.6537016966184,12.));
#220149=CARTESIAN_POINT('Ctrl Pts',(17.1493641837558,-14.655024862281,0.));
#220150=CARTESIAN_POINT('Ctrl Pts',(17.1493641837558,-14.655024862281,12.));
#220151=CARTESIAN_POINT('Ctrl Pts',(17.1511476869496,-14.6566237952435,
0.));
#220152=CARTESIAN_POINT('Ctrl Pts',(17.1511476869496,-14.6566237952435,
12.));
#220153=CARTESIAN_POINT('Ctrl Pts',(17.1532107762718,-14.6584900555302,
0.));
#220154=CARTESIAN_POINT('Ctrl Pts',(17.1532107762718,-14.6584900555302,
12.));
#220155=CARTESIAN_POINT('Ctrl Pts',(17.1555401986401,-14.6606167169642,
0.));
#220156=CARTESIAN_POINT('Ctrl Pts',(17.1555401986401,-14.6606167169642,
12.));
#220157=CARTESIAN_POINT('Ctrl Pts',(17.1581262646789,-14.6629987285992,
0.));
#220158=CARTESIAN_POINT('Ctrl Pts',(17.1581262646789,-14.6629987285992,
12.));
#220159=CARTESIAN_POINT('Ctrl Pts',(17.1609609517369,-14.6656319165057,
0.));
#220160=CARTESIAN_POINT('Ctrl Pts',(17.1609609517369,-14.6656319165057,
12.));
#220161=CARTESIAN_POINT('Ctrl Pts',(17.1640366762305,-14.6685123374423,
0.));
#220162=CARTESIAN_POINT('Ctrl Pts',(17.1640366762305,-14.6685123374423,
12.));
#220163=CARTESIAN_POINT('Ctrl Pts',(17.167344972302,-14.671635583332,0.));
#220164=CARTESIAN_POINT('Ctrl Pts',(17.167344972302,-14.671635583332,12.));
#220165=CARTESIAN_POINT('Ctrl Pts',(17.1708771619129,-14.6749971333867,
0.));
#220166=CARTESIAN_POINT('Ctrl Pts',(17.1708771619129,-14.6749971333867,
12.));
#220167=CARTESIAN_POINT('Ctrl Pts',(17.1746247499057,-14.6785925615677,
0.));
#220168=CARTESIAN_POINT('Ctrl Pts',(17.1746247499057,-14.6785925615677,
12.));
#220169=CARTESIAN_POINT('Ctrl Pts',(17.1785800350826,-14.6824178576167,
0.));
#220170=CARTESIAN_POINT('Ctrl Pts',(17.1785800350826,-14.6824178576167,
12.));
#220171=CARTESIAN_POINT('Ctrl Pts',(17.182736158472,-14.686469452232,0.));
#220172=CARTESIAN_POINT('Ctrl Pts',(17.182736158472,-14.686469452232,12.));
#220173=CARTESIAN_POINT('Ctrl Pts',(17.1870867909918,-14.6907440526958,
0.));
#220174=CARTESIAN_POINT('Ctrl Pts',(17.1870867909918,-14.6907440526958,
12.));
#220175=CARTESIAN_POINT('Ctrl Pts',(17.1916259308415,-14.6952385361706,
0.));
#220176=CARTESIAN_POINT('Ctrl Pts',(17.1916259308415,-14.6952385361706,
12.));
#220177=CARTESIAN_POINT('Ctrl Pts',(17.1963476411694,-14.699949811582,0.));
#220178=CARTESIAN_POINT('Ctrl Pts',(17.1963476411694,-14.699949811582,12.));
#220179=CARTESIAN_POINT('Ctrl Pts',(17.2012461084268,-14.7048748502663,
0.));
#220180=CARTESIAN_POINT('Ctrl Pts',(17.2012461084268,-14.7048748502663,
12.));
#220181=CARTESIAN_POINT('Ctrl Pts',(17.2063157097315,-14.7100107213586,
0.));
#220182=CARTESIAN_POINT('Ctrl Pts',(17.2063157097315,-14.7100107213586,
12.));
#220183=CARTESIAN_POINT('Ctrl Pts',(17.2115510835989,-14.7153546289339,
0.));
#220184=CARTESIAN_POINT('Ctrl Pts',(17.2115510835989,-14.7153546289339,
12.));
#220185=CARTESIAN_POINT('Ctrl Pts',(17.2169471814256,-14.7209039390327,
0.));
#220186=CARTESIAN_POINT('Ctrl Pts',(17.2169471814256,-14.7209039390327,
12.));
#220187=CARTESIAN_POINT('Ctrl Pts',(17.2224992099667,-14.7266561494282,
0.));
#220188=CARTESIAN_POINT('Ctrl Pts',(17.2224992099667,-14.7266561494282,
12.));
#220189=CARTESIAN_POINT('Ctrl Pts',(17.2282025904314,-14.7326088681163,
0.));
#220190=CARTESIAN_POINT('Ctrl Pts',(17.2282025904314,-14.7326088681163,
12.));
#220191=CARTESIAN_POINT('Ctrl Pts',(17.2340529062076,-14.7387597858117,
0.));
#220192=CARTESIAN_POINT('Ctrl Pts',(17.2340529062076,-14.7387597858117,
12.));
#220193=CARTESIAN_POINT('Ctrl Pts',(17.2400458713565,-14.7451066593792,
0.));
#220194=CARTESIAN_POINT('Ctrl Pts',(17.2400458713565,-14.7451066593792,
12.));
#220195=CARTESIAN_POINT('Ctrl Pts',(17.2461773413288,-14.7516473175124,
0.));
#220196=CARTESIAN_POINT('Ctrl Pts',(17.2461773413288,-14.7516473175124,
12.));
#220197=CARTESIAN_POINT('Ctrl Pts',(17.2524433146837,-14.7583796616617,
0.));
#220198=CARTESIAN_POINT('Ctrl Pts',(17.2524433146837,-14.7583796616617,
12.));
#220199=CARTESIAN_POINT('Ctrl Pts',(17.2588399401465,-14.7653016697591,
0.));
#220200=CARTESIAN_POINT('Ctrl Pts',(17.2588399401465,-14.7653016697591,
12.));
#220201=CARTESIAN_POINT('Ctrl Pts',(17.2653635155319,-14.7724113956731,
0.));
#220202=CARTESIAN_POINT('Ctrl Pts',(17.2653635155319,-14.7724113956731,
12.));
#220203=CARTESIAN_POINT('Ctrl Pts',(17.2720104735194,-14.7797069617804,
0.));
#220204=CARTESIAN_POINT('Ctrl Pts',(17.2720104735194,-14.7797069617804,
12.));
#220205=CARTESIAN_POINT('Ctrl Pts',(17.2787773704849,-14.787186553128,0.));
#220206=CARTESIAN_POINT('Ctrl Pts',(17.2787773704849,-14.787186553128,12.));
#220207=CARTESIAN_POINT('Ctrl Pts',(17.2856608733196,-14.7948484105249,
0.));
#220208=CARTESIAN_POINT('Ctrl Pts',(17.2856608733196,-14.7948484105249,
12.));
#220209=CARTESIAN_POINT('Ctrl Pts',(17.2926577496513,-14.8026908254276,
0.));
#220210=CARTESIAN_POINT('Ctrl Pts',(17.2926577496513,-14.8026908254276,
12.));
#220211=CARTESIAN_POINT('Ctrl Pts',(17.299764866148,-14.8107121391035,0.));
#220212=CARTESIAN_POINT('Ctrl Pts',(17.299764866148,-14.8107121391035,12.));
#220213=CARTESIAN_POINT('Ctrl Pts',(17.3069791853706,-14.8189107410162,
0.));
#220214=CARTESIAN_POINT('Ctrl Pts',(17.3069791853706,-14.8189107410162,
12.));
#220215=CARTESIAN_POINT('Ctrl Pts',(17.3142977632659,-14.8272850675379,
0.));
#220216=CARTESIAN_POINT('Ctrl Pts',(17.3142977632659,-14.8272850675379,
12.));
#220217=CARTESIAN_POINT('Ctrl Pts',(17.3217177462101,-14.8358336004197,
0.));
#220218=CARTESIAN_POINT('Ctrl Pts',(17.3217177462101,-14.8358336004197,
12.));
#220219=CARTESIAN_POINT('Ctrl Pts',(17.3292363662605,-14.8445548643508,
0.));
#220220=CARTESIAN_POINT('Ctrl Pts',(17.3292363662605,-14.8445548643508,
12.));
#220221=CARTESIAN_POINT('Ctrl Pts',(17.336850936485,-14.8534474245434,0.));
#220222=CARTESIAN_POINT('Ctrl Pts',(17.336850936485,-14.8534474245434,12.));
#220223=CARTESIAN_POINT('Ctrl Pts',(17.3445588463474,-14.8625098843417,
0.));
#220224=CARTESIAN_POINT('Ctrl Pts',(17.3445588463474,-14.8625098843417,
12.));
#220225=CARTESIAN_POINT('Ctrl Pts',(17.3523575568645,-14.8717408826956,
0.));
#220226=CARTESIAN_POINT('Ctrl Pts',(17.3523575568645,-14.8717408826956,
12.));
#220227=CARTESIAN_POINT('Ctrl Pts',(17.3602445978161,-14.8811390927423,
0.));
#220228=CARTESIAN_POINT('Ctrl Pts',(17.3602445978161,-14.8811390927423,
12.));
#220229=CARTESIAN_POINT('Ctrl Pts',(17.3682175653235,-14.8907032205788,
0.));
#220230=CARTESIAN_POINT('Ctrl Pts',(17.3682175653235,-14.8907032205788,
12.));
#220231=CARTESIAN_POINT('Ctrl Pts',(17.3762741193076,-14.900432003961,0.));
#220232=CARTESIAN_POINT('Ctrl Pts',(17.3762741193076,-14.900432003961,12.));
#220233=CARTESIAN_POINT('Ctrl Pts',(17.3844119809824,-14.9103242110057,
0.));
#220234=CARTESIAN_POINT('Ctrl Pts',(17.3844119809824,-14.9103242110057,
12.));
#220235=CARTESIAN_POINT('Ctrl Pts',(17.3926289303986,-14.9203786389342,
0.));
#220236=CARTESIAN_POINT('Ctrl Pts',(17.3926289303986,-14.9203786389342,
12.));
#220237=CARTESIAN_POINT('Ctrl Pts',(17.4009228040749,-14.9305941128757,
0.));
#220238=CARTESIAN_POINT('Ctrl Pts',(17.4009228040749,-14.9305941128757,
12.));
#220239=CARTESIAN_POINT('Ctrl Pts',(17.4092914926071,-14.940969484645,0.));
#220240=CARTESIAN_POINT('Ctrl Pts',(17.4092914926071,-14.940969484645,12.));
#220241=CARTESIAN_POINT('Ctrl Pts',(17.4177329382828,-14.9515036315143,
0.));
#220242=CARTESIAN_POINT('Ctrl Pts',(17.4177329382828,-14.9515036315143,
12.));
#220243=CARTESIAN_POINT('Ctrl Pts',(17.426245132709,-14.9621954549827,0.));
#220244=CARTESIAN_POINT('Ctrl Pts',(17.426245132709,-14.9621954549827,12.));
#220245=CARTESIAN_POINT('Ctrl Pts',(17.4348261151396,-14.9730438799452,
0.));
#220246=CARTESIAN_POINT('Ctrl Pts',(17.4348261151396,-14.9730438799452,
12.));
#220247=CARTESIAN_POINT('Ctrl Pts',(17.4434739707773,-14.9840478538358,
0.));
#220248=CARTESIAN_POINT('Ctrl Pts',(17.4434739707773,-14.9840478538358,
12.));
#220249=CARTESIAN_POINT('Ctrl Pts',(17.4521868291004,-14.9952063457778,
0.));
#220250=CARTESIAN_POINT('Ctrl Pts',(17.4521868291004,-14.9952063457778,
12.));
#220251=CARTESIAN_POINT('Ctrl Pts',(17.4609628621418,-15.0065183456921,
0.));
#220252=CARTESIAN_POINT('Ctrl Pts',(17.4609628621418,-15.0065183456921,
12.));
#220253=CARTESIAN_POINT('Ctrl Pts',(17.4698002829357,-15.0179828635086,
0.));
#220254=CARTESIAN_POINT('Ctrl Pts',(17.4698002829357,-15.0179828635086,
12.));
#220255=CARTESIAN_POINT('Ctrl Pts',(17.4786973441417,-15.029598928488,0.));
#220256=CARTESIAN_POINT('Ctrl Pts',(17.4786973441417,-15.029598928488,12.));
#220257=CARTESIAN_POINT('Ctrl Pts',(17.4876523366178,-15.0413655884993,
0.));
#220258=CARTESIAN_POINT('Ctrl Pts',(17.4876523366178,-15.0413655884993,
12.));
#220259=CARTESIAN_POINT('Ctrl Pts',(17.4966635880245,-15.0532819093085,
0.));
#220260=CARTESIAN_POINT('Ctrl Pts',(17.4966635880245,-15.0532819093085,
12.));
#220261=CARTESIAN_POINT('Ctrl Pts',(17.5057294613874,-15.0653469738306,
0.));
#220262=CARTESIAN_POINT('Ctrl Pts',(17.5057294613874,-15.0653469738306,
12.));
#220263=CARTESIAN_POINT('Ctrl Pts',(17.5148483539683,-15.0775598815748,
0.));
#220264=CARTESIAN_POINT('Ctrl Pts',(17.5148483539683,-15.0775598815748,
12.));
#220265=CARTESIAN_POINT('Ctrl Pts',(17.5240186961788,-15.0899197481082,
0.));
#220266=CARTESIAN_POINT('Ctrl Pts',(17.5240186961788,-15.0899197481082,
12.));
#220267=CARTESIAN_POINT('Ctrl Pts',(17.5332389504829,-15.1024257045033,
0.));
#220268=CARTESIAN_POINT('Ctrl Pts',(17.5332389504829,-15.1024257045033,
12.));
#220269=CARTESIAN_POINT('Ctrl Pts',(17.5425076102966,-15.1150768967729,
0.));
#220270=CARTESIAN_POINT('Ctrl Pts',(17.5425076102966,-15.1150768967729,
12.));
#220271=CARTESIAN_POINT('Ctrl Pts',(17.5518231989122,-15.127872485314,0.));
#220272=CARTESIAN_POINT('Ctrl Pts',(17.5518231989122,-15.127872485314,12.));
#220273=CARTESIAN_POINT('Ctrl Pts',(17.5611842686196,-15.1408116444877,
0.));
#220274=CARTESIAN_POINT('Ctrl Pts',(17.5611842686196,-15.1408116444877,
12.));
#220275=CARTESIAN_POINT('Ctrl Pts',(17.570589399803,-15.1538935621715,0.));
#220276=CARTESIAN_POINT('Ctrl Pts',(17.570589399803,-15.1538935621715,12.));
#220277=CARTESIAN_POINT('Ctrl Pts',(17.5800372000539,-15.1671174393136,
0.));
#220278=CARTESIAN_POINT('Ctrl Pts',(17.5800372000539,-15.1671174393136,
12.));
#220279=CARTESIAN_POINT('Ctrl Pts',(17.5895263032592,-15.1804824894605,
0.));
#220280=CARTESIAN_POINT('Ctrl Pts',(17.5895263032592,-15.1804824894605,
12.));
#220281=CARTESIAN_POINT('Ctrl Pts',(17.5990553687595,-15.1939879383268,
0.));
#220282=CARTESIAN_POINT('Ctrl Pts',(17.5990553687595,-15.1939879383268,
12.));
#220283=CARTESIAN_POINT('Ctrl Pts',(17.6086230806497,-15.2076330234686,
0.));
#220284=CARTESIAN_POINT('Ctrl Pts',(17.6086230806497,-15.2076330234686,
12.));
#220285=CARTESIAN_POINT('Ctrl Pts',(17.6182281470467,-15.22141699392,0.));
#220286=CARTESIAN_POINT('Ctrl Pts',(17.6182281470467,-15.22141699392,12.));
#220287=CARTESIAN_POINT('Ctrl Pts',(17.6278692993765,-15.2353391098367,
0.));
#220288=CARTESIAN_POINT('Ctrl Pts',(17.6278692993765,-15.2353391098367,
12.));
#220289=CARTESIAN_POINT('Ctrl Pts',(17.637545291637,-15.2493986421091,0.));
#220290=CARTESIAN_POINT('Ctrl Pts',(17.637545291637,-15.2493986421091,12.));
#220291=CARTESIAN_POINT('Ctrl Pts',(17.6472548997329,-15.263594872029,0.));
#220292=CARTESIAN_POINT('Ctrl Pts',(17.6472548997329,-15.263594872029,12.));
#220293=CARTESIAN_POINT('Ctrl Pts',(17.6569969209,-15.2779270910238,0.));
#220294=CARTESIAN_POINT('Ctrl Pts',(17.6569969209,-15.2779270910238,12.));
#220295=CARTESIAN_POINT('Ctrl Pts',(17.6667701731041,-15.2923946003598,
0.));
#220296=CARTESIAN_POINT('Ctrl Pts',(17.6667701731041,-15.2923946003598,
12.));
#220297=CARTESIAN_POINT('Ctrl Pts',(17.6765734944559,-15.3069967108501,
0.));
#220298=CARTESIAN_POINT('Ctrl Pts',(17.6765734944559,-15.3069967108501,
12.));
#220299=CARTESIAN_POINT('Ctrl Pts',(17.6864057426052,-15.3217327425341,
0.));
#220300=CARTESIAN_POINT('Ctrl Pts',(17.6864057426052,-15.3217327425341,
12.));
#220301=CARTESIAN_POINT('Ctrl Pts',(17.6962657941984,-15.3366020244069,
0.));
#220302=CARTESIAN_POINT('Ctrl Pts',(17.6962657941984,-15.3366020244069,
12.));
#220303=CARTESIAN_POINT('Ctrl Pts',(17.7061525444044,-15.3516038942064,
0.));
#220304=CARTESIAN_POINT('Ctrl Pts',(17.7061525444044,-15.3516038942064,
12.));
#220305=CARTESIAN_POINT('Ctrl Pts',(17.7160649064208,-15.3667376981702,
0.));
#220306=CARTESIAN_POINT('Ctrl Pts',(17.7160649064208,-15.3667376981702,
12.));
#220307=CARTESIAN_POINT('Ctrl Pts',(17.7260018109923,-15.3820027907965,
0.));
#220308=CARTESIAN_POINT('Ctrl Pts',(17.7260018109923,-15.3820027907965,
12.));
#220309=CARTESIAN_POINT('Ctrl Pts',(17.7359622059143,-15.3973985345796,
0.));
#220310=CARTESIAN_POINT('Ctrl Pts',(17.7359622059143,-15.3973985345796,
12.));
#220311=CARTESIAN_POINT('Ctrl Pts',(17.7459450555803,-15.4129242997828,
0.));
#220312=CARTESIAN_POINT('Ctrl Pts',(17.7459450555803,-15.4129242997828,
12.));
#220313=CARTESIAN_POINT('Ctrl Pts',(17.7559493405871,-15.4285794642658,
0.));
#220314=CARTESIAN_POINT('Ctrl Pts',(17.7559493405871,-15.4285794642658,
12.));
#220315=CARTESIAN_POINT('Ctrl Pts',(17.765974057326,-15.4443634132865,0.));
#220316=CARTESIAN_POINT('Ctrl Pts',(17.765974057326,-15.4443634132865,12.));
#220317=CARTESIAN_POINT('Ctrl Pts',(17.7760182175817,-15.4602755393019,
0.));
#220318=CARTESIAN_POINT('Ctrl Pts',(17.7760182175817,-15.4602755393019,
12.));
#220319=CARTESIAN_POINT('Ctrl Pts',(17.7860808481229,-15.4763152417506,
0.));
#220320=CARTESIAN_POINT('Ctrl Pts',(17.7860808481229,-15.4763152417506,
12.));
#220321=CARTESIAN_POINT('Ctrl Pts',(17.7961609903161,-15.4924819268529,
0.));
#220322=CARTESIAN_POINT('Ctrl Pts',(17.7961609903161,-15.4924819268529,
12.));
#220323=CARTESIAN_POINT('Ctrl Pts',(17.8062576997964,-15.5087750074728,
0.));
#220324=CARTESIAN_POINT('Ctrl Pts',(17.8062576997964,-15.5087750074728,
12.));
#220325=CARTESIAN_POINT('Ctrl Pts',(17.8163700461263,-15.5251939029558,
0.));
#220326=CARTESIAN_POINT('Ctrl Pts',(17.8163700461263,-15.5251939029558,
12.));
#220327=CARTESIAN_POINT('Ctrl Pts',(17.8264971124606,-15.5417380389639,
0.));
#220328=CARTESIAN_POINT('Ctrl Pts',(17.8264971124606,-15.5417380389639,
12.));
#220329=CARTESIAN_POINT('Ctrl Pts',(17.8366379952078,-15.5584068472976,
0.));
#220330=CARTESIAN_POINT('Ctrl Pts',(17.8366379952078,-15.5584068472976,
12.));
#220331=CARTESIAN_POINT('Ctrl Pts',(17.8467918036976,-15.5751997657153,
0.));
#220332=CARTESIAN_POINT('Ctrl Pts',(17.8467918036976,-15.5751997657153,
12.));
#220333=CARTESIAN_POINT('Ctrl Pts',(17.8569576598996,-15.5921162378183,
0.));
#220334=CARTESIAN_POINT('Ctrl Pts',(17.8569576598996,-15.5921162378183,
12.));
#220335=CARTESIAN_POINT('Ctrl Pts',(17.8671346981388,-15.6091557129205,
0.));
#220336=CARTESIAN_POINT('Ctrl Pts',(17.8671346981388,-15.6091557129205,
12.));
#220337=CARTESIAN_POINT('Ctrl Pts',(17.8773220648125,-15.6263176459107,
0.));
#220338=CARTESIAN_POINT('Ctrl Pts',(17.8773220648125,-15.6263176459107,
12.));
#220339=CARTESIAN_POINT('Ctrl Pts',(17.8875189181095,-15.6436014971088,
0.));
#220340=CARTESIAN_POINT('Ctrl Pts',(17.8875189181095,-15.6436014971088,
12.));
#220341=CARTESIAN_POINT('Ctrl Pts',(17.8977244277247,-15.6610067321036,
0.));
#220342=CARTESIAN_POINT('Ctrl Pts',(17.8977244277247,-15.6610067321036,
12.));
#220343=CARTESIAN_POINT('Ctrl Pts',(17.9079377746118,-15.6785328216467,
0.));
#220344=CARTESIAN_POINT('Ctrl Pts',(17.9079377746118,-15.6785328216467,
12.));
#220345=CARTESIAN_POINT('Ctrl Pts',(17.918158150746,-15.6961792415526,0.));
#220346=CARTESIAN_POINT('Ctrl Pts',(17.918158150746,-15.6961792415526,12.));
#220347=CARTESIAN_POINT('Ctrl Pts',(17.9283847588837,-15.713945472584,0.));
#220348=CARTESIAN_POINT('Ctrl Pts',(17.9283847588837,-15.713945472584,12.));
#220349=CARTESIAN_POINT('Ctrl Pts',(17.9386168123261,-15.7318310003334,
0.));
#220350=CARTESIAN_POINT('Ctrl Pts',(17.9386168123261,-15.7318310003334,
12.));
#220351=CARTESIAN_POINT('Ctrl Pts',(17.9488535346776,-15.7498353150856,
0.));
#220352=CARTESIAN_POINT('Ctrl Pts',(17.9488535346776,-15.7498353150856,
12.));
#220353=CARTESIAN_POINT('Ctrl Pts',(17.9590941596236,-15.7679579117072,
0.));
#220354=CARTESIAN_POINT('Ctrl Pts',(17.9590941596236,-15.7679579117072,
12.));
#220355=CARTESIAN_POINT('Ctrl Pts',(17.9693379307297,-15.786198289572,0.));
#220356=CARTESIAN_POINT('Ctrl Pts',(17.9693379307297,-15.786198289572,12.));
#220357=CARTESIAN_POINT('Ctrl Pts',(17.9795841012383,-15.8045559524674,
0.));
#220358=CARTESIAN_POINT('Ctrl Pts',(17.9795841012383,-15.8045559524674,
12.));
#220359=CARTESIAN_POINT('Ctrl Pts',(17.9898319338664,-15.8230304084963,
0.));
#220360=CARTESIAN_POINT('Ctrl Pts',(17.9898319338664,-15.8230304084963,
12.));
#220361=CARTESIAN_POINT('Ctrl Pts',(18.0000807006055,-15.8416211699682,
0.));
#220362=CARTESIAN_POINT('Ctrl Pts',(18.0000807006055,-15.8416211699682,
12.));
#220363=CARTESIAN_POINT('Ctrl Pts',(18.010329682521,-15.8603277532834,0.));
#220364=CARTESIAN_POINT('Ctrl Pts',(18.010329682521,-15.8603277532834,12.));
#220365=CARTESIAN_POINT('Ctrl Pts',(18.0205781695773,-15.8791496788685,
0.));
#220366=CARTESIAN_POINT('Ctrl Pts',(18.0205781695773,-15.8791496788685,
12.));
#220367=CARTESIAN_POINT('Ctrl Pts',(18.0308254604638,-15.8980864711043,
0.));
#220368=CARTESIAN_POINT('Ctrl Pts',(18.0308254604638,-15.8980864711043,
12.));
#220369=CARTESIAN_POINT('Ctrl Pts',(18.0410708624208,-15.9171376582436,
0.));
#220370=CARTESIAN_POINT('Ctrl Pts',(18.0410708624208,-15.9171376582436,
12.));
#220371=CARTESIAN_POINT('Ctrl Pts',(18.0513136910691,-15.9363027723244,
0.));
#220372=CARTESIAN_POINT('Ctrl Pts',(18.0513136910691,-15.9363027723244,
12.));
#220373=CARTESIAN_POINT('Ctrl Pts',(18.061553270236,-15.9555813490645,0.));
#220374=CARTESIAN_POINT('Ctrl Pts',(18.061553270236,-15.9555813490645,12.));
#220375=CARTESIAN_POINT('Ctrl Pts',(18.071788931796,-15.9749729277848,0.));
#220376=CARTESIAN_POINT('Ctrl Pts',(18.071788931796,-15.9749729277848,12.));
#220377=CARTESIAN_POINT('Ctrl Pts',(18.0820200155239,-15.9944770513616,
0.));
#220378=CARTESIAN_POINT('Ctrl Pts',(18.0820200155239,-15.9944770513616,
12.));
#220379=CARTESIAN_POINT('Ctrl Pts',(18.0922458689464,-16.0140932661612,
0.));
#220380=CARTESIAN_POINT('Ctrl Pts',(18.0922458689464,-16.0140932661612,
12.));
#220381=CARTESIAN_POINT('Ctrl Pts',(18.1024658471966,-16.0338211219694,
0.));
#220382=CARTESIAN_POINT('Ctrl Pts',(18.1024658471966,-16.0338211219694,
12.));
#220383=CARTESIAN_POINT('Ctrl Pts',(18.1126793128688,-16.0536601719124,
0.));
#220384=CARTESIAN_POINT('Ctrl Pts',(18.1126793128688,-16.0536601719124,
12.));
#220385=CARTESIAN_POINT('Ctrl Pts',(18.1228856358746,-16.0736099723664,
0.));
#220386=CARTESIAN_POINT('Ctrl Pts',(18.1228856358746,-16.0736099723664,
12.));
#220387=CARTESIAN_POINT('Ctrl Pts',(18.1330841933099,-16.0936700829108,
0.));
#220388=CARTESIAN_POINT('Ctrl Pts',(18.1330841933099,-16.0936700829108,
12.));
#220389=CARTESIAN_POINT('Ctrl Pts',(18.1432743693231,-16.113840066279,0.));
#220390=CARTESIAN_POINT('Ctrl Pts',(18.1432743693231,-16.113840066279,12.));
#220391=CARTESIAN_POINT('Ctrl Pts',(18.153455554985,-16.1341194882987,0.));
#220392=CARTESIAN_POINT('Ctrl Pts',(18.153455554985,-16.1341194882987,12.));
#220393=CARTESIAN_POINT('Ctrl Pts',(18.1636271481616,-16.1545079178261,
0.));
#220394=CARTESIAN_POINT('Ctrl Pts',(18.1636271481616,-16.1545079178261,
12.));
#220395=CARTESIAN_POINT('Ctrl Pts',(18.1737885533852,-16.1750049266673,
0.));
#220396=CARTESIAN_POINT('Ctrl Pts',(18.1737885533852,-16.1750049266673,
12.));
#220397=CARTESIAN_POINT('Ctrl Pts',(18.1839391817335,-16.1956100895076,
0.));
#220398=CARTESIAN_POINT('Ctrl Pts',(18.1839391817335,-16.1956100895076,
12.));
#220399=CARTESIAN_POINT('Ctrl Pts',(18.1940784507232,-16.2163229838878,
0.));
#220400=CARTESIAN_POINT('Ctrl Pts',(18.1940784507232,-16.2163229838878,
12.));
#220401=CARTESIAN_POINT('Ctrl Pts',(18.2042057842037,-16.237143190164,0.));
#220402=CARTESIAN_POINT('Ctrl Pts',(18.2042057842037,-16.237143190164,12.));
#220403=CARTESIAN_POINT('Ctrl Pts',(18.214320612253,-16.2580702914615,0.));
#220404=CARTESIAN_POINT('Ctrl Pts',(18.214320612253,-16.2580702914615,12.));
#220405=CARTESIAN_POINT('Ctrl Pts',(18.2244223710745,-16.2791038736223,
0.));
#220406=CARTESIAN_POINT('Ctrl Pts',(18.2244223710745,-16.2791038736223,
12.));
#220407=CARTESIAN_POINT('Ctrl Pts',(18.2345105028981,-16.3002435251378,
0.));
#220408=CARTESIAN_POINT('Ctrl Pts',(18.2345105028981,-16.3002435251378,
12.));
#220409=CARTESIAN_POINT('Ctrl Pts',(18.2445844558742,-16.3214888370988,
0.));
#220410=CARTESIAN_POINT('Ctrl Pts',(18.2445844558742,-16.3214888370988,
12.));
#220411=CARTESIAN_POINT('Ctrl Pts',(18.2546436839609,-16.342839403159,0.));
#220412=CARTESIAN_POINT('Ctrl Pts',(18.2546436839609,-16.342839403159,12.));
#220413=CARTESIAN_POINT('Ctrl Pts',(18.2646876468169,-16.3642948194869,
0.));
#220414=CARTESIAN_POINT('Ctrl Pts',(18.2646876468169,-16.3642948194869,
12.));
#220415=CARTESIAN_POINT('Ctrl Pts',(18.2747158096934,-16.385854684708,0.));
#220416=CARTESIAN_POINT('Ctrl Pts',(18.2747158096934,-16.385854684708,12.));
#220417=CARTESIAN_POINT('Ctrl Pts',(18.2847276433308,-16.4075185998454,
0.));
#220418=CARTESIAN_POINT('Ctrl Pts',(18.2847276433308,-16.4075185998454,
12.));
#220419=CARTESIAN_POINT('Ctrl Pts',(18.2947226238509,-16.4292861682377,
0.));
#220420=CARTESIAN_POINT('Ctrl Pts',(18.2947226238509,-16.4292861682377,
12.));
#220421=CARTESIAN_POINT('Ctrl Pts',(18.3047002326858,-16.4511569955231,
0.));
#220422=CARTESIAN_POINT('Ctrl Pts',(18.3047002326858,-16.4511569955231,
12.));
#220423=CARTESIAN_POINT('Ctrl Pts',(18.3146599565229,-16.4731306896439,
0.));
#220424=CARTESIAN_POINT('Ctrl Pts',(18.3146599565229,-16.4731306896439,
12.));
#220425=CARTESIAN_POINT('Ctrl Pts',(18.3246012872468,-16.4952068608344,
0.));
#220426=CARTESIAN_POINT('Ctrl Pts',(18.3246012872468,-16.4952068608344,
12.));
#220427=CARTESIAN_POINT('Ctrl Pts',(18.3345237218864,-16.5173851216045,
0.));
#220428=CARTESIAN_POINT('Ctrl Pts',(18.3345237218864,-16.5173851216045,
12.));
#220429=CARTESIAN_POINT('Ctrl Pts',(18.3444267625601,-16.5396650867139,
0.));
#220430=CARTESIAN_POINT('Ctrl Pts',(18.3444267625601,-16.5396650867139,
12.));
#220431=CARTESIAN_POINT('Ctrl Pts',(18.3543099164331,-16.5620463731414,
0.));
#220432=CARTESIAN_POINT('Ctrl Pts',(18.3543099164331,-16.5620463731414,
12.));
#220433=CARTESIAN_POINT('Ctrl Pts',(18.364172695589,-16.5845286000218,0.));
#220434=CARTESIAN_POINT('Ctrl Pts',(18.364172695589,-16.5845286000218,12.));
#220435=CARTESIAN_POINT('Ctrl Pts',(18.3740146168879,-16.6071113885711,
0.));
#220436=CARTESIAN_POINT('Ctrl Pts',(18.3740146168879,-16.6071113885711,
12.));
#220437=CARTESIAN_POINT('Ctrl Pts',(18.3838352018327,-16.6297943620056,
0.));
#220438=CARTESIAN_POINT('Ctrl Pts',(18.3838352018327,-16.6297943620056,
12.));
#220439=CARTESIAN_POINT('Ctrl Pts',(18.3936339764332,-16.6525771454513,
0.));
#220440=CARTESIAN_POINT('Ctrl Pts',(18.3936339764332,-16.6525771454513,
12.));
#220441=CARTESIAN_POINT('Ctrl Pts',(18.4034104710789,-16.6754593658513,
0.));
#220442=CARTESIAN_POINT('Ctrl Pts',(18.4034104710789,-16.6754593658513,
12.));
#220443=CARTESIAN_POINT('Ctrl Pts',(18.4131642203989,-16.698440651849,0.));
#220444=CARTESIAN_POINT('Ctrl Pts',(18.4131642203989,-16.698440651849,12.));
#220445=CARTESIAN_POINT('Ctrl Pts',(18.4228947633186,-16.7215206338818,
0.));
#220446=CARTESIAN_POINT('Ctrl Pts',(18.4228947633186,-16.7215206338818,
12.));
#220447=CARTESIAN_POINT('Ctrl Pts',(18.4326016431392,-16.7446989442882,
0.));
#220448=CARTESIAN_POINT('Ctrl Pts',(18.4326016431392,-16.7446989442882,
12.));
#220449=CARTESIAN_POINT('Ctrl Pts',(18.4422844076099,-16.7679752173992,
0.));
#220450=CARTESIAN_POINT('Ctrl Pts',(18.4422844076099,-16.7679752173992,
12.));
#220451=CARTESIAN_POINT('Ctrl Pts',(18.4519426090124,-16.791349089629,0.));
#220452=CARTESIAN_POINT('Ctrl Pts',(18.4519426090124,-16.791349089629,12.));
#220453=CARTESIAN_POINT('Ctrl Pts',(18.4615758042305,-16.8148201995472,
0.));
#220454=CARTESIAN_POINT('Ctrl Pts',(18.4615758042305,-16.8148201995472,
12.));
#220455=CARTESIAN_POINT('Ctrl Pts',(18.4711835548622,-16.8383881879707,
0.));
#220456=CARTESIAN_POINT('Ctrl Pts',(18.4711835548622,-16.8383881879707,
12.));
#220457=CARTESIAN_POINT('Ctrl Pts',(18.4807654268769,-16.8620526977169,
0.));
#220458=CARTESIAN_POINT('Ctrl Pts',(18.4807654268769,-16.8620526977169,
12.));
#220459=CARTESIAN_POINT('Ctrl Pts',(18.4903209902226,-16.8858133733086,
0.));
#220460=CARTESIAN_POINT('Ctrl Pts',(18.4903209902226,-16.8858133733086,
12.));
#220461=CARTESIAN_POINT('Ctrl Pts',(18.4998498184619,-16.9096698606942,
0.));
#220462=CARTESIAN_POINT('Ctrl Pts',(18.4998498184619,-16.9096698606942,
12.));
#220463=CARTESIAN_POINT('Ctrl Pts',(18.5093514883835,-16.9336218069353,
0.));
#220464=CARTESIAN_POINT('Ctrl Pts',(18.5093514883835,-16.9336218069353,
12.));
#220465=CARTESIAN_POINT('Ctrl Pts',(18.518825579666,-16.957668859934,0.));
#220466=CARTESIAN_POINT('Ctrl Pts',(18.518825579666,-16.957668859934,12.));
#220467=CARTESIAN_POINT('Ctrl Pts',(18.5282716744198,-16.9818106680382,
0.));
#220468=CARTESIAN_POINT('Ctrl Pts',(18.5282716744198,-16.9818106680382,
12.));
#220469=CARTESIAN_POINT('Ctrl Pts',(18.5376893576961,-17.0060468805099,
0.));
#220470=CARTESIAN_POINT('Ctrl Pts',(18.5376893576961,-17.0060468805099,
12.));
#220471=CARTESIAN_POINT('Ctrl Pts',(18.5470782182089,-17.030377148174,0.));
#220472=CARTESIAN_POINT('Ctrl Pts',(18.5470782182089,-17.030377148174,12.));
#220473=CARTESIAN_POINT('Ctrl Pts',(18.5564378489628,-17.0548011239751,
0.));
#220474=CARTESIAN_POINT('Ctrl Pts',(18.5564378489628,-17.0548011239751,
12.));
#220475=CARTESIAN_POINT('Ctrl Pts',(18.5657678479788,-17.0793184636079,
0.));
#220476=CARTESIAN_POINT('Ctrl Pts',(18.5657678479788,-17.0793184636079,
12.));
#220477=CARTESIAN_POINT('Ctrl Pts',(18.5750678188543,-17.1039288260002,
0.));
#220478=CARTESIAN_POINT('Ctrl Pts',(18.5750678188543,-17.1039288260002,
12.));
#220479=CARTESIAN_POINT('Ctrl Pts',(18.5843373717253,-17.1286318741185,
0.));
#220480=CARTESIAN_POINT('Ctrl Pts',(18.5843373717253,-17.1286318741185,
12.));
#220481=CARTESIAN_POINT('Ctrl Pts',(18.5935761222833,-17.1534272741646,
0.));
#220482=CARTESIAN_POINT('Ctrl Pts',(18.5935761222833,-17.1534272741646,
12.));
#220483=CARTESIAN_POINT('Ctrl Pts',(18.6027836898826,-17.1783146940131,
0.));
#220484=CARTESIAN_POINT('Ctrl Pts',(18.6027836898826,-17.1783146940131,
12.));
#220485=CARTESIAN_POINT('Ctrl Pts',(18.6119596959957,-17.2032938019288,
0.));
#220486=CARTESIAN_POINT('Ctrl Pts',(18.6119596959957,-17.2032938019288,
12.));
#220487=CARTESIAN_POINT('Ctrl Pts',(18.6211037624041,-17.2283642650519,
0.));
#220488=CARTESIAN_POINT('Ctrl Pts',(18.6211037624041,-17.2283642650519,
12.));
#220489=CARTESIAN_POINT('Ctrl Pts',(18.630215509794,-17.2535257482186,0.));
#220490=CARTESIAN_POINT('Ctrl Pts',(18.630215509794,-17.2535257482186,12.));
#220491=CARTESIAN_POINT('Ctrl Pts',(18.639294555474,-17.278777912021,0.));
#220492=CARTESIAN_POINT('Ctrl Pts',(18.639294555474,-17.278777912021,12.));
#220493=CARTESIAN_POINT('Ctrl Pts',(18.6483405141853,-17.3041204135069,
0.));
#220494=CARTESIAN_POINT('Ctrl Pts',(18.6483405141853,-17.3041204135069,
12.));
#220495=CARTESIAN_POINT('Ctrl Pts',(18.6573530024019,-17.3295529098612,
0.));
#220496=CARTESIAN_POINT('Ctrl Pts',(18.6573530024019,-17.3295529098612,
12.));
#220497=CARTESIAN_POINT('Ctrl Pts',(18.6663316416569,-17.3550750612438,
0.));
#220498=CARTESIAN_POINT('Ctrl Pts',(18.6663316416569,-17.3550750612438,
12.));
#220499=CARTESIAN_POINT('Ctrl Pts',(18.6752760624045,-17.3806865340744,
0.));
#220500=CARTESIAN_POINT('Ctrl Pts',(18.6752760624045,-17.3806865340744,
12.));
#220501=CARTESIAN_POINT('Ctrl Pts',(18.6841859073472,-17.4063870038563,
0.));
#220502=CARTESIAN_POINT('Ctrl Pts',(18.6841859073472,-17.4063870038563,
12.));
#220503=CARTESIAN_POINT('Ctrl Pts',(18.6930608357421,-17.4321761588148,
0.));
#220504=CARTESIAN_POINT('Ctrl Pts',(18.6930608357421,-17.4321761588148,
12.));
#220505=CARTESIAN_POINT('Ctrl Pts',(18.7019005250322,-17.4580537012764,
0.));
#220506=CARTESIAN_POINT('Ctrl Pts',(18.7019005250322,-17.4580537012764,
12.));
#220507=CARTESIAN_POINT('Ctrl Pts',(18.7107046613941,-17.4840193397176,
0.));
#220508=CARTESIAN_POINT('Ctrl Pts',(18.7107046613941,-17.4840193397176,
12.));
#220509=CARTESIAN_POINT('Ctrl Pts',(18.7194729318127,-17.5100727820891,
0.));
#220510=CARTESIAN_POINT('Ctrl Pts',(18.7194729318127,-17.5100727820891,
12.));
#220511=CARTESIAN_POINT('Ctrl Pts',(18.728205015716,-17.5362137287604,0.));
#220512=CARTESIAN_POINT('Ctrl Pts',(18.728205015716,-17.5362137287604,12.));
#220513=CARTESIAN_POINT('Ctrl Pts',(18.7369005764558,-17.5624418653248,
0.));
#220514=CARTESIAN_POINT('Ctrl Pts',(18.7369005764558,-17.5624418653248,
12.));
#220515=CARTESIAN_POINT('Ctrl Pts',(18.7455592536667,-17.5887568561361,
0.));
#220516=CARTESIAN_POINT('Ctrl Pts',(18.7455592536667,-17.5887568561361,
12.));
#220517=CARTESIAN_POINT('Ctrl Pts',(18.7541806530935,-17.6151583356989,
0.));
#220518=CARTESIAN_POINT('Ctrl Pts',(18.7541806530935,-17.6151583356989,
12.));
#220519=CARTESIAN_POINT('Ctrl Pts',(18.7627643613139,-17.6416459210646,
0.));
#220520=CARTESIAN_POINT('Ctrl Pts',(18.7627643613139,-17.6416459210646,
12.));
#220521=CARTESIAN_POINT('Ctrl Pts',(18.7713099642673,-17.6682192274197,
0.));
#220522=CARTESIAN_POINT('Ctrl Pts',(18.7713099642673,-17.6682192274197,
12.));
#220523=CARTESIAN_POINT('Ctrl Pts',(18.7798170641305,-17.6948778822982,
0.));
#220524=CARTESIAN_POINT('Ctrl Pts',(18.7798170641305,-17.6948778822982,
12.));
#220525=CARTESIAN_POINT('Ctrl Pts',(18.7882852976016,-17.7216215409019,
0.));
#220526=CARTESIAN_POINT('Ctrl Pts',(18.7882852976016,-17.7216215409019,
12.));
#220527=CARTESIAN_POINT('Ctrl Pts',(18.7967143519444,-17.7484498996916,
0.));
#220528=CARTESIAN_POINT('Ctrl Pts',(18.7967143519444,-17.7484498996916,
12.));
#220529=CARTESIAN_POINT('Ctrl Pts',(18.8051039860543,-17.7753627137898,
0.));
#220530=CARTESIAN_POINT('Ctrl Pts',(18.8051039860543,-17.7753627137898,
12.));
#220531=CARTESIAN_POINT('Ctrl Pts',(18.8134540340581,-17.8023598011135,
0.));
#220532=CARTESIAN_POINT('Ctrl Pts',(18.8134540340581,-17.8023598011135,
12.));
#220533=CARTESIAN_POINT('Ctrl Pts',(18.8217643886368,-17.8294410311105,
0.));
#220534=CARTESIAN_POINT('Ctrl Pts',(18.8217643886368,-17.8294410311105,
12.));
#220535=CARTESIAN_POINT('Ctrl Pts',(18.8300349896187,-17.8566063174871,
0.));
#220536=CARTESIAN_POINT('Ctrl Pts',(18.8300349896187,-17.8566063174871,
12.));
#220537=CARTESIAN_POINT('Ctrl Pts',(18.8366196462746,-17.8784057509434,
0.));
#220538=CARTESIAN_POINT('Ctrl Pts',(18.8366196462746,-17.8784057509434,
12.));
#220539=CARTESIAN_POINT('Ctrl Pts',(18.8415402351882,-17.8947931177853,
0.));
#220540=CARTESIAN_POINT('Ctrl Pts',(18.8415402351882,-17.8947931177853,
12.));
#220541=CARTESIAN_POINT('Ctrl Pts',(18.8448126709726,-17.9057348246611,
0.));
#220542=CARTESIAN_POINT('Ctrl Pts',(18.8448126709726,-17.9057348246611,
12.));
#220543=CARTESIAN_POINT('Ctrl Pts',(18.8464468996588,-17.9112098770111,
0.));
#220544=CARTESIAN_POINT('Ctrl Pts',(18.8464468996588,-17.9112098770111,
12.));
#220545=CARTESIAN_POINT('',(18.8464468996588,-17.9112098770111,0.));
#220546=CARTESIAN_POINT('Ctrl Pts',(17.1452095830632,-14.6513681262571,
0.));
#220547=CARTESIAN_POINT('Ctrl Pts',(17.1452153999142,-14.6513711852843,
0.));
#220548=CARTESIAN_POINT('Ctrl Pts',(17.1452600887037,-14.6514066997196,
0.));
#220549=CARTESIAN_POINT('Ctrl Pts',(17.1454262858043,-14.6515481598068,
0.));
#220550=CARTESIAN_POINT('Ctrl Pts',(17.1458462295271,-14.6519131634508,
0.));
#220551=CARTESIAN_POINT('Ctrl Pts',(17.1466998098673,-14.6526624064978,
0.));
#220552=CARTESIAN_POINT('Ctrl Pts',(17.147876394491,-14.6537016966184,0.));
#220553=CARTESIAN_POINT('Ctrl Pts',(17.1493641837558,-14.655024862281,0.));
#220554=CARTESIAN_POINT('Ctrl Pts',(17.1511476869496,-14.6566237952435,
0.));
#220555=CARTESIAN_POINT('Ctrl Pts',(17.1532107762718,-14.6584900555302,
0.));
#220556=CARTESIAN_POINT('Ctrl Pts',(17.1555401986401,-14.6606167169642,
0.));
#220557=CARTESIAN_POINT('Ctrl Pts',(17.1581262646789,-14.6629987285992,
0.));
#220558=CARTESIAN_POINT('Ctrl Pts',(17.1609609517369,-14.6656319165057,
0.));
#220559=CARTESIAN_POINT('Ctrl Pts',(17.1640366762305,-14.6685123374423,
0.));
#220560=CARTESIAN_POINT('Ctrl Pts',(17.167344972302,-14.671635583332,0.));
#220561=CARTESIAN_POINT('Ctrl Pts',(17.1708771619129,-14.6749971333867,
0.));
#220562=CARTESIAN_POINT('Ctrl Pts',(17.1746247499057,-14.6785925615677,
0.));
#220563=CARTESIAN_POINT('Ctrl Pts',(17.1785800350826,-14.6824178576167,
0.));
#220564=CARTESIAN_POINT('Ctrl Pts',(17.182736158472,-14.686469452232,0.));
#220565=CARTESIAN_POINT('Ctrl Pts',(17.1870867909918,-14.6907440526958,
0.));
#220566=CARTESIAN_POINT('Ctrl Pts',(17.1916259308415,-14.6952385361706,
0.));
#220567=CARTESIAN_POINT('Ctrl Pts',(17.1963476411694,-14.699949811582,0.));
#220568=CARTESIAN_POINT('Ctrl Pts',(17.2012461084268,-14.7048748502663,
0.));
#220569=CARTESIAN_POINT('Ctrl Pts',(17.2063157097315,-14.7100107213586,
0.));
#220570=CARTESIAN_POINT('Ctrl Pts',(17.2115510835989,-14.7153546289339,
0.));
#220571=CARTESIAN_POINT('Ctrl Pts',(17.2169471814256,-14.7209039390327,
0.));
#220572=CARTESIAN_POINT('Ctrl Pts',(17.2224992099667,-14.7266561494282,
0.));
#220573=CARTESIAN_POINT('Ctrl Pts',(17.2282025904314,-14.7326088681163,
0.));
#220574=CARTESIAN_POINT('Ctrl Pts',(17.2340529062076,-14.7387597858117,
0.));
#220575=CARTESIAN_POINT('Ctrl Pts',(17.2400458713565,-14.7451066593792,
0.));
#220576=CARTESIAN_POINT('Ctrl Pts',(17.2461773413288,-14.7516473175124,
0.));
#220577=CARTESIAN_POINT('Ctrl Pts',(17.2524433146837,-14.7583796616617,
0.));
#220578=CARTESIAN_POINT('Ctrl Pts',(17.2588399401465,-14.7653016697591,
0.));
#220579=CARTESIAN_POINT('Ctrl Pts',(17.2653635155319,-14.7724113956731,
0.));
#220580=CARTESIAN_POINT('Ctrl Pts',(17.2720104735194,-14.7797069617804,
0.));
#220581=CARTESIAN_POINT('Ctrl Pts',(17.2787773704849,-14.787186553128,0.));
#220582=CARTESIAN_POINT('Ctrl Pts',(17.2856608733196,-14.7948484105249,
0.));
#220583=CARTESIAN_POINT('Ctrl Pts',(17.2926577496513,-14.8026908254276,
0.));
#220584=CARTESIAN_POINT('Ctrl Pts',(17.299764866148,-14.8107121391035,0.));
#220585=CARTESIAN_POINT('Ctrl Pts',(17.3069791853706,-14.8189107410162,
0.));
#220586=CARTESIAN_POINT('Ctrl Pts',(17.3142977632659,-14.8272850675379,
0.));
#220587=CARTESIAN_POINT('Ctrl Pts',(17.3217177462101,-14.8358336004197,
0.));
#220588=CARTESIAN_POINT('Ctrl Pts',(17.3292363662605,-14.8445548643508,
0.));
#220589=CARTESIAN_POINT('Ctrl Pts',(17.336850936485,-14.8534474245434,0.));
#220590=CARTESIAN_POINT('Ctrl Pts',(17.3445588463474,-14.8625098843417,
0.));
#220591=CARTESIAN_POINT('Ctrl Pts',(17.3523575568645,-14.8717408826956,
0.));
#220592=CARTESIAN_POINT('Ctrl Pts',(17.3602445978161,-14.8811390927423,
0.));
#220593=CARTESIAN_POINT('Ctrl Pts',(17.3682175653235,-14.8907032205788,
0.));
#220594=CARTESIAN_POINT('Ctrl Pts',(17.3762741193076,-14.900432003961,0.));
#220595=CARTESIAN_POINT('Ctrl Pts',(17.3844119809824,-14.9103242110057,
0.));
#220596=CARTESIAN_POINT('Ctrl Pts',(17.3926289303986,-14.9203786389342,
0.));
#220597=CARTESIAN_POINT('Ctrl Pts',(17.4009228040749,-14.9305941128757,
0.));
#220598=CARTESIAN_POINT('Ctrl Pts',(17.4092914926071,-14.940969484645,0.));
#220599=CARTESIAN_POINT('Ctrl Pts',(17.4177329382828,-14.9515036315143,
0.));
#220600=CARTESIAN_POINT('Ctrl Pts',(17.426245132709,-14.9621954549827,0.));
#220601=CARTESIAN_POINT('Ctrl Pts',(17.4348261151396,-14.9730438799452,
0.));
#220602=CARTESIAN_POINT('Ctrl Pts',(17.4434739707773,-14.9840478538358,
0.));
#220603=CARTESIAN_POINT('Ctrl Pts',(17.4521868291004,-14.9952063457778,
0.));
#220604=CARTESIAN_POINT('Ctrl Pts',(17.4609628621418,-15.0065183456921,
0.));
#220605=CARTESIAN_POINT('Ctrl Pts',(17.4698002829357,-15.0179828635086,
0.));
#220606=CARTESIAN_POINT('Ctrl Pts',(17.4786973441417,-15.029598928488,0.));
#220607=CARTESIAN_POINT('Ctrl Pts',(17.4876523366178,-15.0413655884993,
0.));
#220608=CARTESIAN_POINT('Ctrl Pts',(17.4966635880245,-15.0532819093085,
0.));
#220609=CARTESIAN_POINT('Ctrl Pts',(17.5057294613874,-15.0653469738306,
0.));
#220610=CARTESIAN_POINT('Ctrl Pts',(17.5148483539683,-15.0775598815748,
0.));
#220611=CARTESIAN_POINT('Ctrl Pts',(17.5240186961788,-15.0899197481082,
0.));
#220612=CARTESIAN_POINT('Ctrl Pts',(17.5332389504829,-15.1024257045033,
0.));
#220613=CARTESIAN_POINT('Ctrl Pts',(17.5425076102966,-15.1150768967729,
0.));
#220614=CARTESIAN_POINT('Ctrl Pts',(17.5518231989122,-15.127872485314,0.));
#220615=CARTESIAN_POINT('Ctrl Pts',(17.5611842686196,-15.1408116444877,
0.));
#220616=CARTESIAN_POINT('Ctrl Pts',(17.570589399803,-15.1538935621715,0.));
#220617=CARTESIAN_POINT('Ctrl Pts',(17.5800372000539,-15.1671174393136,
0.));
#220618=CARTESIAN_POINT('Ctrl Pts',(17.5895263032592,-15.1804824894605,
0.));
#220619=CARTESIAN_POINT('Ctrl Pts',(17.5990553687595,-15.1939879383268,
0.));
#220620=CARTESIAN_POINT('Ctrl Pts',(17.6086230806497,-15.2076330234686,
0.));
#220621=CARTESIAN_POINT('Ctrl Pts',(17.6182281470467,-15.22141699392,0.));
#220622=CARTESIAN_POINT('Ctrl Pts',(17.6278692993765,-15.2353391098367,
0.));
#220623=CARTESIAN_POINT('Ctrl Pts',(17.637545291637,-15.2493986421091,0.));
#220624=CARTESIAN_POINT('Ctrl Pts',(17.6472548997329,-15.263594872029,0.));
#220625=CARTESIAN_POINT('Ctrl Pts',(17.6569969209,-15.2779270910238,0.));
#220626=CARTESIAN_POINT('Ctrl Pts',(17.6667701731041,-15.2923946003598,
0.));
#220627=CARTESIAN_POINT('Ctrl Pts',(17.6765734944559,-15.3069967108501,
0.));
#220628=CARTESIAN_POINT('Ctrl Pts',(17.6864057426052,-15.3217327425341,
0.));
#220629=CARTESIAN_POINT('Ctrl Pts',(17.6962657941984,-15.3366020244069,
0.));
#220630=CARTESIAN_POINT('Ctrl Pts',(17.7061525444044,-15.3516038942064,
0.));
#220631=CARTESIAN_POINT('Ctrl Pts',(17.7160649064208,-15.3667376981702,
0.));
#220632=CARTESIAN_POINT('Ctrl Pts',(17.7260018109923,-15.3820027907965,
0.));
#220633=CARTESIAN_POINT('Ctrl Pts',(17.7359622059143,-15.3973985345796,
0.));
#220634=CARTESIAN_POINT('Ctrl Pts',(17.7459450555803,-15.4129242997828,
0.));
#220635=CARTESIAN_POINT('Ctrl Pts',(17.7559493405871,-15.4285794642658,
0.));
#220636=CARTESIAN_POINT('Ctrl Pts',(17.765974057326,-15.4443634132865,0.));
#220637=CARTESIAN_POINT('Ctrl Pts',(17.7760182175817,-15.4602755393019,
0.));
#220638=CARTESIAN_POINT('Ctrl Pts',(17.7860808481229,-15.4763152417506,
0.));
#220639=CARTESIAN_POINT('Ctrl Pts',(17.7961609903161,-15.4924819268529,
0.));
#220640=CARTESIAN_POINT('Ctrl Pts',(17.8062576997964,-15.5087750074728,
0.));
#220641=CARTESIAN_POINT('Ctrl Pts',(17.8163700461263,-15.5251939029558,
0.));
#220642=CARTESIAN_POINT('Ctrl Pts',(17.8264971124606,-15.5417380389639,
0.));
#220643=CARTESIAN_POINT('Ctrl Pts',(17.8366379952078,-15.5584068472976,
0.));
#220644=CARTESIAN_POINT('Ctrl Pts',(17.8467918036976,-15.5751997657153,
0.));
#220645=CARTESIAN_POINT('Ctrl Pts',(17.8569576598996,-15.5921162378183,
0.));
#220646=CARTESIAN_POINT('Ctrl Pts',(17.8671346981388,-15.6091557129205,
0.));
#220647=CARTESIAN_POINT('Ctrl Pts',(17.8773220648125,-15.6263176459107,
0.));
#220648=CARTESIAN_POINT('Ctrl Pts',(17.8875189181095,-15.6436014971088,
0.));
#220649=CARTESIAN_POINT('Ctrl Pts',(17.8977244277247,-15.6610067321036,
0.));
#220650=CARTESIAN_POINT('Ctrl Pts',(17.9079377746118,-15.6785328216467,
0.));
#220651=CARTESIAN_POINT('Ctrl Pts',(17.918158150746,-15.6961792415526,0.));
#220652=CARTESIAN_POINT('Ctrl Pts',(17.9283847588837,-15.713945472584,0.));
#220653=CARTESIAN_POINT('Ctrl Pts',(17.9386168123261,-15.7318310003334,
0.));
#220654=CARTESIAN_POINT('Ctrl Pts',(17.9488535346776,-15.7498353150856,
0.));
#220655=CARTESIAN_POINT('Ctrl Pts',(17.9590941596236,-15.7679579117072,
0.));
#220656=CARTESIAN_POINT('Ctrl Pts',(17.9693379307297,-15.786198289572,0.));
#220657=CARTESIAN_POINT('Ctrl Pts',(17.9795841012383,-15.8045559524674,
0.));
#220658=CARTESIAN_POINT('Ctrl Pts',(17.9898319338664,-15.8230304084963,
0.));
#220659=CARTESIAN_POINT('Ctrl Pts',(18.0000807006055,-15.8416211699682,
0.));
#220660=CARTESIAN_POINT('Ctrl Pts',(18.010329682521,-15.8603277532834,0.));
#220661=CARTESIAN_POINT('Ctrl Pts',(18.0205781695773,-15.8791496788685,
0.));
#220662=CARTESIAN_POINT('Ctrl Pts',(18.0308254604638,-15.8980864711043,
0.));
#220663=CARTESIAN_POINT('Ctrl Pts',(18.0410708624208,-15.9171376582436,
0.));
#220664=CARTESIAN_POINT('Ctrl Pts',(18.0513136910691,-15.9363027723244,
0.));
#220665=CARTESIAN_POINT('Ctrl Pts',(18.061553270236,-15.9555813490645,0.));
#220666=CARTESIAN_POINT('Ctrl Pts',(18.071788931796,-15.9749729277848,0.));
#220667=CARTESIAN_POINT('Ctrl Pts',(18.0820200155239,-15.9944770513616,
0.));
#220668=CARTESIAN_POINT('Ctrl Pts',(18.0922458689464,-16.0140932661612,
0.));
#220669=CARTESIAN_POINT('Ctrl Pts',(18.1024658471966,-16.0338211219694,
0.));
#220670=CARTESIAN_POINT('Ctrl Pts',(18.1126793128688,-16.0536601719124,
0.));
#220671=CARTESIAN_POINT('Ctrl Pts',(18.1228856358746,-16.0736099723664,
0.));
#220672=CARTESIAN_POINT('Ctrl Pts',(18.1330841933099,-16.0936700829108,
0.));
#220673=CARTESIAN_POINT('Ctrl Pts',(18.1432743693231,-16.113840066279,0.));
#220674=CARTESIAN_POINT('Ctrl Pts',(18.153455554985,-16.1341194882987,0.));
#220675=CARTESIAN_POINT('Ctrl Pts',(18.1636271481616,-16.1545079178261,
0.));
#220676=CARTESIAN_POINT('Ctrl Pts',(18.1737885533852,-16.1750049266673,
0.));
#220677=CARTESIAN_POINT('Ctrl Pts',(18.1839391817335,-16.1956100895076,
0.));
#220678=CARTESIAN_POINT('Ctrl Pts',(18.1940784507232,-16.2163229838878,
0.));
#220679=CARTESIAN_POINT('Ctrl Pts',(18.2042057842037,-16.237143190164,0.));
#220680=CARTESIAN_POINT('Ctrl Pts',(18.214320612253,-16.2580702914615,0.));
#220681=CARTESIAN_POINT('Ctrl Pts',(18.2244223710745,-16.2791038736223,
0.));
#220682=CARTESIAN_POINT('Ctrl Pts',(18.2345105028981,-16.3002435251378,
0.));
#220683=CARTESIAN_POINT('Ctrl Pts',(18.2445844558742,-16.3214888370988,
0.));
#220684=CARTESIAN_POINT('Ctrl Pts',(18.2546436839609,-16.342839403159,0.));
#220685=CARTESIAN_POINT('Ctrl Pts',(18.2646876468169,-16.3642948194869,
0.));
#220686=CARTESIAN_POINT('Ctrl Pts',(18.2747158096934,-16.385854684708,0.));
#220687=CARTESIAN_POINT('Ctrl Pts',(18.2847276433308,-16.4075185998454,
0.));
#220688=CARTESIAN_POINT('Ctrl Pts',(18.2947226238509,-16.4292861682377,
0.));
#220689=CARTESIAN_POINT('Ctrl Pts',(18.3047002326858,-16.4511569955231,
0.));
#220690=CARTESIAN_POINT('Ctrl Pts',(18.3146599565229,-16.4731306896439,
0.));
#220691=CARTESIAN_POINT('Ctrl Pts',(18.3246012872468,-16.4952068608344,
0.));
#220692=CARTESIAN_POINT('Ctrl Pts',(18.3345237218864,-16.5173851216045,
0.));
#220693=CARTESIAN_POINT('Ctrl Pts',(18.3444267625601,-16.5396650867139,
0.));
#220694=CARTESIAN_POINT('Ctrl Pts',(18.3543099164331,-16.5620463731414,
0.));
#220695=CARTESIAN_POINT('Ctrl Pts',(18.364172695589,-16.5845286000218,0.));
#220696=CARTESIAN_POINT('Ctrl Pts',(18.3740146168879,-16.6071113885711,
0.));
#220697=CARTESIAN_POINT('Ctrl Pts',(18.3838352018327,-16.6297943620056,
0.));
#220698=CARTESIAN_POINT('Ctrl Pts',(18.3936339764332,-16.6525771454513,
0.));
#220699=CARTESIAN_POINT('Ctrl Pts',(18.4034104710789,-16.6754593658513,
0.));
#220700=CARTESIAN_POINT('Ctrl Pts',(18.4131642203989,-16.698440651849,0.));
#220701=CARTESIAN_POINT('Ctrl Pts',(18.4228947633186,-16.7215206338818,
0.));
#220702=CARTESIAN_POINT('Ctrl Pts',(18.4326016431392,-16.7446989442882,
0.));
#220703=CARTESIAN_POINT('Ctrl Pts',(18.4422844076099,-16.7679752173992,
0.));
#220704=CARTESIAN_POINT('Ctrl Pts',(18.4519426090124,-16.791349089629,0.));
#220705=CARTESIAN_POINT('Ctrl Pts',(18.4615758042305,-16.8148201995472,
0.));
#220706=CARTESIAN_POINT('Ctrl Pts',(18.4711835548622,-16.8383881879707,
0.));
#220707=CARTESIAN_POINT('Ctrl Pts',(18.4807654268769,-16.8620526977169,
0.));
#220708=CARTESIAN_POINT('Ctrl Pts',(18.4903209902226,-16.8858133733086,
0.));
#220709=CARTESIAN_POINT('Ctrl Pts',(18.4998498184619,-16.9096698606942,
0.));
#220710=CARTESIAN_POINT('Ctrl Pts',(18.5093514883835,-16.9336218069353,
0.));
#220711=CARTESIAN_POINT('Ctrl Pts',(18.518825579666,-16.957668859934,0.));
#220712=CARTESIAN_POINT('Ctrl Pts',(18.5282716744198,-16.9818106680382,
0.));
#220713=CARTESIAN_POINT('Ctrl Pts',(18.5376893576961,-17.0060468805099,
0.));
#220714=CARTESIAN_POINT('Ctrl Pts',(18.5470782182089,-17.030377148174,0.));
#220715=CARTESIAN_POINT('Ctrl Pts',(18.5564378489628,-17.0548011239751,
0.));
#220716=CARTESIAN_POINT('Ctrl Pts',(18.5657678479788,-17.0793184636079,
0.));
#220717=CARTESIAN_POINT('Ctrl Pts',(18.5750678188543,-17.1039288260002,
0.));
#220718=CARTESIAN_POINT('Ctrl Pts',(18.5843373717253,-17.1286318741185,
0.));
#220719=CARTESIAN_POINT('Ctrl Pts',(18.5935761222833,-17.1534272741646,
0.));
#220720=CARTESIAN_POINT('Ctrl Pts',(18.6027836898826,-17.1783146940131,
0.));
#220721=CARTESIAN_POINT('Ctrl Pts',(18.6119596959957,-17.2032938019288,
0.));
#220722=CARTESIAN_POINT('Ctrl Pts',(18.6211037624041,-17.2283642650519,
0.));
#220723=CARTESIAN_POINT('Ctrl Pts',(18.630215509794,-17.2535257482186,0.));
#220724=CARTESIAN_POINT('Ctrl Pts',(18.639294555474,-17.278777912021,0.));
#220725=CARTESIAN_POINT('Ctrl Pts',(18.6483405141853,-17.3041204135069,
0.));
#220726=CARTESIAN_POINT('Ctrl Pts',(18.6573530024019,-17.3295529098612,
0.));
#220727=CARTESIAN_POINT('Ctrl Pts',(18.6663316416569,-17.3550750612438,
0.));
#220728=CARTESIAN_POINT('Ctrl Pts',(18.6752760624045,-17.3806865340744,
0.));
#220729=CARTESIAN_POINT('Ctrl Pts',(18.6841859073472,-17.4063870038563,
0.));
#220730=CARTESIAN_POINT('Ctrl Pts',(18.6930608357421,-17.4321761588148,
0.));
#220731=CARTESIAN_POINT('Ctrl Pts',(18.7019005250322,-17.4580537012764,
0.));
#220732=CARTESIAN_POINT('Ctrl Pts',(18.7107046613941,-17.4840193397176,
0.));
#220733=CARTESIAN_POINT('Ctrl Pts',(18.7194729318127,-17.5100727820891,
0.));
#220734=CARTESIAN_POINT('Ctrl Pts',(18.728205015716,-17.5362137287604,0.));
#220735=CARTESIAN_POINT('Ctrl Pts',(18.7369005764558,-17.5624418653248,
0.));
#220736=CARTESIAN_POINT('Ctrl Pts',(18.7455592536667,-17.5887568561361,
0.));
#220737=CARTESIAN_POINT('Ctrl Pts',(18.7541806530935,-17.6151583356989,
0.));
#220738=CARTESIAN_POINT('Ctrl Pts',(18.7627643613139,-17.6416459210646,
0.));
#220739=CARTESIAN_POINT('Ctrl Pts',(18.7713099642673,-17.6682192274197,
0.));
#220740=CARTESIAN_POINT('Ctrl Pts',(18.7798170641305,-17.6948778822982,
0.));
#220741=CARTESIAN_POINT('Ctrl Pts',(18.7882852976016,-17.7216215409019,
0.));
#220742=CARTESIAN_POINT('Ctrl Pts',(18.7967143519444,-17.7484498996916,
0.));
#220743=CARTESIAN_POINT('Ctrl Pts',(18.8051039860543,-17.7753627137898,
0.));
#220744=CARTESIAN_POINT('Ctrl Pts',(18.8134540340581,-17.8023598011135,
0.));
#220745=CARTESIAN_POINT('Ctrl Pts',(18.8217643886368,-17.8294410311105,
0.));
#220746=CARTESIAN_POINT('Ctrl Pts',(18.8300349896187,-17.8566063174871,
0.));
#220747=CARTESIAN_POINT('Ctrl Pts',(18.8366196462746,-17.8784057509434,
0.));
#220748=CARTESIAN_POINT('Ctrl Pts',(18.8415402351882,-17.8947931177853,
0.));
#220749=CARTESIAN_POINT('Ctrl Pts',(18.8448126709726,-17.9057348246611,
0.));
#220750=CARTESIAN_POINT('Ctrl Pts',(18.8464468996588,-17.9112098770111,
0.));
#220751=CARTESIAN_POINT('',(18.8464468996588,-17.9112098770111,12.));
#220752=CARTESIAN_POINT('Ctrl Pts',(18.8464468996588,-17.9112098770111,
12.));
#220753=CARTESIAN_POINT('Ctrl Pts',(18.8448126709726,-17.9057348246611,
12.));
#220754=CARTESIAN_POINT('Ctrl Pts',(18.8415402351882,-17.8947931177853,
12.));
#220755=CARTESIAN_POINT('Ctrl Pts',(18.8366196462746,-17.8784057509434,
12.));
#220756=CARTESIAN_POINT('Ctrl Pts',(18.8300349896187,-17.8566063174871,
12.));
#220757=CARTESIAN_POINT('Ctrl Pts',(18.8217643886368,-17.8294410311105,
12.));
#220758=CARTESIAN_POINT('Ctrl Pts',(18.8134540340581,-17.8023598011135,
12.));
#220759=CARTESIAN_POINT('Ctrl Pts',(18.8051039860543,-17.7753627137898,
12.));
#220760=CARTESIAN_POINT('Ctrl Pts',(18.7967143519444,-17.7484498996916,
12.));
#220761=CARTESIAN_POINT('Ctrl Pts',(18.7882852976016,-17.7216215409019,
12.));
#220762=CARTESIAN_POINT('Ctrl Pts',(18.7798170641305,-17.6948778822982,
12.));
#220763=CARTESIAN_POINT('Ctrl Pts',(18.7713099642673,-17.6682192274197,
12.));
#220764=CARTESIAN_POINT('Ctrl Pts',(18.7627643613139,-17.6416459210646,
12.));
#220765=CARTESIAN_POINT('Ctrl Pts',(18.7541806530935,-17.6151583356989,
12.));
#220766=CARTESIAN_POINT('Ctrl Pts',(18.7455592536667,-17.5887568561361,
12.));
#220767=CARTESIAN_POINT('Ctrl Pts',(18.7369005764558,-17.5624418653248,
12.));
#220768=CARTESIAN_POINT('Ctrl Pts',(18.728205015716,-17.5362137287604,12.));
#220769=CARTESIAN_POINT('Ctrl Pts',(18.7194729318127,-17.5100727820891,
12.));
#220770=CARTESIAN_POINT('Ctrl Pts',(18.7107046613941,-17.4840193397176,
12.));
#220771=CARTESIAN_POINT('Ctrl Pts',(18.7019005250322,-17.4580537012764,
12.));
#220772=CARTESIAN_POINT('Ctrl Pts',(18.6930608357421,-17.4321761588148,
12.));
#220773=CARTESIAN_POINT('Ctrl Pts',(18.6841859073472,-17.4063870038563,
12.));
#220774=CARTESIAN_POINT('Ctrl Pts',(18.6752760624045,-17.3806865340744,
12.));
#220775=CARTESIAN_POINT('Ctrl Pts',(18.6663316416569,-17.3550750612438,
12.));
#220776=CARTESIAN_POINT('Ctrl Pts',(18.6573530024019,-17.3295529098612,
12.));
#220777=CARTESIAN_POINT('Ctrl Pts',(18.6483405141853,-17.3041204135069,
12.));
#220778=CARTESIAN_POINT('Ctrl Pts',(18.639294555474,-17.278777912021,12.));
#220779=CARTESIAN_POINT('Ctrl Pts',(18.630215509794,-17.2535257482186,12.));
#220780=CARTESIAN_POINT('Ctrl Pts',(18.6211037624041,-17.2283642650519,
12.));
#220781=CARTESIAN_POINT('Ctrl Pts',(18.6119596959957,-17.2032938019288,
12.));
#220782=CARTESIAN_POINT('Ctrl Pts',(18.6027836898826,-17.1783146940131,
12.));
#220783=CARTESIAN_POINT('Ctrl Pts',(18.5935761222833,-17.1534272741646,
12.));
#220784=CARTESIAN_POINT('Ctrl Pts',(18.5843373717253,-17.1286318741185,
12.));
#220785=CARTESIAN_POINT('Ctrl Pts',(18.5750678188543,-17.1039288260002,
12.));
#220786=CARTESIAN_POINT('Ctrl Pts',(18.5657678479788,-17.0793184636079,
12.));
#220787=CARTESIAN_POINT('Ctrl Pts',(18.5564378489628,-17.0548011239751,
12.));
#220788=CARTESIAN_POINT('Ctrl Pts',(18.5470782182089,-17.030377148174,12.));
#220789=CARTESIAN_POINT('Ctrl Pts',(18.5376893576961,-17.0060468805099,
12.));
#220790=CARTESIAN_POINT('Ctrl Pts',(18.5282716744198,-16.9818106680382,
12.));
#220791=CARTESIAN_POINT('Ctrl Pts',(18.518825579666,-16.957668859934,12.));
#220792=CARTESIAN_POINT('Ctrl Pts',(18.5093514883835,-16.9336218069353,
12.));
#220793=CARTESIAN_POINT('Ctrl Pts',(18.4998498184619,-16.9096698606942,
12.));
#220794=CARTESIAN_POINT('Ctrl Pts',(18.4903209902226,-16.8858133733086,
12.));
#220795=CARTESIAN_POINT('Ctrl Pts',(18.4807654268769,-16.8620526977169,
12.));
#220796=CARTESIAN_POINT('Ctrl Pts',(18.4711835548622,-16.8383881879707,
12.));
#220797=CARTESIAN_POINT('Ctrl Pts',(18.4615758042305,-16.8148201995472,
12.));
#220798=CARTESIAN_POINT('Ctrl Pts',(18.4519426090124,-16.791349089629,12.));
#220799=CARTESIAN_POINT('Ctrl Pts',(18.4422844076099,-16.7679752173992,
12.));
#220800=CARTESIAN_POINT('Ctrl Pts',(18.4326016431392,-16.7446989442882,
12.));
#220801=CARTESIAN_POINT('Ctrl Pts',(18.4228947633186,-16.7215206338818,
12.));
#220802=CARTESIAN_POINT('Ctrl Pts',(18.4131642203989,-16.698440651849,12.));
#220803=CARTESIAN_POINT('Ctrl Pts',(18.4034104710789,-16.6754593658513,
12.));
#220804=CARTESIAN_POINT('Ctrl Pts',(18.3936339764332,-16.6525771454513,
12.));
#220805=CARTESIAN_POINT('Ctrl Pts',(18.3838352018327,-16.6297943620056,
12.));
#220806=CARTESIAN_POINT('Ctrl Pts',(18.3740146168879,-16.6071113885711,
12.));
#220807=CARTESIAN_POINT('Ctrl Pts',(18.364172695589,-16.5845286000218,12.));
#220808=CARTESIAN_POINT('Ctrl Pts',(18.3543099164331,-16.5620463731414,
12.));
#220809=CARTESIAN_POINT('Ctrl Pts',(18.3444267625601,-16.5396650867139,
12.));
#220810=CARTESIAN_POINT('Ctrl Pts',(18.3345237218864,-16.5173851216045,
12.));
#220811=CARTESIAN_POINT('Ctrl Pts',(18.3246012872468,-16.4952068608344,
12.));
#220812=CARTESIAN_POINT('Ctrl Pts',(18.3146599565229,-16.4731306896439,
12.));
#220813=CARTESIAN_POINT('Ctrl Pts',(18.3047002326858,-16.4511569955231,
12.));
#220814=CARTESIAN_POINT('Ctrl Pts',(18.2947226238509,-16.4292861682377,
12.));
#220815=CARTESIAN_POINT('Ctrl Pts',(18.2847276433308,-16.4075185998454,
12.));
#220816=CARTESIAN_POINT('Ctrl Pts',(18.2747158096934,-16.385854684708,12.));
#220817=CARTESIAN_POINT('Ctrl Pts',(18.2646876468169,-16.3642948194869,
12.));
#220818=CARTESIAN_POINT('Ctrl Pts',(18.2546436839609,-16.342839403159,12.));
#220819=CARTESIAN_POINT('Ctrl Pts',(18.2445844558742,-16.3214888370988,
12.));
#220820=CARTESIAN_POINT('Ctrl Pts',(18.2345105028981,-16.3002435251378,
12.));
#220821=CARTESIAN_POINT('Ctrl Pts',(18.2244223710745,-16.2791038736223,
12.));
#220822=CARTESIAN_POINT('Ctrl Pts',(18.214320612253,-16.2580702914615,12.));
#220823=CARTESIAN_POINT('Ctrl Pts',(18.2042057842037,-16.237143190164,12.));
#220824=CARTESIAN_POINT('Ctrl Pts',(18.1940784507232,-16.2163229838878,
12.));
#220825=CARTESIAN_POINT('Ctrl Pts',(18.1839391817335,-16.1956100895076,
12.));
#220826=CARTESIAN_POINT('Ctrl Pts',(18.1737885533852,-16.1750049266673,
12.));
#220827=CARTESIAN_POINT('Ctrl Pts',(18.1636271481616,-16.1545079178261,
12.));
#220828=CARTESIAN_POINT('Ctrl Pts',(18.153455554985,-16.1341194882987,12.));
#220829=CARTESIAN_POINT('Ctrl Pts',(18.1432743693231,-16.113840066279,12.));
#220830=CARTESIAN_POINT('Ctrl Pts',(18.1330841933099,-16.0936700829108,
12.));
#220831=CARTESIAN_POINT('Ctrl Pts',(18.1228856358746,-16.0736099723664,
12.));
#220832=CARTESIAN_POINT('Ctrl Pts',(18.1126793128688,-16.0536601719124,
12.));
#220833=CARTESIAN_POINT('Ctrl Pts',(18.1024658471966,-16.0338211219694,
12.));
#220834=CARTESIAN_POINT('Ctrl Pts',(18.0922458689464,-16.0140932661612,
12.));
#220835=CARTESIAN_POINT('Ctrl Pts',(18.0820200155239,-15.9944770513616,
12.));
#220836=CARTESIAN_POINT('Ctrl Pts',(18.071788931796,-15.9749729277848,12.));
#220837=CARTESIAN_POINT('Ctrl Pts',(18.061553270236,-15.9555813490645,12.));
#220838=CARTESIAN_POINT('Ctrl Pts',(18.0513136910691,-15.9363027723244,
12.));
#220839=CARTESIAN_POINT('Ctrl Pts',(18.0410708624208,-15.9171376582436,
12.));
#220840=CARTESIAN_POINT('Ctrl Pts',(18.0308254604638,-15.8980864711043,
12.));
#220841=CARTESIAN_POINT('Ctrl Pts',(18.0205781695773,-15.8791496788685,
12.));
#220842=CARTESIAN_POINT('Ctrl Pts',(18.010329682521,-15.8603277532834,12.));
#220843=CARTESIAN_POINT('Ctrl Pts',(18.0000807006055,-15.8416211699682,
12.));
#220844=CARTESIAN_POINT('Ctrl Pts',(17.9898319338664,-15.8230304084963,
12.));
#220845=CARTESIAN_POINT('Ctrl Pts',(17.9795841012383,-15.8045559524674,
12.));
#220846=CARTESIAN_POINT('Ctrl Pts',(17.9693379307297,-15.786198289572,12.));
#220847=CARTESIAN_POINT('Ctrl Pts',(17.9590941596236,-15.7679579117072,
12.));
#220848=CARTESIAN_POINT('Ctrl Pts',(17.9488535346776,-15.7498353150856,
12.));
#220849=CARTESIAN_POINT('Ctrl Pts',(17.9386168123261,-15.7318310003334,
12.));
#220850=CARTESIAN_POINT('Ctrl Pts',(17.9283847588837,-15.713945472584,12.));
#220851=CARTESIAN_POINT('Ctrl Pts',(17.918158150746,-15.6961792415526,12.));
#220852=CARTESIAN_POINT('Ctrl Pts',(17.9079377746118,-15.6785328216467,
12.));
#220853=CARTESIAN_POINT('Ctrl Pts',(17.8977244277247,-15.6610067321036,
12.));
#220854=CARTESIAN_POINT('Ctrl Pts',(17.8875189181095,-15.6436014971088,
12.));
#220855=CARTESIAN_POINT('Ctrl Pts',(17.8773220648125,-15.6263176459107,
12.));
#220856=CARTESIAN_POINT('Ctrl Pts',(17.8671346981388,-15.6091557129205,
12.));
#220857=CARTESIAN_POINT('Ctrl Pts',(17.8569576598996,-15.5921162378183,
12.));
#220858=CARTESIAN_POINT('Ctrl Pts',(17.8467918036976,-15.5751997657153,
12.));
#220859=CARTESIAN_POINT('Ctrl Pts',(17.8366379952078,-15.5584068472976,
12.));
#220860=CARTESIAN_POINT('Ctrl Pts',(17.8264971124606,-15.5417380389639,
12.));
#220861=CARTESIAN_POINT('Ctrl Pts',(17.8163700461263,-15.5251939029558,
12.));
#220862=CARTESIAN_POINT('Ctrl Pts',(17.8062576997964,-15.5087750074728,
12.));
#220863=CARTESIAN_POINT('Ctrl Pts',(17.7961609903161,-15.4924819268529,
12.));
#220864=CARTESIAN_POINT('Ctrl Pts',(17.7860808481229,-15.4763152417506,
12.));
#220865=CARTESIAN_POINT('Ctrl Pts',(17.7760182175817,-15.4602755393019,
12.));
#220866=CARTESIAN_POINT('Ctrl Pts',(17.765974057326,-15.4443634132865,12.));
#220867=CARTESIAN_POINT('Ctrl Pts',(17.7559493405871,-15.4285794642658,
12.));
#220868=CARTESIAN_POINT('Ctrl Pts',(17.7459450555803,-15.4129242997828,
12.));
#220869=CARTESIAN_POINT('Ctrl Pts',(17.7359622059143,-15.3973985345796,
12.));
#220870=CARTESIAN_POINT('Ctrl Pts',(17.7260018109923,-15.3820027907965,
12.));
#220871=CARTESIAN_POINT('Ctrl Pts',(17.7160649064208,-15.3667376981702,
12.));
#220872=CARTESIAN_POINT('Ctrl Pts',(17.7061525444044,-15.3516038942064,
12.));
#220873=CARTESIAN_POINT('Ctrl Pts',(17.6962657941984,-15.3366020244069,
12.));
#220874=CARTESIAN_POINT('Ctrl Pts',(17.6864057426052,-15.3217327425341,
12.));
#220875=CARTESIAN_POINT('Ctrl Pts',(17.6765734944559,-15.3069967108501,
12.));
#220876=CARTESIAN_POINT('Ctrl Pts',(17.6667701731041,-15.2923946003598,
12.));
#220877=CARTESIAN_POINT('Ctrl Pts',(17.6569969209,-15.2779270910238,12.));
#220878=CARTESIAN_POINT('Ctrl Pts',(17.6472548997329,-15.263594872029,12.));
#220879=CARTESIAN_POINT('Ctrl Pts',(17.637545291637,-15.2493986421091,12.));
#220880=CARTESIAN_POINT('Ctrl Pts',(17.6278692993765,-15.2353391098367,
12.));
#220881=CARTESIAN_POINT('Ctrl Pts',(17.6182281470467,-15.22141699392,12.));
#220882=CARTESIAN_POINT('Ctrl Pts',(17.6086230806497,-15.2076330234686,
12.));
#220883=CARTESIAN_POINT('Ctrl Pts',(17.5990553687595,-15.1939879383268,
12.));
#220884=CARTESIAN_POINT('Ctrl Pts',(17.5895263032592,-15.1804824894605,
12.));
#220885=CARTESIAN_POINT('Ctrl Pts',(17.5800372000539,-15.1671174393136,
12.));
#220886=CARTESIAN_POINT('Ctrl Pts',(17.570589399803,-15.1538935621715,12.));
#220887=CARTESIAN_POINT('Ctrl Pts',(17.5611842686196,-15.1408116444877,
12.));
#220888=CARTESIAN_POINT('Ctrl Pts',(17.5518231989122,-15.127872485314,12.));
#220889=CARTESIAN_POINT('Ctrl Pts',(17.5425076102966,-15.1150768967729,
12.));
#220890=CARTESIAN_POINT('Ctrl Pts',(17.5332389504829,-15.1024257045033,
12.));
#220891=CARTESIAN_POINT('Ctrl Pts',(17.5240186961788,-15.0899197481082,
12.));
#220892=CARTESIAN_POINT('Ctrl Pts',(17.5148483539683,-15.0775598815748,
12.));
#220893=CARTESIAN_POINT('Ctrl Pts',(17.5057294613874,-15.0653469738306,
12.));
#220894=CARTESIAN_POINT('Ctrl Pts',(17.4966635880245,-15.0532819093085,
12.));
#220895=CARTESIAN_POINT('Ctrl Pts',(17.4876523366178,-15.0413655884993,
12.));
#220896=CARTESIAN_POINT('Ctrl Pts',(17.4786973441417,-15.029598928488,12.));
#220897=CARTESIAN_POINT('Ctrl Pts',(17.4698002829357,-15.0179828635086,
12.));
#220898=CARTESIAN_POINT('Ctrl Pts',(17.4609628621418,-15.0065183456921,
12.));
#220899=CARTESIAN_POINT('Ctrl Pts',(17.4521868291004,-14.9952063457778,
12.));
#220900=CARTESIAN_POINT('Ctrl Pts',(17.4434739707773,-14.9840478538358,
12.));
#220901=CARTESIAN_POINT('Ctrl Pts',(17.4348261151396,-14.9730438799452,
12.));
#220902=CARTESIAN_POINT('Ctrl Pts',(17.426245132709,-14.9621954549827,12.));
#220903=CARTESIAN_POINT('Ctrl Pts',(17.4177329382828,-14.9515036315143,
12.));
#220904=CARTESIAN_POINT('Ctrl Pts',(17.4092914926071,-14.940969484645,12.));
#220905=CARTESIAN_POINT('Ctrl Pts',(17.4009228040749,-14.9305941128757,
12.));
#220906=CARTESIAN_POINT('Ctrl Pts',(17.3926289303986,-14.9203786389342,
12.));
#220907=CARTESIAN_POINT('Ctrl Pts',(17.3844119809824,-14.9103242110057,
12.));
#220908=CARTESIAN_POINT('Ctrl Pts',(17.3762741193076,-14.900432003961,12.));
#220909=CARTESIAN_POINT('Ctrl Pts',(17.3682175653235,-14.8907032205788,
12.));
#220910=CARTESIAN_POINT('Ctrl Pts',(17.3602445978161,-14.8811390927423,
12.));
#220911=CARTESIAN_POINT('Ctrl Pts',(17.3523575568645,-14.8717408826956,
12.));
#220912=CARTESIAN_POINT('Ctrl Pts',(17.3445588463474,-14.8625098843417,
12.));
#220913=CARTESIAN_POINT('Ctrl Pts',(17.336850936485,-14.8534474245434,12.));
#220914=CARTESIAN_POINT('Ctrl Pts',(17.3292363662605,-14.8445548643508,
12.));
#220915=CARTESIAN_POINT('Ctrl Pts',(17.3217177462101,-14.8358336004197,
12.));
#220916=CARTESIAN_POINT('Ctrl Pts',(17.3142977632659,-14.8272850675379,
12.));
#220917=CARTESIAN_POINT('Ctrl Pts',(17.3069791853706,-14.8189107410162,
12.));
#220918=CARTESIAN_POINT('Ctrl Pts',(17.299764866148,-14.8107121391035,12.));
#220919=CARTESIAN_POINT('Ctrl Pts',(17.2926577496513,-14.8026908254276,
12.));
#220920=CARTESIAN_POINT('Ctrl Pts',(17.2856608733196,-14.7948484105249,
12.));
#220921=CARTESIAN_POINT('Ctrl Pts',(17.2787773704849,-14.787186553128,12.));
#220922=CARTESIAN_POINT('Ctrl Pts',(17.2720104735194,-14.7797069617804,
12.));
#220923=CARTESIAN_POINT('Ctrl Pts',(17.2653635155319,-14.7724113956731,
12.));
#220924=CARTESIAN_POINT('Ctrl Pts',(17.2588399401465,-14.7653016697591,
12.));
#220925=CARTESIAN_POINT('Ctrl Pts',(17.2524433146837,-14.7583796616617,
12.));
#220926=CARTESIAN_POINT('Ctrl Pts',(17.2461773413288,-14.7516473175124,
12.));
#220927=CARTESIAN_POINT('Ctrl Pts',(17.2400458713565,-14.7451066593792,
12.));
#220928=CARTESIAN_POINT('Ctrl Pts',(17.2340529062076,-14.7387597858117,
12.));
#220929=CARTESIAN_POINT('Ctrl Pts',(17.2282025904314,-14.7326088681163,
12.));
#220930=CARTESIAN_POINT('Ctrl Pts',(17.2224992099667,-14.7266561494282,
12.));
#220931=CARTESIAN_POINT('Ctrl Pts',(17.2169471814256,-14.7209039390327,
12.));
#220932=CARTESIAN_POINT('Ctrl Pts',(17.2115510835989,-14.7153546289339,
12.));
#220933=CARTESIAN_POINT('Ctrl Pts',(17.2063157097315,-14.7100107213586,
12.));
#220934=CARTESIAN_POINT('Ctrl Pts',(17.2012461084268,-14.7048748502663,
12.));
#220935=CARTESIAN_POINT('Ctrl Pts',(17.1963476411694,-14.699949811582,12.));
#220936=CARTESIAN_POINT('Ctrl Pts',(17.1916259308415,-14.6952385361706,
12.));
#220937=CARTESIAN_POINT('Ctrl Pts',(17.1870867909918,-14.6907440526958,
12.));
#220938=CARTESIAN_POINT('Ctrl Pts',(17.182736158472,-14.686469452232,12.));
#220939=CARTESIAN_POINT('Ctrl Pts',(17.1785800350826,-14.6824178576167,
12.));
#220940=CARTESIAN_POINT('Ctrl Pts',(17.1746247499057,-14.6785925615677,
12.));
#220941=CARTESIAN_POINT('Ctrl Pts',(17.1708771619129,-14.6749971333867,
12.));
#220942=CARTESIAN_POINT('Ctrl Pts',(17.167344972302,-14.671635583332,12.));
#220943=CARTESIAN_POINT('Ctrl Pts',(17.1640366762305,-14.6685123374423,
12.));
#220944=CARTESIAN_POINT('Ctrl Pts',(17.1609609517369,-14.6656319165057,
12.));
#220945=CARTESIAN_POINT('Ctrl Pts',(17.1581262646789,-14.6629987285992,
12.));
#220946=CARTESIAN_POINT('Ctrl Pts',(17.1555401986401,-14.6606167169642,
12.));
#220947=CARTESIAN_POINT('Ctrl Pts',(17.1532107762718,-14.6584900555302,
12.));
#220948=CARTESIAN_POINT('Ctrl Pts',(17.1511476869496,-14.6566237952435,
12.));
#220949=CARTESIAN_POINT('Ctrl Pts',(17.1493641837558,-14.655024862281,12.));
#220950=CARTESIAN_POINT('Ctrl Pts',(17.147876394491,-14.6537016966184,12.));
#220951=CARTESIAN_POINT('Ctrl Pts',(17.1466998098673,-14.6526624064978,
12.));
#220952=CARTESIAN_POINT('Ctrl Pts',(17.1458462295271,-14.6519131634508,
12.));
#220953=CARTESIAN_POINT('Ctrl Pts',(17.1454262858043,-14.6515481598068,
12.));
#220954=CARTESIAN_POINT('Ctrl Pts',(17.1452600887037,-14.6514066997196,
12.));
#220955=CARTESIAN_POINT('Ctrl Pts',(17.1452153999142,-14.6513711852843,
12.));
#220956=CARTESIAN_POINT('Ctrl Pts',(17.1452095830632,-14.6513681262571,
12.));
#220957=CARTESIAN_POINT('',(18.8464468996588,-17.9112098770111,0.));
#220958=CARTESIAN_POINT('Origin',(12.1729687575668,-17.7219872369693,0.));
#220959=CARTESIAN_POINT('',(12.7689476255362,-18.5896416359912,12.));
#220960=CARTESIAN_POINT('',(6.08648437878337,-8.86099361848466,12.));
#220961=CARTESIAN_POINT('',(12.7689476255362,-18.5896416359912,0.));
#220962=CARTESIAN_POINT('',(12.7689476255362,-18.5896416359912,0.));
#220963=CARTESIAN_POINT('',(6.08648437878337,-8.86099361848466,0.));
#220964=CARTESIAN_POINT('Ctrl Pts',(17.9112098770111,-18.8464468996588,
0.));
#220965=CARTESIAN_POINT('Ctrl Pts',(17.9112098770111,-18.8464468996588,
12.));
#220966=CARTESIAN_POINT('Ctrl Pts',(17.9057348246595,-18.8448126709692,
0.));
#220967=CARTESIAN_POINT('Ctrl Pts',(17.9057348246595,-18.8448126709692,
12.));
#220968=CARTESIAN_POINT('Ctrl Pts',(17.8947931177807,-18.8415402351786,
0.));
#220969=CARTESIAN_POINT('Ctrl Pts',(17.8947931177807,-18.8415402351786,
12.));
#220970=CARTESIAN_POINT('Ctrl Pts',(17.8784057509355,-18.8366196462581,
0.));
#220971=CARTESIAN_POINT('Ctrl Pts',(17.8784057509355,-18.8366196462581,
12.));
#220972=CARTESIAN_POINT('Ctrl Pts',(17.856606317477,-18.8300349895974,0.));
#220973=CARTESIAN_POINT('Ctrl Pts',(17.856606317477,-18.8300349895974,12.));
#220974=CARTESIAN_POINT('Ctrl Pts',(17.8294410311006,-18.8217643886157,
0.));
#220975=CARTESIAN_POINT('Ctrl Pts',(17.8294410311006,-18.8217643886157,
12.));
#220976=CARTESIAN_POINT('Ctrl Pts',(17.8023598011057,-18.8134540340417,
0.));
#220977=CARTESIAN_POINT('Ctrl Pts',(17.8023598011057,-18.8134540340417,
12.));
#220978=CARTESIAN_POINT('Ctrl Pts',(17.7753627137853,-18.8051039860448,
0.));
#220979=CARTESIAN_POINT('Ctrl Pts',(17.7753627137853,-18.8051039860448,
12.));
#220980=CARTESIAN_POINT('Ctrl Pts',(17.7484498996905,-18.7967143519419,
0.));
#220981=CARTESIAN_POINT('Ctrl Pts',(17.7484498996905,-18.7967143519419,
12.));
#220982=CARTESIAN_POINT('Ctrl Pts',(17.7216215409035,-18.788285297605,0.));
#220983=CARTESIAN_POINT('Ctrl Pts',(17.7216215409035,-18.788285297605,12.));
#220984=CARTESIAN_POINT('Ctrl Pts',(17.6948778823014,-18.7798170641374,
0.));
#220985=CARTESIAN_POINT('Ctrl Pts',(17.6948778823014,-18.7798170641374,
12.));
#220986=CARTESIAN_POINT('Ctrl Pts',(17.6682192274236,-18.7713099642754,
0.));
#220987=CARTESIAN_POINT('Ctrl Pts',(17.6682192274236,-18.7713099642754,
12.));
#220988=CARTESIAN_POINT('Ctrl Pts',(17.6416459210681,-18.762764361321,0.));
#220989=CARTESIAN_POINT('Ctrl Pts',(17.6416459210681,-18.762764361321,12.));
#220990=CARTESIAN_POINT('Ctrl Pts',(17.6151583357012,-18.7541806530984,
0.));
#220991=CARTESIAN_POINT('Ctrl Pts',(17.6151583357012,-18.7541806530984,
12.));
#220992=CARTESIAN_POINT('Ctrl Pts',(17.5887568561371,-18.7455592536688,
0.));
#220993=CARTESIAN_POINT('Ctrl Pts',(17.5887568561371,-18.7455592536688,
12.));
#220994=CARTESIAN_POINT('Ctrl Pts',(17.5624418653245,-18.7369005764553,
0.));
#220995=CARTESIAN_POINT('Ctrl Pts',(17.5624418653245,-18.7369005764553,
12.));
#220996=CARTESIAN_POINT('Ctrl Pts',(17.5362137287593,-18.7282050157138,
0.));
#220997=CARTESIAN_POINT('Ctrl Pts',(17.5362137287593,-18.7282050157138,
12.));
#220998=CARTESIAN_POINT('Ctrl Pts',(17.5100727820876,-18.7194729318098,
0.));
#220999=CARTESIAN_POINT('Ctrl Pts',(17.5100727820876,-18.7194729318098,
12.));
#221000=CARTESIAN_POINT('Ctrl Pts',(17.4840193397162,-18.7107046613912,
0.));
#221001=CARTESIAN_POINT('Ctrl Pts',(17.4840193397162,-18.7107046613912,
12.));
#221002=CARTESIAN_POINT('Ctrl Pts',(17.4580537012753,-18.70190052503,0.));
#221003=CARTESIAN_POINT('Ctrl Pts',(17.4580537012753,-18.70190052503,12.));
#221004=CARTESIAN_POINT('Ctrl Pts',(17.4321761588142,-18.6930608357409,
0.));
#221005=CARTESIAN_POINT('Ctrl Pts',(17.4321761588142,-18.6930608357409,
12.));
#221006=CARTESIAN_POINT('Ctrl Pts',(17.4063870038562,-18.6841859073471,
0.));
#221007=CARTESIAN_POINT('Ctrl Pts',(17.4063870038562,-18.6841859073471,
12.));
#221008=CARTESIAN_POINT('Ctrl Pts',(17.3806865340747,-18.6752760624052,
0.));
#221009=CARTESIAN_POINT('Ctrl Pts',(17.3806865340747,-18.6752760624052,
12.));
#221010=CARTESIAN_POINT('Ctrl Pts',(17.3550750612443,-18.6663316416582,
0.));
#221011=CARTESIAN_POINT('Ctrl Pts',(17.3550750612443,-18.6663316416582,
12.));
#221012=CARTESIAN_POINT('Ctrl Pts',(17.3295529098618,-18.6573530024033,
0.));
#221013=CARTESIAN_POINT('Ctrl Pts',(17.3295529098618,-18.6573530024033,
12.));
#221014=CARTESIAN_POINT('Ctrl Pts',(17.3041204135074,-18.6483405141865,
0.));
#221015=CARTESIAN_POINT('Ctrl Pts',(17.3041204135074,-18.6483405141865,
12.));
#221016=CARTESIAN_POINT('Ctrl Pts',(17.2787779120213,-18.6392945554748,
0.));
#221017=CARTESIAN_POINT('Ctrl Pts',(17.2787779120213,-18.6392945554748,
12.));
#221018=CARTESIAN_POINT('Ctrl Pts',(17.2535257482187,-18.6302155097943,
0.));
#221019=CARTESIAN_POINT('Ctrl Pts',(17.2535257482187,-18.6302155097943,
12.));
#221020=CARTESIAN_POINT('Ctrl Pts',(17.2283642650517,-18.6211037624038,
0.));
#221021=CARTESIAN_POINT('Ctrl Pts',(17.2283642650517,-18.6211037624038,
12.));
#221022=CARTESIAN_POINT('Ctrl Pts',(17.2032938019284,-18.6119596959949,
0.));
#221023=CARTESIAN_POINT('Ctrl Pts',(17.2032938019284,-18.6119596959949,
12.));
#221024=CARTESIAN_POINT('Ctrl Pts',(17.1783146940127,-18.6027836898817,
0.));
#221025=CARTESIAN_POINT('Ctrl Pts',(17.1783146940127,-18.6027836898817,
12.));
#221026=CARTESIAN_POINT('Ctrl Pts',(17.1534272741643,-18.5935761222825,
0.));
#221027=CARTESIAN_POINT('Ctrl Pts',(17.1534272741643,-18.5935761222825,
12.));
#221028=CARTESIAN_POINT('Ctrl Pts',(17.1286318741183,-18.5843373717247,
0.));
#221029=CARTESIAN_POINT('Ctrl Pts',(17.1286318741183,-18.5843373717247,
12.));
#221030=CARTESIAN_POINT('Ctrl Pts',(17.1039288260001,-18.5750678188542,
0.));
#221031=CARTESIAN_POINT('Ctrl Pts',(17.1039288260001,-18.5750678188542,
12.));
#221032=CARTESIAN_POINT('Ctrl Pts',(17.0793184636079,-18.5657678479789,
0.));
#221033=CARTESIAN_POINT('Ctrl Pts',(17.0793184636079,-18.5657678479789,
12.));
#221034=CARTESIAN_POINT('Ctrl Pts',(17.0548011239751,-18.556437848963,0.));
#221035=CARTESIAN_POINT('Ctrl Pts',(17.0548011239751,-18.556437848963,12.));
#221036=CARTESIAN_POINT('Ctrl Pts',(17.0303771481738,-18.547078218209,0.));
#221037=CARTESIAN_POINT('Ctrl Pts',(17.0303771481738,-18.547078218209,12.));
#221038=CARTESIAN_POINT('Ctrl Pts',(17.0060468805097,-18.5376893576961,
0.));
#221039=CARTESIAN_POINT('Ctrl Pts',(17.0060468805097,-18.5376893576961,
12.));
#221040=CARTESIAN_POINT('Ctrl Pts',(16.981810668038,-18.5282716744197,0.));
#221041=CARTESIAN_POINT('Ctrl Pts',(16.981810668038,-18.5282716744197,12.));
#221042=CARTESIAN_POINT('Ctrl Pts',(16.9576688599339,-18.5188255796659,
0.));
#221043=CARTESIAN_POINT('Ctrl Pts',(16.9576688599339,-18.5188255796659,
12.));
#221044=CARTESIAN_POINT('Ctrl Pts',(16.9336218069353,-18.5093514883835,
0.));
#221045=CARTESIAN_POINT('Ctrl Pts',(16.9336218069353,-18.5093514883835,
12.));
#221046=CARTESIAN_POINT('Ctrl Pts',(16.9096698606943,-18.499849818462,0.));
#221047=CARTESIAN_POINT('Ctrl Pts',(16.9096698606943,-18.499849818462,12.));
#221048=CARTESIAN_POINT('Ctrl Pts',(16.8858133733088,-18.4903209902227,
0.));
#221049=CARTESIAN_POINT('Ctrl Pts',(16.8858133733088,-18.4903209902227,
12.));
#221050=CARTESIAN_POINT('Ctrl Pts',(16.8620526977171,-18.4807654268771,
0.));
#221051=CARTESIAN_POINT('Ctrl Pts',(16.8620526977171,-18.4807654268771,
12.));
#221052=CARTESIAN_POINT('Ctrl Pts',(16.8383881879709,-18.4711835548623,
0.));
#221053=CARTESIAN_POINT('Ctrl Pts',(16.8383881879709,-18.4711835548623,
12.));
#221054=CARTESIAN_POINT('Ctrl Pts',(16.8148201995472,-18.4615758042305,
0.));
#221055=CARTESIAN_POINT('Ctrl Pts',(16.8148201995472,-18.4615758042305,
12.));
#221056=CARTESIAN_POINT('Ctrl Pts',(16.791349089629,-18.4519426090124,0.));
#221057=CARTESIAN_POINT('Ctrl Pts',(16.791349089629,-18.4519426090124,12.));
#221058=CARTESIAN_POINT('Ctrl Pts',(16.7679752173992,-18.44228440761,0.));
#221059=CARTESIAN_POINT('Ctrl Pts',(16.7679752173992,-18.44228440761,12.));
#221060=CARTESIAN_POINT('Ctrl Pts',(16.7446989442882,-18.4326016431392,
0.));
#221061=CARTESIAN_POINT('Ctrl Pts',(16.7446989442882,-18.4326016431392,
12.));
#221062=CARTESIAN_POINT('Ctrl Pts',(16.7215206338818,-18.4228947633187,
0.));
#221063=CARTESIAN_POINT('Ctrl Pts',(16.7215206338818,-18.4228947633187,
12.));
#221064=CARTESIAN_POINT('Ctrl Pts',(16.698440651849,-18.413164220399,0.));
#221065=CARTESIAN_POINT('Ctrl Pts',(16.698440651849,-18.413164220399,12.));
#221066=CARTESIAN_POINT('Ctrl Pts',(16.6754593658513,-18.403410471079,0.));
#221067=CARTESIAN_POINT('Ctrl Pts',(16.6754593658513,-18.403410471079,12.));
#221068=CARTESIAN_POINT('Ctrl Pts',(16.6525771454513,-18.3936339764332,
0.));
#221069=CARTESIAN_POINT('Ctrl Pts',(16.6525771454513,-18.3936339764332,
12.));
#221070=CARTESIAN_POINT('Ctrl Pts',(16.6297943620056,-18.3838352018327,
0.));
#221071=CARTESIAN_POINT('Ctrl Pts',(16.6297943620056,-18.3838352018327,
12.));
#221072=CARTESIAN_POINT('Ctrl Pts',(16.607111388571,-18.3740146168879,0.));
#221073=CARTESIAN_POINT('Ctrl Pts',(16.607111388571,-18.3740146168879,12.));
#221074=CARTESIAN_POINT('Ctrl Pts',(16.5845286000217,-18.3641726955889,
0.));
#221075=CARTESIAN_POINT('Ctrl Pts',(16.5845286000217,-18.3641726955889,
12.));
#221076=CARTESIAN_POINT('Ctrl Pts',(16.5620463731413,-18.354309916433,0.));
#221077=CARTESIAN_POINT('Ctrl Pts',(16.5620463731413,-18.354309916433,12.));
#221078=CARTESIAN_POINT('Ctrl Pts',(16.5396650867139,-18.34442676256,0.));
#221079=CARTESIAN_POINT('Ctrl Pts',(16.5396650867139,-18.34442676256,12.));
#221080=CARTESIAN_POINT('Ctrl Pts',(16.5173851216045,-18.3345237218864,
0.));
#221081=CARTESIAN_POINT('Ctrl Pts',(16.5173851216045,-18.3345237218864,
12.));
#221082=CARTESIAN_POINT('Ctrl Pts',(16.4952068608345,-18.3246012872469,
0.));
#221083=CARTESIAN_POINT('Ctrl Pts',(16.4952068608345,-18.3246012872469,
12.));
#221084=CARTESIAN_POINT('Ctrl Pts',(16.4731306896441,-18.3146599565231,
0.));
#221085=CARTESIAN_POINT('Ctrl Pts',(16.4731306896441,-18.3146599565231,
12.));
#221086=CARTESIAN_POINT('Ctrl Pts',(16.4511569955233,-18.304700232686,0.));
#221087=CARTESIAN_POINT('Ctrl Pts',(16.4511569955233,-18.304700232686,12.));
#221088=CARTESIAN_POINT('Ctrl Pts',(16.4292861682378,-18.294722623851,0.));
#221089=CARTESIAN_POINT('Ctrl Pts',(16.4292861682378,-18.294722623851,12.));
#221090=CARTESIAN_POINT('Ctrl Pts',(16.4075185998454,-18.2847276433309,
0.));
#221091=CARTESIAN_POINT('Ctrl Pts',(16.4075185998454,-18.2847276433309,
12.));
#221092=CARTESIAN_POINT('Ctrl Pts',(16.385854684708,-18.2747158096934,0.));
#221093=CARTESIAN_POINT('Ctrl Pts',(16.385854684708,-18.2747158096934,12.));
#221094=CARTESIAN_POINT('Ctrl Pts',(16.3642948194868,-18.2646876468169,
0.));
#221095=CARTESIAN_POINT('Ctrl Pts',(16.3642948194868,-18.2646876468169,
12.));
#221096=CARTESIAN_POINT('Ctrl Pts',(16.3428394031589,-18.2546436839608,
0.));
#221097=CARTESIAN_POINT('Ctrl Pts',(16.3428394031589,-18.2546436839608,
12.));
#221098=CARTESIAN_POINT('Ctrl Pts',(16.3214888370987,-18.2445844558742,
0.));
#221099=CARTESIAN_POINT('Ctrl Pts',(16.3214888370987,-18.2445844558742,
12.));
#221100=CARTESIAN_POINT('Ctrl Pts',(16.3002435251378,-18.2345105028982,
0.));
#221101=CARTESIAN_POINT('Ctrl Pts',(16.3002435251378,-18.2345105028982,
12.));
#221102=CARTESIAN_POINT('Ctrl Pts',(16.2791038736223,-18.2244223710746,
0.));
#221103=CARTESIAN_POINT('Ctrl Pts',(16.2791038736223,-18.2244223710746,
12.));
#221104=CARTESIAN_POINT('Ctrl Pts',(16.2580702914615,-18.2143206122529,
0.));
#221105=CARTESIAN_POINT('Ctrl Pts',(16.2580702914615,-18.2143206122529,
12.));
#221106=CARTESIAN_POINT('Ctrl Pts',(16.2371431901638,-18.2042057842035,
0.));
#221107=CARTESIAN_POINT('Ctrl Pts',(16.2371431901638,-18.2042057842035,
12.));
#221108=CARTESIAN_POINT('Ctrl Pts',(16.2163229838875,-18.1940784507229,
0.));
#221109=CARTESIAN_POINT('Ctrl Pts',(16.2163229838875,-18.1940784507229,
12.));
#221110=CARTESIAN_POINT('Ctrl Pts',(16.1956100895073,-18.1839391817331,
0.));
#221111=CARTESIAN_POINT('Ctrl Pts',(16.1956100895073,-18.1839391817331,
12.));
#221112=CARTESIAN_POINT('Ctrl Pts',(16.1750049266671,-18.1737885533849,
0.));
#221113=CARTESIAN_POINT('Ctrl Pts',(16.1750049266671,-18.1737885533849,
12.));
#221114=CARTESIAN_POINT('Ctrl Pts',(16.154507917826,-18.1636271481615,0.));
#221115=CARTESIAN_POINT('Ctrl Pts',(16.154507917826,-18.1636271481615,12.));
#221116=CARTESIAN_POINT('Ctrl Pts',(16.1341194882988,-18.1534555549853,
0.));
#221117=CARTESIAN_POINT('Ctrl Pts',(16.1341194882988,-18.1534555549853,
12.));
#221118=CARTESIAN_POINT('Ctrl Pts',(16.1138400662794,-18.1432743693235,
0.));
#221119=CARTESIAN_POINT('Ctrl Pts',(16.1138400662794,-18.1432743693235,
12.));
#221120=CARTESIAN_POINT('Ctrl Pts',(16.0936700829112,-18.1330841933105,
0.));
#221121=CARTESIAN_POINT('Ctrl Pts',(16.0936700829112,-18.1330841933105,
12.));
#221122=CARTESIAN_POINT('Ctrl Pts',(16.0736099723668,-18.1228856358751,
0.));
#221123=CARTESIAN_POINT('Ctrl Pts',(16.0736099723668,-18.1228856358751,
12.));
#221124=CARTESIAN_POINT('Ctrl Pts',(16.0536601719125,-18.112679312869,0.));
#221125=CARTESIAN_POINT('Ctrl Pts',(16.0536601719125,-18.112679312869,12.));
#221126=CARTESIAN_POINT('Ctrl Pts',(16.0338211219693,-18.1024658471966,
0.));
#221127=CARTESIAN_POINT('Ctrl Pts',(16.0338211219693,-18.1024658471966,
12.));
#221128=CARTESIAN_POINT('Ctrl Pts',(16.014093266161,-18.0922458689462,0.));
#221129=CARTESIAN_POINT('Ctrl Pts',(16.014093266161,-18.0922458689462,12.));
#221130=CARTESIAN_POINT('Ctrl Pts',(15.9944770513613,-18.0820200155236,
0.));
#221131=CARTESIAN_POINT('Ctrl Pts',(15.9944770513613,-18.0820200155236,
12.));
#221132=CARTESIAN_POINT('Ctrl Pts',(15.9749729277846,-18.0717889317958,
0.));
#221133=CARTESIAN_POINT('Ctrl Pts',(15.9749729277846,-18.0717889317958,
12.));
#221134=CARTESIAN_POINT('Ctrl Pts',(15.9555813490644,-18.061553270236,0.));
#221135=CARTESIAN_POINT('Ctrl Pts',(15.9555813490644,-18.061553270236,12.));
#221136=CARTESIAN_POINT('Ctrl Pts',(15.9363027723244,-18.0513136910691,
0.));
#221137=CARTESIAN_POINT('Ctrl Pts',(15.9363027723244,-18.0513136910691,
12.));
#221138=CARTESIAN_POINT('Ctrl Pts',(15.9171376582436,-18.0410708624209,
0.));
#221139=CARTESIAN_POINT('Ctrl Pts',(15.9171376582436,-18.0410708624209,
12.));
#221140=CARTESIAN_POINT('Ctrl Pts',(15.8980864711042,-18.0308254604636,
0.));
#221141=CARTESIAN_POINT('Ctrl Pts',(15.8980864711042,-18.0308254604636,
12.));
#221142=CARTESIAN_POINT('Ctrl Pts',(15.8791496788682,-18.0205781695769,
0.));
#221143=CARTESIAN_POINT('Ctrl Pts',(15.8791496788682,-18.0205781695769,
12.));
#221144=CARTESIAN_POINT('Ctrl Pts',(15.8603277532831,-18.0103296825205,
0.));
#221145=CARTESIAN_POINT('Ctrl Pts',(15.8603277532831,-18.0103296825205,
12.));
#221146=CARTESIAN_POINT('Ctrl Pts',(15.8416211699679,-18.0000807006052,
0.));
#221147=CARTESIAN_POINT('Ctrl Pts',(15.8416211699679,-18.0000807006052,
12.));
#221148=CARTESIAN_POINT('Ctrl Pts',(15.8230304084962,-17.9898319338665,
0.));
#221149=CARTESIAN_POINT('Ctrl Pts',(15.8230304084962,-17.9898319338665,
12.));
#221150=CARTESIAN_POINT('Ctrl Pts',(15.8045559524676,-17.9795841012386,
0.));
#221151=CARTESIAN_POINT('Ctrl Pts',(15.8045559524676,-17.9795841012386,
12.));
#221152=CARTESIAN_POINT('Ctrl Pts',(15.7861982895724,-17.9693379307303,
0.));
#221153=CARTESIAN_POINT('Ctrl Pts',(15.7861982895724,-17.9693379307303,
12.));
#221154=CARTESIAN_POINT('Ctrl Pts',(15.7679579117077,-17.9590941596242,
0.));
#221155=CARTESIAN_POINT('Ctrl Pts',(15.7679579117077,-17.9590941596242,
12.));
#221156=CARTESIAN_POINT('Ctrl Pts',(15.749835315086,-17.9488535346781,0.));
#221157=CARTESIAN_POINT('Ctrl Pts',(15.749835315086,-17.9488535346781,12.));
#221158=CARTESIAN_POINT('Ctrl Pts',(15.7318310003335,-17.9386168123262,
0.));
#221159=CARTESIAN_POINT('Ctrl Pts',(15.7318310003335,-17.9386168123262,
12.));
#221160=CARTESIAN_POINT('Ctrl Pts',(15.7139454725838,-17.9283847588836,
0.));
#221161=CARTESIAN_POINT('Ctrl Pts',(15.7139454725838,-17.9283847588836,
12.));
#221162=CARTESIAN_POINT('Ctrl Pts',(15.6961792415522,-17.9181581507455,
0.));
#221163=CARTESIAN_POINT('Ctrl Pts',(15.6961792415522,-17.9181581507455,
12.));
#221164=CARTESIAN_POINT('Ctrl Pts',(15.678532821646,-17.9079377746111,0.));
#221165=CARTESIAN_POINT('Ctrl Pts',(15.678532821646,-17.9079377746111,12.));
#221166=CARTESIAN_POINT('Ctrl Pts',(15.661006732103,-17.897724427724,0.));
#221167=CARTESIAN_POINT('Ctrl Pts',(15.661006732103,-17.897724427724,12.));
#221168=CARTESIAN_POINT('Ctrl Pts',(15.6436014971084,-17.8875189181091,
0.));
#221169=CARTESIAN_POINT('Ctrl Pts',(15.6436014971084,-17.8875189181091,
12.));
#221170=CARTESIAN_POINT('Ctrl Pts',(15.6263176459108,-17.8773220648125,
0.));
#221171=CARTESIAN_POINT('Ctrl Pts',(15.6263176459108,-17.8773220648125,
12.));
#221172=CARTESIAN_POINT('Ctrl Pts',(15.609155712921,-17.8671346981394,0.));
#221173=CARTESIAN_POINT('Ctrl Pts',(15.609155712921,-17.8671346981394,12.));
#221174=CARTESIAN_POINT('Ctrl Pts',(15.5921162378192,-17.8569576599006,
0.));
#221175=CARTESIAN_POINT('Ctrl Pts',(15.5921162378192,-17.8569576599006,
12.));
#221176=CARTESIAN_POINT('Ctrl Pts',(15.5751997657162,-17.8467918036987,
0.));
#221177=CARTESIAN_POINT('Ctrl Pts',(15.5751997657162,-17.8467918036987,
12.));
#221178=CARTESIAN_POINT('Ctrl Pts',(15.5584068472982,-17.8366379952085,
0.));
#221179=CARTESIAN_POINT('Ctrl Pts',(15.5584068472982,-17.8366379952085,
12.));
#221180=CARTESIAN_POINT('Ctrl Pts',(15.541738038964,-17.8264971124607,0.));
#221181=CARTESIAN_POINT('Ctrl Pts',(15.541738038964,-17.8264971124607,12.));
#221182=CARTESIAN_POINT('Ctrl Pts',(15.5251939029552,-17.8163700461256,
0.));
#221183=CARTESIAN_POINT('Ctrl Pts',(15.5251939029552,-17.8163700461256,
12.));
#221184=CARTESIAN_POINT('Ctrl Pts',(15.5087750074718,-17.8062576997952,
0.));
#221185=CARTESIAN_POINT('Ctrl Pts',(15.5087750074718,-17.8062576997952,
12.));
#221186=CARTESIAN_POINT('Ctrl Pts',(15.4924819268517,-17.7961609903148,
0.));
#221187=CARTESIAN_POINT('Ctrl Pts',(15.4924819268517,-17.7961609903148,
12.));
#221188=CARTESIAN_POINT('Ctrl Pts',(15.4763152417497,-17.786080848122,0.));
#221189=CARTESIAN_POINT('Ctrl Pts',(15.4763152417497,-17.786080848122,12.));
#221190=CARTESIAN_POINT('Ctrl Pts',(15.4602755393017,-17.7760182175815,
0.));
#221191=CARTESIAN_POINT('Ctrl Pts',(15.4602755393017,-17.7760182175815,
12.));
#221192=CARTESIAN_POINT('Ctrl Pts',(15.4443634132869,-17.7659740573265,
0.));
#221193=CARTESIAN_POINT('Ctrl Pts',(15.4443634132869,-17.7659740573265,
12.));
#221194=CARTESIAN_POINT('Ctrl Pts',(15.4285794642667,-17.7559493405881,
0.));
#221195=CARTESIAN_POINT('Ctrl Pts',(15.4285794642667,-17.7559493405881,
12.));
#221196=CARTESIAN_POINT('Ctrl Pts',(15.4129242997837,-17.7459450555813,
0.));
#221197=CARTESIAN_POINT('Ctrl Pts',(15.4129242997837,-17.7459450555813,
12.));
#221198=CARTESIAN_POINT('Ctrl Pts',(15.3973985345802,-17.735962205915,0.));
#221199=CARTESIAN_POINT('Ctrl Pts',(15.3973985345802,-17.735962205915,12.));
#221200=CARTESIAN_POINT('Ctrl Pts',(15.3820027907966,-17.7260018109924,
0.));
#221201=CARTESIAN_POINT('Ctrl Pts',(15.3820027907966,-17.7260018109924,
12.));
#221202=CARTESIAN_POINT('Ctrl Pts',(15.3667376981699,-17.7160649064206,
0.));
#221203=CARTESIAN_POINT('Ctrl Pts',(15.3667376981699,-17.7160649064206,
12.));
#221204=CARTESIAN_POINT('Ctrl Pts',(15.351603894206,-17.7061525444042,0.));
#221205=CARTESIAN_POINT('Ctrl Pts',(15.351603894206,-17.7061525444042,12.));
#221206=CARTESIAN_POINT('Ctrl Pts',(15.3366020244066,-17.6962657941983,
0.));
#221207=CARTESIAN_POINT('Ctrl Pts',(15.3366020244066,-17.6962657941983,
12.));
#221208=CARTESIAN_POINT('Ctrl Pts',(15.3217327425338,-17.6864057426052,
0.));
#221209=CARTESIAN_POINT('Ctrl Pts',(15.3217327425338,-17.6864057426052,
12.));
#221210=CARTESIAN_POINT('Ctrl Pts',(15.30699671085,-17.676573494456,0.));
#221211=CARTESIAN_POINT('Ctrl Pts',(15.30699671085,-17.676573494456,12.));
#221212=CARTESIAN_POINT('Ctrl Pts',(15.2923946003598,-17.6667701731041,
0.));
#221213=CARTESIAN_POINT('Ctrl Pts',(15.2923946003598,-17.6667701731041,
12.));
#221214=CARTESIAN_POINT('Ctrl Pts',(15.2779270910239,-17.6569969209,0.));
#221215=CARTESIAN_POINT('Ctrl Pts',(15.2779270910239,-17.6569969209,12.));
#221216=CARTESIAN_POINT('Ctrl Pts',(15.2635948720292,-17.6472548997328,
0.));
#221217=CARTESIAN_POINT('Ctrl Pts',(15.2635948720292,-17.6472548997328,
12.));
#221218=CARTESIAN_POINT('Ctrl Pts',(15.2493986421092,-17.6375452916369,
0.));
#221219=CARTESIAN_POINT('Ctrl Pts',(15.2493986421092,-17.6375452916369,
12.));
#221220=CARTESIAN_POINT('Ctrl Pts',(15.2353391098366,-17.6278692993764,
0.));
#221221=CARTESIAN_POINT('Ctrl Pts',(15.2353391098366,-17.6278692993764,
12.));
#221222=CARTESIAN_POINT('Ctrl Pts',(15.2214169939199,-17.6182281470468,
0.));
#221223=CARTESIAN_POINT('Ctrl Pts',(15.2214169939199,-17.6182281470468,
12.));
#221224=CARTESIAN_POINT('Ctrl Pts',(15.2076330234686,-17.60862308065,0.));
#221225=CARTESIAN_POINT('Ctrl Pts',(15.2076330234686,-17.60862308065,12.));
#221226=CARTESIAN_POINT('Ctrl Pts',(15.1939879383268,-17.5990553687599,
0.));
#221227=CARTESIAN_POINT('Ctrl Pts',(15.1939879383268,-17.5990553687599,
12.));
#221228=CARTESIAN_POINT('Ctrl Pts',(15.1804824894605,-17.5895263032595,
0.));
#221229=CARTESIAN_POINT('Ctrl Pts',(15.1804824894605,-17.5895263032595,
12.));
#221230=CARTESIAN_POINT('Ctrl Pts',(15.1671174393137,-17.580037200054,0.));
#221231=CARTESIAN_POINT('Ctrl Pts',(15.1671174393137,-17.580037200054,12.));
#221232=CARTESIAN_POINT('Ctrl Pts',(15.1538935621714,-17.5705893998029,
0.));
#221233=CARTESIAN_POINT('Ctrl Pts',(15.1538935621714,-17.5705893998029,
12.));
#221234=CARTESIAN_POINT('Ctrl Pts',(15.1408116444876,-17.5611842686192,
0.));
#221235=CARTESIAN_POINT('Ctrl Pts',(15.1408116444876,-17.5611842686192,
12.));
#221236=CARTESIAN_POINT('Ctrl Pts',(15.1278724853138,-17.5518231989117,
0.));
#221237=CARTESIAN_POINT('Ctrl Pts',(15.1278724853138,-17.5518231989117,
12.));
#221238=CARTESIAN_POINT('Ctrl Pts',(15.1150768967728,-17.5425076102963,
0.));
#221239=CARTESIAN_POINT('Ctrl Pts',(15.1150768967728,-17.5425076102963,
12.));
#221240=CARTESIAN_POINT('Ctrl Pts',(15.1024257045033,-17.5332389504829,
0.));
#221241=CARTESIAN_POINT('Ctrl Pts',(15.1024257045033,-17.5332389504829,
12.));
#221242=CARTESIAN_POINT('Ctrl Pts',(15.0899197481082,-17.5240186961791,
0.));
#221243=CARTESIAN_POINT('Ctrl Pts',(15.0899197481082,-17.5240186961791,
12.));
#221244=CARTESIAN_POINT('Ctrl Pts',(15.0775598815749,-17.5148483539687,
0.));
#221245=CARTESIAN_POINT('Ctrl Pts',(15.0775598815749,-17.5148483539687,
12.));
#221246=CARTESIAN_POINT('Ctrl Pts',(15.0653469738307,-17.5057294613877,
0.));
#221247=CARTESIAN_POINT('Ctrl Pts',(15.0653469738307,-17.5057294613877,
12.));
#221248=CARTESIAN_POINT('Ctrl Pts',(15.0532819093085,-17.4966635880246,
0.));
#221249=CARTESIAN_POINT('Ctrl Pts',(15.0532819093085,-17.4966635880246,
12.));
#221250=CARTESIAN_POINT('Ctrl Pts',(15.0413655884993,-17.4876523366178,
0.));
#221251=CARTESIAN_POINT('Ctrl Pts',(15.0413655884993,-17.4876523366178,
12.));
#221252=CARTESIAN_POINT('Ctrl Pts',(15.029598928488,-17.4786973441417,0.));
#221253=CARTESIAN_POINT('Ctrl Pts',(15.029598928488,-17.4786973441417,12.));
#221254=CARTESIAN_POINT('Ctrl Pts',(15.0179828635087,-17.4698002829357,
0.));
#221255=CARTESIAN_POINT('Ctrl Pts',(15.0179828635087,-17.4698002829357,
12.));
#221256=CARTESIAN_POINT('Ctrl Pts',(15.0065183456922,-17.4609628621419,
0.));
#221257=CARTESIAN_POINT('Ctrl Pts',(15.0065183456922,-17.4609628621419,
12.));
#221258=CARTESIAN_POINT('Ctrl Pts',(14.9952063457779,-17.4521868291005,
0.));
#221259=CARTESIAN_POINT('Ctrl Pts',(14.9952063457779,-17.4521868291005,
12.));
#221260=CARTESIAN_POINT('Ctrl Pts',(14.9840478538357,-17.4434739707773,
0.));
#221261=CARTESIAN_POINT('Ctrl Pts',(14.9840478538357,-17.4434739707773,
12.));
#221262=CARTESIAN_POINT('Ctrl Pts',(14.973043879945,-17.4348261151395,0.));
#221263=CARTESIAN_POINT('Ctrl Pts',(14.973043879945,-17.4348261151395,12.));
#221264=CARTESIAN_POINT('Ctrl Pts',(14.9621954549825,-17.4262451327088,
0.));
#221265=CARTESIAN_POINT('Ctrl Pts',(14.9621954549825,-17.4262451327088,
12.));
#221266=CARTESIAN_POINT('Ctrl Pts',(14.9515036315142,-17.4177329382827,
0.));
#221267=CARTESIAN_POINT('Ctrl Pts',(14.9515036315142,-17.4177329382827,
12.));
#221268=CARTESIAN_POINT('Ctrl Pts',(14.940969484645,-17.4092914926072,0.));
#221269=CARTESIAN_POINT('Ctrl Pts',(14.940969484645,-17.4092914926072,12.));
#221270=CARTESIAN_POINT('Ctrl Pts',(14.9305941128758,-17.400922804075,0.));
#221271=CARTESIAN_POINT('Ctrl Pts',(14.9305941128758,-17.400922804075,12.));
#221272=CARTESIAN_POINT('Ctrl Pts',(14.9203786389343,-17.3926289303987,
0.));
#221273=CARTESIAN_POINT('Ctrl Pts',(14.9203786389343,-17.3926289303987,
12.));
#221274=CARTESIAN_POINT('Ctrl Pts',(14.9103242110057,-17.3844119809823,
0.));
#221275=CARTESIAN_POINT('Ctrl Pts',(14.9103242110057,-17.3844119809823,
12.));
#221276=CARTESIAN_POINT('Ctrl Pts',(14.9004320039609,-17.3762741193075,
0.));
#221277=CARTESIAN_POINT('Ctrl Pts',(14.9004320039609,-17.3762741193075,
12.));
#221278=CARTESIAN_POINT('Ctrl Pts',(14.8907032205789,-17.3682175653236,
0.));
#221279=CARTESIAN_POINT('Ctrl Pts',(14.8907032205789,-17.3682175653236,
12.));
#221280=CARTESIAN_POINT('Ctrl Pts',(14.8811390927424,-17.3602445978163,
0.));
#221281=CARTESIAN_POINT('Ctrl Pts',(14.8811390927424,-17.3602445978163,
12.));
#221282=CARTESIAN_POINT('Ctrl Pts',(14.8717408826957,-17.3523575568648,
0.));
#221283=CARTESIAN_POINT('Ctrl Pts',(14.8717408826957,-17.3523575568648,
12.));
#221284=CARTESIAN_POINT('Ctrl Pts',(14.8625098843419,-17.3445588463477,
0.));
#221285=CARTESIAN_POINT('Ctrl Pts',(14.8625098843419,-17.3445588463477,
12.));
#221286=CARTESIAN_POINT('Ctrl Pts',(14.8534474245433,-17.336850936485,0.));
#221287=CARTESIAN_POINT('Ctrl Pts',(14.8534474245433,-17.336850936485,12.));
#221288=CARTESIAN_POINT('Ctrl Pts',(14.8445548643504,-17.3292363662601,
0.));
#221289=CARTESIAN_POINT('Ctrl Pts',(14.8445548643504,-17.3292363662601,
12.));
#221290=CARTESIAN_POINT('Ctrl Pts',(14.8358336004193,-17.3217177462096,
0.));
#221291=CARTESIAN_POINT('Ctrl Pts',(14.8358336004193,-17.3217177462096,
12.));
#221292=CARTESIAN_POINT('Ctrl Pts',(14.8272850675375,-17.3142977632656,
0.));
#221293=CARTESIAN_POINT('Ctrl Pts',(14.8272850675375,-17.3142977632656,
12.));
#221294=CARTESIAN_POINT('Ctrl Pts',(14.8189107410161,-17.3069791853705,
0.));
#221295=CARTESIAN_POINT('Ctrl Pts',(14.8189107410161,-17.3069791853705,
12.));
#221296=CARTESIAN_POINT('Ctrl Pts',(14.8107121391038,-17.2997648661483,
0.));
#221297=CARTESIAN_POINT('Ctrl Pts',(14.8107121391038,-17.2997648661483,
12.));
#221298=CARTESIAN_POINT('Ctrl Pts',(14.8026908254281,-17.2926577496519,
0.));
#221299=CARTESIAN_POINT('Ctrl Pts',(14.8026908254281,-17.2926577496519,
12.));
#221300=CARTESIAN_POINT('Ctrl Pts',(14.7948484105252,-17.28566087332,0.));
#221301=CARTESIAN_POINT('Ctrl Pts',(14.7948484105252,-17.28566087332,12.));
#221302=CARTESIAN_POINT('Ctrl Pts',(14.787186553128,-17.278777370485,0.));
#221303=CARTESIAN_POINT('Ctrl Pts',(14.787186553128,-17.278777370485,12.));
#221304=CARTESIAN_POINT('Ctrl Pts',(14.7797069617802,-17.2720104735192,
0.));
#221305=CARTESIAN_POINT('Ctrl Pts',(14.7797069617802,-17.2720104735192,
12.));
#221306=CARTESIAN_POINT('Ctrl Pts',(14.7724113956728,-17.2653635155317,
0.));
#221307=CARTESIAN_POINT('Ctrl Pts',(14.7724113956728,-17.2653635155317,
12.));
#221308=CARTESIAN_POINT('Ctrl Pts',(14.7653016697589,-17.2588399401464,
0.));
#221309=CARTESIAN_POINT('Ctrl Pts',(14.7653016697589,-17.2588399401464,
12.));
#221310=CARTESIAN_POINT('Ctrl Pts',(14.7583796616617,-17.2524433146837,
0.));
#221311=CARTESIAN_POINT('Ctrl Pts',(14.7583796616617,-17.2524433146837,
12.));
#221312=CARTESIAN_POINT('Ctrl Pts',(14.7516473175124,-17.2461773413289,
0.));
#221313=CARTESIAN_POINT('Ctrl Pts',(14.7516473175124,-17.2461773413289,
12.));
#221314=CARTESIAN_POINT('Ctrl Pts',(14.7451066593793,-17.2400458713566,
0.));
#221315=CARTESIAN_POINT('Ctrl Pts',(14.7451066593793,-17.2400458713566,
12.));
#221316=CARTESIAN_POINT('Ctrl Pts',(14.7387597858117,-17.2340529062078,
0.));
#221317=CARTESIAN_POINT('Ctrl Pts',(14.7387597858117,-17.2340529062078,
12.));
#221318=CARTESIAN_POINT('Ctrl Pts',(14.7326088681163,-17.2282025904314,
0.));
#221319=CARTESIAN_POINT('Ctrl Pts',(14.7326088681163,-17.2282025904314,
12.));
#221320=CARTESIAN_POINT('Ctrl Pts',(14.7266561494282,-17.2224992099666,
0.));
#221321=CARTESIAN_POINT('Ctrl Pts',(14.7266561494282,-17.2224992099666,
12.));
#221322=CARTESIAN_POINT('Ctrl Pts',(14.7209039390325,-17.2169471814255,
0.));
#221323=CARTESIAN_POINT('Ctrl Pts',(14.7209039390325,-17.2169471814255,
12.));
#221324=CARTESIAN_POINT('Ctrl Pts',(14.7153546289338,-17.2115510835988,
0.));
#221325=CARTESIAN_POINT('Ctrl Pts',(14.7153546289338,-17.2115510835988,
12.));
#221326=CARTESIAN_POINT('Ctrl Pts',(14.7100107213586,-17.2063157097316,
0.));
#221327=CARTESIAN_POINT('Ctrl Pts',(14.7100107213586,-17.2063157097316,
12.));
#221328=CARTESIAN_POINT('Ctrl Pts',(14.7048748502662,-17.2012461084268,
0.));
#221329=CARTESIAN_POINT('Ctrl Pts',(14.7048748502662,-17.2012461084268,
12.));
#221330=CARTESIAN_POINT('Ctrl Pts',(14.699949811582,-17.1963476411694,0.));
#221331=CARTESIAN_POINT('Ctrl Pts',(14.699949811582,-17.1963476411694,12.));
#221332=CARTESIAN_POINT('Ctrl Pts',(14.6952385361706,-17.1916259308416,
0.));
#221333=CARTESIAN_POINT('Ctrl Pts',(14.6952385361706,-17.1916259308416,
12.));
#221334=CARTESIAN_POINT('Ctrl Pts',(14.6907440526957,-17.1870867909918,
0.));
#221335=CARTESIAN_POINT('Ctrl Pts',(14.6907440526957,-17.1870867909918,
12.));
#221336=CARTESIAN_POINT('Ctrl Pts',(14.6864694522319,-17.182736158472,0.));
#221337=CARTESIAN_POINT('Ctrl Pts',(14.6864694522319,-17.182736158472,12.));
#221338=CARTESIAN_POINT('Ctrl Pts',(14.6824178576166,-17.1785800350827,
0.));
#221339=CARTESIAN_POINT('Ctrl Pts',(14.6824178576166,-17.1785800350827,
12.));
#221340=CARTESIAN_POINT('Ctrl Pts',(14.6785925615676,-17.1746247499057,
0.));
#221341=CARTESIAN_POINT('Ctrl Pts',(14.6785925615676,-17.1746247499057,
12.));
#221342=CARTESIAN_POINT('Ctrl Pts',(14.6749971333867,-17.1708771619129,
0.));
#221343=CARTESIAN_POINT('Ctrl Pts',(14.6749971333867,-17.1708771619129,
12.));
#221344=CARTESIAN_POINT('Ctrl Pts',(14.6716355833321,-17.1673449723019,
0.));
#221345=CARTESIAN_POINT('Ctrl Pts',(14.6716355833321,-17.1673449723019,
12.));
#221346=CARTESIAN_POINT('Ctrl Pts',(14.6685123374424,-17.1640366762304,
0.));
#221347=CARTESIAN_POINT('Ctrl Pts',(14.6685123374424,-17.1640366762304,
12.));
#221348=CARTESIAN_POINT('Ctrl Pts',(14.6656319165057,-17.1609609517369,
0.));
#221349=CARTESIAN_POINT('Ctrl Pts',(14.6656319165057,-17.1609609517369,
12.));
#221350=CARTESIAN_POINT('Ctrl Pts',(14.662998728599,-17.1581262646789,0.));
#221351=CARTESIAN_POINT('Ctrl Pts',(14.662998728599,-17.1581262646789,12.));
#221352=CARTESIAN_POINT('Ctrl Pts',(14.660616716964,-17.1555401986403,0.));
#221353=CARTESIAN_POINT('Ctrl Pts',(14.660616716964,-17.1555401986403,12.));
#221354=CARTESIAN_POINT('Ctrl Pts',(14.65849005553,-17.1532107762719,0.));
#221355=CARTESIAN_POINT('Ctrl Pts',(14.65849005553,-17.1532107762719,12.));
#221356=CARTESIAN_POINT('Ctrl Pts',(14.6566237952435,-17.1511476869495,
0.));
#221357=CARTESIAN_POINT('Ctrl Pts',(14.6566237952435,-17.1511476869495,
12.));
#221358=CARTESIAN_POINT('Ctrl Pts',(14.6550248622813,-17.1493641837556,
0.));
#221359=CARTESIAN_POINT('Ctrl Pts',(14.6550248622813,-17.1493641837556,
12.));
#221360=CARTESIAN_POINT('Ctrl Pts',(14.6537016966188,-17.1478763944909,
0.));
#221361=CARTESIAN_POINT('Ctrl Pts',(14.6537016966188,-17.1478763944909,
12.));
#221362=CARTESIAN_POINT('Ctrl Pts',(14.6526624064978,-17.1466998098673,
0.));
#221363=CARTESIAN_POINT('Ctrl Pts',(14.6526624064978,-17.1466998098673,
12.));
#221364=CARTESIAN_POINT('Ctrl Pts',(14.65191316345,-17.1458462295273,0.));
#221365=CARTESIAN_POINT('Ctrl Pts',(14.65191316345,-17.1458462295273,12.));
#221366=CARTESIAN_POINT('Ctrl Pts',(14.6515481598057,-17.1454262858045,
0.));
#221367=CARTESIAN_POINT('Ctrl Pts',(14.6515481598057,-17.1454262858045,
12.));
#221368=CARTESIAN_POINT('Ctrl Pts',(14.6514066997188,-17.1452600887039,
0.));
#221369=CARTESIAN_POINT('Ctrl Pts',(14.6514066997188,-17.1452600887039,
12.));
#221370=CARTESIAN_POINT('Ctrl Pts',(14.6513711852839,-17.1452153999142,
0.));
#221371=CARTESIAN_POINT('Ctrl Pts',(14.6513711852839,-17.1452153999142,
12.));
#221372=CARTESIAN_POINT('Ctrl Pts',(14.6513681262571,-17.1452095830633,
0.));
#221373=CARTESIAN_POINT('Ctrl Pts',(14.6513681262571,-17.1452095830633,
12.));
#221374=CARTESIAN_POINT('',(17.9112098770111,-18.8464468996588,0.));
#221375=CARTESIAN_POINT('Ctrl Pts',(17.9112098770111,-18.8464468996588,
0.));
#221376=CARTESIAN_POINT('Ctrl Pts',(17.9057348246595,-18.8448126709692,
0.));
#221377=CARTESIAN_POINT('Ctrl Pts',(17.8947931177807,-18.8415402351786,
0.));
#221378=CARTESIAN_POINT('Ctrl Pts',(17.8784057509355,-18.8366196462581,
0.));
#221379=CARTESIAN_POINT('Ctrl Pts',(17.856606317477,-18.8300349895974,0.));
#221380=CARTESIAN_POINT('Ctrl Pts',(17.8294410311006,-18.8217643886157,
0.));
#221381=CARTESIAN_POINT('Ctrl Pts',(17.8023598011057,-18.8134540340417,
0.));
#221382=CARTESIAN_POINT('Ctrl Pts',(17.7753627137853,-18.8051039860448,
0.));
#221383=CARTESIAN_POINT('Ctrl Pts',(17.7484498996905,-18.7967143519419,
0.));
#221384=CARTESIAN_POINT('Ctrl Pts',(17.7216215409035,-18.788285297605,0.));
#221385=CARTESIAN_POINT('Ctrl Pts',(17.6948778823014,-18.7798170641374,
0.));
#221386=CARTESIAN_POINT('Ctrl Pts',(17.6682192274236,-18.7713099642754,
0.));
#221387=CARTESIAN_POINT('Ctrl Pts',(17.6416459210681,-18.762764361321,0.));
#221388=CARTESIAN_POINT('Ctrl Pts',(17.6151583357012,-18.7541806530984,
0.));
#221389=CARTESIAN_POINT('Ctrl Pts',(17.5887568561371,-18.7455592536688,
0.));
#221390=CARTESIAN_POINT('Ctrl Pts',(17.5624418653245,-18.7369005764553,
0.));
#221391=CARTESIAN_POINT('Ctrl Pts',(17.5362137287593,-18.7282050157138,
0.));
#221392=CARTESIAN_POINT('Ctrl Pts',(17.5100727820876,-18.7194729318098,
0.));
#221393=CARTESIAN_POINT('Ctrl Pts',(17.4840193397162,-18.7107046613912,
0.));
#221394=CARTESIAN_POINT('Ctrl Pts',(17.4580537012753,-18.70190052503,0.));
#221395=CARTESIAN_POINT('Ctrl Pts',(17.4321761588142,-18.6930608357409,
0.));
#221396=CARTESIAN_POINT('Ctrl Pts',(17.4063870038562,-18.6841859073471,
0.));
#221397=CARTESIAN_POINT('Ctrl Pts',(17.3806865340747,-18.6752760624052,
0.));
#221398=CARTESIAN_POINT('Ctrl Pts',(17.3550750612443,-18.6663316416582,
0.));
#221399=CARTESIAN_POINT('Ctrl Pts',(17.3295529098618,-18.6573530024033,
0.));
#221400=CARTESIAN_POINT('Ctrl Pts',(17.3041204135074,-18.6483405141865,
0.));
#221401=CARTESIAN_POINT('Ctrl Pts',(17.2787779120213,-18.6392945554748,
0.));
#221402=CARTESIAN_POINT('Ctrl Pts',(17.2535257482187,-18.6302155097943,
0.));
#221403=CARTESIAN_POINT('Ctrl Pts',(17.2283642650517,-18.6211037624038,
0.));
#221404=CARTESIAN_POINT('Ctrl Pts',(17.2032938019284,-18.6119596959949,
0.));
#221405=CARTESIAN_POINT('Ctrl Pts',(17.1783146940127,-18.6027836898817,
0.));
#221406=CARTESIAN_POINT('Ctrl Pts',(17.1534272741643,-18.5935761222825,
0.));
#221407=CARTESIAN_POINT('Ctrl Pts',(17.1286318741183,-18.5843373717247,
0.));
#221408=CARTESIAN_POINT('Ctrl Pts',(17.1039288260001,-18.5750678188542,
0.));
#221409=CARTESIAN_POINT('Ctrl Pts',(17.0793184636079,-18.5657678479789,
0.));
#221410=CARTESIAN_POINT('Ctrl Pts',(17.0548011239751,-18.556437848963,0.));
#221411=CARTESIAN_POINT('Ctrl Pts',(17.0303771481738,-18.547078218209,0.));
#221412=CARTESIAN_POINT('Ctrl Pts',(17.0060468805097,-18.5376893576961,
0.));
#221413=CARTESIAN_POINT('Ctrl Pts',(16.981810668038,-18.5282716744197,0.));
#221414=CARTESIAN_POINT('Ctrl Pts',(16.9576688599339,-18.5188255796659,
0.));
#221415=CARTESIAN_POINT('Ctrl Pts',(16.9336218069353,-18.5093514883835,
0.));
#221416=CARTESIAN_POINT('Ctrl Pts',(16.9096698606943,-18.499849818462,0.));
#221417=CARTESIAN_POINT('Ctrl Pts',(16.8858133733088,-18.4903209902227,
0.));
#221418=CARTESIAN_POINT('Ctrl Pts',(16.8620526977171,-18.4807654268771,
0.));
#221419=CARTESIAN_POINT('Ctrl Pts',(16.8383881879709,-18.4711835548623,
0.));
#221420=CARTESIAN_POINT('Ctrl Pts',(16.8148201995472,-18.4615758042305,
0.));
#221421=CARTESIAN_POINT('Ctrl Pts',(16.791349089629,-18.4519426090124,0.));
#221422=CARTESIAN_POINT('Ctrl Pts',(16.7679752173992,-18.44228440761,0.));
#221423=CARTESIAN_POINT('Ctrl Pts',(16.7446989442882,-18.4326016431392,
0.));
#221424=CARTESIAN_POINT('Ctrl Pts',(16.7215206338818,-18.4228947633187,
0.));
#221425=CARTESIAN_POINT('Ctrl Pts',(16.698440651849,-18.413164220399,0.));
#221426=CARTESIAN_POINT('Ctrl Pts',(16.6754593658513,-18.403410471079,0.));
#221427=CARTESIAN_POINT('Ctrl Pts',(16.6525771454513,-18.3936339764332,
0.));
#221428=CARTESIAN_POINT('Ctrl Pts',(16.6297943620056,-18.3838352018327,
0.));
#221429=CARTESIAN_POINT('Ctrl Pts',(16.607111388571,-18.3740146168879,0.));
#221430=CARTESIAN_POINT('Ctrl Pts',(16.5845286000217,-18.3641726955889,
0.));
#221431=CARTESIAN_POINT('Ctrl Pts',(16.5620463731413,-18.354309916433,0.));
#221432=CARTESIAN_POINT('Ctrl Pts',(16.5396650867139,-18.34442676256,0.));
#221433=CARTESIAN_POINT('Ctrl Pts',(16.5173851216045,-18.3345237218864,
0.));
#221434=CARTESIAN_POINT('Ctrl Pts',(16.4952068608345,-18.3246012872469,
0.));
#221435=CARTESIAN_POINT('Ctrl Pts',(16.4731306896441,-18.3146599565231,
0.));
#221436=CARTESIAN_POINT('Ctrl Pts',(16.4511569955233,-18.304700232686,0.));
#221437=CARTESIAN_POINT('Ctrl Pts',(16.4292861682378,-18.294722623851,0.));
#221438=CARTESIAN_POINT('Ctrl Pts',(16.4075185998454,-18.2847276433309,
0.));
#221439=CARTESIAN_POINT('Ctrl Pts',(16.385854684708,-18.2747158096934,0.));
#221440=CARTESIAN_POINT('Ctrl Pts',(16.3642948194868,-18.2646876468169,
0.));
#221441=CARTESIAN_POINT('Ctrl Pts',(16.3428394031589,-18.2546436839608,
0.));
#221442=CARTESIAN_POINT('Ctrl Pts',(16.3214888370987,-18.2445844558742,
0.));
#221443=CARTESIAN_POINT('Ctrl Pts',(16.3002435251378,-18.2345105028982,
0.));
#221444=CARTESIAN_POINT('Ctrl Pts',(16.2791038736223,-18.2244223710746,
0.));
#221445=CARTESIAN_POINT('Ctrl Pts',(16.2580702914615,-18.2143206122529,
0.));
#221446=CARTESIAN_POINT('Ctrl Pts',(16.2371431901638,-18.2042057842035,
0.));
#221447=CARTESIAN_POINT('Ctrl Pts',(16.2163229838875,-18.1940784507229,
0.));
#221448=CARTESIAN_POINT('Ctrl Pts',(16.1956100895073,-18.1839391817331,
0.));
#221449=CARTESIAN_POINT('Ctrl Pts',(16.1750049266671,-18.1737885533849,
0.));
#221450=CARTESIAN_POINT('Ctrl Pts',(16.154507917826,-18.1636271481615,0.));
#221451=CARTESIAN_POINT('Ctrl Pts',(16.1341194882988,-18.1534555549853,
0.));
#221452=CARTESIAN_POINT('Ctrl Pts',(16.1138400662794,-18.1432743693235,
0.));
#221453=CARTESIAN_POINT('Ctrl Pts',(16.0936700829112,-18.1330841933105,
0.));
#221454=CARTESIAN_POINT('Ctrl Pts',(16.0736099723668,-18.1228856358751,
0.));
#221455=CARTESIAN_POINT('Ctrl Pts',(16.0536601719125,-18.112679312869,0.));
#221456=CARTESIAN_POINT('Ctrl Pts',(16.0338211219693,-18.1024658471966,
0.));
#221457=CARTESIAN_POINT('Ctrl Pts',(16.014093266161,-18.0922458689462,0.));
#221458=CARTESIAN_POINT('Ctrl Pts',(15.9944770513613,-18.0820200155236,
0.));
#221459=CARTESIAN_POINT('Ctrl Pts',(15.9749729277846,-18.0717889317958,
0.));
#221460=CARTESIAN_POINT('Ctrl Pts',(15.9555813490644,-18.061553270236,0.));
#221461=CARTESIAN_POINT('Ctrl Pts',(15.9363027723244,-18.0513136910691,
0.));
#221462=CARTESIAN_POINT('Ctrl Pts',(15.9171376582436,-18.0410708624209,
0.));
#221463=CARTESIAN_POINT('Ctrl Pts',(15.8980864711042,-18.0308254604636,
0.));
#221464=CARTESIAN_POINT('Ctrl Pts',(15.8791496788682,-18.0205781695769,
0.));
#221465=CARTESIAN_POINT('Ctrl Pts',(15.8603277532831,-18.0103296825205,
0.));
#221466=CARTESIAN_POINT('Ctrl Pts',(15.8416211699679,-18.0000807006052,
0.));
#221467=CARTESIAN_POINT('Ctrl Pts',(15.8230304084962,-17.9898319338665,
0.));
#221468=CARTESIAN_POINT('Ctrl Pts',(15.8045559524676,-17.9795841012386,
0.));
#221469=CARTESIAN_POINT('Ctrl Pts',(15.7861982895724,-17.9693379307303,
0.));
#221470=CARTESIAN_POINT('Ctrl Pts',(15.7679579117077,-17.9590941596242,
0.));
#221471=CARTESIAN_POINT('Ctrl Pts',(15.749835315086,-17.9488535346781,0.));
#221472=CARTESIAN_POINT('Ctrl Pts',(15.7318310003335,-17.9386168123262,
0.));
#221473=CARTESIAN_POINT('Ctrl Pts',(15.7139454725838,-17.9283847588836,
0.));
#221474=CARTESIAN_POINT('Ctrl Pts',(15.6961792415522,-17.9181581507455,
0.));
#221475=CARTESIAN_POINT('Ctrl Pts',(15.678532821646,-17.9079377746111,0.));
#221476=CARTESIAN_POINT('Ctrl Pts',(15.661006732103,-17.897724427724,0.));
#221477=CARTESIAN_POINT('Ctrl Pts',(15.6436014971084,-17.8875189181091,
0.));
#221478=CARTESIAN_POINT('Ctrl Pts',(15.6263176459108,-17.8773220648125,
0.));
#221479=CARTESIAN_POINT('Ctrl Pts',(15.609155712921,-17.8671346981394,0.));
#221480=CARTESIAN_POINT('Ctrl Pts',(15.5921162378192,-17.8569576599006,
0.));
#221481=CARTESIAN_POINT('Ctrl Pts',(15.5751997657162,-17.8467918036987,
0.));
#221482=CARTESIAN_POINT('Ctrl Pts',(15.5584068472982,-17.8366379952085,
0.));
#221483=CARTESIAN_POINT('Ctrl Pts',(15.541738038964,-17.8264971124607,0.));
#221484=CARTESIAN_POINT('Ctrl Pts',(15.5251939029552,-17.8163700461256,
0.));
#221485=CARTESIAN_POINT('Ctrl Pts',(15.5087750074718,-17.8062576997952,
0.));
#221486=CARTESIAN_POINT('Ctrl Pts',(15.4924819268517,-17.7961609903148,
0.));
#221487=CARTESIAN_POINT('Ctrl Pts',(15.4763152417497,-17.786080848122,0.));
#221488=CARTESIAN_POINT('Ctrl Pts',(15.4602755393017,-17.7760182175815,
0.));
#221489=CARTESIAN_POINT('Ctrl Pts',(15.4443634132869,-17.7659740573265,
0.));
#221490=CARTESIAN_POINT('Ctrl Pts',(15.4285794642667,-17.7559493405881,
0.));
#221491=CARTESIAN_POINT('Ctrl Pts',(15.4129242997837,-17.7459450555813,
0.));
#221492=CARTESIAN_POINT('Ctrl Pts',(15.3973985345802,-17.735962205915,0.));
#221493=CARTESIAN_POINT('Ctrl Pts',(15.3820027907966,-17.7260018109924,
0.));
#221494=CARTESIAN_POINT('Ctrl Pts',(15.3667376981699,-17.7160649064206,
0.));
#221495=CARTESIAN_POINT('Ctrl Pts',(15.351603894206,-17.7061525444042,0.));
#221496=CARTESIAN_POINT('Ctrl Pts',(15.3366020244066,-17.6962657941983,
0.));
#221497=CARTESIAN_POINT('Ctrl Pts',(15.3217327425338,-17.6864057426052,
0.));
#221498=CARTESIAN_POINT('Ctrl Pts',(15.30699671085,-17.676573494456,0.));
#221499=CARTESIAN_POINT('Ctrl Pts',(15.2923946003598,-17.6667701731041,
0.));
#221500=CARTESIAN_POINT('Ctrl Pts',(15.2779270910239,-17.6569969209,0.));
#221501=CARTESIAN_POINT('Ctrl Pts',(15.2635948720292,-17.6472548997328,
0.));
#221502=CARTESIAN_POINT('Ctrl Pts',(15.2493986421092,-17.6375452916369,
0.));
#221503=CARTESIAN_POINT('Ctrl Pts',(15.2353391098366,-17.6278692993764,
0.));
#221504=CARTESIAN_POINT('Ctrl Pts',(15.2214169939199,-17.6182281470468,
0.));
#221505=CARTESIAN_POINT('Ctrl Pts',(15.2076330234686,-17.60862308065,0.));
#221506=CARTESIAN_POINT('Ctrl Pts',(15.1939879383268,-17.5990553687599,
0.));
#221507=CARTESIAN_POINT('Ctrl Pts',(15.1804824894605,-17.5895263032595,
0.));
#221508=CARTESIAN_POINT('Ctrl Pts',(15.1671174393137,-17.580037200054,0.));
#221509=CARTESIAN_POINT('Ctrl Pts',(15.1538935621714,-17.5705893998029,
0.));
#221510=CARTESIAN_POINT('Ctrl Pts',(15.1408116444876,-17.5611842686192,
0.));
#221511=CARTESIAN_POINT('Ctrl Pts',(15.1278724853138,-17.5518231989117,
0.));
#221512=CARTESIAN_POINT('Ctrl Pts',(15.1150768967728,-17.5425076102963,
0.));
#221513=CARTESIAN_POINT('Ctrl Pts',(15.1024257045033,-17.5332389504829,
0.));
#221514=CARTESIAN_POINT('Ctrl Pts',(15.0899197481082,-17.5240186961791,
0.));
#221515=CARTESIAN_POINT('Ctrl Pts',(15.0775598815749,-17.5148483539687,
0.));
#221516=CARTESIAN_POINT('Ctrl Pts',(15.0653469738307,-17.5057294613877,
0.));
#221517=CARTESIAN_POINT('Ctrl Pts',(15.0532819093085,-17.4966635880246,
0.));
#221518=CARTESIAN_POINT('Ctrl Pts',(15.0413655884993,-17.4876523366178,
0.));
#221519=CARTESIAN_POINT('Ctrl Pts',(15.029598928488,-17.4786973441417,0.));
#221520=CARTESIAN_POINT('Ctrl Pts',(15.0179828635087,-17.4698002829357,
0.));
#221521=CARTESIAN_POINT('Ctrl Pts',(15.0065183456922,-17.4609628621419,
0.));
#221522=CARTESIAN_POINT('Ctrl Pts',(14.9952063457779,-17.4521868291005,
0.));
#221523=CARTESIAN_POINT('Ctrl Pts',(14.9840478538357,-17.4434739707773,
0.));
#221524=CARTESIAN_POINT('Ctrl Pts',(14.973043879945,-17.4348261151395,0.));
#221525=CARTESIAN_POINT('Ctrl Pts',(14.9621954549825,-17.4262451327088,
0.));
#221526=CARTESIAN_POINT('Ctrl Pts',(14.9515036315142,-17.4177329382827,
0.));
#221527=CARTESIAN_POINT('Ctrl Pts',(14.940969484645,-17.4092914926072,0.));
#221528=CARTESIAN_POINT('Ctrl Pts',(14.9305941128758,-17.400922804075,0.));
#221529=CARTESIAN_POINT('Ctrl Pts',(14.9203786389343,-17.3926289303987,
0.));
#221530=CARTESIAN_POINT('Ctrl Pts',(14.9103242110057,-17.3844119809823,
0.));
#221531=CARTESIAN_POINT('Ctrl Pts',(14.9004320039609,-17.3762741193075,
0.));
#221532=CARTESIAN_POINT('Ctrl Pts',(14.8907032205789,-17.3682175653236,
0.));
#221533=CARTESIAN_POINT('Ctrl Pts',(14.8811390927424,-17.3602445978163,
0.));
#221534=CARTESIAN_POINT('Ctrl Pts',(14.8717408826957,-17.3523575568648,
0.));
#221535=CARTESIAN_POINT('Ctrl Pts',(14.8625098843419,-17.3445588463477,
0.));
#221536=CARTESIAN_POINT('Ctrl Pts',(14.8534474245433,-17.336850936485,0.));
#221537=CARTESIAN_POINT('Ctrl Pts',(14.8445548643504,-17.3292363662601,
0.));
#221538=CARTESIAN_POINT('Ctrl Pts',(14.8358336004193,-17.3217177462096,
0.));
#221539=CARTESIAN_POINT('Ctrl Pts',(14.8272850675375,-17.3142977632656,
0.));
#221540=CARTESIAN_POINT('Ctrl Pts',(14.8189107410161,-17.3069791853705,
0.));
#221541=CARTESIAN_POINT('Ctrl Pts',(14.8107121391038,-17.2997648661483,
0.));
#221542=CARTESIAN_POINT('Ctrl Pts',(14.8026908254281,-17.2926577496519,
0.));
#221543=CARTESIAN_POINT('Ctrl Pts',(14.7948484105252,-17.28566087332,0.));
#221544=CARTESIAN_POINT('Ctrl Pts',(14.787186553128,-17.278777370485,0.));
#221545=CARTESIAN_POINT('Ctrl Pts',(14.7797069617802,-17.2720104735192,
0.));
#221546=CARTESIAN_POINT('Ctrl Pts',(14.7724113956728,-17.2653635155317,
0.));
#221547=CARTESIAN_POINT('Ctrl Pts',(14.7653016697589,-17.2588399401464,
0.));
#221548=CARTESIAN_POINT('Ctrl Pts',(14.7583796616617,-17.2524433146837,
0.));
#221549=CARTESIAN_POINT('Ctrl Pts',(14.7516473175124,-17.2461773413289,
0.));
#221550=CARTESIAN_POINT('Ctrl Pts',(14.7451066593793,-17.2400458713566,
0.));
#221551=CARTESIAN_POINT('Ctrl Pts',(14.7387597858117,-17.2340529062078,
0.));
#221552=CARTESIAN_POINT('Ctrl Pts',(14.7326088681163,-17.2282025904314,
0.));
#221553=CARTESIAN_POINT('Ctrl Pts',(14.7266561494282,-17.2224992099666,
0.));
#221554=CARTESIAN_POINT('Ctrl Pts',(14.7209039390325,-17.2169471814255,
0.));
#221555=CARTESIAN_POINT('Ctrl Pts',(14.7153546289338,-17.2115510835988,
0.));
#221556=CARTESIAN_POINT('Ctrl Pts',(14.7100107213586,-17.2063157097316,
0.));
#221557=CARTESIAN_POINT('Ctrl Pts',(14.7048748502662,-17.2012461084268,
0.));
#221558=CARTESIAN_POINT('Ctrl Pts',(14.699949811582,-17.1963476411694,0.));
#221559=CARTESIAN_POINT('Ctrl Pts',(14.6952385361706,-17.1916259308416,
0.));
#221560=CARTESIAN_POINT('Ctrl Pts',(14.6907440526957,-17.1870867909918,
0.));
#221561=CARTESIAN_POINT('Ctrl Pts',(14.6864694522319,-17.182736158472,0.));
#221562=CARTESIAN_POINT('Ctrl Pts',(14.6824178576166,-17.1785800350827,
0.));
#221563=CARTESIAN_POINT('Ctrl Pts',(14.6785925615676,-17.1746247499057,
0.));
#221564=CARTESIAN_POINT('Ctrl Pts',(14.6749971333867,-17.1708771619129,
0.));
#221565=CARTESIAN_POINT('Ctrl Pts',(14.6716355833321,-17.1673449723019,
0.));
#221566=CARTESIAN_POINT('Ctrl Pts',(14.6685123374424,-17.1640366762304,
0.));
#221567=CARTESIAN_POINT('Ctrl Pts',(14.6656319165057,-17.1609609517369,
0.));
#221568=CARTESIAN_POINT('Ctrl Pts',(14.662998728599,-17.1581262646789,0.));
#221569=CARTESIAN_POINT('Ctrl Pts',(14.660616716964,-17.1555401986403,0.));
#221570=CARTESIAN_POINT('Ctrl Pts',(14.65849005553,-17.1532107762719,0.));
#221571=CARTESIAN_POINT('Ctrl Pts',(14.6566237952435,-17.1511476869495,
0.));
#221572=CARTESIAN_POINT('Ctrl Pts',(14.6550248622813,-17.1493641837556,
0.));
#221573=CARTESIAN_POINT('Ctrl Pts',(14.6537016966188,-17.1478763944909,
0.));
#221574=CARTESIAN_POINT('Ctrl Pts',(14.6526624064978,-17.1466998098673,
0.));
#221575=CARTESIAN_POINT('Ctrl Pts',(14.65191316345,-17.1458462295273,0.));
#221576=CARTESIAN_POINT('Ctrl Pts',(14.6515481598057,-17.1454262858045,
0.));
#221577=CARTESIAN_POINT('Ctrl Pts',(14.6514066997188,-17.1452600887039,
0.));
#221578=CARTESIAN_POINT('Ctrl Pts',(14.6513711852839,-17.1452153999142,
0.));
#221579=CARTESIAN_POINT('Ctrl Pts',(14.6513681262571,-17.1452095830633,
0.));
#221580=CARTESIAN_POINT('',(17.9112098770111,-18.8464468996588,12.));
#221581=CARTESIAN_POINT('',(17.9112098770111,-18.8464468996588,0.));
#221582=CARTESIAN_POINT('Ctrl Pts',(14.6513681262571,-17.1452095830633,
12.));
#221583=CARTESIAN_POINT('Ctrl Pts',(14.6513711852839,-17.1452153999142,
12.));
#221584=CARTESIAN_POINT('Ctrl Pts',(14.6514066997188,-17.1452600887039,
12.));
#221585=CARTESIAN_POINT('Ctrl Pts',(14.6515481598057,-17.1454262858045,
12.));
#221586=CARTESIAN_POINT('Ctrl Pts',(14.65191316345,-17.1458462295273,12.));
#221587=CARTESIAN_POINT('Ctrl Pts',(14.6526624064978,-17.1466998098673,
12.));
#221588=CARTESIAN_POINT('Ctrl Pts',(14.6537016966188,-17.1478763944909,
12.));
#221589=CARTESIAN_POINT('Ctrl Pts',(14.6550248622813,-17.1493641837556,
12.));
#221590=CARTESIAN_POINT('Ctrl Pts',(14.6566237952435,-17.1511476869495,
12.));
#221591=CARTESIAN_POINT('Ctrl Pts',(14.65849005553,-17.1532107762719,12.));
#221592=CARTESIAN_POINT('Ctrl Pts',(14.660616716964,-17.1555401986403,12.));
#221593=CARTESIAN_POINT('Ctrl Pts',(14.662998728599,-17.1581262646789,12.));
#221594=CARTESIAN_POINT('Ctrl Pts',(14.6656319165057,-17.1609609517369,
12.));
#221595=CARTESIAN_POINT('Ctrl Pts',(14.6685123374424,-17.1640366762304,
12.));
#221596=CARTESIAN_POINT('Ctrl Pts',(14.6716355833321,-17.1673449723019,
12.));
#221597=CARTESIAN_POINT('Ctrl Pts',(14.6749971333867,-17.1708771619129,
12.));
#221598=CARTESIAN_POINT('Ctrl Pts',(14.6785925615676,-17.1746247499057,
12.));
#221599=CARTESIAN_POINT('Ctrl Pts',(14.6824178576166,-17.1785800350827,
12.));
#221600=CARTESIAN_POINT('Ctrl Pts',(14.6864694522319,-17.182736158472,12.));
#221601=CARTESIAN_POINT('Ctrl Pts',(14.6907440526957,-17.1870867909918,
12.));
#221602=CARTESIAN_POINT('Ctrl Pts',(14.6952385361706,-17.1916259308416,
12.));
#221603=CARTESIAN_POINT('Ctrl Pts',(14.699949811582,-17.1963476411694,12.));
#221604=CARTESIAN_POINT('Ctrl Pts',(14.7048748502662,-17.2012461084268,
12.));
#221605=CARTESIAN_POINT('Ctrl Pts',(14.7100107213586,-17.2063157097316,
12.));
#221606=CARTESIAN_POINT('Ctrl Pts',(14.7153546289338,-17.2115510835988,
12.));
#221607=CARTESIAN_POINT('Ctrl Pts',(14.7209039390325,-17.2169471814255,
12.));
#221608=CARTESIAN_POINT('Ctrl Pts',(14.7266561494282,-17.2224992099666,
12.));
#221609=CARTESIAN_POINT('Ctrl Pts',(14.7326088681163,-17.2282025904314,
12.));
#221610=CARTESIAN_POINT('Ctrl Pts',(14.7387597858117,-17.2340529062078,
12.));
#221611=CARTESIAN_POINT('Ctrl Pts',(14.7451066593793,-17.2400458713566,
12.));
#221612=CARTESIAN_POINT('Ctrl Pts',(14.7516473175124,-17.2461773413289,
12.));
#221613=CARTESIAN_POINT('Ctrl Pts',(14.7583796616617,-17.2524433146837,
12.));
#221614=CARTESIAN_POINT('Ctrl Pts',(14.7653016697589,-17.2588399401464,
12.));
#221615=CARTESIAN_POINT('Ctrl Pts',(14.7724113956728,-17.2653635155317,
12.));
#221616=CARTESIAN_POINT('Ctrl Pts',(14.7797069617802,-17.2720104735192,
12.));
#221617=CARTESIAN_POINT('Ctrl Pts',(14.787186553128,-17.278777370485,12.));
#221618=CARTESIAN_POINT('Ctrl Pts',(14.7948484105252,-17.28566087332,12.));
#221619=CARTESIAN_POINT('Ctrl Pts',(14.8026908254281,-17.2926577496519,
12.));
#221620=CARTESIAN_POINT('Ctrl Pts',(14.8107121391038,-17.2997648661483,
12.));
#221621=CARTESIAN_POINT('Ctrl Pts',(14.8189107410161,-17.3069791853705,
12.));
#221622=CARTESIAN_POINT('Ctrl Pts',(14.8272850675375,-17.3142977632656,
12.));
#221623=CARTESIAN_POINT('Ctrl Pts',(14.8358336004193,-17.3217177462096,
12.));
#221624=CARTESIAN_POINT('Ctrl Pts',(14.8445548643504,-17.3292363662601,
12.));
#221625=CARTESIAN_POINT('Ctrl Pts',(14.8534474245433,-17.336850936485,12.));
#221626=CARTESIAN_POINT('Ctrl Pts',(14.8625098843419,-17.3445588463477,
12.));
#221627=CARTESIAN_POINT('Ctrl Pts',(14.8717408826957,-17.3523575568648,
12.));
#221628=CARTESIAN_POINT('Ctrl Pts',(14.8811390927424,-17.3602445978163,
12.));
#221629=CARTESIAN_POINT('Ctrl Pts',(14.8907032205789,-17.3682175653236,
12.));
#221630=CARTESIAN_POINT('Ctrl Pts',(14.9004320039609,-17.3762741193075,
12.));
#221631=CARTESIAN_POINT('Ctrl Pts',(14.9103242110057,-17.3844119809823,
12.));
#221632=CARTESIAN_POINT('Ctrl Pts',(14.9203786389343,-17.3926289303987,
12.));
#221633=CARTESIAN_POINT('Ctrl Pts',(14.9305941128758,-17.400922804075,12.));
#221634=CARTESIAN_POINT('Ctrl Pts',(14.940969484645,-17.4092914926072,12.));
#221635=CARTESIAN_POINT('Ctrl Pts',(14.9515036315142,-17.4177329382827,
12.));
#221636=CARTESIAN_POINT('Ctrl Pts',(14.9621954549825,-17.4262451327088,
12.));
#221637=CARTESIAN_POINT('Ctrl Pts',(14.973043879945,-17.4348261151395,12.));
#221638=CARTESIAN_POINT('Ctrl Pts',(14.9840478538357,-17.4434739707773,
12.));
#221639=CARTESIAN_POINT('Ctrl Pts',(14.9952063457779,-17.4521868291005,
12.));
#221640=CARTESIAN_POINT('Ctrl Pts',(15.0065183456922,-17.4609628621419,
12.));
#221641=CARTESIAN_POINT('Ctrl Pts',(15.0179828635087,-17.4698002829357,
12.));
#221642=CARTESIAN_POINT('Ctrl Pts',(15.029598928488,-17.4786973441417,12.));
#221643=CARTESIAN_POINT('Ctrl Pts',(15.0413655884993,-17.4876523366178,
12.));
#221644=CARTESIAN_POINT('Ctrl Pts',(15.0532819093085,-17.4966635880246,
12.));
#221645=CARTESIAN_POINT('Ctrl Pts',(15.0653469738307,-17.5057294613877,
12.));
#221646=CARTESIAN_POINT('Ctrl Pts',(15.0775598815749,-17.5148483539687,
12.));
#221647=CARTESIAN_POINT('Ctrl Pts',(15.0899197481082,-17.5240186961791,
12.));
#221648=CARTESIAN_POINT('Ctrl Pts',(15.1024257045033,-17.5332389504829,
12.));
#221649=CARTESIAN_POINT('Ctrl Pts',(15.1150768967728,-17.5425076102963,
12.));
#221650=CARTESIAN_POINT('Ctrl Pts',(15.1278724853138,-17.5518231989117,
12.));
#221651=CARTESIAN_POINT('Ctrl Pts',(15.1408116444876,-17.5611842686192,
12.));
#221652=CARTESIAN_POINT('Ctrl Pts',(15.1538935621714,-17.5705893998029,
12.));
#221653=CARTESIAN_POINT('Ctrl Pts',(15.1671174393137,-17.580037200054,12.));
#221654=CARTESIAN_POINT('Ctrl Pts',(15.1804824894605,-17.5895263032595,
12.));
#221655=CARTESIAN_POINT('Ctrl Pts',(15.1939879383268,-17.5990553687599,
12.));
#221656=CARTESIAN_POINT('Ctrl Pts',(15.2076330234686,-17.60862308065,12.));
#221657=CARTESIAN_POINT('Ctrl Pts',(15.2214169939199,-17.6182281470468,
12.));
#221658=CARTESIAN_POINT('Ctrl Pts',(15.2353391098366,-17.6278692993764,
12.));
#221659=CARTESIAN_POINT('Ctrl Pts',(15.2493986421092,-17.6375452916369,
12.));
#221660=CARTESIAN_POINT('Ctrl Pts',(15.2635948720292,-17.6472548997328,
12.));
#221661=CARTESIAN_POINT('Ctrl Pts',(15.2779270910239,-17.6569969209,12.));
#221662=CARTESIAN_POINT('Ctrl Pts',(15.2923946003598,-17.6667701731041,
12.));
#221663=CARTESIAN_POINT('Ctrl Pts',(15.30699671085,-17.676573494456,12.));
#221664=CARTESIAN_POINT('Ctrl Pts',(15.3217327425338,-17.6864057426052,
12.));
#221665=CARTESIAN_POINT('Ctrl Pts',(15.3366020244066,-17.6962657941983,
12.));
#221666=CARTESIAN_POINT('Ctrl Pts',(15.351603894206,-17.7061525444042,12.));
#221667=CARTESIAN_POINT('Ctrl Pts',(15.3667376981699,-17.7160649064206,
12.));
#221668=CARTESIAN_POINT('Ctrl Pts',(15.3820027907966,-17.7260018109924,
12.));
#221669=CARTESIAN_POINT('Ctrl Pts',(15.3973985345802,-17.735962205915,12.));
#221670=CARTESIAN_POINT('Ctrl Pts',(15.4129242997837,-17.7459450555813,
12.));
#221671=CARTESIAN_POINT('Ctrl Pts',(15.4285794642667,-17.7559493405881,
12.));
#221672=CARTESIAN_POINT('Ctrl Pts',(15.4443634132869,-17.7659740573265,
12.));
#221673=CARTESIAN_POINT('Ctrl Pts',(15.4602755393017,-17.7760182175815,
12.));
#221674=CARTESIAN_POINT('Ctrl Pts',(15.4763152417497,-17.786080848122,12.));
#221675=CARTESIAN_POINT('Ctrl Pts',(15.4924819268517,-17.7961609903148,
12.));
#221676=CARTESIAN_POINT('Ctrl Pts',(15.5087750074718,-17.8062576997952,
12.));
#221677=CARTESIAN_POINT('Ctrl Pts',(15.5251939029552,-17.8163700461256,
12.));
#221678=CARTESIAN_POINT('Ctrl Pts',(15.541738038964,-17.8264971124607,12.));
#221679=CARTESIAN_POINT('Ctrl Pts',(15.5584068472982,-17.8366379952085,
12.));
#221680=CARTESIAN_POINT('Ctrl Pts',(15.5751997657162,-17.8467918036987,
12.));
#221681=CARTESIAN_POINT('Ctrl Pts',(15.5921162378192,-17.8569576599006,
12.));
#221682=CARTESIAN_POINT('Ctrl Pts',(15.609155712921,-17.8671346981394,12.));
#221683=CARTESIAN_POINT('Ctrl Pts',(15.6263176459108,-17.8773220648125,
12.));
#221684=CARTESIAN_POINT('Ctrl Pts',(15.6436014971084,-17.8875189181091,
12.));
#221685=CARTESIAN_POINT('Ctrl Pts',(15.661006732103,-17.897724427724,12.));
#221686=CARTESIAN_POINT('Ctrl Pts',(15.678532821646,-17.9079377746111,12.));
#221687=CARTESIAN_POINT('Ctrl Pts',(15.6961792415522,-17.9181581507455,
12.));
#221688=CARTESIAN_POINT('Ctrl Pts',(15.7139454725838,-17.9283847588836,
12.));
#221689=CARTESIAN_POINT('Ctrl Pts',(15.7318310003335,-17.9386168123262,
12.));
#221690=CARTESIAN_POINT('Ctrl Pts',(15.749835315086,-17.9488535346781,12.));
#221691=CARTESIAN_POINT('Ctrl Pts',(15.7679579117077,-17.9590941596242,
12.));
#221692=CARTESIAN_POINT('Ctrl Pts',(15.7861982895724,-17.9693379307303,
12.));
#221693=CARTESIAN_POINT('Ctrl Pts',(15.8045559524676,-17.9795841012386,
12.));
#221694=CARTESIAN_POINT('Ctrl Pts',(15.8230304084962,-17.9898319338665,
12.));
#221695=CARTESIAN_POINT('Ctrl Pts',(15.8416211699679,-18.0000807006052,
12.));
#221696=CARTESIAN_POINT('Ctrl Pts',(15.8603277532831,-18.0103296825205,
12.));
#221697=CARTESIAN_POINT('Ctrl Pts',(15.8791496788682,-18.0205781695769,
12.));
#221698=CARTESIAN_POINT('Ctrl Pts',(15.8980864711042,-18.0308254604636,
12.));
#221699=CARTESIAN_POINT('Ctrl Pts',(15.9171376582436,-18.0410708624209,
12.));
#221700=CARTESIAN_POINT('Ctrl Pts',(15.9363027723244,-18.0513136910691,
12.));
#221701=CARTESIAN_POINT('Ctrl Pts',(15.9555813490644,-18.061553270236,12.));
#221702=CARTESIAN_POINT('Ctrl Pts',(15.9749729277846,-18.0717889317958,
12.));
#221703=CARTESIAN_POINT('Ctrl Pts',(15.9944770513613,-18.0820200155236,
12.));
#221704=CARTESIAN_POINT('Ctrl Pts',(16.014093266161,-18.0922458689462,12.));
#221705=CARTESIAN_POINT('Ctrl Pts',(16.0338211219693,-18.1024658471966,
12.));
#221706=CARTESIAN_POINT('Ctrl Pts',(16.0536601719125,-18.112679312869,12.));
#221707=CARTESIAN_POINT('Ctrl Pts',(16.0736099723668,-18.1228856358751,
12.));
#221708=CARTESIAN_POINT('Ctrl Pts',(16.0936700829112,-18.1330841933105,
12.));
#221709=CARTESIAN_POINT('Ctrl Pts',(16.1138400662794,-18.1432743693235,
12.));
#221710=CARTESIAN_POINT('Ctrl Pts',(16.1341194882988,-18.1534555549853,
12.));
#221711=CARTESIAN_POINT('Ctrl Pts',(16.154507917826,-18.1636271481615,12.));
#221712=CARTESIAN_POINT('Ctrl Pts',(16.1750049266671,-18.1737885533849,
12.));
#221713=CARTESIAN_POINT('Ctrl Pts',(16.1956100895073,-18.1839391817331,
12.));
#221714=CARTESIAN_POINT('Ctrl Pts',(16.2163229838875,-18.1940784507229,
12.));
#221715=CARTESIAN_POINT('Ctrl Pts',(16.2371431901638,-18.2042057842035,
12.));
#221716=CARTESIAN_POINT('Ctrl Pts',(16.2580702914615,-18.2143206122529,
12.));
#221717=CARTESIAN_POINT('Ctrl Pts',(16.2791038736223,-18.2244223710746,
12.));
#221718=CARTESIAN_POINT('Ctrl Pts',(16.3002435251378,-18.2345105028982,
12.));
#221719=CARTESIAN_POINT('Ctrl Pts',(16.3214888370987,-18.2445844558742,
12.));
#221720=CARTESIAN_POINT('Ctrl Pts',(16.3428394031589,-18.2546436839608,
12.));
#221721=CARTESIAN_POINT('Ctrl Pts',(16.3642948194868,-18.2646876468169,
12.));
#221722=CARTESIAN_POINT('Ctrl Pts',(16.385854684708,-18.2747158096934,12.));
#221723=CARTESIAN_POINT('Ctrl Pts',(16.4075185998454,-18.2847276433309,
12.));
#221724=CARTESIAN_POINT('Ctrl Pts',(16.4292861682378,-18.294722623851,12.));
#221725=CARTESIAN_POINT('Ctrl Pts',(16.4511569955233,-18.304700232686,12.));
#221726=CARTESIAN_POINT('Ctrl Pts',(16.4731306896441,-18.3146599565231,
12.));
#221727=CARTESIAN_POINT('Ctrl Pts',(16.4952068608345,-18.3246012872469,
12.));
#221728=CARTESIAN_POINT('Ctrl Pts',(16.5173851216045,-18.3345237218864,
12.));
#221729=CARTESIAN_POINT('Ctrl Pts',(16.5396650867139,-18.34442676256,12.));
#221730=CARTESIAN_POINT('Ctrl Pts',(16.5620463731413,-18.354309916433,12.));
#221731=CARTESIAN_POINT('Ctrl Pts',(16.5845286000217,-18.3641726955889,
12.));
#221732=CARTESIAN_POINT('Ctrl Pts',(16.607111388571,-18.3740146168879,12.));
#221733=CARTESIAN_POINT('Ctrl Pts',(16.6297943620056,-18.3838352018327,
12.));
#221734=CARTESIAN_POINT('Ctrl Pts',(16.6525771454513,-18.3936339764332,
12.));
#221735=CARTESIAN_POINT('Ctrl Pts',(16.6754593658513,-18.403410471079,12.));
#221736=CARTESIAN_POINT('Ctrl Pts',(16.698440651849,-18.413164220399,12.));
#221737=CARTESIAN_POINT('Ctrl Pts',(16.7215206338818,-18.4228947633187,
12.));
#221738=CARTESIAN_POINT('Ctrl Pts',(16.7446989442882,-18.4326016431392,
12.));
#221739=CARTESIAN_POINT('Ctrl Pts',(16.7679752173992,-18.44228440761,12.));
#221740=CARTESIAN_POINT('Ctrl Pts',(16.791349089629,-18.4519426090124,12.));
#221741=CARTESIAN_POINT('Ctrl Pts',(16.8148201995472,-18.4615758042305,
12.));
#221742=CARTESIAN_POINT('Ctrl Pts',(16.8383881879709,-18.4711835548623,
12.));
#221743=CARTESIAN_POINT('Ctrl Pts',(16.8620526977171,-18.4807654268771,
12.));
#221744=CARTESIAN_POINT('Ctrl Pts',(16.8858133733088,-18.4903209902227,
12.));
#221745=CARTESIAN_POINT('Ctrl Pts',(16.9096698606943,-18.499849818462,12.));
#221746=CARTESIAN_POINT('Ctrl Pts',(16.9336218069353,-18.5093514883835,
12.));
#221747=CARTESIAN_POINT('Ctrl Pts',(16.9576688599339,-18.5188255796659,
12.));
#221748=CARTESIAN_POINT('Ctrl Pts',(16.981810668038,-18.5282716744197,12.));
#221749=CARTESIAN_POINT('Ctrl Pts',(17.0060468805097,-18.5376893576961,
12.));
#221750=CARTESIAN_POINT('Ctrl Pts',(17.0303771481738,-18.547078218209,12.));
#221751=CARTESIAN_POINT('Ctrl Pts',(17.0548011239751,-18.556437848963,12.));
#221752=CARTESIAN_POINT('Ctrl Pts',(17.0793184636079,-18.5657678479789,
12.));
#221753=CARTESIAN_POINT('Ctrl Pts',(17.1039288260001,-18.5750678188542,
12.));
#221754=CARTESIAN_POINT('Ctrl Pts',(17.1286318741183,-18.5843373717247,
12.));
#221755=CARTESIAN_POINT('Ctrl Pts',(17.1534272741643,-18.5935761222825,
12.));
#221756=CARTESIAN_POINT('Ctrl Pts',(17.1783146940127,-18.6027836898817,
12.));
#221757=CARTESIAN_POINT('Ctrl Pts',(17.2032938019284,-18.6119596959949,
12.));
#221758=CARTESIAN_POINT('Ctrl Pts',(17.2283642650517,-18.6211037624038,
12.));
#221759=CARTESIAN_POINT('Ctrl Pts',(17.2535257482187,-18.6302155097943,
12.));
#221760=CARTESIAN_POINT('Ctrl Pts',(17.2787779120213,-18.6392945554748,
12.));
#221761=CARTESIAN_POINT('Ctrl Pts',(17.3041204135074,-18.6483405141865,
12.));
#221762=CARTESIAN_POINT('Ctrl Pts',(17.3295529098618,-18.6573530024033,
12.));
#221763=CARTESIAN_POINT('Ctrl Pts',(17.3550750612443,-18.6663316416582,
12.));
#221764=CARTESIAN_POINT('Ctrl Pts',(17.3806865340747,-18.6752760624052,
12.));
#221765=CARTESIAN_POINT('Ctrl Pts',(17.4063870038562,-18.6841859073471,
12.));
#221766=CARTESIAN_POINT('Ctrl Pts',(17.4321761588142,-18.6930608357409,
12.));
#221767=CARTESIAN_POINT('Ctrl Pts',(17.4580537012753,-18.70190052503,12.));
#221768=CARTESIAN_POINT('Ctrl Pts',(17.4840193397162,-18.7107046613912,
12.));
#221769=CARTESIAN_POINT('Ctrl Pts',(17.5100727820876,-18.7194729318098,
12.));
#221770=CARTESIAN_POINT('Ctrl Pts',(17.5362137287593,-18.7282050157138,
12.));
#221771=CARTESIAN_POINT('Ctrl Pts',(17.5624418653245,-18.7369005764553,
12.));
#221772=CARTESIAN_POINT('Ctrl Pts',(17.5887568561371,-18.7455592536688,
12.));
#221773=CARTESIAN_POINT('Ctrl Pts',(17.6151583357012,-18.7541806530984,
12.));
#221774=CARTESIAN_POINT('Ctrl Pts',(17.6416459210681,-18.762764361321,12.));
#221775=CARTESIAN_POINT('Ctrl Pts',(17.6682192274236,-18.7713099642754,
12.));
#221776=CARTESIAN_POINT('Ctrl Pts',(17.6948778823014,-18.7798170641374,
12.));
#221777=CARTESIAN_POINT('Ctrl Pts',(17.7216215409035,-18.788285297605,12.));
#221778=CARTESIAN_POINT('Ctrl Pts',(17.7484498996905,-18.7967143519419,
12.));
#221779=CARTESIAN_POINT('Ctrl Pts',(17.7753627137853,-18.8051039860448,
12.));
#221780=CARTESIAN_POINT('Ctrl Pts',(17.8023598011057,-18.8134540340417,
12.));
#221781=CARTESIAN_POINT('Ctrl Pts',(17.8294410311006,-18.8217643886157,
12.));
#221782=CARTESIAN_POINT('Ctrl Pts',(17.856606317477,-18.8300349895974,12.));
#221783=CARTESIAN_POINT('Ctrl Pts',(17.8784057509355,-18.8366196462581,
12.));
#221784=CARTESIAN_POINT('Ctrl Pts',(17.8947931177807,-18.8415402351786,
12.));
#221785=CARTESIAN_POINT('Ctrl Pts',(17.9057348246595,-18.8448126709692,
12.));
#221786=CARTESIAN_POINT('Ctrl Pts',(17.9112098770111,-18.8464468996588,
12.));
#221787=CARTESIAN_POINT('Ctrl Pts',(12.7689476255362,-18.5896416359912,
0.));
#221788=CARTESIAN_POINT('Ctrl Pts',(12.7689476255362,-18.5896416359912,
12.));
#221789=CARTESIAN_POINT('Ctrl Pts',(12.7689524524483,-18.5896460962964,
0.));
#221790=CARTESIAN_POINT('Ctrl Pts',(12.7689524524483,-18.5896460962964,
12.));
#221791=CARTESIAN_POINT('Ctrl Pts',(12.768986426692,-18.5896919669165,0.));
#221792=CARTESIAN_POINT('Ctrl Pts',(12.768986426692,-18.5896919669165,12.));
#221793=CARTESIAN_POINT('Ctrl Pts',(12.769110348199,-18.589871621843,0.));
#221794=CARTESIAN_POINT('Ctrl Pts',(12.769110348199,-18.589871621843,12.));
#221795=CARTESIAN_POINT('Ctrl Pts',(12.7694215127918,-18.5903328777227,
0.));
#221796=CARTESIAN_POINT('Ctrl Pts',(12.7694215127918,-18.5903328777227,
12.));
#221797=CARTESIAN_POINT('Ctrl Pts',(12.7700520897173,-18.5912775137806,
0.));
#221798=CARTESIAN_POINT('Ctrl Pts',(12.7700520897173,-18.5912775137806,
12.));
#221799=CARTESIAN_POINT('Ctrl Pts',(12.7709195951156,-18.5925859134579,
0.));
#221800=CARTESIAN_POINT('Ctrl Pts',(12.7709195951156,-18.5925859134579,
12.));
#221801=CARTESIAN_POINT('Ctrl Pts',(12.7720142287172,-18.5942490615407,
0.));
#221802=CARTESIAN_POINT('Ctrl Pts',(12.7720142287172,-18.5942490615407,
12.));
#221803=CARTESIAN_POINT('Ctrl Pts',(12.7733231262108,-18.5962551167772,
0.));
#221804=CARTESIAN_POINT('Ctrl Pts',(12.7733231262108,-18.5962551167772,
12.));
#221805=CARTESIAN_POINT('Ctrl Pts',(12.7748328937638,-18.598591752595,0.));
#221806=CARTESIAN_POINT('Ctrl Pts',(12.7748328937638,-18.598591752595,12.));
#221807=CARTESIAN_POINT('Ctrl Pts',(12.7765325225081,-18.6012488486709,
0.));
#221808=CARTESIAN_POINT('Ctrl Pts',(12.7765325225081,-18.6012488486709,
12.));
#221809=CARTESIAN_POINT('Ctrl Pts',(12.7784139605066,-18.6042190183704,
0.));
#221810=CARTESIAN_POINT('Ctrl Pts',(12.7784139605066,-18.6042190183704,
12.));
#221811=CARTESIAN_POINT('Ctrl Pts',(12.7804705387658,-18.6074961535723,
0.));
#221812=CARTESIAN_POINT('Ctrl Pts',(12.7804705387658,-18.6074961535723,
12.));
#221813=CARTESIAN_POINT('Ctrl Pts',(12.7826959526924,-18.611074482622,0.));
#221814=CARTESIAN_POINT('Ctrl Pts',(12.7826959526924,-18.611074482622,12.));
#221815=CARTESIAN_POINT('Ctrl Pts',(12.7850831657901,-18.6149475565188,
0.));
#221816=CARTESIAN_POINT('Ctrl Pts',(12.7850831657901,-18.6149475565188,
12.));
#221817=CARTESIAN_POINT('Ctrl Pts',(12.7876249657834,-18.6191087624752,
0.));
#221818=CARTESIAN_POINT('Ctrl Pts',(12.7876249657834,-18.6191087624752,
12.));
#221819=CARTESIAN_POINT('Ctrl Pts',(12.7903142925234,-18.6235516265575,
0.));
#221820=CARTESIAN_POINT('Ctrl Pts',(12.7903142925234,-18.6235516265575,
12.));
#221821=CARTESIAN_POINT('Ctrl Pts',(12.7931447451555,-18.6282702819371,
0.));
#221822=CARTESIAN_POINT('Ctrl Pts',(12.7931447451555,-18.6282702819371,
12.));
#221823=CARTESIAN_POINT('Ctrl Pts',(12.796110622225,-18.6332595057006,0.));
#221824=CARTESIAN_POINT('Ctrl Pts',(12.796110622225,-18.6332595057006,12.));
#221825=CARTESIAN_POINT('Ctrl Pts',(12.7992066625264,-18.63851447924,0.));
#221826=CARTESIAN_POINT('Ctrl Pts',(12.7992066625264,-18.63851447924,12.));
#221827=CARTESIAN_POINT('Ctrl Pts',(12.8024278770152,-18.6440306327456,
0.));
#221828=CARTESIAN_POINT('Ctrl Pts',(12.8024278770152,-18.6440306327456,
12.));
#221829=CARTESIAN_POINT('Ctrl Pts',(12.805769331162,-18.6498034438987,0.));
#221830=CARTESIAN_POINT('Ctrl Pts',(12.805769331162,-18.6498034438987,12.));
#221831=CARTESIAN_POINT('Ctrl Pts',(12.8092261933858,-18.6558284825773,
0.));
#221832=CARTESIAN_POINT('Ctrl Pts',(12.8092261933858,-18.6558284825773,
12.));
#221833=CARTESIAN_POINT('Ctrl Pts',(12.8127937909631,-18.6621014624746,
0.));
#221834=CARTESIAN_POINT('Ctrl Pts',(12.8127937909631,-18.6621014624746,
12.));
#221835=CARTESIAN_POINT('Ctrl Pts',(12.8164676687362,-18.66861829528,0.));
#221836=CARTESIAN_POINT('Ctrl Pts',(12.8164676687362,-18.66861829528,12.));
#221837=CARTESIAN_POINT('Ctrl Pts',(12.8202436318474,-18.6753751301092,
0.));
#221838=CARTESIAN_POINT('Ctrl Pts',(12.8202436318474,-18.6753751301092,
12.));
#221839=CARTESIAN_POINT('Ctrl Pts',(12.8241176980017,-18.6823683094139,
0.));
#221840=CARTESIAN_POINT('Ctrl Pts',(12.8241176980017,-18.6823683094139,
12.));
#221841=CARTESIAN_POINT('Ctrl Pts',(12.8280860635231,-18.6895943376172,
0.));
#221842=CARTESIAN_POINT('Ctrl Pts',(12.8280860635231,-18.6895943376172,
12.));
#221843=CARTESIAN_POINT('Ctrl Pts',(12.8321450599789,-18.6970498410172,
0.));
#221844=CARTESIAN_POINT('Ctrl Pts',(12.8321450599789,-18.6970498410172,
12.));
#221845=CARTESIAN_POINT('Ctrl Pts',(12.8362911280361,-18.7047315436294,
0.));
#221846=CARTESIAN_POINT('Ctrl Pts',(12.8362911280361,-18.7047315436294,
12.));
#221847=CARTESIAN_POINT('Ctrl Pts',(12.8405208263431,-18.7126362754445,
0.));
#221848=CARTESIAN_POINT('Ctrl Pts',(12.8405208263431,-18.7126362754445,
12.));
#221849=CARTESIAN_POINT('Ctrl Pts',(12.8448308329494,-18.7207609737702,
0.));
#221850=CARTESIAN_POINT('Ctrl Pts',(12.8448308329494,-18.7207609737702,
12.));
#221851=CARTESIAN_POINT('Ctrl Pts',(12.8492179511591,-18.7291026886554,
0.));
#221852=CARTESIAN_POINT('Ctrl Pts',(12.8492179511591,-18.7291026886554,
12.));
#221853=CARTESIAN_POINT('Ctrl Pts',(12.8536791086316,-18.7376585820854,
0.));
#221854=CARTESIAN_POINT('Ctrl Pts',(12.8536791086316,-18.7376585820854,
12.));
#221855=CARTESIAN_POINT('Ctrl Pts',(12.8582113455646,-18.7464259171251,
0.));
#221856=CARTESIAN_POINT('Ctrl Pts',(12.8582113455646,-18.7464259171251,
12.));
#221857=CARTESIAN_POINT('Ctrl Pts',(12.8628118054171,-18.7554020493887,
0.));
#221858=CARTESIAN_POINT('Ctrl Pts',(12.8628118054171,-18.7554020493887,
12.));
#221859=CARTESIAN_POINT('Ctrl Pts',(12.8674777239653,-18.7645844169564,
0.));
#221860=CARTESIAN_POINT('Ctrl Pts',(12.8674777239653,-18.7645844169564,
12.));
#221861=CARTESIAN_POINT('Ctrl Pts',(12.872206421181,-18.7739705329022,0.));
#221862=CARTESIAN_POINT('Ctrl Pts',(12.872206421181,-18.7739705329022,12.));
#221863=CARTESIAN_POINT('Ctrl Pts',(12.8769952998095,-18.7835579840477,
0.));
#221864=CARTESIAN_POINT('Ctrl Pts',(12.8769952998095,-18.7835579840477,
12.));
#221865=CARTESIAN_POINT('Ctrl Pts',(12.8818418427475,-18.7933444285868,
0.));
#221866=CARTESIAN_POINT('Ctrl Pts',(12.8818418427475,-18.7933444285868,
12.));
#221867=CARTESIAN_POINT('Ctrl Pts',(12.8867436109546,-18.8033275941943,
0.));
#221868=CARTESIAN_POINT('Ctrl Pts',(12.8867436109546,-18.8033275941943,
12.));
#221869=CARTESIAN_POINT('Ctrl Pts',(12.8916982409935,-18.813505275782,0.));
#221870=CARTESIAN_POINT('Ctrl Pts',(12.8916982409935,-18.813505275782,12.));
#221871=CARTESIAN_POINT('Ctrl Pts',(12.8967034410754,-18.8238753319129,
0.));
#221872=CARTESIAN_POINT('Ctrl Pts',(12.8967034410754,-18.8238753319129,
12.));
#221873=CARTESIAN_POINT('Ctrl Pts',(12.9017569871738,-18.8344356812591,
0.));
#221874=CARTESIAN_POINT('Ctrl Pts',(12.9017569871738,-18.8344356812591,
12.));
#221875=CARTESIAN_POINT('Ctrl Pts',(12.9068567191854,-18.8451842990984,
0.));
#221876=CARTESIAN_POINT('Ctrl Pts',(12.9068567191854,-18.8451842990984,
12.));
#221877=CARTESIAN_POINT('Ctrl Pts',(12.9120005369063,-18.8561192136198,
0.));
#221878=CARTESIAN_POINT('Ctrl Pts',(12.9120005369063,-18.8561192136198,
12.));
#221879=CARTESIAN_POINT('Ctrl Pts',(12.9171863977045,-18.8672385038326,
0.));
#221880=CARTESIAN_POINT('Ctrl Pts',(12.9171863977045,-18.8672385038326,
12.));
#221881=CARTESIAN_POINT('Ctrl Pts',(12.9224123144981,-18.8785402977528,
0.));
#221882=CARTESIAN_POINT('Ctrl Pts',(12.9224123144981,-18.8785402977528,
12.));
#221883=CARTESIAN_POINT('Ctrl Pts',(12.9276763536373,-18.8900227704889,
0.));
#221884=CARTESIAN_POINT('Ctrl Pts',(12.9276763536373,-18.8900227704889,
12.));
#221885=CARTESIAN_POINT('Ctrl Pts',(12.9329766328184,-18.9016841423403,
0.));
#221886=CARTESIAN_POINT('Ctrl Pts',(12.9329766328184,-18.9016841423403,
12.));
#221887=CARTESIAN_POINT('Ctrl Pts',(12.9383113190374,-18.9135226769466,
0.));
#221888=CARTESIAN_POINT('Ctrl Pts',(12.9383113190374,-18.9135226769466,
12.));
#221889=CARTESIAN_POINT('Ctrl Pts',(12.9436786266105,-18.9255366795195,
0.));
#221890=CARTESIAN_POINT('Ctrl Pts',(12.9436786266105,-18.9255366795195,
12.));
#221891=CARTESIAN_POINT('Ctrl Pts',(12.9490768151821,-18.9377244950435,
0.));
#221892=CARTESIAN_POINT('Ctrl Pts',(12.9490768151821,-18.9377244950435,
12.));
#221893=CARTESIAN_POINT('Ctrl Pts',(12.9545041877377,-18.9500845064715,
0.));
#221894=CARTESIAN_POINT('Ctrl Pts',(12.9545041877377,-18.9500845064715,
12.));
#221895=CARTESIAN_POINT('Ctrl Pts',(12.9599590886319,-18.9626151329229,
0.));
#221896=CARTESIAN_POINT('Ctrl Pts',(12.9599590886319,-18.9626151329229,
12.));
#221897=CARTESIAN_POINT('Ctrl Pts',(12.9654399021869,-18.9753148284475,
0.));
#221898=CARTESIAN_POINT('Ctrl Pts',(12.9654399021869,-18.9753148284475,
12.));
#221899=CARTESIAN_POINT('Ctrl Pts',(12.9709450512747,-18.9881820807586,
0.));
#221900=CARTESIAN_POINT('Ctrl Pts',(12.9709450512747,-18.9881820807586,
12.));
#221901=CARTESIAN_POINT('Ctrl Pts',(12.9764729959205,-19.0012154099791,
0.));
#221902=CARTESIAN_POINT('Ctrl Pts',(12.9764729959205,-19.0012154099791,
12.));
#221903=CARTESIAN_POINT('Ctrl Pts',(12.9820222318715,-19.0144133673348,
0.));
#221904=CARTESIAN_POINT('Ctrl Pts',(12.9820222318715,-19.0144133673348,
12.));
#221905=CARTESIAN_POINT('Ctrl Pts',(12.9875912893003,-19.0277745339908,
0.));
#221906=CARTESIAN_POINT('Ctrl Pts',(12.9875912893003,-19.0277745339908,
12.));
#221907=CARTESIAN_POINT('Ctrl Pts',(12.9931787316514,-19.0412975200398,
0.));
#221908=CARTESIAN_POINT('Ctrl Pts',(12.9931787316514,-19.0412975200398,
12.));
#221909=CARTESIAN_POINT('Ctrl Pts',(12.9987831544502,-19.0549809634355,
0.));
#221910=CARTESIAN_POINT('Ctrl Pts',(12.9987831544502,-19.0549809634355,
12.));
#221911=CARTESIAN_POINT('Ctrl Pts',(13.0044031841381,-19.0688235289437,
0.));
#221912=CARTESIAN_POINT('Ctrl Pts',(13.0044031841381,-19.0688235289437,
12.));
#221913=CARTESIAN_POINT('Ctrl Pts',(13.0100374768785,-19.0828239070482,
0.));
#221914=CARTESIAN_POINT('Ctrl Pts',(13.0100374768785,-19.0828239070482,
12.));
#221915=CARTESIAN_POINT('Ctrl Pts',(13.0156847176093,-19.0969808131226,
0.));
#221916=CARTESIAN_POINT('Ctrl Pts',(13.0156847176093,-19.0969808131226,
12.));
#221917=CARTESIAN_POINT('Ctrl Pts',(13.0213436191326,-19.1112929866308,
0.));
#221918=CARTESIAN_POINT('Ctrl Pts',(13.0213436191326,-19.1112929866308,
12.));
#221919=CARTESIAN_POINT('Ctrl Pts',(13.0270129211976,-19.1257591903099,
0.));
#221920=CARTESIAN_POINT('Ctrl Pts',(13.0270129211976,-19.1257591903099,
12.));
#221921=CARTESIAN_POINT('Ctrl Pts',(13.0326913895841,-19.1403782093389,
0.));
#221922=CARTESIAN_POINT('Ctrl Pts',(13.0326913895841,-19.1403782093389,
12.));
#221923=CARTESIAN_POINT('Ctrl Pts',(13.0383778152072,-19.1551488505233,
0.));
#221924=CARTESIAN_POINT('Ctrl Pts',(13.0383778152072,-19.1551488505233,
12.));
#221925=CARTESIAN_POINT('Ctrl Pts',(13.0440710133775,-19.1700699416625,
0.));
#221926=CARTESIAN_POINT('Ctrl Pts',(13.0440710133775,-19.1700699416625,
12.));
#221927=CARTESIAN_POINT('Ctrl Pts',(13.0497698230442,-19.1851403308826,
0.));
#221928=CARTESIAN_POINT('Ctrl Pts',(13.0497698230442,-19.1851403308826,
12.));
#221929=CARTESIAN_POINT('Ctrl Pts',(13.0554731060537,-19.2003588859771,
0.));
#221930=CARTESIAN_POINT('Ctrl Pts',(13.0554731060537,-19.2003588859771,
12.));
#221931=CARTESIAN_POINT('Ctrl Pts',(13.0611797463912,-19.2157244937141,
0.));
#221932=CARTESIAN_POINT('Ctrl Pts',(13.0611797463912,-19.2157244937141,
12.));
#221933=CARTESIAN_POINT('Ctrl Pts',(13.0668886494791,-19.2312360592031,
0.));
#221934=CARTESIAN_POINT('Ctrl Pts',(13.0668886494791,-19.2312360592031,
12.));
#221935=CARTESIAN_POINT('Ctrl Pts',(13.0725987415856,-19.2468925053988,
0.));
#221936=CARTESIAN_POINT('Ctrl Pts',(13.0725987415856,-19.2468925053988,
12.));
#221937=CARTESIAN_POINT('Ctrl Pts',(13.0783089692117,-19.2626927725596,
0.));
#221938=CARTESIAN_POINT('Ctrl Pts',(13.0783089692117,-19.2626927725596,
12.));
#221939=CARTESIAN_POINT('Ctrl Pts',(13.0840182984949,-19.2786358177198,
0.));
#221940=CARTESIAN_POINT('Ctrl Pts',(13.0840182984949,-19.2786358177198,
12.));
#221941=CARTESIAN_POINT('Ctrl Pts',(13.0897257145969,-19.2947206141246,
0.));
#221942=CARTESIAN_POINT('Ctrl Pts',(13.0897257145969,-19.2947206141246,
12.));
#221943=CARTESIAN_POINT('Ctrl Pts',(13.095430221148,-19.3109461507358,0.));
#221944=CARTESIAN_POINT('Ctrl Pts',(13.095430221148,-19.3109461507358,12.));
#221945=CARTESIAN_POINT('Ctrl Pts',(13.1011308397591,-19.3273114318268,
0.));
#221946=CARTESIAN_POINT('Ctrl Pts',(13.1011308397591,-19.3273114318268,
12.));
#221947=CARTESIAN_POINT('Ctrl Pts',(13.1068266095186,-19.3438154765395,
0.));
#221948=CARTESIAN_POINT('Ctrl Pts',(13.1068266095186,-19.3438154765395,
12.));
#221949=CARTESIAN_POINT('Ctrl Pts',(13.1125165865021,-19.3604573184516,
0.));
#221950=CARTESIAN_POINT('Ctrl Pts',(13.1125165865021,-19.3604573184516,
12.));
#221951=CARTESIAN_POINT('Ctrl Pts',(13.118199843271,-19.3772360051093,0.));
#221952=CARTESIAN_POINT('Ctrl Pts',(13.118199843271,-19.3772360051093,12.));
#221953=CARTESIAN_POINT('Ctrl Pts',(13.1238754684177,-19.3941505976267,
0.));
#221954=CARTESIAN_POINT('Ctrl Pts',(13.1238754684177,-19.3941505976267,
12.));
#221955=CARTESIAN_POINT('Ctrl Pts',(13.1295425661635,-19.4112001703561,
0.));
#221956=CARTESIAN_POINT('Ctrl Pts',(13.1295425661635,-19.4112001703561,
12.));
#221957=CARTESIAN_POINT('Ctrl Pts',(13.1352002559439,-19.4283838105265,
0.));
#221958=CARTESIAN_POINT('Ctrl Pts',(13.1352002559439,-19.4283838105265,
12.));
#221959=CARTESIAN_POINT('Ctrl Pts',(13.140847672006,-19.4457006178875,0.));
#221960=CARTESIAN_POINT('Ctrl Pts',(13.140847672006,-19.4457006178875,12.));
#221961=CARTESIAN_POINT('Ctrl Pts',(13.1464839629966,-19.463149704325,0.));
#221962=CARTESIAN_POINT('Ctrl Pts',(13.1464839629966,-19.463149704325,12.));
#221963=CARTESIAN_POINT('Ctrl Pts',(13.1521082915846,-19.4807301935256,
0.));
#221964=CARTESIAN_POINT('Ctrl Pts',(13.1521082915846,-19.4807301935256,
12.));
#221965=CARTESIAN_POINT('Ctrl Pts',(13.1577198341238,-19.498441220707,0.));
#221966=CARTESIAN_POINT('Ctrl Pts',(13.1577198341238,-19.498441220707,12.));
#221967=CARTESIAN_POINT('Ctrl Pts',(13.1633177803097,-19.5162819323207,
0.));
#221968=CARTESIAN_POINT('Ctrl Pts',(13.1633177803097,-19.5162819323207,
12.));
#221969=CARTESIAN_POINT('Ctrl Pts',(13.1689013328432,-19.5342514857564,
0.));
#221970=CARTESIAN_POINT('Ctrl Pts',(13.1689013328432,-19.5342514857564,
12.));
#221971=CARTESIAN_POINT('Ctrl Pts',(13.1744697070918,-19.5523490490254,
0.));
#221972=CARTESIAN_POINT('Ctrl Pts',(13.1744697070918,-19.5523490490254,
12.));
#221973=CARTESIAN_POINT('Ctrl Pts',(13.1800221307682,-19.5705738004682,
0.));
#221974=CARTESIAN_POINT('Ctrl Pts',(13.1800221307682,-19.5705738004682,
12.));
#221975=CARTESIAN_POINT('Ctrl Pts',(13.1855578436479,-19.5889249285352,
0.));
#221976=CARTESIAN_POINT('Ctrl Pts',(13.1855578436479,-19.5889249285352,
12.));
#221977=CARTESIAN_POINT('Ctrl Pts',(13.1910760972818,-19.6074016315421,
0.));
#221978=CARTESIAN_POINT('Ctrl Pts',(13.1910760972818,-19.6074016315421,
12.));
#221979=CARTESIAN_POINT('Ctrl Pts',(13.196576154715,-19.6260031174244,0.));
#221980=CARTESIAN_POINT('Ctrl Pts',(13.196576154715,-19.6260031174244,12.));
#221981=CARTESIAN_POINT('Ctrl Pts',(13.202057290206,-19.6447286034764,0.));
#221982=CARTESIAN_POINT('Ctrl Pts',(13.202057290206,-19.6447286034764,12.));
#221983=CARTESIAN_POINT('Ctrl Pts',(13.2075187889522,-19.6635773160924,
0.));
#221984=CARTESIAN_POINT('Ctrl Pts',(13.2075187889522,-19.6635773160924,
12.));
#221985=CARTESIAN_POINT('Ctrl Pts',(13.2129599468478,-19.6825484905812,
0.));
#221986=CARTESIAN_POINT('Ctrl Pts',(13.2129599468478,-19.6825484905812,
12.));
#221987=CARTESIAN_POINT('Ctrl Pts',(13.2183800702431,-19.7016413709678,
0.));
#221988=CARTESIAN_POINT('Ctrl Pts',(13.2183800702431,-19.7016413709678,
12.));
#221989=CARTESIAN_POINT('Ctrl Pts',(13.2237784757065,-19.7208552097867,
0.));
#221990=CARTESIAN_POINT('Ctrl Pts',(13.2237784757065,-19.7208552097867,
12.));
#221991=CARTESIAN_POINT('Ctrl Pts',(13.2291544897902,-19.7401892678701,
0.));
#221992=CARTESIAN_POINT('Ctrl Pts',(13.2291544897902,-19.7401892678701,
12.));
#221993=CARTESIAN_POINT('Ctrl Pts',(13.2345074487968,-19.7596428141176,
0.));
#221994=CARTESIAN_POINT('Ctrl Pts',(13.2345074487968,-19.7596428141176,
12.));
#221995=CARTESIAN_POINT('Ctrl Pts',(13.239836698568,-19.7792151253297,0.));
#221996=CARTESIAN_POINT('Ctrl Pts',(13.239836698568,-19.7792151253297,12.));
#221997=CARTESIAN_POINT('Ctrl Pts',(13.2451415942809,-19.7989054860501,
0.));
#221998=CARTESIAN_POINT('Ctrl Pts',(13.2451415942809,-19.7989054860501,
12.));
#221999=CARTESIAN_POINT('Ctrl Pts',(13.2504215002458,-19.8187131883919,
0.));
#222000=CARTESIAN_POINT('Ctrl Pts',(13.2504215002458,-19.8187131883919,
12.));
#222001=CARTESIAN_POINT('Ctrl Pts',(13.2556757897085,-19.8386375318632,
0.));
#222002=CARTESIAN_POINT('Ctrl Pts',(13.2556757897085,-19.8386375318632,
12.));
#222003=CARTESIAN_POINT('Ctrl Pts',(13.2609038446525,-19.8586778231711,
0.));
#222004=CARTESIAN_POINT('Ctrl Pts',(13.2609038446525,-19.8586778231711,
12.));
#222005=CARTESIAN_POINT('Ctrl Pts',(13.2661050556128,-19.8788333760571,
0.));
#222006=CARTESIAN_POINT('Ctrl Pts',(13.2661050556128,-19.8788333760571,
12.));
#222007=CARTESIAN_POINT('Ctrl Pts',(13.2712788215015,-19.8991035111739,
0.));
#222008=CARTESIAN_POINT('Ctrl Pts',(13.2712788215015,-19.8991035111739,
12.));
#222009=CARTESIAN_POINT('Ctrl Pts',(13.2764245494354,-19.9194875559419,
0.));
#222010=CARTESIAN_POINT('Ctrl Pts',(13.2764245494354,-19.9194875559419,
12.));
#222011=CARTESIAN_POINT('Ctrl Pts',(13.2815416545662,-19.939984844402,0.));
#222012=CARTESIAN_POINT('Ctrl Pts',(13.2815416545662,-19.939984844402,12.));
#222013=CARTESIAN_POINT('Ctrl Pts',(13.2866295599152,-19.9605947170589,
0.));
#222014=CARTESIAN_POINT('Ctrl Pts',(13.2866295599152,-19.9605947170589,
12.));
#222015=CARTESIAN_POINT('Ctrl Pts',(13.2916876962098,-19.9813165207174,
0.));
#222016=CARTESIAN_POINT('Ctrl Pts',(13.2916876962098,-19.9813165207174,
12.));
#222017=CARTESIAN_POINT('Ctrl Pts',(13.296715501731,-20.0021496083742,0.));
#222018=CARTESIAN_POINT('Ctrl Pts',(13.296715501731,-20.0021496083742,12.));
#222019=CARTESIAN_POINT('Ctrl Pts',(13.3017124221639,-20.023093339104,0.));
#222020=CARTESIAN_POINT('Ctrl Pts',(13.3017124221639,-20.023093339104,12.));
#222021=CARTESIAN_POINT('Ctrl Pts',(13.3066779104515,-20.0441470779345,
0.));
#222022=CARTESIAN_POINT('Ctrl Pts',(13.3066779104515,-20.0441470779345,
12.));
#222023=CARTESIAN_POINT('Ctrl Pts',(13.3116114266514,-20.0653101957188,
0.));
#222024=CARTESIAN_POINT('Ctrl Pts',(13.3116114266514,-20.0653101957188,
12.));
#222025=CARTESIAN_POINT('Ctrl Pts',(13.3165124377962,-20.0865820689884,
0.));
#222026=CARTESIAN_POINT('Ctrl Pts',(13.3165124377962,-20.0865820689884,
12.));
#222027=CARTESIAN_POINT('Ctrl Pts',(13.3213804177588,-20.1079620798377,
0.));
#222028=CARTESIAN_POINT('Ctrl Pts',(13.3213804177588,-20.1079620798377,
12.));
#222029=CARTESIAN_POINT('Ctrl Pts',(13.3262148471228,-20.1294496158405,
0.));
#222030=CARTESIAN_POINT('Ctrl Pts',(13.3262148471228,-20.1294496158405,
12.));
#222031=CARTESIAN_POINT('Ctrl Pts',(13.3310152130565,-20.1510440699477,
0.));
#222032=CARTESIAN_POINT('Ctrl Pts',(13.3310152130565,-20.1510440699477,
12.));
#222033=CARTESIAN_POINT('Ctrl Pts',(13.3357810091903,-20.1727448403818,
0.));
#222034=CARTESIAN_POINT('Ctrl Pts',(13.3357810091903,-20.1727448403818,
12.));
#222035=CARTESIAN_POINT('Ctrl Pts',(13.3405117354969,-20.1945513305233,
0.));
#222036=CARTESIAN_POINT('Ctrl Pts',(13.3405117354969,-20.1945513305233,
12.));
#222037=CARTESIAN_POINT('Ctrl Pts',(13.3452068981762,-20.2164629487855,
0.));
#222038=CARTESIAN_POINT('Ctrl Pts',(13.3452068981762,-20.2164629487855,
12.));
#222039=CARTESIAN_POINT('Ctrl Pts',(13.3498660095381,-20.2384791085354,
0.));
#222040=CARTESIAN_POINT('Ctrl Pts',(13.3498660095381,-20.2384791085354,
12.));
#222041=CARTESIAN_POINT('Ctrl Pts',(13.3544885878886,-20.2605992280117,
0.));
#222042=CARTESIAN_POINT('Ctrl Pts',(13.3544885878886,-20.2605992280117,
12.));
#222043=CARTESIAN_POINT('Ctrl Pts',(13.3590741574194,-20.2828227302337,
0.));
#222044=CARTESIAN_POINT('Ctrl Pts',(13.3590741574194,-20.2828227302337,
12.));
#222045=CARTESIAN_POINT('Ctrl Pts',(13.3636222481016,-20.3051490429049,
0.));
#222046=CARTESIAN_POINT('Ctrl Pts',(13.3636222481016,-20.3051490429049,
12.));
#222047=CARTESIAN_POINT('Ctrl Pts',(13.3681323955828,-20.3275775983032,
0.));
#222048=CARTESIAN_POINT('Ctrl Pts',(13.3681323955828,-20.3275775983032,
12.));
#222049=CARTESIAN_POINT('Ctrl Pts',(13.3726041410869,-20.3501078331818,
0.));
#222050=CARTESIAN_POINT('Ctrl Pts',(13.3726041410869,-20.3501078331818,
12.));
#222051=CARTESIAN_POINT('Ctrl Pts',(13.377037031319,-20.3727391887187,0.));
#222052=CARTESIAN_POINT('Ctrl Pts',(13.377037031319,-20.3727391887187,12.));
#222053=CARTESIAN_POINT('Ctrl Pts',(13.3814306183721,-20.3954711104505,
0.));
#222054=CARTESIAN_POINT('Ctrl Pts',(13.3814306183721,-20.3954711104505,
12.));
#222055=CARTESIAN_POINT('Ctrl Pts',(13.3857844596387,-20.4183030482002,
0.));
#222056=CARTESIAN_POINT('Ctrl Pts',(13.3857844596387,-20.4183030482002,
12.));
#222057=CARTESIAN_POINT('Ctrl Pts',(13.3900981177254,-20.4412344560007,
0.));
#222058=CARTESIAN_POINT('Ctrl Pts',(13.3900981177254,-20.4412344560007,
12.));
#222059=CARTESIAN_POINT('Ctrl Pts',(13.3943711603739,-20.4642647920038,
0.));
#222060=CARTESIAN_POINT('Ctrl Pts',(13.3943711603739,-20.4642647920038,
12.));
#222061=CARTESIAN_POINT('Ctrl Pts',(13.3986031603716,-20.4873935184041,
0.));
#222062=CARTESIAN_POINT('Ctrl Pts',(13.3986031603716,-20.4873935184041,
12.));
#222063=CARTESIAN_POINT('Ctrl Pts',(13.4027936954529,-20.5106201013755,
0.));
#222064=CARTESIAN_POINT('Ctrl Pts',(13.4027936954529,-20.5106201013755,
12.));
#222065=CARTESIAN_POINT('Ctrl Pts',(13.4069423482076,-20.5339440109958,
0.));
#222066=CARTESIAN_POINT('Ctrl Pts',(13.4069423482076,-20.5339440109958,
12.));
#222067=CARTESIAN_POINT('Ctrl Pts',(13.4110487059912,-20.557364721164,0.));
#222068=CARTESIAN_POINT('Ctrl Pts',(13.4110487059912,-20.557364721164,12.));
#222069=CARTESIAN_POINT('Ctrl Pts',(13.415112360841,-20.5808817095155,0.));
#222070=CARTESIAN_POINT('Ctrl Pts',(13.415112360841,-20.5808817095155,12.));
#222071=CARTESIAN_POINT('Ctrl Pts',(13.4191329093931,-20.6044944573151,
0.));
#222072=CARTESIAN_POINT('Ctrl Pts',(13.4191329093931,-20.6044944573151,
12.));
#222073=CARTESIAN_POINT('Ctrl Pts',(13.4231099528178,-20.6282024494234,
0.));
#222074=CARTESIAN_POINT('Ctrl Pts',(13.4231099528178,-20.6282024494234,
12.));
#222075=CARTESIAN_POINT('Ctrl Pts',(13.427043096765,-20.6520051742868,0.));
#222076=CARTESIAN_POINT('Ctrl Pts',(13.427043096765,-20.6520051742868,12.));
#222077=CARTESIAN_POINT('Ctrl Pts',(13.4309319513119,-20.6759021239102,
0.));
#222078=CARTESIAN_POINT('Ctrl Pts',(13.4309319513119,-20.6759021239102,
12.));
#222079=CARTESIAN_POINT('Ctrl Pts',(13.4347761309154,-20.6998927938288,
0.));
#222080=CARTESIAN_POINT('Ctrl Pts',(13.4347761309154,-20.6998927938288,
12.));
#222081=CARTESIAN_POINT('Ctrl Pts',(13.4385752543663,-20.7239766830676,
0.));
#222082=CARTESIAN_POINT('Ctrl Pts',(13.4385752543663,-20.7239766830676,
12.));
#222083=CARTESIAN_POINT('Ctrl Pts',(13.4423289447561,-20.7481532941014,
0.));
#222084=CARTESIAN_POINT('Ctrl Pts',(13.4423289447561,-20.7481532941014,
12.));
#222085=CARTESIAN_POINT('Ctrl Pts',(13.4460368293689,-20.7724221327609,
0.));
#222086=CARTESIAN_POINT('Ctrl Pts',(13.4460368293689,-20.7724221327609,
12.));
#222087=CARTESIAN_POINT('Ctrl Pts',(13.4496985395637,-20.7967827081228,
0.));
#222088=CARTESIAN_POINT('Ctrl Pts',(13.4496985395637,-20.7967827081228,
12.));
#222089=CARTESIAN_POINT('Ctrl Pts',(13.4533137106667,-20.821234532398,0.));
#222090=CARTESIAN_POINT('Ctrl Pts',(13.4533137106667,-20.821234532398,12.));
#222091=CARTESIAN_POINT('Ctrl Pts',(13.4568819818631,-20.8457771208083,
0.));
#222092=CARTESIAN_POINT('Ctrl Pts',(13.4568819818631,-20.8457771208083,
12.));
#222093=CARTESIAN_POINT('Ctrl Pts',(13.4604029960983,-20.8704099914641,
0.));
#222094=CARTESIAN_POINT('Ctrl Pts',(13.4604029960983,-20.8704099914641,
12.));
#222095=CARTESIAN_POINT('Ctrl Pts',(13.4638763999725,-20.8951326652158,
0.));
#222096=CARTESIAN_POINT('Ctrl Pts',(13.4638763999725,-20.8951326652158,
12.));
#222097=CARTESIAN_POINT('Ctrl Pts',(13.4673018437717,-20.9199446657583,
0.));
#222098=CARTESIAN_POINT('Ctrl Pts',(13.4673018437717,-20.9199446657583,
12.));
#222099=CARTESIAN_POINT('Ctrl Pts',(13.4706789815166,-20.9448455197557,
0.));
#222100=CARTESIAN_POINT('Ctrl Pts',(13.4706789815166,-20.9448455197557,
12.));
#222101=CARTESIAN_POINT('Ctrl Pts',(13.4740074710086,-20.9698347569477,
0.));
#222102=CARTESIAN_POINT('Ctrl Pts',(13.4740074710086,-20.9698347569477,
12.));
#222103=CARTESIAN_POINT('Ctrl Pts',(13.4772869738878,-20.9949119102592,
0.));
#222104=CARTESIAN_POINT('Ctrl Pts',(13.4772869738878,-20.9949119102592,
12.));
#222105=CARTESIAN_POINT('Ctrl Pts',(13.4805171556822,-21.0200765158884,
0.));
#222106=CARTESIAN_POINT('Ctrl Pts',(13.4805171556822,-21.0200765158884,
12.));
#222107=CARTESIAN_POINT('Ctrl Pts',(13.4836976858912,-21.0453281134245,
0.));
#222108=CARTESIAN_POINT('Ctrl Pts',(13.4836976858912,-21.0453281134245,
12.));
#222109=CARTESIAN_POINT('Ctrl Pts',(13.4868282377191,-21.0706662455199,
0.));
#222110=CARTESIAN_POINT('Ctrl Pts',(13.4868282377191,-21.0706662455199,
12.));
#222111=CARTESIAN_POINT('Ctrl Pts',(13.4899084877717,-21.0960904575046,
0.));
#222112=CARTESIAN_POINT('Ctrl Pts',(13.4899084877717,-21.0960904575046,
12.));
#222113=CARTESIAN_POINT('Ctrl Pts',(13.4929381157778,-21.1216002970207,
0.));
#222114=CARTESIAN_POINT('Ctrl Pts',(13.4929381157778,-21.1216002970207,
12.));
#222115=CARTESIAN_POINT('Ctrl Pts',(13.4959168042934,-21.1471953136209,
0.));
#222116=CARTESIAN_POINT('Ctrl Pts',(13.4959168042934,-21.1471953136209,
12.));
#222117=CARTESIAN_POINT('Ctrl Pts',(13.4988442384491,-21.1728750584175,
0.));
#222118=CARTESIAN_POINT('Ctrl Pts',(13.4988442384491,-21.1728750584175,
12.));
#222119=CARTESIAN_POINT('Ctrl Pts',(13.5017201056088,-21.1986390835828,
0.));
#222120=CARTESIAN_POINT('Ctrl Pts',(13.5017201056088,-21.1986390835828,
12.));
#222121=CARTESIAN_POINT('Ctrl Pts',(13.5045440957404,-21.2244869429332,
0.));
#222122=CARTESIAN_POINT('Ctrl Pts',(13.5045440957404,-21.2244869429332,
12.));
#222123=CARTESIAN_POINT('Ctrl Pts',(13.5073159019452,-21.250418192743,0.));
#222124=CARTESIAN_POINT('Ctrl Pts',(13.5073159019452,-21.250418192743,12.));
#222125=CARTESIAN_POINT('Ctrl Pts',(13.5100352209205,-21.2764323924442,
0.));
#222126=CARTESIAN_POINT('Ctrl Pts',(13.5100352209205,-21.2764323924442,
12.));
#222127=CARTESIAN_POINT('Ctrl Pts',(13.5127017534971,-21.3025291054235,
0.));
#222128=CARTESIAN_POINT('Ctrl Pts',(13.5127017534971,-21.3025291054235,
12.));
#222129=CARTESIAN_POINT('Ctrl Pts',(13.5153152050555,-21.3287078996341,
0.));
#222130=CARTESIAN_POINT('Ctrl Pts',(13.5153152050555,-21.3287078996341,
12.));
#222131=CARTESIAN_POINT('Ctrl Pts',(13.5178752862466,-21.3549683486222,
0.));
#222132=CARTESIAN_POINT('Ctrl Pts',(13.5178752862466,-21.3549683486222,
12.));
#222133=CARTESIAN_POINT('Ctrl Pts',(13.5203817122503,-21.3813100304973,
0.));
#222134=CARTESIAN_POINT('Ctrl Pts',(13.5203817122503,-21.3813100304973,
12.));
#222135=CARTESIAN_POINT('Ctrl Pts',(13.5228342013516,-21.4077325259324,
0.));
#222136=CARTESIAN_POINT('Ctrl Pts',(13.5228342013516,-21.4077325259324,
12.));
#222137=CARTESIAN_POINT('Ctrl Pts',(13.5252324737801,-21.4342354165259,
0.));
#222138=CARTESIAN_POINT('Ctrl Pts',(13.5252324737801,-21.4342354165259,
12.));
#222139=CARTESIAN_POINT('Ctrl Pts',(13.5275762503555,-21.4608182828697,
0.));
#222140=CARTESIAN_POINT('Ctrl Pts',(13.5275762503555,-21.4608182828697,
12.));
#222141=CARTESIAN_POINT('Ctrl Pts',(13.5298652514355,-21.4874807030468,
0.));
#222142=CARTESIAN_POINT('Ctrl Pts',(13.5298652514355,-21.4874807030468,
12.));
#222143=CARTESIAN_POINT('Ctrl Pts',(13.5320991952138,-21.5142222501666,
0.));
#222144=CARTESIAN_POINT('Ctrl Pts',(13.5320991952138,-21.5142222501666,
12.));
#222145=CARTESIAN_POINT('Ctrl Pts',(13.5342777983214,-21.5410424932503,
0.));
#222146=CARTESIAN_POINT('Ctrl Pts',(13.5342777983214,-21.5410424932503,
12.));
#222147=CARTESIAN_POINT('Ctrl Pts',(13.536400779028,-21.5679410019002,0.));
#222148=CARTESIAN_POINT('Ctrl Pts',(13.536400779028,-21.5679410019002,12.));
#222149=CARTESIAN_POINT('Ctrl Pts',(13.5384678597195,-21.5949173499013,
0.));
#222150=CARTESIAN_POINT('Ctrl Pts',(13.5384678597195,-21.5949173499013,
12.));
#222151=CARTESIAN_POINT('Ctrl Pts',(13.5404787697791,-21.6219711193946,
0.));
#222152=CARTESIAN_POINT('Ctrl Pts',(13.5404787697791,-21.6219711193946,
12.));
#222153=CARTESIAN_POINT('Ctrl Pts',(13.5424332480699,-21.6491019044648,
0.));
#222154=CARTESIAN_POINT('Ctrl Pts',(13.5424332480699,-21.6491019044648,
12.));
#222155=CARTESIAN_POINT('Ctrl Pts',(13.5443310461526,-21.6763093157699,
0.));
#222156=CARTESIAN_POINT('Ctrl Pts',(13.5443310461526,-21.6763093157699,
12.));
#222157=CARTESIAN_POINT('Ctrl Pts',(13.5461719295048,-21.7035929822955,
0.));
#222158=CARTESIAN_POINT('Ctrl Pts',(13.5461719295048,-21.7035929822955,
12.));
#222159=CARTESIAN_POINT('Ctrl Pts',(13.5479556704481,-21.7309525412281,
0.));
#222160=CARTESIAN_POINT('Ctrl Pts',(13.5479556704481,-21.7309525412281,
12.));
#222161=CARTESIAN_POINT('Ctrl Pts',(13.5496820422211,-21.7583876294554,
0.));
#222162=CARTESIAN_POINT('Ctrl Pts',(13.5496820422211,-21.7583876294554,
12.));
#222163=CARTESIAN_POINT('Ctrl Pts',(13.551350812725,-21.7858978745865,0.));
#222164=CARTESIAN_POINT('Ctrl Pts',(13.551350812725,-21.7858978745865,12.));
#222165=CARTESIAN_POINT('Ctrl Pts',(13.5529617381573,-21.8134828857967,
0.));
#222166=CARTESIAN_POINT('Ctrl Pts',(13.5529617381573,-21.8134828857967,
12.));
#222167=CARTESIAN_POINT('Ctrl Pts',(13.5545145573031,-21.8411422456075,
0.));
#222168=CARTESIAN_POINT('Ctrl Pts',(13.5545145573031,-21.8411422456075,
12.));
#222169=CARTESIAN_POINT('Ctrl Pts',(13.5560089839385,-21.8688754989365,
0.));
#222170=CARTESIAN_POINT('Ctrl Pts',(13.5560089839385,-21.8688754989365,
12.));
#222171=CARTESIAN_POINT('Ctrl Pts',(13.5574447178424,-21.8966821688824,
0.));
#222172=CARTESIAN_POINT('Ctrl Pts',(13.5574447178424,-21.8966821688824,
12.));
#222173=CARTESIAN_POINT('Ctrl Pts',(13.5588214586604,-21.9245617765769,
0.));
#222174=CARTESIAN_POINT('Ctrl Pts',(13.5588214586604,-21.9245617765769,
12.));
#222175=CARTESIAN_POINT('Ctrl Pts',(13.5601389185257,-21.9525138592813,
0.));
#222176=CARTESIAN_POINT('Ctrl Pts',(13.5601389185257,-21.9525138592813,
12.));
#222177=CARTESIAN_POINT('Ctrl Pts',(13.5613968357561,-21.9805379899168,
0.));
#222178=CARTESIAN_POINT('Ctrl Pts',(13.5613968357561,-21.9805379899168,
12.));
#222179=CARTESIAN_POINT('Ctrl Pts',(13.5625949868333,-22.0086337943449,
0.));
#222180=CARTESIAN_POINT('Ctrl Pts',(13.5625949868333,-22.0086337943449,
12.));
#222181=CARTESIAN_POINT('Ctrl Pts',(13.5637332022473,-22.0368009736295,
0.));
#222182=CARTESIAN_POINT('Ctrl Pts',(13.5637332022473,-22.0368009736295,
12.));
#222183=CARTESIAN_POINT('Ctrl Pts',(13.5648113689033,-22.065039308961,0.));
#222184=CARTESIAN_POINT('Ctrl Pts',(13.5648113689033,-22.065039308961,12.));
#222185=CARTESIAN_POINT('Ctrl Pts',(13.5658294169284,-22.0933486464593,
0.));
#222186=CARTESIAN_POINT('Ctrl Pts',(13.5658294169284,-22.0933486464593,
12.));
#222187=CARTESIAN_POINT('Ctrl Pts',(13.5667873105359,-22.1217288871975,
0.));
#222188=CARTESIAN_POINT('Ctrl Pts',(13.5667873105359,-22.1217288871975,
12.));
#222189=CARTESIAN_POINT('Ctrl Pts',(13.5675054919061,-22.1444897575194,
0.));
#222190=CARTESIAN_POINT('Ctrl Pts',(13.5675054919061,-22.1444897575194,
12.));
#222191=CARTESIAN_POINT('Ctrl Pts',(13.5680170531805,-22.1615922805008,
0.));
#222192=CARTESIAN_POINT('Ctrl Pts',(13.5680170531805,-22.1615922805008,
12.));
#222193=CARTESIAN_POINT('Ctrl Pts',(13.5683460612942,-22.1730081264608,
0.));
#222194=CARTESIAN_POINT('Ctrl Pts',(13.5683460612942,-22.1730081264608,
12.));
#222195=CARTESIAN_POINT('Ctrl Pts',(13.5685075571671,-22.178719590434,0.));
#222196=CARTESIAN_POINT('Ctrl Pts',(13.5685075571671,-22.178719590434,12.));
#222197=CARTESIAN_POINT('',(13.5685075571671,-22.178719590434,0.));
#222198=CARTESIAN_POINT('Ctrl Pts',(12.7689476255362,-18.5896416359912,
0.));
#222199=CARTESIAN_POINT('Ctrl Pts',(12.7689524524483,-18.5896460962964,
0.));
#222200=CARTESIAN_POINT('Ctrl Pts',(12.768986426692,-18.5896919669165,0.));
#222201=CARTESIAN_POINT('Ctrl Pts',(12.769110348199,-18.589871621843,0.));
#222202=CARTESIAN_POINT('Ctrl Pts',(12.7694215127918,-18.5903328777227,
0.));
#222203=CARTESIAN_POINT('Ctrl Pts',(12.7700520897173,-18.5912775137806,
0.));
#222204=CARTESIAN_POINT('Ctrl Pts',(12.7709195951156,-18.5925859134579,
0.));
#222205=CARTESIAN_POINT('Ctrl Pts',(12.7720142287172,-18.5942490615407,
0.));
#222206=CARTESIAN_POINT('Ctrl Pts',(12.7733231262108,-18.5962551167772,
0.));
#222207=CARTESIAN_POINT('Ctrl Pts',(12.7748328937638,-18.598591752595,0.));
#222208=CARTESIAN_POINT('Ctrl Pts',(12.7765325225081,-18.6012488486709,
0.));
#222209=CARTESIAN_POINT('Ctrl Pts',(12.7784139605066,-18.6042190183704,
0.));
#222210=CARTESIAN_POINT('Ctrl Pts',(12.7804705387658,-18.6074961535723,
0.));
#222211=CARTESIAN_POINT('Ctrl Pts',(12.7826959526924,-18.611074482622,0.));
#222212=CARTESIAN_POINT('Ctrl Pts',(12.7850831657901,-18.6149475565188,
0.));
#222213=CARTESIAN_POINT('Ctrl Pts',(12.7876249657834,-18.6191087624752,
0.));
#222214=CARTESIAN_POINT('Ctrl Pts',(12.7903142925234,-18.6235516265575,
0.));
#222215=CARTESIAN_POINT('Ctrl Pts',(12.7931447451555,-18.6282702819371,
0.));
#222216=CARTESIAN_POINT('Ctrl Pts',(12.796110622225,-18.6332595057006,0.));
#222217=CARTESIAN_POINT('Ctrl Pts',(12.7992066625264,-18.63851447924,0.));
#222218=CARTESIAN_POINT('Ctrl Pts',(12.8024278770152,-18.6440306327456,
0.));
#222219=CARTESIAN_POINT('Ctrl Pts',(12.805769331162,-18.6498034438987,0.));
#222220=CARTESIAN_POINT('Ctrl Pts',(12.8092261933858,-18.6558284825773,
0.));
#222221=CARTESIAN_POINT('Ctrl Pts',(12.8127937909631,-18.6621014624746,
0.));
#222222=CARTESIAN_POINT('Ctrl Pts',(12.8164676687362,-18.66861829528,0.));
#222223=CARTESIAN_POINT('Ctrl Pts',(12.8202436318474,-18.6753751301092,
0.));
#222224=CARTESIAN_POINT('Ctrl Pts',(12.8241176980017,-18.6823683094139,
0.));
#222225=CARTESIAN_POINT('Ctrl Pts',(12.8280860635231,-18.6895943376172,
0.));
#222226=CARTESIAN_POINT('Ctrl Pts',(12.8321450599789,-18.6970498410172,
0.));
#222227=CARTESIAN_POINT('Ctrl Pts',(12.8362911280361,-18.7047315436294,
0.));
#222228=CARTESIAN_POINT('Ctrl Pts',(12.8405208263431,-18.7126362754445,
0.));
#222229=CARTESIAN_POINT('Ctrl Pts',(12.8448308329494,-18.7207609737702,
0.));
#222230=CARTESIAN_POINT('Ctrl Pts',(12.8492179511591,-18.7291026886554,
0.));
#222231=CARTESIAN_POINT('Ctrl Pts',(12.8536791086316,-18.7376585820854,
0.));
#222232=CARTESIAN_POINT('Ctrl Pts',(12.8582113455646,-18.7464259171251,
0.));
#222233=CARTESIAN_POINT('Ctrl Pts',(12.8628118054171,-18.7554020493887,
0.));
#222234=CARTESIAN_POINT('Ctrl Pts',(12.8674777239653,-18.7645844169564,
0.));
#222235=CARTESIAN_POINT('Ctrl Pts',(12.872206421181,-18.7739705329022,0.));
#222236=CARTESIAN_POINT('Ctrl Pts',(12.8769952998095,-18.7835579840477,
0.));
#222237=CARTESIAN_POINT('Ctrl Pts',(12.8818418427475,-18.7933444285868,
0.));
#222238=CARTESIAN_POINT('Ctrl Pts',(12.8867436109546,-18.8033275941943,
0.));
#222239=CARTESIAN_POINT('Ctrl Pts',(12.8916982409935,-18.813505275782,0.));
#222240=CARTESIAN_POINT('Ctrl Pts',(12.8967034410754,-18.8238753319129,
0.));
#222241=CARTESIAN_POINT('Ctrl Pts',(12.9017569871738,-18.8344356812591,
0.));
#222242=CARTESIAN_POINT('Ctrl Pts',(12.9068567191854,-18.8451842990984,
0.));
#222243=CARTESIAN_POINT('Ctrl Pts',(12.9120005369063,-18.8561192136198,
0.));
#222244=CARTESIAN_POINT('Ctrl Pts',(12.9171863977045,-18.8672385038326,
0.));
#222245=CARTESIAN_POINT('Ctrl Pts',(12.9224123144981,-18.8785402977528,
0.));
#222246=CARTESIAN_POINT('Ctrl Pts',(12.9276763536373,-18.8900227704889,
0.));
#222247=CARTESIAN_POINT('Ctrl Pts',(12.9329766328184,-18.9016841423403,
0.));
#222248=CARTESIAN_POINT('Ctrl Pts',(12.9383113190374,-18.9135226769466,
0.));
#222249=CARTESIAN_POINT('Ctrl Pts',(12.9436786266105,-18.9255366795195,
0.));
#222250=CARTESIAN_POINT('Ctrl Pts',(12.9490768151821,-18.9377244950435,
0.));
#222251=CARTESIAN_POINT('Ctrl Pts',(12.9545041877377,-18.9500845064715,
0.));
#222252=CARTESIAN_POINT('Ctrl Pts',(12.9599590886319,-18.9626151329229,
0.));
#222253=CARTESIAN_POINT('Ctrl Pts',(12.9654399021869,-18.9753148284475,
0.));
#222254=CARTESIAN_POINT('Ctrl Pts',(12.9709450512747,-18.9881820807586,
0.));
#222255=CARTESIAN_POINT('Ctrl Pts',(12.9764729959205,-19.0012154099791,
0.));
#222256=CARTESIAN_POINT('Ctrl Pts',(12.9820222318715,-19.0144133673348,
0.));
#222257=CARTESIAN_POINT('Ctrl Pts',(12.9875912893003,-19.0277745339908,
0.));
#222258=CARTESIAN_POINT('Ctrl Pts',(12.9931787316514,-19.0412975200398,
0.));
#222259=CARTESIAN_POINT('Ctrl Pts',(12.9987831544502,-19.0549809634355,
0.));
#222260=CARTESIAN_POINT('Ctrl Pts',(13.0044031841381,-19.0688235289437,
0.));
#222261=CARTESIAN_POINT('Ctrl Pts',(13.0100374768785,-19.0828239070482,
0.));
#222262=CARTESIAN_POINT('Ctrl Pts',(13.0156847176093,-19.0969808131226,
0.));
#222263=CARTESIAN_POINT('Ctrl Pts',(13.0213436191326,-19.1112929866308,
0.));
#222264=CARTESIAN_POINT('Ctrl Pts',(13.0270129211976,-19.1257591903099,
0.));
#222265=CARTESIAN_POINT('Ctrl Pts',(13.0326913895841,-19.1403782093389,
0.));
#222266=CARTESIAN_POINT('Ctrl Pts',(13.0383778152072,-19.1551488505233,
0.));
#222267=CARTESIAN_POINT('Ctrl Pts',(13.0440710133775,-19.1700699416625,
0.));
#222268=CARTESIAN_POINT('Ctrl Pts',(13.0497698230442,-19.1851403308826,
0.));
#222269=CARTESIAN_POINT('Ctrl Pts',(13.0554731060537,-19.2003588859771,
0.));
#222270=CARTESIAN_POINT('Ctrl Pts',(13.0611797463912,-19.2157244937141,
0.));
#222271=CARTESIAN_POINT('Ctrl Pts',(13.0668886494791,-19.2312360592031,
0.));
#222272=CARTESIAN_POINT('Ctrl Pts',(13.0725987415856,-19.2468925053988,
0.));
#222273=CARTESIAN_POINT('Ctrl Pts',(13.0783089692117,-19.2626927725596,
0.));
#222274=CARTESIAN_POINT('Ctrl Pts',(13.0840182984949,-19.2786358177198,
0.));
#222275=CARTESIAN_POINT('Ctrl Pts',(13.0897257145969,-19.2947206141246,
0.));
#222276=CARTESIAN_POINT('Ctrl Pts',(13.095430221148,-19.3109461507358,0.));
#222277=CARTESIAN_POINT('Ctrl Pts',(13.1011308397591,-19.3273114318268,
0.));
#222278=CARTESIAN_POINT('Ctrl Pts',(13.1068266095186,-19.3438154765395,
0.));
#222279=CARTESIAN_POINT('Ctrl Pts',(13.1125165865021,-19.3604573184516,
0.));
#222280=CARTESIAN_POINT('Ctrl Pts',(13.118199843271,-19.3772360051093,0.));
#222281=CARTESIAN_POINT('Ctrl Pts',(13.1238754684177,-19.3941505976267,
0.));
#222282=CARTESIAN_POINT('Ctrl Pts',(13.1295425661635,-19.4112001703561,
0.));
#222283=CARTESIAN_POINT('Ctrl Pts',(13.1352002559439,-19.4283838105265,
0.));
#222284=CARTESIAN_POINT('Ctrl Pts',(13.140847672006,-19.4457006178875,0.));
#222285=CARTESIAN_POINT('Ctrl Pts',(13.1464839629966,-19.463149704325,0.));
#222286=CARTESIAN_POINT('Ctrl Pts',(13.1521082915846,-19.4807301935256,
0.));
#222287=CARTESIAN_POINT('Ctrl Pts',(13.1577198341238,-19.498441220707,0.));
#222288=CARTESIAN_POINT('Ctrl Pts',(13.1633177803097,-19.5162819323207,
0.));
#222289=CARTESIAN_POINT('Ctrl Pts',(13.1689013328432,-19.5342514857564,
0.));
#222290=CARTESIAN_POINT('Ctrl Pts',(13.1744697070918,-19.5523490490254,
0.));
#222291=CARTESIAN_POINT('Ctrl Pts',(13.1800221307682,-19.5705738004682,
0.));
#222292=CARTESIAN_POINT('Ctrl Pts',(13.1855578436479,-19.5889249285352,
0.));
#222293=CARTESIAN_POINT('Ctrl Pts',(13.1910760972818,-19.6074016315421,
0.));
#222294=CARTESIAN_POINT('Ctrl Pts',(13.196576154715,-19.6260031174244,0.));
#222295=CARTESIAN_POINT('Ctrl Pts',(13.202057290206,-19.6447286034764,0.));
#222296=CARTESIAN_POINT('Ctrl Pts',(13.2075187889522,-19.6635773160924,
0.));
#222297=CARTESIAN_POINT('Ctrl Pts',(13.2129599468478,-19.6825484905812,
0.));
#222298=CARTESIAN_POINT('Ctrl Pts',(13.2183800702431,-19.7016413709678,
0.));
#222299=CARTESIAN_POINT('Ctrl Pts',(13.2237784757065,-19.7208552097867,
0.));
#222300=CARTESIAN_POINT('Ctrl Pts',(13.2291544897902,-19.7401892678701,
0.));
#222301=CARTESIAN_POINT('Ctrl Pts',(13.2345074487968,-19.7596428141176,
0.));
#222302=CARTESIAN_POINT('Ctrl Pts',(13.239836698568,-19.7792151253297,0.));
#222303=CARTESIAN_POINT('Ctrl Pts',(13.2451415942809,-19.7989054860501,
0.));
#222304=CARTESIAN_POINT('Ctrl Pts',(13.2504215002458,-19.8187131883919,
0.));
#222305=CARTESIAN_POINT('Ctrl Pts',(13.2556757897085,-19.8386375318632,
0.));
#222306=CARTESIAN_POINT('Ctrl Pts',(13.2609038446525,-19.8586778231711,
0.));
#222307=CARTESIAN_POINT('Ctrl Pts',(13.2661050556128,-19.8788333760571,
0.));
#222308=CARTESIAN_POINT('Ctrl Pts',(13.2712788215015,-19.8991035111739,
0.));
#222309=CARTESIAN_POINT('Ctrl Pts',(13.2764245494354,-19.9194875559419,
0.));
#222310=CARTESIAN_POINT('Ctrl Pts',(13.2815416545662,-19.939984844402,0.));
#222311=CARTESIAN_POINT('Ctrl Pts',(13.2866295599152,-19.9605947170589,
0.));
#222312=CARTESIAN_POINT('Ctrl Pts',(13.2916876962098,-19.9813165207174,
0.));
#222313=CARTESIAN_POINT('Ctrl Pts',(13.296715501731,-20.0021496083742,0.));
#222314=CARTESIAN_POINT('Ctrl Pts',(13.3017124221639,-20.023093339104,0.));
#222315=CARTESIAN_POINT('Ctrl Pts',(13.3066779104515,-20.0441470779345,
0.));
#222316=CARTESIAN_POINT('Ctrl Pts',(13.3116114266514,-20.0653101957188,
0.));
#222317=CARTESIAN_POINT('Ctrl Pts',(13.3165124377962,-20.0865820689884,
0.));
#222318=CARTESIAN_POINT('Ctrl Pts',(13.3213804177588,-20.1079620798377,
0.));
#222319=CARTESIAN_POINT('Ctrl Pts',(13.3262148471228,-20.1294496158405,
0.));
#222320=CARTESIAN_POINT('Ctrl Pts',(13.3310152130565,-20.1510440699477,
0.));
#222321=CARTESIAN_POINT('Ctrl Pts',(13.3357810091903,-20.1727448403818,
0.));
#222322=CARTESIAN_POINT('Ctrl Pts',(13.3405117354969,-20.1945513305233,
0.));
#222323=CARTESIAN_POINT('Ctrl Pts',(13.3452068981762,-20.2164629487855,
0.));
#222324=CARTESIAN_POINT('Ctrl Pts',(13.3498660095381,-20.2384791085354,
0.));
#222325=CARTESIAN_POINT('Ctrl Pts',(13.3544885878886,-20.2605992280117,
0.));
#222326=CARTESIAN_POINT('Ctrl Pts',(13.3590741574194,-20.2828227302337,
0.));
#222327=CARTESIAN_POINT('Ctrl Pts',(13.3636222481016,-20.3051490429049,
0.));
#222328=CARTESIAN_POINT('Ctrl Pts',(13.3681323955828,-20.3275775983032,
0.));
#222329=CARTESIAN_POINT('Ctrl Pts',(13.3726041410869,-20.3501078331818,
0.));
#222330=CARTESIAN_POINT('Ctrl Pts',(13.377037031319,-20.3727391887187,0.));
#222331=CARTESIAN_POINT('Ctrl Pts',(13.3814306183721,-20.3954711104505,
0.));
#222332=CARTESIAN_POINT('Ctrl Pts',(13.3857844596387,-20.4183030482002,
0.));
#222333=CARTESIAN_POINT('Ctrl Pts',(13.3900981177254,-20.4412344560007,
0.));
#222334=CARTESIAN_POINT('Ctrl Pts',(13.3943711603739,-20.4642647920038,
0.));
#222335=CARTESIAN_POINT('Ctrl Pts',(13.3986031603716,-20.4873935184041,
0.));
#222336=CARTESIAN_POINT('Ctrl Pts',(13.4027936954529,-20.5106201013755,
0.));
#222337=CARTESIAN_POINT('Ctrl Pts',(13.4069423482076,-20.5339440109958,
0.));
#222338=CARTESIAN_POINT('Ctrl Pts',(13.4110487059912,-20.557364721164,0.));
#222339=CARTESIAN_POINT('Ctrl Pts',(13.415112360841,-20.5808817095155,0.));
#222340=CARTESIAN_POINT('Ctrl Pts',(13.4191329093931,-20.6044944573151,
0.));
#222341=CARTESIAN_POINT('Ctrl Pts',(13.4231099528178,-20.6282024494234,
0.));
#222342=CARTESIAN_POINT('Ctrl Pts',(13.427043096765,-20.6520051742868,0.));
#222343=CARTESIAN_POINT('Ctrl Pts',(13.4309319513119,-20.6759021239102,
0.));
#222344=CARTESIAN_POINT('Ctrl Pts',(13.4347761309154,-20.6998927938288,
0.));
#222345=CARTESIAN_POINT('Ctrl Pts',(13.4385752543663,-20.7239766830676,
0.));
#222346=CARTESIAN_POINT('Ctrl Pts',(13.4423289447561,-20.7481532941014,
0.));
#222347=CARTESIAN_POINT('Ctrl Pts',(13.4460368293689,-20.7724221327609,
0.));
#222348=CARTESIAN_POINT('Ctrl Pts',(13.4496985395637,-20.7967827081228,
0.));
#222349=CARTESIAN_POINT('Ctrl Pts',(13.4533137106667,-20.821234532398,0.));
#222350=CARTESIAN_POINT('Ctrl Pts',(13.4568819818631,-20.8457771208083,
0.));
#222351=CARTESIAN_POINT('Ctrl Pts',(13.4604029960983,-20.8704099914641,
0.));
#222352=CARTESIAN_POINT('Ctrl Pts',(13.4638763999725,-20.8951326652158,
0.));
#222353=CARTESIAN_POINT('Ctrl Pts',(13.4673018437717,-20.9199446657583,
0.));
#222354=CARTESIAN_POINT('Ctrl Pts',(13.4706789815166,-20.9448455197557,
0.));
#222355=CARTESIAN_POINT('Ctrl Pts',(13.4740074710086,-20.9698347569477,
0.));
#222356=CARTESIAN_POINT('Ctrl Pts',(13.4772869738878,-20.9949119102592,
0.));
#222357=CARTESIAN_POINT('Ctrl Pts',(13.4805171556822,-21.0200765158884,
0.));
#222358=CARTESIAN_POINT('Ctrl Pts',(13.4836976858912,-21.0453281134245,
0.));
#222359=CARTESIAN_POINT('Ctrl Pts',(13.4868282377191,-21.0706662455199,
0.));
#222360=CARTESIAN_POINT('Ctrl Pts',(13.4899084877717,-21.0960904575046,
0.));
#222361=CARTESIAN_POINT('Ctrl Pts',(13.4929381157778,-21.1216002970207,
0.));
#222362=CARTESIAN_POINT('Ctrl Pts',(13.4959168042934,-21.1471953136209,
0.));
#222363=CARTESIAN_POINT('Ctrl Pts',(13.4988442384491,-21.1728750584175,
0.));
#222364=CARTESIAN_POINT('Ctrl Pts',(13.5017201056088,-21.1986390835828,
0.));
#222365=CARTESIAN_POINT('Ctrl Pts',(13.5045440957404,-21.2244869429332,
0.));
#222366=CARTESIAN_POINT('Ctrl Pts',(13.5073159019452,-21.250418192743,0.));
#222367=CARTESIAN_POINT('Ctrl Pts',(13.5100352209205,-21.2764323924442,
0.));
#222368=CARTESIAN_POINT('Ctrl Pts',(13.5127017534971,-21.3025291054235,
0.));
#222369=CARTESIAN_POINT('Ctrl Pts',(13.5153152050555,-21.3287078996341,
0.));
#222370=CARTESIAN_POINT('Ctrl Pts',(13.5178752862466,-21.3549683486222,
0.));
#222371=CARTESIAN_POINT('Ctrl Pts',(13.5203817122503,-21.3813100304973,
0.));
#222372=CARTESIAN_POINT('Ctrl Pts',(13.5228342013516,-21.4077325259324,
0.));
#222373=CARTESIAN_POINT('Ctrl Pts',(13.5252324737801,-21.4342354165259,
0.));
#222374=CARTESIAN_POINT('Ctrl Pts',(13.5275762503555,-21.4608182828697,
0.));
#222375=CARTESIAN_POINT('Ctrl Pts',(13.5298652514355,-21.4874807030468,
0.));
#222376=CARTESIAN_POINT('Ctrl Pts',(13.5320991952138,-21.5142222501666,
0.));
#222377=CARTESIAN_POINT('Ctrl Pts',(13.5342777983214,-21.5410424932503,
0.));
#222378=CARTESIAN_POINT('Ctrl Pts',(13.536400779028,-21.5679410019002,0.));
#222379=CARTESIAN_POINT('Ctrl Pts',(13.5384678597195,-21.5949173499013,
0.));
#222380=CARTESIAN_POINT('Ctrl Pts',(13.5404787697791,-21.6219711193946,
0.));
#222381=CARTESIAN_POINT('Ctrl Pts',(13.5424332480699,-21.6491019044648,
0.));
#222382=CARTESIAN_POINT('Ctrl Pts',(13.5443310461526,-21.6763093157699,
0.));
#222383=CARTESIAN_POINT('Ctrl Pts',(13.5461719295048,-21.7035929822955,
0.));
#222384=CARTESIAN_POINT('Ctrl Pts',(13.5479556704481,-21.7309525412281,
0.));
#222385=CARTESIAN_POINT('Ctrl Pts',(13.5496820422211,-21.7583876294554,
0.));
#222386=CARTESIAN_POINT('Ctrl Pts',(13.551350812725,-21.7858978745865,0.));
#222387=CARTESIAN_POINT('Ctrl Pts',(13.5529617381573,-21.8134828857967,
0.));
#222388=CARTESIAN_POINT('Ctrl Pts',(13.5545145573031,-21.8411422456075,
0.));
#222389=CARTESIAN_POINT('Ctrl Pts',(13.5560089839385,-21.8688754989365,
0.));
#222390=CARTESIAN_POINT('Ctrl Pts',(13.5574447178424,-21.8966821688824,
0.));
#222391=CARTESIAN_POINT('Ctrl Pts',(13.5588214586604,-21.9245617765769,
0.));
#222392=CARTESIAN_POINT('Ctrl Pts',(13.5601389185257,-21.9525138592813,
0.));
#222393=CARTESIAN_POINT('Ctrl Pts',(13.5613968357561,-21.9805379899168,
0.));
#222394=CARTESIAN_POINT('Ctrl Pts',(13.5625949868333,-22.0086337943449,
0.));
#222395=CARTESIAN_POINT('Ctrl Pts',(13.5637332022473,-22.0368009736295,
0.));
#222396=CARTESIAN_POINT('Ctrl Pts',(13.5648113689033,-22.065039308961,0.));
#222397=CARTESIAN_POINT('Ctrl Pts',(13.5658294169284,-22.0933486464593,
0.));
#222398=CARTESIAN_POINT('Ctrl Pts',(13.5667873105359,-22.1217288871975,
0.));
#222399=CARTESIAN_POINT('Ctrl Pts',(13.5675054919061,-22.1444897575194,
0.));
#222400=CARTESIAN_POINT('Ctrl Pts',(13.5680170531805,-22.1615922805008,
0.));
#222401=CARTESIAN_POINT('Ctrl Pts',(13.5683460612942,-22.1730081264608,
0.));
#222402=CARTESIAN_POINT('Ctrl Pts',(13.5685075571671,-22.178719590434,0.));
#222403=CARTESIAN_POINT('',(13.5685075571671,-22.178719590434,12.));
#222404=CARTESIAN_POINT('Ctrl Pts',(13.5685075571671,-22.178719590434,12.));
#222405=CARTESIAN_POINT('Ctrl Pts',(13.5683460612942,-22.1730081264608,
12.));
#222406=CARTESIAN_POINT('Ctrl Pts',(13.5680170531805,-22.1615922805008,
12.));
#222407=CARTESIAN_POINT('Ctrl Pts',(13.5675054919061,-22.1444897575194,
12.));
#222408=CARTESIAN_POINT('Ctrl Pts',(13.5667873105359,-22.1217288871975,
12.));
#222409=CARTESIAN_POINT('Ctrl Pts',(13.5658294169284,-22.0933486464593,
12.));
#222410=CARTESIAN_POINT('Ctrl Pts',(13.5648113689033,-22.065039308961,12.));
#222411=CARTESIAN_POINT('Ctrl Pts',(13.5637332022473,-22.0368009736295,
12.));
#222412=CARTESIAN_POINT('Ctrl Pts',(13.5625949868333,-22.0086337943449,
12.));
#222413=CARTESIAN_POINT('Ctrl Pts',(13.5613968357561,-21.9805379899168,
12.));
#222414=CARTESIAN_POINT('Ctrl Pts',(13.5601389185257,-21.9525138592813,
12.));
#222415=CARTESIAN_POINT('Ctrl Pts',(13.5588214586604,-21.9245617765769,
12.));
#222416=CARTESIAN_POINT('Ctrl Pts',(13.5574447178424,-21.8966821688824,
12.));
#222417=CARTESIAN_POINT('Ctrl Pts',(13.5560089839385,-21.8688754989365,
12.));
#222418=CARTESIAN_POINT('Ctrl Pts',(13.5545145573031,-21.8411422456075,
12.));
#222419=CARTESIAN_POINT('Ctrl Pts',(13.5529617381573,-21.8134828857967,
12.));
#222420=CARTESIAN_POINT('Ctrl Pts',(13.551350812725,-21.7858978745865,12.));
#222421=CARTESIAN_POINT('Ctrl Pts',(13.5496820422211,-21.7583876294554,
12.));
#222422=CARTESIAN_POINT('Ctrl Pts',(13.5479556704481,-21.7309525412281,
12.));
#222423=CARTESIAN_POINT('Ctrl Pts',(13.5461719295048,-21.7035929822955,
12.));
#222424=CARTESIAN_POINT('Ctrl Pts',(13.5443310461526,-21.6763093157699,
12.));
#222425=CARTESIAN_POINT('Ctrl Pts',(13.5424332480699,-21.6491019044648,
12.));
#222426=CARTESIAN_POINT('Ctrl Pts',(13.5404787697791,-21.6219711193946,
12.));
#222427=CARTESIAN_POINT('Ctrl Pts',(13.5384678597195,-21.5949173499013,
12.));
#222428=CARTESIAN_POINT('Ctrl Pts',(13.536400779028,-21.5679410019002,12.));
#222429=CARTESIAN_POINT('Ctrl Pts',(13.5342777983214,-21.5410424932503,
12.));
#222430=CARTESIAN_POINT('Ctrl Pts',(13.5320991952138,-21.5142222501666,
12.));
#222431=CARTESIAN_POINT('Ctrl Pts',(13.5298652514355,-21.4874807030468,
12.));
#222432=CARTESIAN_POINT('Ctrl Pts',(13.5275762503555,-21.4608182828697,
12.));
#222433=CARTESIAN_POINT('Ctrl Pts',(13.5252324737801,-21.4342354165259,
12.));
#222434=CARTESIAN_POINT('Ctrl Pts',(13.5228342013516,-21.4077325259324,
12.));
#222435=CARTESIAN_POINT('Ctrl Pts',(13.5203817122503,-21.3813100304973,
12.));
#222436=CARTESIAN_POINT('Ctrl Pts',(13.5178752862466,-21.3549683486222,
12.));
#222437=CARTESIAN_POINT('Ctrl Pts',(13.5153152050555,-21.3287078996341,
12.));
#222438=CARTESIAN_POINT('Ctrl Pts',(13.5127017534971,-21.3025291054235,
12.));
#222439=CARTESIAN_POINT('Ctrl Pts',(13.5100352209205,-21.2764323924442,
12.));
#222440=CARTESIAN_POINT('Ctrl Pts',(13.5073159019452,-21.250418192743,12.));
#222441=CARTESIAN_POINT('Ctrl Pts',(13.5045440957404,-21.2244869429332,
12.));
#222442=CARTESIAN_POINT('Ctrl Pts',(13.5017201056088,-21.1986390835828,
12.));
#222443=CARTESIAN_POINT('Ctrl Pts',(13.4988442384491,-21.1728750584175,
12.));
#222444=CARTESIAN_POINT('Ctrl Pts',(13.4959168042934,-21.1471953136209,
12.));
#222445=CARTESIAN_POINT('Ctrl Pts',(13.4929381157778,-21.1216002970207,
12.));
#222446=CARTESIAN_POINT('Ctrl Pts',(13.4899084877717,-21.0960904575046,
12.));
#222447=CARTESIAN_POINT('Ctrl Pts',(13.4868282377191,-21.0706662455199,
12.));
#222448=CARTESIAN_POINT('Ctrl Pts',(13.4836976858912,-21.0453281134245,
12.));
#222449=CARTESIAN_POINT('Ctrl Pts',(13.4805171556822,-21.0200765158884,
12.));
#222450=CARTESIAN_POINT('Ctrl Pts',(13.4772869738878,-20.9949119102592,
12.));
#222451=CARTESIAN_POINT('Ctrl Pts',(13.4740074710086,-20.9698347569477,
12.));
#222452=CARTESIAN_POINT('Ctrl Pts',(13.4706789815166,-20.9448455197557,
12.));
#222453=CARTESIAN_POINT('Ctrl Pts',(13.4673018437717,-20.9199446657583,
12.));
#222454=CARTESIAN_POINT('Ctrl Pts',(13.4638763999725,-20.8951326652158,
12.));
#222455=CARTESIAN_POINT('Ctrl Pts',(13.4604029960983,-20.8704099914641,
12.));
#222456=CARTESIAN_POINT('Ctrl Pts',(13.4568819818631,-20.8457771208083,
12.));
#222457=CARTESIAN_POINT('Ctrl Pts',(13.4533137106667,-20.821234532398,12.));
#222458=CARTESIAN_POINT('Ctrl Pts',(13.4496985395637,-20.7967827081228,
12.));
#222459=CARTESIAN_POINT('Ctrl Pts',(13.4460368293689,-20.7724221327609,
12.));
#222460=CARTESIAN_POINT('Ctrl Pts',(13.4423289447561,-20.7481532941014,
12.));
#222461=CARTESIAN_POINT('Ctrl Pts',(13.4385752543663,-20.7239766830676,
12.));
#222462=CARTESIAN_POINT('Ctrl Pts',(13.4347761309154,-20.6998927938288,
12.));
#222463=CARTESIAN_POINT('Ctrl Pts',(13.4309319513119,-20.6759021239102,
12.));
#222464=CARTESIAN_POINT('Ctrl Pts',(13.427043096765,-20.6520051742868,12.));
#222465=CARTESIAN_POINT('Ctrl Pts',(13.4231099528178,-20.6282024494234,
12.));
#222466=CARTESIAN_POINT('Ctrl Pts',(13.4191329093931,-20.6044944573151,
12.));
#222467=CARTESIAN_POINT('Ctrl Pts',(13.415112360841,-20.5808817095155,12.));
#222468=CARTESIAN_POINT('Ctrl Pts',(13.4110487059912,-20.557364721164,12.));
#222469=CARTESIAN_POINT('Ctrl Pts',(13.4069423482076,-20.5339440109958,
12.));
#222470=CARTESIAN_POINT('Ctrl Pts',(13.4027936954529,-20.5106201013755,
12.));
#222471=CARTESIAN_POINT('Ctrl Pts',(13.3986031603716,-20.4873935184041,
12.));
#222472=CARTESIAN_POINT('Ctrl Pts',(13.3943711603739,-20.4642647920038,
12.));
#222473=CARTESIAN_POINT('Ctrl Pts',(13.3900981177254,-20.4412344560007,
12.));
#222474=CARTESIAN_POINT('Ctrl Pts',(13.3857844596387,-20.4183030482002,
12.));
#222475=CARTESIAN_POINT('Ctrl Pts',(13.3814306183721,-20.3954711104505,
12.));
#222476=CARTESIAN_POINT('Ctrl Pts',(13.377037031319,-20.3727391887187,12.));
#222477=CARTESIAN_POINT('Ctrl Pts',(13.3726041410869,-20.3501078331818,
12.));
#222478=CARTESIAN_POINT('Ctrl Pts',(13.3681323955828,-20.3275775983032,
12.));
#222479=CARTESIAN_POINT('Ctrl Pts',(13.3636222481016,-20.3051490429049,
12.));
#222480=CARTESIAN_POINT('Ctrl Pts',(13.3590741574194,-20.2828227302337,
12.));
#222481=CARTESIAN_POINT('Ctrl Pts',(13.3544885878886,-20.2605992280117,
12.));
#222482=CARTESIAN_POINT('Ctrl Pts',(13.3498660095381,-20.2384791085354,
12.));
#222483=CARTESIAN_POINT('Ctrl Pts',(13.3452068981762,-20.2164629487855,
12.));
#222484=CARTESIAN_POINT('Ctrl Pts',(13.3405117354969,-20.1945513305233,
12.));
#222485=CARTESIAN_POINT('Ctrl Pts',(13.3357810091903,-20.1727448403818,
12.));
#222486=CARTESIAN_POINT('Ctrl Pts',(13.3310152130565,-20.1510440699477,
12.));
#222487=CARTESIAN_POINT('Ctrl Pts',(13.3262148471228,-20.1294496158405,
12.));
#222488=CARTESIAN_POINT('Ctrl Pts',(13.3213804177588,-20.1079620798377,
12.));
#222489=CARTESIAN_POINT('Ctrl Pts',(13.3165124377962,-20.0865820689884,
12.));
#222490=CARTESIAN_POINT('Ctrl Pts',(13.3116114266514,-20.0653101957188,
12.));
#222491=CARTESIAN_POINT('Ctrl Pts',(13.3066779104515,-20.0441470779345,
12.));
#222492=CARTESIAN_POINT('Ctrl Pts',(13.3017124221639,-20.023093339104,12.));
#222493=CARTESIAN_POINT('Ctrl Pts',(13.296715501731,-20.0021496083742,12.));
#222494=CARTESIAN_POINT('Ctrl Pts',(13.2916876962098,-19.9813165207174,
12.));
#222495=CARTESIAN_POINT('Ctrl Pts',(13.2866295599152,-19.9605947170589,
12.));
#222496=CARTESIAN_POINT('Ctrl Pts',(13.2815416545662,-19.939984844402,12.));
#222497=CARTESIAN_POINT('Ctrl Pts',(13.2764245494354,-19.9194875559419,
12.));
#222498=CARTESIAN_POINT('Ctrl Pts',(13.2712788215015,-19.8991035111739,
12.));
#222499=CARTESIAN_POINT('Ctrl Pts',(13.2661050556128,-19.8788333760571,
12.));
#222500=CARTESIAN_POINT('Ctrl Pts',(13.2609038446525,-19.8586778231711,
12.));
#222501=CARTESIAN_POINT('Ctrl Pts',(13.2556757897085,-19.8386375318632,
12.));
#222502=CARTESIAN_POINT('Ctrl Pts',(13.2504215002458,-19.8187131883919,
12.));
#222503=CARTESIAN_POINT('Ctrl Pts',(13.2451415942809,-19.7989054860501,
12.));
#222504=CARTESIAN_POINT('Ctrl Pts',(13.239836698568,-19.7792151253297,12.));
#222505=CARTESIAN_POINT('Ctrl Pts',(13.2345074487968,-19.7596428141176,
12.));
#222506=CARTESIAN_POINT('Ctrl Pts',(13.2291544897902,-19.7401892678701,
12.));
#222507=CARTESIAN_POINT('Ctrl Pts',(13.2237784757065,-19.7208552097867,
12.));
#222508=CARTESIAN_POINT('Ctrl Pts',(13.2183800702431,-19.7016413709678,
12.));
#222509=CARTESIAN_POINT('Ctrl Pts',(13.2129599468478,-19.6825484905812,
12.));
#222510=CARTESIAN_POINT('Ctrl Pts',(13.2075187889522,-19.6635773160924,
12.));
#222511=CARTESIAN_POINT('Ctrl Pts',(13.202057290206,-19.6447286034764,12.));
#222512=CARTESIAN_POINT('Ctrl Pts',(13.196576154715,-19.6260031174244,12.));
#222513=CARTESIAN_POINT('Ctrl Pts',(13.1910760972818,-19.6074016315421,
12.));
#222514=CARTESIAN_POINT('Ctrl Pts',(13.1855578436479,-19.5889249285352,
12.));
#222515=CARTESIAN_POINT('Ctrl Pts',(13.1800221307682,-19.5705738004682,
12.));
#222516=CARTESIAN_POINT('Ctrl Pts',(13.1744697070918,-19.5523490490254,
12.));
#222517=CARTESIAN_POINT('Ctrl Pts',(13.1689013328432,-19.5342514857564,
12.));
#222518=CARTESIAN_POINT('Ctrl Pts',(13.1633177803097,-19.5162819323207,
12.));
#222519=CARTESIAN_POINT('Ctrl Pts',(13.1577198341238,-19.498441220707,12.));
#222520=CARTESIAN_POINT('Ctrl Pts',(13.1521082915846,-19.4807301935256,
12.));
#222521=CARTESIAN_POINT('Ctrl Pts',(13.1464839629966,-19.463149704325,12.));
#222522=CARTESIAN_POINT('Ctrl Pts',(13.140847672006,-19.4457006178875,12.));
#222523=CARTESIAN_POINT('Ctrl Pts',(13.1352002559439,-19.4283838105265,
12.));
#222524=CARTESIAN_POINT('Ctrl Pts',(13.1295425661635,-19.4112001703561,
12.));
#222525=CARTESIAN_POINT('Ctrl Pts',(13.1238754684177,-19.3941505976267,
12.));
#222526=CARTESIAN_POINT('Ctrl Pts',(13.118199843271,-19.3772360051093,12.));
#222527=CARTESIAN_POINT('Ctrl Pts',(13.1125165865021,-19.3604573184516,
12.));
#222528=CARTESIAN_POINT('Ctrl Pts',(13.1068266095186,-19.3438154765395,
12.));
#222529=CARTESIAN_POINT('Ctrl Pts',(13.1011308397591,-19.3273114318268,
12.));
#222530=CARTESIAN_POINT('Ctrl Pts',(13.095430221148,-19.3109461507358,12.));
#222531=CARTESIAN_POINT('Ctrl Pts',(13.0897257145969,-19.2947206141246,
12.));
#222532=CARTESIAN_POINT('Ctrl Pts',(13.0840182984949,-19.2786358177198,
12.));
#222533=CARTESIAN_POINT('Ctrl Pts',(13.0783089692117,-19.2626927725596,
12.));
#222534=CARTESIAN_POINT('Ctrl Pts',(13.0725987415856,-19.2468925053988,
12.));
#222535=CARTESIAN_POINT('Ctrl Pts',(13.0668886494791,-19.2312360592031,
12.));
#222536=CARTESIAN_POINT('Ctrl Pts',(13.0611797463912,-19.2157244937141,
12.));
#222537=CARTESIAN_POINT('Ctrl Pts',(13.0554731060537,-19.2003588859771,
12.));
#222538=CARTESIAN_POINT('Ctrl Pts',(13.0497698230442,-19.1851403308826,
12.));
#222539=CARTESIAN_POINT('Ctrl Pts',(13.0440710133775,-19.1700699416625,
12.));
#222540=CARTESIAN_POINT('Ctrl Pts',(13.0383778152072,-19.1551488505233,
12.));
#222541=CARTESIAN_POINT('Ctrl Pts',(13.0326913895841,-19.1403782093389,
12.));
#222542=CARTESIAN_POINT('Ctrl Pts',(13.0270129211976,-19.1257591903099,
12.));
#222543=CARTESIAN_POINT('Ctrl Pts',(13.0213436191326,-19.1112929866308,
12.));
#222544=CARTESIAN_POINT('Ctrl Pts',(13.0156847176093,-19.0969808131226,
12.));
#222545=CARTESIAN_POINT('Ctrl Pts',(13.0100374768785,-19.0828239070482,
12.));
#222546=CARTESIAN_POINT('Ctrl Pts',(13.0044031841381,-19.0688235289437,
12.));
#222547=CARTESIAN_POINT('Ctrl Pts',(12.9987831544502,-19.0549809634355,
12.));
#222548=CARTESIAN_POINT('Ctrl Pts',(12.9931787316514,-19.0412975200398,
12.));
#222549=CARTESIAN_POINT('Ctrl Pts',(12.9875912893003,-19.0277745339908,
12.));
#222550=CARTESIAN_POINT('Ctrl Pts',(12.9820222318715,-19.0144133673348,
12.));
#222551=CARTESIAN_POINT('Ctrl Pts',(12.9764729959205,-19.0012154099791,
12.));
#222552=CARTESIAN_POINT('Ctrl Pts',(12.9709450512747,-18.9881820807586,
12.));
#222553=CARTESIAN_POINT('Ctrl Pts',(12.9654399021869,-18.9753148284475,
12.));
#222554=CARTESIAN_POINT('Ctrl Pts',(12.9599590886319,-18.9626151329229,
12.));
#222555=CARTESIAN_POINT('Ctrl Pts',(12.9545041877377,-18.9500845064715,
12.));
#222556=CARTESIAN_POINT('Ctrl Pts',(12.9490768151821,-18.9377244950435,
12.));
#222557=CARTESIAN_POINT('Ctrl Pts',(12.9436786266105,-18.9255366795195,
12.));
#222558=CARTESIAN_POINT('Ctrl Pts',(12.9383113190374,-18.9135226769466,
12.));
#222559=CARTESIAN_POINT('Ctrl Pts',(12.9329766328184,-18.9016841423403,
12.));
#222560=CARTESIAN_POINT('Ctrl Pts',(12.9276763536373,-18.8900227704889,
12.));
#222561=CARTESIAN_POINT('Ctrl Pts',(12.9224123144981,-18.8785402977528,
12.));
#222562=CARTESIAN_POINT('Ctrl Pts',(12.9171863977045,-18.8672385038326,
12.));
#222563=CARTESIAN_POINT('Ctrl Pts',(12.9120005369063,-18.8561192136198,
12.));
#222564=CARTESIAN_POINT('Ctrl Pts',(12.9068567191854,-18.8451842990984,
12.));
#222565=CARTESIAN_POINT('Ctrl Pts',(12.9017569871738,-18.8344356812591,
12.));
#222566=CARTESIAN_POINT('Ctrl Pts',(12.8967034410754,-18.8238753319129,
12.));
#222567=CARTESIAN_POINT('Ctrl Pts',(12.8916982409935,-18.813505275782,12.));
#222568=CARTESIAN_POINT('Ctrl Pts',(12.8867436109546,-18.8033275941943,
12.));
#222569=CARTESIAN_POINT('Ctrl Pts',(12.8818418427475,-18.7933444285868,
12.));
#222570=CARTESIAN_POINT('Ctrl Pts',(12.8769952998095,-18.7835579840477,
12.));
#222571=CARTESIAN_POINT('Ctrl Pts',(12.872206421181,-18.7739705329022,12.));
#222572=CARTESIAN_POINT('Ctrl Pts',(12.8674777239653,-18.7645844169564,
12.));
#222573=CARTESIAN_POINT('Ctrl Pts',(12.8628118054171,-18.7554020493887,
12.));
#222574=CARTESIAN_POINT('Ctrl Pts',(12.8582113455646,-18.7464259171251,
12.));
#222575=CARTESIAN_POINT('Ctrl Pts',(12.8536791086316,-18.7376585820854,
12.));
#222576=CARTESIAN_POINT('Ctrl Pts',(12.8492179511591,-18.7291026886554,
12.));
#222577=CARTESIAN_POINT('Ctrl Pts',(12.8448308329494,-18.7207609737702,
12.));
#222578=CARTESIAN_POINT('Ctrl Pts',(12.8405208263431,-18.7126362754445,
12.));
#222579=CARTESIAN_POINT('Ctrl Pts',(12.8362911280361,-18.7047315436294,
12.));
#222580=CARTESIAN_POINT('Ctrl Pts',(12.8321450599789,-18.6970498410172,
12.));
#222581=CARTESIAN_POINT('Ctrl Pts',(12.8280860635231,-18.6895943376172,
12.));
#222582=CARTESIAN_POINT('Ctrl Pts',(12.8241176980017,-18.6823683094139,
12.));
#222583=CARTESIAN_POINT('Ctrl Pts',(12.8202436318474,-18.6753751301092,
12.));
#222584=CARTESIAN_POINT('Ctrl Pts',(12.8164676687362,-18.66861829528,12.));
#222585=CARTESIAN_POINT('Ctrl Pts',(12.8127937909631,-18.6621014624746,
12.));
#222586=CARTESIAN_POINT('Ctrl Pts',(12.8092261933858,-18.6558284825773,
12.));
#222587=CARTESIAN_POINT('Ctrl Pts',(12.805769331162,-18.6498034438987,12.));
#222588=CARTESIAN_POINT('Ctrl Pts',(12.8024278770152,-18.6440306327456,
12.));
#222589=CARTESIAN_POINT('Ctrl Pts',(12.7992066625264,-18.63851447924,12.));
#222590=CARTESIAN_POINT('Ctrl Pts',(12.796110622225,-18.6332595057006,12.));
#222591=CARTESIAN_POINT('Ctrl Pts',(12.7931447451555,-18.6282702819371,
12.));
#222592=CARTESIAN_POINT('Ctrl Pts',(12.7903142925234,-18.6235516265575,
12.));
#222593=CARTESIAN_POINT('Ctrl Pts',(12.7876249657834,-18.6191087624752,
12.));
#222594=CARTESIAN_POINT('Ctrl Pts',(12.7850831657901,-18.6149475565188,
12.));
#222595=CARTESIAN_POINT('Ctrl Pts',(12.7826959526924,-18.611074482622,12.));
#222596=CARTESIAN_POINT('Ctrl Pts',(12.7804705387658,-18.6074961535723,
12.));
#222597=CARTESIAN_POINT('Ctrl Pts',(12.7784139605066,-18.6042190183704,
12.));
#222598=CARTESIAN_POINT('Ctrl Pts',(12.7765325225081,-18.6012488486709,
12.));
#222599=CARTESIAN_POINT('Ctrl Pts',(12.7748328937638,-18.598591752595,12.));
#222600=CARTESIAN_POINT('Ctrl Pts',(12.7733231262108,-18.5962551167772,
12.));
#222601=CARTESIAN_POINT('Ctrl Pts',(12.7720142287172,-18.5942490615407,
12.));
#222602=CARTESIAN_POINT('Ctrl Pts',(12.7709195951156,-18.5925859134579,
12.));
#222603=CARTESIAN_POINT('Ctrl Pts',(12.7700520897173,-18.5912775137806,
12.));
#222604=CARTESIAN_POINT('Ctrl Pts',(12.7694215127918,-18.5903328777227,
12.));
#222605=CARTESIAN_POINT('Ctrl Pts',(12.769110348199,-18.589871621843,12.));
#222606=CARTESIAN_POINT('Ctrl Pts',(12.768986426692,-18.5896919669165,12.));
#222607=CARTESIAN_POINT('Ctrl Pts',(12.7689524524483,-18.5896460962964,
12.));
#222608=CARTESIAN_POINT('Ctrl Pts',(12.7689476255362,-18.5896416359912,
12.));
#222609=CARTESIAN_POINT('',(13.5685075571671,-22.178719590434,0.));
#222610=CARTESIAN_POINT('Origin',(7.17139709155223,-20.2687213152502,0.));
#222611=CARTESIAN_POINT('',(7.52250298901263,-21.2610617890679,12.));
#222612=CARTESIAN_POINT('',(3.58569854577611,-10.1343606576251,12.));
#222613=CARTESIAN_POINT('',(7.52250298901263,-21.2610617890679,0.));
#222614=CARTESIAN_POINT('',(7.52250298901263,-21.2610617890679,0.));
#222615=CARTESIAN_POINT('',(3.58569854577611,-10.1343606576251,0.));
#222616=CARTESIAN_POINT('Ctrl Pts',(12.4230808101438,-22.8400320311649,
0.));
#222617=CARTESIAN_POINT('Ctrl Pts',(12.4230808101438,-22.8400320311649,
12.));
#222618=CARTESIAN_POINT('Ctrl Pts',(12.418215285186,-22.8370364396459,0.));
#222619=CARTESIAN_POINT('Ctrl Pts',(12.418215285186,-22.8370364396459,12.));
#222620=CARTESIAN_POINT('Ctrl Pts',(12.4084933766346,-22.8310435872748,
0.));
#222621=CARTESIAN_POINT('Ctrl Pts',(12.4084933766346,-22.8310435872748,
12.));
#222622=CARTESIAN_POINT('Ctrl Pts',(12.3939379378998,-22.8220493007173,
0.));
#222623=CARTESIAN_POINT('Ctrl Pts',(12.3939379378998,-22.8220493007173,
12.));
#222624=CARTESIAN_POINT('Ctrl Pts',(12.374585536673,-22.81004690224,0.));
#222625=CARTESIAN_POINT('Ctrl Pts',(12.374585536673,-22.81004690224,12.));
#222626=CARTESIAN_POINT('Ctrl Pts',(12.3504864740319,-22.795027221673,0.));
#222627=CARTESIAN_POINT('Ctrl Pts',(12.3504864740319,-22.795027221673,12.));
#222628=CARTESIAN_POINT('Ctrl Pts',(12.3264788926075,-22.7799908974768,
0.));
#222629=CARTESIAN_POINT('Ctrl Pts',(12.3264788926075,-22.7799908974768,
12.));
#222630=CARTESIAN_POINT('Ctrl Pts',(12.3025628601792,-22.764938010105,0.));
#222631=CARTESIAN_POINT('Ctrl Pts',(12.3025628601792,-22.764938010105,12.));
#222632=CARTESIAN_POINT('Ctrl Pts',(12.2787384750742,-22.7498686970069,
0.));
#222633=CARTESIAN_POINT('Ctrl Pts',(12.2787384750742,-22.7498686970069,
12.));
#222634=CARTESIAN_POINT('Ctrl Pts',(12.2550058702395,-22.7347831655287,
0.));
#222635=CARTESIAN_POINT('Ctrl Pts',(12.2550058702395,-22.7347831655287,
12.));
#222636=CARTESIAN_POINT('Ctrl Pts',(12.2313652198061,-22.7196817119374,
0.));
#222637=CARTESIAN_POINT('Ctrl Pts',(12.2313652198061,-22.7196817119374,
12.));
#222638=CARTESIAN_POINT('Ctrl Pts',(12.2078167360284,-22.7045647168747,
0.));
#222639=CARTESIAN_POINT('Ctrl Pts',(12.2078167360284,-22.7045647168747,
12.));
#222640=CARTESIAN_POINT('Ctrl Pts',(12.1843606579261,-22.6894326205037,
0.));
#222641=CARTESIAN_POINT('Ctrl Pts',(12.1843606579261,-22.6894326205037,
12.));
#222642=CARTESIAN_POINT('Ctrl Pts',(12.1609972423099,-22.6742859034944,
0.));
#222643=CARTESIAN_POINT('Ctrl Pts',(12.1609972423099,-22.6742859034944,
12.));
#222644=CARTESIAN_POINT('Ctrl Pts',(12.1377267537145,-22.6591250653965,
0.));
#222645=CARTESIAN_POINT('Ctrl Pts',(12.1377267537145,-22.6591250653965,
12.));
#222646=CARTESIAN_POINT('Ctrl Pts',(12.1145494550383,-22.6439506046605,
0.));
#222647=CARTESIAN_POINT('Ctrl Pts',(12.1145494550383,-22.6439506046605,
12.));
#222648=CARTESIAN_POINT('Ctrl Pts',(12.0914655972823,-22.6287629967056,
0.));
#222649=CARTESIAN_POINT('Ctrl Pts',(12.0914655972823,-22.6287629967056,
12.));
#222650=CARTESIAN_POINT('Ctrl Pts',(12.0684754113862,-22.6135626764898,
0.));
#222651=CARTESIAN_POINT('Ctrl Pts',(12.0684754113862,-22.6135626764898,
12.));
#222652=CARTESIAN_POINT('Ctrl Pts',(12.0455791139128,-22.5983500505644,
0.));
#222653=CARTESIAN_POINT('Ctrl Pts',(12.0455791139128,-22.5983500505644,
12.));
#222654=CARTESIAN_POINT('Ctrl Pts',(12.0227769113127,-22.5831255061282,
0.));
#222655=CARTESIAN_POINT('Ctrl Pts',(12.0227769113127,-22.5831255061282,
12.));
#222656=CARTESIAN_POINT('Ctrl Pts',(12.0000690046694,-22.5678894211181,
0.));
#222657=CARTESIAN_POINT('Ctrl Pts',(12.0000690046694,-22.5678894211181,
12.));
#222658=CARTESIAN_POINT('Ctrl Pts',(11.9774555943496,-22.5526421741158,
0.));
#222659=CARTESIAN_POINT('Ctrl Pts',(11.9774555943496,-22.5526421741158,
12.));
#222660=CARTESIAN_POINT('Ctrl Pts',(11.9549368843997,-22.5373841537307,
0.));
#222661=CARTESIAN_POINT('Ctrl Pts',(11.9549368843997,-22.5373841537307,
12.));
#222662=CARTESIAN_POINT('Ctrl Pts',(11.9325130877803,-22.5221157697883,
0.));
#222663=CARTESIAN_POINT('Ctrl Pts',(11.9325130877803,-22.5221157697883,
12.));
#222664=CARTESIAN_POINT('Ctrl Pts',(11.9101844254557,-22.5068374513973,
0.));
#222665=CARTESIAN_POINT('Ctrl Pts',(11.9101844254557,-22.5068374513973,
12.));
#222666=CARTESIAN_POINT('Ctrl Pts',(11.8879511239942,-22.4915496418485,
0.));
#222667=CARTESIAN_POINT('Ctrl Pts',(11.8879511239942,-22.4915496418485,
12.));
#222668=CARTESIAN_POINT('Ctrl Pts',(11.8658134137019,-22.4762527946702,
0.));
#222669=CARTESIAN_POINT('Ctrl Pts',(11.8658134137019,-22.4762527946702,
12.));
#222670=CARTESIAN_POINT('Ctrl Pts',(11.8437715264487,-22.4609473690472,
0.));
#222671=CARTESIAN_POINT('Ctrl Pts',(11.8437715264487,-22.4609473690472,
12.));
#222672=CARTESIAN_POINT('Ctrl Pts',(11.8218256937889,-22.4456338258735,
0.));
#222673=CARTESIAN_POINT('Ctrl Pts',(11.8218256937889,-22.4456338258735,
12.));
#222674=CARTESIAN_POINT('Ctrl Pts',(11.7999761445173,-22.430312622646,0.));
#222675=CARTESIAN_POINT('Ctrl Pts',(11.7999761445173,-22.430312622646,12.));
#222676=CARTESIAN_POINT('Ctrl Pts',(11.7782231042039,-22.4149842125008,
0.));
#222677=CARTESIAN_POINT('Ctrl Pts',(11.7782231042039,-22.4149842125008,
12.));
#222678=CARTESIAN_POINT('Ctrl Pts',(11.7565667964764,-22.3996490469191,
0.));
#222679=CARTESIAN_POINT('Ctrl Pts',(11.7565667964764,-22.3996490469191,
12.));
#222680=CARTESIAN_POINT('Ctrl Pts',(11.7350074437961,-22.3843075773899,
0.));
#222681=CARTESIAN_POINT('Ctrl Pts',(11.7350074437961,-22.3843075773899,
12.));
#222682=CARTESIAN_POINT('Ctrl Pts',(11.7135452684532,-22.3689602575491,
0.));
#222683=CARTESIAN_POINT('Ctrl Pts',(11.7135452684532,-22.3689602575491,
12.));
#222684=CARTESIAN_POINT('Ctrl Pts',(11.6921804934056,-22.3536075450029,
0.));
#222685=CARTESIAN_POINT('Ctrl Pts',(11.6921804934056,-22.3536075450029,
12.));
#222686=CARTESIAN_POINT('Ctrl Pts',(11.6709133432985,-22.3382499035619,
0.));
#222687=CARTESIAN_POINT('Ctrl Pts',(11.6709133432985,-22.3382499035619,
12.));
#222688=CARTESIAN_POINT('Ctrl Pts',(11.6497440449857,-22.3228878043976,
0.));
#222689=CARTESIAN_POINT('Ctrl Pts',(11.6497440449857,-22.3228878043976,
12.));
#222690=CARTESIAN_POINT('Ctrl Pts',(11.6286728270009,-22.3075217249049,
0.));
#222691=CARTESIAN_POINT('Ctrl Pts',(11.6286728270009,-22.3075217249049,
12.));
#222692=CARTESIAN_POINT('Ctrl Pts',(11.6076999192357,-22.2921521480356,
0.));
#222693=CARTESIAN_POINT('Ctrl Pts',(11.6076999192357,-22.2921521480356,
12.));
#222694=CARTESIAN_POINT('Ctrl Pts',(11.5868255525188,-22.2767795614348,
0.));
#222695=CARTESIAN_POINT('Ctrl Pts',(11.5868255525188,-22.2767795614348,
12.));
#222696=CARTESIAN_POINT('Ctrl Pts',(11.5660499582403,-22.2614044566898,
0.));
#222697=CARTESIAN_POINT('Ctrl Pts',(11.5660499582403,-22.2614044566898,
12.));
#222698=CARTESIAN_POINT('Ctrl Pts',(11.5453733679121,-22.2460273284654,
0.));
#222699=CARTESIAN_POINT('Ctrl Pts',(11.5453733679121,-22.2460273284654,
12.));
#222700=CARTESIAN_POINT('Ctrl Pts',(11.5247960128477,-22.2306486738901,
0.));
#222701=CARTESIAN_POINT('Ctrl Pts',(11.5247960128477,-22.2306486738901,
12.));
#222702=CARTESIAN_POINT('Ctrl Pts',(11.5043181244242,-22.2152689931022,
0.));
#222703=CARTESIAN_POINT('Ctrl Pts',(11.5043181244242,-22.2152689931022,
12.));
#222704=CARTESIAN_POINT('Ctrl Pts',(11.483939934259,-22.1998887896436,0.));
#222705=CARTESIAN_POINT('Ctrl Pts',(11.483939934259,-22.1998887896436,12.));
#222706=CARTESIAN_POINT('Ctrl Pts',(11.463661674411,-22.184508570917,0.));
#222707=CARTESIAN_POINT('Ctrl Pts',(11.463661674411,-22.184508570917,12.));
#222708=CARTESIAN_POINT('Ctrl Pts',(11.443483577557,-22.1691288486096,0.));
#222709=CARTESIAN_POINT('Ctrl Pts',(11.443483577557,-22.1691288486096,12.));
#222710=CARTESIAN_POINT('Ctrl Pts',(11.4234058771742,-22.1537501391487,
0.));
#222711=CARTESIAN_POINT('Ctrl Pts',(11.4234058771742,-22.1537501391487,
12.));
#222712=CARTESIAN_POINT('Ctrl Pts',(11.4034288076908,-22.1383729640964,
0.));
#222713=CARTESIAN_POINT('Ctrl Pts',(11.4034288076908,-22.1383729640964,
12.));
#222714=CARTESIAN_POINT('Ctrl Pts',(11.3835526044256,-22.1229978500186,
0.));
#222715=CARTESIAN_POINT('Ctrl Pts',(11.3835526044256,-22.1229978500186,
12.));
#222716=CARTESIAN_POINT('Ctrl Pts',(11.3637775035367,-22.1076253283979,
0.));
#222717=CARTESIAN_POINT('Ctrl Pts',(11.3637775035367,-22.1076253283979,
12.));
#222718=CARTESIAN_POINT('Ctrl Pts',(11.3441037419553,-22.0922559355294,
0.));
#222719=CARTESIAN_POINT('Ctrl Pts',(11.3441037419553,-22.0922559355294,
12.));
#222720=CARTESIAN_POINT('Ctrl Pts',(11.3245315573168,-22.0768902124267,
0.));
#222721=CARTESIAN_POINT('Ctrl Pts',(11.3245315573168,-22.0768902124267,
12.));
#222722=CARTESIAN_POINT('Ctrl Pts',(11.3050611878771,-22.0615287047179,
0.));
#222723=CARTESIAN_POINT('Ctrl Pts',(11.3050611878771,-22.0615287047179,
12.));
#222724=CARTESIAN_POINT('Ctrl Pts',(11.2856928724374,-22.046171962566,0.));
#222725=CARTESIAN_POINT('Ctrl Pts',(11.2856928724374,-22.046171962566,12.));
#222726=CARTESIAN_POINT('Ctrl Pts',(11.2664268504206,-22.030820540835,0.));
#222727=CARTESIAN_POINT('Ctrl Pts',(11.2664268504206,-22.030820540835,12.));
#222728=CARTESIAN_POINT('Ctrl Pts',(11.2472633619275,-22.0154749992363,
0.));
#222729=CARTESIAN_POINT('Ctrl Pts',(11.2472633619275,-22.0154749992363,
12.));
#222730=CARTESIAN_POINT('Ctrl Pts',(11.2282026477896,-22.0001359024839,
0.));
#222731=CARTESIAN_POINT('Ctrl Pts',(11.2282026477896,-22.0001359024839,
12.));
#222732=CARTESIAN_POINT('Ctrl Pts',(11.2092449496125,-21.9848038204439,
0.));
#222733=CARTESIAN_POINT('Ctrl Pts',(11.2092449496125,-21.9848038204439,
12.));
#222734=CARTESIAN_POINT('Ctrl Pts',(11.190390509811,-21.9694793282914,0.));
#222735=CARTESIAN_POINT('Ctrl Pts',(11.190390509811,-21.9694793282914,12.));
#222736=CARTESIAN_POINT('Ctrl Pts',(11.1716395716376,-21.9541630066506,
0.));
#222737=CARTESIAN_POINT('Ctrl Pts',(11.1716395716376,-21.9541630066506,
12.));
#222738=CARTESIAN_POINT('Ctrl Pts',(11.1529923792003,-21.9388554416439,
0.));
#222739=CARTESIAN_POINT('Ctrl Pts',(11.1529923792003,-21.9388554416439,
12.));
#222740=CARTESIAN_POINT('Ctrl Pts',(11.1344491774741,-21.923557224952,0.));
#222741=CARTESIAN_POINT('Ctrl Pts',(11.1344491774741,-21.923557224952,12.));
#222742=CARTESIAN_POINT('Ctrl Pts',(11.1160102123024,-21.9082689538688,
0.));
#222743=CARTESIAN_POINT('Ctrl Pts',(11.1160102123024,-21.9082689538688,
12.));
#222744=CARTESIAN_POINT('Ctrl Pts',(11.0976757303944,-21.8929912313608,
0.));
#222745=CARTESIAN_POINT('Ctrl Pts',(11.0976757303944,-21.8929912313608,
12.));
#222746=CARTESIAN_POINT('Ctrl Pts',(11.0794459793057,-21.877724666119,0.));
#222747=CARTESIAN_POINT('Ctrl Pts',(11.0794459793057,-21.877724666119,12.));
#222748=CARTESIAN_POINT('Ctrl Pts',(11.0613212074363,-21.8624698726318,
0.));
#222749=CARTESIAN_POINT('Ctrl Pts',(11.0613212074363,-21.8624698726318,
12.));
#222750=CARTESIAN_POINT('Ctrl Pts',(11.0433016640807,-21.8472274713103,
0.));
#222751=CARTESIAN_POINT('Ctrl Pts',(11.0433016640807,-21.8472274713103,
12.));
#222752=CARTESIAN_POINT('Ctrl Pts',(11.0253875994598,-21.8319980886033,
0.));
#222753=CARTESIAN_POINT('Ctrl Pts',(11.0253875994598,-21.8319980886033,
12.));
#222754=CARTESIAN_POINT('Ctrl Pts',(11.0075792647477,-21.8167823571168,
0.));
#222755=CARTESIAN_POINT('Ctrl Pts',(11.0075792647477,-21.8167823571168,
12.));
#222756=CARTESIAN_POINT('Ctrl Pts',(10.9898769120912,-21.8015809157301,
0.));
#222757=CARTESIAN_POINT('Ctrl Pts',(10.9898769120912,-21.8015809157301,
12.));
#222758=CARTESIAN_POINT('Ctrl Pts',(10.9722807946155,-21.7863944097141,
0.));
#222759=CARTESIAN_POINT('Ctrl Pts',(10.9722807946155,-21.7863944097141,
12.));
#222760=CARTESIAN_POINT('Ctrl Pts',(10.9547911664455,-21.7712234908464,
0.));
#222761=CARTESIAN_POINT('Ctrl Pts',(10.9547911664455,-21.7712234908464,
12.));
#222762=CARTESIAN_POINT('Ctrl Pts',(10.9374082827444,-21.7560688175247,
0.));
#222763=CARTESIAN_POINT('Ctrl Pts',(10.9374082827444,-21.7560688175247,
12.));
#222764=CARTESIAN_POINT('Ctrl Pts',(10.9201323997384,-21.7409310548797,
0.));
#222765=CARTESIAN_POINT('Ctrl Pts',(10.9201323997384,-21.7409310548797,
12.));
#222766=CARTESIAN_POINT('Ctrl Pts',(10.902963774734,-21.7258108748873,0.));
#222767=CARTESIAN_POINT('Ctrl Pts',(10.902963774734,-21.7258108748873,12.));
#222768=CARTESIAN_POINT('Ctrl Pts',(10.8859026661293,-21.7107089564825,
0.));
#222769=CARTESIAN_POINT('Ctrl Pts',(10.8859026661293,-21.7107089564825,
12.));
#222770=CARTESIAN_POINT('Ctrl Pts',(10.8689493334095,-21.6956259856672,
0.));
#222771=CARTESIAN_POINT('Ctrl Pts',(10.8689493334095,-21.6956259856672,
12.));
#222772=CARTESIAN_POINT('Ctrl Pts',(10.8521040371835,-21.6805626556467,
0.));
#222773=CARTESIAN_POINT('Ctrl Pts',(10.8521040371835,-21.6805626556467,
12.));
#222774=CARTESIAN_POINT('Ctrl Pts',(10.8353670392272,-21.6655196669732,
0.));
#222775=CARTESIAN_POINT('Ctrl Pts',(10.8353670392272,-21.6655196669732,
12.));
#222776=CARTESIAN_POINT('Ctrl Pts',(10.8187386025136,-21.6504977276866,
0.));
#222777=CARTESIAN_POINT('Ctrl Pts',(10.8187386025136,-21.6504977276866,
12.));
#222778=CARTESIAN_POINT('Ctrl Pts',(10.8022189912369,-21.6354975534557,
0.));
#222779=CARTESIAN_POINT('Ctrl Pts',(10.8022189912369,-21.6354975534557,
12.));
#222780=CARTESIAN_POINT('Ctrl Pts',(10.7858084708261,-21.6205198677173,
0.));
#222781=CARTESIAN_POINT('Ctrl Pts',(10.7858084708261,-21.6205198677173,
12.));
#222782=CARTESIAN_POINT('Ctrl Pts',(10.7695073079552,-21.6055654018176,
0.));
#222783=CARTESIAN_POINT('Ctrl Pts',(10.7695073079552,-21.6055654018176,
12.));
#222784=CARTESIAN_POINT('Ctrl Pts',(10.7533157705941,-21.5906348951743,
0.));
#222785=CARTESIAN_POINT('Ctrl Pts',(10.7533157705941,-21.5906348951743,
12.));
#222786=CARTESIAN_POINT('Ctrl Pts',(10.7372341280467,-21.5757290954371,
0.));
#222787=CARTESIAN_POINT('Ctrl Pts',(10.7372341280467,-21.5757290954371,
12.));
#222788=CARTESIAN_POINT('Ctrl Pts',(10.7212626509816,-21.5608487586468,
0.));
#222789=CARTESIAN_POINT('Ctrl Pts',(10.7212626509816,-21.5608487586468,
12.));
#222790=CARTESIAN_POINT('Ctrl Pts',(10.7054016114571,-21.5459946493955,
0.));
#222791=CARTESIAN_POINT('Ctrl Pts',(10.7054016114571,-21.5459946493955,
12.));
#222792=CARTESIAN_POINT('Ctrl Pts',(10.689651282929,-21.5311675409807,0.));
#222793=CARTESIAN_POINT('Ctrl Pts',(10.689651282929,-21.5311675409807,12.));
#222794=CARTESIAN_POINT('Ctrl Pts',(10.6740119402834,-21.51636821558,0.));
#222795=CARTESIAN_POINT('Ctrl Pts',(10.6740119402834,-21.51636821558,12.));
#222796=CARTESIAN_POINT('Ctrl Pts',(10.6584838598939,-21.5015974644449,
0.));
#222797=CARTESIAN_POINT('Ctrl Pts',(10.6584838598939,-21.5015974644449,
12.));
#222798=CARTESIAN_POINT('Ctrl Pts',(10.6430673196607,-21.4868560880889,
0.));
#222799=CARTESIAN_POINT('Ctrl Pts',(10.6430673196607,-21.4868560880889,
12.));
#222800=CARTESIAN_POINT('Ctrl Pts',(10.6277625990456,-21.4721448964766,
0.));
#222801=CARTESIAN_POINT('Ctrl Pts',(10.6277625990456,-21.4721448964766,
12.));
#222802=CARTESIAN_POINT('Ctrl Pts',(10.6125699790961,-21.4574647092097,
0.));
#222803=CARTESIAN_POINT('Ctrl Pts',(10.6125699790961,-21.4574647092097,
12.));
#222804=CARTESIAN_POINT('Ctrl Pts',(10.5974897424622,-21.4428163557144,
0.));
#222805=CARTESIAN_POINT('Ctrl Pts',(10.5974897424622,-21.4428163557144,
12.));
#222806=CARTESIAN_POINT('Ctrl Pts',(10.5825221734573,-21.4282006754631,
0.));
#222807=CARTESIAN_POINT('Ctrl Pts',(10.5825221734573,-21.4282006754631,
12.));
#222808=CARTESIAN_POINT('Ctrl Pts',(10.5676675581108,-21.4136185181979,
0.));
#222809=CARTESIAN_POINT('Ctrl Pts',(10.5676675581108,-21.4136185181979,
12.));
#222810=CARTESIAN_POINT('Ctrl Pts',(10.5529261842108,-21.3990707441497,
0.));
#222811=CARTESIAN_POINT('Ctrl Pts',(10.5529261842108,-21.3990707441497,
12.));
#222812=CARTESIAN_POINT('Ctrl Pts',(10.5382983413421,-21.3845582242602,
0.));
#222813=CARTESIAN_POINT('Ctrl Pts',(10.5382983413421,-21.3845582242602,
12.));
#222814=CARTESIAN_POINT('Ctrl Pts',(10.5237843209057,-21.3700818403936,
0.));
#222815=CARTESIAN_POINT('Ctrl Pts',(10.5237843209057,-21.3700818403936,
12.));
#222816=CARTESIAN_POINT('Ctrl Pts',(10.5093844161685,-21.3556424855814,
0.));
#222817=CARTESIAN_POINT('Ctrl Pts',(10.5093844161685,-21.3556424855814,
12.));
#222818=CARTESIAN_POINT('Ctrl Pts',(10.4950989223336,-21.3412410642904,
0.));
#222819=CARTESIAN_POINT('Ctrl Pts',(10.4950989223336,-21.3412410642904,
12.));
#222820=CARTESIAN_POINT('Ctrl Pts',(10.4809281365931,-21.3268784926819,
0.));
#222821=CARTESIAN_POINT('Ctrl Pts',(10.4809281365931,-21.3268784926819,
12.));
#222822=CARTESIAN_POINT('Ctrl Pts',(10.4668723581768,-21.3125556988731,
0.));
#222823=CARTESIAN_POINT('Ctrl Pts',(10.4668723581768,-21.3125556988731,
12.));
#222824=CARTESIAN_POINT('Ctrl Pts',(10.4529318883874,-21.2982736231931,
0.));
#222825=CARTESIAN_POINT('Ctrl Pts',(10.4529318883874,-21.2982736231931,
12.));
#222826=CARTESIAN_POINT('Ctrl Pts',(10.4391070306391,-21.2840332184483,
0.));
#222827=CARTESIAN_POINT('Ctrl Pts',(10.4391070306391,-21.2840332184483,
12.));
#222828=CARTESIAN_POINT('Ctrl Pts',(10.42539809054,-21.2698354502403,0.));
#222829=CARTESIAN_POINT('Ctrl Pts',(10.42539809054,-21.2698354502403,12.));
#222830=CARTESIAN_POINT('Ctrl Pts',(10.4118053759588,-21.255681297275,0.));
#222831=CARTESIAN_POINT('Ctrl Pts',(10.4118053759588,-21.255681297275,12.));
#222832=CARTESIAN_POINT('Ctrl Pts',(10.3983291970846,-21.2415717516714,
0.));
#222833=CARTESIAN_POINT('Ctrl Pts',(10.3983291970846,-21.2415717516714,
12.));
#222834=CARTESIAN_POINT('Ctrl Pts',(10.3849698664786,-21.22750781927,0.));
#222835=CARTESIAN_POINT('Ctrl Pts',(10.3849698664786,-21.22750781927,12.));
#222836=CARTESIAN_POINT('Ctrl Pts',(10.371727699113,-21.2134905199345,0.));
#222837=CARTESIAN_POINT('Ctrl Pts',(10.371727699113,-21.2134905199345,12.));
#222838=CARTESIAN_POINT('Ctrl Pts',(10.3586030124587,-21.199520887919,0.));
#222839=CARTESIAN_POINT('Ctrl Pts',(10.3586030124587,-21.199520887919,12.));
#222840=CARTESIAN_POINT('Ctrl Pts',(10.34559612657,-21.1855999722416,0.));
#222841=CARTESIAN_POINT('Ctrl Pts',(10.34559612657,-21.1855999722416,12.));
#222842=CARTESIAN_POINT('Ctrl Pts',(10.3327073641572,-21.1717288370509,
0.));
#222843=CARTESIAN_POINT('Ctrl Pts',(10.3327073641572,-21.1717288370509,
12.));
#222844=CARTESIAN_POINT('Ctrl Pts',(10.3199370506544,-21.1579085619965,
0.));
#222845=CARTESIAN_POINT('Ctrl Pts',(10.3199370506544,-21.1579085619965,
12.));
#222846=CARTESIAN_POINT('Ctrl Pts',(10.3072855142687,-21.1441402425843,
0.));
#222847=CARTESIAN_POINT('Ctrl Pts',(10.3072855142687,-21.1441402425843,
12.));
#222848=CARTESIAN_POINT('Ctrl Pts',(10.2947530860721,-21.1304249906002,
0.));
#222849=CARTESIAN_POINT('Ctrl Pts',(10.2947530860721,-21.1304249906002,
12.));
#222850=CARTESIAN_POINT('Ctrl Pts',(10.2823401001072,-21.1167639345631,
0.));
#222851=CARTESIAN_POINT('Ctrl Pts',(10.2823401001072,-21.1167639345631,
12.));
#222852=CARTESIAN_POINT('Ctrl Pts',(10.2700468934744,-21.1031582201627,
0.));
#222853=CARTESIAN_POINT('Ctrl Pts',(10.2700468934744,-21.1031582201627,
12.));
#222854=CARTESIAN_POINT('Ctrl Pts',(10.2578738064181,-21.0896090107063,
0.));
#222855=CARTESIAN_POINT('Ctrl Pts',(10.2578738064181,-21.0896090107063,
12.));
#222856=CARTESIAN_POINT('Ctrl Pts',(10.2458211823912,-21.0761174875445,
0.));
#222857=CARTESIAN_POINT('Ctrl Pts',(10.2458211823912,-21.0761174875445,
12.));
#222858=CARTESIAN_POINT('Ctrl Pts',(10.2338893681567,-21.0626848505663,
0.));
#222859=CARTESIAN_POINT('Ctrl Pts',(10.2338893681567,-21.0626848505663,
12.));
#222860=CARTESIAN_POINT('Ctrl Pts',(10.2220787139154,-21.0493123187483,
0.));
#222861=CARTESIAN_POINT('Ctrl Pts',(10.2220787139154,-21.0493123187483,
12.));
#222862=CARTESIAN_POINT('Ctrl Pts',(10.2103895734123,-21.0360011306815,
0.));
#222863=CARTESIAN_POINT('Ctrl Pts',(10.2103895734123,-21.0360011306815,
12.));
#222864=CARTESIAN_POINT('Ctrl Pts',(10.1988223040425,-21.0227525451107,
0.));
#222865=CARTESIAN_POINT('Ctrl Pts',(10.1988223040425,-21.0227525451107,
12.));
#222866=CARTESIAN_POINT('Ctrl Pts',(10.187377266936,-21.0095678414486,0.));
#222867=CARTESIAN_POINT('Ctrl Pts',(10.187377266936,-21.0095678414486,12.));
#222868=CARTESIAN_POINT('Ctrl Pts',(10.1760548270767,-20.9964483203686,
0.));
#222869=CARTESIAN_POINT('Ctrl Pts',(10.1760548270767,-20.9964483203686,
12.));
#222870=CARTESIAN_POINT('Ctrl Pts',(10.1648553534568,-20.9833953044736,
0.));
#222871=CARTESIAN_POINT('Ctrl Pts',(10.1648553534568,-20.9833953044736,
12.));
#222872=CARTESIAN_POINT('Ctrl Pts',(10.1537792192065,-20.9704101389369,
0.));
#222873=CARTESIAN_POINT('Ctrl Pts',(10.1537792192065,-20.9704101389369,
12.));
#222874=CARTESIAN_POINT('Ctrl Pts',(10.1428268017256,-20.9574941921591,
0.));
#222875=CARTESIAN_POINT('Ctrl Pts',(10.1428268017256,-20.9574941921591,
12.));
#222876=CARTESIAN_POINT('Ctrl Pts',(10.1319984827908,-20.9446488563933,
0.));
#222877=CARTESIAN_POINT('Ctrl Pts',(10.1319984827908,-20.9446488563933,
12.));
#222878=CARTESIAN_POINT('Ctrl Pts',(10.1212946487057,-20.9318755484734,
0.));
#222879=CARTESIAN_POINT('Ctrl Pts',(10.1212946487057,-20.9318755484734,
12.));
#222880=CARTESIAN_POINT('Ctrl Pts',(10.1107156904836,-20.919175710627,0.));
#222881=CARTESIAN_POINT('Ctrl Pts',(10.1107156904836,-20.919175710627,12.));
#222882=CARTESIAN_POINT('Ctrl Pts',(10.1002620040076,-20.9065508112557,
0.));
#222883=CARTESIAN_POINT('Ctrl Pts',(10.1002620040076,-20.9065508112557,
12.));
#222884=CARTESIAN_POINT('Ctrl Pts',(10.0899339901915,-20.894002345737,0.));
#222885=CARTESIAN_POINT('Ctrl Pts',(10.0899339901915,-20.894002345737,12.));
#222886=CARTESIAN_POINT('Ctrl Pts',(10.0797320551154,-20.881531837184,0.));
#222887=CARTESIAN_POINT('Ctrl Pts',(10.0797320551154,-20.881531837184,12.));
#222888=CARTESIAN_POINT('Ctrl Pts',(10.0696566102218,-20.86914083737,0.));
#222889=CARTESIAN_POINT('Ctrl Pts',(10.0696566102218,-20.86914083737,12.));
#222890=CARTESIAN_POINT('Ctrl Pts',(10.0597080725375,-20.8568309277316,
0.));
#222891=CARTESIAN_POINT('Ctrl Pts',(10.0597080725375,-20.8568309277316,
12.));
#222892=CARTESIAN_POINT('Ctrl Pts',(10.0498868648733,-20.8446037203402,
0.));
#222893=CARTESIAN_POINT('Ctrl Pts',(10.0498868648733,-20.8446037203402,
12.));
#222894=CARTESIAN_POINT('Ctrl Pts',(10.0401934160234,-20.8324608588909,
0.));
#222895=CARTESIAN_POINT('Ctrl Pts',(10.0401934160234,-20.8324608588909,
12.));
#222896=CARTESIAN_POINT('Ctrl Pts',(10.0306281609435,-20.8204040196602,
0.));
#222897=CARTESIAN_POINT('Ctrl Pts',(10.0306281609435,-20.8204040196602,
12.));
#222898=CARTESIAN_POINT('Ctrl Pts',(10.0211915410095,-20.8084349126888,
0.));
#222899=CARTESIAN_POINT('Ctrl Pts',(10.0211915410095,-20.8084349126888,
12.));
#222900=CARTESIAN_POINT('Ctrl Pts',(10.0118840042786,-20.7965552829908,
0.));
#222901=CARTESIAN_POINT('Ctrl Pts',(10.0118840042786,-20.7965552829908,
12.));
#222902=CARTESIAN_POINT('Ctrl Pts',(10.0027060057389,-20.7847669117568,
0.));
#222903=CARTESIAN_POINT('Ctrl Pts',(10.0027060057389,-20.7847669117568,
12.));
#222904=CARTESIAN_POINT('Ctrl Pts',(9.9936580075464,-20.7730716175417,0.));
#222905=CARTESIAN_POINT('Ctrl Pts',(9.9936580075464,-20.7730716175417,12.));
#222906=CARTESIAN_POINT('Ctrl Pts',(9.98474047926852,-20.761471257499,0.));
#222907=CARTESIAN_POINT('Ctrl Pts',(9.98474047926852,-20.761471257499,12.));
#222908=CARTESIAN_POINT('Ctrl Pts',(9.97595389823469,-20.7499677289627,
0.));
#222909=CARTESIAN_POINT('Ctrl Pts',(9.97595389823469,-20.7499677289627,
12.));
#222910=CARTESIAN_POINT('Ctrl Pts',(9.96729874986201,-20.7385629709795,
0.));
#222911=CARTESIAN_POINT('Ctrl Pts',(9.96729874986201,-20.7385629709795,
12.));
#222912=CARTESIAN_POINT('Ctrl Pts',(9.95877552798397,-20.7272589658751,
0.));
#222913=CARTESIAN_POINT('Ctrl Pts',(9.95877552798397,-20.7272589658751,
12.));
#222914=CARTESIAN_POINT('Ctrl Pts',(9.95038473514948,-20.7160577407579,
0.));
#222915=CARTESIAN_POINT('Ctrl Pts',(9.95038473514948,-20.7160577407579,
12.));
#222916=CARTESIAN_POINT('Ctrl Pts',(9.94212688298236,-20.7049613692234,
0.));
#222917=CARTESIAN_POINT('Ctrl Pts',(9.94212688298236,-20.7049613692234,
12.));
#222918=CARTESIAN_POINT('Ctrl Pts',(9.93400249259729,-20.6939719732484,
0.));
#222919=CARTESIAN_POINT('Ctrl Pts',(9.93400249259729,-20.6939719732484,
12.));
#222920=CARTESIAN_POINT('Ctrl Pts',(9.92601209498748,-20.6830917250255,
0.));
#222921=CARTESIAN_POINT('Ctrl Pts',(9.92601209498748,-20.6830917250255,
12.));
#222922=CARTESIAN_POINT('Ctrl Pts',(9.91815623141288,-20.6723228488263,
0.));
#222923=CARTESIAN_POINT('Ctrl Pts',(9.91815623141288,-20.6723228488263,
12.));
#222924=CARTESIAN_POINT('Ctrl Pts',(9.91043545377007,-20.6616676228315,
0.));
#222925=CARTESIAN_POINT('Ctrl Pts',(9.91043545377007,-20.6616676228315,
12.));
#222926=CARTESIAN_POINT('Ctrl Pts',(9.90285032516692,-20.6511283817414,
0.));
#222927=CARTESIAN_POINT('Ctrl Pts',(9.90285032516692,-20.6511283817414,
12.));
#222928=CARTESIAN_POINT('Ctrl Pts',(9.89540142049119,-20.6407075193976,
0.));
#222929=CARTESIAN_POINT('Ctrl Pts',(9.89540142049119,-20.6407075193976,
12.));
#222930=CARTESIAN_POINT('Ctrl Pts',(9.88808932697305,-20.6304074914087,
0.));
#222931=CARTESIAN_POINT('Ctrl Pts',(9.88808932697305,-20.6304074914087,
12.));
#222932=CARTESIAN_POINT('Ctrl Pts',(9.88091464472675,-20.6202308177475,
0.));
#222933=CARTESIAN_POINT('Ctrl Pts',(9.88091464472675,-20.6202308177475,
12.));
#222934=CARTESIAN_POINT('Ctrl Pts',(9.87387798732955,-20.6101800854494,
0.));
#222935=CARTESIAN_POINT('Ctrl Pts',(9.87387798732955,-20.6101800854494,
12.));
#222936=CARTESIAN_POINT('Ctrl Pts',(9.86697998242622,-20.6002579513699,
0.));
#222937=CARTESIAN_POINT('Ctrl Pts',(9.86697998242622,-20.6002579513699,
12.));
#222938=CARTESIAN_POINT('Ctrl Pts',(9.86022127232747,-20.5904671449754,
0.));
#222939=CARTESIAN_POINT('Ctrl Pts',(9.86022127232747,-20.5904671449754,
12.));
#222940=CARTESIAN_POINT('Ctrl Pts',(9.8536025145698,-20.5808104710015,0.));
#222941=CARTESIAN_POINT('Ctrl Pts',(9.8536025145698,-20.5808104710015,12.));
#222942=CARTESIAN_POINT('Ctrl Pts',(9.84712438256277,-20.5712908125139,
0.));
#222943=CARTESIAN_POINT('Ctrl Pts',(9.84712438256277,-20.5712908125139,
12.));
#222944=CARTESIAN_POINT('Ctrl Pts',(9.84078756677565,-20.5619111362402,
0.));
#222945=CARTESIAN_POINT('Ctrl Pts',(9.84078756677565,-20.5619111362402,
12.));
#222946=CARTESIAN_POINT('Ctrl Pts',(9.83459277585315,-20.552674497646,0.));
#222947=CARTESIAN_POINT('Ctrl Pts',(9.83459277585315,-20.552674497646,12.));
#222948=CARTESIAN_POINT('Ctrl Pts',(9.82854073773876,-20.5435840460721,
0.));
#222949=CARTESIAN_POINT('Ctrl Pts',(9.82854073773876,-20.5435840460721,
12.));
#222950=CARTESIAN_POINT('Ctrl Pts',(9.82263220080362,-20.5346430299517,
0.));
#222951=CARTESIAN_POINT('Ctrl Pts',(9.82263220080362,-20.5346430299517,
12.));
#222952=CARTESIAN_POINT('Ctrl Pts',(9.81686793455942,-20.5258548000629,
0.));
#222953=CARTESIAN_POINT('Ctrl Pts',(9.81686793455942,-20.5258548000629,
12.));
#222954=CARTESIAN_POINT('Ctrl Pts',(9.81124873025281,-20.517222812284,0.));
#222955=CARTESIAN_POINT('Ctrl Pts',(9.81124873025281,-20.517222812284,12.));
#222956=CARTESIAN_POINT('Ctrl Pts',(9.80577540161087,-20.5087506310505,
0.));
#222957=CARTESIAN_POINT('Ctrl Pts',(9.80577540161087,-20.5087506310505,
12.));
#222958=CARTESIAN_POINT('Ctrl Pts',(9.80044878520948,-20.5004419312107,
0.));
#222959=CARTESIAN_POINT('Ctrl Pts',(9.80044878520948,-20.5004419312107,
12.));
#222960=CARTESIAN_POINT('Ctrl Pts',(9.7952697428833,-20.4923005087943,0.));
#222961=CARTESIAN_POINT('Ctrl Pts',(9.7952697428833,-20.4923005087943,12.));
#222962=CARTESIAN_POINT('Ctrl Pts',(9.79023916498655,-20.4843302955329,
0.));
#222963=CARTESIAN_POINT('Ctrl Pts',(9.79023916498655,-20.4843302955329,
12.));
#222964=CARTESIAN_POINT('Ctrl Pts',(9.78535797314166,-20.4765353711586,
0.));
#222965=CARTESIAN_POINT('Ctrl Pts',(9.78535797314166,-20.4765353711586,
12.));
#222966=CARTESIAN_POINT('Ctrl Pts',(9.7806271237332,-20.4689199790669,0.));
#222967=CARTESIAN_POINT('Ctrl Pts',(9.7806271237332,-20.4689199790669,12.));
#222968=CARTESIAN_POINT('Ctrl Pts',(9.77604760815528,-20.4614885274975,
0.));
#222969=CARTESIAN_POINT('Ctrl Pts',(9.77604760815528,-20.4614885274975,
12.));
#222970=CARTESIAN_POINT('Ctrl Pts',(9.77162045104069,-20.4542455817527,
0.));
#222971=CARTESIAN_POINT('Ctrl Pts',(9.77162045104069,-20.4542455817527,
12.));
#222972=CARTESIAN_POINT('Ctrl Pts',(9.76734670980891,-20.447195862298,0.));
#222973=CARTESIAN_POINT('Ctrl Pts',(9.76734670980891,-20.447195862298,12.));
#222974=CARTESIAN_POINT('Ctrl Pts',(9.76322747195494,-20.44034423294,0.));
#222975=CARTESIAN_POINT('Ctrl Pts',(9.76322747195494,-20.44034423294,12.));
#222976=CARTESIAN_POINT('Ctrl Pts',(9.75926386289922,-20.4336957355473,
0.));
#222977=CARTESIAN_POINT('Ctrl Pts',(9.75926386289922,-20.4336957355473,
12.));
#222978=CARTESIAN_POINT('Ctrl Pts',(9.75545705902417,-20.4272556476629,
0.));
#222979=CARTESIAN_POINT('Ctrl Pts',(9.75545705902417,-20.4272556476629,
12.));
#222980=CARTESIAN_POINT('Ctrl Pts',(9.75180829786429,-20.4210295275817,
0.));
#222981=CARTESIAN_POINT('Ctrl Pts',(9.75180829786429,-20.4210295275817,
12.));
#222982=CARTESIAN_POINT('Ctrl Pts',(9.74831889242173,-20.4150232777393,
0.));
#222983=CARTESIAN_POINT('Ctrl Pts',(9.74831889242173,-20.4150232777393,
12.));
#222984=CARTESIAN_POINT('Ctrl Pts',(9.74499021838537,-20.4092430879861,
0.));
#222985=CARTESIAN_POINT('Ctrl Pts',(9.74499021838537,-20.4092430879861,
12.));
#222986=CARTESIAN_POINT('Ctrl Pts',(9.74182369656271,-20.4036953576549,
0.));
#222987=CARTESIAN_POINT('Ctrl Pts',(9.74182369656271,-20.4036953576549,
12.));
#222988=CARTESIAN_POINT('Ctrl Pts',(9.738820776132,-20.3983866213331,0.));
#222989=CARTESIAN_POINT('Ctrl Pts',(9.738820776132,-20.3983866213331,12.));
#222990=CARTESIAN_POINT('Ctrl Pts',(9.73598292014242,-20.3933234845647,
0.));
#222991=CARTESIAN_POINT('Ctrl Pts',(9.73598292014242,-20.3933234845647,
12.));
#222992=CARTESIAN_POINT('Ctrl Pts',(9.73331167102807,-20.3885129129912,
0.));
#222993=CARTESIAN_POINT('Ctrl Pts',(9.73331167102807,-20.3885129129912,
12.));
#222994=CARTESIAN_POINT('Ctrl Pts',(9.73080870123726,-20.3839624556742,
0.));
#222995=CARTESIAN_POINT('Ctrl Pts',(9.73080870123726,-20.3839624556742,
12.));
#222996=CARTESIAN_POINT('Ctrl Pts',(9.72847589116541,-20.3796805893304,
0.));
#222997=CARTESIAN_POINT('Ctrl Pts',(9.72847589116541,-20.3796805893304,
12.));
#222998=CARTESIAN_POINT('Ctrl Pts',(9.7263153173288,-20.3756766651951,0.));
#222999=CARTESIAN_POINT('Ctrl Pts',(9.7263153173288,-20.3756766651951,12.));
#223000=CARTESIAN_POINT('Ctrl Pts',(9.72432910043194,-20.371960235676,0.));
#223001=CARTESIAN_POINT('Ctrl Pts',(9.72432910043194,-20.371960235676,12.));
#223002=CARTESIAN_POINT('Ctrl Pts',(9.72251930722489,-20.3685406190576,
0.));
#223003=CARTESIAN_POINT('Ctrl Pts',(9.72251930722489,-20.3685406190576,
12.));
#223004=CARTESIAN_POINT('Ctrl Pts',(9.7208877838108,-20.3654261611056,0.));
#223005=CARTESIAN_POINT('Ctrl Pts',(9.7208877838108,-20.3654261611056,12.));
#223006=CARTESIAN_POINT('Ctrl Pts',(9.71943648548099,-20.3626256913981,
0.));
#223007=CARTESIAN_POINT('Ctrl Pts',(9.71943648548099,-20.3626256913981,
12.));
#223008=CARTESIAN_POINT('Ctrl Pts',(9.71816778328006,-20.3601498764344,
0.));
#223009=CARTESIAN_POINT('Ctrl Pts',(9.71816778328006,-20.3601498764344,
12.));
#223010=CARTESIAN_POINT('Ctrl Pts',(9.71708493723096,-20.3580133103356,
0.));
#223011=CARTESIAN_POINT('Ctrl Pts',(9.71708493723096,-20.3580133103356,
12.));
#223012=CARTESIAN_POINT('Ctrl Pts',(9.71619192554185,-20.3562337557875,
0.));
#223013=CARTESIAN_POINT('Ctrl Pts',(9.71619192554185,-20.3562337557875,
12.));
#223014=CARTESIAN_POINT('Ctrl Pts',(9.71549257088172,-20.3548282742361,
0.));
#223015=CARTESIAN_POINT('Ctrl Pts',(9.71549257088172,-20.3548282742361,
12.));
#223016=CARTESIAN_POINT('Ctrl Pts',(9.7149897805202,-20.3538098605706,0.));
#223017=CARTESIAN_POINT('Ctrl Pts',(9.7149897805202,-20.3538098605706,12.));
#223018=CARTESIAN_POINT('Ctrl Pts',(9.7147459035068,-20.3533097561886,0.));
#223019=CARTESIAN_POINT('Ctrl Pts',(9.7147459035068,-20.3533097561886,12.));
#223020=CARTESIAN_POINT('Ctrl Pts',(9.71465227853041,-20.3531126095522,
0.));
#223021=CARTESIAN_POINT('Ctrl Pts',(9.71465227853041,-20.3531126095522,
12.));
#223022=CARTESIAN_POINT('Ctrl Pts',(9.71462954053041,-20.353060251684,0.));
#223023=CARTESIAN_POINT('Ctrl Pts',(9.71462954053041,-20.353060251684,12.));
#223024=CARTESIAN_POINT('Ctrl Pts',(9.71462809124915,-20.353053841303,0.));
#223025=CARTESIAN_POINT('Ctrl Pts',(9.71462809124915,-20.353053841303,12.));
#223026=CARTESIAN_POINT('',(12.4230808101438,-22.8400320311649,0.));
#223027=CARTESIAN_POINT('Ctrl Pts',(12.4230808101438,-22.8400320311649,
0.));
#223028=CARTESIAN_POINT('Ctrl Pts',(12.418215285186,-22.8370364396459,0.));
#223029=CARTESIAN_POINT('Ctrl Pts',(12.4084933766346,-22.8310435872748,
0.));
#223030=CARTESIAN_POINT('Ctrl Pts',(12.3939379378998,-22.8220493007173,
0.));
#223031=CARTESIAN_POINT('Ctrl Pts',(12.374585536673,-22.81004690224,0.));
#223032=CARTESIAN_POINT('Ctrl Pts',(12.3504864740319,-22.795027221673,0.));
#223033=CARTESIAN_POINT('Ctrl Pts',(12.3264788926075,-22.7799908974768,
0.));
#223034=CARTESIAN_POINT('Ctrl Pts',(12.3025628601792,-22.764938010105,0.));
#223035=CARTESIAN_POINT('Ctrl Pts',(12.2787384750742,-22.7498686970069,
0.));
#223036=CARTESIAN_POINT('Ctrl Pts',(12.2550058702395,-22.7347831655287,
0.));
#223037=CARTESIAN_POINT('Ctrl Pts',(12.2313652198061,-22.7196817119374,
0.));
#223038=CARTESIAN_POINT('Ctrl Pts',(12.2078167360284,-22.7045647168747,
0.));
#223039=CARTESIAN_POINT('Ctrl Pts',(12.1843606579261,-22.6894326205037,
0.));
#223040=CARTESIAN_POINT('Ctrl Pts',(12.1609972423099,-22.6742859034944,
0.));
#223041=CARTESIAN_POINT('Ctrl Pts',(12.1377267537145,-22.6591250653965,
0.));
#223042=CARTESIAN_POINT('Ctrl Pts',(12.1145494550383,-22.6439506046605,
0.));
#223043=CARTESIAN_POINT('Ctrl Pts',(12.0914655972823,-22.6287629967056,
0.));
#223044=CARTESIAN_POINT('Ctrl Pts',(12.0684754113862,-22.6135626764898,
0.));
#223045=CARTESIAN_POINT('Ctrl Pts',(12.0455791139128,-22.5983500505644,
0.));
#223046=CARTESIAN_POINT('Ctrl Pts',(12.0227769113127,-22.5831255061282,
0.));
#223047=CARTESIAN_POINT('Ctrl Pts',(12.0000690046694,-22.5678894211181,
0.));
#223048=CARTESIAN_POINT('Ctrl Pts',(11.9774555943496,-22.5526421741158,
0.));
#223049=CARTESIAN_POINT('Ctrl Pts',(11.9549368843997,-22.5373841537307,
0.));
#223050=CARTESIAN_POINT('Ctrl Pts',(11.9325130877803,-22.5221157697883,
0.));
#223051=CARTESIAN_POINT('Ctrl Pts',(11.9101844254557,-22.5068374513973,
0.));
#223052=CARTESIAN_POINT('Ctrl Pts',(11.8879511239942,-22.4915496418485,
0.));
#223053=CARTESIAN_POINT('Ctrl Pts',(11.8658134137019,-22.4762527946702,
0.));
#223054=CARTESIAN_POINT('Ctrl Pts',(11.8437715264487,-22.4609473690472,
0.));
#223055=CARTESIAN_POINT('Ctrl Pts',(11.8218256937889,-22.4456338258735,
0.));
#223056=CARTESIAN_POINT('Ctrl Pts',(11.7999761445173,-22.430312622646,0.));
#223057=CARTESIAN_POINT('Ctrl Pts',(11.7782231042039,-22.4149842125008,
0.));
#223058=CARTESIAN_POINT('Ctrl Pts',(11.7565667964764,-22.3996490469191,
0.));
#223059=CARTESIAN_POINT('Ctrl Pts',(11.7350074437961,-22.3843075773899,
0.));
#223060=CARTESIAN_POINT('Ctrl Pts',(11.7135452684532,-22.3689602575491,
0.));
#223061=CARTESIAN_POINT('Ctrl Pts',(11.6921804934056,-22.3536075450029,
0.));
#223062=CARTESIAN_POINT('Ctrl Pts',(11.6709133432985,-22.3382499035619,
0.));
#223063=CARTESIAN_POINT('Ctrl Pts',(11.6497440449857,-22.3228878043976,
0.));
#223064=CARTESIAN_POINT('Ctrl Pts',(11.6286728270009,-22.3075217249049,
0.));
#223065=CARTESIAN_POINT('Ctrl Pts',(11.6076999192357,-22.2921521480356,
0.));
#223066=CARTESIAN_POINT('Ctrl Pts',(11.5868255525188,-22.2767795614348,
0.));
#223067=CARTESIAN_POINT('Ctrl Pts',(11.5660499582403,-22.2614044566898,
0.));
#223068=CARTESIAN_POINT('Ctrl Pts',(11.5453733679121,-22.2460273284654,
0.));
#223069=CARTESIAN_POINT('Ctrl Pts',(11.5247960128477,-22.2306486738901,
0.));
#223070=CARTESIAN_POINT('Ctrl Pts',(11.5043181244242,-22.2152689931022,
0.));
#223071=CARTESIAN_POINT('Ctrl Pts',(11.483939934259,-22.1998887896436,0.));
#223072=CARTESIAN_POINT('Ctrl Pts',(11.463661674411,-22.184508570917,0.));
#223073=CARTESIAN_POINT('Ctrl Pts',(11.443483577557,-22.1691288486096,0.));
#223074=CARTESIAN_POINT('Ctrl Pts',(11.4234058771742,-22.1537501391487,
0.));
#223075=CARTESIAN_POINT('Ctrl Pts',(11.4034288076908,-22.1383729640964,
0.));
#223076=CARTESIAN_POINT('Ctrl Pts',(11.3835526044256,-22.1229978500186,
0.));
#223077=CARTESIAN_POINT('Ctrl Pts',(11.3637775035367,-22.1076253283979,
0.));
#223078=CARTESIAN_POINT('Ctrl Pts',(11.3441037419553,-22.0922559355294,
0.));
#223079=CARTESIAN_POINT('Ctrl Pts',(11.3245315573168,-22.0768902124267,
0.));
#223080=CARTESIAN_POINT('Ctrl Pts',(11.3050611878771,-22.0615287047179,
0.));
#223081=CARTESIAN_POINT('Ctrl Pts',(11.2856928724374,-22.046171962566,0.));
#223082=CARTESIAN_POINT('Ctrl Pts',(11.2664268504206,-22.030820540835,0.));
#223083=CARTESIAN_POINT('Ctrl Pts',(11.2472633619275,-22.0154749992363,
0.));
#223084=CARTESIAN_POINT('Ctrl Pts',(11.2282026477896,-22.0001359024839,
0.));
#223085=CARTESIAN_POINT('Ctrl Pts',(11.2092449496125,-21.9848038204439,
0.));
#223086=CARTESIAN_POINT('Ctrl Pts',(11.190390509811,-21.9694793282914,0.));
#223087=CARTESIAN_POINT('Ctrl Pts',(11.1716395716376,-21.9541630066506,
0.));
#223088=CARTESIAN_POINT('Ctrl Pts',(11.1529923792003,-21.9388554416439,
0.));
#223089=CARTESIAN_POINT('Ctrl Pts',(11.1344491774741,-21.923557224952,0.));
#223090=CARTESIAN_POINT('Ctrl Pts',(11.1160102123024,-21.9082689538688,
0.));
#223091=CARTESIAN_POINT('Ctrl Pts',(11.0976757303944,-21.8929912313608,
0.));
#223092=CARTESIAN_POINT('Ctrl Pts',(11.0794459793057,-21.877724666119,0.));
#223093=CARTESIAN_POINT('Ctrl Pts',(11.0613212074363,-21.8624698726318,
0.));
#223094=CARTESIAN_POINT('Ctrl Pts',(11.0433016640807,-21.8472274713103,
0.));
#223095=CARTESIAN_POINT('Ctrl Pts',(11.0253875994598,-21.8319980886033,
0.));
#223096=CARTESIAN_POINT('Ctrl Pts',(11.0075792647477,-21.8167823571168,
0.));
#223097=CARTESIAN_POINT('Ctrl Pts',(10.9898769120912,-21.8015809157301,
0.));
#223098=CARTESIAN_POINT('Ctrl Pts',(10.9722807946155,-21.7863944097141,
0.));
#223099=CARTESIAN_POINT('Ctrl Pts',(10.9547911664455,-21.7712234908464,
0.));
#223100=CARTESIAN_POINT('Ctrl Pts',(10.9374082827444,-21.7560688175247,
0.));
#223101=CARTESIAN_POINT('Ctrl Pts',(10.9201323997384,-21.7409310548797,
0.));
#223102=CARTESIAN_POINT('Ctrl Pts',(10.902963774734,-21.7258108748873,0.));
#223103=CARTESIAN_POINT('Ctrl Pts',(10.8859026661293,-21.7107089564825,
0.));
#223104=CARTESIAN_POINT('Ctrl Pts',(10.8689493334095,-21.6956259856672,
0.));
#223105=CARTESIAN_POINT('Ctrl Pts',(10.8521040371835,-21.6805626556467,
0.));
#223106=CARTESIAN_POINT('Ctrl Pts',(10.8353670392272,-21.6655196669732,
0.));
#223107=CARTESIAN_POINT('Ctrl Pts',(10.8187386025136,-21.6504977276866,
0.));
#223108=CARTESIAN_POINT('Ctrl Pts',(10.8022189912369,-21.6354975534557,
0.));
#223109=CARTESIAN_POINT('Ctrl Pts',(10.7858084708261,-21.6205198677173,
0.));
#223110=CARTESIAN_POINT('Ctrl Pts',(10.7695073079552,-21.6055654018176,
0.));
#223111=CARTESIAN_POINT('Ctrl Pts',(10.7533157705941,-21.5906348951743,
0.));
#223112=CARTESIAN_POINT('Ctrl Pts',(10.7372341280467,-21.5757290954371,
0.));
#223113=CARTESIAN_POINT('Ctrl Pts',(10.7212626509816,-21.5608487586468,
0.));
#223114=CARTESIAN_POINT('Ctrl Pts',(10.7054016114571,-21.5459946493955,
0.));
#223115=CARTESIAN_POINT('Ctrl Pts',(10.689651282929,-21.5311675409807,0.));
#223116=CARTESIAN_POINT('Ctrl Pts',(10.6740119402834,-21.51636821558,0.));
#223117=CARTESIAN_POINT('Ctrl Pts',(10.6584838598939,-21.5015974644449,
0.));
#223118=CARTESIAN_POINT('Ctrl Pts',(10.6430673196607,-21.4868560880889,
0.));
#223119=CARTESIAN_POINT('Ctrl Pts',(10.6277625990456,-21.4721448964766,
0.));
#223120=CARTESIAN_POINT('Ctrl Pts',(10.6125699790961,-21.4574647092097,
0.));
#223121=CARTESIAN_POINT('Ctrl Pts',(10.5974897424622,-21.4428163557144,
0.));
#223122=CARTESIAN_POINT('Ctrl Pts',(10.5825221734573,-21.4282006754631,
0.));
#223123=CARTESIAN_POINT('Ctrl Pts',(10.5676675581108,-21.4136185181979,
0.));
#223124=CARTESIAN_POINT('Ctrl Pts',(10.5529261842108,-21.3990707441497,
0.));
#223125=CARTESIAN_POINT('Ctrl Pts',(10.5382983413421,-21.3845582242602,
0.));
#223126=CARTESIAN_POINT('Ctrl Pts',(10.5237843209057,-21.3700818403936,
0.));
#223127=CARTESIAN_POINT('Ctrl Pts',(10.5093844161685,-21.3556424855814,
0.));
#223128=CARTESIAN_POINT('Ctrl Pts',(10.4950989223336,-21.3412410642904,
0.));
#223129=CARTESIAN_POINT('Ctrl Pts',(10.4809281365931,-21.3268784926819,
0.));
#223130=CARTESIAN_POINT('Ctrl Pts',(10.4668723581768,-21.3125556988731,
0.));
#223131=CARTESIAN_POINT('Ctrl Pts',(10.4529318883874,-21.2982736231931,
0.));
#223132=CARTESIAN_POINT('Ctrl Pts',(10.4391070306391,-21.2840332184483,
0.));
#223133=CARTESIAN_POINT('Ctrl Pts',(10.42539809054,-21.2698354502403,0.));
#223134=CARTESIAN_POINT('Ctrl Pts',(10.4118053759588,-21.255681297275,0.));
#223135=CARTESIAN_POINT('Ctrl Pts',(10.3983291970846,-21.2415717516714,
0.));
#223136=CARTESIAN_POINT('Ctrl Pts',(10.3849698664786,-21.22750781927,0.));
#223137=CARTESIAN_POINT('Ctrl Pts',(10.371727699113,-21.2134905199345,0.));
#223138=CARTESIAN_POINT('Ctrl Pts',(10.3586030124587,-21.199520887919,0.));
#223139=CARTESIAN_POINT('Ctrl Pts',(10.34559612657,-21.1855999722416,0.));
#223140=CARTESIAN_POINT('Ctrl Pts',(10.3327073641572,-21.1717288370509,
0.));
#223141=CARTESIAN_POINT('Ctrl Pts',(10.3199370506544,-21.1579085619965,
0.));
#223142=CARTESIAN_POINT('Ctrl Pts',(10.3072855142687,-21.1441402425843,
0.));
#223143=CARTESIAN_POINT('Ctrl Pts',(10.2947530860721,-21.1304249906002,
0.));
#223144=CARTESIAN_POINT('Ctrl Pts',(10.2823401001072,-21.1167639345631,
0.));
#223145=CARTESIAN_POINT('Ctrl Pts',(10.2700468934744,-21.1031582201627,
0.));
#223146=CARTESIAN_POINT('Ctrl Pts',(10.2578738064181,-21.0896090107063,
0.));
#223147=CARTESIAN_POINT('Ctrl Pts',(10.2458211823912,-21.0761174875445,
0.));
#223148=CARTESIAN_POINT('Ctrl Pts',(10.2338893681567,-21.0626848505663,
0.));
#223149=CARTESIAN_POINT('Ctrl Pts',(10.2220787139154,-21.0493123187483,
0.));
#223150=CARTESIAN_POINT('Ctrl Pts',(10.2103895734123,-21.0360011306815,
0.));
#223151=CARTESIAN_POINT('Ctrl Pts',(10.1988223040425,-21.0227525451107,
0.));
#223152=CARTESIAN_POINT('Ctrl Pts',(10.187377266936,-21.0095678414486,0.));
#223153=CARTESIAN_POINT('Ctrl Pts',(10.1760548270767,-20.9964483203686,
0.));
#223154=CARTESIAN_POINT('Ctrl Pts',(10.1648553534568,-20.9833953044736,
0.));
#223155=CARTESIAN_POINT('Ctrl Pts',(10.1537792192065,-20.9704101389369,
0.));
#223156=CARTESIAN_POINT('Ctrl Pts',(10.1428268017256,-20.9574941921591,
0.));
#223157=CARTESIAN_POINT('Ctrl Pts',(10.1319984827908,-20.9446488563933,
0.));
#223158=CARTESIAN_POINT('Ctrl Pts',(10.1212946487057,-20.9318755484734,
0.));
#223159=CARTESIAN_POINT('Ctrl Pts',(10.1107156904836,-20.919175710627,0.));
#223160=CARTESIAN_POINT('Ctrl Pts',(10.1002620040076,-20.9065508112557,
0.));
#223161=CARTESIAN_POINT('Ctrl Pts',(10.0899339901915,-20.894002345737,0.));
#223162=CARTESIAN_POINT('Ctrl Pts',(10.0797320551154,-20.881531837184,0.));
#223163=CARTESIAN_POINT('Ctrl Pts',(10.0696566102218,-20.86914083737,0.));
#223164=CARTESIAN_POINT('Ctrl Pts',(10.0597080725375,-20.8568309277316,
0.));
#223165=CARTESIAN_POINT('Ctrl Pts',(10.0498868648733,-20.8446037203402,
0.));
#223166=CARTESIAN_POINT('Ctrl Pts',(10.0401934160234,-20.8324608588909,
0.));
#223167=CARTESIAN_POINT('Ctrl Pts',(10.0306281609435,-20.8204040196602,
0.));
#223168=CARTESIAN_POINT('Ctrl Pts',(10.0211915410095,-20.8084349126888,
0.));
#223169=CARTESIAN_POINT('Ctrl Pts',(10.0118840042786,-20.7965552829908,
0.));
#223170=CARTESIAN_POINT('Ctrl Pts',(10.0027060057389,-20.7847669117568,
0.));
#223171=CARTESIAN_POINT('Ctrl Pts',(9.9936580075464,-20.7730716175417,0.));
#223172=CARTESIAN_POINT('Ctrl Pts',(9.98474047926852,-20.761471257499,0.));
#223173=CARTESIAN_POINT('Ctrl Pts',(9.97595389823469,-20.7499677289627,
0.));
#223174=CARTESIAN_POINT('Ctrl Pts',(9.96729874986201,-20.7385629709795,
0.));
#223175=CARTESIAN_POINT('Ctrl Pts',(9.95877552798397,-20.7272589658751,
0.));
#223176=CARTESIAN_POINT('Ctrl Pts',(9.95038473514948,-20.7160577407579,
0.));
#223177=CARTESIAN_POINT('Ctrl Pts',(9.94212688298236,-20.7049613692234,
0.));
#223178=CARTESIAN_POINT('Ctrl Pts',(9.93400249259729,-20.6939719732484,
0.));
#223179=CARTESIAN_POINT('Ctrl Pts',(9.92601209498748,-20.6830917250255,
0.));
#223180=CARTESIAN_POINT('Ctrl Pts',(9.91815623141288,-20.6723228488263,
0.));
#223181=CARTESIAN_POINT('Ctrl Pts',(9.91043545377007,-20.6616676228315,
0.));
#223182=CARTESIAN_POINT('Ctrl Pts',(9.90285032516692,-20.6511283817414,
0.));
#223183=CARTESIAN_POINT('Ctrl Pts',(9.89540142049119,-20.6407075193976,
0.));
#223184=CARTESIAN_POINT('Ctrl Pts',(9.88808932697305,-20.6304074914087,
0.));
#223185=CARTESIAN_POINT('Ctrl Pts',(9.88091464472675,-20.6202308177475,
0.));
#223186=CARTESIAN_POINT('Ctrl Pts',(9.87387798732955,-20.6101800854494,
0.));
#223187=CARTESIAN_POINT('Ctrl Pts',(9.86697998242622,-20.6002579513699,
0.));
#223188=CARTESIAN_POINT('Ctrl Pts',(9.86022127232747,-20.5904671449754,
0.));
#223189=CARTESIAN_POINT('Ctrl Pts',(9.8536025145698,-20.5808104710015,0.));
#223190=CARTESIAN_POINT('Ctrl Pts',(9.84712438256277,-20.5712908125139,
0.));
#223191=CARTESIAN_POINT('Ctrl Pts',(9.84078756677565,-20.5619111362402,
0.));
#223192=CARTESIAN_POINT('Ctrl Pts',(9.83459277585315,-20.552674497646,0.));
#223193=CARTESIAN_POINT('Ctrl Pts',(9.82854073773876,-20.5435840460721,
0.));
#223194=CARTESIAN_POINT('Ctrl Pts',(9.82263220080362,-20.5346430299517,
0.));
#223195=CARTESIAN_POINT('Ctrl Pts',(9.81686793455942,-20.5258548000629,
0.));
#223196=CARTESIAN_POINT('Ctrl Pts',(9.81124873025281,-20.517222812284,0.));
#223197=CARTESIAN_POINT('Ctrl Pts',(9.80577540161087,-20.5087506310505,
0.));
#223198=CARTESIAN_POINT('Ctrl Pts',(9.80044878520948,-20.5004419312107,
0.));
#223199=CARTESIAN_POINT('Ctrl Pts',(9.7952697428833,-20.4923005087943,0.));
#223200=CARTESIAN_POINT('Ctrl Pts',(9.79023916498655,-20.4843302955329,
0.));
#223201=CARTESIAN_POINT('Ctrl Pts',(9.78535797314166,-20.4765353711586,
0.));
#223202=CARTESIAN_POINT('Ctrl Pts',(9.7806271237332,-20.4689199790669,0.));
#223203=CARTESIAN_POINT('Ctrl Pts',(9.77604760815528,-20.4614885274975,
0.));
#223204=CARTESIAN_POINT('Ctrl Pts',(9.77162045104069,-20.4542455817527,
0.));
#223205=CARTESIAN_POINT('Ctrl Pts',(9.76734670980891,-20.447195862298,0.));
#223206=CARTESIAN_POINT('Ctrl Pts',(9.76322747195494,-20.44034423294,0.));
#223207=CARTESIAN_POINT('Ctrl Pts',(9.75926386289922,-20.4336957355473,
0.));
#223208=CARTESIAN_POINT('Ctrl Pts',(9.75545705902417,-20.4272556476629,
0.));
#223209=CARTESIAN_POINT('Ctrl Pts',(9.75180829786429,-20.4210295275817,
0.));
#223210=CARTESIAN_POINT('Ctrl Pts',(9.74831889242173,-20.4150232777393,
0.));
#223211=CARTESIAN_POINT('Ctrl Pts',(9.74499021838537,-20.4092430879861,
0.));
#223212=CARTESIAN_POINT('Ctrl Pts',(9.74182369656271,-20.4036953576549,
0.));
#223213=CARTESIAN_POINT('Ctrl Pts',(9.738820776132,-20.3983866213331,0.));
#223214=CARTESIAN_POINT('Ctrl Pts',(9.73598292014242,-20.3933234845647,
0.));
#223215=CARTESIAN_POINT('Ctrl Pts',(9.73331167102807,-20.3885129129912,
0.));
#223216=CARTESIAN_POINT('Ctrl Pts',(9.73080870123726,-20.3839624556742,
0.));
#223217=CARTESIAN_POINT('Ctrl Pts',(9.72847589116541,-20.3796805893304,
0.));
#223218=CARTESIAN_POINT('Ctrl Pts',(9.7263153173288,-20.3756766651951,0.));
#223219=CARTESIAN_POINT('Ctrl Pts',(9.72432910043194,-20.371960235676,0.));
#223220=CARTESIAN_POINT('Ctrl Pts',(9.72251930722489,-20.3685406190576,
0.));
#223221=CARTESIAN_POINT('Ctrl Pts',(9.7208877838108,-20.3654261611056,0.));
#223222=CARTESIAN_POINT('Ctrl Pts',(9.71943648548099,-20.3626256913981,
0.));
#223223=CARTESIAN_POINT('Ctrl Pts',(9.71816778328006,-20.3601498764344,
0.));
#223224=CARTESIAN_POINT('Ctrl Pts',(9.71708493723096,-20.3580133103356,
0.));
#223225=CARTESIAN_POINT('Ctrl Pts',(9.71619192554185,-20.3562337557875,
0.));
#223226=CARTESIAN_POINT('Ctrl Pts',(9.71549257088172,-20.3548282742361,
0.));
#223227=CARTESIAN_POINT('Ctrl Pts',(9.7149897805202,-20.3538098605706,0.));
#223228=CARTESIAN_POINT('Ctrl Pts',(9.7147459035068,-20.3533097561886,0.));
#223229=CARTESIAN_POINT('Ctrl Pts',(9.71465227853041,-20.3531126095522,
0.));
#223230=CARTESIAN_POINT('Ctrl Pts',(9.71462954053041,-20.353060251684,0.));
#223231=CARTESIAN_POINT('Ctrl Pts',(9.71462809124915,-20.353053841303,0.));
#223232=CARTESIAN_POINT('',(12.4230808101438,-22.8400320311649,12.));
#223233=CARTESIAN_POINT('',(12.4230808101438,-22.8400320311649,0.));
#223234=CARTESIAN_POINT('Ctrl Pts',(9.71462809124915,-20.353053841303,12.));
#223235=CARTESIAN_POINT('Ctrl Pts',(9.71462954053041,-20.353060251684,12.));
#223236=CARTESIAN_POINT('Ctrl Pts',(9.71465227853041,-20.3531126095522,
12.));
#223237=CARTESIAN_POINT('Ctrl Pts',(9.7147459035068,-20.3533097561886,12.));
#223238=CARTESIAN_POINT('Ctrl Pts',(9.7149897805202,-20.3538098605706,12.));
#223239=CARTESIAN_POINT('Ctrl Pts',(9.71549257088172,-20.3548282742361,
12.));
#223240=CARTESIAN_POINT('Ctrl Pts',(9.71619192554185,-20.3562337557875,
12.));
#223241=CARTESIAN_POINT('Ctrl Pts',(9.71708493723096,-20.3580133103356,
12.));
#223242=CARTESIAN_POINT('Ctrl Pts',(9.71816778328006,-20.3601498764344,
12.));
#223243=CARTESIAN_POINT('Ctrl Pts',(9.71943648548099,-20.3626256913981,
12.));
#223244=CARTESIAN_POINT('Ctrl Pts',(9.7208877838108,-20.3654261611056,12.));
#223245=CARTESIAN_POINT('Ctrl Pts',(9.72251930722489,-20.3685406190576,
12.));
#223246=CARTESIAN_POINT('Ctrl Pts',(9.72432910043194,-20.371960235676,12.));
#223247=CARTESIAN_POINT('Ctrl Pts',(9.7263153173288,-20.3756766651951,12.));
#223248=CARTESIAN_POINT('Ctrl Pts',(9.72847589116541,-20.3796805893304,
12.));
#223249=CARTESIAN_POINT('Ctrl Pts',(9.73080870123726,-20.3839624556742,
12.));
#223250=CARTESIAN_POINT('Ctrl Pts',(9.73331167102807,-20.3885129129912,
12.));
#223251=CARTESIAN_POINT('Ctrl Pts',(9.73598292014242,-20.3933234845647,
12.));
#223252=CARTESIAN_POINT('Ctrl Pts',(9.738820776132,-20.3983866213331,12.));
#223253=CARTESIAN_POINT('Ctrl Pts',(9.74182369656271,-20.4036953576549,
12.));
#223254=CARTESIAN_POINT('Ctrl Pts',(9.74499021838537,-20.4092430879861,
12.));
#223255=CARTESIAN_POINT('Ctrl Pts',(9.74831889242173,-20.4150232777393,
12.));
#223256=CARTESIAN_POINT('Ctrl Pts',(9.75180829786429,-20.4210295275817,
12.));
#223257=CARTESIAN_POINT('Ctrl Pts',(9.75545705902417,-20.4272556476629,
12.));
#223258=CARTESIAN_POINT('Ctrl Pts',(9.75926386289922,-20.4336957355473,
12.));
#223259=CARTESIAN_POINT('Ctrl Pts',(9.76322747195494,-20.44034423294,12.));
#223260=CARTESIAN_POINT('Ctrl Pts',(9.76734670980891,-20.447195862298,12.));
#223261=CARTESIAN_POINT('Ctrl Pts',(9.77162045104069,-20.4542455817527,
12.));
#223262=CARTESIAN_POINT('Ctrl Pts',(9.77604760815528,-20.4614885274975,
12.));
#223263=CARTESIAN_POINT('Ctrl Pts',(9.7806271237332,-20.4689199790669,12.));
#223264=CARTESIAN_POINT('Ctrl Pts',(9.78535797314166,-20.4765353711586,
12.));
#223265=CARTESIAN_POINT('Ctrl Pts',(9.79023916498655,-20.4843302955329,
12.));
#223266=CARTESIAN_POINT('Ctrl Pts',(9.7952697428833,-20.4923005087943,12.));
#223267=CARTESIAN_POINT('Ctrl Pts',(9.80044878520948,-20.5004419312107,
12.));
#223268=CARTESIAN_POINT('Ctrl Pts',(9.80577540161087,-20.5087506310505,
12.));
#223269=CARTESIAN_POINT('Ctrl Pts',(9.81124873025281,-20.517222812284,12.));
#223270=CARTESIAN_POINT('Ctrl Pts',(9.81686793455942,-20.5258548000629,
12.));
#223271=CARTESIAN_POINT('Ctrl Pts',(9.82263220080362,-20.5346430299517,
12.));
#223272=CARTESIAN_POINT('Ctrl Pts',(9.82854073773876,-20.5435840460721,
12.));
#223273=CARTESIAN_POINT('Ctrl Pts',(9.83459277585315,-20.552674497646,12.));
#223274=CARTESIAN_POINT('Ctrl Pts',(9.84078756677565,-20.5619111362402,
12.));
#223275=CARTESIAN_POINT('Ctrl Pts',(9.84712438256277,-20.5712908125139,
12.));
#223276=CARTESIAN_POINT('Ctrl Pts',(9.8536025145698,-20.5808104710015,12.));
#223277=CARTESIAN_POINT('Ctrl Pts',(9.86022127232747,-20.5904671449754,
12.));
#223278=CARTESIAN_POINT('Ctrl Pts',(9.86697998242622,-20.6002579513699,
12.));
#223279=CARTESIAN_POINT('Ctrl Pts',(9.87387798732955,-20.6101800854494,
12.));
#223280=CARTESIAN_POINT('Ctrl Pts',(9.88091464472675,-20.6202308177475,
12.));
#223281=CARTESIAN_POINT('Ctrl Pts',(9.88808932697305,-20.6304074914087,
12.));
#223282=CARTESIAN_POINT('Ctrl Pts',(9.89540142049119,-20.6407075193976,
12.));
#223283=CARTESIAN_POINT('Ctrl Pts',(9.90285032516692,-20.6511283817414,
12.));
#223284=CARTESIAN_POINT('Ctrl Pts',(9.91043545377007,-20.6616676228315,
12.));
#223285=CARTESIAN_POINT('Ctrl Pts',(9.91815623141288,-20.6723228488263,
12.));
#223286=CARTESIAN_POINT('Ctrl Pts',(9.92601209498748,-20.6830917250255,
12.));
#223287=CARTESIAN_POINT('Ctrl Pts',(9.93400249259729,-20.6939719732484,
12.));
#223288=CARTESIAN_POINT('Ctrl Pts',(9.94212688298236,-20.7049613692234,
12.));
#223289=CARTESIAN_POINT('Ctrl Pts',(9.95038473514948,-20.7160577407579,
12.));
#223290=CARTESIAN_POINT('Ctrl Pts',(9.95877552798397,-20.7272589658751,
12.));
#223291=CARTESIAN_POINT('Ctrl Pts',(9.96729874986201,-20.7385629709795,
12.));
#223292=CARTESIAN_POINT('Ctrl Pts',(9.97595389823469,-20.7499677289627,
12.));
#223293=CARTESIAN_POINT('Ctrl Pts',(9.98474047926852,-20.761471257499,12.));
#223294=CARTESIAN_POINT('Ctrl Pts',(9.9936580075464,-20.7730716175417,12.));
#223295=CARTESIAN_POINT('Ctrl Pts',(10.0027060057389,-20.7847669117568,
12.));
#223296=CARTESIAN_POINT('Ctrl Pts',(10.0118840042786,-20.7965552829908,
12.));
#223297=CARTESIAN_POINT('Ctrl Pts',(10.0211915410095,-20.8084349126888,
12.));
#223298=CARTESIAN_POINT('Ctrl Pts',(10.0306281609435,-20.8204040196602,
12.));
#223299=CARTESIAN_POINT('Ctrl Pts',(10.0401934160234,-20.8324608588909,
12.));
#223300=CARTESIAN_POINT('Ctrl Pts',(10.0498868648733,-20.8446037203402,
12.));
#223301=CARTESIAN_POINT('Ctrl Pts',(10.0597080725375,-20.8568309277316,
12.));
#223302=CARTESIAN_POINT('Ctrl Pts',(10.0696566102218,-20.86914083737,12.));
#223303=CARTESIAN_POINT('Ctrl Pts',(10.0797320551154,-20.881531837184,12.));
#223304=CARTESIAN_POINT('Ctrl Pts',(10.0899339901915,-20.894002345737,12.));
#223305=CARTESIAN_POINT('Ctrl Pts',(10.1002620040076,-20.9065508112557,
12.));
#223306=CARTESIAN_POINT('Ctrl Pts',(10.1107156904836,-20.919175710627,12.));
#223307=CARTESIAN_POINT('Ctrl Pts',(10.1212946487057,-20.9318755484734,
12.));
#223308=CARTESIAN_POINT('Ctrl Pts',(10.1319984827908,-20.9446488563933,
12.));
#223309=CARTESIAN_POINT('Ctrl Pts',(10.1428268017256,-20.9574941921591,
12.));
#223310=CARTESIAN_POINT('Ctrl Pts',(10.1537792192065,-20.9704101389369,
12.));
#223311=CARTESIAN_POINT('Ctrl Pts',(10.1648553534568,-20.9833953044736,
12.));
#223312=CARTESIAN_POINT('Ctrl Pts',(10.1760548270767,-20.9964483203686,
12.));
#223313=CARTESIAN_POINT('Ctrl Pts',(10.187377266936,-21.0095678414486,12.));
#223314=CARTESIAN_POINT('Ctrl Pts',(10.1988223040425,-21.0227525451107,
12.));
#223315=CARTESIAN_POINT('Ctrl Pts',(10.2103895734123,-21.0360011306815,
12.));
#223316=CARTESIAN_POINT('Ctrl Pts',(10.2220787139154,-21.0493123187483,
12.));
#223317=CARTESIAN_POINT('Ctrl Pts',(10.2338893681567,-21.0626848505663,
12.));
#223318=CARTESIAN_POINT('Ctrl Pts',(10.2458211823912,-21.0761174875445,
12.));
#223319=CARTESIAN_POINT('Ctrl Pts',(10.2578738064181,-21.0896090107063,
12.));
#223320=CARTESIAN_POINT('Ctrl Pts',(10.2700468934744,-21.1031582201627,
12.));
#223321=CARTESIAN_POINT('Ctrl Pts',(10.2823401001072,-21.1167639345631,
12.));
#223322=CARTESIAN_POINT('Ctrl Pts',(10.2947530860721,-21.1304249906002,
12.));
#223323=CARTESIAN_POINT('Ctrl Pts',(10.3072855142687,-21.1441402425843,
12.));
#223324=CARTESIAN_POINT('Ctrl Pts',(10.3199370506544,-21.1579085619965,
12.));
#223325=CARTESIAN_POINT('Ctrl Pts',(10.3327073641572,-21.1717288370509,
12.));
#223326=CARTESIAN_POINT('Ctrl Pts',(10.34559612657,-21.1855999722416,12.));
#223327=CARTESIAN_POINT('Ctrl Pts',(10.3586030124587,-21.199520887919,12.));
#223328=CARTESIAN_POINT('Ctrl Pts',(10.371727699113,-21.2134905199345,12.));
#223329=CARTESIAN_POINT('Ctrl Pts',(10.3849698664786,-21.22750781927,12.));
#223330=CARTESIAN_POINT('Ctrl Pts',(10.3983291970846,-21.2415717516714,
12.));
#223331=CARTESIAN_POINT('Ctrl Pts',(10.4118053759588,-21.255681297275,12.));
#223332=CARTESIAN_POINT('Ctrl Pts',(10.42539809054,-21.2698354502403,12.));
#223333=CARTESIAN_POINT('Ctrl Pts',(10.4391070306391,-21.2840332184483,
12.));
#223334=CARTESIAN_POINT('Ctrl Pts',(10.4529318883874,-21.2982736231931,
12.));
#223335=CARTESIAN_POINT('Ctrl Pts',(10.4668723581768,-21.3125556988731,
12.));
#223336=CARTESIAN_POINT('Ctrl Pts',(10.4809281365931,-21.3268784926819,
12.));
#223337=CARTESIAN_POINT('Ctrl Pts',(10.4950989223336,-21.3412410642904,
12.));
#223338=CARTESIAN_POINT('Ctrl Pts',(10.5093844161685,-21.3556424855814,
12.));
#223339=CARTESIAN_POINT('Ctrl Pts',(10.5237843209057,-21.3700818403936,
12.));
#223340=CARTESIAN_POINT('Ctrl Pts',(10.5382983413421,-21.3845582242602,
12.));
#223341=CARTESIAN_POINT('Ctrl Pts',(10.5529261842108,-21.3990707441497,
12.));
#223342=CARTESIAN_POINT('Ctrl Pts',(10.5676675581108,-21.4136185181979,
12.));
#223343=CARTESIAN_POINT('Ctrl Pts',(10.5825221734573,-21.4282006754631,
12.));
#223344=CARTESIAN_POINT('Ctrl Pts',(10.5974897424622,-21.4428163557144,
12.));
#223345=CARTESIAN_POINT('Ctrl Pts',(10.6125699790961,-21.4574647092097,
12.));
#223346=CARTESIAN_POINT('Ctrl Pts',(10.6277625990456,-21.4721448964766,
12.));
#223347=CARTESIAN_POINT('Ctrl Pts',(10.6430673196607,-21.4868560880889,
12.));
#223348=CARTESIAN_POINT('Ctrl Pts',(10.6584838598939,-21.5015974644449,
12.));
#223349=CARTESIAN_POINT('Ctrl Pts',(10.6740119402834,-21.51636821558,12.));
#223350=CARTESIAN_POINT('Ctrl Pts',(10.689651282929,-21.5311675409807,12.));
#223351=CARTESIAN_POINT('Ctrl Pts',(10.7054016114571,-21.5459946493955,
12.));
#223352=CARTESIAN_POINT('Ctrl Pts',(10.7212626509816,-21.5608487586468,
12.));
#223353=CARTESIAN_POINT('Ctrl Pts',(10.7372341280467,-21.5757290954371,
12.));
#223354=CARTESIAN_POINT('Ctrl Pts',(10.7533157705941,-21.5906348951743,
12.));
#223355=CARTESIAN_POINT('Ctrl Pts',(10.7695073079552,-21.6055654018176,
12.));
#223356=CARTESIAN_POINT('Ctrl Pts',(10.7858084708261,-21.6205198677173,
12.));
#223357=CARTESIAN_POINT('Ctrl Pts',(10.8022189912369,-21.6354975534557,
12.));
#223358=CARTESIAN_POINT('Ctrl Pts',(10.8187386025136,-21.6504977276866,
12.));
#223359=CARTESIAN_POINT('Ctrl Pts',(10.8353670392272,-21.6655196669732,
12.));
#223360=CARTESIAN_POINT('Ctrl Pts',(10.8521040371835,-21.6805626556467,
12.));
#223361=CARTESIAN_POINT('Ctrl Pts',(10.8689493334095,-21.6956259856672,
12.));
#223362=CARTESIAN_POINT('Ctrl Pts',(10.8859026661293,-21.7107089564825,
12.));
#223363=CARTESIAN_POINT('Ctrl Pts',(10.902963774734,-21.7258108748873,12.));
#223364=CARTESIAN_POINT('Ctrl Pts',(10.9201323997384,-21.7409310548797,
12.));
#223365=CARTESIAN_POINT('Ctrl Pts',(10.9374082827444,-21.7560688175247,
12.));
#223366=CARTESIAN_POINT('Ctrl Pts',(10.9547911664455,-21.7712234908464,
12.));
#223367=CARTESIAN_POINT('Ctrl Pts',(10.9722807946155,-21.7863944097141,
12.));
#223368=CARTESIAN_POINT('Ctrl Pts',(10.9898769120912,-21.8015809157301,
12.));
#223369=CARTESIAN_POINT('Ctrl Pts',(11.0075792647477,-21.8167823571168,
12.));
#223370=CARTESIAN_POINT('Ctrl Pts',(11.0253875994598,-21.8319980886033,
12.));
#223371=CARTESIAN_POINT('Ctrl Pts',(11.0433016640807,-21.8472274713103,
12.));
#223372=CARTESIAN_POINT('Ctrl Pts',(11.0613212074363,-21.8624698726318,
12.));
#223373=CARTESIAN_POINT('Ctrl Pts',(11.0794459793057,-21.877724666119,12.));
#223374=CARTESIAN_POINT('Ctrl Pts',(11.0976757303944,-21.8929912313608,
12.));
#223375=CARTESIAN_POINT('Ctrl Pts',(11.1160102123024,-21.9082689538688,
12.));
#223376=CARTESIAN_POINT('Ctrl Pts',(11.1344491774741,-21.923557224952,12.));
#223377=CARTESIAN_POINT('Ctrl Pts',(11.1529923792003,-21.9388554416439,
12.));
#223378=CARTESIAN_POINT('Ctrl Pts',(11.1716395716376,-21.9541630066506,
12.));
#223379=CARTESIAN_POINT('Ctrl Pts',(11.190390509811,-21.9694793282914,12.));
#223380=CARTESIAN_POINT('Ctrl Pts',(11.2092449496125,-21.9848038204439,
12.));
#223381=CARTESIAN_POINT('Ctrl Pts',(11.2282026477896,-22.0001359024839,
12.));
#223382=CARTESIAN_POINT('Ctrl Pts',(11.2472633619275,-22.0154749992363,
12.));
#223383=CARTESIAN_POINT('Ctrl Pts',(11.2664268504206,-22.030820540835,12.));
#223384=CARTESIAN_POINT('Ctrl Pts',(11.2856928724374,-22.046171962566,12.));
#223385=CARTESIAN_POINT('Ctrl Pts',(11.3050611878771,-22.0615287047179,
12.));
#223386=CARTESIAN_POINT('Ctrl Pts',(11.3245315573168,-22.0768902124267,
12.));
#223387=CARTESIAN_POINT('Ctrl Pts',(11.3441037419553,-22.0922559355294,
12.));
#223388=CARTESIAN_POINT('Ctrl Pts',(11.3637775035367,-22.1076253283979,
12.));
#223389=CARTESIAN_POINT('Ctrl Pts',(11.3835526044256,-22.1229978500186,
12.));
#223390=CARTESIAN_POINT('Ctrl Pts',(11.4034288076908,-22.1383729640964,
12.));
#223391=CARTESIAN_POINT('Ctrl Pts',(11.4234058771742,-22.1537501391487,
12.));
#223392=CARTESIAN_POINT('Ctrl Pts',(11.443483577557,-22.1691288486096,12.));
#223393=CARTESIAN_POINT('Ctrl Pts',(11.463661674411,-22.184508570917,12.));
#223394=CARTESIAN_POINT('Ctrl Pts',(11.483939934259,-22.1998887896436,12.));
#223395=CARTESIAN_POINT('Ctrl Pts',(11.5043181244242,-22.2152689931022,
12.));
#223396=CARTESIAN_POINT('Ctrl Pts',(11.5247960128477,-22.2306486738901,
12.));
#223397=CARTESIAN_POINT('Ctrl Pts',(11.5453733679121,-22.2460273284654,
12.));
#223398=CARTESIAN_POINT('Ctrl Pts',(11.5660499582403,-22.2614044566898,
12.));
#223399=CARTESIAN_POINT('Ctrl Pts',(11.5868255525188,-22.2767795614348,
12.));
#223400=CARTESIAN_POINT('Ctrl Pts',(11.6076999192357,-22.2921521480356,
12.));
#223401=CARTESIAN_POINT('Ctrl Pts',(11.6286728270009,-22.3075217249049,
12.));
#223402=CARTESIAN_POINT('Ctrl Pts',(11.6497440449857,-22.3228878043976,
12.));
#223403=CARTESIAN_POINT('Ctrl Pts',(11.6709133432985,-22.3382499035619,
12.));
#223404=CARTESIAN_POINT('Ctrl Pts',(11.6921804934056,-22.3536075450029,
12.));
#223405=CARTESIAN_POINT('Ctrl Pts',(11.7135452684532,-22.3689602575491,
12.));
#223406=CARTESIAN_POINT('Ctrl Pts',(11.7350074437961,-22.3843075773899,
12.));
#223407=CARTESIAN_POINT('Ctrl Pts',(11.7565667964764,-22.3996490469191,
12.));
#223408=CARTESIAN_POINT('Ctrl Pts',(11.7782231042039,-22.4149842125008,
12.));
#223409=CARTESIAN_POINT('Ctrl Pts',(11.7999761445173,-22.430312622646,12.));
#223410=CARTESIAN_POINT('Ctrl Pts',(11.8218256937889,-22.4456338258735,
12.));
#223411=CARTESIAN_POINT('Ctrl Pts',(11.8437715264487,-22.4609473690472,
12.));
#223412=CARTESIAN_POINT('Ctrl Pts',(11.8658134137019,-22.4762527946702,
12.));
#223413=CARTESIAN_POINT('Ctrl Pts',(11.8879511239942,-22.4915496418485,
12.));
#223414=CARTESIAN_POINT('Ctrl Pts',(11.9101844254557,-22.5068374513973,
12.));
#223415=CARTESIAN_POINT('Ctrl Pts',(11.9325130877803,-22.5221157697883,
12.));
#223416=CARTESIAN_POINT('Ctrl Pts',(11.9549368843997,-22.5373841537307,
12.));
#223417=CARTESIAN_POINT('Ctrl Pts',(11.9774555943496,-22.5526421741158,
12.));
#223418=CARTESIAN_POINT('Ctrl Pts',(12.0000690046694,-22.5678894211181,
12.));
#223419=CARTESIAN_POINT('Ctrl Pts',(12.0227769113127,-22.5831255061282,
12.));
#223420=CARTESIAN_POINT('Ctrl Pts',(12.0455791139128,-22.5983500505644,
12.));
#223421=CARTESIAN_POINT('Ctrl Pts',(12.0684754113862,-22.6135626764898,
12.));
#223422=CARTESIAN_POINT('Ctrl Pts',(12.0914655972823,-22.6287629967056,
12.));
#223423=CARTESIAN_POINT('Ctrl Pts',(12.1145494550383,-22.6439506046605,
12.));
#223424=CARTESIAN_POINT('Ctrl Pts',(12.1377267537145,-22.6591250653965,
12.));
#223425=CARTESIAN_POINT('Ctrl Pts',(12.1609972423099,-22.6742859034944,
12.));
#223426=CARTESIAN_POINT('Ctrl Pts',(12.1843606579261,-22.6894326205037,
12.));
#223427=CARTESIAN_POINT('Ctrl Pts',(12.2078167360284,-22.7045647168747,
12.));
#223428=CARTESIAN_POINT('Ctrl Pts',(12.2313652198061,-22.7196817119374,
12.));
#223429=CARTESIAN_POINT('Ctrl Pts',(12.2550058702395,-22.7347831655287,
12.));
#223430=CARTESIAN_POINT('Ctrl Pts',(12.2787384750742,-22.7498686970069,
12.));
#223431=CARTESIAN_POINT('Ctrl Pts',(12.3025628601792,-22.764938010105,12.));
#223432=CARTESIAN_POINT('Ctrl Pts',(12.3264788926075,-22.7799908974768,
12.));
#223433=CARTESIAN_POINT('Ctrl Pts',(12.3504864740319,-22.795027221673,12.));
#223434=CARTESIAN_POINT('Ctrl Pts',(12.374585536673,-22.81004690224,12.));
#223435=CARTESIAN_POINT('Ctrl Pts',(12.3939379378998,-22.8220493007173,
12.));
#223436=CARTESIAN_POINT('Ctrl Pts',(12.4084933766346,-22.8310435872748,
12.));
#223437=CARTESIAN_POINT('Ctrl Pts',(12.418215285186,-22.8370364396459,12.));
#223438=CARTESIAN_POINT('Ctrl Pts',(12.4230808101438,-22.8400320311649,
12.));
#223439=CARTESIAN_POINT('Ctrl Pts',(7.52250298901263,-21.2610617890679,
0.));
#223440=CARTESIAN_POINT('Ctrl Pts',(7.52250298901263,-21.2610617890679,
12.));
#223441=CARTESIAN_POINT('Ctrl Pts',(7.52250649703969,-21.2610673466886,
0.));
#223442=CARTESIAN_POINT('Ctrl Pts',(7.52250649703969,-21.2610673466886,
12.));
#223443=CARTESIAN_POINT('Ctrl Pts',(7.52252744144903,-21.2611204474866,
0.));
#223444=CARTESIAN_POINT('Ctrl Pts',(7.52252744144903,-21.2611204474866,
12.));
#223445=CARTESIAN_POINT('Ctrl Pts',(7.5226006423166,-21.261326054066,0.));
#223446=CARTESIAN_POINT('Ctrl Pts',(7.5226006423166,-21.261326054066,12.));
#223447=CARTESIAN_POINT('Ctrl Pts',(7.52278182242669,-21.2618521283555,
0.));
#223448=CARTESIAN_POINT('Ctrl Pts',(7.52278182242669,-21.2618521283555,
12.));
#223449=CARTESIAN_POINT('Ctrl Pts',(7.52314642316199,-21.262927782038,0.));
#223450=CARTESIAN_POINT('Ctrl Pts',(7.52314642316199,-21.262927782038,12.));
#223451=CARTESIAN_POINT('Ctrl Pts',(7.52364573027552,-21.2644161259962,
0.));
#223452=CARTESIAN_POINT('Ctrl Pts',(7.52364573027552,-21.2644161259962,
12.));
#223453=CARTESIAN_POINT('Ctrl Pts',(7.52427261074297,-21.2663059157058,
0.));
#223454=CARTESIAN_POINT('Ctrl Pts',(7.52427261074297,-21.2663059157058,
12.));
#223455=CARTESIAN_POINT('Ctrl Pts',(7.5250177033353,-21.2685823838671,0.));
#223456=CARTESIAN_POINT('Ctrl Pts',(7.5250177033353,-21.2685823838671,12.));
#223457=CARTESIAN_POINT('Ctrl Pts',(7.52587126095529,-21.2712301573466,
0.));
#223458=CARTESIAN_POINT('Ctrl Pts',(7.52587126095529,-21.2712301573466,
12.));
#223459=CARTESIAN_POINT('Ctrl Pts',(7.5268252691854,-21.2742366113579,0.));
#223460=CARTESIAN_POINT('Ctrl Pts',(7.5268252691854,-21.2742366113579,12.));
#223461=CARTESIAN_POINT('Ctrl Pts',(7.52787386225332,-21.2775925269652,
0.));
#223462=CARTESIAN_POINT('Ctrl Pts',(7.52787386225332,-21.2775925269652,
12.));
#223463=CARTESIAN_POINT('Ctrl Pts',(7.52901217930407,-21.2812902781143,
0.));
#223464=CARTESIAN_POINT('Ctrl Pts',(7.52901217930407,-21.2812902781143,
12.));
#223465=CARTESIAN_POINT('Ctrl Pts',(7.53023562438229,-21.2853226580657,
0.));
#223466=CARTESIAN_POINT('Ctrl Pts',(7.53023562438229,-21.2853226580657,
12.));
#223467=CARTESIAN_POINT('Ctrl Pts',(7.53153906987855,-21.2896816163842,
0.));
#223468=CARTESIAN_POINT('Ctrl Pts',(7.53153906987855,-21.2896816163842,
12.));
#223469=CARTESIAN_POINT('Ctrl Pts',(7.53291726078526,-21.2943588989331,
0.));
#223470=CARTESIAN_POINT('Ctrl Pts',(7.53291726078526,-21.2943588989331,
12.));
#223471=CARTESIAN_POINT('Ctrl Pts',(7.53436505309942,-21.2993464250717,
0.));
#223472=CARTESIAN_POINT('Ctrl Pts',(7.53436505309942,-21.2993464250717,
12.));
#223473=CARTESIAN_POINT('Ctrl Pts',(7.53587778251735,-21.3046368712157,
0.));
#223474=CARTESIAN_POINT('Ctrl Pts',(7.53587778251735,-21.3046368712157,
12.));
#223475=CARTESIAN_POINT('Ctrl Pts',(7.53745129364615,-21.310223716773,0.));
#223476=CARTESIAN_POINT('Ctrl Pts',(7.53745129364615,-21.310223716773,12.));
#223477=CARTESIAN_POINT('Ctrl Pts',(7.53908175169898,-21.3161009456256,
0.));
#223478=CARTESIAN_POINT('Ctrl Pts',(7.53908175169898,-21.3161009456256,
12.));
#223479=CARTESIAN_POINT('Ctrl Pts',(7.54076552038278,-21.3222628524165,
0.));
#223480=CARTESIAN_POINT('Ctrl Pts',(7.54076552038278,-21.3222628524165,
12.));
#223481=CARTESIAN_POINT('Ctrl Pts',(7.5424990037703,-21.328703791771,0.));
#223482=CARTESIAN_POINT('Ctrl Pts',(7.5424990037703,-21.328703791771,12.));
#223483=CARTESIAN_POINT('Ctrl Pts',(7.54427868151267,-21.3354182340149,
0.));
#223484=CARTESIAN_POINT('Ctrl Pts',(7.54427868151267,-21.3354182340149,
12.));
#223485=CARTESIAN_POINT('Ctrl Pts',(7.54610114948346,-21.3424008295038,
0.));
#223486=CARTESIAN_POINT('Ctrl Pts',(7.54610114948346,-21.3424008295038,
12.));
#223487=CARTESIAN_POINT('Ctrl Pts',(7.5479631624633,-21.3496464761531,0.));
#223488=CARTESIAN_POINT('Ctrl Pts',(7.5479631624633,-21.3496464761531,12.));
#223489=CARTESIAN_POINT('Ctrl Pts',(7.54986166521309,-21.3571503685855,
0.));
#223490=CARTESIAN_POINT('Ctrl Pts',(7.54986166521309,-21.3571503685855,
12.));
#223491=CARTESIAN_POINT('Ctrl Pts',(7.55179375777443,-21.3649079431865,
0.));
#223492=CARTESIAN_POINT('Ctrl Pts',(7.55179375777443,-21.3649079431865,
12.));
#223493=CARTESIAN_POINT('Ctrl Pts',(7.55375667080028,-21.3729148390243,
0.));
#223494=CARTESIAN_POINT('Ctrl Pts',(7.55375667080028,-21.3729148390243,
12.));
#223495=CARTESIAN_POINT('Ctrl Pts',(7.55574773403502,-21.3811668478932,
0.));
#223496=CARTESIAN_POINT('Ctrl Pts',(7.55574773403502,-21.3811668478932,
12.));
#223497=CARTESIAN_POINT('Ctrl Pts',(7.55776435731416,-21.3896598842117,
0.));
#223498=CARTESIAN_POINT('Ctrl Pts',(7.55776435731416,-21.3896598842117,
12.));
#223499=CARTESIAN_POINT('Ctrl Pts',(7.5598040370061,-21.3983899952987,0.));
#223500=CARTESIAN_POINT('Ctrl Pts',(7.5598040370061,-21.3983899952987,12.));
#223501=CARTESIAN_POINT('Ctrl Pts',(7.56186435703621,-21.4073533630365,
0.));
#223502=CARTESIAN_POINT('Ctrl Pts',(7.56186435703621,-21.4073533630365,
12.));
#223503=CARTESIAN_POINT('Ctrl Pts',(7.56394299313684,-21.4165463106254,
0.));
#223504=CARTESIAN_POINT('Ctrl Pts',(7.56394299313684,-21.4165463106254,
12.));
#223505=CARTESIAN_POINT('Ctrl Pts',(7.56603771218711,-21.4259653015736,
0.));
#223506=CARTESIAN_POINT('Ctrl Pts',(7.56603771218711,-21.4259653015736,
12.));
#223507=CARTESIAN_POINT('Ctrl Pts',(7.56814636360847,-21.4356069261513,
0.));
#223508=CARTESIAN_POINT('Ctrl Pts',(7.56814636360847,-21.4356069261513,
12.));
#223509=CARTESIAN_POINT('Ctrl Pts',(7.57026687261165,-21.4454678907509,
0.));
#223510=CARTESIAN_POINT('Ctrl Pts',(7.57026687261165,-21.4454678907509,
12.));
#223511=CARTESIAN_POINT('Ctrl Pts',(7.57239723223505,-21.4555450053142,
0.));
#223512=CARTESIAN_POINT('Ctrl Pts',(7.57239723223505,-21.4555450053142,
12.));
#223513=CARTESIAN_POINT('Ctrl Pts',(7.57453549743411,-21.4658351740128,
0.));
#223514=CARTESIAN_POINT('Ctrl Pts',(7.57453549743411,-21.4658351740128,
12.));
#223515=CARTESIAN_POINT('Ctrl Pts',(7.57667978402986,-21.4763353936762,
0.));
#223516=CARTESIAN_POINT('Ctrl Pts',(7.57667978402986,-21.4763353936762,
12.));
#223517=CARTESIAN_POINT('Ctrl Pts',(7.57882826679131,-21.4870427508194,
0.));
#223518=CARTESIAN_POINT('Ctrl Pts',(7.57882826679131,-21.4870427508194,
12.));
#223519=CARTESIAN_POINT('Ctrl Pts',(7.58097917790743,-21.4979544192744,
0.));
#223520=CARTESIAN_POINT('Ctrl Pts',(7.58097917790743,-21.4979544192744,
12.));
#223521=CARTESIAN_POINT('Ctrl Pts',(7.58313080519179,-21.5090676573873,
0.));
#223522=CARTESIAN_POINT('Ctrl Pts',(7.58313080519179,-21.5090676573873,
12.));
#223523=CARTESIAN_POINT('Ctrl Pts',(7.58528148919129,-21.5203798035299,
0.));
#223524=CARTESIAN_POINT('Ctrl Pts',(7.58528148919129,-21.5203798035299,
12.));
#223525=CARTESIAN_POINT('Ctrl Pts',(7.58742962034833,-21.5318882716736,
0.));
#223526=CARTESIAN_POINT('Ctrl Pts',(7.58742962034833,-21.5318882716736,
12.));
#223527=CARTESIAN_POINT('Ctrl Pts',(7.58957363620013,-21.543590547011,0.));
#223528=CARTESIAN_POINT('Ctrl Pts',(7.58957363620013,-21.543590547011,12.));
#223529=CARTESIAN_POINT('Ctrl Pts',(7.59171201844776,-21.5554841813462,
0.));
#223530=CARTESIAN_POINT('Ctrl Pts',(7.59171201844776,-21.5554841813462,
12.));
#223531=CARTESIAN_POINT('Ctrl Pts',(7.59384329124918,-21.5675667904726,
0.));
#223532=CARTESIAN_POINT('Ctrl Pts',(7.59384329124918,-21.5675667904726,
12.));
#223533=CARTESIAN_POINT('Ctrl Pts',(7.59596601973583,-21.5798360518978,
0.));
#223534=CARTESIAN_POINT('Ctrl Pts',(7.59596601973583,-21.5798360518978,
12.));
#223535=CARTESIAN_POINT('Ctrl Pts',(7.59807880846194,-21.5922897024466,
0.));
#223536=CARTESIAN_POINT('Ctrl Pts',(7.59807880846194,-21.5922897024466,
12.));
#223537=CARTESIAN_POINT('Ctrl Pts',(7.6001802998824,-21.6049255358843,0.));
#223538=CARTESIAN_POINT('Ctrl Pts',(7.6001802998824,-21.6049255358843,12.));
#223539=CARTESIAN_POINT('Ctrl Pts',(7.60226917285428,-21.617741400599,0.));
#223540=CARTESIAN_POINT('Ctrl Pts',(7.60226917285428,-21.617741400599,12.));
#223541=CARTESIAN_POINT('Ctrl Pts',(7.60434414118295,-21.6307351973822,
0.));
#223542=CARTESIAN_POINT('Ctrl Pts',(7.60434414118295,-21.6307351973822,
12.));
#223543=CARTESIAN_POINT('Ctrl Pts',(7.60640395216356,-21.6439048771743,
0.));
#223544=CARTESIAN_POINT('Ctrl Pts',(7.60640395216356,-21.6439048771743,
12.));
#223545=CARTESIAN_POINT('Ctrl Pts',(7.60844738512873,-21.6572484388081,
0.));
#223546=CARTESIAN_POINT('Ctrl Pts',(7.60844738512873,-21.6572484388081,
12.));
#223547=CARTESIAN_POINT('Ctrl Pts',(7.61047325000955,-21.6707639267576,
0.));
#223548=CARTESIAN_POINT('Ctrl Pts',(7.61047325000955,-21.6707639267576,
12.));
#223549=CARTESIAN_POINT('Ctrl Pts',(7.61248038630268,-21.6844494295815,
0.));
#223550=CARTESIAN_POINT('Ctrl Pts',(7.61248038630268,-21.6844494295815,
12.));
#223551=CARTESIAN_POINT('Ctrl Pts',(7.61446766202786,-21.6983030783322,
0.));
#223552=CARTESIAN_POINT('Ctrl Pts',(7.61446766202786,-21.6983030783322,
12.));
#223553=CARTESIAN_POINT('Ctrl Pts',(7.6164339727042,-21.7123230449834,0.));
#223554=CARTESIAN_POINT('Ctrl Pts',(7.6164339727042,-21.7123230449834,12.));
#223555=CARTESIAN_POINT('Ctrl Pts',(7.61837824030537,-21.7265075407975,
0.));
#223556=CARTESIAN_POINT('Ctrl Pts',(7.61837824030537,-21.7265075407975,
12.));
#223557=CARTESIAN_POINT('Ctrl Pts',(7.62029941230854,-21.7408548148656,
0.));
#223558=CARTESIAN_POINT('Ctrl Pts',(7.62029941230854,-21.7408548148656,
12.));
#223559=CARTESIAN_POINT('Ctrl Pts',(7.62219646084228,-21.7553631528328,
0.));
#223560=CARTESIAN_POINT('Ctrl Pts',(7.62219646084228,-21.7553631528328,
12.));
#223561=CARTESIAN_POINT('Ctrl Pts',(7.62406838181165,-21.7700308755584,
0.));
#223562=CARTESIAN_POINT('Ctrl Pts',(7.62406838181165,-21.7700308755584,
12.));
#223563=CARTESIAN_POINT('Ctrl Pts',(7.62591419404512,-21.7848563378021,
0.));
#223564=CARTESIAN_POINT('Ctrl Pts',(7.62591419404512,-21.7848563378021,
12.));
#223565=CARTESIAN_POINT('Ctrl Pts',(7.62773293842388,-21.799837926858,0.));
#223566=CARTESIAN_POINT('Ctrl Pts',(7.62773293842388,-21.799837926858,12.));
#223567=CARTESIAN_POINT('Ctrl Pts',(7.62952367718126,-21.814974061509,0.));
#223568=CARTESIAN_POINT('Ctrl Pts',(7.62952367718126,-21.814974061509,12.));
#223569=CARTESIAN_POINT('Ctrl Pts',(7.63128549323022,-21.8302631910195,
0.));
#223570=CARTESIAN_POINT('Ctrl Pts',(7.63128549323022,-21.8302631910195,
12.));
#223571=CARTESIAN_POINT('Ctrl Pts',(7.63301748948935,-21.8457037941084,
0.));
#223572=CARTESIAN_POINT('Ctrl Pts',(7.63301748948935,-21.8457037941084,
12.));
#223573=CARTESIAN_POINT('Ctrl Pts',(7.63471878821225,-21.8612943779089,
0.));
#223574=CARTESIAN_POINT('Ctrl Pts',(7.63471878821225,-21.8612943779089,
12.));
#223575=CARTESIAN_POINT('Ctrl Pts',(7.63638853033399,-21.8770334769496,
0.));
#223576=CARTESIAN_POINT('Ctrl Pts',(7.63638853033399,-21.8770334769496,
12.));
#223577=CARTESIAN_POINT('Ctrl Pts',(7.63802587492034,-21.8929196523514,
0.));
#223578=CARTESIAN_POINT('Ctrl Pts',(7.63802587492034,-21.8929196523514,
12.));
#223579=CARTESIAN_POINT('Ctrl Pts',(7.63962999860926,-21.9089514909874,
0.));
#223580=CARTESIAN_POINT('Ctrl Pts',(7.63962999860926,-21.9089514909874,
12.));
#223581=CARTESIAN_POINT('Ctrl Pts',(7.64120009506531,-21.9251276046546,
0.));
#223582=CARTESIAN_POINT('Ctrl Pts',(7.64120009506531,-21.9251276046546,
12.));
#223583=CARTESIAN_POINT('Ctrl Pts',(7.64273537442681,-21.9414466292072,
0.));
#223584=CARTESIAN_POINT('Ctrl Pts',(7.64273537442681,-21.9414466292072,
12.));
#223585=CARTESIAN_POINT('Ctrl Pts',(7.64423506279122,-21.9579072237651,
0.));
#223586=CARTESIAN_POINT('Ctrl Pts',(7.64423506279122,-21.9579072237651,
12.));
#223587=CARTESIAN_POINT('Ctrl Pts',(7.64569840177335,-21.9745080700798,
0.));
#223588=CARTESIAN_POINT('Ctrl Pts',(7.64569840177335,-21.9745080700798,
12.));
#223589=CARTESIAN_POINT('Ctrl Pts',(7.64712464805249,-21.9912478718542,
0.));
#223590=CARTESIAN_POINT('Ctrl Pts',(7.64712464805249,-21.9912478718542,
12.));
#223591=CARTESIAN_POINT('Ctrl Pts',(7.64851307293351,-22.0081253540774,
0.));
#223592=CARTESIAN_POINT('Ctrl Pts',(7.64851307293351,-22.0081253540774,
12.));
#223593=CARTESIAN_POINT('Ctrl Pts',(7.64986296190168,-22.0251392623209,
0.));
#223594=CARTESIAN_POINT('Ctrl Pts',(7.64986296190168,-22.0251392623209,
12.));
#223595=CARTESIAN_POINT('Ctrl Pts',(7.65117361421358,-22.0422883621174,
0.));
#223596=CARTESIAN_POINT('Ctrl Pts',(7.65117361421358,-22.0422883621174,
12.));
#223597=CARTESIAN_POINT('Ctrl Pts',(7.65244434253112,-22.0595714384431,
0.));
#223598=CARTESIAN_POINT('Ctrl Pts',(7.65244434253112,-22.0595714384431,
12.));
#223599=CARTESIAN_POINT('Ctrl Pts',(7.65367447254949,-22.0769872951596,
0.));
#223600=CARTESIAN_POINT('Ctrl Pts',(7.65367447254949,-22.0769872951596,
12.));
#223601=CARTESIAN_POINT('Ctrl Pts',(7.65486334263643,-22.094534754469,0.));
#223602=CARTESIAN_POINT('Ctrl Pts',(7.65486334263643,-22.094534754469,12.));
#223603=CARTESIAN_POINT('Ctrl Pts',(7.65601030346806,-22.1122126563329,
0.));
#223604=CARTESIAN_POINT('Ctrl Pts',(7.65601030346806,-22.1122126563329,
12.));
#223605=CARTESIAN_POINT('Ctrl Pts',(7.65711471769396,-22.1300198579675,
0.));
#223606=CARTESIAN_POINT('Ctrl Pts',(7.65711471769396,-22.1300198579675,
12.));
#223607=CARTESIAN_POINT('Ctrl Pts',(7.65817595963348,-22.1479552334211,
0.));
#223608=CARTESIAN_POINT('Ctrl Pts',(7.65817595963348,-22.1479552334211,
12.));
#223609=CARTESIAN_POINT('Ctrl Pts',(7.6591934149693,-22.1660176731178,0.));
#223610=CARTESIAN_POINT('Ctrl Pts',(7.6591934149693,-22.1660176731178,12.));
#223611=CARTESIAN_POINT('Ctrl Pts',(7.66016648045004,-22.1842060834091,
0.));
#223612=CARTESIAN_POINT('Ctrl Pts',(7.66016648045004,-22.1842060834091,
12.));
#223613=CARTESIAN_POINT('Ctrl Pts',(7.6610945635927,-22.2025193860964,0.));
#223614=CARTESIAN_POINT('Ctrl Pts',(7.6610945635927,-22.2025193860964,12.));
#223615=CARTESIAN_POINT('Ctrl Pts',(7.66197708240399,-22.2209565180085,
0.));
#223616=CARTESIAN_POINT('Ctrl Pts',(7.66197708240399,-22.2209565180085,
12.));
#223617=CARTESIAN_POINT('Ctrl Pts',(7.66281346512508,-22.2395164306547,
0.));
#223618=CARTESIAN_POINT('Ctrl Pts',(7.66281346512508,-22.2395164306547,
12.));
#223619=CARTESIAN_POINT('Ctrl Pts',(7.6636031499764,-22.258198089848,0.));
#223620=CARTESIAN_POINT('Ctrl Pts',(7.6636031499764,-22.258198089848,12.));
#223621=CARTESIAN_POINT('Ctrl Pts',(7.66434558490978,-22.2770004753335,
0.));
#223622=CARTESIAN_POINT('Ctrl Pts',(7.66434558490978,-22.2770004753335,
12.));
#223623=CARTESIAN_POINT('Ctrl Pts',(7.66504022736298,-22.2959225803937,
0.));
#223624=CARTESIAN_POINT('Ctrl Pts',(7.66504022736298,-22.2959225803937,
12.));
#223625=CARTESIAN_POINT('Ctrl Pts',(7.66568654402493,-22.314963411484,0.));
#223626=CARTESIAN_POINT('Ctrl Pts',(7.66568654402493,-22.314963411484,12.));
#223627=CARTESIAN_POINT('Ctrl Pts',(7.66628401061951,-22.3341219879469,
0.));
#223628=CARTESIAN_POINT('Ctrl Pts',(7.66628401061951,-22.3341219879469,
12.));
#223629=CARTESIAN_POINT('Ctrl Pts',(7.66683211169157,-22.3533973417021,
0.));
#223630=CARTESIAN_POINT('Ctrl Pts',(7.66683211169157,-22.3533973417021,
12.));
#223631=CARTESIAN_POINT('Ctrl Pts',(7.66733034039882,-22.372788516936,0.));
#223632=CARTESIAN_POINT('Ctrl Pts',(7.66733034039882,-22.372788516936,12.));
#223633=CARTESIAN_POINT('Ctrl Pts',(7.66777819830789,-22.3922945697773,
0.));
#223634=CARTESIAN_POINT('Ctrl Pts',(7.66777819830789,-22.3922945697773,
12.));
#223635=CARTESIAN_POINT('Ctrl Pts',(7.66817519519639,-22.4119145679758,
0.));
#223636=CARTESIAN_POINT('Ctrl Pts',(7.66817519519639,-22.4119145679758,
12.));
#223637=CARTESIAN_POINT('Ctrl Pts',(7.66852084886703,-22.4316475906603,
0.));
#223638=CARTESIAN_POINT('Ctrl Pts',(7.66852084886703,-22.4316475906603,
12.));
#223639=CARTESIAN_POINT('Ctrl Pts',(7.66881468496634,-22.4514927280855,
0.));
#223640=CARTESIAN_POINT('Ctrl Pts',(7.66881468496634,-22.4514927280855,
12.));
#223641=CARTESIAN_POINT('Ctrl Pts',(7.6690562368083,-22.47144908137,0.));
#223642=CARTESIAN_POINT('Ctrl Pts',(7.6690562368083,-22.47144908137,12.));
#223643=CARTESIAN_POINT('Ctrl Pts',(7.66924504520314,-22.4915157622312,
0.));
#223644=CARTESIAN_POINT('Ctrl Pts',(7.66924504520314,-22.4915157622312,
12.));
#223645=CARTESIAN_POINT('Ctrl Pts',(7.66938065829107,-22.5116918927032,
0.));
#223646=CARTESIAN_POINT('Ctrl Pts',(7.66938065829107,-22.5116918927032,
12.));
#223647=CARTESIAN_POINT('Ctrl Pts',(7.66946263138143,-22.53197660492,0.));
#223648=CARTESIAN_POINT('Ctrl Pts',(7.66946263138143,-22.53197660492,12.));
#223649=CARTESIAN_POINT('Ctrl Pts',(7.66949052679692,-22.5523690409116,
0.));
#223650=CARTESIAN_POINT('Ctrl Pts',(7.66949052679692,-22.5523690409116,
12.));
#223651=CARTESIAN_POINT('Ctrl Pts',(7.66946391372305,-22.5728683523831,
0.));
#223652=CARTESIAN_POINT('Ctrl Pts',(7.66946391372305,-22.5728683523831,
12.));
#223653=CARTESIAN_POINT('Ctrl Pts',(7.66938236806232,-22.5934737004953,
0.));
#223654=CARTESIAN_POINT('Ctrl Pts',(7.66938236806232,-22.5934737004953,
12.));
#223655=CARTESIAN_POINT('Ctrl Pts',(7.66924547229413,-22.6141842556243,
0.));
#223656=CARTESIAN_POINT('Ctrl Pts',(7.66924547229413,-22.6141842556243,
12.));
#223657=CARTESIAN_POINT('Ctrl Pts',(7.66905281533714,-22.6349991971541,
0.));
#223658=CARTESIAN_POINT('Ctrl Pts',(7.66905281533714,-22.6349991971541,
12.));
#223659=CARTESIAN_POINT('Ctrl Pts',(7.66880399241322,-22.6559177133127,
0.));
#223660=CARTESIAN_POINT('Ctrl Pts',(7.66880399241322,-22.6559177133127,
12.));
#223661=CARTESIAN_POINT('Ctrl Pts',(7.66849860491742,-22.6769390009885,
0.));
#223662=CARTESIAN_POINT('Ctrl Pts',(7.66849860491742,-22.6769390009885,
12.));
#223663=CARTESIAN_POINT('Ctrl Pts',(7.66813626029274,-22.6980622655446,
0.));
#223664=CARTESIAN_POINT('Ctrl Pts',(7.66813626029274,-22.6980622655446,
12.));
#223665=CARTESIAN_POINT('Ctrl Pts',(7.66771657191027,-22.7192867206245,
0.));
#223666=CARTESIAN_POINT('Ctrl Pts',(7.66771657191027,-22.7192867206245,
12.));
#223667=CARTESIAN_POINT('Ctrl Pts',(7.66723915895439,-22.7406115879513,
0.));
#223668=CARTESIAN_POINT('Ctrl Pts',(7.66723915895439,-22.7406115879513,
12.));
#223669=CARTESIAN_POINT('Ctrl Pts',(7.66670364630298,-22.7620360971843,
0.));
#223670=CARTESIAN_POINT('Ctrl Pts',(7.66670364630298,-22.7620360971843,
12.));
#223671=CARTESIAN_POINT('Ctrl Pts',(7.66610966441272,-22.7835594857699,
0.));
#223672=CARTESIAN_POINT('Ctrl Pts',(7.66610966441272,-22.7835594857699,
12.));
#223673=CARTESIAN_POINT('Ctrl Pts',(7.66545684920986,-22.8051809987833,
0.));
#223674=CARTESIAN_POINT('Ctrl Pts',(7.66545684920986,-22.8051809987833,
12.));
#223675=CARTESIAN_POINT('Ctrl Pts',(7.66474484198548,-22.8268998887678,
0.));
#223676=CARTESIAN_POINT('Ctrl Pts',(7.66474484198548,-22.8268998887678,
12.));
#223677=CARTESIAN_POINT('Ctrl Pts',(7.66397328929802,-22.848715415557,0.));
#223678=CARTESIAN_POINT('Ctrl Pts',(7.66397328929802,-22.848715415557,12.));
#223679=CARTESIAN_POINT('Ctrl Pts',(7.66314184287336,-22.8706268461283,
0.));
#223680=CARTESIAN_POINT('Ctrl Pts',(7.66314184287336,-22.8706268461283,
12.));
#223681=CARTESIAN_POINT('Ctrl Pts',(7.66225015950155,-22.8926334544883,
0.));
#223682=CARTESIAN_POINT('Ctrl Pts',(7.66225015950155,-22.8926334544883,
12.));
#223683=CARTESIAN_POINT('Ctrl Pts',(7.66129790094107,-22.9147345215421,
0.));
#223684=CARTESIAN_POINT('Ctrl Pts',(7.66129790094107,-22.9147345215421,
12.));
#223685=CARTESIAN_POINT('Ctrl Pts',(7.66028473382777,-22.9369293349593,
0.));
#223686=CARTESIAN_POINT('Ctrl Pts',(7.66028473382777,-22.9369293349593,
12.));
#223687=CARTESIAN_POINT('Ctrl Pts',(7.65921032958901,-22.959217189033,0.));
#223688=CARTESIAN_POINT('Ctrl Pts',(7.65921032958901,-22.959217189033,12.));
#223689=CARTESIAN_POINT('Ctrl Pts',(7.65807436436431,-22.9815973845296,
0.));
#223690=CARTESIAN_POINT('Ctrl Pts',(7.65807436436431,-22.9815973845296,
12.));
#223691=CARTESIAN_POINT('Ctrl Pts',(7.65687651891303,-23.0040692285814,
0.));
#223692=CARTESIAN_POINT('Ctrl Pts',(7.65687651891303,-23.0040692285814,
12.));
#223693=CARTESIAN_POINT('Ctrl Pts',(7.65561647852533,-23.0266320345787,
0.));
#223694=CARTESIAN_POINT('Ctrl Pts',(7.65561647852533,-23.0266320345787,
12.));
#223695=CARTESIAN_POINT('Ctrl Pts',(7.65429393293945,-23.0492851220528,
0.));
#223696=CARTESIAN_POINT('Ctrl Pts',(7.65429393293945,-23.0492851220528,
12.));
#223697=CARTESIAN_POINT('Ctrl Pts',(7.65290857626357,-23.072027816555,0.));
#223698=CARTESIAN_POINT('Ctrl Pts',(7.65290857626357,-23.072027816555,12.));
#223699=CARTESIAN_POINT('Ctrl Pts',(7.65146010690475,-23.094859449525,0.));
#223700=CARTESIAN_POINT('Ctrl Pts',(7.65146010690475,-23.094859449525,12.));
#223701=CARTESIAN_POINT('Ctrl Pts',(7.64994822749859,-23.1177793581679,
0.));
#223702=CARTESIAN_POINT('Ctrl Pts',(7.64994822749859,-23.1177793581679,
12.));
#223703=CARTESIAN_POINT('Ctrl Pts',(7.64837264482942,-23.1407868853819,
0.));
#223704=CARTESIAN_POINT('Ctrl Pts',(7.64837264482942,-23.1407868853819,
12.));
#223705=CARTESIAN_POINT('Ctrl Pts',(7.64673306975804,-23.1638813796694,
0.));
#223706=CARTESIAN_POINT('Ctrl Pts',(7.64673306975804,-23.1638813796694,
12.));
#223707=CARTESIAN_POINT('Ctrl Pts',(7.64502921715482,-23.1870621950452,
0.));
#223708=CARTESIAN_POINT('Ctrl Pts',(7.64502921715482,-23.1870621950452,
12.));
#223709=CARTESIAN_POINT('Ctrl Pts',(7.64326080583679,-23.2103286909398,
0.));
#223710=CARTESIAN_POINT('Ctrl Pts',(7.64326080583679,-23.2103286909398,
12.));
#223711=CARTESIAN_POINT('Ctrl Pts',(7.64142755851504,-23.2336802320912,
0.));
#223712=CARTESIAN_POINT('Ctrl Pts',(7.64142755851504,-23.2336802320912,
12.));
#223713=CARTESIAN_POINT('Ctrl Pts',(7.63952920172834,-23.2571161884488,
0.));
#223714=CARTESIAN_POINT('Ctrl Pts',(7.63952920172834,-23.2571161884488,
12.));
#223715=CARTESIAN_POINT('Ctrl Pts',(7.63756546576373,-23.2806359350855,
0.));
#223716=CARTESIAN_POINT('Ctrl Pts',(7.63756546576373,-23.2806359350855,
12.));
#223717=CARTESIAN_POINT('Ctrl Pts',(7.63553608458782,-23.3042388521022,
0.));
#223718=CARTESIAN_POINT('Ctrl Pts',(7.63553608458782,-23.3042388521022,
12.));
#223719=CARTESIAN_POINT('Ctrl Pts',(7.63344079578161,-23.3279243245241,
0.));
#223720=CARTESIAN_POINT('Ctrl Pts',(7.63344079578161,-23.3279243245241,
12.));
#223721=CARTESIAN_POINT('Ctrl Pts',(7.63127934048136,-23.3516917421972,
0.));
#223722=CARTESIAN_POINT('Ctrl Pts',(7.63127934048136,-23.3516917421972,
12.));
#223723=CARTESIAN_POINT('Ctrl Pts',(7.62905146332592,-23.3755404996636,
0.));
#223724=CARTESIAN_POINT('Ctrl Pts',(7.62905146332592,-23.3755404996636,
12.));
#223725=CARTESIAN_POINT('Ctrl Pts',(7.62675691240328,-23.399469996112,0.));
#223726=CARTESIAN_POINT('Ctrl Pts',(7.62675691240328,-23.399469996112,12.));
#223727=CARTESIAN_POINT('Ctrl Pts',(7.62439543920049,-23.4234796353542,
0.));
#223728=CARTESIAN_POINT('Ctrl Pts',(7.62439543920049,-23.4234796353542,
12.));
#223729=CARTESIAN_POINT('Ctrl Pts',(7.62196679855954,-23.4475688257854,
0.));
#223730=CARTESIAN_POINT('Ctrl Pts',(7.62196679855954,-23.4475688257854,
12.));
#223731=CARTESIAN_POINT('Ctrl Pts',(7.61947074863976,-23.4717369803438,
0.));
#223732=CARTESIAN_POINT('Ctrl Pts',(7.61947074863976,-23.4717369803438,
12.));
#223733=CARTESIAN_POINT('Ctrl Pts',(7.61690705088318,-23.4959835164609,
0.));
#223734=CARTESIAN_POINT('Ctrl Pts',(7.61690705088318,-23.4959835164609,
12.));
#223735=CARTESIAN_POINT('Ctrl Pts',(7.61427546999297,-23.5203078560129,
0.));
#223736=CARTESIAN_POINT('Ctrl Pts',(7.61427546999297,-23.5203078560129,
12.));
#223737=CARTESIAN_POINT('Ctrl Pts',(7.61157577385371,-23.544709425203,0.));
#223738=CARTESIAN_POINT('Ctrl Pts',(7.61157577385371,-23.544709425203,12.));
#223739=CARTESIAN_POINT('Ctrl Pts',(7.60880773344599,-23.5691876544244,
0.));
#223740=CARTESIAN_POINT('Ctrl Pts',(7.60880773344599,-23.5691876544244,
12.));
#223741=CARTESIAN_POINT('Ctrl Pts',(7.60597112277093,-23.5937419781245,
0.));
#223742=CARTESIAN_POINT('Ctrl Pts',(7.60597112277093,-23.5937419781245,
12.));
#223743=CARTESIAN_POINT('Ctrl Pts',(7.60306571877805,-23.6183718346576,
0.));
#223744=CARTESIAN_POINT('Ctrl Pts',(7.60306571877805,-23.6183718346576,
12.));
#223745=CARTESIAN_POINT('Ctrl Pts',(7.60009130130125,-23.6430766661418,
0.));
#223746=CARTESIAN_POINT('Ctrl Pts',(7.60009130130125,-23.6430766661418,
12.));
#223747=CARTESIAN_POINT('Ctrl Pts',(7.59704765299566,-23.6678559182875,
0.));
#223748=CARTESIAN_POINT('Ctrl Pts',(7.59704765299566,-23.6678559182875,
12.));
#223749=CARTESIAN_POINT('Ctrl Pts',(7.59393455934034,-23.6927090405066,
0.));
#223750=CARTESIAN_POINT('Ctrl Pts',(7.59393455934034,-23.6927090405066,
12.));
#223751=CARTESIAN_POINT('Ctrl Pts',(7.5907518086532,-23.7176354860457,0.));
#223752=CARTESIAN_POINT('Ctrl Pts',(7.5907518086532,-23.7176354860457,12.));
#223753=CARTESIAN_POINT('Ctrl Pts',(7.58749919210825,-23.7426347121006,
0.));
#223754=CARTESIAN_POINT('Ctrl Pts',(7.58749919210825,-23.7426347121006,
12.));
#223755=CARTESIAN_POINT('Ctrl Pts',(7.5841765037627,-23.7677061799376,0.));
#223756=CARTESIAN_POINT('Ctrl Pts',(7.5841765037627,-23.7677061799376,12.));
#223757=CARTESIAN_POINT('Ctrl Pts',(7.58078354058212,-23.7928493549908,
0.));
#223758=CARTESIAN_POINT('Ctrl Pts',(7.58078354058212,-23.7928493549908,
12.));
#223759=CARTESIAN_POINT('Ctrl Pts',(7.57732010249065,-23.8180637069976,
0.));
#223760=CARTESIAN_POINT('Ctrl Pts',(7.57732010249065,-23.8180637069976,
12.));
#223761=CARTESIAN_POINT('Ctrl Pts',(7.57378599219813,-23.8433487096132,
0.));
#223762=CARTESIAN_POINT('Ctrl Pts',(7.57378599219813,-23.8433487096132,
12.));
#223763=CARTESIAN_POINT('Ctrl Pts',(7.57018101500708,-23.8687038399595,
0.));
#223764=CARTESIAN_POINT('Ctrl Pts',(7.57018101500708,-23.8687038399595,
12.));
#223765=CARTESIAN_POINT('Ctrl Pts',(7.5665049786379,-23.8941285782002,0.));
#223766=CARTESIAN_POINT('Ctrl Pts',(7.5665049786379,-23.8941285782002,12.));
#223767=CARTESIAN_POINT('Ctrl Pts',(7.56275769304772,-23.9196224070759,
0.));
#223768=CARTESIAN_POINT('Ctrl Pts',(7.56275769304772,-23.9196224070759,
12.));
#223769=CARTESIAN_POINT('Ctrl Pts',(7.55893897027679,-23.9451848115002,
0.));
#223770=CARTESIAN_POINT('Ctrl Pts',(7.55893897027679,-23.9451848115002,
12.));
#223771=CARTESIAN_POINT('Ctrl Pts',(7.55504862424807,-23.9708152779886,
0.));
#223772=CARTESIAN_POINT('Ctrl Pts',(7.55504862424807,-23.9708152779886,
12.));
#223773=CARTESIAN_POINT('Ctrl Pts',(7.55108647097431,-23.9965132953187,
0.));
#223774=CARTESIAN_POINT('Ctrl Pts',(7.55108647097431,-23.9965132953187,
12.));
#223775=CARTESIAN_POINT('Ctrl Pts',(7.54705232885894,-24.0222783554531,
0.));
#223776=CARTESIAN_POINT('Ctrl Pts',(7.54705232885894,-24.0222783554531,
12.));
#223777=CARTESIAN_POINT('Ctrl Pts',(7.54294601896127,-24.0481099543353,
0.));
#223778=CARTESIAN_POINT('Ctrl Pts',(7.54294601896127,-24.0481099543353,
12.));
#223779=CARTESIAN_POINT('Ctrl Pts',(7.53876736531004,-24.0740075927984,
0.));
#223780=CARTESIAN_POINT('Ctrl Pts',(7.53876736531004,-24.0740075927984,
12.));
#223781=CARTESIAN_POINT('Ctrl Pts',(7.53451619514658,-24.0999707772643,
0.));
#223782=CARTESIAN_POINT('Ctrl Pts',(7.53451619514658,-24.0999707772643,
12.));
#223783=CARTESIAN_POINT('Ctrl Pts',(7.53019233935536,-24.1259990209211,
0.));
#223784=CARTESIAN_POINT('Ctrl Pts',(7.53019233935536,-24.1259990209211,
12.));
#223785=CARTESIAN_POINT('Ctrl Pts',(7.52579563201478,-24.152091842537,0.));
#223786=CARTESIAN_POINT('Ctrl Pts',(7.52579563201478,-24.152091842537,12.));
#223787=CARTESIAN_POINT('Ctrl Pts',(7.52132590953862,-24.1782487641602,
0.));
#223788=CARTESIAN_POINT('Ctrl Pts',(7.52132590953862,-24.1782487641602,
12.));
#223789=CARTESIAN_POINT('Ctrl Pts',(7.51678300997997,-24.2044693092356,
0.));
#223790=CARTESIAN_POINT('Ctrl Pts',(7.51678300997997,-24.2044693092356,
12.));
#223791=CARTESIAN_POINT('Ctrl Pts',(7.51216677222198,-24.230753000389,0.));
#223792=CARTESIAN_POINT('Ctrl Pts',(7.51216677222198,-24.230753000389,12.));
#223793=CARTESIAN_POINT('Ctrl Pts',(7.50747703535114,-24.2570993577032,
0.));
#223794=CARTESIAN_POINT('Ctrl Pts',(7.50747703535114,-24.2570993577032,
12.));
#223795=CARTESIAN_POINT('Ctrl Pts',(7.50271363765098,-24.2835078958966,
0.));
#223796=CARTESIAN_POINT('Ctrl Pts',(7.50271363765098,-24.2835078958966,
12.));
#223797=CARTESIAN_POINT('Ctrl Pts',(7.49787641695358,-24.3099781253345,
0.));
#223798=CARTESIAN_POINT('Ctrl Pts',(7.49787641695358,-24.3099781253345,
12.));
#223799=CARTESIAN_POINT('Ctrl Pts',(7.49296521252329,-24.3365095573673,
0.));
#223800=CARTESIAN_POINT('Ctrl Pts',(7.49296521252329,-24.3365095573673,
12.));
#223801=CARTESIAN_POINT('Ctrl Pts',(7.48797986651827,-24.3631017084513,
0.));
#223802=CARTESIAN_POINT('Ctrl Pts',(7.48797986651827,-24.3631017084513,
12.));
#223803=CARTESIAN_POINT('Ctrl Pts',(7.48292022569253,-24.3897541049248,
0.));
#223804=CARTESIAN_POINT('Ctrl Pts',(7.48292022569253,-24.3897541049248,
12.));
#223805=CARTESIAN_POINT('Ctrl Pts',(7.47778614286572,-24.4164662871165,
0.));
#223806=CARTESIAN_POINT('Ctrl Pts',(7.47778614286572,-24.4164662871165,
12.));
#223807=CARTESIAN_POINT('Ctrl Pts',(7.47257747883318,-24.4432378146501,
0.));
#223808=CARTESIAN_POINT('Ctrl Pts',(7.47257747883318,-24.4432378146501,
12.));
#223809=CARTESIAN_POINT('Ctrl Pts',(7.46729410308922,-24.4700682684544,
0.));
#223810=CARTESIAN_POINT('Ctrl Pts',(7.46729410308922,-24.4700682684544,
12.));
#223811=CARTESIAN_POINT('Ctrl Pts',(7.46193588961641,-24.4969572391509,
0.));
#223812=CARTESIAN_POINT('Ctrl Pts',(7.46193588961641,-24.4969572391509,
12.));
#223813=CARTESIAN_POINT('Ctrl Pts',(7.45650271336044,-24.52390431731,0.));
#223814=CARTESIAN_POINT('Ctrl Pts',(7.45650271336044,-24.52390431731,12.));
#223815=CARTESIAN_POINT('Ctrl Pts',(7.45099444651295,-24.550909083158,0.));
#223816=CARTESIAN_POINT('Ctrl Pts',(7.45099444651295,-24.550909083158,12.));
#223817=CARTESIAN_POINT('Ctrl Pts',(7.44541095473162,-24.5779710960865,
0.));
#223818=CARTESIAN_POINT('Ctrl Pts',(7.44541095473162,-24.5779710960865,
12.));
#223819=CARTESIAN_POINT('Ctrl Pts',(7.43975209375374,-24.6050898852349,
0.));
#223820=CARTESIAN_POINT('Ctrl Pts',(7.43975209375374,-24.6050898852349,
12.));
#223821=CARTESIAN_POINT('Ctrl Pts',(7.4340177048922,-24.6322649369472,0.));
#223822=CARTESIAN_POINT('Ctrl Pts',(7.4340177048922,-24.6322649369472,12.));
#223823=CARTESIAN_POINT('Ctrl Pts',(7.4282076215868,-24.659495712869,0.));
#223824=CARTESIAN_POINT('Ctrl Pts',(7.4282076215868,-24.659495712869,12.));
#223825=CARTESIAN_POINT('Ctrl Pts',(7.42232167765762,-24.6867816727118,
0.));
#223826=CARTESIAN_POINT('Ctrl Pts',(7.42232167765762,-24.6867816727118,
12.));
#223827=CARTESIAN_POINT('Ctrl Pts',(7.41635971481242,-24.7141222949988,
0.));
#223828=CARTESIAN_POINT('Ctrl Pts',(7.41635971481242,-24.7141222949988,
12.));
#223829=CARTESIAN_POINT('Ctrl Pts',(7.41032159082172,-24.7415170994754,
0.));
#223830=CARTESIAN_POINT('Ctrl Pts',(7.41032159082172,-24.7415170994754,
12.));
#223831=CARTESIAN_POINT('Ctrl Pts',(7.40420718661754,-24.7689656669005,
0.));
#223832=CARTESIAN_POINT('Ctrl Pts',(7.40420718661754,-24.7689656669005,
12.));
#223833=CARTESIAN_POINT('Ctrl Pts',(7.39801641583612,-24.7964676646518,
0.));
#223834=CARTESIAN_POINT('Ctrl Pts',(7.39801641583612,-24.7964676646518,
12.));
#223835=CARTESIAN_POINT('Ctrl Pts',(7.3917492258684,-24.8240228521042,0.));
#223836=CARTESIAN_POINT('Ctrl Pts',(7.3917492258684,-24.8240228521042,12.));
#223837=CARTESIAN_POINT('Ctrl Pts',(7.38540558904945,-24.8516310625367,
0.));
#223838=CARTESIAN_POINT('Ctrl Pts',(7.38540558904945,-24.8516310625367,
12.));
#223839=CARTESIAN_POINT('Ctrl Pts',(7.37898549641609,-24.8792921911309,
0.));
#223840=CARTESIAN_POINT('Ctrl Pts',(7.37898549641609,-24.8792921911309,
12.));
#223841=CARTESIAN_POINT('Ctrl Pts',(7.37378825962717,-24.9014633826201,
0.));
#223842=CARTESIAN_POINT('Ctrl Pts',(7.37378825962717,-24.9014633826201,
12.));
#223843=CARTESIAN_POINT('Ctrl Pts',(7.36985593120695,-24.9181155530631,
0.));
#223844=CARTESIAN_POINT('Ctrl Pts',(7.36985593120695,-24.9181155530631,
12.));
#223845=CARTESIAN_POINT('Ctrl Pts',(7.36721909029059,-24.9292275670705,
0.));
#223846=CARTESIAN_POINT('Ctrl Pts',(7.36721909029059,-24.9292275670705,
12.));
#223847=CARTESIAN_POINT('Ctrl Pts',(7.36589684767343,-24.9347862158358,
0.));
#223848=CARTESIAN_POINT('Ctrl Pts',(7.36589684767343,-24.9347862158358,
12.));
#223849=CARTESIAN_POINT('',(7.36589684767343,-24.9347862158358,0.));
#223850=CARTESIAN_POINT('Ctrl Pts',(7.52250298901263,-21.2610617890679,
0.));
#223851=CARTESIAN_POINT('Ctrl Pts',(7.52250649703969,-21.2610673466886,
0.));
#223852=CARTESIAN_POINT('Ctrl Pts',(7.52252744144903,-21.2611204474866,
0.));
#223853=CARTESIAN_POINT('Ctrl Pts',(7.5226006423166,-21.261326054066,0.));
#223854=CARTESIAN_POINT('Ctrl Pts',(7.52278182242669,-21.2618521283555,
0.));
#223855=CARTESIAN_POINT('Ctrl Pts',(7.52314642316199,-21.262927782038,0.));
#223856=CARTESIAN_POINT('Ctrl Pts',(7.52364573027552,-21.2644161259962,
0.));
#223857=CARTESIAN_POINT('Ctrl Pts',(7.52427261074297,-21.2663059157058,
0.));
#223858=CARTESIAN_POINT('Ctrl Pts',(7.5250177033353,-21.2685823838671,0.));
#223859=CARTESIAN_POINT('Ctrl Pts',(7.52587126095529,-21.2712301573466,
0.));
#223860=CARTESIAN_POINT('Ctrl Pts',(7.5268252691854,-21.2742366113579,0.));
#223861=CARTESIAN_POINT('Ctrl Pts',(7.52787386225332,-21.2775925269652,
0.));
#223862=CARTESIAN_POINT('Ctrl Pts',(7.52901217930407,-21.2812902781143,
0.));
#223863=CARTESIAN_POINT('Ctrl Pts',(7.53023562438229,-21.2853226580657,
0.));
#223864=CARTESIAN_POINT('Ctrl Pts',(7.53153906987855,-21.2896816163842,
0.));
#223865=CARTESIAN_POINT('Ctrl Pts',(7.53291726078526,-21.2943588989331,
0.));
#223866=CARTESIAN_POINT('Ctrl Pts',(7.53436505309942,-21.2993464250717,
0.));
#223867=CARTESIAN_POINT('Ctrl Pts',(7.53587778251735,-21.3046368712157,
0.));
#223868=CARTESIAN_POINT('Ctrl Pts',(7.53745129364615,-21.310223716773,0.));
#223869=CARTESIAN_POINT('Ctrl Pts',(7.53908175169898,-21.3161009456256,
0.));
#223870=CARTESIAN_POINT('Ctrl Pts',(7.54076552038278,-21.3222628524165,
0.));
#223871=CARTESIAN_POINT('Ctrl Pts',(7.5424990037703,-21.328703791771,0.));
#223872=CARTESIAN_POINT('Ctrl Pts',(7.54427868151267,-21.3354182340149,
0.));
#223873=CARTESIAN_POINT('Ctrl Pts',(7.54610114948346,-21.3424008295038,
0.));
#223874=CARTESIAN_POINT('Ctrl Pts',(7.5479631624633,-21.3496464761531,0.));
#223875=CARTESIAN_POINT('Ctrl Pts',(7.54986166521309,-21.3571503685855,
0.));
#223876=CARTESIAN_POINT('Ctrl Pts',(7.55179375777443,-21.3649079431865,
0.));
#223877=CARTESIAN_POINT('Ctrl Pts',(7.55375667080028,-21.3729148390243,
0.));
#223878=CARTESIAN_POINT('Ctrl Pts',(7.55574773403502,-21.3811668478932,
0.));
#223879=CARTESIAN_POINT('Ctrl Pts',(7.55776435731416,-21.3896598842117,
0.));
#223880=CARTESIAN_POINT('Ctrl Pts',(7.5598040370061,-21.3983899952987,0.));
#223881=CARTESIAN_POINT('Ctrl Pts',(7.56186435703621,-21.4073533630365,
0.));
#223882=CARTESIAN_POINT('Ctrl Pts',(7.56394299313684,-21.4165463106254,
0.));
#223883=CARTESIAN_POINT('Ctrl Pts',(7.56603771218711,-21.4259653015736,
0.));
#223884=CARTESIAN_POINT('Ctrl Pts',(7.56814636360847,-21.4356069261513,
0.));
#223885=CARTESIAN_POINT('Ctrl Pts',(7.57026687261165,-21.4454678907509,
0.));
#223886=CARTESIAN_POINT('Ctrl Pts',(7.57239723223505,-21.4555450053142,
0.));
#223887=CARTESIAN_POINT('Ctrl Pts',(7.57453549743411,-21.4658351740128,
0.));
#223888=CARTESIAN_POINT('Ctrl Pts',(7.57667978402986,-21.4763353936762,
0.));
#223889=CARTESIAN_POINT('Ctrl Pts',(7.57882826679131,-21.4870427508194,
0.));
#223890=CARTESIAN_POINT('Ctrl Pts',(7.58097917790743,-21.4979544192744,
0.));
#223891=CARTESIAN_POINT('Ctrl Pts',(7.58313080519179,-21.5090676573873,
0.));
#223892=CARTESIAN_POINT('Ctrl Pts',(7.58528148919129,-21.5203798035299,
0.));
#223893=CARTESIAN_POINT('Ctrl Pts',(7.58742962034833,-21.5318882716736,
0.));
#223894=CARTESIAN_POINT('Ctrl Pts',(7.58957363620013,-21.543590547011,0.));
#223895=CARTESIAN_POINT('Ctrl Pts',(7.59171201844776,-21.5554841813462,
0.));
#223896=CARTESIAN_POINT('Ctrl Pts',(7.59384329124918,-21.5675667904726,
0.));
#223897=CARTESIAN_POINT('Ctrl Pts',(7.59596601973583,-21.5798360518978,
0.));
#223898=CARTESIAN_POINT('Ctrl Pts',(7.59807880846194,-21.5922897024466,
0.));
#223899=CARTESIAN_POINT('Ctrl Pts',(7.6001802998824,-21.6049255358843,0.));
#223900=CARTESIAN_POINT('Ctrl Pts',(7.60226917285428,-21.617741400599,0.));
#223901=CARTESIAN_POINT('Ctrl Pts',(7.60434414118295,-21.6307351973822,
0.));
#223902=CARTESIAN_POINT('Ctrl Pts',(7.60640395216356,-21.6439048771743,
0.));
#223903=CARTESIAN_POINT('Ctrl Pts',(7.60844738512873,-21.6572484388081,
0.));
#223904=CARTESIAN_POINT('Ctrl Pts',(7.61047325000955,-21.6707639267576,
0.));
#223905=CARTESIAN_POINT('Ctrl Pts',(7.61248038630268,-21.6844494295815,
0.));
#223906=CARTESIAN_POINT('Ctrl Pts',(7.61446766202786,-21.6983030783322,
0.));
#223907=CARTESIAN_POINT('Ctrl Pts',(7.6164339727042,-21.7123230449834,0.));
#223908=CARTESIAN_POINT('Ctrl Pts',(7.61837824030537,-21.7265075407975,
0.));
#223909=CARTESIAN_POINT('Ctrl Pts',(7.62029941230854,-21.7408548148656,
0.));
#223910=CARTESIAN_POINT('Ctrl Pts',(7.62219646084228,-21.7553631528328,
0.));
#223911=CARTESIAN_POINT('Ctrl Pts',(7.62406838181165,-21.7700308755584,
0.));
#223912=CARTESIAN_POINT('Ctrl Pts',(7.62591419404512,-21.7848563378021,
0.));
#223913=CARTESIAN_POINT('Ctrl Pts',(7.62773293842388,-21.799837926858,0.));
#223914=CARTESIAN_POINT('Ctrl Pts',(7.62952367718126,-21.814974061509,0.));
#223915=CARTESIAN_POINT('Ctrl Pts',(7.63128549323022,-21.8302631910195,
0.));
#223916=CARTESIAN_POINT('Ctrl Pts',(7.63301748948935,-21.8457037941084,
0.));
#223917=CARTESIAN_POINT('Ctrl Pts',(7.63471878821225,-21.8612943779089,
0.));
#223918=CARTESIAN_POINT('Ctrl Pts',(7.63638853033399,-21.8770334769496,
0.));
#223919=CARTESIAN_POINT('Ctrl Pts',(7.63802587492034,-21.8929196523514,
0.));
#223920=CARTESIAN_POINT('Ctrl Pts',(7.63962999860926,-21.9089514909874,
0.));
#223921=CARTESIAN_POINT('Ctrl Pts',(7.64120009506531,-21.9251276046546,
0.));
#223922=CARTESIAN_POINT('Ctrl Pts',(7.64273537442681,-21.9414466292072,
0.));
#223923=CARTESIAN_POINT('Ctrl Pts',(7.64423506279122,-21.9579072237651,
0.));
#223924=CARTESIAN_POINT('Ctrl Pts',(7.64569840177335,-21.9745080700798,
0.));
#223925=CARTESIAN_POINT('Ctrl Pts',(7.64712464805249,-21.9912478718542,
0.));
#223926=CARTESIAN_POINT('Ctrl Pts',(7.64851307293351,-22.0081253540774,
0.));
#223927=CARTESIAN_POINT('Ctrl Pts',(7.64986296190168,-22.0251392623209,
0.));
#223928=CARTESIAN_POINT('Ctrl Pts',(7.65117361421358,-22.0422883621174,
0.));
#223929=CARTESIAN_POINT('Ctrl Pts',(7.65244434253112,-22.0595714384431,
0.));
#223930=CARTESIAN_POINT('Ctrl Pts',(7.65367447254949,-22.0769872951596,
0.));
#223931=CARTESIAN_POINT('Ctrl Pts',(7.65486334263643,-22.094534754469,0.));
#223932=CARTESIAN_POINT('Ctrl Pts',(7.65601030346806,-22.1122126563329,
0.));
#223933=CARTESIAN_POINT('Ctrl Pts',(7.65711471769396,-22.1300198579675,
0.));
#223934=CARTESIAN_POINT('Ctrl Pts',(7.65817595963348,-22.1479552334211,
0.));
#223935=CARTESIAN_POINT('Ctrl Pts',(7.6591934149693,-22.1660176731178,0.));
#223936=CARTESIAN_POINT('Ctrl Pts',(7.66016648045004,-22.1842060834091,
0.));
#223937=CARTESIAN_POINT('Ctrl Pts',(7.6610945635927,-22.2025193860964,0.));
#223938=CARTESIAN_POINT('Ctrl Pts',(7.66197708240399,-22.2209565180085,
0.));
#223939=CARTESIAN_POINT('Ctrl Pts',(7.66281346512508,-22.2395164306547,
0.));
#223940=CARTESIAN_POINT('Ctrl Pts',(7.6636031499764,-22.258198089848,0.));
#223941=CARTESIAN_POINT('Ctrl Pts',(7.66434558490978,-22.2770004753335,
0.));
#223942=CARTESIAN_POINT('Ctrl Pts',(7.66504022736298,-22.2959225803937,
0.));
#223943=CARTESIAN_POINT('Ctrl Pts',(7.66568654402493,-22.314963411484,0.));
#223944=CARTESIAN_POINT('Ctrl Pts',(7.66628401061951,-22.3341219879469,
0.));
#223945=CARTESIAN_POINT('Ctrl Pts',(7.66683211169157,-22.3533973417021,
0.));
#223946=CARTESIAN_POINT('Ctrl Pts',(7.66733034039882,-22.372788516936,0.));
#223947=CARTESIAN_POINT('Ctrl Pts',(7.66777819830789,-22.3922945697773,
0.));
#223948=CARTESIAN_POINT('Ctrl Pts',(7.66817519519639,-22.4119145679758,
0.));
#223949=CARTESIAN_POINT('Ctrl Pts',(7.66852084886703,-22.4316475906603,
0.));
#223950=CARTESIAN_POINT('Ctrl Pts',(7.66881468496634,-22.4514927280855,
0.));
#223951=CARTESIAN_POINT('Ctrl Pts',(7.6690562368083,-22.47144908137,0.));
#223952=CARTESIAN_POINT('Ctrl Pts',(7.66924504520314,-22.4915157622312,
0.));
#223953=CARTESIAN_POINT('Ctrl Pts',(7.66938065829107,-22.5116918927032,
0.));
#223954=CARTESIAN_POINT('Ctrl Pts',(7.66946263138143,-22.53197660492,0.));
#223955=CARTESIAN_POINT('Ctrl Pts',(7.66949052679692,-22.5523690409116,
0.));
#223956=CARTESIAN_POINT('Ctrl Pts',(7.66946391372305,-22.5728683523831,
0.));
#223957=CARTESIAN_POINT('Ctrl Pts',(7.66938236806232,-22.5934737004953,
0.));
#223958=CARTESIAN_POINT('Ctrl Pts',(7.66924547229413,-22.6141842556243,
0.));
#223959=CARTESIAN_POINT('Ctrl Pts',(7.66905281533714,-22.6349991971541,
0.));
#223960=CARTESIAN_POINT('Ctrl Pts',(7.66880399241322,-22.6559177133127,
0.));
#223961=CARTESIAN_POINT('Ctrl Pts',(7.66849860491742,-22.6769390009885,
0.));
#223962=CARTESIAN_POINT('Ctrl Pts',(7.66813626029274,-22.6980622655446,
0.));
#223963=CARTESIAN_POINT('Ctrl Pts',(7.66771657191027,-22.7192867206245,
0.));
#223964=CARTESIAN_POINT('Ctrl Pts',(7.66723915895439,-22.7406115879513,
0.));
#223965=CARTESIAN_POINT('Ctrl Pts',(7.66670364630298,-22.7620360971843,
0.));
#223966=CARTESIAN_POINT('Ctrl Pts',(7.66610966441272,-22.7835594857699,
0.));
#223967=CARTESIAN_POINT('Ctrl Pts',(7.66545684920986,-22.8051809987833,
0.));
#223968=CARTESIAN_POINT('Ctrl Pts',(7.66474484198548,-22.8268998887678,
0.));
#223969=CARTESIAN_POINT('Ctrl Pts',(7.66397328929802,-22.848715415557,0.));
#223970=CARTESIAN_POINT('Ctrl Pts',(7.66314184287336,-22.8706268461283,
0.));
#223971=CARTESIAN_POINT('Ctrl Pts',(7.66225015950155,-22.8926334544883,
0.));
#223972=CARTESIAN_POINT('Ctrl Pts',(7.66129790094107,-22.9147345215421,
0.));
#223973=CARTESIAN_POINT('Ctrl Pts',(7.66028473382777,-22.9369293349593,
0.));
#223974=CARTESIAN_POINT('Ctrl Pts',(7.65921032958901,-22.959217189033,0.));
#223975=CARTESIAN_POINT('Ctrl Pts',(7.65807436436431,-22.9815973845296,
0.));
#223976=CARTESIAN_POINT('Ctrl Pts',(7.65687651891303,-23.0040692285814,
0.));
#223977=CARTESIAN_POINT('Ctrl Pts',(7.65561647852533,-23.0266320345787,
0.));
#223978=CARTESIAN_POINT('Ctrl Pts',(7.65429393293945,-23.0492851220528,
0.));
#223979=CARTESIAN_POINT('Ctrl Pts',(7.65290857626357,-23.072027816555,0.));
#223980=CARTESIAN_POINT('Ctrl Pts',(7.65146010690475,-23.094859449525,0.));
#223981=CARTESIAN_POINT('Ctrl Pts',(7.64994822749859,-23.1177793581679,
0.));
#223982=CARTESIAN_POINT('Ctrl Pts',(7.64837264482942,-23.1407868853819,
0.));
#223983=CARTESIAN_POINT('Ctrl Pts',(7.64673306975804,-23.1638813796694,
0.));
#223984=CARTESIAN_POINT('Ctrl Pts',(7.64502921715482,-23.1870621950452,
0.));
#223985=CARTESIAN_POINT('Ctrl Pts',(7.64326080583679,-23.2103286909398,
0.));
#223986=CARTESIAN_POINT('Ctrl Pts',(7.64142755851504,-23.2336802320912,
0.));
#223987=CARTESIAN_POINT('Ctrl Pts',(7.63952920172834,-23.2571161884488,
0.));
#223988=CARTESIAN_POINT('Ctrl Pts',(7.63756546576373,-23.2806359350855,
0.));
#223989=CARTESIAN_POINT('Ctrl Pts',(7.63553608458782,-23.3042388521022,
0.));
#223990=CARTESIAN_POINT('Ctrl Pts',(7.63344079578161,-23.3279243245241,
0.));
#223991=CARTESIAN_POINT('Ctrl Pts',(7.63127934048136,-23.3516917421972,
0.));
#223992=CARTESIAN_POINT('Ctrl Pts',(7.62905146332592,-23.3755404996636,
0.));
#223993=CARTESIAN_POINT('Ctrl Pts',(7.62675691240328,-23.399469996112,0.));
#223994=CARTESIAN_POINT('Ctrl Pts',(7.62439543920049,-23.4234796353542,
0.));
#223995=CARTESIAN_POINT('Ctrl Pts',(7.62196679855954,-23.4475688257854,
0.));
#223996=CARTESIAN_POINT('Ctrl Pts',(7.61947074863976,-23.4717369803438,
0.));
#223997=CARTESIAN_POINT('Ctrl Pts',(7.61690705088318,-23.4959835164609,
0.));
#223998=CARTESIAN_POINT('Ctrl Pts',(7.61427546999297,-23.5203078560129,
0.));
#223999=CARTESIAN_POINT('Ctrl Pts',(7.61157577385371,-23.544709425203,0.));
#224000=CARTESIAN_POINT('Ctrl Pts',(7.60880773344599,-23.5691876544244,
0.));
#224001=CARTESIAN_POINT('Ctrl Pts',(7.60597112277093,-23.5937419781245,
0.));
#224002=CARTESIAN_POINT('Ctrl Pts',(7.60306571877805,-23.6183718346576,
0.));
#224003=CARTESIAN_POINT('Ctrl Pts',(7.60009130130125,-23.6430766661418,
0.));
#224004=CARTESIAN_POINT('Ctrl Pts',(7.59704765299566,-23.6678559182875,
0.));
#224005=CARTESIAN_POINT('Ctrl Pts',(7.59393455934034,-23.6927090405066,
0.));
#224006=CARTESIAN_POINT('Ctrl Pts',(7.5907518086532,-23.7176354860457,0.));
#224007=CARTESIAN_POINT('Ctrl Pts',(7.58749919210825,-23.7426347121006,
0.));
#224008=CARTESIAN_POINT('Ctrl Pts',(7.5841765037627,-23.7677061799376,0.));
#224009=CARTESIAN_POINT('Ctrl Pts',(7.58078354058212,-23.7928493549908,
0.));
#224010=CARTESIAN_POINT('Ctrl Pts',(7.57732010249065,-23.8180637069976,
0.));
#224011=CARTESIAN_POINT('Ctrl Pts',(7.57378599219813,-23.8433487096132,
0.));
#224012=CARTESIAN_POINT('Ctrl Pts',(7.57018101500708,-23.8687038399595,
0.));
#224013=CARTESIAN_POINT('Ctrl Pts',(7.5665049786379,-23.8941285782002,0.));
#224014=CARTESIAN_POINT('Ctrl Pts',(7.56275769304772,-23.9196224070759,
0.));
#224015=CARTESIAN_POINT('Ctrl Pts',(7.55893897027679,-23.9451848115002,
0.));
#224016=CARTESIAN_POINT('Ctrl Pts',(7.55504862424807,-23.9708152779886,
0.));
#224017=CARTESIAN_POINT('Ctrl Pts',(7.55108647097431,-23.9965132953187,
0.));
#224018=CARTESIAN_POINT('Ctrl Pts',(7.54705232885894,-24.0222783554531,
0.));
#224019=CARTESIAN_POINT('Ctrl Pts',(7.54294601896127,-24.0481099543353,
0.));
#224020=CARTESIAN_POINT('Ctrl Pts',(7.53876736531004,-24.0740075927984,
0.));
#224021=CARTESIAN_POINT('Ctrl Pts',(7.53451619514658,-24.0999707772643,
0.));
#224022=CARTESIAN_POINT('Ctrl Pts',(7.53019233935536,-24.1259990209211,
0.));
#224023=CARTESIAN_POINT('Ctrl Pts',(7.52579563201478,-24.152091842537,0.));
#224024=CARTESIAN_POINT('Ctrl Pts',(7.52132590953862,-24.1782487641602,
0.));
#224025=CARTESIAN_POINT('Ctrl Pts',(7.51678300997997,-24.2044693092356,
0.));
#224026=CARTESIAN_POINT('Ctrl Pts',(7.51216677222198,-24.230753000389,0.));
#224027=CARTESIAN_POINT('Ctrl Pts',(7.50747703535114,-24.2570993577032,
0.));
#224028=CARTESIAN_POINT('Ctrl Pts',(7.50271363765098,-24.2835078958966,
0.));
#224029=CARTESIAN_POINT('Ctrl Pts',(7.49787641695358,-24.3099781253345,
0.));
#224030=CARTESIAN_POINT('Ctrl Pts',(7.49296521252329,-24.3365095573673,
0.));
#224031=CARTESIAN_POINT('Ctrl Pts',(7.48797986651827,-24.3631017084513,
0.));
#224032=CARTESIAN_POINT('Ctrl Pts',(7.48292022569253,-24.3897541049248,
0.));
#224033=CARTESIAN_POINT('Ctrl Pts',(7.47778614286572,-24.4164662871165,
0.));
#224034=CARTESIAN_POINT('Ctrl Pts',(7.47257747883318,-24.4432378146501,
0.));
#224035=CARTESIAN_POINT('Ctrl Pts',(7.46729410308922,-24.4700682684544,
0.));
#224036=CARTESIAN_POINT('Ctrl Pts',(7.46193588961641,-24.4969572391509,
0.));
#224037=CARTESIAN_POINT('Ctrl Pts',(7.45650271336044,-24.52390431731,0.));
#224038=CARTESIAN_POINT('Ctrl Pts',(7.45099444651295,-24.550909083158,0.));
#224039=CARTESIAN_POINT('Ctrl Pts',(7.44541095473162,-24.5779710960865,
0.));
#224040=CARTESIAN_POINT('Ctrl Pts',(7.43975209375374,-24.6050898852349,
0.));
#224041=CARTESIAN_POINT('Ctrl Pts',(7.4340177048922,-24.6322649369472,0.));
#224042=CARTESIAN_POINT('Ctrl Pts',(7.4282076215868,-24.659495712869,0.));
#224043=CARTESIAN_POINT('Ctrl Pts',(7.42232167765762,-24.6867816727118,
0.));
#224044=CARTESIAN_POINT('Ctrl Pts',(7.41635971481242,-24.7141222949988,
0.));
#224045=CARTESIAN_POINT('Ctrl Pts',(7.41032159082172,-24.7415170994754,
0.));
#224046=CARTESIAN_POINT('Ctrl Pts',(7.40420718661754,-24.7689656669005,
0.));
#224047=CARTESIAN_POINT('Ctrl Pts',(7.39801641583612,-24.7964676646518,
0.));
#224048=CARTESIAN_POINT('Ctrl Pts',(7.3917492258684,-24.8240228521042,0.));
#224049=CARTESIAN_POINT('Ctrl Pts',(7.38540558904945,-24.8516310625367,
0.));
#224050=CARTESIAN_POINT('Ctrl Pts',(7.37898549641609,-24.8792921911309,
0.));
#224051=CARTESIAN_POINT('Ctrl Pts',(7.37378825962717,-24.9014633826201,
0.));
#224052=CARTESIAN_POINT('Ctrl Pts',(7.36985593120695,-24.9181155530631,
0.));
#224053=CARTESIAN_POINT('Ctrl Pts',(7.36721909029059,-24.9292275670705,
0.));
#224054=CARTESIAN_POINT('Ctrl Pts',(7.36589684767343,-24.9347862158358,
0.));
#224055=CARTESIAN_POINT('',(7.36589684767343,-24.9347862158358,12.));
#224056=CARTESIAN_POINT('Ctrl Pts',(7.36589684767343,-24.9347862158358,
12.));
#224057=CARTESIAN_POINT('Ctrl Pts',(7.36721909029059,-24.9292275670705,
12.));
#224058=CARTESIAN_POINT('Ctrl Pts',(7.36985593120695,-24.9181155530631,
12.));
#224059=CARTESIAN_POINT('Ctrl Pts',(7.37378825962717,-24.9014633826201,
12.));
#224060=CARTESIAN_POINT('Ctrl Pts',(7.37898549641609,-24.8792921911309,
12.));
#224061=CARTESIAN_POINT('Ctrl Pts',(7.38540558904945,-24.8516310625367,
12.));
#224062=CARTESIAN_POINT('Ctrl Pts',(7.3917492258684,-24.8240228521042,12.));
#224063=CARTESIAN_POINT('Ctrl Pts',(7.39801641583612,-24.7964676646518,
12.));
#224064=CARTESIAN_POINT('Ctrl Pts',(7.40420718661754,-24.7689656669005,
12.));
#224065=CARTESIAN_POINT('Ctrl Pts',(7.41032159082172,-24.7415170994754,
12.));
#224066=CARTESIAN_POINT('Ctrl Pts',(7.41635971481242,-24.7141222949988,
12.));
#224067=CARTESIAN_POINT('Ctrl Pts',(7.42232167765762,-24.6867816727118,
12.));
#224068=CARTESIAN_POINT('Ctrl Pts',(7.4282076215868,-24.659495712869,12.));
#224069=CARTESIAN_POINT('Ctrl Pts',(7.4340177048922,-24.6322649369472,12.));
#224070=CARTESIAN_POINT('Ctrl Pts',(7.43975209375374,-24.6050898852349,
12.));
#224071=CARTESIAN_POINT('Ctrl Pts',(7.44541095473162,-24.5779710960865,
12.));
#224072=CARTESIAN_POINT('Ctrl Pts',(7.45099444651295,-24.550909083158,12.));
#224073=CARTESIAN_POINT('Ctrl Pts',(7.45650271336044,-24.52390431731,12.));
#224074=CARTESIAN_POINT('Ctrl Pts',(7.46193588961641,-24.4969572391509,
12.));
#224075=CARTESIAN_POINT('Ctrl Pts',(7.46729410308922,-24.4700682684544,
12.));
#224076=CARTESIAN_POINT('Ctrl Pts',(7.47257747883318,-24.4432378146501,
12.));
#224077=CARTESIAN_POINT('Ctrl Pts',(7.47778614286572,-24.4164662871165,
12.));
#224078=CARTESIAN_POINT('Ctrl Pts',(7.48292022569253,-24.3897541049248,
12.));
#224079=CARTESIAN_POINT('Ctrl Pts',(7.48797986651827,-24.3631017084513,
12.));
#224080=CARTESIAN_POINT('Ctrl Pts',(7.49296521252329,-24.3365095573673,
12.));
#224081=CARTESIAN_POINT('Ctrl Pts',(7.49787641695358,-24.3099781253345,
12.));
#224082=CARTESIAN_POINT('Ctrl Pts',(7.50271363765098,-24.2835078958966,
12.));
#224083=CARTESIAN_POINT('Ctrl Pts',(7.50747703535114,-24.2570993577032,
12.));
#224084=CARTESIAN_POINT('Ctrl Pts',(7.51216677222198,-24.230753000389,12.));
#224085=CARTESIAN_POINT('Ctrl Pts',(7.51678300997997,-24.2044693092356,
12.));
#224086=CARTESIAN_POINT('Ctrl Pts',(7.52132590953862,-24.1782487641602,
12.));
#224087=CARTESIAN_POINT('Ctrl Pts',(7.52579563201478,-24.152091842537,12.));
#224088=CARTESIAN_POINT('Ctrl Pts',(7.53019233935536,-24.1259990209211,
12.));
#224089=CARTESIAN_POINT('Ctrl Pts',(7.53451619514658,-24.0999707772643,
12.));
#224090=CARTESIAN_POINT('Ctrl Pts',(7.53876736531004,-24.0740075927984,
12.));
#224091=CARTESIAN_POINT('Ctrl Pts',(7.54294601896127,-24.0481099543353,
12.));
#224092=CARTESIAN_POINT('Ctrl Pts',(7.54705232885894,-24.0222783554531,
12.));
#224093=CARTESIAN_POINT('Ctrl Pts',(7.55108647097431,-23.9965132953187,
12.));
#224094=CARTESIAN_POINT('Ctrl Pts',(7.55504862424807,-23.9708152779886,
12.));
#224095=CARTESIAN_POINT('Ctrl Pts',(7.55893897027679,-23.9451848115002,
12.));
#224096=CARTESIAN_POINT('Ctrl Pts',(7.56275769304772,-23.9196224070759,
12.));
#224097=CARTESIAN_POINT('Ctrl Pts',(7.5665049786379,-23.8941285782002,12.));
#224098=CARTESIAN_POINT('Ctrl Pts',(7.57018101500708,-23.8687038399595,
12.));
#224099=CARTESIAN_POINT('Ctrl Pts',(7.57378599219813,-23.8433487096132,
12.));
#224100=CARTESIAN_POINT('Ctrl Pts',(7.57732010249065,-23.8180637069976,
12.));
#224101=CARTESIAN_POINT('Ctrl Pts',(7.58078354058212,-23.7928493549908,
12.));
#224102=CARTESIAN_POINT('Ctrl Pts',(7.5841765037627,-23.7677061799376,12.));
#224103=CARTESIAN_POINT('Ctrl Pts',(7.58749919210825,-23.7426347121006,
12.));
#224104=CARTESIAN_POINT('Ctrl Pts',(7.5907518086532,-23.7176354860457,12.));
#224105=CARTESIAN_POINT('Ctrl Pts',(7.59393455934034,-23.6927090405066,
12.));
#224106=CARTESIAN_POINT('Ctrl Pts',(7.59704765299566,-23.6678559182875,
12.));
#224107=CARTESIAN_POINT('Ctrl Pts',(7.60009130130125,-23.6430766661418,
12.));
#224108=CARTESIAN_POINT('Ctrl Pts',(7.60306571877805,-23.6183718346576,
12.));
#224109=CARTESIAN_POINT('Ctrl Pts',(7.60597112277093,-23.5937419781245,
12.));
#224110=CARTESIAN_POINT('Ctrl Pts',(7.60880773344599,-23.5691876544244,
12.));
#224111=CARTESIAN_POINT('Ctrl Pts',(7.61157577385371,-23.544709425203,12.));
#224112=CARTESIAN_POINT('Ctrl Pts',(7.61427546999297,-23.5203078560129,
12.));
#224113=CARTESIAN_POINT('Ctrl Pts',(7.61690705088318,-23.4959835164609,
12.));
#224114=CARTESIAN_POINT('Ctrl Pts',(7.61947074863976,-23.4717369803438,
12.));
#224115=CARTESIAN_POINT('Ctrl Pts',(7.62196679855954,-23.4475688257854,
12.));
#224116=CARTESIAN_POINT('Ctrl Pts',(7.62439543920049,-23.4234796353542,
12.));
#224117=CARTESIAN_POINT('Ctrl Pts',(7.62675691240328,-23.399469996112,12.));
#224118=CARTESIAN_POINT('Ctrl Pts',(7.62905146332592,-23.3755404996636,
12.));
#224119=CARTESIAN_POINT('Ctrl Pts',(7.63127934048136,-23.3516917421972,
12.));
#224120=CARTESIAN_POINT('Ctrl Pts',(7.63344079578161,-23.3279243245241,
12.));
#224121=CARTESIAN_POINT('Ctrl Pts',(7.63553608458782,-23.3042388521022,
12.));
#224122=CARTESIAN_POINT('Ctrl Pts',(7.63756546576373,-23.2806359350855,
12.));
#224123=CARTESIAN_POINT('Ctrl Pts',(7.63952920172834,-23.2571161884488,
12.));
#224124=CARTESIAN_POINT('Ctrl Pts',(7.64142755851504,-23.2336802320912,
12.));
#224125=CARTESIAN_POINT('Ctrl Pts',(7.64326080583679,-23.2103286909398,
12.));
#224126=CARTESIAN_POINT('Ctrl Pts',(7.64502921715482,-23.1870621950452,
12.));
#224127=CARTESIAN_POINT('Ctrl Pts',(7.64673306975804,-23.1638813796694,
12.));
#224128=CARTESIAN_POINT('Ctrl Pts',(7.64837264482942,-23.1407868853819,
12.));
#224129=CARTESIAN_POINT('Ctrl Pts',(7.64994822749859,-23.1177793581679,
12.));
#224130=CARTESIAN_POINT('Ctrl Pts',(7.65146010690475,-23.094859449525,12.));
#224131=CARTESIAN_POINT('Ctrl Pts',(7.65290857626357,-23.072027816555,12.));
#224132=CARTESIAN_POINT('Ctrl Pts',(7.65429393293945,-23.0492851220528,
12.));
#224133=CARTESIAN_POINT('Ctrl Pts',(7.65561647852533,-23.0266320345787,
12.));
#224134=CARTESIAN_POINT('Ctrl Pts',(7.65687651891303,-23.0040692285814,
12.));
#224135=CARTESIAN_POINT('Ctrl Pts',(7.65807436436431,-22.9815973845296,
12.));
#224136=CARTESIAN_POINT('Ctrl Pts',(7.65921032958901,-22.959217189033,12.));
#224137=CARTESIAN_POINT('Ctrl Pts',(7.66028473382777,-22.9369293349593,
12.));
#224138=CARTESIAN_POINT('Ctrl Pts',(7.66129790094107,-22.9147345215421,
12.));
#224139=CARTESIAN_POINT('Ctrl Pts',(7.66225015950155,-22.8926334544883,
12.));
#224140=CARTESIAN_POINT('Ctrl Pts',(7.66314184287336,-22.8706268461283,
12.));
#224141=CARTESIAN_POINT('Ctrl Pts',(7.66397328929802,-22.848715415557,12.));
#224142=CARTESIAN_POINT('Ctrl Pts',(7.66474484198548,-22.8268998887678,
12.));
#224143=CARTESIAN_POINT('Ctrl Pts',(7.66545684920986,-22.8051809987833,
12.));
#224144=CARTESIAN_POINT('Ctrl Pts',(7.66610966441272,-22.7835594857699,
12.));
#224145=CARTESIAN_POINT('Ctrl Pts',(7.66670364630298,-22.7620360971843,
12.));
#224146=CARTESIAN_POINT('Ctrl Pts',(7.66723915895439,-22.7406115879513,
12.));
#224147=CARTESIAN_POINT('Ctrl Pts',(7.66771657191027,-22.7192867206245,
12.));
#224148=CARTESIAN_POINT('Ctrl Pts',(7.66813626029274,-22.6980622655446,
12.));
#224149=CARTESIAN_POINT('Ctrl Pts',(7.66849860491742,-22.6769390009885,
12.));
#224150=CARTESIAN_POINT('Ctrl Pts',(7.66880399241322,-22.6559177133127,
12.));
#224151=CARTESIAN_POINT('Ctrl Pts',(7.66905281533714,-22.6349991971541,
12.));
#224152=CARTESIAN_POINT('Ctrl Pts',(7.66924547229413,-22.6141842556243,
12.));
#224153=CARTESIAN_POINT('Ctrl Pts',(7.66938236806232,-22.5934737004953,
12.));
#224154=CARTESIAN_POINT('Ctrl Pts',(7.66946391372305,-22.5728683523831,
12.));
#224155=CARTESIAN_POINT('Ctrl Pts',(7.66949052679692,-22.5523690409116,
12.));
#224156=CARTESIAN_POINT('Ctrl Pts',(7.66946263138143,-22.53197660492,12.));
#224157=CARTESIAN_POINT('Ctrl Pts',(7.66938065829107,-22.5116918927032,
12.));
#224158=CARTESIAN_POINT('Ctrl Pts',(7.66924504520314,-22.4915157622312,
12.));
#224159=CARTESIAN_POINT('Ctrl Pts',(7.6690562368083,-22.47144908137,12.));
#224160=CARTESIAN_POINT('Ctrl Pts',(7.66881468496634,-22.4514927280855,
12.));
#224161=CARTESIAN_POINT('Ctrl Pts',(7.66852084886703,-22.4316475906603,
12.));
#224162=CARTESIAN_POINT('Ctrl Pts',(7.66817519519639,-22.4119145679758,
12.));
#224163=CARTESIAN_POINT('Ctrl Pts',(7.66777819830789,-22.3922945697773,
12.));
#224164=CARTESIAN_POINT('Ctrl Pts',(7.66733034039882,-22.372788516936,12.));
#224165=CARTESIAN_POINT('Ctrl Pts',(7.66683211169157,-22.3533973417021,
12.));
#224166=CARTESIAN_POINT('Ctrl Pts',(7.66628401061951,-22.3341219879469,
12.));
#224167=CARTESIAN_POINT('Ctrl Pts',(7.66568654402493,-22.314963411484,12.));
#224168=CARTESIAN_POINT('Ctrl Pts',(7.66504022736298,-22.2959225803937,
12.));
#224169=CARTESIAN_POINT('Ctrl Pts',(7.66434558490978,-22.2770004753335,
12.));
#224170=CARTESIAN_POINT('Ctrl Pts',(7.6636031499764,-22.258198089848,12.));
#224171=CARTESIAN_POINT('Ctrl Pts',(7.66281346512508,-22.2395164306547,
12.));
#224172=CARTESIAN_POINT('Ctrl Pts',(7.66197708240399,-22.2209565180085,
12.));
#224173=CARTESIAN_POINT('Ctrl Pts',(7.6610945635927,-22.2025193860964,12.));
#224174=CARTESIAN_POINT('Ctrl Pts',(7.66016648045004,-22.1842060834091,
12.));
#224175=CARTESIAN_POINT('Ctrl Pts',(7.6591934149693,-22.1660176731178,12.));
#224176=CARTESIAN_POINT('Ctrl Pts',(7.65817595963348,-22.1479552334211,
12.));
#224177=CARTESIAN_POINT('Ctrl Pts',(7.65711471769396,-22.1300198579675,
12.));
#224178=CARTESIAN_POINT('Ctrl Pts',(7.65601030346806,-22.1122126563329,
12.));
#224179=CARTESIAN_POINT('Ctrl Pts',(7.65486334263643,-22.094534754469,12.));
#224180=CARTESIAN_POINT('Ctrl Pts',(7.65367447254949,-22.0769872951596,
12.));
#224181=CARTESIAN_POINT('Ctrl Pts',(7.65244434253112,-22.0595714384431,
12.));
#224182=CARTESIAN_POINT('Ctrl Pts',(7.65117361421358,-22.0422883621174,
12.));
#224183=CARTESIAN_POINT('Ctrl Pts',(7.64986296190168,-22.0251392623209,
12.));
#224184=CARTESIAN_POINT('Ctrl Pts',(7.64851307293351,-22.0081253540774,
12.));
#224185=CARTESIAN_POINT('Ctrl Pts',(7.64712464805249,-21.9912478718542,
12.));
#224186=CARTESIAN_POINT('Ctrl Pts',(7.64569840177335,-21.9745080700798,
12.));
#224187=CARTESIAN_POINT('Ctrl Pts',(7.64423506279122,-21.9579072237651,
12.));
#224188=CARTESIAN_POINT('Ctrl Pts',(7.64273537442681,-21.9414466292072,
12.));
#224189=CARTESIAN_POINT('Ctrl Pts',(7.64120009506531,-21.9251276046546,
12.));
#224190=CARTESIAN_POINT('Ctrl Pts',(7.63962999860926,-21.9089514909874,
12.));
#224191=CARTESIAN_POINT('Ctrl Pts',(7.63802587492034,-21.8929196523514,
12.));
#224192=CARTESIAN_POINT('Ctrl Pts',(7.63638853033399,-21.8770334769496,
12.));
#224193=CARTESIAN_POINT('Ctrl Pts',(7.63471878821225,-21.8612943779089,
12.));
#224194=CARTESIAN_POINT('Ctrl Pts',(7.63301748948935,-21.8457037941084,
12.));
#224195=CARTESIAN_POINT('Ctrl Pts',(7.63128549323022,-21.8302631910195,
12.));
#224196=CARTESIAN_POINT('Ctrl Pts',(7.62952367718126,-21.814974061509,12.));
#224197=CARTESIAN_POINT('Ctrl Pts',(7.62773293842388,-21.799837926858,12.));
#224198=CARTESIAN_POINT('Ctrl Pts',(7.62591419404512,-21.7848563378021,
12.));
#224199=CARTESIAN_POINT('Ctrl Pts',(7.62406838181165,-21.7700308755584,
12.));
#224200=CARTESIAN_POINT('Ctrl Pts',(7.62219646084228,-21.7553631528328,
12.));
#224201=CARTESIAN_POINT('Ctrl Pts',(7.62029941230854,-21.7408548148656,
12.));
#224202=CARTESIAN_POINT('Ctrl Pts',(7.61837824030537,-21.7265075407975,
12.));
#224203=CARTESIAN_POINT('Ctrl Pts',(7.6164339727042,-21.7123230449834,12.));
#224204=CARTESIAN_POINT('Ctrl Pts',(7.61446766202786,-21.6983030783322,
12.));
#224205=CARTESIAN_POINT('Ctrl Pts',(7.61248038630268,-21.6844494295815,
12.));
#224206=CARTESIAN_POINT('Ctrl Pts',(7.61047325000955,-21.6707639267576,
12.));
#224207=CARTESIAN_POINT('Ctrl Pts',(7.60844738512873,-21.6572484388081,
12.));
#224208=CARTESIAN_POINT('Ctrl Pts',(7.60640395216356,-21.6439048771743,
12.));
#224209=CARTESIAN_POINT('Ctrl Pts',(7.60434414118295,-21.6307351973822,
12.));
#224210=CARTESIAN_POINT('Ctrl Pts',(7.60226917285428,-21.617741400599,12.));
#224211=CARTESIAN_POINT('Ctrl Pts',(7.6001802998824,-21.6049255358843,12.));
#224212=CARTESIAN_POINT('Ctrl Pts',(7.59807880846194,-21.5922897024466,
12.));
#224213=CARTESIAN_POINT('Ctrl Pts',(7.59596601973583,-21.5798360518978,
12.));
#224214=CARTESIAN_POINT('Ctrl Pts',(7.59384329124918,-21.5675667904726,
12.));
#224215=CARTESIAN_POINT('Ctrl Pts',(7.59171201844776,-21.5554841813462,
12.));
#224216=CARTESIAN_POINT('Ctrl Pts',(7.58957363620013,-21.543590547011,12.));
#224217=CARTESIAN_POINT('Ctrl Pts',(7.58742962034833,-21.5318882716736,
12.));
#224218=CARTESIAN_POINT('Ctrl Pts',(7.58528148919129,-21.5203798035299,
12.));
#224219=CARTESIAN_POINT('Ctrl Pts',(7.58313080519179,-21.5090676573873,
12.));
#224220=CARTESIAN_POINT('Ctrl Pts',(7.58097917790743,-21.4979544192744,
12.));
#224221=CARTESIAN_POINT('Ctrl Pts',(7.57882826679131,-21.4870427508194,
12.));
#224222=CARTESIAN_POINT('Ctrl Pts',(7.57667978402986,-21.4763353936762,
12.));
#224223=CARTESIAN_POINT('Ctrl Pts',(7.57453549743411,-21.4658351740128,
12.));
#224224=CARTESIAN_POINT('Ctrl Pts',(7.57239723223505,-21.4555450053142,
12.));
#224225=CARTESIAN_POINT('Ctrl Pts',(7.57026687261165,-21.4454678907509,
12.));
#224226=CARTESIAN_POINT('Ctrl Pts',(7.56814636360847,-21.4356069261513,
12.));
#224227=CARTESIAN_POINT('Ctrl Pts',(7.56603771218711,-21.4259653015736,
12.));
#224228=CARTESIAN_POINT('Ctrl Pts',(7.56394299313684,-21.4165463106254,
12.));
#224229=CARTESIAN_POINT('Ctrl Pts',(7.56186435703621,-21.4073533630365,
12.));
#224230=CARTESIAN_POINT('Ctrl Pts',(7.5598040370061,-21.3983899952987,12.));
#224231=CARTESIAN_POINT('Ctrl Pts',(7.55776435731416,-21.3896598842117,
12.));
#224232=CARTESIAN_POINT('Ctrl Pts',(7.55574773403502,-21.3811668478932,
12.));
#224233=CARTESIAN_POINT('Ctrl Pts',(7.55375667080028,-21.3729148390243,
12.));
#224234=CARTESIAN_POINT('Ctrl Pts',(7.55179375777443,-21.3649079431865,
12.));
#224235=CARTESIAN_POINT('Ctrl Pts',(7.54986166521309,-21.3571503685855,
12.));
#224236=CARTESIAN_POINT('Ctrl Pts',(7.5479631624633,-21.3496464761531,12.));
#224237=CARTESIAN_POINT('Ctrl Pts',(7.54610114948346,-21.3424008295038,
12.));
#224238=CARTESIAN_POINT('Ctrl Pts',(7.54427868151267,-21.3354182340149,
12.));
#224239=CARTESIAN_POINT('Ctrl Pts',(7.5424990037703,-21.328703791771,12.));
#224240=CARTESIAN_POINT('Ctrl Pts',(7.54076552038278,-21.3222628524165,
12.));
#224241=CARTESIAN_POINT('Ctrl Pts',(7.53908175169898,-21.3161009456256,
12.));
#224242=CARTESIAN_POINT('Ctrl Pts',(7.53745129364615,-21.310223716773,12.));
#224243=CARTESIAN_POINT('Ctrl Pts',(7.53587778251735,-21.3046368712157,
12.));
#224244=CARTESIAN_POINT('Ctrl Pts',(7.53436505309942,-21.2993464250717,
12.));
#224245=CARTESIAN_POINT('Ctrl Pts',(7.53291726078526,-21.2943588989331,
12.));
#224246=CARTESIAN_POINT('Ctrl Pts',(7.53153906987855,-21.2896816163842,
12.));
#224247=CARTESIAN_POINT('Ctrl Pts',(7.53023562438229,-21.2853226580657,
12.));
#224248=CARTESIAN_POINT('Ctrl Pts',(7.52901217930407,-21.2812902781143,
12.));
#224249=CARTESIAN_POINT('Ctrl Pts',(7.52787386225332,-21.2775925269652,
12.));
#224250=CARTESIAN_POINT('Ctrl Pts',(7.5268252691854,-21.2742366113579,12.));
#224251=CARTESIAN_POINT('Ctrl Pts',(7.52587126095529,-21.2712301573466,
12.));
#224252=CARTESIAN_POINT('Ctrl Pts',(7.5250177033353,-21.2685823838671,12.));
#224253=CARTESIAN_POINT('Ctrl Pts',(7.52427261074297,-21.2663059157058,
12.));
#224254=CARTESIAN_POINT('Ctrl Pts',(7.52364573027552,-21.2644161259962,
12.));
#224255=CARTESIAN_POINT('Ctrl Pts',(7.52314642316199,-21.262927782038,12.));
#224256=CARTESIAN_POINT('Ctrl Pts',(7.52278182242669,-21.2618521283555,
12.));
#224257=CARTESIAN_POINT('Ctrl Pts',(7.5226006423166,-21.261326054066,12.));
#224258=CARTESIAN_POINT('Ctrl Pts',(7.52252744144903,-21.2611204474866,
12.));
#224259=CARTESIAN_POINT('Ctrl Pts',(7.52250649703969,-21.2610673466886,
12.));
#224260=CARTESIAN_POINT('Ctrl Pts',(7.52250298901263,-21.2610617890679,
12.));
#224261=CARTESIAN_POINT('',(7.36589684767343,-24.9347862158358,0.));
#224262=CARTESIAN_POINT('Origin',(1.68110656504246,-21.4341755315424,0.));
#224263=CARTESIAN_POINT('',(1.76341220531179,-22.4835757167854,12.));
#224264=CARTESIAN_POINT('',(0.840553282521226,-10.7170877657712,12.));
#224265=CARTESIAN_POINT('',(1.76341220531179,-22.4835757167854,0.));
#224266=CARTESIAN_POINT('',(1.76341220531179,-22.4835757167854,0.));
#224267=CARTESIAN_POINT('',(0.840553282521226,-10.7170877657712,0.));
#224268=CARTESIAN_POINT('Ctrl Pts',(6.08833931617698,-25.2771067246846,
0.));
#224269=CARTESIAN_POINT('Ctrl Pts',(6.08833931617698,-25.2771067246846,
12.));
#224270=CARTESIAN_POINT('Ctrl Pts',(6.08441489609824,-25.2729539149479,
0.));
#224271=CARTESIAN_POINT('Ctrl Pts',(6.08441489609824,-25.2729539149479,
12.));
#224272=CARTESIAN_POINT('Ctrl Pts',(6.07657531787577,-25.2646490489816,
0.));
#224273=CARTESIAN_POINT('Ctrl Pts',(6.07657531787577,-25.2646490489816,
12.));
#224274=CARTESIAN_POINT('Ctrl Pts',(6.06484373634696,-25.2521940105523,
0.));
#224275=CARTESIAN_POINT('Ctrl Pts',(6.06484373634696,-25.2521940105523,
12.));
#224276=CARTESIAN_POINT('Ctrl Pts',(6.04925720151412,-25.2355918138798,
0.));
#224277=CARTESIAN_POINT('Ctrl Pts',(6.04925720151412,-25.2355918138798,
12.));
#224278=CARTESIAN_POINT('Ctrl Pts',(6.02986667390187,-25.2148466201368,
0.));
#224279=CARTESIAN_POINT('Ctrl Pts',(6.02986667390187,-25.2148466201368,
12.));
#224280=CARTESIAN_POINT('Ctrl Pts',(6.0105688180476,-25.1941090269638,0.));
#224281=CARTESIAN_POINT('Ctrl Pts',(6.0105688180476,-25.1941090269638,12.));
#224282=CARTESIAN_POINT('Ctrl Pts',(5.99136367859838,-25.1733791296154,
0.));
#224283=CARTESIAN_POINT('Ctrl Pts',(5.99136367859838,-25.1733791296154,
12.));
#224284=CARTESIAN_POINT('Ctrl Pts',(5.97225131495636,-25.1526570863065,
0.));
#224285=CARTESIAN_POINT('Ctrl Pts',(5.97225131495636,-25.1526570863065,
12.));
#224286=CARTESIAN_POINT('Ctrl Pts',(5.95323180187347,-25.1319431317273,
0.));
#224287=CARTESIAN_POINT('Ctrl Pts',(5.95323180187347,-25.1319431317273,
12.));
#224288=CARTESIAN_POINT('Ctrl Pts',(5.93430523086776,-25.1112375971182,
0.));
#224289=CARTESIAN_POINT('Ctrl Pts',(5.93430523086776,-25.1112375971182,
12.));
#224290=CARTESIAN_POINT('Ctrl Pts',(5.91547170844382,-25.0905409050863,
0.));
#224291=CARTESIAN_POINT('Ctrl Pts',(5.91547170844382,-25.0905409050863,
12.));
#224292=CARTESIAN_POINT('Ctrl Pts',(5.89673135155458,-25.0698535426593,
0.));
#224293=CARTESIAN_POINT('Ctrl Pts',(5.89673135155458,-25.0698535426593,
12.));
#224294=CARTESIAN_POINT('Ctrl Pts',(5.87808428385329,-25.0491760405965,
0.));
#224295=CARTESIAN_POINT('Ctrl Pts',(5.87808428385329,-25.0491760405965,
12.));
#224296=CARTESIAN_POINT('Ctrl Pts',(5.8595306315681,-25.0285089498922,0.));
#224297=CARTESIAN_POINT('Ctrl Pts',(5.8595306315681,-25.0285089498922,12.));
#224298=CARTESIAN_POINT('Ctrl Pts',(5.84107051963073,-25.0078528200558,
0.));
#224299=CARTESIAN_POINT('Ctrl Pts',(5.84107051963073,-25.0078528200558,
12.));
#224300=CARTESIAN_POINT('Ctrl Pts',(5.82270406744213,-24.9872081752709,
0.));
#224301=CARTESIAN_POINT('Ctrl Pts',(5.82270406744213,-24.9872081752709,
12.));
#224302=CARTESIAN_POINT('Ctrl Pts',(5.80443138549747,-24.9665754954463,
0.));
#224303=CARTESIAN_POINT('Ctrl Pts',(5.80443138549747,-24.9665754954463,
12.));
#224304=CARTESIAN_POINT('Ctrl Pts',(5.78625257775702,-24.9459552293308,
0.));
#224305=CARTESIAN_POINT('Ctrl Pts',(5.78625257775702,-24.9459552293308,
12.));
#224306=CARTESIAN_POINT('Ctrl Pts',(5.76816774342236,-24.9253478043632,
0.));
#224307=CARTESIAN_POINT('Ctrl Pts',(5.76816774342236,-24.9253478043632,
12.));
#224308=CARTESIAN_POINT('Ctrl Pts',(5.75017697890812,-24.9047536376467,
0.));
#224309=CARTESIAN_POINT('Ctrl Pts',(5.75017697890812,-24.9047536376467,
12.));
#224310=CARTESIAN_POINT('Ctrl Pts',(5.73228037976926,-24.8841731467219,
0.));
#224311=CARTESIAN_POINT('Ctrl Pts',(5.73228037976926,-24.8841731467219,
12.));
#224312=CARTESIAN_POINT('Ctrl Pts',(5.71447804252019,-24.8636067597677,
0.));
#224313=CARTESIAN_POINT('Ctrl Pts',(5.71447804252019,-24.8636067597677,
12.));
#224314=CARTESIAN_POINT('Ctrl Pts',(5.69677006679429,-24.8430549277634,
0.));
#224315=CARTESIAN_POINT('Ctrl Pts',(5.69677006679429,-24.8430549277634,
12.));
#224316=CARTESIAN_POINT('Ctrl Pts',(5.67915655496524,-24.822518122386,0.));
#224317=CARTESIAN_POINT('Ctrl Pts',(5.67915655496524,-24.822518122386,12.));
#224318=CARTESIAN_POINT('Ctrl Pts',(5.66163761114903,-24.8019968304618,
0.));
#224319=CARTESIAN_POINT('Ctrl Pts',(5.66163761114903,-24.8019968304618,
12.));
#224320=CARTESIAN_POINT('Ctrl Pts',(5.64421334042247,-24.7814915496728,
0.));
#224321=CARTESIAN_POINT('Ctrl Pts',(5.64421334042247,-24.7814915496728,
12.));
#224322=CARTESIAN_POINT('Ctrl Pts',(5.62688384790918,-24.76100278357,0.));
#224323=CARTESIAN_POINT('Ctrl Pts',(5.62688384790918,-24.76100278357,12.));
#224324=CARTESIAN_POINT('Ctrl Pts',(5.60964923798494,-24.7405310372736,
0.));
#224325=CARTESIAN_POINT('Ctrl Pts',(5.60964923798494,-24.7405310372736,
12.));
#224326=CARTESIAN_POINT('Ctrl Pts',(5.59250961323995,-24.7200768119079,
0.));
#224327=CARTESIAN_POINT('Ctrl Pts',(5.59250961323995,-24.7200768119079,
12.));
#224328=CARTESIAN_POINT('Ctrl Pts',(5.57546507427766,-24.6996406035507,
0.));
#224329=CARTESIAN_POINT('Ctrl Pts',(5.57546507427766,-24.6996406035507,
12.));
#224330=CARTESIAN_POINT('Ctrl Pts',(5.55851572025389,-24.6792229061785,
0.));
#224331=CARTESIAN_POINT('Ctrl Pts',(5.55851572025389,-24.6792229061785,
12.));
#224332=CARTESIAN_POINT('Ctrl Pts',(5.54166164919592,-24.6588242134733,
0.));
#224333=CARTESIAN_POINT('Ctrl Pts',(5.54166164919592,-24.6588242134733,
12.));
#224334=CARTESIAN_POINT('Ctrl Pts',(5.52490295840996,-24.6384450211466,
0.));
#224335=CARTESIAN_POINT('Ctrl Pts',(5.52490295840996,-24.6384450211466,
12.));
#224336=CARTESIAN_POINT('Ctrl Pts',(5.50823974481959,-24.618085828918,0.));
#224337=CARTESIAN_POINT('Ctrl Pts',(5.50823974481959,-24.618085828918,12.));
#224338=CARTESIAN_POINT('Ctrl Pts',(5.49167210537235,-24.5977471429365,
0.));
#224339=CARTESIAN_POINT('Ctrl Pts',(5.49167210537235,-24.5977471429365,
12.));
#224340=CARTESIAN_POINT('Ctrl Pts',(5.47520013724403,-24.5774294770329,
0.));
#224341=CARTESIAN_POINT('Ctrl Pts',(5.47520013724403,-24.5774294770329,
12.));
#224342=CARTESIAN_POINT('Ctrl Pts',(5.45882393762244,-24.5571333514841,
0.));
#224343=CARTESIAN_POINT('Ctrl Pts',(5.45882393762244,-24.5571333514841,
12.));
#224344=CARTESIAN_POINT('Ctrl Pts',(5.44254360356865,-24.5368592922861,
0.));
#224345=CARTESIAN_POINT('Ctrl Pts',(5.44254360356865,-24.5368592922861,
12.));
#224346=CARTESIAN_POINT('Ctrl Pts',(5.42635923183411,-24.5166078302107,
0.));
#224347=CARTESIAN_POINT('Ctrl Pts',(5.42635923183411,-24.5166078302107,
12.));
#224348=CARTESIAN_POINT('Ctrl Pts',(5.41027091869242,-24.4963794999831,
0.));
#224349=CARTESIAN_POINT('Ctrl Pts',(5.41027091869242,-24.4963794999831,
12.));
#224350=CARTESIAN_POINT('Ctrl Pts',(5.3942787597383,-24.4761748393322,0.));
#224351=CARTESIAN_POINT('Ctrl Pts',(5.3942787597383,-24.4761748393322,12.));
#224352=CARTESIAN_POINT('Ctrl Pts',(5.37838284973706,-24.4559943883159,
0.));
#224353=CARTESIAN_POINT('Ctrl Pts',(5.37838284973706,-24.4559943883159,
12.));
#224354=CARTESIAN_POINT('Ctrl Pts',(5.36258328273639,-24.4358386899152,
0.));
#224355=CARTESIAN_POINT('Ctrl Pts',(5.36258328273639,-24.4358386899152,
12.));
#224356=CARTESIAN_POINT('Ctrl Pts',(5.34688015213546,-24.4157082904615,
0.));
#224357=CARTESIAN_POINT('Ctrl Pts',(5.34688015213546,-24.4157082904615,
12.));
#224358=CARTESIAN_POINT('Ctrl Pts',(5.33127355076036,-24.3956037401293,
0.));
#224359=CARTESIAN_POINT('Ctrl Pts',(5.33127355076036,-24.3956037401293,
12.));
#224360=CARTESIAN_POINT('Ctrl Pts',(5.31576357092524,-24.3755255933917,
0.));
#224361=CARTESIAN_POINT('Ctrl Pts',(5.31576357092524,-24.3755255933917,
12.));
#224362=CARTESIAN_POINT('Ctrl Pts',(5.30035030449058,-24.3554744095075,
0.));
#224363=CARTESIAN_POINT('Ctrl Pts',(5.30035030449058,-24.3554744095075,
12.));
#224364=CARTESIAN_POINT('Ctrl Pts',(5.28503384290644,-24.3354507529415,
0.));
#224365=CARTESIAN_POINT('Ctrl Pts',(5.28503384290644,-24.3354507529415,
12.));
#224366=CARTESIAN_POINT('Ctrl Pts',(5.26981427718796,-24.3154551932222,
0.));
#224367=CARTESIAN_POINT('Ctrl Pts',(5.26981427718796,-24.3154551932222,
12.));
#224368=CARTESIAN_POINT('Ctrl Pts',(5.25469169788855,-24.2954883048448,
0.));
#224369=CARTESIAN_POINT('Ctrl Pts',(5.25469169788855,-24.2954883048448,
12.));
#224370=CARTESIAN_POINT('Ctrl Pts',(5.23966619506289,-24.2755506671526,
0.));
#224371=CARTESIAN_POINT('Ctrl Pts',(5.23966619506289,-24.2755506671526,
12.));
#224372=CARTESIAN_POINT('Ctrl Pts',(5.22473785822441,-24.2556428642294,
0.));
#224373=CARTESIAN_POINT('Ctrl Pts',(5.22473785822441,-24.2556428642294,
12.));
#224374=CARTESIAN_POINT('Ctrl Pts',(5.20990677629173,-24.2357654847765,
0.));
#224375=CARTESIAN_POINT('Ctrl Pts',(5.20990677629173,-24.2357654847765,
12.));
#224376=CARTESIAN_POINT('Ctrl Pts',(5.19517303753642,-24.215919122017,0.));
#224377=CARTESIAN_POINT('Ctrl Pts',(5.19517303753642,-24.215919122017,12.));
#224378=CARTESIAN_POINT('Ctrl Pts',(5.18053672961392,-24.1961043738754,
0.));
#224379=CARTESIAN_POINT('Ctrl Pts',(5.18053672961392,-24.1961043738754,
12.));
#224380=CARTESIAN_POINT('Ctrl Pts',(5.16599793957979,-24.1763218431343,
0.));
#224381=CARTESIAN_POINT('Ctrl Pts',(5.16599793957979,-24.1763218431343,
12.));
#224382=CARTESIAN_POINT('Ctrl Pts',(5.15155675390075,-24.1565721375971,
0.));
#224383=CARTESIAN_POINT('Ctrl Pts',(5.15155675390075,-24.1565721375971,
12.));
#224384=CARTESIAN_POINT('Ctrl Pts',(5.13721325845744,-24.1368558702443,
0.));
#224385=CARTESIAN_POINT('Ctrl Pts',(5.13721325845744,-24.1368558702443,
12.));
#224386=CARTESIAN_POINT('Ctrl Pts',(5.12296753853859,-24.117173659394,0.));
#224387=CARTESIAN_POINT('Ctrl Pts',(5.12296753853859,-24.117173659394,12.));
#224388=CARTESIAN_POINT('Ctrl Pts',(5.10881967883132,-24.0975261288446,
0.));
#224389=CARTESIAN_POINT('Ctrl Pts',(5.10881967883132,-24.0975261288446,
12.));
#224390=CARTESIAN_POINT('Ctrl Pts',(5.09476976342625,-24.0779139079266,
0.));
#224391=CARTESIAN_POINT('Ctrl Pts',(5.09476976342625,-24.0779139079266,
12.));
#224392=CARTESIAN_POINT('Ctrl Pts',(5.08081787581276,-24.0583376315638,
0.));
#224393=CARTESIAN_POINT('Ctrl Pts',(5.08081787581276,-24.0583376315638,
12.));
#224394=CARTESIAN_POINT('Ctrl Pts',(5.06696409886641,-24.0387979403268,
0.));
#224395=CARTESIAN_POINT('Ctrl Pts',(5.06696409886641,-24.0387979403268,
12.));
#224396=CARTESIAN_POINT('Ctrl Pts',(5.05320851483065,-24.0192954804896,
0.));
#224397=CARTESIAN_POINT('Ctrl Pts',(5.05320851483065,-24.0192954804896,
12.));
#224398=CARTESIAN_POINT('Ctrl Pts',(5.03955120528521,-23.9998309040746,
0.));
#224399=CARTESIAN_POINT('Ctrl Pts',(5.03955120528521,-23.9998309040746,
12.));
#224400=CARTESIAN_POINT('Ctrl Pts',(5.02599225112454,-23.9804048689227,
0.));
#224401=CARTESIAN_POINT('Ctrl Pts',(5.02599225112454,-23.9804048689227,
12.));
#224402=CARTESIAN_POINT('Ctrl Pts',(5.01253173257452,-23.9610180388271,
0.));
#224403=CARTESIAN_POINT('Ctrl Pts',(5.01253173257452,-23.9610180388271,
12.));
#224404=CARTESIAN_POINT('Ctrl Pts',(4.99916972919306,-23.9416710836529,
0.));
#224405=CARTESIAN_POINT('Ctrl Pts',(4.99916972919306,-23.9416710836529,
12.));
#224406=CARTESIAN_POINT('Ctrl Pts',(4.98590631986532,-23.9223646794592,
0.));
#224407=CARTESIAN_POINT('Ctrl Pts',(4.98590631986532,-23.9223646794592,
12.));
#224408=CARTESIAN_POINT('Ctrl Pts',(4.97274158279226,-23.9030995086163,
0.));
#224409=CARTESIAN_POINT('Ctrl Pts',(4.97274158279226,-23.9030995086163,
12.));
#224410=CARTESIAN_POINT('Ctrl Pts',(4.9596755954656,-23.8838762599218,0.));
#224411=CARTESIAN_POINT('Ctrl Pts',(4.9596755954656,-23.8838762599218,12.));
#224412=CARTESIAN_POINT('Ctrl Pts',(4.9467084346586,-23.8646956287168,0.));
#224413=CARTESIAN_POINT('Ctrl Pts',(4.9467084346586,-23.8646956287168,12.));
#224414=CARTESIAN_POINT('Ctrl Pts',(4.93384017643432,-23.8455583170057,
0.));
#224415=CARTESIAN_POINT('Ctrl Pts',(4.93384017643432,-23.8455583170057,
12.));
#224416=CARTESIAN_POINT('Ctrl Pts',(4.92107089613968,-23.8264650335717,
0.));
#224417=CARTESIAN_POINT('Ctrl Pts',(4.92107089613968,-23.8264650335717,
12.));
#224418=CARTESIAN_POINT('Ctrl Pts',(4.90840066839344,-23.8074164940896,
0.));
#224419=CARTESIAN_POINT('Ctrl Pts',(4.90840066839344,-23.8074164940896,
12.));
#224420=CARTESIAN_POINT('Ctrl Pts',(4.89582956706775,-23.7884134212384,
0.));
#224421=CARTESIAN_POINT('Ctrl Pts',(4.89582956706775,-23.7884134212384,
12.));
#224422=CARTESIAN_POINT('Ctrl Pts',(4.88335766525573,-23.7694565448049,
0.));
#224423=CARTESIAN_POINT('Ctrl Pts',(4.88335766525573,-23.7694565448049,
12.));
#224424=CARTESIAN_POINT('Ctrl Pts',(4.87098503527152,-23.7505466018245,
0.));
#224425=CARTESIAN_POINT('Ctrl Pts',(4.87098503527152,-23.7505466018245,
12.));
#224426=CARTESIAN_POINT('Ctrl Pts',(4.85871174865499,-23.7316843367313,
0.));
#224427=CARTESIAN_POINT('Ctrl Pts',(4.85871174865499,-23.7316843367313,
12.));
#224428=CARTESIAN_POINT('Ctrl Pts',(4.84653787616425,-23.7128705015017,
0.));
#224429=CARTESIAN_POINT('Ctrl Pts',(4.84653787616425,-23.7128705015017,
12.));
#224430=CARTESIAN_POINT('Ctrl Pts',(4.83446348776265,-23.6941058557971,
0.));
#224431=CARTESIAN_POINT('Ctrl Pts',(4.83446348776265,-23.6941058557971,
12.));
#224432=CARTESIAN_POINT('Ctrl Pts',(4.82248865259562,-23.675391167102,0.));
#224433=CARTESIAN_POINT('Ctrl Pts',(4.82248865259562,-23.675391167102,12.));
#224434=CARTESIAN_POINT('Ctrl Pts',(4.81061343896432,-23.6567272108628,
0.));
#224435=CARTESIAN_POINT('Ctrl Pts',(4.81061343896432,-23.6567272108628,
12.));
#224436=CARTESIAN_POINT('Ctrl Pts',(4.7988379143322,-23.6381147706579,0.));
#224437=CARTESIAN_POINT('Ctrl Pts',(4.7988379143322,-23.6381147706579,12.));
#224438=CARTESIAN_POINT('Ctrl Pts',(4.78716214532097,-23.6195546383624,
0.));
#224439=CARTESIAN_POINT('Ctrl Pts',(4.78716214532097,-23.6195546383624,
12.));
#224440=CARTESIAN_POINT('Ctrl Pts',(4.77558619769872,-23.6010476143099,
0.));
#224441=CARTESIAN_POINT('Ctrl Pts',(4.77558619769872,-23.6010476143099,
12.));
#224442=CARTESIAN_POINT('Ctrl Pts',(4.76411013636251,-23.5825945074535,
0.));
#224443=CARTESIAN_POINT('Ctrl Pts',(4.76411013636251,-23.5825945074535,
12.));
#224444=CARTESIAN_POINT('Ctrl Pts',(4.75273402530617,-23.5641961355168,
0.));
#224445=CARTESIAN_POINT('Ctrl Pts',(4.75273402530617,-23.5641961355168,
12.));
#224446=CARTESIAN_POINT('Ctrl Pts',(4.74145792760698,-23.545853325171,0.));
#224447=CARTESIAN_POINT('Ctrl Pts',(4.74145792760698,-23.545853325171,12.));
#224448=CARTESIAN_POINT('Ctrl Pts',(4.73028190543029,-23.5275669122372,
0.));
#224449=CARTESIAN_POINT('Ctrl Pts',(4.73028190543029,-23.5275669122372,
12.));
#224450=CARTESIAN_POINT('Ctrl Pts',(4.71920602001901,-23.509337741878,0.));
#224451=CARTESIAN_POINT('Ctrl Pts',(4.71920602001901,-23.509337741878,12.));
#224452=CARTESIAN_POINT('Ctrl Pts',(4.70823033167818,-23.491166668789,0.));
#224453=CARTESIAN_POINT('Ctrl Pts',(4.70823033167818,-23.491166668789,12.));
#224454=CARTESIAN_POINT('Ctrl Pts',(4.69735489975024,-23.4730545573853,
0.));
#224455=CARTESIAN_POINT('Ctrl Pts',(4.69735489975024,-23.4730545573853,
12.));
#224456=CARTESIAN_POINT('Ctrl Pts',(4.68657978258303,-23.455002281986,0.));
#224457=CARTESIAN_POINT('Ctrl Pts',(4.68657978258303,-23.455002281986,12.));
#224458=CARTESIAN_POINT('Ctrl Pts',(4.67590503753058,-23.4370107270451,
0.));
#224459=CARTESIAN_POINT('Ctrl Pts',(4.67590503753058,-23.4370107270451,
12.));
#224460=CARTESIAN_POINT('Ctrl Pts',(4.6653307209467,-23.4190807873803,0.));
#224461=CARTESIAN_POINT('Ctrl Pts',(4.6653307209467,-23.4190807873803,12.));
#224462=CARTESIAN_POINT('Ctrl Pts',(4.65485688816924,-23.4012133683959,
0.));
#224463=CARTESIAN_POINT('Ctrl Pts',(4.65485688816924,-23.4012133683959,
12.));
#224464=CARTESIAN_POINT('Ctrl Pts',(4.6444835934993,-23.3834093863068,0.));
#224465=CARTESIAN_POINT('Ctrl Pts',(4.6444835934993,-23.3834093863068,12.));
#224466=CARTESIAN_POINT('Ctrl Pts',(4.63421089016541,-23.3656697683489,
0.));
#224467=CARTESIAN_POINT('Ctrl Pts',(4.63421089016541,-23.3656697683489,
12.));
#224468=CARTESIAN_POINT('Ctrl Pts',(4.62403883030805,-23.3479954530272,
0.));
#224469=CARTESIAN_POINT('Ctrl Pts',(4.62403883030805,-23.3479954530272,
12.));
#224470=CARTESIAN_POINT('Ctrl Pts',(4.6139674649783,-23.3303873903938,0.));
#224471=CARTESIAN_POINT('Ctrl Pts',(4.6139674649783,-23.3303873903938,12.));
#224472=CARTESIAN_POINT('Ctrl Pts',(4.60399684412163,-23.3128465423115,
0.));
#224473=CARTESIAN_POINT('Ctrl Pts',(4.60399684412163,-23.3128465423115,
12.));
#224474=CARTESIAN_POINT('Ctrl Pts',(4.5941270165575,-23.2953738827191,0.));
#224475=CARTESIAN_POINT('Ctrl Pts',(4.5941270165575,-23.2953738827191,12.));
#224476=CARTESIAN_POINT('Ctrl Pts',(4.5843580299469,-23.2779703978876,0.));
#224477=CARTESIAN_POINT('Ctrl Pts',(4.5843580299469,-23.2779703978876,12.));
#224478=CARTESIAN_POINT('Ctrl Pts',(4.57468993076097,-23.2606370866866,
0.));
#224479=CARTESIAN_POINT('Ctrl Pts',(4.57468993076097,-23.2606370866866,
12.));
#224480=CARTESIAN_POINT('Ctrl Pts',(4.56512276427839,-23.2433749609131,
0.));
#224481=CARTESIAN_POINT('Ctrl Pts',(4.56512276427839,-23.2433749609131,
12.));
#224482=CARTESIAN_POINT('Ctrl Pts',(4.55565657456975,-23.2261850456064,
0.));
#224483=CARTESIAN_POINT('Ctrl Pts',(4.55565657456975,-23.2261850456064,
12.));
#224484=CARTESIAN_POINT('Ctrl Pts',(4.54629140447544,-23.2090683793629,
0.));
#224485=CARTESIAN_POINT('Ctrl Pts',(4.54629140447544,-23.2090683793629,
12.));
#224486=CARTESIAN_POINT('Ctrl Pts',(4.53702729557566,-23.1920260146465,
0.));
#224487=CARTESIAN_POINT('Ctrl Pts',(4.53702729557566,-23.1920260146465,
12.));
#224488=CARTESIAN_POINT('Ctrl Pts',(4.52786428815014,-23.1750590180908,
0.));
#224489=CARTESIAN_POINT('Ctrl Pts',(4.52786428815014,-23.1750590180908,
12.));
#224490=CARTESIAN_POINT('Ctrl Pts',(4.51880242116748,-23.1581684708761,
0.));
#224491=CARTESIAN_POINT('Ctrl Pts',(4.51880242116748,-23.1581684708761,
12.));
#224492=CARTESIAN_POINT('Ctrl Pts',(4.5098417322706,-23.1413554691123,0.));
#224493=CARTESIAN_POINT('Ctrl Pts',(4.5098417322706,-23.1413554691123,12.));
#224494=CARTESIAN_POINT('Ctrl Pts',(4.50098225775171,-23.1246211242115,
0.));
#224495=CARTESIAN_POINT('Ctrl Pts',(4.50098225775171,-23.1246211242115,
12.));
#224496=CARTESIAN_POINT('Ctrl Pts',(4.49222403252216,-23.1079665632636,
0.));
#224497=CARTESIAN_POINT('Ctrl Pts',(4.49222403252216,-23.1079665632636,
12.));
#224498=CARTESIAN_POINT('Ctrl Pts',(4.48356709006788,-23.0913929293922,
0.));
#224499=CARTESIAN_POINT('Ctrl Pts',(4.48356709006788,-23.0913929293922,
12.));
#224500=CARTESIAN_POINT('Ctrl Pts',(4.47501146242856,-23.0749013821881,
0.));
#224501=CARTESIAN_POINT('Ctrl Pts',(4.47501146242856,-23.0749013821881,
12.));
#224502=CARTESIAN_POINT('Ctrl Pts',(4.4665571801823,-23.0584930981732,0.));
#224503=CARTESIAN_POINT('Ctrl Pts',(4.4665571801823,-23.0584930981732,12.));
#224504=CARTESIAN_POINT('Ctrl Pts',(4.45820427241683,-23.0421692712467,
0.));
#224505=CARTESIAN_POINT('Ctrl Pts',(4.45820427241683,-23.0421692712467,
12.));
#224506=CARTESIAN_POINT('Ctrl Pts',(4.44995276669686,-23.0259311131392,
0.));
#224507=CARTESIAN_POINT('Ctrl Pts',(4.44995276669686,-23.0259311131392,
12.));
#224508=CARTESIAN_POINT('Ctrl Pts',(4.44180268901643,-23.0097798538395,
0.));
#224509=CARTESIAN_POINT('Ctrl Pts',(4.44180268901643,-23.0097798538395,
12.));
#224510=CARTESIAN_POINT('Ctrl Pts',(4.43375406376879,-22.9937167421006,
0.));
#224511=CARTESIAN_POINT('Ctrl Pts',(4.43375406376879,-22.9937167421006,
12.));
#224512=CARTESIAN_POINT('Ctrl Pts',(4.42580691372751,-22.977743046002,0.));
#224513=CARTESIAN_POINT('Ctrl Pts',(4.42580691372751,-22.977743046002,12.));
#224514=CARTESIAN_POINT('Ctrl Pts',(4.41796126001302,-22.9618600534866,
0.));
#224515=CARTESIAN_POINT('Ctrl Pts',(4.41796126001302,-22.9618600534866,
12.));
#224516=CARTESIAN_POINT('Ctrl Pts',(4.41021712205553,-22.9460690729093,
0.));
#224517=CARTESIAN_POINT('Ctrl Pts',(4.41021712205553,-22.9460690729093,
12.));
#224518=CARTESIAN_POINT('Ctrl Pts',(4.40257451754323,-22.930371433555,0.));
#224519=CARTESIAN_POINT('Ctrl Pts',(4.40257451754323,-22.930371433555,12.));
#224520=CARTESIAN_POINT('Ctrl Pts',(4.39503346238473,-22.9147684862426,
0.));
#224521=CARTESIAN_POINT('Ctrl Pts',(4.39503346238473,-22.9147684862426,
12.));
#224522=CARTESIAN_POINT('Ctrl Pts',(4.38759397068405,-22.8992616040108,
0.));
#224523=CARTESIAN_POINT('Ctrl Pts',(4.38759397068405,-22.8992616040108,
12.));
#224524=CARTESIAN_POINT('Ctrl Pts',(4.38025605470092,-22.8838521827701,
0.));
#224525=CARTESIAN_POINT('Ctrl Pts',(4.38025605470092,-22.8838521827701,
12.));
#224526=CARTESIAN_POINT('Ctrl Pts',(4.37301972480745,-22.8685416419725,
0.));
#224527=CARTESIAN_POINT('Ctrl Pts',(4.37301972480745,-22.8685416419725,
12.));
#224528=CARTESIAN_POINT('Ctrl Pts',(4.36588498942997,-22.8533314252422,
0.));
#224529=CARTESIAN_POINT('Ctrl Pts',(4.36588498942997,-22.8533314252422,
12.));
#224530=CARTESIAN_POINT('Ctrl Pts',(4.35885185500546,-22.8382230011184,
0.));
#224531=CARTESIAN_POINT('Ctrl Pts',(4.35885185500546,-22.8382230011184,
12.));
#224532=CARTESIAN_POINT('Ctrl Pts',(4.3519203259479,-22.8232178638876,0.));
#224533=CARTESIAN_POINT('Ctrl Pts',(4.3519203259479,-22.8232178638876,12.));
#224534=CARTESIAN_POINT('Ctrl Pts',(4.34509040460062,-22.8083175343791,
0.));
#224535=CARTESIAN_POINT('Ctrl Pts',(4.34509040460062,-22.8083175343791,
12.));
#224536=CARTESIAN_POINT('Ctrl Pts',(4.33836209118446,-22.7935235607806,
0.));
#224537=CARTESIAN_POINT('Ctrl Pts',(4.33836209118446,-22.7935235607806,
12.));
#224538=CARTESIAN_POINT('Ctrl Pts',(4.33173538373189,-22.7788375194076,
0.));
#224539=CARTESIAN_POINT('Ctrl Pts',(4.33173538373189,-22.7788375194076,
12.));
#224540=CARTESIAN_POINT('Ctrl Pts',(4.32521027803754,-22.7642610156475,
0.));
#224541=CARTESIAN_POINT('Ctrl Pts',(4.32521027803754,-22.7642610156475,
12.));
#224542=CARTESIAN_POINT('Ctrl Pts',(4.31878676761235,-22.7497956849848,
0.));
#224543=CARTESIAN_POINT('Ctrl Pts',(4.31878676761235,-22.7497956849848,
12.));
#224544=CARTESIAN_POINT('Ctrl Pts',(4.31246484362549,-22.7354431939926,
0.));
#224545=CARTESIAN_POINT('Ctrl Pts',(4.31246484362549,-22.7354431939926,
12.));
#224546=CARTESIAN_POINT('Ctrl Pts',(4.30624449484069,-22.7212052413386,
0.));
#224547=CARTESIAN_POINT('Ctrl Pts',(4.30624449484069,-22.7212052413386,
12.));
#224548=CARTESIAN_POINT('Ctrl Pts',(4.3001257075406,-22.7070835587564,0.));
#224549=CARTESIAN_POINT('Ctrl Pts',(4.3001257075406,-22.7070835587564,12.));
#224550=CARTESIAN_POINT('Ctrl Pts',(4.29410846547056,-22.6930799122548,
0.));
#224551=CARTESIAN_POINT('Ctrl Pts',(4.29410846547056,-22.6930799122548,
12.));
#224552=CARTESIAN_POINT('Ctrl Pts',(4.28819274977763,-22.6791961033538,
0.));
#224553=CARTESIAN_POINT('Ctrl Pts',(4.28819274977763,-22.6791961033538,
12.));
#224554=CARTESIAN_POINT('Ctrl Pts',(4.28237853894058,-22.6654339703109,
0.));
#224555=CARTESIAN_POINT('Ctrl Pts',(4.28237853894058,-22.6654339703109,
12.));
#224556=CARTESIAN_POINT('Ctrl Pts',(4.2766658086912,-22.6517953893303,0.));
#224557=CARTESIAN_POINT('Ctrl Pts',(4.2766658086912,-22.6517953893303,12.));
#224558=CARTESIAN_POINT('Ctrl Pts',(4.27105453193004,-22.6382822758172,
0.));
#224559=CARTESIAN_POINT('Ctrl Pts',(4.27105453193004,-22.6382822758172,
12.));
#224560=CARTESIAN_POINT('Ctrl Pts',(4.26554467865576,-22.6248965859977,
0.));
#224561=CARTESIAN_POINT('Ctrl Pts',(4.26554467865576,-22.6248965859977,
12.));
#224562=CARTESIAN_POINT('Ctrl Pts',(4.26013621588305,-22.6116403184821,
0.));
#224563=CARTESIAN_POINT('Ctrl Pts',(4.26013621588305,-22.6116403184821,
12.));
#224564=CARTESIAN_POINT('Ctrl Pts',(4.25482910755481,-22.5985155158636,
0.));
#224565=CARTESIAN_POINT('Ctrl Pts',(4.25482910755481,-22.5985155158636,
12.));
#224566=CARTESIAN_POINT('Ctrl Pts',(4.24962331444177,-22.5855242662477,
0.));
#224567=CARTESIAN_POINT('Ctrl Pts',(4.24962331444177,-22.5855242662477,
12.));
#224568=CARTESIAN_POINT('Ctrl Pts',(4.24451879404851,-22.572668704992,0.));
#224569=CARTESIAN_POINT('Ctrl Pts',(4.24451879404851,-22.572668704992,12.));
#224570=CARTESIAN_POINT('Ctrl Pts',(4.23951550052522,-22.5599510166429,
0.));
#224571=CARTESIAN_POINT('Ctrl Pts',(4.23951550052522,-22.5599510166429,
12.));
#224572=CARTESIAN_POINT('Ctrl Pts',(4.23461338456712,-22.5473734368086,
0.));
#224573=CARTESIAN_POINT('Ctrl Pts',(4.23461338456712,-22.5473734368086,
12.));
#224574=CARTESIAN_POINT('Ctrl Pts',(4.22981239330733,-22.5349382540588,
0.));
#224575=CARTESIAN_POINT('Ctrl Pts',(4.22981239330733,-22.5349382540588,
12.));
#224576=CARTESIAN_POINT('Ctrl Pts',(4.22511247020041,-22.5226478117886,
0.));
#224577=CARTESIAN_POINT('Ctrl Pts',(4.22511247020041,-22.5226478117886,
12.));
#224578=CARTESIAN_POINT('Ctrl Pts',(4.22051355490196,-22.5105045108881,
0.));
#224579=CARTESIAN_POINT('Ctrl Pts',(4.22051355490196,-22.5105045108881,
12.));
#224580=CARTESIAN_POINT('Ctrl Pts',(4.21601558313906,-22.4985108124228,
0.));
#224581=CARTESIAN_POINT('Ctrl Pts',(4.21601558313906,-22.4985108124228,
12.));
#224582=CARTESIAN_POINT('Ctrl Pts',(4.21161848657428,-22.4866692403147,
0.));
#224583=CARTESIAN_POINT('Ctrl Pts',(4.21161848657428,-22.4866692403147,
12.));
#224584=CARTESIAN_POINT('Ctrl Pts',(4.20732219265648,-22.4749823839917,
0.));
#224585=CARTESIAN_POINT('Ctrl Pts',(4.20732219265648,-22.4749823839917,
12.));
#224586=CARTESIAN_POINT('Ctrl Pts',(4.20312662448174,-22.4634529011437,
0.));
#224587=CARTESIAN_POINT('Ctrl Pts',(4.20312662448174,-22.4634529011437,
12.));
#224588=CARTESIAN_POINT('Ctrl Pts',(4.19903170066358,-22.4520835205422,
0.));
#224589=CARTESIAN_POINT('Ctrl Pts',(4.19903170066358,-22.4520835205422,
12.));
#224590=CARTESIAN_POINT('Ctrl Pts',(4.1950373351886,-22.4408770448917,0.));
#224591=CARTESIAN_POINT('Ctrl Pts',(4.1950373351886,-22.4408770448917,12.));
#224592=CARTESIAN_POINT('Ctrl Pts',(4.19114343726932,-22.4298363535416,
0.));
#224593=CARTESIAN_POINT('Ctrl Pts',(4.19114343726932,-22.4298363535416,
12.));
#224594=CARTESIAN_POINT('Ctrl Pts',(4.18734991117707,-22.4189644056109,
0.));
#224595=CARTESIAN_POINT('Ctrl Pts',(4.18734991117707,-22.4189644056109,
12.));
#224596=CARTESIAN_POINT('Ctrl Pts',(4.18365665600839,-22.4082642454448,
0.));
#224597=CARTESIAN_POINT('Ctrl Pts',(4.18365665600839,-22.4082642454448,
12.));
#224598=CARTESIAN_POINT('Ctrl Pts',(4.18006356544879,-22.3977390078074,
0.));
#224599=CARTESIAN_POINT('Ctrl Pts',(4.18006356544879,-22.3977390078074,
12.));
#224600=CARTESIAN_POINT('Ctrl Pts',(4.17657052752834,-22.3873919231339,
0.));
#224601=CARTESIAN_POINT('Ctrl Pts',(4.17657052752834,-22.3873919231339,
12.));
#224602=CARTESIAN_POINT('Ctrl Pts',(4.17317742436162,-22.3772263228624,
0.));
#224603=CARTESIAN_POINT('Ctrl Pts',(4.17317742436162,-22.3772263228624,
12.));
#224604=CARTESIAN_POINT('Ctrl Pts',(4.16988413199469,-22.3672456427605,
0.));
#224605=CARTESIAN_POINT('Ctrl Pts',(4.16988413199469,-22.3672456427605,
12.));
#224606=CARTESIAN_POINT('Ctrl Pts',(4.16669052026602,-22.3574534257397,
0.));
#224607=CARTESIAN_POINT('Ctrl Pts',(4.16669052026602,-22.3574534257397,
12.));
#224608=CARTESIAN_POINT('Ctrl Pts',(4.1635964526318,-22.3478533253886,0.));
#224609=CARTESIAN_POINT('Ctrl Pts',(4.1635964526318,-22.3478533253886,12.));
#224610=CARTESIAN_POINT('Ctrl Pts',(4.16060178604153,-22.3384491078599,
0.));
#224611=CARTESIAN_POINT('Ctrl Pts',(4.16060178604153,-22.3384491078599,
12.));
#224612=CARTESIAN_POINT('Ctrl Pts',(4.15770637047882,-22.3292446628957,
0.));
#224613=CARTESIAN_POINT('Ctrl Pts',(4.15770637047882,-22.3292446628957,
12.));
#224614=CARTESIAN_POINT('Ctrl Pts',(4.15491004835278,-22.3202440186979,
0.));
#224615=CARTESIAN_POINT('Ctrl Pts',(4.15491004835278,-22.3202440186979,
12.));
#224616=CARTESIAN_POINT('Ctrl Pts',(4.15221265396992,-22.3114513545186,
0.));
#224617=CARTESIAN_POINT('Ctrl Pts',(4.15221265396992,-22.3114513545186,
12.));
#224618=CARTESIAN_POINT('Ctrl Pts',(4.14961401285525,-22.3028710166935,
0.));
#224619=CARTESIAN_POINT('Ctrl Pts',(4.14961401285525,-22.3028710166935,
12.));
#224620=CARTESIAN_POINT('Ctrl Pts',(4.14711394168559,-22.2945075198468,
0.));
#224621=CARTESIAN_POINT('Ctrl Pts',(4.14711394168559,-22.2945075198468,
12.));
#224622=CARTESIAN_POINT('Ctrl Pts',(4.14471224859295,-22.2863655389167,
0.));
#224623=CARTESIAN_POINT('Ctrl Pts',(4.14471224859295,-22.2863655389167,
12.));
#224624=CARTESIAN_POINT('Ctrl Pts',(4.14240873321982,-22.2784499072026,
0.));
#224625=CARTESIAN_POINT('Ctrl Pts',(4.14240873321982,-22.2784499072026,
12.));
#224626=CARTESIAN_POINT('Ctrl Pts',(4.14020318715987,-22.2707656042456,
0.));
#224627=CARTESIAN_POINT('Ctrl Pts',(4.14020318715987,-22.2707656042456,
12.));
#224628=CARTESIAN_POINT('Ctrl Pts',(4.13809539255418,-22.263317791397,0.));
#224629=CARTESIAN_POINT('Ctrl Pts',(4.13809539255418,-22.263317791397,12.));
#224630=CARTESIAN_POINT('Ctrl Pts',(4.13608511977226,-22.2561118708422,
0.));
#224631=CARTESIAN_POINT('Ctrl Pts',(4.13608511977226,-22.2561118708422,
12.));
#224632=CARTESIAN_POINT('Ctrl Pts',(4.13417212558808,-22.2491535317789,
0.));
#224633=CARTESIAN_POINT('Ctrl Pts',(4.13417212558808,-22.2491535317789,
12.));
#224634=CARTESIAN_POINT('Ctrl Pts',(4.1323561506016,-22.2424488153523,0.));
#224635=CARTESIAN_POINT('Ctrl Pts',(4.1323561506016,-22.2424488153523,12.));
#224636=CARTESIAN_POINT('Ctrl Pts',(4.13063692157499,-22.2360040565534,
0.));
#224637=CARTESIAN_POINT('Ctrl Pts',(4.13063692157499,-22.2360040565534,
12.));
#224638=CARTESIAN_POINT('Ctrl Pts',(4.12901415463378,-22.2298258043947,
0.));
#224639=CARTESIAN_POINT('Ctrl Pts',(4.12901415463378,-22.2298258043947,
12.));
#224640=CARTESIAN_POINT('Ctrl Pts',(4.12748755830099,-22.2239207458781,
0.));
#224641=CARTESIAN_POINT('Ctrl Pts',(4.12748755830099,-22.2239207458781,
12.));
#224642=CARTESIAN_POINT('Ctrl Pts',(4.12605683613299,-22.2182956401341,
0.));
#224643=CARTESIAN_POINT('Ctrl Pts',(4.12605683613299,-22.2182956401341,
12.));
#224644=CARTESIAN_POINT('Ctrl Pts',(4.12472167516602,-22.2129576146671,
0.));
#224645=CARTESIAN_POINT('Ctrl Pts',(4.12472167516602,-22.2129576146671,
12.));
#224646=CARTESIAN_POINT('Ctrl Pts',(4.12348173702024,-22.2079143941719,
0.));
#224647=CARTESIAN_POINT('Ctrl Pts',(4.12348173702024,-22.2079143941719,
12.));
#224648=CARTESIAN_POINT('Ctrl Pts',(4.12233664408237,-22.2031746532106,
0.));
#224649=CARTESIAN_POINT('Ctrl Pts',(4.12233664408237,-22.2031746532106,
12.));
#224650=CARTESIAN_POINT('Ctrl Pts',(4.12128598183533,-22.1987479618246,
0.));
#224651=CARTESIAN_POINT('Ctrl Pts',(4.12128598183533,-22.1987479618246,
12.));
#224652=CARTESIAN_POINT('Ctrl Pts',(4.12032932637738,-22.1946440958098,
0.));
#224653=CARTESIAN_POINT('Ctrl Pts',(4.12032932637738,-22.1946440958098,
12.));
#224654=CARTESIAN_POINT('Ctrl Pts',(4.11946626228623,-22.1908725908525,
0.));
#224655=CARTESIAN_POINT('Ctrl Pts',(4.11946626228623,-22.1908725908525,
12.));
#224656=CARTESIAN_POINT('Ctrl Pts',(4.11869641271752,-22.1874419861496,
0.));
#224657=CARTESIAN_POINT('Ctrl Pts',(4.11869641271752,-22.1874419861496,
12.));
#224658=CARTESIAN_POINT('Ctrl Pts',(4.11801938107464,-22.1843613164855,
0.));
#224659=CARTESIAN_POINT('Ctrl Pts',(4.11801938107464,-22.1843613164855,
12.));
#224660=CARTESIAN_POINT('Ctrl Pts',(4.11743469691765,-22.1816414985788,
0.));
#224661=CARTESIAN_POINT('Ctrl Pts',(4.11743469691765,-22.1816414985788,
12.));
#224662=CARTESIAN_POINT('Ctrl Pts',(4.11694173195041,-22.179297473024,0.));
#224663=CARTESIAN_POINT('Ctrl Pts',(4.11694173195041,-22.179297473024,12.));
#224664=CARTESIAN_POINT('Ctrl Pts',(4.11653973150558,-22.177347426894,0.));
#224665=CARTESIAN_POINT('Ctrl Pts',(4.11653973150558,-22.177347426894,12.));
#224666=CARTESIAN_POINT('Ctrl Pts',(4.11622797217066,-22.1758088296598,
0.));
#224667=CARTESIAN_POINT('Ctrl Pts',(4.11622797217066,-22.1758088296598,
12.));
#224668=CARTESIAN_POINT('Ctrl Pts',(4.11600589882767,-22.1746949858773,
0.));
#224669=CARTESIAN_POINT('Ctrl Pts',(4.11600589882767,-22.1746949858773,
12.));
#224670=CARTESIAN_POINT('Ctrl Pts',(4.11589976826061,-22.174148802123,0.));
#224671=CARTESIAN_POINT('Ctrl Pts',(4.11589976826061,-22.174148802123,12.));
#224672=CARTESIAN_POINT('Ctrl Pts',(4.1158603587821,-22.1739341411684,0.));
#224673=CARTESIAN_POINT('Ctrl Pts',(4.1158603587821,-22.1739341411684,12.));
#224674=CARTESIAN_POINT('Ctrl Pts',(4.11585194677412,-22.1738776823239,
0.));
#224675=CARTESIAN_POINT('Ctrl Pts',(4.11585194677412,-22.1738776823239,
12.));
#224676=CARTESIAN_POINT('Ctrl Pts',(4.11585220600461,-22.1738711152697,
0.));
#224677=CARTESIAN_POINT('Ctrl Pts',(4.11585220600461,-22.1738711152697,
12.));
#224678=CARTESIAN_POINT('',(6.08833931617698,-25.2771067246846,0.));
#224679=CARTESIAN_POINT('Ctrl Pts',(6.08833931617698,-25.2771067246846,
0.));
#224680=CARTESIAN_POINT('Ctrl Pts',(6.08441489609824,-25.2729539149479,
0.));
#224681=CARTESIAN_POINT('Ctrl Pts',(6.07657531787577,-25.2646490489816,
0.));
#224682=CARTESIAN_POINT('Ctrl Pts',(6.06484373634696,-25.2521940105523,
0.));
#224683=CARTESIAN_POINT('Ctrl Pts',(6.04925720151412,-25.2355918138798,
0.));
#224684=CARTESIAN_POINT('Ctrl Pts',(6.02986667390187,-25.2148466201368,
0.));
#224685=CARTESIAN_POINT('Ctrl Pts',(6.0105688180476,-25.1941090269638,0.));
#224686=CARTESIAN_POINT('Ctrl Pts',(5.99136367859838,-25.1733791296154,
0.));
#224687=CARTESIAN_POINT('Ctrl Pts',(5.97225131495636,-25.1526570863065,
0.));
#224688=CARTESIAN_POINT('Ctrl Pts',(5.95323180187347,-25.1319431317273,
0.));
#224689=CARTESIAN_POINT('Ctrl Pts',(5.93430523086776,-25.1112375971182,
0.));
#224690=CARTESIAN_POINT('Ctrl Pts',(5.91547170844382,-25.0905409050863,
0.));
#224691=CARTESIAN_POINT('Ctrl Pts',(5.89673135155458,-25.0698535426593,
0.));
#224692=CARTESIAN_POINT('Ctrl Pts',(5.87808428385329,-25.0491760405965,
0.));
#224693=CARTESIAN_POINT('Ctrl Pts',(5.8595306315681,-25.0285089498922,0.));
#224694=CARTESIAN_POINT('Ctrl Pts',(5.84107051963073,-25.0078528200558,
0.));
#224695=CARTESIAN_POINT('Ctrl Pts',(5.82270406744213,-24.9872081752709,
0.));
#224696=CARTESIAN_POINT('Ctrl Pts',(5.80443138549747,-24.9665754954463,
0.));
#224697=CARTESIAN_POINT('Ctrl Pts',(5.78625257775702,-24.9459552293308,
0.));
#224698=CARTESIAN_POINT('Ctrl Pts',(5.76816774342236,-24.9253478043632,
0.));
#224699=CARTESIAN_POINT('Ctrl Pts',(5.75017697890812,-24.9047536376467,
0.));
#224700=CARTESIAN_POINT('Ctrl Pts',(5.73228037976926,-24.8841731467219,
0.));
#224701=CARTESIAN_POINT('Ctrl Pts',(5.71447804252019,-24.8636067597677,
0.));
#224702=CARTESIAN_POINT('Ctrl Pts',(5.69677006679429,-24.8430549277634,
0.));
#224703=CARTESIAN_POINT('Ctrl Pts',(5.67915655496524,-24.822518122386,0.));
#224704=CARTESIAN_POINT('Ctrl Pts',(5.66163761114903,-24.8019968304618,
0.));
#224705=CARTESIAN_POINT('Ctrl Pts',(5.64421334042247,-24.7814915496728,
0.));
#224706=CARTESIAN_POINT('Ctrl Pts',(5.62688384790918,-24.76100278357,0.));
#224707=CARTESIAN_POINT('Ctrl Pts',(5.60964923798494,-24.7405310372736,
0.));
#224708=CARTESIAN_POINT('Ctrl Pts',(5.59250961323995,-24.7200768119079,
0.));
#224709=CARTESIAN_POINT('Ctrl Pts',(5.57546507427766,-24.6996406035507,
0.));
#224710=CARTESIAN_POINT('Ctrl Pts',(5.55851572025389,-24.6792229061785,
0.));
#224711=CARTESIAN_POINT('Ctrl Pts',(5.54166164919592,-24.6588242134733,
0.));
#224712=CARTESIAN_POINT('Ctrl Pts',(5.52490295840996,-24.6384450211466,
0.));
#224713=CARTESIAN_POINT('Ctrl Pts',(5.50823974481959,-24.618085828918,0.));
#224714=CARTESIAN_POINT('Ctrl Pts',(5.49167210537235,-24.5977471429365,
0.));
#224715=CARTESIAN_POINT('Ctrl Pts',(5.47520013724403,-24.5774294770329,
0.));
#224716=CARTESIAN_POINT('Ctrl Pts',(5.45882393762244,-24.5571333514841,
0.));
#224717=CARTESIAN_POINT('Ctrl Pts',(5.44254360356865,-24.5368592922861,
0.));
#224718=CARTESIAN_POINT('Ctrl Pts',(5.42635923183411,-24.5166078302107,
0.));
#224719=CARTESIAN_POINT('Ctrl Pts',(5.41027091869242,-24.4963794999831,
0.));
#224720=CARTESIAN_POINT('Ctrl Pts',(5.3942787597383,-24.4761748393322,0.));
#224721=CARTESIAN_POINT('Ctrl Pts',(5.37838284973706,-24.4559943883159,
0.));
#224722=CARTESIAN_POINT('Ctrl Pts',(5.36258328273639,-24.4358386899152,
0.));
#224723=CARTESIAN_POINT('Ctrl Pts',(5.34688015213546,-24.4157082904615,
0.));
#224724=CARTESIAN_POINT('Ctrl Pts',(5.33127355076036,-24.3956037401293,
0.));
#224725=CARTESIAN_POINT('Ctrl Pts',(5.31576357092524,-24.3755255933917,
0.));
#224726=CARTESIAN_POINT('Ctrl Pts',(5.30035030449058,-24.3554744095075,
0.));
#224727=CARTESIAN_POINT('Ctrl Pts',(5.28503384290644,-24.3354507529415,
0.));
#224728=CARTESIAN_POINT('Ctrl Pts',(5.26981427718796,-24.3154551932222,
0.));
#224729=CARTESIAN_POINT('Ctrl Pts',(5.25469169788855,-24.2954883048448,
0.));
#224730=CARTESIAN_POINT('Ctrl Pts',(5.23966619506289,-24.2755506671526,
0.));
#224731=CARTESIAN_POINT('Ctrl Pts',(5.22473785822441,-24.2556428642294,
0.));
#224732=CARTESIAN_POINT('Ctrl Pts',(5.20990677629173,-24.2357654847765,
0.));
#224733=CARTESIAN_POINT('Ctrl Pts',(5.19517303753642,-24.215919122017,0.));
#224734=CARTESIAN_POINT('Ctrl Pts',(5.18053672961392,-24.1961043738754,
0.));
#224735=CARTESIAN_POINT('Ctrl Pts',(5.16599793957979,-24.1763218431343,
0.));
#224736=CARTESIAN_POINT('Ctrl Pts',(5.15155675390075,-24.1565721375971,
0.));
#224737=CARTESIAN_POINT('Ctrl Pts',(5.13721325845744,-24.1368558702443,
0.));
#224738=CARTESIAN_POINT('Ctrl Pts',(5.12296753853859,-24.117173659394,0.));
#224739=CARTESIAN_POINT('Ctrl Pts',(5.10881967883132,-24.0975261288446,
0.));
#224740=CARTESIAN_POINT('Ctrl Pts',(5.09476976342625,-24.0779139079266,
0.));
#224741=CARTESIAN_POINT('Ctrl Pts',(5.08081787581276,-24.0583376315638,
0.));
#224742=CARTESIAN_POINT('Ctrl Pts',(5.06696409886641,-24.0387979403268,
0.));
#224743=CARTESIAN_POINT('Ctrl Pts',(5.05320851483065,-24.0192954804896,
0.));
#224744=CARTESIAN_POINT('Ctrl Pts',(5.03955120528521,-23.9998309040746,
0.));
#224745=CARTESIAN_POINT('Ctrl Pts',(5.02599225112454,-23.9804048689227,
0.));
#224746=CARTESIAN_POINT('Ctrl Pts',(5.01253173257452,-23.9610180388271,
0.));
#224747=CARTESIAN_POINT('Ctrl Pts',(4.99916972919306,-23.9416710836529,
0.));
#224748=CARTESIAN_POINT('Ctrl Pts',(4.98590631986532,-23.9223646794592,
0.));
#224749=CARTESIAN_POINT('Ctrl Pts',(4.97274158279226,-23.9030995086163,
0.));
#224750=CARTESIAN_POINT('Ctrl Pts',(4.9596755954656,-23.8838762599218,0.));
#224751=CARTESIAN_POINT('Ctrl Pts',(4.9467084346586,-23.8646956287168,0.));
#224752=CARTESIAN_POINT('Ctrl Pts',(4.93384017643432,-23.8455583170057,
0.));
#224753=CARTESIAN_POINT('Ctrl Pts',(4.92107089613968,-23.8264650335717,
0.));
#224754=CARTESIAN_POINT('Ctrl Pts',(4.90840066839344,-23.8074164940896,
0.));
#224755=CARTESIAN_POINT('Ctrl Pts',(4.89582956706775,-23.7884134212384,
0.));
#224756=CARTESIAN_POINT('Ctrl Pts',(4.88335766525573,-23.7694565448049,
0.));
#224757=CARTESIAN_POINT('Ctrl Pts',(4.87098503527152,-23.7505466018245,
0.));
#224758=CARTESIAN_POINT('Ctrl Pts',(4.85871174865499,-23.7316843367313,
0.));
#224759=CARTESIAN_POINT('Ctrl Pts',(4.84653787616425,-23.7128705015017,
0.));
#224760=CARTESIAN_POINT('Ctrl Pts',(4.83446348776265,-23.6941058557971,
0.));
#224761=CARTESIAN_POINT('Ctrl Pts',(4.82248865259562,-23.675391167102,0.));
#224762=CARTESIAN_POINT('Ctrl Pts',(4.81061343896432,-23.6567272108628,
0.));
#224763=CARTESIAN_POINT('Ctrl Pts',(4.7988379143322,-23.6381147706579,0.));
#224764=CARTESIAN_POINT('Ctrl Pts',(4.78716214532097,-23.6195546383624,
0.));
#224765=CARTESIAN_POINT('Ctrl Pts',(4.77558619769872,-23.6010476143099,
0.));
#224766=CARTESIAN_POINT('Ctrl Pts',(4.76411013636251,-23.5825945074535,
0.));
#224767=CARTESIAN_POINT('Ctrl Pts',(4.75273402530617,-23.5641961355168,
0.));
#224768=CARTESIAN_POINT('Ctrl Pts',(4.74145792760698,-23.545853325171,0.));
#224769=CARTESIAN_POINT('Ctrl Pts',(4.73028190543029,-23.5275669122372,
0.));
#224770=CARTESIAN_POINT('Ctrl Pts',(4.71920602001901,-23.509337741878,0.));
#224771=CARTESIAN_POINT('Ctrl Pts',(4.70823033167818,-23.491166668789,0.));
#224772=CARTESIAN_POINT('Ctrl Pts',(4.69735489975024,-23.4730545573853,
0.));
#224773=CARTESIAN_POINT('Ctrl Pts',(4.68657978258303,-23.455002281986,0.));
#224774=CARTESIAN_POINT('Ctrl Pts',(4.67590503753058,-23.4370107270451,
0.));
#224775=CARTESIAN_POINT('Ctrl Pts',(4.6653307209467,-23.4190807873803,0.));
#224776=CARTESIAN_POINT('Ctrl Pts',(4.65485688816924,-23.4012133683959,
0.));
#224777=CARTESIAN_POINT('Ctrl Pts',(4.6444835934993,-23.3834093863068,0.));
#224778=CARTESIAN_POINT('Ctrl Pts',(4.63421089016541,-23.3656697683489,
0.));
#224779=CARTESIAN_POINT('Ctrl Pts',(4.62403883030805,-23.3479954530272,
0.));
#224780=CARTESIAN_POINT('Ctrl Pts',(4.6139674649783,-23.3303873903938,0.));
#224781=CARTESIAN_POINT('Ctrl Pts',(4.60399684412163,-23.3128465423115,
0.));
#224782=CARTESIAN_POINT('Ctrl Pts',(4.5941270165575,-23.2953738827191,0.));
#224783=CARTESIAN_POINT('Ctrl Pts',(4.5843580299469,-23.2779703978876,0.));
#224784=CARTESIAN_POINT('Ctrl Pts',(4.57468993076097,-23.2606370866866,
0.));
#224785=CARTESIAN_POINT('Ctrl Pts',(4.56512276427839,-23.2433749609131,
0.));
#224786=CARTESIAN_POINT('Ctrl Pts',(4.55565657456975,-23.2261850456064,
0.));
#224787=CARTESIAN_POINT('Ctrl Pts',(4.54629140447544,-23.2090683793629,
0.));
#224788=CARTESIAN_POINT('Ctrl Pts',(4.53702729557566,-23.1920260146465,
0.));
#224789=CARTESIAN_POINT('Ctrl Pts',(4.52786428815014,-23.1750590180908,
0.));
#224790=CARTESIAN_POINT('Ctrl Pts',(4.51880242116748,-23.1581684708761,
0.));
#224791=CARTESIAN_POINT('Ctrl Pts',(4.5098417322706,-23.1413554691123,0.));
#224792=CARTESIAN_POINT('Ctrl Pts',(4.50098225775171,-23.1246211242115,
0.));
#224793=CARTESIAN_POINT('Ctrl Pts',(4.49222403252216,-23.1079665632636,
0.));
#224794=CARTESIAN_POINT('Ctrl Pts',(4.48356709006788,-23.0913929293922,
0.));
#224795=CARTESIAN_POINT('Ctrl Pts',(4.47501146242856,-23.0749013821881,
0.));
#224796=CARTESIAN_POINT('Ctrl Pts',(4.4665571801823,-23.0584930981732,0.));
#224797=CARTESIAN_POINT('Ctrl Pts',(4.45820427241683,-23.0421692712467,
0.));
#224798=CARTESIAN_POINT('Ctrl Pts',(4.44995276669686,-23.0259311131392,
0.));
#224799=CARTESIAN_POINT('Ctrl Pts',(4.44180268901643,-23.0097798538395,
0.));
#224800=CARTESIAN_POINT('Ctrl Pts',(4.43375406376879,-22.9937167421006,
0.));
#224801=CARTESIAN_POINT('Ctrl Pts',(4.42580691372751,-22.977743046002,0.));
#224802=CARTESIAN_POINT('Ctrl Pts',(4.41796126001302,-22.9618600534866,
0.));
#224803=CARTESIAN_POINT('Ctrl Pts',(4.41021712205553,-22.9460690729093,
0.));
#224804=CARTESIAN_POINT('Ctrl Pts',(4.40257451754323,-22.930371433555,0.));
#224805=CARTESIAN_POINT('Ctrl Pts',(4.39503346238473,-22.9147684862426,
0.));
#224806=CARTESIAN_POINT('Ctrl Pts',(4.38759397068405,-22.8992616040108,
0.));
#224807=CARTESIAN_POINT('Ctrl Pts',(4.38025605470092,-22.8838521827701,
0.));
#224808=CARTESIAN_POINT('Ctrl Pts',(4.37301972480745,-22.8685416419725,
0.));
#224809=CARTESIAN_POINT('Ctrl Pts',(4.36588498942997,-22.8533314252422,
0.));
#224810=CARTESIAN_POINT('Ctrl Pts',(4.35885185500546,-22.8382230011184,
0.));
#224811=CARTESIAN_POINT('Ctrl Pts',(4.3519203259479,-22.8232178638876,0.));
#224812=CARTESIAN_POINT('Ctrl Pts',(4.34509040460062,-22.8083175343791,
0.));
#224813=CARTESIAN_POINT('Ctrl Pts',(4.33836209118446,-22.7935235607806,
0.));
#224814=CARTESIAN_POINT('Ctrl Pts',(4.33173538373189,-22.7788375194076,
0.));
#224815=CARTESIAN_POINT('Ctrl Pts',(4.32521027803754,-22.7642610156475,
0.));
#224816=CARTESIAN_POINT('Ctrl Pts',(4.31878676761235,-22.7497956849848,
0.));
#224817=CARTESIAN_POINT('Ctrl Pts',(4.31246484362549,-22.7354431939926,
0.));
#224818=CARTESIAN_POINT('Ctrl Pts',(4.30624449484069,-22.7212052413386,
0.));
#224819=CARTESIAN_POINT('Ctrl Pts',(4.3001257075406,-22.7070835587564,0.));
#224820=CARTESIAN_POINT('Ctrl Pts',(4.29410846547056,-22.6930799122548,
0.));
#224821=CARTESIAN_POINT('Ctrl Pts',(4.28819274977763,-22.6791961033538,
0.));
#224822=CARTESIAN_POINT('Ctrl Pts',(4.28237853894058,-22.6654339703109,
0.));
#224823=CARTESIAN_POINT('Ctrl Pts',(4.2766658086912,-22.6517953893303,0.));
#224824=CARTESIAN_POINT('Ctrl Pts',(4.27105453193004,-22.6382822758172,
0.));
#224825=CARTESIAN_POINT('Ctrl Pts',(4.26554467865576,-22.6248965859977,
0.));
#224826=CARTESIAN_POINT('Ctrl Pts',(4.26013621588305,-22.6116403184821,
0.));
#224827=CARTESIAN_POINT('Ctrl Pts',(4.25482910755481,-22.5985155158636,
0.));
#224828=CARTESIAN_POINT('Ctrl Pts',(4.24962331444177,-22.5855242662477,
0.));
#224829=CARTESIAN_POINT('Ctrl Pts',(4.24451879404851,-22.572668704992,0.));
#224830=CARTESIAN_POINT('Ctrl Pts',(4.23951550052522,-22.5599510166429,
0.));
#224831=CARTESIAN_POINT('Ctrl Pts',(4.23461338456712,-22.5473734368086,
0.));
#224832=CARTESIAN_POINT('Ctrl Pts',(4.22981239330733,-22.5349382540588,
0.));
#224833=CARTESIAN_POINT('Ctrl Pts',(4.22511247020041,-22.5226478117886,
0.));
#224834=CARTESIAN_POINT('Ctrl Pts',(4.22051355490196,-22.5105045108881,
0.));
#224835=CARTESIAN_POINT('Ctrl Pts',(4.21601558313906,-22.4985108124228,
0.));
#224836=CARTESIAN_POINT('Ctrl Pts',(4.21161848657428,-22.4866692403147,
0.));
#224837=CARTESIAN_POINT('Ctrl Pts',(4.20732219265648,-22.4749823839917,
0.));
#224838=CARTESIAN_POINT('Ctrl Pts',(4.20312662448174,-22.4634529011437,
0.));
#224839=CARTESIAN_POINT('Ctrl Pts',(4.19903170066358,-22.4520835205422,
0.));
#224840=CARTESIAN_POINT('Ctrl Pts',(4.1950373351886,-22.4408770448917,0.));
#224841=CARTESIAN_POINT('Ctrl Pts',(4.19114343726932,-22.4298363535416,
0.));
#224842=CARTESIAN_POINT('Ctrl Pts',(4.18734991117707,-22.4189644056109,
0.));
#224843=CARTESIAN_POINT('Ctrl Pts',(4.18365665600839,-22.4082642454448,
0.));
#224844=CARTESIAN_POINT('Ctrl Pts',(4.18006356544879,-22.3977390078074,
0.));
#224845=CARTESIAN_POINT('Ctrl Pts',(4.17657052752834,-22.3873919231339,
0.));
#224846=CARTESIAN_POINT('Ctrl Pts',(4.17317742436162,-22.3772263228624,
0.));
#224847=CARTESIAN_POINT('Ctrl Pts',(4.16988413199469,-22.3672456427605,
0.));
#224848=CARTESIAN_POINT('Ctrl Pts',(4.16669052026602,-22.3574534257397,
0.));
#224849=CARTESIAN_POINT('Ctrl Pts',(4.1635964526318,-22.3478533253886,0.));
#224850=CARTESIAN_POINT('Ctrl Pts',(4.16060178604153,-22.3384491078599,
0.));
#224851=CARTESIAN_POINT('Ctrl Pts',(4.15770637047882,-22.3292446628957,
0.));
#224852=CARTESIAN_POINT('Ctrl Pts',(4.15491004835278,-22.3202440186979,
0.));
#224853=CARTESIAN_POINT('Ctrl Pts',(4.15221265396992,-22.3114513545186,
0.));
#224854=CARTESIAN_POINT('Ctrl Pts',(4.14961401285525,-22.3028710166935,
0.));
#224855=CARTESIAN_POINT('Ctrl Pts',(4.14711394168559,-22.2945075198468,
0.));
#224856=CARTESIAN_POINT('Ctrl Pts',(4.14471224859295,-22.2863655389167,
0.));
#224857=CARTESIAN_POINT('Ctrl Pts',(4.14240873321982,-22.2784499072026,
0.));
#224858=CARTESIAN_POINT('Ctrl Pts',(4.14020318715987,-22.2707656042456,
0.));
#224859=CARTESIAN_POINT('Ctrl Pts',(4.13809539255418,-22.263317791397,0.));
#224860=CARTESIAN_POINT('Ctrl Pts',(4.13608511977226,-22.2561118708422,
0.));
#224861=CARTESIAN_POINT('Ctrl Pts',(4.13417212558808,-22.2491535317789,
0.));
#224862=CARTESIAN_POINT('Ctrl Pts',(4.1323561506016,-22.2424488153523,0.));
#224863=CARTESIAN_POINT('Ctrl Pts',(4.13063692157499,-22.2360040565534,
0.));
#224864=CARTESIAN_POINT('Ctrl Pts',(4.12901415463378,-22.2298258043947,
0.));
#224865=CARTESIAN_POINT('Ctrl Pts',(4.12748755830099,-22.2239207458781,
0.));
#224866=CARTESIAN_POINT('Ctrl Pts',(4.12605683613299,-22.2182956401341,
0.));
#224867=CARTESIAN_POINT('Ctrl Pts',(4.12472167516602,-22.2129576146671,
0.));
#224868=CARTESIAN_POINT('Ctrl Pts',(4.12348173702024,-22.2079143941719,
0.));
#224869=CARTESIAN_POINT('Ctrl Pts',(4.12233664408237,-22.2031746532106,
0.));
#224870=CARTESIAN_POINT('Ctrl Pts',(4.12128598183533,-22.1987479618246,
0.));
#224871=CARTESIAN_POINT('Ctrl Pts',(4.12032932637738,-22.1946440958098,
0.));
#224872=CARTESIAN_POINT('Ctrl Pts',(4.11946626228623,-22.1908725908525,
0.));
#224873=CARTESIAN_POINT('Ctrl Pts',(4.11869641271752,-22.1874419861496,
0.));
#224874=CARTESIAN_POINT('Ctrl Pts',(4.11801938107464,-22.1843613164855,
0.));
#224875=CARTESIAN_POINT('Ctrl Pts',(4.11743469691765,-22.1816414985788,
0.));
#224876=CARTESIAN_POINT('Ctrl Pts',(4.11694173195041,-22.179297473024,0.));
#224877=CARTESIAN_POINT('Ctrl Pts',(4.11653973150558,-22.177347426894,0.));
#224878=CARTESIAN_POINT('Ctrl Pts',(4.11622797217066,-22.1758088296598,
0.));
#224879=CARTESIAN_POINT('Ctrl Pts',(4.11600589882767,-22.1746949858773,
0.));
#224880=CARTESIAN_POINT('Ctrl Pts',(4.11589976826061,-22.174148802123,0.));
#224881=CARTESIAN_POINT('Ctrl Pts',(4.1158603587821,-22.1739341411684,0.));
#224882=CARTESIAN_POINT('Ctrl Pts',(4.11585194677412,-22.1738776823239,
0.));
#224883=CARTESIAN_POINT('Ctrl Pts',(4.11585220600461,-22.1738711152697,
0.));
#224884=CARTESIAN_POINT('',(6.08833931617698,-25.2771067246846,12.));
#224885=CARTESIAN_POINT('',(6.08833931617698,-25.2771067246846,0.));
#224886=CARTESIAN_POINT('Ctrl Pts',(4.11585220600461,-22.1738711152697,
12.));
#224887=CARTESIAN_POINT('Ctrl Pts',(4.11585194677412,-22.1738776823239,
12.));
#224888=CARTESIAN_POINT('Ctrl Pts',(4.1158603587821,-22.1739341411684,12.));
#224889=CARTESIAN_POINT('Ctrl Pts',(4.11589976826061,-22.174148802123,12.));
#224890=CARTESIAN_POINT('Ctrl Pts',(4.11600589882767,-22.1746949858773,
12.));
#224891=CARTESIAN_POINT('Ctrl Pts',(4.11622797217066,-22.1758088296598,
12.));
#224892=CARTESIAN_POINT('Ctrl Pts',(4.11653973150558,-22.177347426894,12.));
#224893=CARTESIAN_POINT('Ctrl Pts',(4.11694173195041,-22.179297473024,12.));
#224894=CARTESIAN_POINT('Ctrl Pts',(4.11743469691765,-22.1816414985788,
12.));
#224895=CARTESIAN_POINT('Ctrl Pts',(4.11801938107464,-22.1843613164855,
12.));
#224896=CARTESIAN_POINT('Ctrl Pts',(4.11869641271752,-22.1874419861496,
12.));
#224897=CARTESIAN_POINT('Ctrl Pts',(4.11946626228623,-22.1908725908525,
12.));
#224898=CARTESIAN_POINT('Ctrl Pts',(4.12032932637738,-22.1946440958098,
12.));
#224899=CARTESIAN_POINT('Ctrl Pts',(4.12128598183533,-22.1987479618246,
12.));
#224900=CARTESIAN_POINT('Ctrl Pts',(4.12233664408237,-22.2031746532106,
12.));
#224901=CARTESIAN_POINT('Ctrl Pts',(4.12348173702024,-22.2079143941719,
12.));
#224902=CARTESIAN_POINT('Ctrl Pts',(4.12472167516602,-22.2129576146671,
12.));
#224903=CARTESIAN_POINT('Ctrl Pts',(4.12605683613299,-22.2182956401341,
12.));
#224904=CARTESIAN_POINT('Ctrl Pts',(4.12748755830099,-22.2239207458781,
12.));
#224905=CARTESIAN_POINT('Ctrl Pts',(4.12901415463378,-22.2298258043947,
12.));
#224906=CARTESIAN_POINT('Ctrl Pts',(4.13063692157499,-22.2360040565534,
12.));
#224907=CARTESIAN_POINT('Ctrl Pts',(4.1323561506016,-22.2424488153523,12.));
#224908=CARTESIAN_POINT('Ctrl Pts',(4.13417212558808,-22.2491535317789,
12.));
#224909=CARTESIAN_POINT('Ctrl Pts',(4.13608511977226,-22.2561118708422,
12.));
#224910=CARTESIAN_POINT('Ctrl Pts',(4.13809539255418,-22.263317791397,12.));
#224911=CARTESIAN_POINT('Ctrl Pts',(4.14020318715987,-22.2707656042456,
12.));
#224912=CARTESIAN_POINT('Ctrl Pts',(4.14240873321982,-22.2784499072026,
12.));
#224913=CARTESIAN_POINT('Ctrl Pts',(4.14471224859295,-22.2863655389167,
12.));
#224914=CARTESIAN_POINT('Ctrl Pts',(4.14711394168559,-22.2945075198468,
12.));
#224915=CARTESIAN_POINT('Ctrl Pts',(4.14961401285525,-22.3028710166935,
12.));
#224916=CARTESIAN_POINT('Ctrl Pts',(4.15221265396992,-22.3114513545186,
12.));
#224917=CARTESIAN_POINT('Ctrl Pts',(4.15491004835278,-22.3202440186979,
12.));
#224918=CARTESIAN_POINT('Ctrl Pts',(4.15770637047882,-22.3292446628957,
12.));
#224919=CARTESIAN_POINT('Ctrl Pts',(4.16060178604153,-22.3384491078599,
12.));
#224920=CARTESIAN_POINT('Ctrl Pts',(4.1635964526318,-22.3478533253886,12.));
#224921=CARTESIAN_POINT('Ctrl Pts',(4.16669052026602,-22.3574534257397,
12.));
#224922=CARTESIAN_POINT('Ctrl Pts',(4.16988413199469,-22.3672456427605,
12.));
#224923=CARTESIAN_POINT('Ctrl Pts',(4.17317742436162,-22.3772263228624,
12.));
#224924=CARTESIAN_POINT('Ctrl Pts',(4.17657052752834,-22.3873919231339,
12.));
#224925=CARTESIAN_POINT('Ctrl Pts',(4.18006356544879,-22.3977390078074,
12.));
#224926=CARTESIAN_POINT('Ctrl Pts',(4.18365665600839,-22.4082642454448,
12.));
#224927=CARTESIAN_POINT('Ctrl Pts',(4.18734991117707,-22.4189644056109,
12.));
#224928=CARTESIAN_POINT('Ctrl Pts',(4.19114343726932,-22.4298363535416,
12.));
#224929=CARTESIAN_POINT('Ctrl Pts',(4.1950373351886,-22.4408770448917,12.));
#224930=CARTESIAN_POINT('Ctrl Pts',(4.19903170066358,-22.4520835205422,
12.));
#224931=CARTESIAN_POINT('Ctrl Pts',(4.20312662448174,-22.4634529011437,
12.));
#224932=CARTESIAN_POINT('Ctrl Pts',(4.20732219265648,-22.4749823839917,
12.));
#224933=CARTESIAN_POINT('Ctrl Pts',(4.21161848657428,-22.4866692403147,
12.));
#224934=CARTESIAN_POINT('Ctrl Pts',(4.21601558313906,-22.4985108124228,
12.));
#224935=CARTESIAN_POINT('Ctrl Pts',(4.22051355490196,-22.5105045108881,
12.));
#224936=CARTESIAN_POINT('Ctrl Pts',(4.22511247020041,-22.5226478117886,
12.));
#224937=CARTESIAN_POINT('Ctrl Pts',(4.22981239330733,-22.5349382540588,
12.));
#224938=CARTESIAN_POINT('Ctrl Pts',(4.23461338456712,-22.5473734368086,
12.));
#224939=CARTESIAN_POINT('Ctrl Pts',(4.23951550052522,-22.5599510166429,
12.));
#224940=CARTESIAN_POINT('Ctrl Pts',(4.24451879404851,-22.572668704992,12.));
#224941=CARTESIAN_POINT('Ctrl Pts',(4.24962331444177,-22.5855242662477,
12.));
#224942=CARTESIAN_POINT('Ctrl Pts',(4.25482910755481,-22.5985155158636,
12.));
#224943=CARTESIAN_POINT('Ctrl Pts',(4.26013621588305,-22.6116403184821,
12.));
#224944=CARTESIAN_POINT('Ctrl Pts',(4.26554467865576,-22.6248965859977,
12.));
#224945=CARTESIAN_POINT('Ctrl Pts',(4.27105453193004,-22.6382822758172,
12.));
#224946=CARTESIAN_POINT('Ctrl Pts',(4.2766658086912,-22.6517953893303,12.));
#224947=CARTESIAN_POINT('Ctrl Pts',(4.28237853894058,-22.6654339703109,
12.));
#224948=CARTESIAN_POINT('Ctrl Pts',(4.28819274977763,-22.6791961033538,
12.));
#224949=CARTESIAN_POINT('Ctrl Pts',(4.29410846547056,-22.6930799122548,
12.));
#224950=CARTESIAN_POINT('Ctrl Pts',(4.3001257075406,-22.7070835587564,12.));
#224951=CARTESIAN_POINT('Ctrl Pts',(4.30624449484069,-22.7212052413386,
12.));
#224952=CARTESIAN_POINT('Ctrl Pts',(4.31246484362549,-22.7354431939926,
12.));
#224953=CARTESIAN_POINT('Ctrl Pts',(4.31878676761235,-22.7497956849848,
12.));
#224954=CARTESIAN_POINT('Ctrl Pts',(4.32521027803754,-22.7642610156475,
12.));
#224955=CARTESIAN_POINT('Ctrl Pts',(4.33173538373189,-22.7788375194076,
12.));
#224956=CARTESIAN_POINT('Ctrl Pts',(4.33836209118446,-22.7935235607806,
12.));
#224957=CARTESIAN_POINT('Ctrl Pts',(4.34509040460062,-22.8083175343791,
12.));
#224958=CARTESIAN_POINT('Ctrl Pts',(4.3519203259479,-22.8232178638876,12.));
#224959=CARTESIAN_POINT('Ctrl Pts',(4.35885185500546,-22.8382230011184,
12.));
#224960=CARTESIAN_POINT('Ctrl Pts',(4.36588498942997,-22.8533314252422,
12.));
#224961=CARTESIAN_POINT('Ctrl Pts',(4.37301972480745,-22.8685416419725,
12.));
#224962=CARTESIAN_POINT('Ctrl Pts',(4.38025605470092,-22.8838521827701,
12.));
#224963=CARTESIAN_POINT('Ctrl Pts',(4.38759397068405,-22.8992616040108,
12.));
#224964=CARTESIAN_POINT('Ctrl Pts',(4.39503346238473,-22.9147684862426,
12.));
#224965=CARTESIAN_POINT('Ctrl Pts',(4.40257451754323,-22.930371433555,12.));
#224966=CARTESIAN_POINT('Ctrl Pts',(4.41021712205553,-22.9460690729093,
12.));
#224967=CARTESIAN_POINT('Ctrl Pts',(4.41796126001302,-22.9618600534866,
12.));
#224968=CARTESIAN_POINT('Ctrl Pts',(4.42580691372751,-22.977743046002,12.));
#224969=CARTESIAN_POINT('Ctrl Pts',(4.43375406376879,-22.9937167421006,
12.));
#224970=CARTESIAN_POINT('Ctrl Pts',(4.44180268901643,-23.0097798538395,
12.));
#224971=CARTESIAN_POINT('Ctrl Pts',(4.44995276669686,-23.0259311131392,
12.));
#224972=CARTESIAN_POINT('Ctrl Pts',(4.45820427241683,-23.0421692712467,
12.));
#224973=CARTESIAN_POINT('Ctrl Pts',(4.4665571801823,-23.0584930981732,12.));
#224974=CARTESIAN_POINT('Ctrl Pts',(4.47501146242856,-23.0749013821881,
12.));
#224975=CARTESIAN_POINT('Ctrl Pts',(4.48356709006788,-23.0913929293922,
12.));
#224976=CARTESIAN_POINT('Ctrl Pts',(4.49222403252216,-23.1079665632636,
12.));
#224977=CARTESIAN_POINT('Ctrl Pts',(4.50098225775171,-23.1246211242115,
12.));
#224978=CARTESIAN_POINT('Ctrl Pts',(4.5098417322706,-23.1413554691123,12.));
#224979=CARTESIAN_POINT('Ctrl Pts',(4.51880242116748,-23.1581684708761,
12.));
#224980=CARTESIAN_POINT('Ctrl Pts',(4.52786428815014,-23.1750590180908,
12.));
#224981=CARTESIAN_POINT('Ctrl Pts',(4.53702729557566,-23.1920260146465,
12.));
#224982=CARTESIAN_POINT('Ctrl Pts',(4.54629140447544,-23.2090683793629,
12.));
#224983=CARTESIAN_POINT('Ctrl Pts',(4.55565657456975,-23.2261850456064,
12.));
#224984=CARTESIAN_POINT('Ctrl Pts',(4.56512276427839,-23.2433749609131,
12.));
#224985=CARTESIAN_POINT('Ctrl Pts',(4.57468993076097,-23.2606370866866,
12.));
#224986=CARTESIAN_POINT('Ctrl Pts',(4.5843580299469,-23.2779703978876,12.));
#224987=CARTESIAN_POINT('Ctrl Pts',(4.5941270165575,-23.2953738827191,12.));
#224988=CARTESIAN_POINT('Ctrl Pts',(4.60399684412163,-23.3128465423115,
12.));
#224989=CARTESIAN_POINT('Ctrl Pts',(4.6139674649783,-23.3303873903938,12.));
#224990=CARTESIAN_POINT('Ctrl Pts',(4.62403883030805,-23.3479954530272,
12.));
#224991=CARTESIAN_POINT('Ctrl Pts',(4.63421089016541,-23.3656697683489,
12.));
#224992=CARTESIAN_POINT('Ctrl Pts',(4.6444835934993,-23.3834093863068,12.));
#224993=CARTESIAN_POINT('Ctrl Pts',(4.65485688816924,-23.4012133683959,
12.));
#224994=CARTESIAN_POINT('Ctrl Pts',(4.6653307209467,-23.4190807873803,12.));
#224995=CARTESIAN_POINT('Ctrl Pts',(4.67590503753058,-23.4370107270451,
12.));
#224996=CARTESIAN_POINT('Ctrl Pts',(4.68657978258303,-23.455002281986,12.));
#224997=CARTESIAN_POINT('Ctrl Pts',(4.69735489975024,-23.4730545573853,
12.));
#224998=CARTESIAN_POINT('Ctrl Pts',(4.70823033167818,-23.491166668789,12.));
#224999=CARTESIAN_POINT('Ctrl Pts',(4.71920602001901,-23.509337741878,12.));
#225000=CARTESIAN_POINT('Ctrl Pts',(4.73028190543029,-23.5275669122372,
12.));
#225001=CARTESIAN_POINT('Ctrl Pts',(4.74145792760698,-23.545853325171,12.));
#225002=CARTESIAN_POINT('Ctrl Pts',(4.75273402530617,-23.5641961355168,
12.));
#225003=CARTESIAN_POINT('Ctrl Pts',(4.76411013636251,-23.5825945074535,
12.));
#225004=CARTESIAN_POINT('Ctrl Pts',(4.77558619769872,-23.6010476143099,
12.));
#225005=CARTESIAN_POINT('Ctrl Pts',(4.78716214532097,-23.6195546383624,
12.));
#225006=CARTESIAN_POINT('Ctrl Pts',(4.7988379143322,-23.6381147706579,12.));
#225007=CARTESIAN_POINT('Ctrl Pts',(4.81061343896432,-23.6567272108628,
12.));
#225008=CARTESIAN_POINT('Ctrl Pts',(4.82248865259562,-23.675391167102,12.));
#225009=CARTESIAN_POINT('Ctrl Pts',(4.83446348776265,-23.6941058557971,
12.));
#225010=CARTESIAN_POINT('Ctrl Pts',(4.84653787616425,-23.7128705015017,
12.));
#225011=CARTESIAN_POINT('Ctrl Pts',(4.85871174865499,-23.7316843367313,
12.));
#225012=CARTESIAN_POINT('Ctrl Pts',(4.87098503527152,-23.7505466018245,
12.));
#225013=CARTESIAN_POINT('Ctrl Pts',(4.88335766525573,-23.7694565448049,
12.));
#225014=CARTESIAN_POINT('Ctrl Pts',(4.89582956706775,-23.7884134212384,
12.));
#225015=CARTESIAN_POINT('Ctrl Pts',(4.90840066839344,-23.8074164940896,
12.));
#225016=CARTESIAN_POINT('Ctrl Pts',(4.92107089613968,-23.8264650335717,
12.));
#225017=CARTESIAN_POINT('Ctrl Pts',(4.93384017643432,-23.8455583170057,
12.));
#225018=CARTESIAN_POINT('Ctrl Pts',(4.9467084346586,-23.8646956287168,12.));
#225019=CARTESIAN_POINT('Ctrl Pts',(4.9596755954656,-23.8838762599218,12.));
#225020=CARTESIAN_POINT('Ctrl Pts',(4.97274158279226,-23.9030995086163,
12.));
#225021=CARTESIAN_POINT('Ctrl Pts',(4.98590631986532,-23.9223646794592,
12.));
#225022=CARTESIAN_POINT('Ctrl Pts',(4.99916972919306,-23.9416710836529,
12.));
#225023=CARTESIAN_POINT('Ctrl Pts',(5.01253173257452,-23.9610180388271,
12.));
#225024=CARTESIAN_POINT('Ctrl Pts',(5.02599225112454,-23.9804048689227,
12.));
#225025=CARTESIAN_POINT('Ctrl Pts',(5.03955120528521,-23.9998309040746,
12.));
#225026=CARTESIAN_POINT('Ctrl Pts',(5.05320851483065,-24.0192954804896,
12.));
#225027=CARTESIAN_POINT('Ctrl Pts',(5.06696409886641,-24.0387979403268,
12.));
#225028=CARTESIAN_POINT('Ctrl Pts',(5.08081787581276,-24.0583376315638,
12.));
#225029=CARTESIAN_POINT('Ctrl Pts',(5.09476976342625,-24.0779139079266,
12.));
#225030=CARTESIAN_POINT('Ctrl Pts',(5.10881967883132,-24.0975261288446,
12.));
#225031=CARTESIAN_POINT('Ctrl Pts',(5.12296753853859,-24.117173659394,12.));
#225032=CARTESIAN_POINT('Ctrl Pts',(5.13721325845744,-24.1368558702443,
12.));
#225033=CARTESIAN_POINT('Ctrl Pts',(5.15155675390075,-24.1565721375971,
12.));
#225034=CARTESIAN_POINT('Ctrl Pts',(5.16599793957979,-24.1763218431343,
12.));
#225035=CARTESIAN_POINT('Ctrl Pts',(5.18053672961392,-24.1961043738754,
12.));
#225036=CARTESIAN_POINT('Ctrl Pts',(5.19517303753642,-24.215919122017,12.));
#225037=CARTESIAN_POINT('Ctrl Pts',(5.20990677629173,-24.2357654847765,
12.));
#225038=CARTESIAN_POINT('Ctrl Pts',(5.22473785822441,-24.2556428642294,
12.));
#225039=CARTESIAN_POINT('Ctrl Pts',(5.23966619506289,-24.2755506671526,
12.));
#225040=CARTESIAN_POINT('Ctrl Pts',(5.25469169788855,-24.2954883048448,
12.));
#225041=CARTESIAN_POINT('Ctrl Pts',(5.26981427718796,-24.3154551932222,
12.));
#225042=CARTESIAN_POINT('Ctrl Pts',(5.28503384290644,-24.3354507529415,
12.));
#225043=CARTESIAN_POINT('Ctrl Pts',(5.30035030449058,-24.3554744095075,
12.));
#225044=CARTESIAN_POINT('Ctrl Pts',(5.31576357092524,-24.3755255933917,
12.));
#225045=CARTESIAN_POINT('Ctrl Pts',(5.33127355076036,-24.3956037401293,
12.));
#225046=CARTESIAN_POINT('Ctrl Pts',(5.34688015213546,-24.4157082904615,
12.));
#225047=CARTESIAN_POINT('Ctrl Pts',(5.36258328273639,-24.4358386899152,
12.));
#225048=CARTESIAN_POINT('Ctrl Pts',(5.37838284973706,-24.4559943883159,
12.));
#225049=CARTESIAN_POINT('Ctrl Pts',(5.3942787597383,-24.4761748393322,12.));
#225050=CARTESIAN_POINT('Ctrl Pts',(5.41027091869242,-24.4963794999831,
12.));
#225051=CARTESIAN_POINT('Ctrl Pts',(5.42635923183411,-24.5166078302107,
12.));
#225052=CARTESIAN_POINT('Ctrl Pts',(5.44254360356865,-24.5368592922861,
12.));
#225053=CARTESIAN_POINT('Ctrl Pts',(5.45882393762244,-24.5571333514841,
12.));
#225054=CARTESIAN_POINT('Ctrl Pts',(5.47520013724403,-24.5774294770329,
12.));
#225055=CARTESIAN_POINT('Ctrl Pts',(5.49167210537235,-24.5977471429365,
12.));
#225056=CARTESIAN_POINT('Ctrl Pts',(5.50823974481959,-24.618085828918,12.));
#225057=CARTESIAN_POINT('Ctrl Pts',(5.52490295840996,-24.6384450211466,
12.));
#225058=CARTESIAN_POINT('Ctrl Pts',(5.54166164919592,-24.6588242134733,
12.));
#225059=CARTESIAN_POINT('Ctrl Pts',(5.55851572025389,-24.6792229061785,
12.));
#225060=CARTESIAN_POINT('Ctrl Pts',(5.57546507427766,-24.6996406035507,
12.));
#225061=CARTESIAN_POINT('Ctrl Pts',(5.59250961323995,-24.7200768119079,
12.));
#225062=CARTESIAN_POINT('Ctrl Pts',(5.60964923798494,-24.7405310372736,
12.));
#225063=CARTESIAN_POINT('Ctrl Pts',(5.62688384790918,-24.76100278357,12.));
#225064=CARTESIAN_POINT('Ctrl Pts',(5.64421334042247,-24.7814915496728,
12.));
#225065=CARTESIAN_POINT('Ctrl Pts',(5.66163761114903,-24.8019968304618,
12.));
#225066=CARTESIAN_POINT('Ctrl Pts',(5.67915655496524,-24.822518122386,12.));
#225067=CARTESIAN_POINT('Ctrl Pts',(5.69677006679429,-24.8430549277634,
12.));
#225068=CARTESIAN_POINT('Ctrl Pts',(5.71447804252019,-24.8636067597677,
12.));
#225069=CARTESIAN_POINT('Ctrl Pts',(5.73228037976926,-24.8841731467219,
12.));
#225070=CARTESIAN_POINT('Ctrl Pts',(5.75017697890812,-24.9047536376467,
12.));
#225071=CARTESIAN_POINT('Ctrl Pts',(5.76816774342236,-24.9253478043632,
12.));
#225072=CARTESIAN_POINT('Ctrl Pts',(5.78625257775702,-24.9459552293308,
12.));
#225073=CARTESIAN_POINT('Ctrl Pts',(5.80443138549747,-24.9665754954463,
12.));
#225074=CARTESIAN_POINT('Ctrl Pts',(5.82270406744213,-24.9872081752709,
12.));
#225075=CARTESIAN_POINT('Ctrl Pts',(5.84107051963073,-25.0078528200558,
12.));
#225076=CARTESIAN_POINT('Ctrl Pts',(5.8595306315681,-25.0285089498922,12.));
#225077=CARTESIAN_POINT('Ctrl Pts',(5.87808428385329,-25.0491760405965,
12.));
#225078=CARTESIAN_POINT('Ctrl Pts',(5.89673135155458,-25.0698535426593,
12.));
#225079=CARTESIAN_POINT('Ctrl Pts',(5.91547170844382,-25.0905409050863,
12.));
#225080=CARTESIAN_POINT('Ctrl Pts',(5.93430523086776,-25.1112375971182,
12.));
#225081=CARTESIAN_POINT('Ctrl Pts',(5.95323180187347,-25.1319431317273,
12.));
#225082=CARTESIAN_POINT('Ctrl Pts',(5.97225131495636,-25.1526570863065,
12.));
#225083=CARTESIAN_POINT('Ctrl Pts',(5.99136367859838,-25.1733791296154,
12.));
#225084=CARTESIAN_POINT('Ctrl Pts',(6.0105688180476,-25.1941090269638,12.));
#225085=CARTESIAN_POINT('Ctrl Pts',(6.02986667390187,-25.2148466201368,
12.));
#225086=CARTESIAN_POINT('Ctrl Pts',(6.04925720151412,-25.2355918138798,
12.));
#225087=CARTESIAN_POINT('Ctrl Pts',(6.06484373634696,-25.2521940105523,
12.));
#225088=CARTESIAN_POINT('Ctrl Pts',(6.07657531787577,-25.2646490489816,
12.));
#225089=CARTESIAN_POINT('Ctrl Pts',(6.08441489609824,-25.2729539149479,
12.));
#225090=CARTESIAN_POINT('Ctrl Pts',(6.08833931617698,-25.2771067246846,
12.));
#225091=CARTESIAN_POINT('Ctrl Pts',(1.76341220531179,-22.4835757167854,
0.));
#225092=CARTESIAN_POINT('Ctrl Pts',(1.76341220531179,-22.4835757167854,
12.));
#225093=CARTESIAN_POINT('Ctrl Pts',(1.76341415538764,-22.483581992979,0.));
#225094=CARTESIAN_POINT('Ctrl Pts',(1.76341415538764,-22.483581992979,12.));
#225095=CARTESIAN_POINT('Ctrl Pts',(1.7634206426357,-22.4836387052232,0.));
#225096=CARTESIAN_POINT('Ctrl Pts',(1.7634206426357,-22.4836387052232,12.));
#225097=CARTESIAN_POINT('Ctrl Pts',(1.76343813434565,-22.483856251707,0.));
#225098=CARTESIAN_POINT('Ctrl Pts',(1.76343813434565,-22.483856251707,12.));
#225099=CARTESIAN_POINT('Ctrl Pts',(1.76347698284791,-22.4844112933129,
0.));
#225100=CARTESIAN_POINT('Ctrl Pts',(1.76347698284791,-22.4844112933129,
12.));
#225101=CARTESIAN_POINT('Ctrl Pts',(1.76355076045546,-22.4855446605991,
0.));
#225102=CARTESIAN_POINT('Ctrl Pts',(1.76355076045546,-22.4855446605991,
12.));
#225103=CARTESIAN_POINT('Ctrl Pts',(1.76364784232963,-22.4871115206571,
0.));
#225104=CARTESIAN_POINT('Ctrl Pts',(1.76364784232963,-22.4871115206571,
12.));
#225105=CARTESIAN_POINT('Ctrl Pts',(1.76376424879504,-22.4890991659478,
0.));
#225106=CARTESIAN_POINT('Ctrl Pts',(1.76376424879504,-22.4890991659478,
12.));
#225107=CARTESIAN_POINT('Ctrl Pts',(1.76389475965723,-22.4914909094908,
0.));
#225108=CARTESIAN_POINT('Ctrl Pts',(1.76389475965723,-22.4914909094908,
12.));
#225109=CARTESIAN_POINT('Ctrl Pts',(1.764033938803,-22.4942693792449,0.));
#225110=CARTESIAN_POINT('Ctrl Pts',(1.764033938803,-22.4942693792449,12.));
#225111=CARTESIAN_POINT('Ctrl Pts',(1.76417731243462,-22.4974203063191,
0.));
#225112=CARTESIAN_POINT('Ctrl Pts',(1.76417731243462,-22.4974203063191,
12.));
#225113=CARTESIAN_POINT('Ctrl Pts',(1.76432160068725,-22.5009332677316,
0.));
#225114=CARTESIAN_POINT('Ctrl Pts',(1.76432160068725,-22.5009332677316,
12.));
#225115=CARTESIAN_POINT('Ctrl Pts',(1.76446408210366,-22.5047996391978,
0.));
#225116=CARTESIAN_POINT('Ctrl Pts',(1.76446408210366,-22.5047996391978,
12.));
#225117=CARTESIAN_POINT('Ctrl Pts',(1.76460218257323,-22.5090112700212,
0.));
#225118=CARTESIAN_POINT('Ctrl Pts',(1.76460218257323,-22.5090112700212,
12.));
#225119=CARTESIAN_POINT('Ctrl Pts',(1.76473303281158,-22.5135590569554,
0.));
#225120=CARTESIAN_POINT('Ctrl Pts',(1.76473303281158,-22.5135590569554,
12.));
#225121=CARTESIAN_POINT('Ctrl Pts',(1.76485369319896,-22.5184336670207,
0.));
#225122=CARTESIAN_POINT('Ctrl Pts',(1.76485369319896,-22.5184336670207,
12.));
#225123=CARTESIAN_POINT('Ctrl Pts',(1.76496128643369,-22.5236259635515,
0.));
#225124=CARTESIAN_POINT('Ctrl Pts',(1.76496128643369,-22.5236259635515,
12.));
#225125=CARTESIAN_POINT('Ctrl Pts',(1.76505320262751,-22.529127665298,0.));
#225126=CARTESIAN_POINT('Ctrl Pts',(1.76505320262751,-22.529127665298,12.));
#225127=CARTESIAN_POINT('Ctrl Pts',(1.7651271156325,-22.5349313983571,0.));
#225128=CARTESIAN_POINT('Ctrl Pts',(1.7651271156325,-22.5349313983571,12.));
#225129=CARTESIAN_POINT('Ctrl Pts',(1.76518087841492,-22.5410303590891,
0.));
#225130=CARTESIAN_POINT('Ctrl Pts',(1.76518087841492,-22.5410303590891,
12.));
#225131=CARTESIAN_POINT('Ctrl Pts',(1.76521245524047,-22.5474180954006,
0.));
#225132=CARTESIAN_POINT('Ctrl Pts',(1.76521245524047,-22.5474180954006,
12.));
#225133=CARTESIAN_POINT('Ctrl Pts',(1.76521983384062,-22.5540882235837,
0.));
#225134=CARTESIAN_POINT('Ctrl Pts',(1.76521983384062,-22.5540882235837,
12.));
#225135=CARTESIAN_POINT('Ctrl Pts',(1.76520104500449,-22.5610344912501,
0.));
#225136=CARTESIAN_POINT('Ctrl Pts',(1.76520104500449,-22.5610344912501,
12.));
#225137=CARTESIAN_POINT('Ctrl Pts',(1.76515418518829,-22.5682508499873,
0.));
#225138=CARTESIAN_POINT('Ctrl Pts',(1.76515418518829,-22.5682508499873,
12.));
#225139=CARTESIAN_POINT('Ctrl Pts',(1.76507744026747,-22.5757315316355,
0.));
#225140=CARTESIAN_POINT('Ctrl Pts',(1.76507744026747,-22.5757315316355,
12.));
#225141=CARTESIAN_POINT('Ctrl Pts',(1.76496910283088,-22.5834711038024,
0.));
#225142=CARTESIAN_POINT('Ctrl Pts',(1.76496910283088,-22.5834711038024,
12.));
#225143=CARTESIAN_POINT('Ctrl Pts',(1.76482755288411,-22.5914644078106,
0.));
#225144=CARTESIAN_POINT('Ctrl Pts',(1.76482755288411,-22.5914644078106,
12.));
#225145=CARTESIAN_POINT('Ctrl Pts',(1.76465124413556,-22.5997065145638,
0.));
#225146=CARTESIAN_POINT('Ctrl Pts',(1.76465124413556,-22.5997065145638,
12.));
#225147=CARTESIAN_POINT('Ctrl Pts',(1.76443868648015,-22.6081926681342,
0.));
#225148=CARTESIAN_POINT('Ctrl Pts',(1.76443868648015,-22.6081926681342,
12.));
#225149=CARTESIAN_POINT('Ctrl Pts',(1.76418843543739,-22.6169182517693,
0.));
#225150=CARTESIAN_POINT('Ctrl Pts',(1.76418843543739,-22.6169182517693,
12.));
#225151=CARTESIAN_POINT('Ctrl Pts',(1.76389909571402,-22.6258787994847,
0.));
#225152=CARTESIAN_POINT('Ctrl Pts',(1.76389909571402,-22.6258787994847,
12.));
#225153=CARTESIAN_POINT('Ctrl Pts',(1.76356932176272,-22.635069997936,0.));
#225154=CARTESIAN_POINT('Ctrl Pts',(1.76356932176272,-22.635069997936,12.));
#225155=CARTESIAN_POINT('Ctrl Pts',(1.76319782013913,-22.6444876940425,
0.));
#225156=CARTESIAN_POINT('Ctrl Pts',(1.76319782013913,-22.6444876940425,
12.));
#225157=CARTESIAN_POINT('Ctrl Pts',(1.76278334912559,-22.6541278938413,
0.));
#225158=CARTESIAN_POINT('Ctrl Pts',(1.76278334912559,-22.6541278938413,
12.));
#225159=CARTESIAN_POINT('Ctrl Pts',(1.76232471392567,-22.6639867471756,
0.));
#225160=CARTESIAN_POINT('Ctrl Pts',(1.76232471392567,-22.6639867471756,
12.));
#225161=CARTESIAN_POINT('Ctrl Pts',(1.76182076289525,-22.6740605356699,
0.));
#225162=CARTESIAN_POINT('Ctrl Pts',(1.76182076289525,-22.6740605356699,
12.));
#225163=CARTESIAN_POINT('Ctrl Pts',(1.76127038310612,-22.6843456585245,
0.));
#225164=CARTESIAN_POINT('Ctrl Pts',(1.76127038310612,-22.6843456585245,
12.));
#225165=CARTESIAN_POINT('Ctrl Pts',(1.76067249704884,-22.6948386219843,
0.));
#225166=CARTESIAN_POINT('Ctrl Pts',(1.76067249704884,-22.6948386219843,
12.));
#225167=CARTESIAN_POINT('Ctrl Pts',(1.76002606202398,-22.7055360375481,
0.));
#225168=CARTESIAN_POINT('Ctrl Pts',(1.76002606202398,-22.7055360375481,
12.));
#225169=CARTESIAN_POINT('Ctrl Pts',(1.75933006905924,-22.7164346186007,
0.));
#225170=CARTESIAN_POINT('Ctrl Pts',(1.75933006905924,-22.7164346186007,
12.));
#225171=CARTESIAN_POINT('Ctrl Pts',(1.75858354204634,-22.7275311777305,
0.));
#225172=CARTESIAN_POINT('Ctrl Pts',(1.75858354204634,-22.7275311777305,
12.));
#225173=CARTESIAN_POINT('Ctrl Pts',(1.75778553673249,-22.7388226235565,
0.));
#225174=CARTESIAN_POINT('Ctrl Pts',(1.75778553673249,-22.7388226235565,
12.));
#225175=CARTESIAN_POINT('Ctrl Pts',(1.75693513908911,-22.7503059556455,
0.));
#225176=CARTESIAN_POINT('Ctrl Pts',(1.75693513908911,-22.7503059556455,
12.));
#225177=CARTESIAN_POINT('Ctrl Pts',(1.7560314637164,-22.7619782595013,0.));
#225178=CARTESIAN_POINT('Ctrl Pts',(1.7560314637164,-22.7619782595013,12.));
#225179=CARTESIAN_POINT('Ctrl Pts',(1.75507365227127,-22.7738367016115,
0.));
#225180=CARTESIAN_POINT('Ctrl Pts',(1.75507365227127,-22.7738367016115,
12.));
#225181=CARTESIAN_POINT('Ctrl Pts',(1.75406087182929,-22.7858785242358,
0.));
#225182=CARTESIAN_POINT('Ctrl Pts',(1.75406087182929,-22.7858785242358,
12.));
#225183=CARTESIAN_POINT('Ctrl Pts',(1.75299231391461,-22.7981010424312,
0.));
#225184=CARTESIAN_POINT('Ctrl Pts',(1.75299231391461,-22.7981010424312,
12.));
#225185=CARTESIAN_POINT('Ctrl Pts',(1.75186719365589,-22.8105016414712,
0.));
#225186=CARTESIAN_POINT('Ctrl Pts',(1.75186719365589,-22.8105016414712,
12.));
#225187=CARTESIAN_POINT('Ctrl Pts',(1.75068474890883,-22.8230777741285,
0.));
#225188=CARTESIAN_POINT('Ctrl Pts',(1.75068474890883,-22.8230777741285,
12.));
#225189=CARTESIAN_POINT('Ctrl Pts',(1.74944423940117,-22.8358269579854,
0.));
#225190=CARTESIAN_POINT('Ctrl Pts',(1.74944423940117,-22.8358269579854,
12.));
#225191=CARTESIAN_POINT('Ctrl Pts',(1.74814494588491,-22.8487467728075,
0.));
#225192=CARTESIAN_POINT('Ctrl Pts',(1.74814494588491,-22.8487467728075,
12.));
#225193=CARTESIAN_POINT('Ctrl Pts',(1.74678616930663,-22.8618348580234,
0.));
#225194=CARTESIAN_POINT('Ctrl Pts',(1.74678616930663,-22.8618348580234,
12.));
#225195=CARTESIAN_POINT('Ctrl Pts',(1.74536722998199,-22.8750889101696,
0.));
#225196=CARTESIAN_POINT('Ctrl Pts',(1.74536722998199,-22.8750889101696,
12.));
#225197=CARTESIAN_POINT('Ctrl Pts',(1.74388746677702,-22.8885066803351,
0.));
#225198=CARTESIAN_POINT('Ctrl Pts',(1.74388746677702,-22.8885066803351,
12.));
#225199=CARTESIAN_POINT('Ctrl Pts',(1.74234623630079,-22.9020859716144,
0.));
#225200=CARTESIAN_POINT('Ctrl Pts',(1.74234623630079,-22.9020859716144,
12.));
#225201=CARTESIAN_POINT('Ctrl Pts',(1.74074291231056,-22.9158246373365,
0.));
#225202=CARTESIAN_POINT('Ctrl Pts',(1.74074291231056,-22.9158246373365,
12.));
#225203=CARTESIAN_POINT('Ctrl Pts',(1.73907688511664,-22.9297205792587,
0.));
#225204=CARTESIAN_POINT('Ctrl Pts',(1.73907688511664,-22.9297205792587,
12.));
#225205=CARTESIAN_POINT('Ctrl Pts',(1.73734756100038,-22.9437717457825,
0.));
#225206=CARTESIAN_POINT('Ctrl Pts',(1.73734756100038,-22.9437717457825,
12.));
#225207=CARTESIAN_POINT('Ctrl Pts',(1.73555436162771,-22.9579761301062,
0.));
#225208=CARTESIAN_POINT('Ctrl Pts',(1.73555436162771,-22.9579761301062,
12.));
#225209=CARTESIAN_POINT('Ctrl Pts',(1.73369672350817,-22.9723317685688,
0.));
#225210=CARTESIAN_POINT('Ctrl Pts',(1.73369672350817,-22.9723317685688,
12.));
#225211=CARTESIAN_POINT('Ctrl Pts',(1.73177409750193,-22.9868367391978,
0.));
#225212=CARTESIAN_POINT('Ctrl Pts',(1.73177409750193,-22.9868367391978,
12.));
#225213=CARTESIAN_POINT('Ctrl Pts',(1.72978594832137,-23.0014891601891,
0.));
#225214=CARTESIAN_POINT('Ctrl Pts',(1.72978594832137,-23.0014891601891,
12.));
#225215=CARTESIAN_POINT('Ctrl Pts',(1.72773175404702,-23.0162871884167,
0.));
#225216=CARTESIAN_POINT('Ctrl Pts',(1.72773175404702,-23.0162871884167,
12.));
#225217=CARTESIAN_POINT('Ctrl Pts',(1.72561100564033,-23.031229017888,0.));
#225218=CARTESIAN_POINT('Ctrl Pts',(1.72561100564033,-23.031229017888,12.));
#225219=CARTESIAN_POINT('Ctrl Pts',(1.72342320653731,-23.0463128785528,
0.));
#225220=CARTESIAN_POINT('Ctrl Pts',(1.72342320653731,-23.0463128785528,
12.));
#225221=CARTESIAN_POINT('Ctrl Pts',(1.7211678722598,-23.061537035156,0.));
#225222=CARTESIAN_POINT('Ctrl Pts',(1.7211678722598,-23.061537035156,12.));
#225223=CARTESIAN_POINT('Ctrl Pts',(1.71884453003027,-23.0768997860709,
0.));
#225224=CARTESIAN_POINT('Ctrl Pts',(1.71884453003027,-23.0768997860709,
12.));
#225225=CARTESIAN_POINT('Ctrl Pts',(1.71645271839311,-23.0923994621216,
0.));
#225226=CARTESIAN_POINT('Ctrl Pts',(1.71645271839311,-23.0923994621216,
12.));
#225227=CARTESIAN_POINT('Ctrl Pts',(1.71399198684724,-23.1080344254291,
0.));
#225228=CARTESIAN_POINT('Ctrl Pts',(1.71399198684724,-23.1080344254291,
12.));
#225229=CARTESIAN_POINT('Ctrl Pts',(1.71146189552192,-23.1238030684929,
0.));
#225230=CARTESIAN_POINT('Ctrl Pts',(1.71146189552192,-23.1238030684929,
12.));
#225231=CARTESIAN_POINT('Ctrl Pts',(1.70886201485459,-23.1397038132358,
0.));
#225232=CARTESIAN_POINT('Ctrl Pts',(1.70886201485459,-23.1397038132358,
12.));
#225233=CARTESIAN_POINT('Ctrl Pts',(1.70619192527846,-23.1557351100613,
0.));
#225234=CARTESIAN_POINT('Ctrl Pts',(1.70619192527846,-23.1557351100613,
12.));
#225235=CARTESIAN_POINT('Ctrl Pts',(1.70345121691259,-23.1718954368749,
0.));
#225236=CARTESIAN_POINT('Ctrl Pts',(1.70345121691259,-23.1718954368749,
12.));
#225237=CARTESIAN_POINT('Ctrl Pts',(1.70063948926987,-23.1881832981848,
0.));
#225238=CARTESIAN_POINT('Ctrl Pts',(1.70063948926987,-23.1881832981848,
12.));
#225239=CARTESIAN_POINT('Ctrl Pts',(1.69775635099425,-23.2045972243765,
0.));
#225240=CARTESIAN_POINT('Ctrl Pts',(1.69775635099425,-23.2045972243765,
12.));
#225241=CARTESIAN_POINT('Ctrl Pts',(1.69480141959945,-23.2211357709374,
0.));
#225242=CARTESIAN_POINT('Ctrl Pts',(1.69480141959945,-23.2211357709374,
12.));
#225243=CARTESIAN_POINT('Ctrl Pts',(1.69177432121716,-23.2377975177014,
0.));
#225244=CARTESIAN_POINT('Ctrl Pts',(1.69177432121716,-23.2377975177014,
12.));
#225245=CARTESIAN_POINT('Ctrl Pts',(1.6886746903491,-23.2545810680536,0.));
#225246=CARTESIAN_POINT('Ctrl Pts',(1.6886746903491,-23.2545810680536,12.));
#225247=CARTESIAN_POINT('Ctrl Pts',(1.68550216963274,-23.2714850482245,
0.));
#225248=CARTESIAN_POINT('Ctrl Pts',(1.68550216963274,-23.2714850482245,
12.));
#225249=CARTESIAN_POINT('Ctrl Pts',(1.68225640962181,-23.2885081066949,
0.));
#225250=CARTESIAN_POINT('Ctrl Pts',(1.68225640962181,-23.2885081066949,
12.));
#225251=CARTESIAN_POINT('Ctrl Pts',(1.67893706857123,-23.3056489135611,
0.));
#225252=CARTESIAN_POINT('Ctrl Pts',(1.67893706857123,-23.3056489135611,
12.));
#225253=CARTESIAN_POINT('Ctrl Pts',(1.67554381222987,-23.3229061599145,
0.));
#225254=CARTESIAN_POINT('Ctrl Pts',(1.67554381222987,-23.3229061599145,
12.));
#225255=CARTESIAN_POINT('Ctrl Pts',(1.67207631363905,-23.3402785571866,
0.));
#225256=CARTESIAN_POINT('Ctrl Pts',(1.67207631363905,-23.3402785571866,
12.));
#225257=CARTESIAN_POINT('Ctrl Pts',(1.66853425293977,-23.3577648365747,
0.));
#225258=CARTESIAN_POINT('Ctrl Pts',(1.66853425293977,-23.3577648365747,
12.));
#225259=CARTESIAN_POINT('Ctrl Pts',(1.66491731718864,-23.375363748555,0.));
#225260=CARTESIAN_POINT('Ctrl Pts',(1.66491731718864,-23.375363748555,12.));
#225261=CARTESIAN_POINT('Ctrl Pts',(1.66122520018008,-23.3930740623622,
0.));
#225262=CARTESIAN_POINT('Ctrl Pts',(1.66122520018008,-23.3930740623622,
12.));
#225263=CARTESIAN_POINT('Ctrl Pts',(1.65745760227507,-23.4108945654803,
0.));
#225264=CARTESIAN_POINT('Ctrl Pts',(1.65745760227507,-23.4108945654803,
12.));
#225265=CARTESIAN_POINT('Ctrl Pts',(1.6536142302373,-23.4288240631034,0.));
#225266=CARTESIAN_POINT('Ctrl Pts',(1.6536142302373,-23.4288240631034,12.));
#225267=CARTESIAN_POINT('Ctrl Pts',(1.64969479707339,-23.446861377656,0.));
#225268=CARTESIAN_POINT('Ctrl Pts',(1.64969479707339,-23.446861377656,12.));
#225269=CARTESIAN_POINT('Ctrl Pts',(1.64569902187608,-23.4650053483919,
0.));
#225270=CARTESIAN_POINT('Ctrl Pts',(1.64569902187608,-23.4650053483919,
12.));
#225271=CARTESIAN_POINT('Ctrl Pts',(1.64162662967524,-23.4832548309638,
0.));
#225272=CARTESIAN_POINT('Ctrl Pts',(1.64162662967524,-23.4832548309638,
12.));
#225273=CARTESIAN_POINT('Ctrl Pts',(1.63747735129474,-23.5016086970006,
0.));
#225274=CARTESIAN_POINT('Ctrl Pts',(1.63747735129474,-23.5016086970006,
12.));
#225275=CARTESIAN_POINT('Ctrl Pts',(1.63325092321731,-23.5200658336624,
0.));
#225276=CARTESIAN_POINT('Ctrl Pts',(1.63325092321731,-23.5200658336624,
12.));
#225277=CARTESIAN_POINT('Ctrl Pts',(1.62894708745231,-23.5386251432278,
0.));
#225278=CARTESIAN_POINT('Ctrl Pts',(1.62894708745231,-23.5386251432278,
12.));
#225279=CARTESIAN_POINT('Ctrl Pts',(1.62456559140071,-23.5572855427617,
0.));
#225280=CARTESIAN_POINT('Ctrl Pts',(1.62456559140071,-23.5572855427617,
12.));
#225281=CARTESIAN_POINT('Ctrl Pts',(1.62010618772869,-23.5760459637608,
0.));
#225282=CARTESIAN_POINT('Ctrl Pts',(1.62010618772869,-23.5760459637608,
12.));
#225283=CARTESIAN_POINT('Ctrl Pts',(1.61556863424697,-23.5949053517996,
0.));
#225284=CARTESIAN_POINT('Ctrl Pts',(1.61556863424697,-23.5949053517996,
12.));
#225285=CARTESIAN_POINT('Ctrl Pts',(1.61095269379773,-23.6138626661644,
0.));
#225286=CARTESIAN_POINT('Ctrl Pts',(1.61095269379773,-23.6138626661644,
12.));
#225287=CARTESIAN_POINT('Ctrl Pts',(1.60625813414666,-23.6329168794916,
0.));
#225288=CARTESIAN_POINT('Ctrl Pts',(1.60625813414666,-23.6329168794916,
12.));
#225289=CARTESIAN_POINT('Ctrl Pts',(1.60148472786588,-23.6520669774863,
0.));
#225290=CARTESIAN_POINT('Ctrl Pts',(1.60148472786588,-23.6520669774863,
12.));
#225291=CARTESIAN_POINT('Ctrl Pts',(1.59663225222458,-23.6713119586302,
0.));
#225292=CARTESIAN_POINT('Ctrl Pts',(1.59663225222458,-23.6713119586302,
12.));
#225293=CARTESIAN_POINT('Ctrl Pts',(1.59170048908631,-23.6906508338833,
0.));
#225294=CARTESIAN_POINT('Ctrl Pts',(1.59170048908631,-23.6906508338833,
12.));
#225295=CARTESIAN_POINT('Ctrl Pts',(1.58668922481222,-23.7100826263835,
0.));
#225296=CARTESIAN_POINT('Ctrl Pts',(1.58668922481222,-23.7100826263835,
12.));
#225297=CARTESIAN_POINT('Ctrl Pts',(1.58159825017362,-23.7296063711308,
0.));
#225298=CARTESIAN_POINT('Ctrl Pts',(1.58159825017362,-23.7296063711308,
12.));
#225299=CARTESIAN_POINT('Ctrl Pts',(1.57642736025251,-23.7492211147369,
0.));
#225300=CARTESIAN_POINT('Ctrl Pts',(1.57642736025251,-23.7492211147369,
12.));
#225301=CARTESIAN_POINT('Ctrl Pts',(1.57117635434412,-23.7689259151869,
0.));
#225302=CARTESIAN_POINT('Ctrl Pts',(1.57117635434412,-23.7689259151869,
12.));
#225303=CARTESIAN_POINT('Ctrl Pts',(1.56584503586844,-23.788719841588,0.));
#225304=CARTESIAN_POINT('Ctrl Pts',(1.56584503586844,-23.788719841588,12.));
#225305=CARTESIAN_POINT('Ctrl Pts',(1.56043321228631,-23.8086019739192,
0.));
#225306=CARTESIAN_POINT('Ctrl Pts',(1.56043321228631,-23.8086019739192,
12.));
#225307=CARTESIAN_POINT('Ctrl Pts',(1.55494069502627,-23.8285714027631,
0.));
#225308=CARTESIAN_POINT('Ctrl Pts',(1.55494069502627,-23.8285714027631,
12.));
#225309=CARTESIAN_POINT('Ctrl Pts',(1.5493672994053,-23.8486272290698,0.));
#225310=CARTESIAN_POINT('Ctrl Pts',(1.5493672994053,-23.8486272290698,12.));
#225311=CARTESIAN_POINT('Ctrl Pts',(1.54371284453977,-23.8687685639635,
0.));
#225312=CARTESIAN_POINT('Ctrl Pts',(1.54371284453977,-23.8687685639635,
12.));
#225313=CARTESIAN_POINT('Ctrl Pts',(1.53797715326748,-23.8889945285313,
0.));
#225314=CARTESIAN_POINT('Ctrl Pts',(1.53797715326748,-23.8889945285313,
12.));
#225315=CARTESIAN_POINT('Ctrl Pts',(1.53216005207462,-23.9093042536119,
0.));
#225316=CARTESIAN_POINT('Ctrl Pts',(1.53216005207462,-23.9093042536119,
12.));
#225317=CARTESIAN_POINT('Ctrl Pts',(1.52626137103039,-23.9296968795761,
0.));
#225318=CARTESIAN_POINT('Ctrl Pts',(1.52626137103039,-23.9296968795761,
12.));
#225319=CARTESIAN_POINT('Ctrl Pts',(1.52028094372806,-23.9501715561038,
0.));
#225320=CARTESIAN_POINT('Ctrl Pts',(1.52028094372806,-23.9501715561038,
12.));
#225321=CARTESIAN_POINT('Ctrl Pts',(1.51421860720628,-23.9707274420145,
0.));
#225322=CARTESIAN_POINT('Ctrl Pts',(1.51421860720628,-23.9707274420145,
12.));
#225323=CARTESIAN_POINT('Ctrl Pts',(1.50807420187702,-23.991363705093,0.));
#225324=CARTESIAN_POINT('Ctrl Pts',(1.50807420187702,-23.991363705093,12.));
#225325=CARTESIAN_POINT('Ctrl Pts',(1.50184757146099,-24.0120795219086,
0.));
#225326=CARTESIAN_POINT('Ctrl Pts',(1.50184757146099,-24.0120795219086,
12.));
#225327=CARTESIAN_POINT('Ctrl Pts',(1.49553856292798,-24.0328740776331,
0.));
#225328=CARTESIAN_POINT('Ctrl Pts',(1.49553856292798,-24.0328740776331,
12.));
#225329=CARTESIAN_POINT('Ctrl Pts',(1.48914702644883,-24.053746565843,0.));
#225330=CARTESIAN_POINT('Ctrl Pts',(1.48914702644883,-24.053746565843,12.));
#225331=CARTESIAN_POINT('Ctrl Pts',(1.4826728153368,-24.074696188353,0.));
#225332=CARTESIAN_POINT('Ctrl Pts',(1.4826728153368,-24.074696188353,12.));
#225333=CARTESIAN_POINT('Ctrl Pts',(1.47611578597741,-24.0957221550782,
0.));
#225334=CARTESIAN_POINT('Ctrl Pts',(1.47611578597741,-24.0957221550782,
12.));
#225335=CARTESIAN_POINT('Ctrl Pts',(1.46947579776991,-24.1168236838827,
0.));
#225336=CARTESIAN_POINT('Ctrl Pts',(1.46947579776991,-24.1168236838827,
12.));
#225337=CARTESIAN_POINT('Ctrl Pts',(1.46275271307398,-24.1380000004272,
0.));
#225338=CARTESIAN_POINT('Ctrl Pts',(1.46275271307398,-24.1380000004272,
12.));
#225339=CARTESIAN_POINT('Ctrl Pts',(1.45594639716314,-24.1592503380105,
0.));
#225340=CARTESIAN_POINT('Ctrl Pts',(1.45594639716314,-24.1592503380105,
12.));
#225341=CARTESIAN_POINT('Ctrl Pts',(1.4490567181872,-24.1805739374033,0.));
#225342=CARTESIAN_POINT('Ctrl Pts',(1.4490567181872,-24.1805739374033,12.));
#225343=CARTESIAN_POINT('Ctrl Pts',(1.44208354711074,-24.2019700467214,
0.));
#225344=CARTESIAN_POINT('Ctrl Pts',(1.44208354711074,-24.2019700467214,
12.));
#225345=CARTESIAN_POINT('Ctrl Pts',(1.43502675765502,-24.2234379212978,
0.));
#225346=CARTESIAN_POINT('Ctrl Pts',(1.43502675765502,-24.2234379212978,
12.));
#225347=CARTESIAN_POINT('Ctrl Pts',(1.42788622624851,-24.2449768235485,
0.));
#225348=CARTESIAN_POINT('Ctrl Pts',(1.42788622624851,-24.2449768235485,
12.));
#225349=CARTESIAN_POINT('Ctrl Pts',(1.42066183198252,-24.2665860228357,
0.));
#225350=CARTESIAN_POINT('Ctrl Pts',(1.42066183198252,-24.2665860228357,
12.));
#225351=CARTESIAN_POINT('Ctrl Pts',(1.41335345657684,-24.2882647953214,
0.));
#225352=CARTESIAN_POINT('Ctrl Pts',(1.41335345657684,-24.2882647953214,
12.));
#225353=CARTESIAN_POINT('Ctrl Pts',(1.4059609843434,-24.3100124238316,0.));
#225354=CARTESIAN_POINT('Ctrl Pts',(1.4059609843434,-24.3100124238316,12.));
#225355=CARTESIAN_POINT('Ctrl Pts',(1.3984843021281,-24.3318281977647,0.));
#225356=CARTESIAN_POINT('Ctrl Pts',(1.3984843021281,-24.3318281977647,12.));
#225357=CARTESIAN_POINT('Ctrl Pts',(1.3909232992639,-24.3537114129877,0.));
#225358=CARTESIAN_POINT('Ctrl Pts',(1.3909232992639,-24.3537114129877,12.));
#225359=CARTESIAN_POINT('Ctrl Pts',(1.38327786752998,-24.37566137173,0.));
#225360=CARTESIAN_POINT('Ctrl Pts',(1.38327786752998,-24.37566137173,12.));
#225361=CARTESIAN_POINT('Ctrl Pts',(1.37554790111607,-24.3976773824731,
0.));
#225362=CARTESIAN_POINT('Ctrl Pts',(1.37554790111607,-24.3976773824731,
12.));
#225363=CARTESIAN_POINT('Ctrl Pts',(1.36773329659954,-24.4197587598337,
0.));
#225364=CARTESIAN_POINT('Ctrl Pts',(1.36773329659954,-24.4197587598337,
12.));
#225365=CARTESIAN_POINT('Ctrl Pts',(1.35983395290624,-24.4419048244524,
0.));
#225366=CARTESIAN_POINT('Ctrl Pts',(1.35983395290624,-24.4419048244524,
12.));
#225367=CARTESIAN_POINT('Ctrl Pts',(1.35184977125644,-24.4641149028894,
0.));
#225368=CARTESIAN_POINT('Ctrl Pts',(1.35184977125644,-24.4641149028894,
12.));
#225369=CARTESIAN_POINT('Ctrl Pts',(1.34378065512335,-24.4863883275135,
0.));
#225370=CARTESIAN_POINT('Ctrl Pts',(1.34378065512335,-24.4863883275135,
12.));
#225371=CARTESIAN_POINT('Ctrl Pts',(1.33562651019684,-24.5087244363856,
0.));
#225372=CARTESIAN_POINT('Ctrl Pts',(1.33562651019684,-24.5087244363856,
12.));
#225373=CARTESIAN_POINT('Ctrl Pts',(1.32738724435326,-24.5311225731434,
0.));
#225374=CARTESIAN_POINT('Ctrl Pts',(1.32738724435326,-24.5311225731434,
12.));
#225375=CARTESIAN_POINT('Ctrl Pts',(1.31906276763669,-24.5535820868671,
0.));
#225376=CARTESIAN_POINT('Ctrl Pts',(1.31906276763669,-24.5535820868671,
12.));
#225377=CARTESIAN_POINT('Ctrl Pts',(1.31065299222023,-24.576102332018,0.));
#225378=CARTESIAN_POINT('Ctrl Pts',(1.31065299222023,-24.576102332018,12.));
#225379=CARTESIAN_POINT('Ctrl Pts',(1.30215783236363,-24.5986826684025,
0.));
#225380=CARTESIAN_POINT('Ctrl Pts',(1.30215783236363,-24.5986826684025,
12.));
#225381=CARTESIAN_POINT('Ctrl Pts',(1.29357720438107,-24.6213224611228,
0.));
#225382=CARTESIAN_POINT('Ctrl Pts',(1.29357720438107,-24.6213224611228,
12.));
#225383=CARTESIAN_POINT('Ctrl Pts',(1.28491102661513,-24.6440210805278,
0.));
#225384=CARTESIAN_POINT('Ctrl Pts',(1.28491102661513,-24.6440210805278,
12.));
#225385=CARTESIAN_POINT('Ctrl Pts',(1.2761592194164,-24.666777902156,0.));
#225386=CARTESIAN_POINT('Ctrl Pts',(1.2761592194164,-24.666777902156,12.));
#225387=CARTESIAN_POINT('Ctrl Pts',(1.26732170513497,-24.6895923066837,
0.));
#225388=CARTESIAN_POINT('Ctrl Pts',(1.26732170513497,-24.6895923066837,
12.));
#225389=CARTESIAN_POINT('Ctrl Pts',(1.25839840807414,-24.7124636797895,
0.));
#225390=CARTESIAN_POINT('Ctrl Pts',(1.25839840807414,-24.7124636797895,
12.));
#225391=CARTESIAN_POINT('Ctrl Pts',(1.24938925444323,-24.7353914120012,
0.));
#225392=CARTESIAN_POINT('Ctrl Pts',(1.24938925444323,-24.7353914120012,
12.));
#225393=CARTESIAN_POINT('Ctrl Pts',(1.24029417231987,-24.7583748985439,
0.));
#225394=CARTESIAN_POINT('Ctrl Pts',(1.24029417231987,-24.7583748985439,
12.));
#225395=CARTESIAN_POINT('Ctrl Pts',(1.23111309161843,-24.78141353918,0.));
#225396=CARTESIAN_POINT('Ctrl Pts',(1.23111309161843,-24.78141353918,12.));
#225397=CARTESIAN_POINT('Ctrl Pts',(1.22184594406526,-24.8045067380536,
0.));
#225398=CARTESIAN_POINT('Ctrl Pts',(1.22184594406526,-24.8045067380536,
12.));
#225399=CARTESIAN_POINT('Ctrl Pts',(1.21249266318205,-24.8276539035092,
0.));
#225400=CARTESIAN_POINT('Ctrl Pts',(1.21249266318205,-24.8276539035092,
12.));
#225401=CARTESIAN_POINT('Ctrl Pts',(1.20305318426015,-24.8508544481973,
0.));
#225402=CARTESIAN_POINT('Ctrl Pts',(1.20305318426015,-24.8508544481973,
12.));
#225403=CARTESIAN_POINT('Ctrl Pts',(1.19352744434059,-24.8741077892074,
0.));
#225404=CARTESIAN_POINT('Ctrl Pts',(1.19352744434059,-24.8741077892074,
12.));
#225405=CARTESIAN_POINT('Ctrl Pts',(1.18391538220098,-24.8974133481829,
0.));
#225406=CARTESIAN_POINT('Ctrl Pts',(1.18391538220098,-24.8974133481829,
12.));
#225407=CARTESIAN_POINT('Ctrl Pts',(1.17421693835039,-24.9207705514449,
0.));
#225408=CARTESIAN_POINT('Ctrl Pts',(1.17421693835039,-24.9207705514449,
12.));
#225409=CARTESIAN_POINT('Ctrl Pts',(1.16443205502852,-24.9441788300932,
0.));
#225410=CARTESIAN_POINT('Ctrl Pts',(1.16443205502852,-24.9441788300932,
12.));
#225411=CARTESIAN_POINT('Ctrl Pts',(1.15456067621894,-24.9676376201501,
0.));
#225412=CARTESIAN_POINT('Ctrl Pts',(1.15456067621894,-24.9676376201501,
12.));
#225413=CARTESIAN_POINT('Ctrl Pts',(1.14460274758206,-24.9911463621431,
0.));
#225414=CARTESIAN_POINT('Ctrl Pts',(1.14460274758206,-24.9911463621431,
12.));
#225415=CARTESIAN_POINT('Ctrl Pts',(1.13455821638535,-25.0147045006193,
0.));
#225416=CARTESIAN_POINT('Ctrl Pts',(1.13455821638535,-25.0147045006193,
12.));
#225417=CARTESIAN_POINT('Ctrl Pts',(1.12442703144455,-25.0383114836898,
0.));
#225418=CARTESIAN_POINT('Ctrl Pts',(1.12442703144455,-25.0383114836898,
12.));
#225419=CARTESIAN_POINT('Ctrl Pts',(1.1142091430689,-25.0619667625336,0.));
#225420=CARTESIAN_POINT('Ctrl Pts',(1.1142091430689,-25.0619667625336,12.));
#225421=CARTESIAN_POINT('Ctrl Pts',(1.1039045030174,-25.085669790968,0.));
#225422=CARTESIAN_POINT('Ctrl Pts',(1.1039045030174,-25.085669790968,12.));
#225423=CARTESIAN_POINT('Ctrl Pts',(1.09351306445299,-25.1094200248448,
0.));
#225424=CARTESIAN_POINT('Ctrl Pts',(1.09351306445299,-25.1094200248448,
12.));
#225425=CARTESIAN_POINT('Ctrl Pts',(1.08303478197174,-25.1332169227415,
0.));
#225426=CARTESIAN_POINT('Ctrl Pts',(1.08303478197174,-25.1332169227415,
12.));
#225427=CARTESIAN_POINT('Ctrl Pts',(1.07246961165459,-25.1570599469311,
0.));
#225428=CARTESIAN_POINT('Ctrl Pts',(1.07246961165459,-25.1570599469311,
12.));
#225429=CARTESIAN_POINT('Ctrl Pts',(1.06181751111754,-25.1809485642191,
0.));
#225430=CARTESIAN_POINT('Ctrl Pts',(1.06181751111754,-25.1809485642191,
12.));
#225431=CARTESIAN_POINT('Ctrl Pts',(1.05107843957925,-25.2048822469027,
0.));
#225432=CARTESIAN_POINT('Ctrl Pts',(1.05107843957925,-25.2048822469027,
12.));
#225433=CARTESIAN_POINT('Ctrl Pts',(1.04025235791514,-25.2288604735087,
0.));
#225434=CARTESIAN_POINT('Ctrl Pts',(1.04025235791514,-25.2288604735087,
12.));
#225435=CARTESIAN_POINT('Ctrl Pts',(1.0293392287683,-25.2528827300427,0.));
#225436=CARTESIAN_POINT('Ctrl Pts',(1.0293392287683,-25.2528827300427,12.));
#225437=CARTESIAN_POINT('Ctrl Pts',(1.01833901642272,-25.2769485087268,
0.));
#225438=CARTESIAN_POINT('Ctrl Pts',(1.01833901642272,-25.2769485087268,
12.));
#225439=CARTESIAN_POINT('Ctrl Pts',(1.00725168656933,-25.3010573055557,
0.));
#225440=CARTESIAN_POINT('Ctrl Pts',(1.00725168656933,-25.3010573055557,
12.));
#225441=CARTESIAN_POINT('Ctrl Pts',(0.996077206120918,-25.3252086182976,
0.));
#225442=CARTESIAN_POINT('Ctrl Pts',(0.996077206120918,-25.3252086182976,
12.));
#225443=CARTESIAN_POINT('Ctrl Pts',(0.984815543004088,-25.3494019441444,
0.));
#225444=CARTESIAN_POINT('Ctrl Pts',(0.984815543004088,-25.3494019441444,
12.));
#225445=CARTESIAN_POINT('Ctrl Pts',(0.973466666000047,-25.3736367778842,
0.));
#225446=CARTESIAN_POINT('Ctrl Pts',(0.973466666000047,-25.3736367778842,
12.));
#225447=CARTESIAN_POINT('Ctrl Pts',(0.962030544502801,-25.3979126089155,
0.));
#225448=CARTESIAN_POINT('Ctrl Pts',(0.962030544502801,-25.3979126089155,
12.));
#225449=CARTESIAN_POINT('Ctrl Pts',(0.950507148596967,-25.4222289223155,
0.));
#225450=CARTESIAN_POINT('Ctrl Pts',(0.950507148596967,-25.4222289223155,
12.));
#225451=CARTESIAN_POINT('Ctrl Pts',(0.938896449495631,-25.4465852044835,
0.));
#225452=CARTESIAN_POINT('Ctrl Pts',(0.938896449495631,-25.4465852044835,
12.));
#225453=CARTESIAN_POINT('Ctrl Pts',(0.927198419885603,-25.4709809474996,
0.));
#225454=CARTESIAN_POINT('Ctrl Pts',(0.927198419885603,-25.4709809474996,
12.));
#225455=CARTESIAN_POINT('Ctrl Pts',(0.915413034335331,-25.4954156541787,
0.));
#225456=CARTESIAN_POINT('Ctrl Pts',(0.915413034335331,-25.4954156541787,
12.));
#225457=CARTESIAN_POINT('Ctrl Pts',(0.903540269651152,-25.5198888424195,
0.));
#225458=CARTESIAN_POINT('Ctrl Pts',(0.903540269651152,-25.5198888424195,
12.));
#225459=CARTESIAN_POINT('Ctrl Pts',(0.891580105349464,-25.5444000508223,
0.));
#225460=CARTESIAN_POINT('Ctrl Pts',(0.891580105349464,-25.5444000508223,
12.));
#225461=CARTESIAN_POINT('Ctrl Pts',(0.879532523835088,-25.568948840818,
0.));
#225462=CARTESIAN_POINT('Ctrl Pts',(0.879532523835088,-25.568948840818,
12.));
#225463=CARTESIAN_POINT('Ctrl Pts',(0.867397509339468,-25.5935347843616,
0.));
#225464=CARTESIAN_POINT('Ctrl Pts',(0.867397509339468,-25.5935347843616,
12.));
#225465=CARTESIAN_POINT('Ctrl Pts',(0.855175047037614,-25.618157453608,
0.));
#225466=CARTESIAN_POINT('Ctrl Pts',(0.855175047037614,-25.618157453608,
12.));
#225467=CARTESIAN_POINT('Ctrl Pts',(0.842865122121542,-25.6428164100078,
0.));
#225468=CARTESIAN_POINT('Ctrl Pts',(0.842865122121542,-25.6428164100078,
12.));
#225469=CARTESIAN_POINT('Ctrl Pts',(0.830467718864366,-25.6675111931957,
0.));
#225470=CARTESIAN_POINT('Ctrl Pts',(0.830467718864366,-25.6675111931957,
12.));
#225471=CARTESIAN_POINT('Ctrl Pts',(0.817982819786718,-25.6922413110172,
0.));
#225472=CARTESIAN_POINT('Ctrl Pts',(0.817982819786718,-25.6922413110172,
12.));
#225473=CARTESIAN_POINT('Ctrl Pts',(0.805410404552592,-25.7170062262474,
0.));
#225474=CARTESIAN_POINT('Ctrl Pts',(0.805410404552592,-25.7170062262474,
12.));
#225475=CARTESIAN_POINT('Ctrl Pts',(0.792750451613533,-25.7418053757671,
0.));
#225476=CARTESIAN_POINT('Ctrl Pts',(0.792750451613533,-25.7418053757671,
12.));
#225477=CARTESIAN_POINT('Ctrl Pts',(0.780002940289024,-25.7666381946871,
0.));
#225478=CARTESIAN_POINT('Ctrl Pts',(0.780002940289024,-25.7666381946871,
12.));
#225479=CARTESIAN_POINT('Ctrl Pts',(0.767167852648638,-25.7915041383304,
0.));
#225480=CARTESIAN_POINT('Ctrl Pts',(0.767167852648638,-25.7915041383304,
12.));
#225481=CARTESIAN_POINT('Ctrl Pts',(0.754245175608287,-25.816402705995,
0.));
#225482=CARTESIAN_POINT('Ctrl Pts',(0.754245175608287,-25.816402705995,
12.));
#225483=CARTESIAN_POINT('Ctrl Pts',(0.741234902664695,-25.841333461908,
0.));
#225484=CARTESIAN_POINT('Ctrl Pts',(0.741234902664695,-25.841333461908,
12.));
#225485=CARTESIAN_POINT('Ctrl Pts',(0.728137036485876,-25.8662960624285,
0.));
#225486=CARTESIAN_POINT('Ctrl Pts',(0.728137036485876,-25.8662960624285,
12.));
#225487=CARTESIAN_POINT('Ctrl Pts',(0.714951588533752,-25.8912902615141,
0.));
#225488=CARTESIAN_POINT('Ctrl Pts',(0.714951588533752,-25.8912902615141,
12.));
#225489=CARTESIAN_POINT('Ctrl Pts',(0.701678575236601,-25.9163158909645,
0.));
#225490=CARTESIAN_POINT('Ctrl Pts',(0.701678575236601,-25.9163158909645,
12.));
#225491=CARTESIAN_POINT('Ctrl Pts',(0.688318015065675,-25.941372847213,
0.));
#225492=CARTESIAN_POINT('Ctrl Pts',(0.688318015065675,-25.941372847213,
12.));
#225493=CARTESIAN_POINT('Ctrl Pts',(0.677559543215902,-25.9614434298092,
0.));
#225494=CARTESIAN_POINT('Ctrl Pts',(0.677559543215902,-25.9614434298092,
12.));
#225495=CARTESIAN_POINT('Ctrl Pts',(0.669451306784414,-25.9765104298171,
0.));
#225496=CARTESIAN_POINT('Ctrl Pts',(0.669451306784414,-25.9765104298171,
12.));
#225497=CARTESIAN_POINT('Ctrl Pts',(0.664028313188911,-25.9865613464809,
0.));
#225498=CARTESIAN_POINT('Ctrl Pts',(0.664028313188911,-25.9865613464809,
12.));
#225499=CARTESIAN_POINT('Ctrl Pts',(0.66131244073089,-25.991588367311,0.));
#225500=CARTESIAN_POINT('Ctrl Pts',(0.66131244073089,-25.991588367311,12.));
#225501=CARTESIAN_POINT('',(0.66131244073089,-25.991588367311,0.));
#225502=CARTESIAN_POINT('Ctrl Pts',(1.76341220531179,-22.4835757167854,
0.));
#225503=CARTESIAN_POINT('Ctrl Pts',(1.76341415538764,-22.483581992979,0.));
#225504=CARTESIAN_POINT('Ctrl Pts',(1.7634206426357,-22.4836387052232,0.));
#225505=CARTESIAN_POINT('Ctrl Pts',(1.76343813434565,-22.483856251707,0.));
#225506=CARTESIAN_POINT('Ctrl Pts',(1.76347698284791,-22.4844112933129,
0.));
#225507=CARTESIAN_POINT('Ctrl Pts',(1.76355076045546,-22.4855446605991,
0.));
#225508=CARTESIAN_POINT('Ctrl Pts',(1.76364784232963,-22.4871115206571,
0.));
#225509=CARTESIAN_POINT('Ctrl Pts',(1.76376424879504,-22.4890991659478,
0.));
#225510=CARTESIAN_POINT('Ctrl Pts',(1.76389475965723,-22.4914909094908,
0.));
#225511=CARTESIAN_POINT('Ctrl Pts',(1.764033938803,-22.4942693792449,0.));
#225512=CARTESIAN_POINT('Ctrl Pts',(1.76417731243462,-22.4974203063191,
0.));
#225513=CARTESIAN_POINT('Ctrl Pts',(1.76432160068725,-22.5009332677316,
0.));
#225514=CARTESIAN_POINT('Ctrl Pts',(1.76446408210366,-22.5047996391978,
0.));
#225515=CARTESIAN_POINT('Ctrl Pts',(1.76460218257323,-22.5090112700212,
0.));
#225516=CARTESIAN_POINT('Ctrl Pts',(1.76473303281158,-22.5135590569554,
0.));
#225517=CARTESIAN_POINT('Ctrl Pts',(1.76485369319896,-22.5184336670207,
0.));
#225518=CARTESIAN_POINT('Ctrl Pts',(1.76496128643369,-22.5236259635515,
0.));
#225519=CARTESIAN_POINT('Ctrl Pts',(1.76505320262751,-22.529127665298,0.));
#225520=CARTESIAN_POINT('Ctrl Pts',(1.7651271156325,-22.5349313983571,0.));
#225521=CARTESIAN_POINT('Ctrl Pts',(1.76518087841492,-22.5410303590891,
0.));
#225522=CARTESIAN_POINT('Ctrl Pts',(1.76521245524047,-22.5474180954006,
0.));
#225523=CARTESIAN_POINT('Ctrl Pts',(1.76521983384062,-22.5540882235837,
0.));
#225524=CARTESIAN_POINT('Ctrl Pts',(1.76520104500449,-22.5610344912501,
0.));
#225525=CARTESIAN_POINT('Ctrl Pts',(1.76515418518829,-22.5682508499873,
0.));
#225526=CARTESIAN_POINT('Ctrl Pts',(1.76507744026747,-22.5757315316355,
0.));
#225527=CARTESIAN_POINT('Ctrl Pts',(1.76496910283088,-22.5834711038024,
0.));
#225528=CARTESIAN_POINT('Ctrl Pts',(1.76482755288411,-22.5914644078106,
0.));
#225529=CARTESIAN_POINT('Ctrl Pts',(1.76465124413556,-22.5997065145638,
0.));
#225530=CARTESIAN_POINT('Ctrl Pts',(1.76443868648015,-22.6081926681342,
0.));
#225531=CARTESIAN_POINT('Ctrl Pts',(1.76418843543739,-22.6169182517693,
0.));
#225532=CARTESIAN_POINT('Ctrl Pts',(1.76389909571402,-22.6258787994847,
0.));
#225533=CARTESIAN_POINT('Ctrl Pts',(1.76356932176272,-22.635069997936,0.));
#225534=CARTESIAN_POINT('Ctrl Pts',(1.76319782013913,-22.6444876940425,
0.));
#225535=CARTESIAN_POINT('Ctrl Pts',(1.76278334912559,-22.6541278938413,
0.));
#225536=CARTESIAN_POINT('Ctrl Pts',(1.76232471392567,-22.6639867471756,
0.));
#225537=CARTESIAN_POINT('Ctrl Pts',(1.76182076289525,-22.6740605356699,
0.));
#225538=CARTESIAN_POINT('Ctrl Pts',(1.76127038310612,-22.6843456585245,
0.));
#225539=CARTESIAN_POINT('Ctrl Pts',(1.76067249704884,-22.6948386219843,
0.));
#225540=CARTESIAN_POINT('Ctrl Pts',(1.76002606202398,-22.7055360375481,
0.));
#225541=CARTESIAN_POINT('Ctrl Pts',(1.75933006905924,-22.7164346186007,
0.));
#225542=CARTESIAN_POINT('Ctrl Pts',(1.75858354204634,-22.7275311777305,
0.));
#225543=CARTESIAN_POINT('Ctrl Pts',(1.75778553673249,-22.7388226235565,
0.));
#225544=CARTESIAN_POINT('Ctrl Pts',(1.75693513908911,-22.7503059556455,
0.));
#225545=CARTESIAN_POINT('Ctrl Pts',(1.7560314637164,-22.7619782595013,0.));
#225546=CARTESIAN_POINT('Ctrl Pts',(1.75507365227127,-22.7738367016115,
0.));
#225547=CARTESIAN_POINT('Ctrl Pts',(1.75406087182929,-22.7858785242358,
0.));
#225548=CARTESIAN_POINT('Ctrl Pts',(1.75299231391461,-22.7981010424312,
0.));
#225549=CARTESIAN_POINT('Ctrl Pts',(1.75186719365589,-22.8105016414712,
0.));
#225550=CARTESIAN_POINT('Ctrl Pts',(1.75068474890883,-22.8230777741285,
0.));
#225551=CARTESIAN_POINT('Ctrl Pts',(1.74944423940117,-22.8358269579854,
0.));
#225552=CARTESIAN_POINT('Ctrl Pts',(1.74814494588491,-22.8487467728075,
0.));
#225553=CARTESIAN_POINT('Ctrl Pts',(1.74678616930663,-22.8618348580234,
0.));
#225554=CARTESIAN_POINT('Ctrl Pts',(1.74536722998199,-22.8750889101696,
0.));
#225555=CARTESIAN_POINT('Ctrl Pts',(1.74388746677702,-22.8885066803351,
0.));
#225556=CARTESIAN_POINT('Ctrl Pts',(1.74234623630079,-22.9020859716144,
0.));
#225557=CARTESIAN_POINT('Ctrl Pts',(1.74074291231056,-22.9158246373365,
0.));
#225558=CARTESIAN_POINT('Ctrl Pts',(1.73907688511664,-22.9297205792587,
0.));
#225559=CARTESIAN_POINT('Ctrl Pts',(1.73734756100038,-22.9437717457825,
0.));
#225560=CARTESIAN_POINT('Ctrl Pts',(1.73555436162771,-22.9579761301062,
0.));
#225561=CARTESIAN_POINT('Ctrl Pts',(1.73369672350817,-22.9723317685688,
0.));
#225562=CARTESIAN_POINT('Ctrl Pts',(1.73177409750193,-22.9868367391978,
0.));
#225563=CARTESIAN_POINT('Ctrl Pts',(1.72978594832137,-23.0014891601891,
0.));
#225564=CARTESIAN_POINT('Ctrl Pts',(1.72773175404702,-23.0162871884167,
0.));
#225565=CARTESIAN_POINT('Ctrl Pts',(1.72561100564033,-23.031229017888,0.));
#225566=CARTESIAN_POINT('Ctrl Pts',(1.72342320653731,-23.0463128785528,
0.));
#225567=CARTESIAN_POINT('Ctrl Pts',(1.7211678722598,-23.061537035156,0.));
#225568=CARTESIAN_POINT('Ctrl Pts',(1.71884453003027,-23.0768997860709,
0.));
#225569=CARTESIAN_POINT('Ctrl Pts',(1.71645271839311,-23.0923994621216,
0.));
#225570=CARTESIAN_POINT('Ctrl Pts',(1.71399198684724,-23.1080344254291,
0.));
#225571=CARTESIAN_POINT('Ctrl Pts',(1.71146189552192,-23.1238030684929,
0.));
#225572=CARTESIAN_POINT('Ctrl Pts',(1.70886201485459,-23.1397038132358,
0.));
#225573=CARTESIAN_POINT('Ctrl Pts',(1.70619192527846,-23.1557351100613,
0.));
#225574=CARTESIAN_POINT('Ctrl Pts',(1.70345121691259,-23.1718954368749,
0.));
#225575=CARTESIAN_POINT('Ctrl Pts',(1.70063948926987,-23.1881832981848,
0.));
#225576=CARTESIAN_POINT('Ctrl Pts',(1.69775635099425,-23.2045972243765,
0.));
#225577=CARTESIAN_POINT('Ctrl Pts',(1.69480141959945,-23.2211357709374,
0.));
#225578=CARTESIAN_POINT('Ctrl Pts',(1.69177432121716,-23.2377975177014,
0.));
#225579=CARTESIAN_POINT('Ctrl Pts',(1.6886746903491,-23.2545810680536,0.));
#225580=CARTESIAN_POINT('Ctrl Pts',(1.68550216963274,-23.2714850482245,
0.));
#225581=CARTESIAN_POINT('Ctrl Pts',(1.68225640962181,-23.2885081066949,
0.));
#225582=CARTESIAN_POINT('Ctrl Pts',(1.67893706857123,-23.3056489135611,
0.));
#225583=CARTESIAN_POINT('Ctrl Pts',(1.67554381222987,-23.3229061599145,
0.));
#225584=CARTESIAN_POINT('Ctrl Pts',(1.67207631363905,-23.3402785571866,
0.));
#225585=CARTESIAN_POINT('Ctrl Pts',(1.66853425293977,-23.3577648365747,
0.));
#225586=CARTESIAN_POINT('Ctrl Pts',(1.66491731718864,-23.375363748555,0.));
#225587=CARTESIAN_POINT('Ctrl Pts',(1.66122520018008,-23.3930740623622,
0.));
#225588=CARTESIAN_POINT('Ctrl Pts',(1.65745760227507,-23.4108945654803,
0.));
#225589=CARTESIAN_POINT('Ctrl Pts',(1.6536142302373,-23.4288240631034,0.));
#225590=CARTESIAN_POINT('Ctrl Pts',(1.64969479707339,-23.446861377656,0.));
#225591=CARTESIAN_POINT('Ctrl Pts',(1.64569902187608,-23.4650053483919,
0.));
#225592=CARTESIAN_POINT('Ctrl Pts',(1.64162662967524,-23.4832548309638,
0.));
#225593=CARTESIAN_POINT('Ctrl Pts',(1.63747735129474,-23.5016086970006,
0.));
#225594=CARTESIAN_POINT('Ctrl Pts',(1.63325092321731,-23.5200658336624,
0.));
#225595=CARTESIAN_POINT('Ctrl Pts',(1.62894708745231,-23.5386251432278,
0.));
#225596=CARTESIAN_POINT('Ctrl Pts',(1.62456559140071,-23.5572855427617,
0.));
#225597=CARTESIAN_POINT('Ctrl Pts',(1.62010618772869,-23.5760459637608,
0.));
#225598=CARTESIAN_POINT('Ctrl Pts',(1.61556863424697,-23.5949053517996,
0.));
#225599=CARTESIAN_POINT('Ctrl Pts',(1.61095269379773,-23.6138626661644,
0.));
#225600=CARTESIAN_POINT('Ctrl Pts',(1.60625813414666,-23.6329168794916,
0.));
#225601=CARTESIAN_POINT('Ctrl Pts',(1.60148472786588,-23.6520669774863,
0.));
#225602=CARTESIAN_POINT('Ctrl Pts',(1.59663225222458,-23.6713119586302,
0.));
#225603=CARTESIAN_POINT('Ctrl Pts',(1.59170048908631,-23.6906508338833,
0.));
#225604=CARTESIAN_POINT('Ctrl Pts',(1.58668922481222,-23.7100826263835,
0.));
#225605=CARTESIAN_POINT('Ctrl Pts',(1.58159825017362,-23.7296063711308,
0.));
#225606=CARTESIAN_POINT('Ctrl Pts',(1.57642736025251,-23.7492211147369,
0.));
#225607=CARTESIAN_POINT('Ctrl Pts',(1.57117635434412,-23.7689259151869,
0.));
#225608=CARTESIAN_POINT('Ctrl Pts',(1.56584503586844,-23.788719841588,0.));
#225609=CARTESIAN_POINT('Ctrl Pts',(1.56043321228631,-23.8086019739192,
0.));
#225610=CARTESIAN_POINT('Ctrl Pts',(1.55494069502627,-23.8285714027631,
0.));
#225611=CARTESIAN_POINT('Ctrl Pts',(1.5493672994053,-23.8486272290698,0.));
#225612=CARTESIAN_POINT('Ctrl Pts',(1.54371284453977,-23.8687685639635,
0.));
#225613=CARTESIAN_POINT('Ctrl Pts',(1.53797715326748,-23.8889945285313,
0.));
#225614=CARTESIAN_POINT('Ctrl Pts',(1.53216005207462,-23.9093042536119,
0.));
#225615=CARTESIAN_POINT('Ctrl Pts',(1.52626137103039,-23.9296968795761,
0.));
#225616=CARTESIAN_POINT('Ctrl Pts',(1.52028094372806,-23.9501715561038,
0.));
#225617=CARTESIAN_POINT('Ctrl Pts',(1.51421860720628,-23.9707274420145,
0.));
#225618=CARTESIAN_POINT('Ctrl Pts',(1.50807420187702,-23.991363705093,0.));
#225619=CARTESIAN_POINT('Ctrl Pts',(1.50184757146099,-24.0120795219086,
0.));
#225620=CARTESIAN_POINT('Ctrl Pts',(1.49553856292798,-24.0328740776331,
0.));
#225621=CARTESIAN_POINT('Ctrl Pts',(1.48914702644883,-24.053746565843,0.));
#225622=CARTESIAN_POINT('Ctrl Pts',(1.4826728153368,-24.074696188353,0.));
#225623=CARTESIAN_POINT('Ctrl Pts',(1.47611578597741,-24.0957221550782,
0.));
#225624=CARTESIAN_POINT('Ctrl Pts',(1.46947579776991,-24.1168236838827,
0.));
#225625=CARTESIAN_POINT('Ctrl Pts',(1.46275271307398,-24.1380000004272,
0.));
#225626=CARTESIAN_POINT('Ctrl Pts',(1.45594639716314,-24.1592503380105,
0.));
#225627=CARTESIAN_POINT('Ctrl Pts',(1.4490567181872,-24.1805739374033,0.));
#225628=CARTESIAN_POINT('Ctrl Pts',(1.44208354711074,-24.2019700467214,
0.));
#225629=CARTESIAN_POINT('Ctrl Pts',(1.43502675765502,-24.2234379212978,
0.));
#225630=CARTESIAN_POINT('Ctrl Pts',(1.42788622624851,-24.2449768235485,
0.));
#225631=CARTESIAN_POINT('Ctrl Pts',(1.42066183198252,-24.2665860228357,
0.));
#225632=CARTESIAN_POINT('Ctrl Pts',(1.41335345657684,-24.2882647953214,
0.));
#225633=CARTESIAN_POINT('Ctrl Pts',(1.4059609843434,-24.3100124238316,0.));
#225634=CARTESIAN_POINT('Ctrl Pts',(1.3984843021281,-24.3318281977647,0.));
#225635=CARTESIAN_POINT('Ctrl Pts',(1.3909232992639,-24.3537114129877,0.));
#225636=CARTESIAN_POINT('Ctrl Pts',(1.38327786752998,-24.37566137173,0.));
#225637=CARTESIAN_POINT('Ctrl Pts',(1.37554790111607,-24.3976773824731,
0.));
#225638=CARTESIAN_POINT('Ctrl Pts',(1.36773329659954,-24.4197587598337,
0.));
#225639=CARTESIAN_POINT('Ctrl Pts',(1.35983395290624,-24.4419048244524,
0.));
#225640=CARTESIAN_POINT('Ctrl Pts',(1.35184977125644,-24.4641149028894,
0.));
#225641=CARTESIAN_POINT('Ctrl Pts',(1.34378065512335,-24.4863883275135,
0.));
#225642=CARTESIAN_POINT('Ctrl Pts',(1.33562651019684,-24.5087244363856,
0.));
#225643=CARTESIAN_POINT('Ctrl Pts',(1.32738724435326,-24.5311225731434,
0.));
#225644=CARTESIAN_POINT('Ctrl Pts',(1.31906276763669,-24.5535820868671,
0.));
#225645=CARTESIAN_POINT('Ctrl Pts',(1.31065299222023,-24.576102332018,0.));
#225646=CARTESIAN_POINT('Ctrl Pts',(1.30215783236363,-24.5986826684025,
0.));
#225647=CARTESIAN_POINT('Ctrl Pts',(1.29357720438107,-24.6213224611228,
0.));
#225648=CARTESIAN_POINT('Ctrl Pts',(1.28491102661513,-24.6440210805278,
0.));
#225649=CARTESIAN_POINT('Ctrl Pts',(1.2761592194164,-24.666777902156,0.));
#225650=CARTESIAN_POINT('Ctrl Pts',(1.26732170513497,-24.6895923066837,
0.));
#225651=CARTESIAN_POINT('Ctrl Pts',(1.25839840807414,-24.7124636797895,
0.));
#225652=CARTESIAN_POINT('Ctrl Pts',(1.24938925444323,-24.7353914120012,
0.));
#225653=CARTESIAN_POINT('Ctrl Pts',(1.24029417231987,-24.7583748985439,
0.));
#225654=CARTESIAN_POINT('Ctrl Pts',(1.23111309161843,-24.78141353918,0.));
#225655=CARTESIAN_POINT('Ctrl Pts',(1.22184594406526,-24.8045067380536,
0.));
#225656=CARTESIAN_POINT('Ctrl Pts',(1.21249266318205,-24.8276539035092,
0.));
#225657=CARTESIAN_POINT('Ctrl Pts',(1.20305318426015,-24.8508544481973,
0.));
#225658=CARTESIAN_POINT('Ctrl Pts',(1.19352744434059,-24.8741077892074,
0.));
#225659=CARTESIAN_POINT('Ctrl Pts',(1.18391538220098,-24.8974133481829,
0.));
#225660=CARTESIAN_POINT('Ctrl Pts',(1.17421693835039,-24.9207705514449,
0.));
#225661=CARTESIAN_POINT('Ctrl Pts',(1.16443205502852,-24.9441788300932,
0.));
#225662=CARTESIAN_POINT('Ctrl Pts',(1.15456067621894,-24.9676376201501,
0.));
#225663=CARTESIAN_POINT('Ctrl Pts',(1.14460274758206,-24.9911463621431,
0.));
#225664=CARTESIAN_POINT('Ctrl Pts',(1.13455821638535,-25.0147045006193,
0.));
#225665=CARTESIAN_POINT('Ctrl Pts',(1.12442703144455,-25.0383114836898,
0.));
#225666=CARTESIAN_POINT('Ctrl Pts',(1.1142091430689,-25.0619667625336,0.));
#225667=CARTESIAN_POINT('Ctrl Pts',(1.1039045030174,-25.085669790968,0.));
#225668=CARTESIAN_POINT('Ctrl Pts',(1.09351306445299,-25.1094200248448,
0.));
#225669=CARTESIAN_POINT('Ctrl Pts',(1.08303478197174,-25.1332169227415,
0.));
#225670=CARTESIAN_POINT('Ctrl Pts',(1.07246961165459,-25.1570599469311,
0.));
#225671=CARTESIAN_POINT('Ctrl Pts',(1.06181751111754,-25.1809485642191,
0.));
#225672=CARTESIAN_POINT('Ctrl Pts',(1.05107843957925,-25.2048822469027,
0.));
#225673=CARTESIAN_POINT('Ctrl Pts',(1.04025235791514,-25.2288604735087,
0.));
#225674=CARTESIAN_POINT('Ctrl Pts',(1.0293392287683,-25.2528827300427,0.));
#225675=CARTESIAN_POINT('Ctrl Pts',(1.01833901642272,-25.2769485087268,
0.));
#225676=CARTESIAN_POINT('Ctrl Pts',(1.00725168656933,-25.3010573055557,
0.));
#225677=CARTESIAN_POINT('Ctrl Pts',(0.996077206120918,-25.3252086182976,
0.));
#225678=CARTESIAN_POINT('Ctrl Pts',(0.984815543004088,-25.3494019441444,
0.));
#225679=CARTESIAN_POINT('Ctrl Pts',(0.973466666000047,-25.3736367778842,
0.));
#225680=CARTESIAN_POINT('Ctrl Pts',(0.962030544502801,-25.3979126089155,
0.));
#225681=CARTESIAN_POINT('Ctrl Pts',(0.950507148596967,-25.4222289223155,
0.));
#225682=CARTESIAN_POINT('Ctrl Pts',(0.938896449495631,-25.4465852044835,
0.));
#225683=CARTESIAN_POINT('Ctrl Pts',(0.927198419885603,-25.4709809474996,
0.));
#225684=CARTESIAN_POINT('Ctrl Pts',(0.915413034335331,-25.4954156541787,
0.));
#225685=CARTESIAN_POINT('Ctrl Pts',(0.903540269651152,-25.5198888424195,
0.));
#225686=CARTESIAN_POINT('Ctrl Pts',(0.891580105349464,-25.5444000508223,
0.));
#225687=CARTESIAN_POINT('Ctrl Pts',(0.879532523835088,-25.568948840818,
0.));
#225688=CARTESIAN_POINT('Ctrl Pts',(0.867397509339468,-25.5935347843616,
0.));
#225689=CARTESIAN_POINT('Ctrl Pts',(0.855175047037614,-25.618157453608,
0.));
#225690=CARTESIAN_POINT('Ctrl Pts',(0.842865122121542,-25.6428164100078,
0.));
#225691=CARTESIAN_POINT('Ctrl Pts',(0.830467718864366,-25.6675111931957,
0.));
#225692=CARTESIAN_POINT('Ctrl Pts',(0.817982819786718,-25.6922413110172,
0.));
#225693=CARTESIAN_POINT('Ctrl Pts',(0.805410404552592,-25.7170062262474,
0.));
#225694=CARTESIAN_POINT('Ctrl Pts',(0.792750451613533,-25.7418053757671,
0.));
#225695=CARTESIAN_POINT('Ctrl Pts',(0.780002940289024,-25.7666381946871,
0.));
#225696=CARTESIAN_POINT('Ctrl Pts',(0.767167852648638,-25.7915041383304,
0.));
#225697=CARTESIAN_POINT('Ctrl Pts',(0.754245175608287,-25.816402705995,
0.));
#225698=CARTESIAN_POINT('Ctrl Pts',(0.741234902664695,-25.841333461908,
0.));
#225699=CARTESIAN_POINT('Ctrl Pts',(0.728137036485876,-25.8662960624285,
0.));
#225700=CARTESIAN_POINT('Ctrl Pts',(0.714951588533752,-25.8912902615141,
0.));
#225701=CARTESIAN_POINT('Ctrl Pts',(0.701678575236601,-25.9163158909645,
0.));
#225702=CARTESIAN_POINT('Ctrl Pts',(0.688318015065675,-25.941372847213,
0.));
#225703=CARTESIAN_POINT('Ctrl Pts',(0.677559543215902,-25.9614434298092,
0.));
#225704=CARTESIAN_POINT('Ctrl Pts',(0.669451306784414,-25.9765104298171,
0.));
#225705=CARTESIAN_POINT('Ctrl Pts',(0.664028313188911,-25.9865613464809,
0.));
#225706=CARTESIAN_POINT('Ctrl Pts',(0.66131244073089,-25.991588367311,0.));
#225707=CARTESIAN_POINT('',(0.66131244073089,-25.991588367311,12.));
#225708=CARTESIAN_POINT('Ctrl Pts',(0.66131244073089,-25.991588367311,12.));
#225709=CARTESIAN_POINT('Ctrl Pts',(0.664028313188911,-25.9865613464809,
12.));
#225710=CARTESIAN_POINT('Ctrl Pts',(0.669451306784414,-25.9765104298171,
12.));
#225711=CARTESIAN_POINT('Ctrl Pts',(0.677559543215902,-25.9614434298092,
12.));
#225712=CARTESIAN_POINT('Ctrl Pts',(0.688318015065675,-25.941372847213,
12.));
#225713=CARTESIAN_POINT('Ctrl Pts',(0.701678575236601,-25.9163158909645,
12.));
#225714=CARTESIAN_POINT('Ctrl Pts',(0.714951588533752,-25.8912902615141,
12.));
#225715=CARTESIAN_POINT('Ctrl Pts',(0.728137036485876,-25.8662960624285,
12.));
#225716=CARTESIAN_POINT('Ctrl Pts',(0.741234902664695,-25.841333461908,
12.));
#225717=CARTESIAN_POINT('Ctrl Pts',(0.754245175608287,-25.816402705995,
12.));
#225718=CARTESIAN_POINT('Ctrl Pts',(0.767167852648638,-25.7915041383304,
12.));
#225719=CARTESIAN_POINT('Ctrl Pts',(0.780002940289024,-25.7666381946871,
12.));
#225720=CARTESIAN_POINT('Ctrl Pts',(0.792750451613533,-25.7418053757671,
12.));
#225721=CARTESIAN_POINT('Ctrl Pts',(0.805410404552592,-25.7170062262474,
12.));
#225722=CARTESIAN_POINT('Ctrl Pts',(0.817982819786718,-25.6922413110172,
12.));
#225723=CARTESIAN_POINT('Ctrl Pts',(0.830467718864366,-25.6675111931957,
12.));
#225724=CARTESIAN_POINT('Ctrl Pts',(0.842865122121542,-25.6428164100078,
12.));
#225725=CARTESIAN_POINT('Ctrl Pts',(0.855175047037614,-25.618157453608,
12.));
#225726=CARTESIAN_POINT('Ctrl Pts',(0.867397509339468,-25.5935347843616,
12.));
#225727=CARTESIAN_POINT('Ctrl Pts',(0.879532523835088,-25.568948840818,
12.));
#225728=CARTESIAN_POINT('Ctrl Pts',(0.891580105349464,-25.5444000508223,
12.));
#225729=CARTESIAN_POINT('Ctrl Pts',(0.903540269651152,-25.5198888424195,
12.));
#225730=CARTESIAN_POINT('Ctrl Pts',(0.915413034335331,-25.4954156541787,
12.));
#225731=CARTESIAN_POINT('Ctrl Pts',(0.927198419885603,-25.4709809474996,
12.));
#225732=CARTESIAN_POINT('Ctrl Pts',(0.938896449495631,-25.4465852044835,
12.));
#225733=CARTESIAN_POINT('Ctrl Pts',(0.950507148596967,-25.4222289223155,
12.));
#225734=CARTESIAN_POINT('Ctrl Pts',(0.962030544502801,-25.3979126089155,
12.));
#225735=CARTESIAN_POINT('Ctrl Pts',(0.973466666000047,-25.3736367778842,
12.));
#225736=CARTESIAN_POINT('Ctrl Pts',(0.984815543004088,-25.3494019441444,
12.));
#225737=CARTESIAN_POINT('Ctrl Pts',(0.996077206120918,-25.3252086182976,
12.));
#225738=CARTESIAN_POINT('Ctrl Pts',(1.00725168656933,-25.3010573055557,
12.));
#225739=CARTESIAN_POINT('Ctrl Pts',(1.01833901642272,-25.2769485087268,
12.));
#225740=CARTESIAN_POINT('Ctrl Pts',(1.0293392287683,-25.2528827300427,12.));
#225741=CARTESIAN_POINT('Ctrl Pts',(1.04025235791514,-25.2288604735087,
12.));
#225742=CARTESIAN_POINT('Ctrl Pts',(1.05107843957925,-25.2048822469027,
12.));
#225743=CARTESIAN_POINT('Ctrl Pts',(1.06181751111754,-25.1809485642191,
12.));
#225744=CARTESIAN_POINT('Ctrl Pts',(1.07246961165459,-25.1570599469311,
12.));
#225745=CARTESIAN_POINT('Ctrl Pts',(1.08303478197174,-25.1332169227415,
12.));
#225746=CARTESIAN_POINT('Ctrl Pts',(1.09351306445299,-25.1094200248448,
12.));
#225747=CARTESIAN_POINT('Ctrl Pts',(1.1039045030174,-25.085669790968,12.));
#225748=CARTESIAN_POINT('Ctrl Pts',(1.1142091430689,-25.0619667625336,12.));
#225749=CARTESIAN_POINT('Ctrl Pts',(1.12442703144455,-25.0383114836898,
12.));
#225750=CARTESIAN_POINT('Ctrl Pts',(1.13455821638535,-25.0147045006193,
12.));
#225751=CARTESIAN_POINT('Ctrl Pts',(1.14460274758206,-24.9911463621431,
12.));
#225752=CARTESIAN_POINT('Ctrl Pts',(1.15456067621894,-24.9676376201501,
12.));
#225753=CARTESIAN_POINT('Ctrl Pts',(1.16443205502852,-24.9441788300932,
12.));
#225754=CARTESIAN_POINT('Ctrl Pts',(1.17421693835039,-24.9207705514449,
12.));
#225755=CARTESIAN_POINT('Ctrl Pts',(1.18391538220098,-24.8974133481829,
12.));
#225756=CARTESIAN_POINT('Ctrl Pts',(1.19352744434059,-24.8741077892074,
12.));
#225757=CARTESIAN_POINT('Ctrl Pts',(1.20305318426015,-24.8508544481973,
12.));
#225758=CARTESIAN_POINT('Ctrl Pts',(1.21249266318205,-24.8276539035092,
12.));
#225759=CARTESIAN_POINT('Ctrl Pts',(1.22184594406526,-24.8045067380536,
12.));
#225760=CARTESIAN_POINT('Ctrl Pts',(1.23111309161843,-24.78141353918,12.));
#225761=CARTESIAN_POINT('Ctrl Pts',(1.24029417231987,-24.7583748985439,
12.));
#225762=CARTESIAN_POINT('Ctrl Pts',(1.24938925444323,-24.7353914120012,
12.));
#225763=CARTESIAN_POINT('Ctrl Pts',(1.25839840807414,-24.7124636797895,
12.));
#225764=CARTESIAN_POINT('Ctrl Pts',(1.26732170513497,-24.6895923066837,
12.));
#225765=CARTESIAN_POINT('Ctrl Pts',(1.2761592194164,-24.666777902156,12.));
#225766=CARTESIAN_POINT('Ctrl Pts',(1.28491102661513,-24.6440210805278,
12.));
#225767=CARTESIAN_POINT('Ctrl Pts',(1.29357720438107,-24.6213224611228,
12.));
#225768=CARTESIAN_POINT('Ctrl Pts',(1.30215783236363,-24.5986826684025,
12.));
#225769=CARTESIAN_POINT('Ctrl Pts',(1.31065299222023,-24.576102332018,12.));
#225770=CARTESIAN_POINT('Ctrl Pts',(1.31906276763669,-24.5535820868671,
12.));
#225771=CARTESIAN_POINT('Ctrl Pts',(1.32738724435326,-24.5311225731434,
12.));
#225772=CARTESIAN_POINT('Ctrl Pts',(1.33562651019684,-24.5087244363856,
12.));
#225773=CARTESIAN_POINT('Ctrl Pts',(1.34378065512335,-24.4863883275135,
12.));
#225774=CARTESIAN_POINT('Ctrl Pts',(1.35184977125644,-24.4641149028894,
12.));
#225775=CARTESIAN_POINT('Ctrl Pts',(1.35983395290624,-24.4419048244524,
12.));
#225776=CARTESIAN_POINT('Ctrl Pts',(1.36773329659954,-24.4197587598337,
12.));
#225777=CARTESIAN_POINT('Ctrl Pts',(1.37554790111607,-24.3976773824731,
12.));
#225778=CARTESIAN_POINT('Ctrl Pts',(1.38327786752998,-24.37566137173,12.));
#225779=CARTESIAN_POINT('Ctrl Pts',(1.3909232992639,-24.3537114129877,12.));
#225780=CARTESIAN_POINT('Ctrl Pts',(1.3984843021281,-24.3318281977647,12.));
#225781=CARTESIAN_POINT('Ctrl Pts',(1.4059609843434,-24.3100124238316,12.));
#225782=CARTESIAN_POINT('Ctrl Pts',(1.41335345657684,-24.2882647953214,
12.));
#225783=CARTESIAN_POINT('Ctrl Pts',(1.42066183198252,-24.2665860228357,
12.));
#225784=CARTESIAN_POINT('Ctrl Pts',(1.42788622624851,-24.2449768235485,
12.));
#225785=CARTESIAN_POINT('Ctrl Pts',(1.43502675765502,-24.2234379212978,
12.));
#225786=CARTESIAN_POINT('Ctrl Pts',(1.44208354711074,-24.2019700467214,
12.));
#225787=CARTESIAN_POINT('Ctrl Pts',(1.4490567181872,-24.1805739374033,12.));
#225788=CARTESIAN_POINT('Ctrl Pts',(1.45594639716314,-24.1592503380105,
12.));
#225789=CARTESIAN_POINT('Ctrl Pts',(1.46275271307398,-24.1380000004272,
12.));
#225790=CARTESIAN_POINT('Ctrl Pts',(1.46947579776991,-24.1168236838827,
12.));
#225791=CARTESIAN_POINT('Ctrl Pts',(1.47611578597741,-24.0957221550782,
12.));
#225792=CARTESIAN_POINT('Ctrl Pts',(1.4826728153368,-24.074696188353,12.));
#225793=CARTESIAN_POINT('Ctrl Pts',(1.48914702644883,-24.053746565843,12.));
#225794=CARTESIAN_POINT('Ctrl Pts',(1.49553856292798,-24.0328740776331,
12.));
#225795=CARTESIAN_POINT('Ctrl Pts',(1.50184757146099,-24.0120795219086,
12.));
#225796=CARTESIAN_POINT('Ctrl Pts',(1.50807420187702,-23.991363705093,12.));
#225797=CARTESIAN_POINT('Ctrl Pts',(1.51421860720628,-23.9707274420145,
12.));
#225798=CARTESIAN_POINT('Ctrl Pts',(1.52028094372806,-23.9501715561038,
12.));
#225799=CARTESIAN_POINT('Ctrl Pts',(1.52626137103039,-23.9296968795761,
12.));
#225800=CARTESIAN_POINT('Ctrl Pts',(1.53216005207462,-23.9093042536119,
12.));
#225801=CARTESIAN_POINT('Ctrl Pts',(1.53797715326748,-23.8889945285313,
12.));
#225802=CARTESIAN_POINT('Ctrl Pts',(1.54371284453977,-23.8687685639635,
12.));
#225803=CARTESIAN_POINT('Ctrl Pts',(1.5493672994053,-23.8486272290698,12.));
#225804=CARTESIAN_POINT('Ctrl Pts',(1.55494069502627,-23.8285714027631,
12.));
#225805=CARTESIAN_POINT('Ctrl Pts',(1.56043321228631,-23.8086019739192,
12.));
#225806=CARTESIAN_POINT('Ctrl Pts',(1.56584503586844,-23.788719841588,12.));
#225807=CARTESIAN_POINT('Ctrl Pts',(1.57117635434412,-23.7689259151869,
12.));
#225808=CARTESIAN_POINT('Ctrl Pts',(1.57642736025251,-23.7492211147369,
12.));
#225809=CARTESIAN_POINT('Ctrl Pts',(1.58159825017362,-23.7296063711308,
12.));
#225810=CARTESIAN_POINT('Ctrl Pts',(1.58668922481222,-23.7100826263835,
12.));
#225811=CARTESIAN_POINT('Ctrl Pts',(1.59170048908631,-23.6906508338833,
12.));
#225812=CARTESIAN_POINT('Ctrl Pts',(1.59663225222458,-23.6713119586302,
12.));
#225813=CARTESIAN_POINT('Ctrl Pts',(1.60148472786588,-23.6520669774863,
12.));
#225814=CARTESIAN_POINT('Ctrl Pts',(1.60625813414666,-23.6329168794916,
12.));
#225815=CARTESIAN_POINT('Ctrl Pts',(1.61095269379773,-23.6138626661644,
12.));
#225816=CARTESIAN_POINT('Ctrl Pts',(1.61556863424697,-23.5949053517996,
12.));
#225817=CARTESIAN_POINT('Ctrl Pts',(1.62010618772869,-23.5760459637608,
12.));
#225818=CARTESIAN_POINT('Ctrl Pts',(1.62456559140071,-23.5572855427617,
12.));
#225819=CARTESIAN_POINT('Ctrl Pts',(1.62894708745231,-23.5386251432278,
12.));
#225820=CARTESIAN_POINT('Ctrl Pts',(1.63325092321731,-23.5200658336624,
12.));
#225821=CARTESIAN_POINT('Ctrl Pts',(1.63747735129474,-23.5016086970006,
12.));
#225822=CARTESIAN_POINT('Ctrl Pts',(1.64162662967524,-23.4832548309638,
12.));
#225823=CARTESIAN_POINT('Ctrl Pts',(1.64569902187608,-23.4650053483919,
12.));
#225824=CARTESIAN_POINT('Ctrl Pts',(1.64969479707339,-23.446861377656,12.));
#225825=CARTESIAN_POINT('Ctrl Pts',(1.6536142302373,-23.4288240631034,12.));
#225826=CARTESIAN_POINT('Ctrl Pts',(1.65745760227507,-23.4108945654803,
12.));
#225827=CARTESIAN_POINT('Ctrl Pts',(1.66122520018008,-23.3930740623622,
12.));
#225828=CARTESIAN_POINT('Ctrl Pts',(1.66491731718864,-23.375363748555,12.));
#225829=CARTESIAN_POINT('Ctrl Pts',(1.66853425293977,-23.3577648365747,
12.));
#225830=CARTESIAN_POINT('Ctrl Pts',(1.67207631363905,-23.3402785571866,
12.));
#225831=CARTESIAN_POINT('Ctrl Pts',(1.67554381222987,-23.3229061599145,
12.));
#225832=CARTESIAN_POINT('Ctrl Pts',(1.67893706857123,-23.3056489135611,
12.));
#225833=CARTESIAN_POINT('Ctrl Pts',(1.68225640962181,-23.2885081066949,
12.));
#225834=CARTESIAN_POINT('Ctrl Pts',(1.68550216963274,-23.2714850482245,
12.));
#225835=CARTESIAN_POINT('Ctrl Pts',(1.6886746903491,-23.2545810680536,12.));
#225836=CARTESIAN_POINT('Ctrl Pts',(1.69177432121716,-23.2377975177014,
12.));
#225837=CARTESIAN_POINT('Ctrl Pts',(1.69480141959945,-23.2211357709374,
12.));
#225838=CARTESIAN_POINT('Ctrl Pts',(1.69775635099425,-23.2045972243765,
12.));
#225839=CARTESIAN_POINT('Ctrl Pts',(1.70063948926987,-23.1881832981848,
12.));
#225840=CARTESIAN_POINT('Ctrl Pts',(1.70345121691259,-23.1718954368749,
12.));
#225841=CARTESIAN_POINT('Ctrl Pts',(1.70619192527846,-23.1557351100613,
12.));
#225842=CARTESIAN_POINT('Ctrl Pts',(1.70886201485459,-23.1397038132358,
12.));
#225843=CARTESIAN_POINT('Ctrl Pts',(1.71146189552192,-23.1238030684929,
12.));
#225844=CARTESIAN_POINT('Ctrl Pts',(1.71399198684724,-23.1080344254291,
12.));
#225845=CARTESIAN_POINT('Ctrl Pts',(1.71645271839311,-23.0923994621216,
12.));
#225846=CARTESIAN_POINT('Ctrl Pts',(1.71884453003027,-23.0768997860709,
12.));
#225847=CARTESIAN_POINT('Ctrl Pts',(1.7211678722598,-23.061537035156,12.));
#225848=CARTESIAN_POINT('Ctrl Pts',(1.72342320653731,-23.0463128785528,
12.));
#225849=CARTESIAN_POINT('Ctrl Pts',(1.72561100564033,-23.031229017888,12.));
#225850=CARTESIAN_POINT('Ctrl Pts',(1.72773175404702,-23.0162871884167,
12.));
#225851=CARTESIAN_POINT('Ctrl Pts',(1.72978594832137,-23.0014891601891,
12.));
#225852=CARTESIAN_POINT('Ctrl Pts',(1.73177409750193,-22.9868367391978,
12.));
#225853=CARTESIAN_POINT('Ctrl Pts',(1.73369672350817,-22.9723317685688,
12.));
#225854=CARTESIAN_POINT('Ctrl Pts',(1.73555436162771,-22.9579761301062,
12.));
#225855=CARTESIAN_POINT('Ctrl Pts',(1.73734756100038,-22.9437717457825,
12.));
#225856=CARTESIAN_POINT('Ctrl Pts',(1.73907688511664,-22.9297205792587,
12.));
#225857=CARTESIAN_POINT('Ctrl Pts',(1.74074291231056,-22.9158246373365,
12.));
#225858=CARTESIAN_POINT('Ctrl Pts',(1.74234623630079,-22.9020859716144,
12.));
#225859=CARTESIAN_POINT('Ctrl Pts',(1.74388746677702,-22.8885066803351,
12.));
#225860=CARTESIAN_POINT('Ctrl Pts',(1.74536722998199,-22.8750889101696,
12.));
#225861=CARTESIAN_POINT('Ctrl Pts',(1.74678616930663,-22.8618348580234,
12.));
#225862=CARTESIAN_POINT('Ctrl Pts',(1.74814494588491,-22.8487467728075,
12.));
#225863=CARTESIAN_POINT('Ctrl Pts',(1.74944423940117,-22.8358269579854,
12.));
#225864=CARTESIAN_POINT('Ctrl Pts',(1.75068474890883,-22.8230777741285,
12.));
#225865=CARTESIAN_POINT('Ctrl Pts',(1.75186719365589,-22.8105016414712,
12.));
#225866=CARTESIAN_POINT('Ctrl Pts',(1.75299231391461,-22.7981010424312,
12.));
#225867=CARTESIAN_POINT('Ctrl Pts',(1.75406087182929,-22.7858785242358,
12.));
#225868=CARTESIAN_POINT('Ctrl Pts',(1.75507365227127,-22.7738367016115,
12.));
#225869=CARTESIAN_POINT('Ctrl Pts',(1.7560314637164,-22.7619782595013,12.));
#225870=CARTESIAN_POINT('Ctrl Pts',(1.75693513908911,-22.7503059556455,
12.));
#225871=CARTESIAN_POINT('Ctrl Pts',(1.75778553673249,-22.7388226235565,
12.));
#225872=CARTESIAN_POINT('Ctrl Pts',(1.75858354204634,-22.7275311777305,
12.));
#225873=CARTESIAN_POINT('Ctrl Pts',(1.75933006905924,-22.7164346186007,
12.));
#225874=CARTESIAN_POINT('Ctrl Pts',(1.76002606202398,-22.7055360375481,
12.));
#225875=CARTESIAN_POINT('Ctrl Pts',(1.76067249704884,-22.6948386219843,
12.));
#225876=CARTESIAN_POINT('Ctrl Pts',(1.76127038310612,-22.6843456585245,
12.));
#225877=CARTESIAN_POINT('Ctrl Pts',(1.76182076289525,-22.6740605356699,
12.));
#225878=CARTESIAN_POINT('Ctrl Pts',(1.76232471392567,-22.6639867471756,
12.));
#225879=CARTESIAN_POINT('Ctrl Pts',(1.76278334912559,-22.6541278938413,
12.));
#225880=CARTESIAN_POINT('Ctrl Pts',(1.76319782013913,-22.6444876940425,
12.));
#225881=CARTESIAN_POINT('Ctrl Pts',(1.76356932176272,-22.635069997936,12.));
#225882=CARTESIAN_POINT('Ctrl Pts',(1.76389909571402,-22.6258787994847,
12.));
#225883=CARTESIAN_POINT('Ctrl Pts',(1.76418843543739,-22.6169182517693,
12.));
#225884=CARTESIAN_POINT('Ctrl Pts',(1.76443868648015,-22.6081926681342,
12.));
#225885=CARTESIAN_POINT('Ctrl Pts',(1.76465124413556,-22.5997065145638,
12.));
#225886=CARTESIAN_POINT('Ctrl Pts',(1.76482755288411,-22.5914644078106,
12.));
#225887=CARTESIAN_POINT('Ctrl Pts',(1.76496910283088,-22.5834711038024,
12.));
#225888=CARTESIAN_POINT('Ctrl Pts',(1.76507744026747,-22.5757315316355,
12.));
#225889=CARTESIAN_POINT('Ctrl Pts',(1.76515418518829,-22.5682508499873,
12.));
#225890=CARTESIAN_POINT('Ctrl Pts',(1.76520104500449,-22.5610344912501,
12.));
#225891=CARTESIAN_POINT('Ctrl Pts',(1.76521983384062,-22.5540882235837,
12.));
#225892=CARTESIAN_POINT('Ctrl Pts',(1.76521245524047,-22.5474180954006,
12.));
#225893=CARTESIAN_POINT('Ctrl Pts',(1.76518087841492,-22.5410303590891,
12.));
#225894=CARTESIAN_POINT('Ctrl Pts',(1.7651271156325,-22.5349313983571,12.));
#225895=CARTESIAN_POINT('Ctrl Pts',(1.76505320262751,-22.529127665298,12.));
#225896=CARTESIAN_POINT('Ctrl Pts',(1.76496128643369,-22.5236259635515,
12.));
#225897=CARTESIAN_POINT('Ctrl Pts',(1.76485369319896,-22.5184336670207,
12.));
#225898=CARTESIAN_POINT('Ctrl Pts',(1.76473303281158,-22.5135590569554,
12.));
#225899=CARTESIAN_POINT('Ctrl Pts',(1.76460218257323,-22.5090112700212,
12.));
#225900=CARTESIAN_POINT('Ctrl Pts',(1.76446408210366,-22.5047996391978,
12.));
#225901=CARTESIAN_POINT('Ctrl Pts',(1.76432160068725,-22.5009332677316,
12.));
#225902=CARTESIAN_POINT('Ctrl Pts',(1.76417731243462,-22.4974203063191,
12.));
#225903=CARTESIAN_POINT('Ctrl Pts',(1.764033938803,-22.4942693792449,12.));
#225904=CARTESIAN_POINT('Ctrl Pts',(1.76389475965723,-22.4914909094908,
12.));
#225905=CARTESIAN_POINT('Ctrl Pts',(1.76376424879504,-22.4890991659478,
12.));
#225906=CARTESIAN_POINT('Ctrl Pts',(1.76364784232963,-22.4871115206571,
12.));
#225907=CARTESIAN_POINT('Ctrl Pts',(1.76355076045546,-22.4855446605991,
12.));
#225908=CARTESIAN_POINT('Ctrl Pts',(1.76347698284791,-22.4844112933129,
12.));
#225909=CARTESIAN_POINT('Ctrl Pts',(1.76343813434565,-22.483856251707,12.));
#225910=CARTESIAN_POINT('Ctrl Pts',(1.7634206426357,-22.4836387052232,12.));
#225911=CARTESIAN_POINT('Ctrl Pts',(1.76341415538764,-22.483581992979,12.));
#225912=CARTESIAN_POINT('Ctrl Pts',(1.76341220531179,-22.4835757167854,
12.));
#225913=CARTESIAN_POINT('',(0.66131244073089,-25.991588367311,0.));
#225914=CARTESIAN_POINT('Origin',(-3.92374859571502,-21.1389261070099,0.));
#225915=CARTESIAN_POINT('',(-4.11585220600463,-22.1738711152697,12.));
#225916=CARTESIAN_POINT('',(-1.96187429785751,-10.5694630535049,12.));
#225917=CARTESIAN_POINT('',(-4.11585220600463,-22.1738711152697,0.));
#225918=CARTESIAN_POINT('',(-4.11585220600463,-22.1738711152697,0.));
#225919=CARTESIAN_POINT('',(-1.96187429785751,-10.5694630535049,0.));
#225920=CARTESIAN_POINT('Ctrl Pts',(-0.661312440730913,-25.991588367311,
0.));
#225921=CARTESIAN_POINT('Ctrl Pts',(-0.661312440730913,-25.991588367311,
12.));
#225922=CARTESIAN_POINT('Ctrl Pts',(-0.664028313187638,-25.9865613464773,
0.));
#225923=CARTESIAN_POINT('Ctrl Pts',(-0.664028313187638,-25.9865613464773,
12.));
#225924=CARTESIAN_POINT('Ctrl Pts',(-0.669451306780837,-25.9765104298071,
0.));
#225925=CARTESIAN_POINT('Ctrl Pts',(-0.669451306780837,-25.9765104298071,
12.));
#225926=CARTESIAN_POINT('Ctrl Pts',(-0.677559543209739,-25.9614434297919,
0.));
#225927=CARTESIAN_POINT('Ctrl Pts',(-0.677559543209739,-25.9614434297919,
12.));
#225928=CARTESIAN_POINT('Ctrl Pts',(-0.688318015057743,-25.9413728471909,
0.));
#225929=CARTESIAN_POINT('Ctrl Pts',(-0.688318015057743,-25.9413728471909,
12.));
#225930=CARTESIAN_POINT('Ctrl Pts',(-0.701678575228768,-25.9163158909426,
0.));
#225931=CARTESIAN_POINT('Ctrl Pts',(-0.701678575228768,-25.9163158909426,
12.));
#225932=CARTESIAN_POINT('Ctrl Pts',(-0.714951588527651,-25.891290261497,
0.));
#225933=CARTESIAN_POINT('Ctrl Pts',(-0.714951588527651,-25.891290261497,
12.));
#225934=CARTESIAN_POINT('Ctrl Pts',(-0.728137036482348,-25.8662960624185,
0.));
#225935=CARTESIAN_POINT('Ctrl Pts',(-0.728137036482348,-25.8662960624185,
12.));
#225936=CARTESIAN_POINT('Ctrl Pts',(-0.741234902663818,-25.8413334619055,
0.));
#225937=CARTESIAN_POINT('Ctrl Pts',(-0.741234902663818,-25.8413334619055,
12.));
#225938=CARTESIAN_POINT('Ctrl Pts',(-0.754245175609535,-25.8164027059984,
0.));
#225939=CARTESIAN_POINT('Ctrl Pts',(-0.754245175609535,-25.8164027059984,
12.));
#225940=CARTESIAN_POINT('Ctrl Pts',(-0.76716785265118,-25.7915041383376,
0.));
#225941=CARTESIAN_POINT('Ctrl Pts',(-0.76716785265118,-25.7915041383376,
12.));
#225942=CARTESIAN_POINT('Ctrl Pts',(-0.780002940291976,-25.7666381946955,
0.));
#225943=CARTESIAN_POINT('Ctrl Pts',(-0.780002940291976,-25.7666381946955,
12.));
#225944=CARTESIAN_POINT('Ctrl Pts',(-0.792750451616139,-25.7418053757746,
0.));
#225945=CARTESIAN_POINT('Ctrl Pts',(-0.792750451616139,-25.7418053757746,
12.));
#225946=CARTESIAN_POINT('Ctrl Pts',(-0.805410404554365,-25.7170062262525,
0.));
#225947=CARTESIAN_POINT('Ctrl Pts',(-0.805410404554365,-25.7170062262525,
12.));
#225948=CARTESIAN_POINT('Ctrl Pts',(-0.817982819787476,-25.6922413110194,
0.));
#225949=CARTESIAN_POINT('Ctrl Pts',(-0.817982819787476,-25.6922413110194,
12.));
#225950=CARTESIAN_POINT('Ctrl Pts',(-0.830467718864218,-25.6675111931952,
0.));
#225951=CARTESIAN_POINT('Ctrl Pts',(-0.830467718864218,-25.6675111931952,
12.));
#225952=CARTESIAN_POINT('Ctrl Pts',(-0.842865122120771,-25.6428164100055,
0.));
#225953=CARTESIAN_POINT('Ctrl Pts',(-0.842865122120771,-25.6428164100055,
12.));
#225954=CARTESIAN_POINT('Ctrl Pts',(-0.85517504703656,-25.6181574536049,
0.));
#225955=CARTESIAN_POINT('Ctrl Pts',(-0.85517504703656,-25.6181574536049,
12.));
#225956=CARTESIAN_POINT('Ctrl Pts',(-0.867397509338443,-25.5935347843585,
0.));
#225957=CARTESIAN_POINT('Ctrl Pts',(-0.867397509338443,-25.5935347843585,
12.));
#225958=CARTESIAN_POINT('Ctrl Pts',(-0.879532523834307,-25.5689488408156,
0.));
#225959=CARTESIAN_POINT('Ctrl Pts',(-0.879532523834307,-25.5689488408156,
12.));
#225960=CARTESIAN_POINT('Ctrl Pts',(-0.891580105349052,-25.5444000508211,
0.));
#225961=CARTESIAN_POINT('Ctrl Pts',(-0.891580105349052,-25.5444000508211,
12.));
#225962=CARTESIAN_POINT('Ctrl Pts',(-0.903540269651119,-25.5198888424194,
0.));
#225963=CARTESIAN_POINT('Ctrl Pts',(-0.903540269651119,-25.5198888424194,
12.));
#225964=CARTESIAN_POINT('Ctrl Pts',(-0.915413034335626,-25.4954156541795,
0.));
#225965=CARTESIAN_POINT('Ctrl Pts',(-0.915413034335626,-25.4954156541795,
12.));
#225966=CARTESIAN_POINT('Ctrl Pts',(-0.927198419886107,-25.4709809475009,
0.));
#225967=CARTESIAN_POINT('Ctrl Pts',(-0.927198419886107,-25.4709809475009,
12.));
#225968=CARTESIAN_POINT('Ctrl Pts',(-0.938896449496205,-25.4465852044849,
0.));
#225969=CARTESIAN_POINT('Ctrl Pts',(-0.938896449496205,-25.4465852044849,
12.));
#225970=CARTESIAN_POINT('Ctrl Pts',(-0.950507148597481,-25.4222289223167,
0.));
#225971=CARTESIAN_POINT('Ctrl Pts',(-0.950507148597481,-25.4222289223167,
12.));
#225972=CARTESIAN_POINT('Ctrl Pts',(-0.962030544503155,-25.3979126089163,
0.));
#225973=CARTESIAN_POINT('Ctrl Pts',(-0.962030544503155,-25.3979126089163,
12.));
#225974=CARTESIAN_POINT('Ctrl Pts',(-0.973466666000176,-25.3736367778845,
0.));
#225975=CARTESIAN_POINT('Ctrl Pts',(-0.973466666000176,-25.3736367778845,
12.));
#225976=CARTESIAN_POINT('Ctrl Pts',(-0.984815543003984,-25.3494019441441,
0.));
#225977=CARTESIAN_POINT('Ctrl Pts',(-0.984815543003984,-25.3494019441441,
12.));
#225978=CARTESIAN_POINT('Ctrl Pts',(-0.996077206120636,-25.3252086182968,
0.));
#225979=CARTESIAN_POINT('Ctrl Pts',(-0.996077206120636,-25.3252086182968,
12.));
#225980=CARTESIAN_POINT('Ctrl Pts',(-1.00725168656897,-25.3010573055548,
0.));
#225981=CARTESIAN_POINT('Ctrl Pts',(-1.00725168656897,-25.3010573055548,
12.));
#225982=CARTESIAN_POINT('Ctrl Pts',(-1.01833901642238,-25.276948508726,
0.));
#225983=CARTESIAN_POINT('Ctrl Pts',(-1.01833901642238,-25.276948508726,
12.));
#225984=CARTESIAN_POINT('Ctrl Pts',(-1.02933922876807,-25.2528827300422,
0.));
#225985=CARTESIAN_POINT('Ctrl Pts',(-1.02933922876807,-25.2528827300422,
12.));
#225986=CARTESIAN_POINT('Ctrl Pts',(-1.04025235791508,-25.2288604735086,
0.));
#225987=CARTESIAN_POINT('Ctrl Pts',(-1.04025235791508,-25.2288604735086,
12.));
#225988=CARTESIAN_POINT('Ctrl Pts',(-1.05107843957933,-25.2048822469028,
0.));
#225989=CARTESIAN_POINT('Ctrl Pts',(-1.05107843957933,-25.2048822469028,
12.));
#225990=CARTESIAN_POINT('Ctrl Pts',(-1.06181751111769,-25.1809485642192,
0.));
#225991=CARTESIAN_POINT('Ctrl Pts',(-1.06181751111769,-25.1809485642192,
12.));
#225992=CARTESIAN_POINT('Ctrl Pts',(-1.07246961165477,-25.157059946931,
0.));
#225993=CARTESIAN_POINT('Ctrl Pts',(-1.07246961165477,-25.157059946931,
12.));
#225994=CARTESIAN_POINT('Ctrl Pts',(-1.08303478197189,-25.1332169227413,
0.));
#225995=CARTESIAN_POINT('Ctrl Pts',(-1.08303478197189,-25.1332169227413,
12.));
#225996=CARTESIAN_POINT('Ctrl Pts',(-1.09351306445309,-25.1094200248446,
0.));
#225997=CARTESIAN_POINT('Ctrl Pts',(-1.09351306445309,-25.1094200248446,
12.));
#225998=CARTESIAN_POINT('Ctrl Pts',(-1.10390450301746,-25.0856697909679,
0.));
#225999=CARTESIAN_POINT('Ctrl Pts',(-1.10390450301746,-25.0856697909679,
12.));
#226000=CARTESIAN_POINT('Ctrl Pts',(-1.1142091430689,-25.0619667625336,
0.));
#226001=CARTESIAN_POINT('Ctrl Pts',(-1.1142091430689,-25.0619667625336,
12.));
#226002=CARTESIAN_POINT('Ctrl Pts',(-1.12442703144453,-25.0383114836899,
0.));
#226003=CARTESIAN_POINT('Ctrl Pts',(-1.12442703144453,-25.0383114836899,
12.));
#226004=CARTESIAN_POINT('Ctrl Pts',(-1.13455821638531,-25.0147045006196,
0.));
#226005=CARTESIAN_POINT('Ctrl Pts',(-1.13455821638531,-25.0147045006196,
12.));
#226006=CARTESIAN_POINT('Ctrl Pts',(-1.14460274758202,-24.9911463621433,
0.));
#226007=CARTESIAN_POINT('Ctrl Pts',(-1.14460274758202,-24.9911463621433,
12.));
#226008=CARTESIAN_POINT('Ctrl Pts',(-1.1545606762189,-24.9676376201502,
0.));
#226009=CARTESIAN_POINT('Ctrl Pts',(-1.1545606762189,-24.9676376201502,
12.));
#226010=CARTESIAN_POINT('Ctrl Pts',(-1.16443205502851,-24.9441788300932,
0.));
#226011=CARTESIAN_POINT('Ctrl Pts',(-1.16443205502851,-24.9441788300932,
12.));
#226012=CARTESIAN_POINT('Ctrl Pts',(-1.17421693835042,-24.9207705514448,
0.));
#226013=CARTESIAN_POINT('Ctrl Pts',(-1.17421693835042,-24.9207705514448,
12.));
#226014=CARTESIAN_POINT('Ctrl Pts',(-1.18391538220104,-24.8974133481829,
0.));
#226015=CARTESIAN_POINT('Ctrl Pts',(-1.18391538220104,-24.8974133481829,
12.));
#226016=CARTESIAN_POINT('Ctrl Pts',(-1.19352744434065,-24.8741077892075,
0.));
#226017=CARTESIAN_POINT('Ctrl Pts',(-1.19352744434065,-24.8741077892075,
12.));
#226018=CARTESIAN_POINT('Ctrl Pts',(-1.20305318426021,-24.8508544481974,
0.));
#226019=CARTESIAN_POINT('Ctrl Pts',(-1.20305318426021,-24.8508544481974,
12.));
#226020=CARTESIAN_POINT('Ctrl Pts',(-1.21249266318209,-24.8276539035092,
0.));
#226021=CARTESIAN_POINT('Ctrl Pts',(-1.21249266318209,-24.8276539035092,
12.));
#226022=CARTESIAN_POINT('Ctrl Pts',(-1.22184594406529,-24.8045067380536,
0.));
#226023=CARTESIAN_POINT('Ctrl Pts',(-1.22184594406529,-24.8045067380536,
12.));
#226024=CARTESIAN_POINT('Ctrl Pts',(-1.23111309161845,-24.7814135391799,
0.));
#226025=CARTESIAN_POINT('Ctrl Pts',(-1.23111309161845,-24.7814135391799,
12.));
#226026=CARTESIAN_POINT('Ctrl Pts',(-1.2402941723199,-24.7583748985438,
0.));
#226027=CARTESIAN_POINT('Ctrl Pts',(-1.2402941723199,-24.7583748985438,
12.));
#226028=CARTESIAN_POINT('Ctrl Pts',(-1.24938925444327,-24.7353914120011,
0.));
#226029=CARTESIAN_POINT('Ctrl Pts',(-1.24938925444327,-24.7353914120011,
12.));
#226030=CARTESIAN_POINT('Ctrl Pts',(-1.25839840807419,-24.7124636797894,
0.));
#226031=CARTESIAN_POINT('Ctrl Pts',(-1.25839840807419,-24.7124636797894,
12.));
#226032=CARTESIAN_POINT('Ctrl Pts',(-1.26732170513501,-24.6895923066836,
0.));
#226033=CARTESIAN_POINT('Ctrl Pts',(-1.26732170513501,-24.6895923066836,
12.));
#226034=CARTESIAN_POINT('Ctrl Pts',(-1.27615921941643,-24.6667779021559,
0.));
#226035=CARTESIAN_POINT('Ctrl Pts',(-1.27615921941643,-24.6667779021559,
12.));
#226036=CARTESIAN_POINT('Ctrl Pts',(-1.28491102661515,-24.6440210805278,
0.));
#226037=CARTESIAN_POINT('Ctrl Pts',(-1.28491102661515,-24.6440210805278,
12.));
#226038=CARTESIAN_POINT('Ctrl Pts',(-1.29357720438108,-24.6213224611229,
0.));
#226039=CARTESIAN_POINT('Ctrl Pts',(-1.29357720438108,-24.6213224611229,
12.));
#226040=CARTESIAN_POINT('Ctrl Pts',(-1.30215783236363,-24.5986826684027,
0.));
#226041=CARTESIAN_POINT('Ctrl Pts',(-1.30215783236363,-24.5986826684027,
12.));
#226042=CARTESIAN_POINT('Ctrl Pts',(-1.31065299222023,-24.5761023320183,
0.));
#226043=CARTESIAN_POINT('Ctrl Pts',(-1.31065299222023,-24.5761023320183,
12.));
#226044=CARTESIAN_POINT('Ctrl Pts',(-1.31906276763669,-24.5535820868674,
0.));
#226045=CARTESIAN_POINT('Ctrl Pts',(-1.31906276763669,-24.5535820868674,
12.));
#226046=CARTESIAN_POINT('Ctrl Pts',(-1.32738724435327,-24.5311225731435,
0.));
#226047=CARTESIAN_POINT('Ctrl Pts',(-1.32738724435327,-24.5311225731435,
12.));
#226048=CARTESIAN_POINT('Ctrl Pts',(-1.33562651019687,-24.5087244363856,
0.));
#226049=CARTESIAN_POINT('Ctrl Pts',(-1.33562651019687,-24.5087244363856,
12.));
#226050=CARTESIAN_POINT('Ctrl Pts',(-1.34378065512339,-24.4863883275134,
0.));
#226051=CARTESIAN_POINT('Ctrl Pts',(-1.34378065512339,-24.4863883275134,
12.));
#226052=CARTESIAN_POINT('Ctrl Pts',(-1.35184977125649,-24.4641149028892,
0.));
#226053=CARTESIAN_POINT('Ctrl Pts',(-1.35184977125649,-24.4641149028892,
12.));
#226054=CARTESIAN_POINT('Ctrl Pts',(-1.35983395290628,-24.4419048244523,
0.));
#226055=CARTESIAN_POINT('Ctrl Pts',(-1.35983395290628,-24.4419048244523,
12.));
#226056=CARTESIAN_POINT('Ctrl Pts',(-1.36773329659957,-24.4197587598337,
0.));
#226057=CARTESIAN_POINT('Ctrl Pts',(-1.36773329659957,-24.4197587598337,
12.));
#226058=CARTESIAN_POINT('Ctrl Pts',(-1.3755479011161,-24.3976773824732,
0.));
#226059=CARTESIAN_POINT('Ctrl Pts',(-1.3755479011161,-24.3976773824732,
12.));
#226060=CARTESIAN_POINT('Ctrl Pts',(-1.38327786753,-24.3756613717299,0.));
#226061=CARTESIAN_POINT('Ctrl Pts',(-1.38327786753,-24.3756613717299,12.));
#226062=CARTESIAN_POINT('Ctrl Pts',(-1.39092329926389,-24.3537114129875,
0.));
#226063=CARTESIAN_POINT('Ctrl Pts',(-1.39092329926389,-24.3537114129875,
12.));
#226064=CARTESIAN_POINT('Ctrl Pts',(-1.39848430212808,-24.3318281977643,
0.));
#226065=CARTESIAN_POINT('Ctrl Pts',(-1.39848430212808,-24.3318281977643,
12.));
#226066=CARTESIAN_POINT('Ctrl Pts',(-1.40596098434338,-24.3100124238311,
0.));
#226067=CARTESIAN_POINT('Ctrl Pts',(-1.40596098434338,-24.3100124238311,
12.));
#226068=CARTESIAN_POINT('Ctrl Pts',(-1.41335345657684,-24.288264795321,
0.));
#226069=CARTESIAN_POINT('Ctrl Pts',(-1.41335345657684,-24.288264795321,
12.));
#226070=CARTESIAN_POINT('Ctrl Pts',(-1.42066183198254,-24.2665860228356,
0.));
#226071=CARTESIAN_POINT('Ctrl Pts',(-1.42066183198254,-24.2665860228356,
12.));
#226072=CARTESIAN_POINT('Ctrl Pts',(-1.42788622624855,-24.2449768235488,
0.));
#226073=CARTESIAN_POINT('Ctrl Pts',(-1.42788622624855,-24.2449768235488,
12.));
#226074=CARTESIAN_POINT('Ctrl Pts',(-1.43502675765509,-24.2234379212984,
0.));
#226075=CARTESIAN_POINT('Ctrl Pts',(-1.43502675765509,-24.2234379212984,
12.));
#226076=CARTESIAN_POINT('Ctrl Pts',(-1.44208354711083,-24.201970046722,
0.));
#226077=CARTESIAN_POINT('Ctrl Pts',(-1.44208354711083,-24.201970046722,
12.));
#226078=CARTESIAN_POINT('Ctrl Pts',(-1.44905671818729,-24.1805739374038,
0.));
#226079=CARTESIAN_POINT('Ctrl Pts',(-1.44905671818729,-24.1805739374038,
12.));
#226080=CARTESIAN_POINT('Ctrl Pts',(-1.45594639716319,-24.1592503380107,
0.));
#226081=CARTESIAN_POINT('Ctrl Pts',(-1.45594639716319,-24.1592503380107,
12.));
#226082=CARTESIAN_POINT('Ctrl Pts',(-1.46275271307399,-24.1380000004272,
0.));
#226083=CARTESIAN_POINT('Ctrl Pts',(-1.46275271307399,-24.1380000004272,
12.));
#226084=CARTESIAN_POINT('Ctrl Pts',(-1.46947579776992,-24.1168236838824,
0.));
#226085=CARTESIAN_POINT('Ctrl Pts',(-1.46947579776992,-24.1168236838824,
12.));
#226086=CARTESIAN_POINT('Ctrl Pts',(-1.47611578597743,-24.0957221550778,
0.));
#226087=CARTESIAN_POINT('Ctrl Pts',(-1.47611578597743,-24.0957221550778,
12.));
#226088=CARTESIAN_POINT('Ctrl Pts',(-1.48267281533684,-24.0746961883528,
0.));
#226089=CARTESIAN_POINT('Ctrl Pts',(-1.48267281533684,-24.0746961883528,
12.));
#226090=CARTESIAN_POINT('Ctrl Pts',(-1.48914702644888,-24.0537465658429,
0.));
#226091=CARTESIAN_POINT('Ctrl Pts',(-1.48914702644888,-24.0537465658429,
12.));
#226092=CARTESIAN_POINT('Ctrl Pts',(-1.49553856292802,-24.0328740776331,
0.));
#226093=CARTESIAN_POINT('Ctrl Pts',(-1.49553856292802,-24.0328740776331,
12.));
#226094=CARTESIAN_POINT('Ctrl Pts',(-1.501847571461,-24.0120795219086,0.));
#226095=CARTESIAN_POINT('Ctrl Pts',(-1.501847571461,-24.0120795219086,12.));
#226096=CARTESIAN_POINT('Ctrl Pts',(-1.50807420187695,-23.9913637050927,
0.));
#226097=CARTESIAN_POINT('Ctrl Pts',(-1.50807420187695,-23.9913637050927,
12.));
#226098=CARTESIAN_POINT('Ctrl Pts',(-1.51421860720615,-23.970727442014,
0.));
#226099=CARTESIAN_POINT('Ctrl Pts',(-1.51421860720615,-23.970727442014,
12.));
#226100=CARTESIAN_POINT('Ctrl Pts',(-1.52028094372793,-23.9501715561033,
0.));
#226101=CARTESIAN_POINT('Ctrl Pts',(-1.52028094372793,-23.9501715561033,
12.));
#226102=CARTESIAN_POINT('Ctrl Pts',(-1.52626137103033,-23.9296968795757,
0.));
#226103=CARTESIAN_POINT('Ctrl Pts',(-1.52626137103033,-23.9296968795757,
12.));
#226104=CARTESIAN_POINT('Ctrl Pts',(-1.53216005207464,-23.9093042536119,
0.));
#226105=CARTESIAN_POINT('Ctrl Pts',(-1.53216005207464,-23.9093042536119,
12.));
#226106=CARTESIAN_POINT('Ctrl Pts',(-1.53797715326759,-23.8889945285318,
0.));
#226107=CARTESIAN_POINT('Ctrl Pts',(-1.53797715326759,-23.8889945285318,
12.));
#226108=CARTESIAN_POINT('Ctrl Pts',(-1.54371284453991,-23.8687685639642,
0.));
#226109=CARTESIAN_POINT('Ctrl Pts',(-1.54371284453991,-23.8687685639642,
12.));
#226110=CARTESIAN_POINT('Ctrl Pts',(-1.54936729940542,-23.8486272290705,
0.));
#226111=CARTESIAN_POINT('Ctrl Pts',(-1.54936729940542,-23.8486272290705,
12.));
#226112=CARTESIAN_POINT('Ctrl Pts',(-1.55494069502636,-23.8285714027636,
0.));
#226113=CARTESIAN_POINT('Ctrl Pts',(-1.55494069502636,-23.8285714027636,
12.));
#226114=CARTESIAN_POINT('Ctrl Pts',(-1.56043321228635,-23.8086019739194,
0.));
#226115=CARTESIAN_POINT('Ctrl Pts',(-1.56043321228635,-23.8086019739194,
12.));
#226116=CARTESIAN_POINT('Ctrl Pts',(-1.56584503586844,-23.7887198415878,
0.));
#226117=CARTESIAN_POINT('Ctrl Pts',(-1.56584503586844,-23.7887198415878,
12.));
#226118=CARTESIAN_POINT('Ctrl Pts',(-1.57117635434409,-23.7689259151862,
0.));
#226119=CARTESIAN_POINT('Ctrl Pts',(-1.57117635434409,-23.7689259151862,
12.));
#226120=CARTESIAN_POINT('Ctrl Pts',(-1.57642736025247,-23.749221114736,
0.));
#226121=CARTESIAN_POINT('Ctrl Pts',(-1.57642736025247,-23.749221114736,
12.));
#226122=CARTESIAN_POINT('Ctrl Pts',(-1.58159825017359,-23.72960637113,0.));
#226123=CARTESIAN_POINT('Ctrl Pts',(-1.58159825017359,-23.72960637113,12.));
#226124=CARTESIAN_POINT('Ctrl Pts',(-1.58668922481222,-23.710082626383,
0.));
#226125=CARTESIAN_POINT('Ctrl Pts',(-1.58668922481222,-23.710082626383,
12.));
#226126=CARTESIAN_POINT('Ctrl Pts',(-1.59170048908634,-23.6906508338833,
0.));
#226127=CARTESIAN_POINT('Ctrl Pts',(-1.59170048908634,-23.6906508338833,
12.));
#226128=CARTESIAN_POINT('Ctrl Pts',(-1.59663225222464,-23.671311958631,
0.));
#226129=CARTESIAN_POINT('Ctrl Pts',(-1.59663225222464,-23.671311958631,
12.));
#226130=CARTESIAN_POINT('Ctrl Pts',(-1.60148472786596,-23.6520669774876,
0.));
#226131=CARTESIAN_POINT('Ctrl Pts',(-1.60148472786596,-23.6520669774876,
12.));
#226132=CARTESIAN_POINT('Ctrl Pts',(-1.60625813414674,-23.6329168794929,
0.));
#226133=CARTESIAN_POINT('Ctrl Pts',(-1.60625813414674,-23.6329168794929,
12.));
#226134=CARTESIAN_POINT('Ctrl Pts',(-1.61095269379779,-23.6138626661653,
0.));
#226135=CARTESIAN_POINT('Ctrl Pts',(-1.61095269379779,-23.6138626661653,
12.));
#226136=CARTESIAN_POINT('Ctrl Pts',(-1.61556863424699,-23.5949053517997,
0.));
#226137=CARTESIAN_POINT('Ctrl Pts',(-1.61556863424699,-23.5949053517997,
12.));
#226138=CARTESIAN_POINT('Ctrl Pts',(-1.62010618772867,-23.57604596376,0.));
#226139=CARTESIAN_POINT('Ctrl Pts',(-1.62010618772867,-23.57604596376,12.));
#226140=CARTESIAN_POINT('Ctrl Pts',(-1.62456559140065,-23.5572855427601,
0.));
#226141=CARTESIAN_POINT('Ctrl Pts',(-1.62456559140065,-23.5572855427601,
12.));
#226142=CARTESIAN_POINT('Ctrl Pts',(-1.62894708745224,-23.538625143226,
0.));
#226143=CARTESIAN_POINT('Ctrl Pts',(-1.62894708745224,-23.538625143226,
12.));
#226144=CARTESIAN_POINT('Ctrl Pts',(-1.63325092321727,-23.5200658336612,
0.));
#226145=CARTESIAN_POINT('Ctrl Pts',(-1.63325092321727,-23.5200658336612,
12.));
#226146=CARTESIAN_POINT('Ctrl Pts',(-1.63747735129475,-23.5016086970003,
0.));
#226147=CARTESIAN_POINT('Ctrl Pts',(-1.63747735129475,-23.5016086970003,
12.));
#226148=CARTESIAN_POINT('Ctrl Pts',(-1.64162662967529,-23.4832548309645,
0.));
#226149=CARTESIAN_POINT('Ctrl Pts',(-1.64162662967529,-23.4832548309645,
12.));
#226150=CARTESIAN_POINT('Ctrl Pts',(-1.64569902187612,-23.4650053483932,
0.));
#226151=CARTESIAN_POINT('Ctrl Pts',(-1.64569902187612,-23.4650053483932,
12.));
#226152=CARTESIAN_POINT('Ctrl Pts',(-1.64969479707341,-23.4468613776574,
0.));
#226153=CARTESIAN_POINT('Ctrl Pts',(-1.64969479707341,-23.4468613776574,
12.));
#226154=CARTESIAN_POINT('Ctrl Pts',(-1.65361423023729,-23.4288240631043,
0.));
#226155=CARTESIAN_POINT('Ctrl Pts',(-1.65361423023729,-23.4288240631043,
12.));
#226156=CARTESIAN_POINT('Ctrl Pts',(-1.65745760227506,-23.4108945654805,
0.));
#226157=CARTESIAN_POINT('Ctrl Pts',(-1.65745760227506,-23.4108945654805,
12.));
#226158=CARTESIAN_POINT('Ctrl Pts',(-1.66122520018012,-23.3930740623619,
0.));
#226159=CARTESIAN_POINT('Ctrl Pts',(-1.66122520018012,-23.3930740623619,
12.));
#226160=CARTESIAN_POINT('Ctrl Pts',(-1.66491731718878,-23.3753637485545,
0.));
#226161=CARTESIAN_POINT('Ctrl Pts',(-1.66491731718878,-23.3753637485545,
12.));
#226162=CARTESIAN_POINT('Ctrl Pts',(-1.66853425293997,-23.3577648365744,
0.));
#226163=CARTESIAN_POINT('Ctrl Pts',(-1.66853425293997,-23.3577648365744,
12.));
#226164=CARTESIAN_POINT('Ctrl Pts',(-1.67207631363923,-23.3402785571865,
0.));
#226165=CARTESIAN_POINT('Ctrl Pts',(-1.67207631363923,-23.3402785571865,
12.));
#226166=CARTESIAN_POINT('Ctrl Pts',(-1.67554381222995,-23.3229061599145,
0.));
#226167=CARTESIAN_POINT('Ctrl Pts',(-1.67554381222995,-23.3229061599145,
12.));
#226168=CARTESIAN_POINT('Ctrl Pts',(-1.67893706857118,-23.3056489135611,
0.));
#226169=CARTESIAN_POINT('Ctrl Pts',(-1.67893706857118,-23.3056489135611,
12.));
#226170=CARTESIAN_POINT('Ctrl Pts',(-1.68225640962169,-23.2885081066951,
0.));
#226171=CARTESIAN_POINT('Ctrl Pts',(-1.68225640962169,-23.2885081066951,
12.));
#226172=CARTESIAN_POINT('Ctrl Pts',(-1.68550216963259,-23.2714850482246,
0.));
#226173=CARTESIAN_POINT('Ctrl Pts',(-1.68550216963259,-23.2714850482246,
12.));
#226174=CARTESIAN_POINT('Ctrl Pts',(-1.68867469034897,-23.2545810680537,
0.));
#226175=CARTESIAN_POINT('Ctrl Pts',(-1.68867469034897,-23.2545810680537,
12.));
#226176=CARTESIAN_POINT('Ctrl Pts',(-1.69177432121712,-23.2377975177013,
0.));
#226177=CARTESIAN_POINT('Ctrl Pts',(-1.69177432121712,-23.2377975177013,
12.));
#226178=CARTESIAN_POINT('Ctrl Pts',(-1.69480141959954,-23.2211357709374,
0.));
#226179=CARTESIAN_POINT('Ctrl Pts',(-1.69480141959954,-23.2211357709374,
12.));
#226180=CARTESIAN_POINT('Ctrl Pts',(-1.69775635099444,-23.2045972243767,
0.));
#226181=CARTESIAN_POINT('Ctrl Pts',(-1.69775635099444,-23.2045972243767,
12.));
#226182=CARTESIAN_POINT('Ctrl Pts',(-1.70063948927011,-23.1881832981851,
0.));
#226183=CARTESIAN_POINT('Ctrl Pts',(-1.70063948927011,-23.1881832981851,
12.));
#226184=CARTESIAN_POINT('Ctrl Pts',(-1.70345121691277,-23.1718954368751,
0.));
#226185=CARTESIAN_POINT('Ctrl Pts',(-1.70345121691277,-23.1718954368751,
12.));
#226186=CARTESIAN_POINT('Ctrl Pts',(-1.70619192527853,-23.1557351100614,
0.));
#226187=CARTESIAN_POINT('Ctrl Pts',(-1.70619192527853,-23.1557351100614,
12.));
#226188=CARTESIAN_POINT('Ctrl Pts',(-1.70886201485453,-23.1397038132356,
0.));
#226189=CARTESIAN_POINT('Ctrl Pts',(-1.70886201485453,-23.1397038132356,
12.));
#226190=CARTESIAN_POINT('Ctrl Pts',(-1.71146189552175,-23.1238030684925,
0.));
#226191=CARTESIAN_POINT('Ctrl Pts',(-1.71146189552175,-23.1238030684925,
12.));
#226192=CARTESIAN_POINT('Ctrl Pts',(-1.71399198684705,-23.1080344254286,
0.));
#226193=CARTESIAN_POINT('Ctrl Pts',(-1.71399198684705,-23.1080344254286,
12.));
#226194=CARTESIAN_POINT('Ctrl Pts',(-1.71645271839298,-23.0923994621213,
0.));
#226195=CARTESIAN_POINT('Ctrl Pts',(-1.71645271839298,-23.0923994621213,
12.));
#226196=CARTESIAN_POINT('Ctrl Pts',(-1.71884453003028,-23.0768997860709,
0.));
#226197=CARTESIAN_POINT('Ctrl Pts',(-1.71884453003028,-23.0768997860709,
12.));
#226198=CARTESIAN_POINT('Ctrl Pts',(-1.72116787225993,-23.0615370351562,
0.));
#226199=CARTESIAN_POINT('Ctrl Pts',(-1.72116787225993,-23.0615370351562,
12.));
#226200=CARTESIAN_POINT('Ctrl Pts',(-1.72342320653748,-23.0463128785531,
0.));
#226201=CARTESIAN_POINT('Ctrl Pts',(-1.72342320653748,-23.0463128785531,
12.));
#226202=CARTESIAN_POINT('Ctrl Pts',(-1.72561100564047,-23.0312290178883,
0.));
#226203=CARTESIAN_POINT('Ctrl Pts',(-1.72561100564047,-23.0312290178883,
12.));
#226204=CARTESIAN_POINT('Ctrl Pts',(-1.7277317540471,-23.0162871884168,
0.));
#226205=CARTESIAN_POINT('Ctrl Pts',(-1.7277317540471,-23.0162871884168,
12.));
#226206=CARTESIAN_POINT('Ctrl Pts',(-1.72978594832137,-23.001489160189,
0.));
#226207=CARTESIAN_POINT('Ctrl Pts',(-1.72978594832137,-23.001489160189,
12.));
#226208=CARTESIAN_POINT('Ctrl Pts',(-1.73177409750192,-22.9868367391978,
0.));
#226209=CARTESIAN_POINT('Ctrl Pts',(-1.73177409750192,-22.9868367391978,
12.));
#226210=CARTESIAN_POINT('Ctrl Pts',(-1.73369672350816,-22.9723317685688,
0.));
#226211=CARTESIAN_POINT('Ctrl Pts',(-1.73369672350816,-22.9723317685688,
12.));
#226212=CARTESIAN_POINT('Ctrl Pts',(-1.7355543616277,-22.9579761301063,
0.));
#226213=CARTESIAN_POINT('Ctrl Pts',(-1.7355543616277,-22.9579761301063,
12.));
#226214=CARTESIAN_POINT('Ctrl Pts',(-1.7373475610004,-22.9437717457826,
0.));
#226215=CARTESIAN_POINT('Ctrl Pts',(-1.7373475610004,-22.9437717457826,
12.));
#226216=CARTESIAN_POINT('Ctrl Pts',(-1.73907688511667,-22.9297205792586,
0.));
#226217=CARTESIAN_POINT('Ctrl Pts',(-1.73907688511667,-22.9297205792586,
12.));
#226218=CARTESIAN_POINT('Ctrl Pts',(-1.74074291231059,-22.9158246373363,
0.));
#226219=CARTESIAN_POINT('Ctrl Pts',(-1.74074291231059,-22.9158246373363,
12.));
#226220=CARTESIAN_POINT('Ctrl Pts',(-1.74234623630081,-22.9020859716141,
0.));
#226221=CARTESIAN_POINT('Ctrl Pts',(-1.74234623630081,-22.9020859716141,
12.));
#226222=CARTESIAN_POINT('Ctrl Pts',(-1.74388746677703,-22.888506680335,
0.));
#226223=CARTESIAN_POINT('Ctrl Pts',(-1.74388746677703,-22.888506680335,
12.));
#226224=CARTESIAN_POINT('Ctrl Pts',(-1.74536722998202,-22.8750889101696,
0.));
#226225=CARTESIAN_POINT('Ctrl Pts',(-1.74536722998202,-22.8750889101696,
12.));
#226226=CARTESIAN_POINT('Ctrl Pts',(-1.74678616930666,-22.8618348580235,
0.));
#226227=CARTESIAN_POINT('Ctrl Pts',(-1.74678616930666,-22.8618348580235,
12.));
#226228=CARTESIAN_POINT('Ctrl Pts',(-1.74814494588494,-22.8487467728076,
0.));
#226229=CARTESIAN_POINT('Ctrl Pts',(-1.74814494588494,-22.8487467728076,
12.));
#226230=CARTESIAN_POINT('Ctrl Pts',(-1.74944423940117,-22.8358269579853,
0.));
#226231=CARTESIAN_POINT('Ctrl Pts',(-1.74944423940117,-22.8358269579853,
12.));
#226232=CARTESIAN_POINT('Ctrl Pts',(-1.75068474890884,-22.8230777741284,
0.));
#226233=CARTESIAN_POINT('Ctrl Pts',(-1.75068474890884,-22.8230777741284,
12.));
#226234=CARTESIAN_POINT('Ctrl Pts',(-1.75186719365593,-22.8105016414713,
0.));
#226235=CARTESIAN_POINT('Ctrl Pts',(-1.75186719365593,-22.8105016414713,
12.));
#226236=CARTESIAN_POINT('Ctrl Pts',(-1.75299231391467,-22.7981010424314,
0.));
#226237=CARTESIAN_POINT('Ctrl Pts',(-1.75299231391467,-22.7981010424314,
12.));
#226238=CARTESIAN_POINT('Ctrl Pts',(-1.75406087182937,-22.7858785242361,
0.));
#226239=CARTESIAN_POINT('Ctrl Pts',(-1.75406087182937,-22.7858785242361,
12.));
#226240=CARTESIAN_POINT('Ctrl Pts',(-1.75507365227133,-22.7738367016118,
0.));
#226241=CARTESIAN_POINT('Ctrl Pts',(-1.75507365227133,-22.7738367016118,
12.));
#226242=CARTESIAN_POINT('Ctrl Pts',(-1.75603146371642,-22.7619782595013,
0.));
#226243=CARTESIAN_POINT('Ctrl Pts',(-1.75603146371642,-22.7619782595013,
12.));
#226244=CARTESIAN_POINT('Ctrl Pts',(-1.75693513908908,-22.750305955645,
0.));
#226245=CARTESIAN_POINT('Ctrl Pts',(-1.75693513908908,-22.750305955645,
12.));
#226246=CARTESIAN_POINT('Ctrl Pts',(-1.75778553673245,-22.7388226235559,
0.));
#226247=CARTESIAN_POINT('Ctrl Pts',(-1.75778553673245,-22.7388226235559,
12.));
#226248=CARTESIAN_POINT('Ctrl Pts',(-1.75858354204634,-22.72753117773,0.));
#226249=CARTESIAN_POINT('Ctrl Pts',(-1.75858354204634,-22.72753117773,12.));
#226250=CARTESIAN_POINT('Ctrl Pts',(-1.75933006905926,-22.7164346186006,
0.));
#226251=CARTESIAN_POINT('Ctrl Pts',(-1.75933006905926,-22.7164346186006,
12.));
#226252=CARTESIAN_POINT('Ctrl Pts',(-1.76002606202402,-22.7055360375485,
0.));
#226253=CARTESIAN_POINT('Ctrl Pts',(-1.76002606202402,-22.7055360375485,
12.));
#226254=CARTESIAN_POINT('Ctrl Pts',(-1.76067249704888,-22.6948386219851,
0.));
#226255=CARTESIAN_POINT('Ctrl Pts',(-1.76067249704888,-22.6948386219851,
12.));
#226256=CARTESIAN_POINT('Ctrl Pts',(-1.76127038310615,-22.684345658525,
0.));
#226257=CARTESIAN_POINT('Ctrl Pts',(-1.76127038310615,-22.684345658525,
12.));
#226258=CARTESIAN_POINT('Ctrl Pts',(-1.76182076289527,-22.67406053567,0.));
#226259=CARTESIAN_POINT('Ctrl Pts',(-1.76182076289527,-22.67406053567,12.));
#226260=CARTESIAN_POINT('Ctrl Pts',(-1.7623247139257,-22.6639867471753,
0.));
#226261=CARTESIAN_POINT('Ctrl Pts',(-1.7623247139257,-22.6639867471753,
12.));
#226262=CARTESIAN_POINT('Ctrl Pts',(-1.76278334912562,-22.654127893841,
0.));
#226263=CARTESIAN_POINT('Ctrl Pts',(-1.76278334912562,-22.654127893841,
12.));
#226264=CARTESIAN_POINT('Ctrl Pts',(-1.76319782013917,-22.6444876940423,
0.));
#226265=CARTESIAN_POINT('Ctrl Pts',(-1.76319782013917,-22.6444876940423,
12.));
#226266=CARTESIAN_POINT('Ctrl Pts',(-1.76356932176274,-22.6350699979359,
0.));
#226267=CARTESIAN_POINT('Ctrl Pts',(-1.76356932176274,-22.6350699979359,
12.));
#226268=CARTESIAN_POINT('Ctrl Pts',(-1.76389909571404,-22.6258787994848,
0.));
#226269=CARTESIAN_POINT('Ctrl Pts',(-1.76389909571404,-22.6258787994848,
12.));
#226270=CARTESIAN_POINT('Ctrl Pts',(-1.7641884354374,-22.6169182517694,
0.));
#226271=CARTESIAN_POINT('Ctrl Pts',(-1.7641884354374,-22.6169182517694,
12.));
#226272=CARTESIAN_POINT('Ctrl Pts',(-1.76443868648017,-22.6081926681343,
0.));
#226273=CARTESIAN_POINT('Ctrl Pts',(-1.76443868648017,-22.6081926681343,
12.));
#226274=CARTESIAN_POINT('Ctrl Pts',(-1.76465124413558,-22.5997065145638,
0.));
#226275=CARTESIAN_POINT('Ctrl Pts',(-1.76465124413558,-22.5997065145638,
12.));
#226276=CARTESIAN_POINT('Ctrl Pts',(-1.76482755288412,-22.5914644078106,
0.));
#226277=CARTESIAN_POINT('Ctrl Pts',(-1.76482755288412,-22.5914644078106,
12.));
#226278=CARTESIAN_POINT('Ctrl Pts',(-1.76496910283089,-22.5834711038022,
0.));
#226279=CARTESIAN_POINT('Ctrl Pts',(-1.76496910283089,-22.5834711038022,
12.));
#226280=CARTESIAN_POINT('Ctrl Pts',(-1.76507744026747,-22.5757315316353,
0.));
#226281=CARTESIAN_POINT('Ctrl Pts',(-1.76507744026747,-22.5757315316353,
12.));
#226282=CARTESIAN_POINT('Ctrl Pts',(-1.76515418518832,-22.5682508499874,
0.));
#226283=CARTESIAN_POINT('Ctrl Pts',(-1.76515418518832,-22.5682508499874,
12.));
#226284=CARTESIAN_POINT('Ctrl Pts',(-1.76520104500451,-22.5610344912501,
0.));
#226285=CARTESIAN_POINT('Ctrl Pts',(-1.76520104500451,-22.5610344912501,
12.));
#226286=CARTESIAN_POINT('Ctrl Pts',(-1.76521983384063,-22.5540882235837,
0.));
#226287=CARTESIAN_POINT('Ctrl Pts',(-1.76521983384063,-22.5540882235837,
12.));
#226288=CARTESIAN_POINT('Ctrl Pts',(-1.76521245524048,-22.5474180954006,
0.));
#226289=CARTESIAN_POINT('Ctrl Pts',(-1.76521245524048,-22.5474180954006,
12.));
#226290=CARTESIAN_POINT('Ctrl Pts',(-1.76518087841494,-22.5410303590892,
0.));
#226291=CARTESIAN_POINT('Ctrl Pts',(-1.76518087841494,-22.5410303590892,
12.));
#226292=CARTESIAN_POINT('Ctrl Pts',(-1.76512711563255,-22.5349313983571,
0.));
#226293=CARTESIAN_POINT('Ctrl Pts',(-1.76512711563255,-22.5349313983571,
12.));
#226294=CARTESIAN_POINT('Ctrl Pts',(-1.7650532026276,-22.529127665298,0.));
#226295=CARTESIAN_POINT('Ctrl Pts',(-1.7650532026276,-22.529127665298,12.));
#226296=CARTESIAN_POINT('Ctrl Pts',(-1.76496128643376,-22.5236259635515,
0.));
#226297=CARTESIAN_POINT('Ctrl Pts',(-1.76496128643376,-22.5236259635515,
12.));
#226298=CARTESIAN_POINT('Ctrl Pts',(-1.76485369319896,-22.5184336670207,
0.));
#226299=CARTESIAN_POINT('Ctrl Pts',(-1.76485369319896,-22.5184336670207,
12.));
#226300=CARTESIAN_POINT('Ctrl Pts',(-1.7647330328115,-22.5135590569554,
0.));
#226301=CARTESIAN_POINT('Ctrl Pts',(-1.7647330328115,-22.5135590569554,
12.));
#226302=CARTESIAN_POINT('Ctrl Pts',(-1.76460218257314,-22.5090112700212,
0.));
#226303=CARTESIAN_POINT('Ctrl Pts',(-1.76460218257314,-22.5090112700212,
12.));
#226304=CARTESIAN_POINT('Ctrl Pts',(-1.76446408210366,-22.5047996391978,
0.));
#226305=CARTESIAN_POINT('Ctrl Pts',(-1.76446408210366,-22.5047996391978,
12.));
#226306=CARTESIAN_POINT('Ctrl Pts',(-1.76432160068739,-22.5009332677316,
0.));
#226307=CARTESIAN_POINT('Ctrl Pts',(-1.76432160068739,-22.5009332677316,
12.));
#226308=CARTESIAN_POINT('Ctrl Pts',(-1.76417731243484,-22.4974203063191,
0.));
#226309=CARTESIAN_POINT('Ctrl Pts',(-1.76417731243484,-22.4974203063191,
12.));
#226310=CARTESIAN_POINT('Ctrl Pts',(-1.76403393880317,-22.4942693792449,
0.));
#226311=CARTESIAN_POINT('Ctrl Pts',(-1.76403393880317,-22.4942693792449,
12.));
#226312=CARTESIAN_POINT('Ctrl Pts',(-1.76389475965715,-22.4914909094908,
0.));
#226313=CARTESIAN_POINT('Ctrl Pts',(-1.76389475965715,-22.4914909094908,
12.));
#226314=CARTESIAN_POINT('Ctrl Pts',(-1.76376424879469,-22.4890991659479,
0.));
#226315=CARTESIAN_POINT('Ctrl Pts',(-1.76376424879469,-22.4890991659479,
12.));
#226316=CARTESIAN_POINT('Ctrl Pts',(-1.76364784232926,-22.4871115206572,
0.));
#226317=CARTESIAN_POINT('Ctrl Pts',(-1.76364784232926,-22.4871115206572,
12.));
#226318=CARTESIAN_POINT('Ctrl Pts',(-1.7635507604555,-22.4855446605991,
0.));
#226319=CARTESIAN_POINT('Ctrl Pts',(-1.7635507604555,-22.4855446605991,
12.));
#226320=CARTESIAN_POINT('Ctrl Pts',(-1.76347698284863,-22.4844112933125,
0.));
#226321=CARTESIAN_POINT('Ctrl Pts',(-1.76347698284863,-22.4844112933125,
12.));
#226322=CARTESIAN_POINT('Ctrl Pts',(-1.7634381343466,-22.4838562517064,
0.));
#226323=CARTESIAN_POINT('Ctrl Pts',(-1.7634381343466,-22.4838562517064,
12.));
#226324=CARTESIAN_POINT('Ctrl Pts',(-1.76342064263638,-22.4836387052228,
0.));
#226325=CARTESIAN_POINT('Ctrl Pts',(-1.76342064263638,-22.4836387052228,
12.));
#226326=CARTESIAN_POINT('Ctrl Pts',(-1.76341415538792,-22.4835819929788,
0.));
#226327=CARTESIAN_POINT('Ctrl Pts',(-1.76341415538792,-22.4835819929788,
12.));
#226328=CARTESIAN_POINT('Ctrl Pts',(-1.76341220531181,-22.4835757167854,
0.));
#226329=CARTESIAN_POINT('Ctrl Pts',(-1.76341220531181,-22.4835757167854,
12.));
#226330=CARTESIAN_POINT('',(-0.661312440730913,-25.991588367311,0.));
#226331=CARTESIAN_POINT('Ctrl Pts',(-0.661312440730913,-25.991588367311,
0.));
#226332=CARTESIAN_POINT('Ctrl Pts',(-0.664028313187638,-25.9865613464773,
0.));
#226333=CARTESIAN_POINT('Ctrl Pts',(-0.669451306780837,-25.9765104298071,
0.));
#226334=CARTESIAN_POINT('Ctrl Pts',(-0.677559543209739,-25.9614434297919,
0.));
#226335=CARTESIAN_POINT('Ctrl Pts',(-0.688318015057743,-25.9413728471909,
0.));
#226336=CARTESIAN_POINT('Ctrl Pts',(-0.701678575228768,-25.9163158909426,
0.));
#226337=CARTESIAN_POINT('Ctrl Pts',(-0.714951588527651,-25.891290261497,
0.));
#226338=CARTESIAN_POINT('Ctrl Pts',(-0.728137036482348,-25.8662960624185,
0.));
#226339=CARTESIAN_POINT('Ctrl Pts',(-0.741234902663818,-25.8413334619055,
0.));
#226340=CARTESIAN_POINT('Ctrl Pts',(-0.754245175609535,-25.8164027059984,
0.));
#226341=CARTESIAN_POINT('Ctrl Pts',(-0.76716785265118,-25.7915041383376,
0.));
#226342=CARTESIAN_POINT('Ctrl Pts',(-0.780002940291976,-25.7666381946955,
0.));
#226343=CARTESIAN_POINT('Ctrl Pts',(-0.792750451616139,-25.7418053757746,
0.));
#226344=CARTESIAN_POINT('Ctrl Pts',(-0.805410404554365,-25.7170062262525,
0.));
#226345=CARTESIAN_POINT('Ctrl Pts',(-0.817982819787476,-25.6922413110194,
0.));
#226346=CARTESIAN_POINT('Ctrl Pts',(-0.830467718864218,-25.6675111931952,
0.));
#226347=CARTESIAN_POINT('Ctrl Pts',(-0.842865122120771,-25.6428164100055,
0.));
#226348=CARTESIAN_POINT('Ctrl Pts',(-0.85517504703656,-25.6181574536049,
0.));
#226349=CARTESIAN_POINT('Ctrl Pts',(-0.867397509338443,-25.5935347843585,
0.));
#226350=CARTESIAN_POINT('Ctrl Pts',(-0.879532523834307,-25.5689488408156,
0.));
#226351=CARTESIAN_POINT('Ctrl Pts',(-0.891580105349052,-25.5444000508211,
0.));
#226352=CARTESIAN_POINT('Ctrl Pts',(-0.903540269651119,-25.5198888424194,
0.));
#226353=CARTESIAN_POINT('Ctrl Pts',(-0.915413034335626,-25.4954156541795,
0.));
#226354=CARTESIAN_POINT('Ctrl Pts',(-0.927198419886107,-25.4709809475009,
0.));
#226355=CARTESIAN_POINT('Ctrl Pts',(-0.938896449496205,-25.4465852044849,
0.));
#226356=CARTESIAN_POINT('Ctrl Pts',(-0.950507148597481,-25.4222289223167,
0.));
#226357=CARTESIAN_POINT('Ctrl Pts',(-0.962030544503155,-25.3979126089163,
0.));
#226358=CARTESIAN_POINT('Ctrl Pts',(-0.973466666000176,-25.3736367778845,
0.));
#226359=CARTESIAN_POINT('Ctrl Pts',(-0.984815543003984,-25.3494019441441,
0.));
#226360=CARTESIAN_POINT('Ctrl Pts',(-0.996077206120636,-25.3252086182968,
0.));
#226361=CARTESIAN_POINT('Ctrl Pts',(-1.00725168656897,-25.3010573055548,
0.));
#226362=CARTESIAN_POINT('Ctrl Pts',(-1.01833901642238,-25.276948508726,
0.));
#226363=CARTESIAN_POINT('Ctrl Pts',(-1.02933922876807,-25.2528827300422,
0.));
#226364=CARTESIAN_POINT('Ctrl Pts',(-1.04025235791508,-25.2288604735086,
0.));
#226365=CARTESIAN_POINT('Ctrl Pts',(-1.05107843957933,-25.2048822469028,
0.));
#226366=CARTESIAN_POINT('Ctrl Pts',(-1.06181751111769,-25.1809485642192,
0.));
#226367=CARTESIAN_POINT('Ctrl Pts',(-1.07246961165477,-25.157059946931,
0.));
#226368=CARTESIAN_POINT('Ctrl Pts',(-1.08303478197189,-25.1332169227413,
0.));
#226369=CARTESIAN_POINT('Ctrl Pts',(-1.09351306445309,-25.1094200248446,
0.));
#226370=CARTESIAN_POINT('Ctrl Pts',(-1.10390450301746,-25.0856697909679,
0.));
#226371=CARTESIAN_POINT('Ctrl Pts',(-1.1142091430689,-25.0619667625336,
0.));
#226372=CARTESIAN_POINT('Ctrl Pts',(-1.12442703144453,-25.0383114836899,
0.));
#226373=CARTESIAN_POINT('Ctrl Pts',(-1.13455821638531,-25.0147045006196,
0.));
#226374=CARTESIAN_POINT('Ctrl Pts',(-1.14460274758202,-24.9911463621433,
0.));
#226375=CARTESIAN_POINT('Ctrl Pts',(-1.1545606762189,-24.9676376201502,
0.));
#226376=CARTESIAN_POINT('Ctrl Pts',(-1.16443205502851,-24.9441788300932,
0.));
#226377=CARTESIAN_POINT('Ctrl Pts',(-1.17421693835042,-24.9207705514448,
0.));
#226378=CARTESIAN_POINT('Ctrl Pts',(-1.18391538220104,-24.8974133481829,
0.));
#226379=CARTESIAN_POINT('Ctrl Pts',(-1.19352744434065,-24.8741077892075,
0.));
#226380=CARTESIAN_POINT('Ctrl Pts',(-1.20305318426021,-24.8508544481974,
0.));
#226381=CARTESIAN_POINT('Ctrl Pts',(-1.21249266318209,-24.8276539035092,
0.));
#226382=CARTESIAN_POINT('Ctrl Pts',(-1.22184594406529,-24.8045067380536,
0.));
#226383=CARTESIAN_POINT('Ctrl Pts',(-1.23111309161845,-24.7814135391799,
0.));
#226384=CARTESIAN_POINT('Ctrl Pts',(-1.2402941723199,-24.7583748985438,
0.));
#226385=CARTESIAN_POINT('Ctrl Pts',(-1.24938925444327,-24.7353914120011,
0.));
#226386=CARTESIAN_POINT('Ctrl Pts',(-1.25839840807419,-24.7124636797894,
0.));
#226387=CARTESIAN_POINT('Ctrl Pts',(-1.26732170513501,-24.6895923066836,
0.));
#226388=CARTESIAN_POINT('Ctrl Pts',(-1.27615921941643,-24.6667779021559,
0.));
#226389=CARTESIAN_POINT('Ctrl Pts',(-1.28491102661515,-24.6440210805278,
0.));
#226390=CARTESIAN_POINT('Ctrl Pts',(-1.29357720438108,-24.6213224611229,
0.));
#226391=CARTESIAN_POINT('Ctrl Pts',(-1.30215783236363,-24.5986826684027,
0.));
#226392=CARTESIAN_POINT('Ctrl Pts',(-1.31065299222023,-24.5761023320183,
0.));
#226393=CARTESIAN_POINT('Ctrl Pts',(-1.31906276763669,-24.5535820868674,
0.));
#226394=CARTESIAN_POINT('Ctrl Pts',(-1.32738724435327,-24.5311225731435,
0.));
#226395=CARTESIAN_POINT('Ctrl Pts',(-1.33562651019687,-24.5087244363856,
0.));
#226396=CARTESIAN_POINT('Ctrl Pts',(-1.34378065512339,-24.4863883275134,
0.));
#226397=CARTESIAN_POINT('Ctrl Pts',(-1.35184977125649,-24.4641149028892,
0.));
#226398=CARTESIAN_POINT('Ctrl Pts',(-1.35983395290628,-24.4419048244523,
0.));
#226399=CARTESIAN_POINT('Ctrl Pts',(-1.36773329659957,-24.4197587598337,
0.));
#226400=CARTESIAN_POINT('Ctrl Pts',(-1.3755479011161,-24.3976773824732,
0.));
#226401=CARTESIAN_POINT('Ctrl Pts',(-1.38327786753,-24.3756613717299,0.));
#226402=CARTESIAN_POINT('Ctrl Pts',(-1.39092329926389,-24.3537114129875,
0.));
#226403=CARTESIAN_POINT('Ctrl Pts',(-1.39848430212808,-24.3318281977643,
0.));
#226404=CARTESIAN_POINT('Ctrl Pts',(-1.40596098434338,-24.3100124238311,
0.));
#226405=CARTESIAN_POINT('Ctrl Pts',(-1.41335345657684,-24.288264795321,
0.));
#226406=CARTESIAN_POINT('Ctrl Pts',(-1.42066183198254,-24.2665860228356,
0.));
#226407=CARTESIAN_POINT('Ctrl Pts',(-1.42788622624855,-24.2449768235488,
0.));
#226408=CARTESIAN_POINT('Ctrl Pts',(-1.43502675765509,-24.2234379212984,
0.));
#226409=CARTESIAN_POINT('Ctrl Pts',(-1.44208354711083,-24.201970046722,
0.));
#226410=CARTESIAN_POINT('Ctrl Pts',(-1.44905671818729,-24.1805739374038,
0.));
#226411=CARTESIAN_POINT('Ctrl Pts',(-1.45594639716319,-24.1592503380107,
0.));
#226412=CARTESIAN_POINT('Ctrl Pts',(-1.46275271307399,-24.1380000004272,
0.));
#226413=CARTESIAN_POINT('Ctrl Pts',(-1.46947579776992,-24.1168236838824,
0.));
#226414=CARTESIAN_POINT('Ctrl Pts',(-1.47611578597743,-24.0957221550778,
0.));
#226415=CARTESIAN_POINT('Ctrl Pts',(-1.48267281533684,-24.0746961883528,
0.));
#226416=CARTESIAN_POINT('Ctrl Pts',(-1.48914702644888,-24.0537465658429,
0.));
#226417=CARTESIAN_POINT('Ctrl Pts',(-1.49553856292802,-24.0328740776331,
0.));
#226418=CARTESIAN_POINT('Ctrl Pts',(-1.501847571461,-24.0120795219086,0.));
#226419=CARTESIAN_POINT('Ctrl Pts',(-1.50807420187695,-23.9913637050927,
0.));
#226420=CARTESIAN_POINT('Ctrl Pts',(-1.51421860720615,-23.970727442014,
0.));
#226421=CARTESIAN_POINT('Ctrl Pts',(-1.52028094372793,-23.9501715561033,
0.));
#226422=CARTESIAN_POINT('Ctrl Pts',(-1.52626137103033,-23.9296968795757,
0.));
#226423=CARTESIAN_POINT('Ctrl Pts',(-1.53216005207464,-23.9093042536119,
0.));
#226424=CARTESIAN_POINT('Ctrl Pts',(-1.53797715326759,-23.8889945285318,
0.));
#226425=CARTESIAN_POINT('Ctrl Pts',(-1.54371284453991,-23.8687685639642,
0.));
#226426=CARTESIAN_POINT('Ctrl Pts',(-1.54936729940542,-23.8486272290705,
0.));
#226427=CARTESIAN_POINT('Ctrl Pts',(-1.55494069502636,-23.8285714027636,
0.));
#226428=CARTESIAN_POINT('Ctrl Pts',(-1.56043321228635,-23.8086019739194,
0.));
#226429=CARTESIAN_POINT('Ctrl Pts',(-1.56584503586844,-23.7887198415878,
0.));
#226430=CARTESIAN_POINT('Ctrl Pts',(-1.57117635434409,-23.7689259151862,
0.));
#226431=CARTESIAN_POINT('Ctrl Pts',(-1.57642736025247,-23.749221114736,
0.));
#226432=CARTESIAN_POINT('Ctrl Pts',(-1.58159825017359,-23.72960637113,0.));
#226433=CARTESIAN_POINT('Ctrl Pts',(-1.58668922481222,-23.710082626383,
0.));
#226434=CARTESIAN_POINT('Ctrl Pts',(-1.59170048908634,-23.6906508338833,
0.));
#226435=CARTESIAN_POINT('Ctrl Pts',(-1.59663225222464,-23.671311958631,
0.));
#226436=CARTESIAN_POINT('Ctrl Pts',(-1.60148472786596,-23.6520669774876,
0.));
#226437=CARTESIAN_POINT('Ctrl Pts',(-1.60625813414674,-23.6329168794929,
0.));
#226438=CARTESIAN_POINT('Ctrl Pts',(-1.61095269379779,-23.6138626661653,
0.));
#226439=CARTESIAN_POINT('Ctrl Pts',(-1.61556863424699,-23.5949053517997,
0.));
#226440=CARTESIAN_POINT('Ctrl Pts',(-1.62010618772867,-23.57604596376,0.));
#226441=CARTESIAN_POINT('Ctrl Pts',(-1.62456559140065,-23.5572855427601,
0.));
#226442=CARTESIAN_POINT('Ctrl Pts',(-1.62894708745224,-23.538625143226,
0.));
#226443=CARTESIAN_POINT('Ctrl Pts',(-1.63325092321727,-23.5200658336612,
0.));
#226444=CARTESIAN_POINT('Ctrl Pts',(-1.63747735129475,-23.5016086970003,
0.));
#226445=CARTESIAN_POINT('Ctrl Pts',(-1.64162662967529,-23.4832548309645,
0.));
#226446=CARTESIAN_POINT('Ctrl Pts',(-1.64569902187612,-23.4650053483932,
0.));
#226447=CARTESIAN_POINT('Ctrl Pts',(-1.64969479707341,-23.4468613776574,
0.));
#226448=CARTESIAN_POINT('Ctrl Pts',(-1.65361423023729,-23.4288240631043,
0.));
#226449=CARTESIAN_POINT('Ctrl Pts',(-1.65745760227506,-23.4108945654805,
0.));
#226450=CARTESIAN_POINT('Ctrl Pts',(-1.66122520018012,-23.3930740623619,
0.));
#226451=CARTESIAN_POINT('Ctrl Pts',(-1.66491731718878,-23.3753637485545,
0.));
#226452=CARTESIAN_POINT('Ctrl Pts',(-1.66853425293997,-23.3577648365744,
0.));
#226453=CARTESIAN_POINT('Ctrl Pts',(-1.67207631363923,-23.3402785571865,
0.));
#226454=CARTESIAN_POINT('Ctrl Pts',(-1.67554381222995,-23.3229061599145,
0.));
#226455=CARTESIAN_POINT('Ctrl Pts',(-1.67893706857118,-23.3056489135611,
0.));
#226456=CARTESIAN_POINT('Ctrl Pts',(-1.68225640962169,-23.2885081066951,
0.));
#226457=CARTESIAN_POINT('Ctrl Pts',(-1.68550216963259,-23.2714850482246,
0.));
#226458=CARTESIAN_POINT('Ctrl Pts',(-1.68867469034897,-23.2545810680537,
0.));
#226459=CARTESIAN_POINT('Ctrl Pts',(-1.69177432121712,-23.2377975177013,
0.));
#226460=CARTESIAN_POINT('Ctrl Pts',(-1.69480141959954,-23.2211357709374,
0.));
#226461=CARTESIAN_POINT('Ctrl Pts',(-1.69775635099444,-23.2045972243767,
0.));
#226462=CARTESIAN_POINT('Ctrl Pts',(-1.70063948927011,-23.1881832981851,
0.));
#226463=CARTESIAN_POINT('Ctrl Pts',(-1.70345121691277,-23.1718954368751,
0.));
#226464=CARTESIAN_POINT('Ctrl Pts',(-1.70619192527853,-23.1557351100614,
0.));
#226465=CARTESIAN_POINT('Ctrl Pts',(-1.70886201485453,-23.1397038132356,
0.));
#226466=CARTESIAN_POINT('Ctrl Pts',(-1.71146189552175,-23.1238030684925,
0.));
#226467=CARTESIAN_POINT('Ctrl Pts',(-1.71399198684705,-23.1080344254286,
0.));
#226468=CARTESIAN_POINT('Ctrl Pts',(-1.71645271839298,-23.0923994621213,
0.));
#226469=CARTESIAN_POINT('Ctrl Pts',(-1.71884453003028,-23.0768997860709,
0.));
#226470=CARTESIAN_POINT('Ctrl Pts',(-1.72116787225993,-23.0615370351562,
0.));
#226471=CARTESIAN_POINT('Ctrl Pts',(-1.72342320653748,-23.0463128785531,
0.));
#226472=CARTESIAN_POINT('Ctrl Pts',(-1.72561100564047,-23.0312290178883,
0.));
#226473=CARTESIAN_POINT('Ctrl Pts',(-1.7277317540471,-23.0162871884168,
0.));
#226474=CARTESIAN_POINT('Ctrl Pts',(-1.72978594832137,-23.001489160189,
0.));
#226475=CARTESIAN_POINT('Ctrl Pts',(-1.73177409750192,-22.9868367391978,
0.));
#226476=CARTESIAN_POINT('Ctrl Pts',(-1.73369672350816,-22.9723317685688,
0.));
#226477=CARTESIAN_POINT('Ctrl Pts',(-1.7355543616277,-22.9579761301063,
0.));
#226478=CARTESIAN_POINT('Ctrl Pts',(-1.7373475610004,-22.9437717457826,
0.));
#226479=CARTESIAN_POINT('Ctrl Pts',(-1.73907688511667,-22.9297205792586,
0.));
#226480=CARTESIAN_POINT('Ctrl Pts',(-1.74074291231059,-22.9158246373363,
0.));
#226481=CARTESIAN_POINT('Ctrl Pts',(-1.74234623630081,-22.9020859716141,
0.));
#226482=CARTESIAN_POINT('Ctrl Pts',(-1.74388746677703,-22.888506680335,
0.));
#226483=CARTESIAN_POINT('Ctrl Pts',(-1.74536722998202,-22.8750889101696,
0.));
#226484=CARTESIAN_POINT('Ctrl Pts',(-1.74678616930666,-22.8618348580235,
0.));
#226485=CARTESIAN_POINT('Ctrl Pts',(-1.74814494588494,-22.8487467728076,
0.));
#226486=CARTESIAN_POINT('Ctrl Pts',(-1.74944423940117,-22.8358269579853,
0.));
#226487=CARTESIAN_POINT('Ctrl Pts',(-1.75068474890884,-22.8230777741284,
0.));
#226488=CARTESIAN_POINT('Ctrl Pts',(-1.75186719365593,-22.8105016414713,
0.));
#226489=CARTESIAN_POINT('Ctrl Pts',(-1.75299231391467,-22.7981010424314,
0.));
#226490=CARTESIAN_POINT('Ctrl Pts',(-1.75406087182937,-22.7858785242361,
0.));
#226491=CARTESIAN_POINT('Ctrl Pts',(-1.75507365227133,-22.7738367016118,
0.));
#226492=CARTESIAN_POINT('Ctrl Pts',(-1.75603146371642,-22.7619782595013,
0.));
#226493=CARTESIAN_POINT('Ctrl Pts',(-1.75693513908908,-22.750305955645,
0.));
#226494=CARTESIAN_POINT('Ctrl Pts',(-1.75778553673245,-22.7388226235559,
0.));
#226495=CARTESIAN_POINT('Ctrl Pts',(-1.75858354204634,-22.72753117773,0.));
#226496=CARTESIAN_POINT('Ctrl Pts',(-1.75933006905926,-22.7164346186006,
0.));
#226497=CARTESIAN_POINT('Ctrl Pts',(-1.76002606202402,-22.7055360375485,
0.));
#226498=CARTESIAN_POINT('Ctrl Pts',(-1.76067249704888,-22.6948386219851,
0.));
#226499=CARTESIAN_POINT('Ctrl Pts',(-1.76127038310615,-22.684345658525,
0.));
#226500=CARTESIAN_POINT('Ctrl Pts',(-1.76182076289527,-22.67406053567,0.));
#226501=CARTESIAN_POINT('Ctrl Pts',(-1.7623247139257,-22.6639867471753,
0.));
#226502=CARTESIAN_POINT('Ctrl Pts',(-1.76278334912562,-22.654127893841,
0.));
#226503=CARTESIAN_POINT('Ctrl Pts',(-1.76319782013917,-22.6444876940423,
0.));
#226504=CARTESIAN_POINT('Ctrl Pts',(-1.76356932176274,-22.6350699979359,
0.));
#226505=CARTESIAN_POINT('Ctrl Pts',(-1.76389909571404,-22.6258787994848,
0.));
#226506=CARTESIAN_POINT('Ctrl Pts',(-1.7641884354374,-22.6169182517694,
0.));
#226507=CARTESIAN_POINT('Ctrl Pts',(-1.76443868648017,-22.6081926681343,
0.));
#226508=CARTESIAN_POINT('Ctrl Pts',(-1.76465124413558,-22.5997065145638,
0.));
#226509=CARTESIAN_POINT('Ctrl Pts',(-1.76482755288412,-22.5914644078106,
0.));
#226510=CARTESIAN_POINT('Ctrl Pts',(-1.76496910283089,-22.5834711038022,
0.));
#226511=CARTESIAN_POINT('Ctrl Pts',(-1.76507744026747,-22.5757315316353,
0.));
#226512=CARTESIAN_POINT('Ctrl Pts',(-1.76515418518832,-22.5682508499874,
0.));
#226513=CARTESIAN_POINT('Ctrl Pts',(-1.76520104500451,-22.5610344912501,
0.));
#226514=CARTESIAN_POINT('Ctrl Pts',(-1.76521983384063,-22.5540882235837,
0.));
#226515=CARTESIAN_POINT('Ctrl Pts',(-1.76521245524048,-22.5474180954006,
0.));
#226516=CARTESIAN_POINT('Ctrl Pts',(-1.76518087841494,-22.5410303590892,
0.));
#226517=CARTESIAN_POINT('Ctrl Pts',(-1.76512711563255,-22.5349313983571,
0.));
#226518=CARTESIAN_POINT('Ctrl Pts',(-1.7650532026276,-22.529127665298,0.));
#226519=CARTESIAN_POINT('Ctrl Pts',(-1.76496128643376,-22.5236259635515,
0.));
#226520=CARTESIAN_POINT('Ctrl Pts',(-1.76485369319896,-22.5184336670207,
0.));
#226521=CARTESIAN_POINT('Ctrl Pts',(-1.7647330328115,-22.5135590569554,
0.));
#226522=CARTESIAN_POINT('Ctrl Pts',(-1.76460218257314,-22.5090112700212,
0.));
#226523=CARTESIAN_POINT('Ctrl Pts',(-1.76446408210366,-22.5047996391978,
0.));
#226524=CARTESIAN_POINT('Ctrl Pts',(-1.76432160068739,-22.5009332677316,
0.));
#226525=CARTESIAN_POINT('Ctrl Pts',(-1.76417731243484,-22.4974203063191,
0.));
#226526=CARTESIAN_POINT('Ctrl Pts',(-1.76403393880317,-22.4942693792449,
0.));
#226527=CARTESIAN_POINT('Ctrl Pts',(-1.76389475965715,-22.4914909094908,
0.));
#226528=CARTESIAN_POINT('Ctrl Pts',(-1.76376424879469,-22.4890991659479,
0.));
#226529=CARTESIAN_POINT('Ctrl Pts',(-1.76364784232926,-22.4871115206572,
0.));
#226530=CARTESIAN_POINT('Ctrl Pts',(-1.7635507604555,-22.4855446605991,
0.));
#226531=CARTESIAN_POINT('Ctrl Pts',(-1.76347698284863,-22.4844112933125,
0.));
#226532=CARTESIAN_POINT('Ctrl Pts',(-1.7634381343466,-22.4838562517064,
0.));
#226533=CARTESIAN_POINT('Ctrl Pts',(-1.76342064263638,-22.4836387052228,
0.));
#226534=CARTESIAN_POINT('Ctrl Pts',(-1.76341415538792,-22.4835819929788,
0.));
#226535=CARTESIAN_POINT('Ctrl Pts',(-1.76341220531181,-22.4835757167854,
0.));
#226536=CARTESIAN_POINT('',(-0.661312440730913,-25.991588367311,12.));
#226537=CARTESIAN_POINT('',(-0.661312440730913,-25.991588367311,0.));
#226538=CARTESIAN_POINT('Ctrl Pts',(-1.76341220531181,-22.4835757167854,
12.));
#226539=CARTESIAN_POINT('Ctrl Pts',(-1.76341415538792,-22.4835819929788,
12.));
#226540=CARTESIAN_POINT('Ctrl Pts',(-1.76342064263638,-22.4836387052228,
12.));
#226541=CARTESIAN_POINT('Ctrl Pts',(-1.7634381343466,-22.4838562517064,
12.));
#226542=CARTESIAN_POINT('Ctrl Pts',(-1.76347698284863,-22.4844112933125,
12.));
#226543=CARTESIAN_POINT('Ctrl Pts',(-1.7635507604555,-22.4855446605991,
12.));
#226544=CARTESIAN_POINT('Ctrl Pts',(-1.76364784232926,-22.4871115206572,
12.));
#226545=CARTESIAN_POINT('Ctrl Pts',(-1.76376424879469,-22.4890991659479,
12.));
#226546=CARTESIAN_POINT('Ctrl Pts',(-1.76389475965715,-22.4914909094908,
12.));
#226547=CARTESIAN_POINT('Ctrl Pts',(-1.76403393880317,-22.4942693792449,
12.));
#226548=CARTESIAN_POINT('Ctrl Pts',(-1.76417731243484,-22.4974203063191,
12.));
#226549=CARTESIAN_POINT('Ctrl Pts',(-1.76432160068739,-22.5009332677316,
12.));
#226550=CARTESIAN_POINT('Ctrl Pts',(-1.76446408210366,-22.5047996391978,
12.));
#226551=CARTESIAN_POINT('Ctrl Pts',(-1.76460218257314,-22.5090112700212,
12.));
#226552=CARTESIAN_POINT('Ctrl Pts',(-1.7647330328115,-22.5135590569554,
12.));
#226553=CARTESIAN_POINT('Ctrl Pts',(-1.76485369319896,-22.5184336670207,
12.));
#226554=CARTESIAN_POINT('Ctrl Pts',(-1.76496128643376,-22.5236259635515,
12.));
#226555=CARTESIAN_POINT('Ctrl Pts',(-1.7650532026276,-22.529127665298,12.));
#226556=CARTESIAN_POINT('Ctrl Pts',(-1.76512711563255,-22.5349313983571,
12.));
#226557=CARTESIAN_POINT('Ctrl Pts',(-1.76518087841494,-22.5410303590892,
12.));
#226558=CARTESIAN_POINT('Ctrl Pts',(-1.76521245524048,-22.5474180954006,
12.));
#226559=CARTESIAN_POINT('Ctrl Pts',(-1.76521983384063,-22.5540882235837,
12.));
#226560=CARTESIAN_POINT('Ctrl Pts',(-1.76520104500451,-22.5610344912501,
12.));
#226561=CARTESIAN_POINT('Ctrl Pts',(-1.76515418518832,-22.5682508499874,
12.));
#226562=CARTESIAN_POINT('Ctrl Pts',(-1.76507744026747,-22.5757315316353,
12.));
#226563=CARTESIAN_POINT('Ctrl Pts',(-1.76496910283089,-22.5834711038022,
12.));
#226564=CARTESIAN_POINT('Ctrl Pts',(-1.76482755288412,-22.5914644078106,
12.));
#226565=CARTESIAN_POINT('Ctrl Pts',(-1.76465124413558,-22.5997065145638,
12.));
#226566=CARTESIAN_POINT('Ctrl Pts',(-1.76443868648017,-22.6081926681343,
12.));
#226567=CARTESIAN_POINT('Ctrl Pts',(-1.7641884354374,-22.6169182517694,
12.));
#226568=CARTESIAN_POINT('Ctrl Pts',(-1.76389909571404,-22.6258787994848,
12.));
#226569=CARTESIAN_POINT('Ctrl Pts',(-1.76356932176274,-22.6350699979359,
12.));
#226570=CARTESIAN_POINT('Ctrl Pts',(-1.76319782013917,-22.6444876940423,
12.));
#226571=CARTESIAN_POINT('Ctrl Pts',(-1.76278334912562,-22.654127893841,
12.));
#226572=CARTESIAN_POINT('Ctrl Pts',(-1.7623247139257,-22.6639867471753,
12.));
#226573=CARTESIAN_POINT('Ctrl Pts',(-1.76182076289527,-22.67406053567,12.));
#226574=CARTESIAN_POINT('Ctrl Pts',(-1.76127038310615,-22.684345658525,
12.));
#226575=CARTESIAN_POINT('Ctrl Pts',(-1.76067249704888,-22.6948386219851,
12.));
#226576=CARTESIAN_POINT('Ctrl Pts',(-1.76002606202402,-22.7055360375485,
12.));
#226577=CARTESIAN_POINT('Ctrl Pts',(-1.75933006905926,-22.7164346186006,
12.));
#226578=CARTESIAN_POINT('Ctrl Pts',(-1.75858354204634,-22.72753117773,12.));
#226579=CARTESIAN_POINT('Ctrl Pts',(-1.75778553673245,-22.7388226235559,
12.));
#226580=CARTESIAN_POINT('Ctrl Pts',(-1.75693513908908,-22.750305955645,
12.));
#226581=CARTESIAN_POINT('Ctrl Pts',(-1.75603146371642,-22.7619782595013,
12.));
#226582=CARTESIAN_POINT('Ctrl Pts',(-1.75507365227133,-22.7738367016118,
12.));
#226583=CARTESIAN_POINT('Ctrl Pts',(-1.75406087182937,-22.7858785242361,
12.));
#226584=CARTESIAN_POINT('Ctrl Pts',(-1.75299231391467,-22.7981010424314,
12.));
#226585=CARTESIAN_POINT('Ctrl Pts',(-1.75186719365593,-22.8105016414713,
12.));
#226586=CARTESIAN_POINT('Ctrl Pts',(-1.75068474890884,-22.8230777741284,
12.));
#226587=CARTESIAN_POINT('Ctrl Pts',(-1.74944423940117,-22.8358269579853,
12.));
#226588=CARTESIAN_POINT('Ctrl Pts',(-1.74814494588494,-22.8487467728076,
12.));
#226589=CARTESIAN_POINT('Ctrl Pts',(-1.74678616930666,-22.8618348580235,
12.));
#226590=CARTESIAN_POINT('Ctrl Pts',(-1.74536722998202,-22.8750889101696,
12.));
#226591=CARTESIAN_POINT('Ctrl Pts',(-1.74388746677703,-22.888506680335,
12.));
#226592=CARTESIAN_POINT('Ctrl Pts',(-1.74234623630081,-22.9020859716141,
12.));
#226593=CARTESIAN_POINT('Ctrl Pts',(-1.74074291231059,-22.9158246373363,
12.));
#226594=CARTESIAN_POINT('Ctrl Pts',(-1.73907688511667,-22.9297205792586,
12.));
#226595=CARTESIAN_POINT('Ctrl Pts',(-1.7373475610004,-22.9437717457826,
12.));
#226596=CARTESIAN_POINT('Ctrl Pts',(-1.7355543616277,-22.9579761301063,
12.));
#226597=CARTESIAN_POINT('Ctrl Pts',(-1.73369672350816,-22.9723317685688,
12.));
#226598=CARTESIAN_POINT('Ctrl Pts',(-1.73177409750192,-22.9868367391978,
12.));
#226599=CARTESIAN_POINT('Ctrl Pts',(-1.72978594832137,-23.001489160189,
12.));
#226600=CARTESIAN_POINT('Ctrl Pts',(-1.7277317540471,-23.0162871884168,
12.));
#226601=CARTESIAN_POINT('Ctrl Pts',(-1.72561100564047,-23.0312290178883,
12.));
#226602=CARTESIAN_POINT('Ctrl Pts',(-1.72342320653748,-23.0463128785531,
12.));
#226603=CARTESIAN_POINT('Ctrl Pts',(-1.72116787225993,-23.0615370351562,
12.));
#226604=CARTESIAN_POINT('Ctrl Pts',(-1.71884453003028,-23.0768997860709,
12.));
#226605=CARTESIAN_POINT('Ctrl Pts',(-1.71645271839298,-23.0923994621213,
12.));
#226606=CARTESIAN_POINT('Ctrl Pts',(-1.71399198684705,-23.1080344254286,
12.));
#226607=CARTESIAN_POINT('Ctrl Pts',(-1.71146189552175,-23.1238030684925,
12.));
#226608=CARTESIAN_POINT('Ctrl Pts',(-1.70886201485453,-23.1397038132356,
12.));
#226609=CARTESIAN_POINT('Ctrl Pts',(-1.70619192527853,-23.1557351100614,
12.));
#226610=CARTESIAN_POINT('Ctrl Pts',(-1.70345121691277,-23.1718954368751,
12.));
#226611=CARTESIAN_POINT('Ctrl Pts',(-1.70063948927011,-23.1881832981851,
12.));
#226612=CARTESIAN_POINT('Ctrl Pts',(-1.69775635099444,-23.2045972243767,
12.));
#226613=CARTESIAN_POINT('Ctrl Pts',(-1.69480141959954,-23.2211357709374,
12.));
#226614=CARTESIAN_POINT('Ctrl Pts',(-1.69177432121712,-23.2377975177013,
12.));
#226615=CARTESIAN_POINT('Ctrl Pts',(-1.68867469034897,-23.2545810680537,
12.));
#226616=CARTESIAN_POINT('Ctrl Pts',(-1.68550216963259,-23.2714850482246,
12.));
#226617=CARTESIAN_POINT('Ctrl Pts',(-1.68225640962169,-23.2885081066951,
12.));
#226618=CARTESIAN_POINT('Ctrl Pts',(-1.67893706857118,-23.3056489135611,
12.));
#226619=CARTESIAN_POINT('Ctrl Pts',(-1.67554381222995,-23.3229061599145,
12.));
#226620=CARTESIAN_POINT('Ctrl Pts',(-1.67207631363923,-23.3402785571865,
12.));
#226621=CARTESIAN_POINT('Ctrl Pts',(-1.66853425293997,-23.3577648365744,
12.));
#226622=CARTESIAN_POINT('Ctrl Pts',(-1.66491731718878,-23.3753637485545,
12.));
#226623=CARTESIAN_POINT('Ctrl Pts',(-1.66122520018012,-23.3930740623619,
12.));
#226624=CARTESIAN_POINT('Ctrl Pts',(-1.65745760227506,-23.4108945654805,
12.));
#226625=CARTESIAN_POINT('Ctrl Pts',(-1.65361423023729,-23.4288240631043,
12.));
#226626=CARTESIAN_POINT('Ctrl Pts',(-1.64969479707341,-23.4468613776574,
12.));
#226627=CARTESIAN_POINT('Ctrl Pts',(-1.64569902187612,-23.4650053483932,
12.));
#226628=CARTESIAN_POINT('Ctrl Pts',(-1.64162662967529,-23.4832548309645,
12.));
#226629=CARTESIAN_POINT('Ctrl Pts',(-1.63747735129475,-23.5016086970003,
12.));
#226630=CARTESIAN_POINT('Ctrl Pts',(-1.63325092321727,-23.5200658336612,
12.));
#226631=CARTESIAN_POINT('Ctrl Pts',(-1.62894708745224,-23.538625143226,
12.));
#226632=CARTESIAN_POINT('Ctrl Pts',(-1.62456559140065,-23.5572855427601,
12.));
#226633=CARTESIAN_POINT('Ctrl Pts',(-1.62010618772867,-23.57604596376,12.));
#226634=CARTESIAN_POINT('Ctrl Pts',(-1.61556863424699,-23.5949053517997,
12.));
#226635=CARTESIAN_POINT('Ctrl Pts',(-1.61095269379779,-23.6138626661653,
12.));
#226636=CARTESIAN_POINT('Ctrl Pts',(-1.60625813414674,-23.6329168794929,
12.));
#226637=CARTESIAN_POINT('Ctrl Pts',(-1.60148472786596,-23.6520669774876,
12.));
#226638=CARTESIAN_POINT('Ctrl Pts',(-1.59663225222464,-23.671311958631,
12.));
#226639=CARTESIAN_POINT('Ctrl Pts',(-1.59170048908634,-23.6906508338833,
12.));
#226640=CARTESIAN_POINT('Ctrl Pts',(-1.58668922481222,-23.710082626383,
12.));
#226641=CARTESIAN_POINT('Ctrl Pts',(-1.58159825017359,-23.72960637113,12.));
#226642=CARTESIAN_POINT('Ctrl Pts',(-1.57642736025247,-23.749221114736,
12.));
#226643=CARTESIAN_POINT('Ctrl Pts',(-1.57117635434409,-23.7689259151862,
12.));
#226644=CARTESIAN_POINT('Ctrl Pts',(-1.56584503586844,-23.7887198415878,
12.));
#226645=CARTESIAN_POINT('Ctrl Pts',(-1.56043321228635,-23.8086019739194,
12.));
#226646=CARTESIAN_POINT('Ctrl Pts',(-1.55494069502636,-23.8285714027636,
12.));
#226647=CARTESIAN_POINT('Ctrl Pts',(-1.54936729940542,-23.8486272290705,
12.));
#226648=CARTESIAN_POINT('Ctrl Pts',(-1.54371284453991,-23.8687685639642,
12.));
#226649=CARTESIAN_POINT('Ctrl Pts',(-1.53797715326759,-23.8889945285318,
12.));
#226650=CARTESIAN_POINT('Ctrl Pts',(-1.53216005207464,-23.9093042536119,
12.));
#226651=CARTESIAN_POINT('Ctrl Pts',(-1.52626137103033,-23.9296968795757,
12.));
#226652=CARTESIAN_POINT('Ctrl Pts',(-1.52028094372793,-23.9501715561033,
12.));
#226653=CARTESIAN_POINT('Ctrl Pts',(-1.51421860720615,-23.970727442014,
12.));
#226654=CARTESIAN_POINT('Ctrl Pts',(-1.50807420187695,-23.9913637050927,
12.));
#226655=CARTESIAN_POINT('Ctrl Pts',(-1.501847571461,-24.0120795219086,12.));
#226656=CARTESIAN_POINT('Ctrl Pts',(-1.49553856292802,-24.0328740776331,
12.));
#226657=CARTESIAN_POINT('Ctrl Pts',(-1.48914702644888,-24.0537465658429,
12.));
#226658=CARTESIAN_POINT('Ctrl Pts',(-1.48267281533684,-24.0746961883528,
12.));
#226659=CARTESIAN_POINT('Ctrl Pts',(-1.47611578597743,-24.0957221550778,
12.));
#226660=CARTESIAN_POINT('Ctrl Pts',(-1.46947579776992,-24.1168236838824,
12.));
#226661=CARTESIAN_POINT('Ctrl Pts',(-1.46275271307399,-24.1380000004272,
12.));
#226662=CARTESIAN_POINT('Ctrl Pts',(-1.45594639716319,-24.1592503380107,
12.));
#226663=CARTESIAN_POINT('Ctrl Pts',(-1.44905671818729,-24.1805739374038,
12.));
#226664=CARTESIAN_POINT('Ctrl Pts',(-1.44208354711083,-24.201970046722,
12.));
#226665=CARTESIAN_POINT('Ctrl Pts',(-1.43502675765509,-24.2234379212984,
12.));
#226666=CARTESIAN_POINT('Ctrl Pts',(-1.42788622624855,-24.2449768235488,
12.));
#226667=CARTESIAN_POINT('Ctrl Pts',(-1.42066183198254,-24.2665860228356,
12.));
#226668=CARTESIAN_POINT('Ctrl Pts',(-1.41335345657684,-24.288264795321,
12.));
#226669=CARTESIAN_POINT('Ctrl Pts',(-1.40596098434338,-24.3100124238311,
12.));
#226670=CARTESIAN_POINT('Ctrl Pts',(-1.39848430212808,-24.3318281977643,
12.));
#226671=CARTESIAN_POINT('Ctrl Pts',(-1.39092329926389,-24.3537114129875,
12.));
#226672=CARTESIAN_POINT('Ctrl Pts',(-1.38327786753,-24.3756613717299,12.));
#226673=CARTESIAN_POINT('Ctrl Pts',(-1.3755479011161,-24.3976773824732,
12.));
#226674=CARTESIAN_POINT('Ctrl Pts',(-1.36773329659957,-24.4197587598337,
12.));
#226675=CARTESIAN_POINT('Ctrl Pts',(-1.35983395290628,-24.4419048244523,
12.));
#226676=CARTESIAN_POINT('Ctrl Pts',(-1.35184977125649,-24.4641149028892,
12.));
#226677=CARTESIAN_POINT('Ctrl Pts',(-1.34378065512339,-24.4863883275134,
12.));
#226678=CARTESIAN_POINT('Ctrl Pts',(-1.33562651019687,-24.5087244363856,
12.));
#226679=CARTESIAN_POINT('Ctrl Pts',(-1.32738724435327,-24.5311225731435,
12.));
#226680=CARTESIAN_POINT('Ctrl Pts',(-1.31906276763669,-24.5535820868674,
12.));
#226681=CARTESIAN_POINT('Ctrl Pts',(-1.31065299222023,-24.5761023320183,
12.));
#226682=CARTESIAN_POINT('Ctrl Pts',(-1.30215783236363,-24.5986826684027,
12.));
#226683=CARTESIAN_POINT('Ctrl Pts',(-1.29357720438108,-24.6213224611229,
12.));
#226684=CARTESIAN_POINT('Ctrl Pts',(-1.28491102661515,-24.6440210805278,
12.));
#226685=CARTESIAN_POINT('Ctrl Pts',(-1.27615921941643,-24.6667779021559,
12.));
#226686=CARTESIAN_POINT('Ctrl Pts',(-1.26732170513501,-24.6895923066836,
12.));
#226687=CARTESIAN_POINT('Ctrl Pts',(-1.25839840807419,-24.7124636797894,
12.));
#226688=CARTESIAN_POINT('Ctrl Pts',(-1.24938925444327,-24.7353914120011,
12.));
#226689=CARTESIAN_POINT('Ctrl Pts',(-1.2402941723199,-24.7583748985438,
12.));
#226690=CARTESIAN_POINT('Ctrl Pts',(-1.23111309161845,-24.7814135391799,
12.));
#226691=CARTESIAN_POINT('Ctrl Pts',(-1.22184594406529,-24.8045067380536,
12.));
#226692=CARTESIAN_POINT('Ctrl Pts',(-1.21249266318209,-24.8276539035092,
12.));
#226693=CARTESIAN_POINT('Ctrl Pts',(-1.20305318426021,-24.8508544481974,
12.));
#226694=CARTESIAN_POINT('Ctrl Pts',(-1.19352744434065,-24.8741077892075,
12.));
#226695=CARTESIAN_POINT('Ctrl Pts',(-1.18391538220104,-24.8974133481829,
12.));
#226696=CARTESIAN_POINT('Ctrl Pts',(-1.17421693835042,-24.9207705514448,
12.));
#226697=CARTESIAN_POINT('Ctrl Pts',(-1.16443205502851,-24.9441788300932,
12.));
#226698=CARTESIAN_POINT('Ctrl Pts',(-1.1545606762189,-24.9676376201502,
12.));
#226699=CARTESIAN_POINT('Ctrl Pts',(-1.14460274758202,-24.9911463621433,
12.));
#226700=CARTESIAN_POINT('Ctrl Pts',(-1.13455821638531,-25.0147045006196,
12.));
#226701=CARTESIAN_POINT('Ctrl Pts',(-1.12442703144453,-25.0383114836899,
12.));
#226702=CARTESIAN_POINT('Ctrl Pts',(-1.1142091430689,-25.0619667625336,
12.));
#226703=CARTESIAN_POINT('Ctrl Pts',(-1.10390450301746,-25.0856697909679,
12.));
#226704=CARTESIAN_POINT('Ctrl Pts',(-1.09351306445309,-25.1094200248446,
12.));
#226705=CARTESIAN_POINT('Ctrl Pts',(-1.08303478197189,-25.1332169227413,
12.));
#226706=CARTESIAN_POINT('Ctrl Pts',(-1.07246961165477,-25.157059946931,
12.));
#226707=CARTESIAN_POINT('Ctrl Pts',(-1.06181751111769,-25.1809485642192,
12.));
#226708=CARTESIAN_POINT('Ctrl Pts',(-1.05107843957933,-25.2048822469028,
12.));
#226709=CARTESIAN_POINT('Ctrl Pts',(-1.04025235791508,-25.2288604735086,
12.));
#226710=CARTESIAN_POINT('Ctrl Pts',(-1.02933922876807,-25.2528827300422,
12.));
#226711=CARTESIAN_POINT('Ctrl Pts',(-1.01833901642238,-25.276948508726,
12.));
#226712=CARTESIAN_POINT('Ctrl Pts',(-1.00725168656897,-25.3010573055548,
12.));
#226713=CARTESIAN_POINT('Ctrl Pts',(-0.996077206120636,-25.3252086182968,
12.));
#226714=CARTESIAN_POINT('Ctrl Pts',(-0.984815543003984,-25.3494019441441,
12.));
#226715=CARTESIAN_POINT('Ctrl Pts',(-0.973466666000176,-25.3736367778845,
12.));
#226716=CARTESIAN_POINT('Ctrl Pts',(-0.962030544503155,-25.3979126089163,
12.));
#226717=CARTESIAN_POINT('Ctrl Pts',(-0.950507148597481,-25.4222289223167,
12.));
#226718=CARTESIAN_POINT('Ctrl Pts',(-0.938896449496205,-25.4465852044849,
12.));
#226719=CARTESIAN_POINT('Ctrl Pts',(-0.927198419886107,-25.4709809475009,
12.));
#226720=CARTESIAN_POINT('Ctrl Pts',(-0.915413034335626,-25.4954156541795,
12.));
#226721=CARTESIAN_POINT('Ctrl Pts',(-0.903540269651119,-25.5198888424194,
12.));
#226722=CARTESIAN_POINT('Ctrl Pts',(-0.891580105349052,-25.5444000508211,
12.));
#226723=CARTESIAN_POINT('Ctrl Pts',(-0.879532523834307,-25.5689488408156,
12.));
#226724=CARTESIAN_POINT('Ctrl Pts',(-0.867397509338443,-25.5935347843585,
12.));
#226725=CARTESIAN_POINT('Ctrl Pts',(-0.85517504703656,-25.6181574536049,
12.));
#226726=CARTESIAN_POINT('Ctrl Pts',(-0.842865122120771,-25.6428164100055,
12.));
#226727=CARTESIAN_POINT('Ctrl Pts',(-0.830467718864218,-25.6675111931952,
12.));
#226728=CARTESIAN_POINT('Ctrl Pts',(-0.817982819787476,-25.6922413110194,
12.));
#226729=CARTESIAN_POINT('Ctrl Pts',(-0.805410404554365,-25.7170062262525,
12.));
#226730=CARTESIAN_POINT('Ctrl Pts',(-0.792750451616139,-25.7418053757746,
12.));
#226731=CARTESIAN_POINT('Ctrl Pts',(-0.780002940291976,-25.7666381946955,
12.));
#226732=CARTESIAN_POINT('Ctrl Pts',(-0.76716785265118,-25.7915041383376,
12.));
#226733=CARTESIAN_POINT('Ctrl Pts',(-0.754245175609535,-25.8164027059984,
12.));
#226734=CARTESIAN_POINT('Ctrl Pts',(-0.741234902663818,-25.8413334619055,
12.));
#226735=CARTESIAN_POINT('Ctrl Pts',(-0.728137036482348,-25.8662960624185,
12.));
#226736=CARTESIAN_POINT('Ctrl Pts',(-0.714951588527651,-25.891290261497,
12.));
#226737=CARTESIAN_POINT('Ctrl Pts',(-0.701678575228768,-25.9163158909426,
12.));
#226738=CARTESIAN_POINT('Ctrl Pts',(-0.688318015057743,-25.9413728471909,
12.));
#226739=CARTESIAN_POINT('Ctrl Pts',(-0.677559543209739,-25.9614434297919,
12.));
#226740=CARTESIAN_POINT('Ctrl Pts',(-0.669451306780837,-25.9765104298071,
12.));
#226741=CARTESIAN_POINT('Ctrl Pts',(-0.664028313187638,-25.9865613464773,
12.));
#226742=CARTESIAN_POINT('Ctrl Pts',(-0.661312440730913,-25.991588367311,
12.));
#226743=CARTESIAN_POINT('Ctrl Pts',(-4.11585220600463,-22.1738711152697,
0.));
#226744=CARTESIAN_POINT('Ctrl Pts',(-4.11585220600463,-22.1738711152697,
12.));
#226745=CARTESIAN_POINT('Ctrl Pts',(-4.11585194677443,-22.173877682324,
0.));
#226746=CARTESIAN_POINT('Ctrl Pts',(-4.11585194677443,-22.173877682324,
12.));
#226747=CARTESIAN_POINT('Ctrl Pts',(-4.11586035878288,-22.1739341411687,
0.));
#226748=CARTESIAN_POINT('Ctrl Pts',(-4.11586035878288,-22.1739341411687,
12.));
#226749=CARTESIAN_POINT('Ctrl Pts',(-4.11589976826167,-22.1741488021234,
0.));
#226750=CARTESIAN_POINT('Ctrl Pts',(-4.11589976826167,-22.1741488021234,
12.));
#226751=CARTESIAN_POINT('Ctrl Pts',(-4.11600589882846,-22.1746949858775,
0.));
#226752=CARTESIAN_POINT('Ctrl Pts',(-4.11600589882846,-22.1746949858775,
12.));
#226753=CARTESIAN_POINT('Ctrl Pts',(-4.11622797217069,-22.1758088296598,
0.));
#226754=CARTESIAN_POINT('Ctrl Pts',(-4.11622797217069,-22.1758088296598,
12.));
#226755=CARTESIAN_POINT('Ctrl Pts',(-4.11653973150519,-22.177347426894,
0.));
#226756=CARTESIAN_POINT('Ctrl Pts',(-4.11653973150519,-22.177347426894,
12.));
#226757=CARTESIAN_POINT('Ctrl Pts',(-4.11694173195005,-22.179297473024,
0.));
#226758=CARTESIAN_POINT('Ctrl Pts',(-4.11694173195005,-22.179297473024,
12.));
#226759=CARTESIAN_POINT('Ctrl Pts',(-4.11743469691757,-22.1816414985788,
0.));
#226760=CARTESIAN_POINT('Ctrl Pts',(-4.11743469691757,-22.1816414985788,
12.));
#226761=CARTESIAN_POINT('Ctrl Pts',(-4.11801938107481,-22.1843613164855,
0.));
#226762=CARTESIAN_POINT('Ctrl Pts',(-4.11801938107481,-22.1843613164855,
12.));
#226763=CARTESIAN_POINT('Ctrl Pts',(-4.11869641271774,-22.1874419861496,
0.));
#226764=CARTESIAN_POINT('Ctrl Pts',(-4.11869641271774,-22.1874419861496,
12.));
#226765=CARTESIAN_POINT('Ctrl Pts',(-4.11946626228637,-22.1908725908525,
0.));
#226766=CARTESIAN_POINT('Ctrl Pts',(-4.11946626228637,-22.1908725908525,
12.));
#226767=CARTESIAN_POINT('Ctrl Pts',(-4.12032932637737,-22.1946440958098,
0.));
#226768=CARTESIAN_POINT('Ctrl Pts',(-4.12032932637737,-22.1946440958098,
12.));
#226769=CARTESIAN_POINT('Ctrl Pts',(-4.12128598183523,-22.1987479618246,
0.));
#226770=CARTESIAN_POINT('Ctrl Pts',(-4.12128598183523,-22.1987479618246,
12.));
#226771=CARTESIAN_POINT('Ctrl Pts',(-4.12233664408228,-22.2031746532106,
0.));
#226772=CARTESIAN_POINT('Ctrl Pts',(-4.12233664408228,-22.2031746532106,
12.));
#226773=CARTESIAN_POINT('Ctrl Pts',(-4.12348173702024,-22.2079143941719,
0.));
#226774=CARTESIAN_POINT('Ctrl Pts',(-4.12348173702024,-22.2079143941719,
12.));
#226775=CARTESIAN_POINT('Ctrl Pts',(-4.12472167516608,-22.2129576146671,
0.));
#226776=CARTESIAN_POINT('Ctrl Pts',(-4.12472167516608,-22.2129576146671,
12.));
#226777=CARTESIAN_POINT('Ctrl Pts',(-4.12605683613308,-22.2182956401341,
0.));
#226778=CARTESIAN_POINT('Ctrl Pts',(-4.12605683613308,-22.2182956401341,
12.));
#226779=CARTESIAN_POINT('Ctrl Pts',(-4.12748755830105,-22.2239207458781,
0.));
#226780=CARTESIAN_POINT('Ctrl Pts',(-4.12748755830105,-22.2239207458781,
12.));
#226781=CARTESIAN_POINT('Ctrl Pts',(-4.1290141546338,-22.2298258043947,
0.));
#226782=CARTESIAN_POINT('Ctrl Pts',(-4.1290141546338,-22.2298258043947,
12.));
#226783=CARTESIAN_POINT('Ctrl Pts',(-4.13063692157499,-22.2360040565533,
0.));
#226784=CARTESIAN_POINT('Ctrl Pts',(-4.13063692157499,-22.2360040565533,
12.));
#226785=CARTESIAN_POINT('Ctrl Pts',(-4.13235615060161,-22.2424488153523,
0.));
#226786=CARTESIAN_POINT('Ctrl Pts',(-4.13235615060161,-22.2424488153523,
12.));
#226787=CARTESIAN_POINT('Ctrl Pts',(-4.13417212558811,-22.249153531779,
0.));
#226788=CARTESIAN_POINT('Ctrl Pts',(-4.13417212558811,-22.249153531779,
12.));
#226789=CARTESIAN_POINT('Ctrl Pts',(-4.13608511977226,-22.2561118708421,
0.));
#226790=CARTESIAN_POINT('Ctrl Pts',(-4.13608511977226,-22.2561118708421,
12.));
#226791=CARTESIAN_POINT('Ctrl Pts',(-4.13809539255423,-22.2633177913972,
0.));
#226792=CARTESIAN_POINT('Ctrl Pts',(-4.13809539255423,-22.2633177913972,
12.));
#226793=CARTESIAN_POINT('Ctrl Pts',(-4.14020318715992,-22.2707656042457,
0.));
#226794=CARTESIAN_POINT('Ctrl Pts',(-4.14020318715992,-22.2707656042457,
12.));
#226795=CARTESIAN_POINT('Ctrl Pts',(-4.14240873321985,-22.2784499072027,
0.));
#226796=CARTESIAN_POINT('Ctrl Pts',(-4.14240873321985,-22.2784499072027,
12.));
#226797=CARTESIAN_POINT('Ctrl Pts',(-4.14471224859296,-22.2863655389166,
0.));
#226798=CARTESIAN_POINT('Ctrl Pts',(-4.14471224859296,-22.2863655389166,
12.));
#226799=CARTESIAN_POINT('Ctrl Pts',(-4.14711394168557,-22.2945075198467,
0.));
#226800=CARTESIAN_POINT('Ctrl Pts',(-4.14711394168557,-22.2945075198467,
12.));
#226801=CARTESIAN_POINT('Ctrl Pts',(-4.14961401285523,-22.3028710166933,
0.));
#226802=CARTESIAN_POINT('Ctrl Pts',(-4.14961401285523,-22.3028710166933,
12.));
#226803=CARTESIAN_POINT('Ctrl Pts',(-4.15221265396991,-22.3114513545185,
0.));
#226804=CARTESIAN_POINT('Ctrl Pts',(-4.15221265396991,-22.3114513545185,
12.));
#226805=CARTESIAN_POINT('Ctrl Pts',(-4.15491004835282,-22.320244018698,
0.));
#226806=CARTESIAN_POINT('Ctrl Pts',(-4.15491004835282,-22.320244018698,
12.));
#226807=CARTESIAN_POINT('Ctrl Pts',(-4.15770637047891,-22.3292446628959,
0.));
#226808=CARTESIAN_POINT('Ctrl Pts',(-4.15770637047891,-22.3292446628959,
12.));
#226809=CARTESIAN_POINT('Ctrl Pts',(-4.16060178604165,-22.3384491078602,
0.));
#226810=CARTESIAN_POINT('Ctrl Pts',(-4.16060178604165,-22.3384491078602,
12.));
#226811=CARTESIAN_POINT('Ctrl Pts',(-4.16359645263189,-22.3478533253889,
0.));
#226812=CARTESIAN_POINT('Ctrl Pts',(-4.16359645263189,-22.3478533253889,
12.));
#226813=CARTESIAN_POINT('Ctrl Pts',(-4.16669052026601,-22.3574534257396,
0.));
#226814=CARTESIAN_POINT('Ctrl Pts',(-4.16669052026601,-22.3574534257396,
12.));
#226815=CARTESIAN_POINT('Ctrl Pts',(-4.16988413199458,-22.36724564276,0.));
#226816=CARTESIAN_POINT('Ctrl Pts',(-4.16988413199458,-22.36724564276,12.));
#226817=CARTESIAN_POINT('Ctrl Pts',(-4.17317742436146,-22.3772263228617,
0.));
#226818=CARTESIAN_POINT('Ctrl Pts',(-4.17317742436146,-22.3772263228617,
12.));
#226819=CARTESIAN_POINT('Ctrl Pts',(-4.17657052752826,-22.3873919231334,
0.));
#226820=CARTESIAN_POINT('Ctrl Pts',(-4.17657052752826,-22.3873919231334,
12.));
#226821=CARTESIAN_POINT('Ctrl Pts',(-4.18006356544883,-22.3977390078075,
0.));
#226822=CARTESIAN_POINT('Ctrl Pts',(-4.18006356544883,-22.3977390078075,
12.));
#226823=CARTESIAN_POINT('Ctrl Pts',(-4.18365665600851,-22.4082642454453,
0.));
#226824=CARTESIAN_POINT('Ctrl Pts',(-4.18365665600851,-22.4082642454453,
12.));
#226825=CARTESIAN_POINT('Ctrl Pts',(-4.18734991117722,-22.4189644056115,
0.));
#226826=CARTESIAN_POINT('Ctrl Pts',(-4.18734991117722,-22.4189644056115,
12.));
#226827=CARTESIAN_POINT('Ctrl Pts',(-4.19114343726943,-22.4298363535421,
0.));
#226828=CARTESIAN_POINT('Ctrl Pts',(-4.19114343726943,-22.4298363535421,
12.));
#226829=CARTESIAN_POINT('Ctrl Pts',(-4.19503733518862,-22.4408770448917,
0.));
#226830=CARTESIAN_POINT('Ctrl Pts',(-4.19503733518862,-22.4408770448917,
12.));
#226831=CARTESIAN_POINT('Ctrl Pts',(-4.19903170066356,-22.4520835205419,
0.));
#226832=CARTESIAN_POINT('Ctrl Pts',(-4.19903170066356,-22.4520835205419,
12.));
#226833=CARTESIAN_POINT('Ctrl Pts',(-4.20312662448172,-22.4634529011433,
0.));
#226834=CARTESIAN_POINT('Ctrl Pts',(-4.20312662448172,-22.4634529011433,
12.));
#226835=CARTESIAN_POINT('Ctrl Pts',(-4.20732219265649,-22.4749823839915,
0.));
#226836=CARTESIAN_POINT('Ctrl Pts',(-4.20732219265649,-22.4749823839915,
12.));
#226837=CARTESIAN_POINT('Ctrl Pts',(-4.21161848657429,-22.4866692403147,
0.));
#226838=CARTESIAN_POINT('Ctrl Pts',(-4.21161848657429,-22.4866692403147,
12.));
#226839=CARTESIAN_POINT('Ctrl Pts',(-4.21601558313909,-22.4985108124229,
0.));
#226840=CARTESIAN_POINT('Ctrl Pts',(-4.21601558313909,-22.4985108124229,
12.));
#226841=CARTESIAN_POINT('Ctrl Pts',(-4.22051355490198,-22.5105045108882,
0.));
#226842=CARTESIAN_POINT('Ctrl Pts',(-4.22051355490198,-22.5105045108882,
12.));
#226843=CARTESIAN_POINT('Ctrl Pts',(-4.22511247020041,-22.5226478117885,
0.));
#226844=CARTESIAN_POINT('Ctrl Pts',(-4.22511247020041,-22.5226478117885,
12.));
#226845=CARTESIAN_POINT('Ctrl Pts',(-4.22981239330732,-22.5349382540587,
0.));
#226846=CARTESIAN_POINT('Ctrl Pts',(-4.22981239330732,-22.5349382540587,
12.));
#226847=CARTESIAN_POINT('Ctrl Pts',(-4.23461338456714,-22.5473734368086,
0.));
#226848=CARTESIAN_POINT('Ctrl Pts',(-4.23461338456714,-22.5473734368086,
12.));
#226849=CARTESIAN_POINT('Ctrl Pts',(-4.23951550052527,-22.559951016643,
0.));
#226850=CARTESIAN_POINT('Ctrl Pts',(-4.23951550052527,-22.559951016643,
12.));
#226851=CARTESIAN_POINT('Ctrl Pts',(-4.2445187940486,-22.5726687049922,
0.));
#226852=CARTESIAN_POINT('Ctrl Pts',(-4.2445187940486,-22.5726687049922,
12.));
#226853=CARTESIAN_POINT('Ctrl Pts',(-4.24962331444186,-22.5855242662479,
0.));
#226854=CARTESIAN_POINT('Ctrl Pts',(-4.24962331444186,-22.5855242662479,
12.));
#226855=CARTESIAN_POINT('Ctrl Pts',(-4.25482910755486,-22.5985155158637,
0.));
#226856=CARTESIAN_POINT('Ctrl Pts',(-4.25482910755486,-22.5985155158637,
12.));
#226857=CARTESIAN_POINT('Ctrl Pts',(-4.26013621588304,-22.611640318482,
0.));
#226858=CARTESIAN_POINT('Ctrl Pts',(-4.26013621588304,-22.611640318482,
12.));
#226859=CARTESIAN_POINT('Ctrl Pts',(-4.26554467865572,-22.6248965859975,
0.));
#226860=CARTESIAN_POINT('Ctrl Pts',(-4.26554467865572,-22.6248965859975,
12.));
#226861=CARTESIAN_POINT('Ctrl Pts',(-4.27105453193,-22.6382822758171,0.));
#226862=CARTESIAN_POINT('Ctrl Pts',(-4.27105453193,-22.6382822758171,12.));
#226863=CARTESIAN_POINT('Ctrl Pts',(-4.27666580869118,-22.6517953893303,
0.));
#226864=CARTESIAN_POINT('Ctrl Pts',(-4.27666580869118,-22.6517953893303,
12.));
#226865=CARTESIAN_POINT('Ctrl Pts',(-4.2823785389406,-22.665433970311,0.));
#226866=CARTESIAN_POINT('Ctrl Pts',(-4.2823785389406,-22.665433970311,12.));
#226867=CARTESIAN_POINT('Ctrl Pts',(-4.28819274977767,-22.6791961033536,
0.));
#226868=CARTESIAN_POINT('Ctrl Pts',(-4.28819274977767,-22.6791961033536,
12.));
#226869=CARTESIAN_POINT('Ctrl Pts',(-4.29410846547062,-22.6930799122545,
0.));
#226870=CARTESIAN_POINT('Ctrl Pts',(-4.29410846547062,-22.6930799122545,
12.));
#226871=CARTESIAN_POINT('Ctrl Pts',(-4.30012570754067,-22.707083558756,
0.));
#226872=CARTESIAN_POINT('Ctrl Pts',(-4.30012570754067,-22.707083558756,
12.));
#226873=CARTESIAN_POINT('Ctrl Pts',(-4.30624449484075,-22.7212052413384,
0.));
#226874=CARTESIAN_POINT('Ctrl Pts',(-4.30624449484075,-22.7212052413384,
12.));
#226875=CARTESIAN_POINT('Ctrl Pts',(-4.31246484362551,-22.7354431939926,
0.));
#226876=CARTESIAN_POINT('Ctrl Pts',(-4.31246484362551,-22.7354431939926,
12.));
#226877=CARTESIAN_POINT('Ctrl Pts',(-4.31878676761231,-22.7497956849852,
0.));
#226878=CARTESIAN_POINT('Ctrl Pts',(-4.31878676761231,-22.7497956849852,
12.));
#226879=CARTESIAN_POINT('Ctrl Pts',(-4.32521027803748,-22.764261015648,
0.));
#226880=CARTESIAN_POINT('Ctrl Pts',(-4.32521027803748,-22.764261015648,
12.));
#226881=CARTESIAN_POINT('Ctrl Pts',(-4.33173538373183,-22.7788375194081,
0.));
#226882=CARTESIAN_POINT('Ctrl Pts',(-4.33173538373183,-22.7788375194081,
12.));
#226883=CARTESIAN_POINT('Ctrl Pts',(-4.33836209118444,-22.7935235607807,
0.));
#226884=CARTESIAN_POINT('Ctrl Pts',(-4.33836209118444,-22.7935235607807,
12.));
#226885=CARTESIAN_POINT('Ctrl Pts',(-4.34509040460066,-22.808317534379,
0.));
#226886=CARTESIAN_POINT('Ctrl Pts',(-4.34509040460066,-22.808317534379,
12.));
#226887=CARTESIAN_POINT('Ctrl Pts',(-4.35192032594802,-22.8232178638873,
0.));
#226888=CARTESIAN_POINT('Ctrl Pts',(-4.35192032594802,-22.8232178638873,
12.));
#226889=CARTESIAN_POINT('Ctrl Pts',(-4.3588518550056,-22.838223001118,0.));
#226890=CARTESIAN_POINT('Ctrl Pts',(-4.3588518550056,-22.838223001118,12.));
#226891=CARTESIAN_POINT('Ctrl Pts',(-4.36588498943011,-22.8533314252419,
0.));
#226892=CARTESIAN_POINT('Ctrl Pts',(-4.36588498943011,-22.8533314252419,
12.));
#226893=CARTESIAN_POINT('Ctrl Pts',(-4.37301972480753,-22.8685416419725,
0.));
#226894=CARTESIAN_POINT('Ctrl Pts',(-4.37301972480753,-22.8685416419725,
12.));
#226895=CARTESIAN_POINT('Ctrl Pts',(-4.38025605470091,-22.8838521827702,
0.));
#226896=CARTESIAN_POINT('Ctrl Pts',(-4.38025605470091,-22.8838521827702,
12.));
#226897=CARTESIAN_POINT('Ctrl Pts',(-4.38759397068393,-22.8992616040108,
0.));
#226898=CARTESIAN_POINT('Ctrl Pts',(-4.38759397068393,-22.8992616040108,
12.));
#226899=CARTESIAN_POINT('Ctrl Pts',(-4.39503346238455,-22.9147684862425,
0.));
#226900=CARTESIAN_POINT('Ctrl Pts',(-4.39503346238455,-22.9147684862425,
12.));
#226901=CARTESIAN_POINT('Ctrl Pts',(-4.40257451754308,-22.9303714335549,
0.));
#226902=CARTESIAN_POINT('Ctrl Pts',(-4.40257451754308,-22.9303714335549,
12.));
#226903=CARTESIAN_POINT('Ctrl Pts',(-4.41021712205549,-22.9460690729093,
0.));
#226904=CARTESIAN_POINT('Ctrl Pts',(-4.41021712205549,-22.9460690729093,
12.));
#226905=CARTESIAN_POINT('Ctrl Pts',(-4.41796126001311,-22.9618600534866,
0.));
#226906=CARTESIAN_POINT('Ctrl Pts',(-4.41796126001311,-22.9618600534866,
12.));
#226907=CARTESIAN_POINT('Ctrl Pts',(-4.42580691372772,-22.9777430460021,
0.));
#226908=CARTESIAN_POINT('Ctrl Pts',(-4.42580691372772,-22.9777430460021,
12.));
#226909=CARTESIAN_POINT('Ctrl Pts',(-4.43375406376906,-22.9937167421009,
0.));
#226910=CARTESIAN_POINT('Ctrl Pts',(-4.43375406376906,-22.9937167421009,
12.));
#226911=CARTESIAN_POINT('Ctrl Pts',(-4.44180268901667,-23.0097798538399,
0.));
#226912=CARTESIAN_POINT('Ctrl Pts',(-4.44180268901667,-23.0097798538399,
12.));
#226913=CARTESIAN_POINT('Ctrl Pts',(-4.44995276669699,-23.0259311131395,
0.));
#226914=CARTESIAN_POINT('Ctrl Pts',(-4.44995276669699,-23.0259311131395,
12.));
#226915=CARTESIAN_POINT('Ctrl Pts',(-4.45820427241677,-23.0421692712466,
0.));
#226916=CARTESIAN_POINT('Ctrl Pts',(-4.45820427241677,-23.0421692712466,
12.));
#226917=CARTESIAN_POINT('Ctrl Pts',(-4.46655718018206,-23.0584930981723,
0.));
#226918=CARTESIAN_POINT('Ctrl Pts',(-4.46655718018206,-23.0584930981723,
12.));
#226919=CARTESIAN_POINT('Ctrl Pts',(-4.47501146242822,-23.0749013821867,
0.));
#226920=CARTESIAN_POINT('Ctrl Pts',(-4.47501146242822,-23.0749013821867,
12.));
#226921=CARTESIAN_POINT('Ctrl Pts',(-4.48356709006757,-23.0913929293909,
0.));
#226922=CARTESIAN_POINT('Ctrl Pts',(-4.48356709006757,-23.0913929293909,
12.));
#226923=CARTESIAN_POINT('Ctrl Pts',(-4.49222403252202,-23.1079665632629,
0.));
#226924=CARTESIAN_POINT('Ctrl Pts',(-4.49222403252202,-23.1079665632629,
12.));
#226925=CARTESIAN_POINT('Ctrl Pts',(-4.50098225775179,-23.1246211242117,
0.));
#226926=CARTESIAN_POINT('Ctrl Pts',(-4.50098225775179,-23.1246211242117,
12.));
#226927=CARTESIAN_POINT('Ctrl Pts',(-4.50984173227088,-23.1413554691136,
0.));
#226928=CARTESIAN_POINT('Ctrl Pts',(-4.50984173227088,-23.1413554691136,
12.));
#226929=CARTESIAN_POINT('Ctrl Pts',(-4.51880242116786,-23.1581684708778,
0.));
#226930=CARTESIAN_POINT('Ctrl Pts',(-4.51880242116786,-23.1581684708778,
12.));
#226931=CARTESIAN_POINT('Ctrl Pts',(-4.52786428815049,-23.1750590180923,
0.));
#226932=CARTESIAN_POINT('Ctrl Pts',(-4.52786428815049,-23.1750590180923,
12.));
#226933=CARTESIAN_POINT('Ctrl Pts',(-4.53702729557586,-23.1920260146474,
0.));
#226934=CARTESIAN_POINT('Ctrl Pts',(-4.53702729557586,-23.1920260146474,
12.));
#226935=CARTESIAN_POINT('Ctrl Pts',(-4.54629140447543,-23.2090683793627,
0.));
#226936=CARTESIAN_POINT('Ctrl Pts',(-4.54629140447543,-23.2090683793627,
12.));
#226937=CARTESIAN_POINT('Ctrl Pts',(-4.55565657456957,-23.2261850456055,
0.));
#226938=CARTESIAN_POINT('Ctrl Pts',(-4.55565657456957,-23.2261850456055,
12.));
#226939=CARTESIAN_POINT('Ctrl Pts',(-4.56512276427812,-23.2433749609117,
0.));
#226940=CARTESIAN_POINT('Ctrl Pts',(-4.56512276427812,-23.2433749609117,
12.));
#226941=CARTESIAN_POINT('Ctrl Pts',(-4.57468993076071,-23.2606370866854,
0.));
#226942=CARTESIAN_POINT('Ctrl Pts',(-4.57468993076071,-23.2606370866854,
12.));
#226943=CARTESIAN_POINT('Ctrl Pts',(-4.58435802994675,-23.2779703978868,
0.));
#226944=CARTESIAN_POINT('Ctrl Pts',(-4.58435802994675,-23.2779703978868,
12.));
#226945=CARTESIAN_POINT('Ctrl Pts',(-4.5941270165575,-23.295373882719,0.));
#226946=CARTESIAN_POINT('Ctrl Pts',(-4.5941270165575,-23.295373882719,12.));
#226947=CARTESIAN_POINT('Ctrl Pts',(-4.60399684412176,-23.3128465423119,
0.));
#226948=CARTESIAN_POINT('Ctrl Pts',(-4.60399684412176,-23.3128465423119,
12.));
#226949=CARTESIAN_POINT('Ctrl Pts',(-4.61396746497849,-23.3303873903947,
0.));
#226950=CARTESIAN_POINT('Ctrl Pts',(-4.61396746497849,-23.3303873903947,
12.));
#226951=CARTESIAN_POINT('Ctrl Pts',(-4.62403883030825,-23.3479954530281,
0.));
#226952=CARTESIAN_POINT('Ctrl Pts',(-4.62403883030825,-23.3479954530281,
12.));
#226953=CARTESIAN_POINT('Ctrl Pts',(-4.63421089016555,-23.3656697683496,
0.));
#226954=CARTESIAN_POINT('Ctrl Pts',(-4.63421089016555,-23.3656697683496,
12.));
#226955=CARTESIAN_POINT('Ctrl Pts',(-4.64448359349936,-23.383409386307,
0.));
#226956=CARTESIAN_POINT('Ctrl Pts',(-4.64448359349936,-23.383409386307,
12.));
#226957=CARTESIAN_POINT('Ctrl Pts',(-4.65485688816923,-23.4012133683957,
0.));
#226958=CARTESIAN_POINT('Ctrl Pts',(-4.65485688816923,-23.4012133683957,
12.));
#226959=CARTESIAN_POINT('Ctrl Pts',(-4.66533072094664,-23.4190807873798,
0.));
#226960=CARTESIAN_POINT('Ctrl Pts',(-4.66533072094664,-23.4190807873798,
12.));
#226961=CARTESIAN_POINT('Ctrl Pts',(-4.67590503753051,-23.4370107270444,
0.));
#226962=CARTESIAN_POINT('Ctrl Pts',(-4.67590503753051,-23.4370107270444,
12.));
#226963=CARTESIAN_POINT('Ctrl Pts',(-4.68657978258298,-23.4550022819852,
0.));
#226964=CARTESIAN_POINT('Ctrl Pts',(-4.68657978258298,-23.4550022819852,
12.));
#226965=CARTESIAN_POINT('Ctrl Pts',(-4.69735489975024,-23.4730545573849,
0.));
#226966=CARTESIAN_POINT('Ctrl Pts',(-4.69735489975024,-23.4730545573849,
12.));
#226967=CARTESIAN_POINT('Ctrl Pts',(-4.70823033167821,-23.491166668789,
0.));
#226968=CARTESIAN_POINT('Ctrl Pts',(-4.70823033167821,-23.491166668789,
12.));
#226969=CARTESIAN_POINT('Ctrl Pts',(-4.71920602001905,-23.5093377418784,
0.));
#226970=CARTESIAN_POINT('Ctrl Pts',(-4.71920602001905,-23.5093377418784,
12.));
#226971=CARTESIAN_POINT('Ctrl Pts',(-4.73028190543032,-23.5275669122378,
0.));
#226972=CARTESIAN_POINT('Ctrl Pts',(-4.73028190543032,-23.5275669122378,
12.));
#226973=CARTESIAN_POINT('Ctrl Pts',(-4.74145792760699,-23.5458533251715,
0.));
#226974=CARTESIAN_POINT('Ctrl Pts',(-4.74145792760699,-23.5458533251715,
12.));
#226975=CARTESIAN_POINT('Ctrl Pts',(-4.75273402530616,-23.564196135517,
0.));
#226976=CARTESIAN_POINT('Ctrl Pts',(-4.75273402530616,-23.564196135517,
12.));
#226977=CARTESIAN_POINT('Ctrl Pts',(-4.76411013636252,-23.5825945074535,
0.));
#226978=CARTESIAN_POINT('Ctrl Pts',(-4.76411013636252,-23.5825945074535,
12.));
#226979=CARTESIAN_POINT('Ctrl Pts',(-4.77558619769876,-23.6010476143099,
0.));
#226980=CARTESIAN_POINT('Ctrl Pts',(-4.77558619769876,-23.6010476143099,
12.));
#226981=CARTESIAN_POINT('Ctrl Pts',(-4.78716214532105,-23.6195546383625,
0.));
#226982=CARTESIAN_POINT('Ctrl Pts',(-4.78716214532105,-23.6195546383625,
12.));
#226983=CARTESIAN_POINT('Ctrl Pts',(-4.79883791433231,-23.6381147706581,
0.));
#226984=CARTESIAN_POINT('Ctrl Pts',(-4.79883791433231,-23.6381147706581,
12.));
#226985=CARTESIAN_POINT('Ctrl Pts',(-4.81061343896443,-23.6567272108631,
0.));
#226986=CARTESIAN_POINT('Ctrl Pts',(-4.81061343896443,-23.6567272108631,
12.));
#226987=CARTESIAN_POINT('Ctrl Pts',(-4.82248865259571,-23.6753911671023,
0.));
#226988=CARTESIAN_POINT('Ctrl Pts',(-4.82248865259571,-23.6753911671023,
12.));
#226989=CARTESIAN_POINT('Ctrl Pts',(-4.83446348776268,-23.6941058557971,
0.));
#226990=CARTESIAN_POINT('Ctrl Pts',(-4.83446348776268,-23.6941058557971,
12.));
#226991=CARTESIAN_POINT('Ctrl Pts',(-4.84653787616424,-23.7128705015014,
0.));
#226992=CARTESIAN_POINT('Ctrl Pts',(-4.84653787616424,-23.7128705015014,
12.));
#226993=CARTESIAN_POINT('Ctrl Pts',(-4.85871174865492,-23.7316843367308,
0.));
#226994=CARTESIAN_POINT('Ctrl Pts',(-4.85871174865492,-23.7316843367308,
12.));
#226995=CARTESIAN_POINT('Ctrl Pts',(-4.87098503527144,-23.7505466018239,
0.));
#226996=CARTESIAN_POINT('Ctrl Pts',(-4.87098503527144,-23.7505466018239,
12.));
#226997=CARTESIAN_POINT('Ctrl Pts',(-4.88335766525566,-23.7694565448044,
0.));
#226998=CARTESIAN_POINT('Ctrl Pts',(-4.88335766525566,-23.7694565448044,
12.));
#226999=CARTESIAN_POINT('Ctrl Pts',(-4.89582956706772,-23.7884134212381,
0.));
#227000=CARTESIAN_POINT('Ctrl Pts',(-4.89582956706772,-23.7884134212381,
12.));
#227001=CARTESIAN_POINT('Ctrl Pts',(-4.90840066839348,-23.8074164940897,
0.));
#227002=CARTESIAN_POINT('Ctrl Pts',(-4.90840066839348,-23.8074164940897,
12.));
#227003=CARTESIAN_POINT('Ctrl Pts',(-4.92107089613977,-23.8264650335721,
0.));
#227004=CARTESIAN_POINT('Ctrl Pts',(-4.92107089613977,-23.8264650335721,
12.));
#227005=CARTESIAN_POINT('Ctrl Pts',(-4.93384017643442,-23.8455583170062,
0.));
#227006=CARTESIAN_POINT('Ctrl Pts',(-4.93384017643442,-23.8455583170062,
12.));
#227007=CARTESIAN_POINT('Ctrl Pts',(-4.94670843465869,-23.8646956287172,
0.));
#227008=CARTESIAN_POINT('Ctrl Pts',(-4.94670843465869,-23.8646956287172,
12.));
#227009=CARTESIAN_POINT('Ctrl Pts',(-4.95967559546566,-23.883876259922,
0.));
#227010=CARTESIAN_POINT('Ctrl Pts',(-4.95967559546566,-23.883876259922,
12.));
#227011=CARTESIAN_POINT('Ctrl Pts',(-4.9727415827923,-23.9030995086164,
0.));
#227012=CARTESIAN_POINT('Ctrl Pts',(-4.9727415827923,-23.9030995086164,
12.));
#227013=CARTESIAN_POINT('Ctrl Pts',(-4.98590631986534,-23.9223646794591,
0.));
#227014=CARTESIAN_POINT('Ctrl Pts',(-4.98590631986534,-23.9223646794591,
12.));
#227015=CARTESIAN_POINT('Ctrl Pts',(-4.9991697291931,-23.9416710836529,
0.));
#227016=CARTESIAN_POINT('Ctrl Pts',(-4.9991697291931,-23.9416710836529,
12.));
#227017=CARTESIAN_POINT('Ctrl Pts',(-5.01253173257459,-23.9610180388271,
0.));
#227018=CARTESIAN_POINT('Ctrl Pts',(-5.01253173257459,-23.9610180388271,
12.));
#227019=CARTESIAN_POINT('Ctrl Pts',(-5.02599225112462,-23.9804048689228,
0.));
#227020=CARTESIAN_POINT('Ctrl Pts',(-5.02599225112462,-23.9804048689228,
12.));
#227021=CARTESIAN_POINT('Ctrl Pts',(-5.03955120528528,-23.9998309040747,
0.));
#227022=CARTESIAN_POINT('Ctrl Pts',(-5.03955120528528,-23.9998309040747,
12.));
#227023=CARTESIAN_POINT('Ctrl Pts',(-5.05320851483069,-24.0192954804896,
0.));
#227024=CARTESIAN_POINT('Ctrl Pts',(-5.05320851483069,-24.0192954804896,
12.));
#227025=CARTESIAN_POINT('Ctrl Pts',(-5.0669640988664,-24.0387979403268,
0.));
#227026=CARTESIAN_POINT('Ctrl Pts',(-5.0669640988664,-24.0387979403268,
12.));
#227027=CARTESIAN_POINT('Ctrl Pts',(-5.08081787581271,-24.0583376315636,
0.));
#227028=CARTESIAN_POINT('Ctrl Pts',(-5.08081787581271,-24.0583376315636,
12.));
#227029=CARTESIAN_POINT('Ctrl Pts',(-5.09476976342618,-24.0779139079264,
0.));
#227030=CARTESIAN_POINT('Ctrl Pts',(-5.09476976342618,-24.0779139079264,
12.));
#227031=CARTESIAN_POINT('Ctrl Pts',(-5.10881967883126,-24.0975261288444,
0.));
#227032=CARTESIAN_POINT('Ctrl Pts',(-5.10881967883126,-24.0975261288444,
12.));
#227033=CARTESIAN_POINT('Ctrl Pts',(-5.12296753853858,-24.117173659394,
0.));
#227034=CARTESIAN_POINT('Ctrl Pts',(-5.12296753853858,-24.117173659394,
12.));
#227035=CARTESIAN_POINT('Ctrl Pts',(-5.13721325845746,-24.1368558702443,
0.));
#227036=CARTESIAN_POINT('Ctrl Pts',(-5.13721325845746,-24.1368558702443,
12.));
#227037=CARTESIAN_POINT('Ctrl Pts',(-5.1515567539008,-24.1565721375971,
0.));
#227038=CARTESIAN_POINT('Ctrl Pts',(-5.1515567539008,-24.1565721375971,
12.));
#227039=CARTESIAN_POINT('Ctrl Pts',(-5.16599793957987,-24.1763218431344,
0.));
#227040=CARTESIAN_POINT('Ctrl Pts',(-5.16599793957987,-24.1763218431344,
12.));
#227041=CARTESIAN_POINT('Ctrl Pts',(-5.180536729614,-24.1961043738756,0.));
#227042=CARTESIAN_POINT('Ctrl Pts',(-5.180536729614,-24.1961043738756,12.));
#227043=CARTESIAN_POINT('Ctrl Pts',(-5.19517303753648,-24.2159191220171,
0.));
#227044=CARTESIAN_POINT('Ctrl Pts',(-5.19517303753648,-24.2159191220171,
12.));
#227045=CARTESIAN_POINT('Ctrl Pts',(-5.20990677629177,-24.2357654847766,
0.));
#227046=CARTESIAN_POINT('Ctrl Pts',(-5.20990677629177,-24.2357654847766,
12.));
#227047=CARTESIAN_POINT('Ctrl Pts',(-5.22473785822443,-24.2556428642294,
0.));
#227048=CARTESIAN_POINT('Ctrl Pts',(-5.22473785822443,-24.2556428642294,
12.));
#227049=CARTESIAN_POINT('Ctrl Pts',(-5.2396661950629,-24.2755506671525,
0.));
#227050=CARTESIAN_POINT('Ctrl Pts',(-5.2396661950629,-24.2755506671525,
12.));
#227051=CARTESIAN_POINT('Ctrl Pts',(-5.25469169788857,-24.2954883048447,
0.));
#227052=CARTESIAN_POINT('Ctrl Pts',(-5.25469169788857,-24.2954883048447,
12.));
#227053=CARTESIAN_POINT('Ctrl Pts',(-5.269814277188,-24.3154551932221,0.));
#227054=CARTESIAN_POINT('Ctrl Pts',(-5.269814277188,-24.3154551932221,12.));
#227055=CARTESIAN_POINT('Ctrl Pts',(-5.28503384290649,-24.3354507529414,
0.));
#227056=CARTESIAN_POINT('Ctrl Pts',(-5.28503384290649,-24.3354507529414,
12.));
#227057=CARTESIAN_POINT('Ctrl Pts',(-5.30035030449064,-24.3554744095075,
0.));
#227058=CARTESIAN_POINT('Ctrl Pts',(-5.30035030449064,-24.3554744095075,
12.));
#227059=CARTESIAN_POINT('Ctrl Pts',(-5.31576357092527,-24.3755255933917,
0.));
#227060=CARTESIAN_POINT('Ctrl Pts',(-5.31576357092527,-24.3755255933917,
12.));
#227061=CARTESIAN_POINT('Ctrl Pts',(-5.33127355076035,-24.3956037401293,
0.));
#227062=CARTESIAN_POINT('Ctrl Pts',(-5.33127355076035,-24.3956037401293,
12.));
#227063=CARTESIAN_POINT('Ctrl Pts',(-5.34688015213538,-24.4157082904614,
0.));
#227064=CARTESIAN_POINT('Ctrl Pts',(-5.34688015213538,-24.4157082904614,
12.));
#227065=CARTESIAN_POINT('Ctrl Pts',(-5.36258328273628,-24.435838689915,
0.));
#227066=CARTESIAN_POINT('Ctrl Pts',(-5.36258328273628,-24.435838689915,
12.));
#227067=CARTESIAN_POINT('Ctrl Pts',(-5.37838284973696,-24.4559943883157,
0.));
#227068=CARTESIAN_POINT('Ctrl Pts',(-5.37838284973696,-24.4559943883157,
12.));
#227069=CARTESIAN_POINT('Ctrl Pts',(-5.39427875973825,-24.4761748393321,
0.));
#227070=CARTESIAN_POINT('Ctrl Pts',(-5.39427875973825,-24.4761748393321,
12.));
#227071=CARTESIAN_POINT('Ctrl Pts',(-5.41027091869242,-24.496379499983,
0.));
#227072=CARTESIAN_POINT('Ctrl Pts',(-5.41027091869242,-24.496379499983,
12.));
#227073=CARTESIAN_POINT('Ctrl Pts',(-5.4263592318342,-24.5166078302108,
0.));
#227074=CARTESIAN_POINT('Ctrl Pts',(-5.4263592318342,-24.5166078302108,
12.));
#227075=CARTESIAN_POINT('Ctrl Pts',(-5.44254360356881,-24.5368592922863,
0.));
#227076=CARTESIAN_POINT('Ctrl Pts',(-5.44254360356881,-24.5368592922863,
12.));
#227077=CARTESIAN_POINT('Ctrl Pts',(-5.45882393762262,-24.5571333514842,
0.));
#227078=CARTESIAN_POINT('Ctrl Pts',(-5.45882393762262,-24.5571333514842,
12.));
#227079=CARTESIAN_POINT('Ctrl Pts',(-5.4752001372442,-24.5774294770329,
0.));
#227080=CARTESIAN_POINT('Ctrl Pts',(-5.4752001372442,-24.5774294770329,
12.));
#227081=CARTESIAN_POINT('Ctrl Pts',(-5.49167210537248,-24.5977471429364,
0.));
#227082=CARTESIAN_POINT('Ctrl Pts',(-5.49167210537248,-24.5977471429364,
12.));
#227083=CARTESIAN_POINT('Ctrl Pts',(-5.50823974481963,-24.6180858289179,
0.));
#227084=CARTESIAN_POINT('Ctrl Pts',(-5.50823974481963,-24.6180858289179,
12.));
#227085=CARTESIAN_POINT('Ctrl Pts',(-5.52490295840993,-24.6384450211467,
0.));
#227086=CARTESIAN_POINT('Ctrl Pts',(-5.52490295840993,-24.6384450211467,
12.));
#227087=CARTESIAN_POINT('Ctrl Pts',(-5.54166164919584,-24.6588242134738,
0.));
#227088=CARTESIAN_POINT('Ctrl Pts',(-5.54166164919584,-24.6588242134738,
12.));
#227089=CARTESIAN_POINT('Ctrl Pts',(-5.55851572025377,-24.6792229061794,
0.));
#227090=CARTESIAN_POINT('Ctrl Pts',(-5.55851572025377,-24.6792229061794,
12.));
#227091=CARTESIAN_POINT('Ctrl Pts',(-5.57546507427756,-24.6996406035517,
0.));
#227092=CARTESIAN_POINT('Ctrl Pts',(-5.57546507427756,-24.6996406035517,
12.));
#227093=CARTESIAN_POINT('Ctrl Pts',(-5.59250961323988,-24.7200768119088,
0.));
#227094=CARTESIAN_POINT('Ctrl Pts',(-5.59250961323988,-24.7200768119088,
12.));
#227095=CARTESIAN_POINT('Ctrl Pts',(-5.60964923798492,-24.7405310372739,
0.));
#227096=CARTESIAN_POINT('Ctrl Pts',(-5.60964923798492,-24.7405310372739,
12.));
#227097=CARTESIAN_POINT('Ctrl Pts',(-5.62688384790924,-24.7610027835697,
0.));
#227098=CARTESIAN_POINT('Ctrl Pts',(-5.62688384790924,-24.7610027835697,
12.));
#227099=CARTESIAN_POINT('Ctrl Pts',(-5.64421334042262,-24.781491549672,
0.));
#227100=CARTESIAN_POINT('Ctrl Pts',(-5.64421334042262,-24.781491549672,
12.));
#227101=CARTESIAN_POINT('Ctrl Pts',(-5.66163761114922,-24.8019968304605,
0.));
#227102=CARTESIAN_POINT('Ctrl Pts',(-5.66163761114922,-24.8019968304605,
12.));
#227103=CARTESIAN_POINT('Ctrl Pts',(-5.67915655496543,-24.8225181223845,
0.));
#227104=CARTESIAN_POINT('Ctrl Pts',(-5.67915655496543,-24.8225181223845,
12.));
#227105=CARTESIAN_POINT('Ctrl Pts',(-5.69677006679445,-24.8430549277621,
0.));
#227106=CARTESIAN_POINT('Ctrl Pts',(-5.69677006679445,-24.8430549277621,
12.));
#227107=CARTESIAN_POINT('Ctrl Pts',(-5.71447804252028,-24.8636067597669,
0.));
#227108=CARTESIAN_POINT('Ctrl Pts',(-5.71447804252028,-24.8636067597669,
12.));
#227109=CARTESIAN_POINT('Ctrl Pts',(-5.73228037976928,-24.884173146722,
0.));
#227110=CARTESIAN_POINT('Ctrl Pts',(-5.73228037976928,-24.884173146722,
12.));
#227111=CARTESIAN_POINT('Ctrl Pts',(-5.75017697890805,-24.904753637648,
0.));
#227112=CARTESIAN_POINT('Ctrl Pts',(-5.75017697890805,-24.904753637648,
12.));
#227113=CARTESIAN_POINT('Ctrl Pts',(-5.76816774342221,-24.9253478043656,
0.));
#227114=CARTESIAN_POINT('Ctrl Pts',(-5.76816774342221,-24.9253478043656,
12.));
#227115=CARTESIAN_POINT('Ctrl Pts',(-5.78625257775682,-24.945955229334,
0.));
#227116=CARTESIAN_POINT('Ctrl Pts',(-5.78625257775682,-24.945955229334,
12.));
#227117=CARTESIAN_POINT('Ctrl Pts',(-5.80443138549727,-24.9665754954496,
0.));
#227118=CARTESIAN_POINT('Ctrl Pts',(-5.80443138549727,-24.9665754954496,
12.));
#227119=CARTESIAN_POINT('Ctrl Pts',(-5.822704067442,-24.9872081752734,0.));
#227120=CARTESIAN_POINT('Ctrl Pts',(-5.822704067442,-24.9872081752734,12.));
#227121=CARTESIAN_POINT('Ctrl Pts',(-5.84107051963072,-25.0078528200564,
0.));
#227122=CARTESIAN_POINT('Ctrl Pts',(-5.84107051963072,-25.0078528200564,
12.));
#227123=CARTESIAN_POINT('Ctrl Pts',(-5.85953063156827,-25.0285089498899,
0.));
#227124=CARTESIAN_POINT('Ctrl Pts',(-5.85953063156827,-25.0285089498899,
12.));
#227125=CARTESIAN_POINT('Ctrl Pts',(-5.87808428385367,-25.049176040591,
0.));
#227126=CARTESIAN_POINT('Ctrl Pts',(-5.87808428385367,-25.049176040591,
12.));
#227127=CARTESIAN_POINT('Ctrl Pts',(-5.89673135155515,-25.0698535426514,
0.));
#227128=CARTESIAN_POINT('Ctrl Pts',(-5.89673135155515,-25.0698535426514,
12.));
#227129=CARTESIAN_POINT('Ctrl Pts',(-5.91547170844448,-25.0905409050773,
0.));
#227130=CARTESIAN_POINT('Ctrl Pts',(-5.91547170844448,-25.0905409050773,
12.));
#227131=CARTESIAN_POINT('Ctrl Pts',(-5.93430523086836,-25.1112375971106,
0.));
#227132=CARTESIAN_POINT('Ctrl Pts',(-5.93430523086836,-25.1112375971106,
12.));
#227133=CARTESIAN_POINT('Ctrl Pts',(-5.95323180187379,-25.1319431317237,
0.));
#227134=CARTESIAN_POINT('Ctrl Pts',(-5.95323180187379,-25.1319431317237,
12.));
#227135=CARTESIAN_POINT('Ctrl Pts',(-5.97225131495618,-25.1526570863092,
0.));
#227136=CARTESIAN_POINT('Ctrl Pts',(-5.97225131495618,-25.1526570863092,
12.));
#227137=CARTESIAN_POINT('Ctrl Pts',(-5.99136367859755,-25.1733791296259,
0.));
#227138=CARTESIAN_POINT('Ctrl Pts',(-5.99136367859755,-25.1733791296259,
12.));
#227139=CARTESIAN_POINT('Ctrl Pts',(-6.01056881804614,-25.1941090269819,
0.));
#227140=CARTESIAN_POINT('Ctrl Pts',(-6.01056881804614,-25.1941090269819,
12.));
#227141=CARTESIAN_POINT('Ctrl Pts',(-6.02986667389998,-25.21484662016,0.));
#227142=CARTESIAN_POINT('Ctrl Pts',(-6.02986667389998,-25.21484662016,12.));
#227143=CARTESIAN_POINT('Ctrl Pts',(-6.04925720151219,-25.2355918139032,
0.));
#227144=CARTESIAN_POINT('Ctrl Pts',(-6.04925720151219,-25.2355918139032,
12.));
#227145=CARTESIAN_POINT('Ctrl Pts',(-6.06484373634547,-25.2521940105705,
0.));
#227146=CARTESIAN_POINT('Ctrl Pts',(-6.06484373634547,-25.2521940105705,
12.));
#227147=CARTESIAN_POINT('Ctrl Pts',(-6.07657531787491,-25.2646490489922,
0.));
#227148=CARTESIAN_POINT('Ctrl Pts',(-6.07657531787491,-25.2646490489922,
12.));
#227149=CARTESIAN_POINT('Ctrl Pts',(-6.08441489609794,-25.2729539149517,
0.));
#227150=CARTESIAN_POINT('Ctrl Pts',(-6.08441489609794,-25.2729539149517,
12.));
#227151=CARTESIAN_POINT('Ctrl Pts',(-6.088339316177,-25.2771067246846,0.));
#227152=CARTESIAN_POINT('Ctrl Pts',(-6.088339316177,-25.2771067246846,12.));
#227153=CARTESIAN_POINT('',(-6.088339316177,-25.2771067246846,0.));
#227154=CARTESIAN_POINT('Ctrl Pts',(-4.11585220600463,-22.1738711152697,
0.));
#227155=CARTESIAN_POINT('Ctrl Pts',(-4.11585194677443,-22.173877682324,
0.));
#227156=CARTESIAN_POINT('Ctrl Pts',(-4.11586035878288,-22.1739341411687,
0.));
#227157=CARTESIAN_POINT('Ctrl Pts',(-4.11589976826167,-22.1741488021234,
0.));
#227158=CARTESIAN_POINT('Ctrl Pts',(-4.11600589882846,-22.1746949858775,
0.));
#227159=CARTESIAN_POINT('Ctrl Pts',(-4.11622797217069,-22.1758088296598,
0.));
#227160=CARTESIAN_POINT('Ctrl Pts',(-4.11653973150519,-22.177347426894,
0.));
#227161=CARTESIAN_POINT('Ctrl Pts',(-4.11694173195005,-22.179297473024,
0.));
#227162=CARTESIAN_POINT('Ctrl Pts',(-4.11743469691757,-22.1816414985788,
0.));
#227163=CARTESIAN_POINT('Ctrl Pts',(-4.11801938107481,-22.1843613164855,
0.));
#227164=CARTESIAN_POINT('Ctrl Pts',(-4.11869641271774,-22.1874419861496,
0.));
#227165=CARTESIAN_POINT('Ctrl Pts',(-4.11946626228637,-22.1908725908525,
0.));
#227166=CARTESIAN_POINT('Ctrl Pts',(-4.12032932637737,-22.1946440958098,
0.));
#227167=CARTESIAN_POINT('Ctrl Pts',(-4.12128598183523,-22.1987479618246,
0.));
#227168=CARTESIAN_POINT('Ctrl Pts',(-4.12233664408228,-22.2031746532106,
0.));
#227169=CARTESIAN_POINT('Ctrl Pts',(-4.12348173702024,-22.2079143941719,
0.));
#227170=CARTESIAN_POINT('Ctrl Pts',(-4.12472167516608,-22.2129576146671,
0.));
#227171=CARTESIAN_POINT('Ctrl Pts',(-4.12605683613308,-22.2182956401341,
0.));
#227172=CARTESIAN_POINT('Ctrl Pts',(-4.12748755830105,-22.2239207458781,
0.));
#227173=CARTESIAN_POINT('Ctrl Pts',(-4.1290141546338,-22.2298258043947,
0.));
#227174=CARTESIAN_POINT('Ctrl Pts',(-4.13063692157499,-22.2360040565533,
0.));
#227175=CARTESIAN_POINT('Ctrl Pts',(-4.13235615060161,-22.2424488153523,
0.));
#227176=CARTESIAN_POINT('Ctrl Pts',(-4.13417212558811,-22.249153531779,
0.));
#227177=CARTESIAN_POINT('Ctrl Pts',(-4.13608511977226,-22.2561118708421,
0.));
#227178=CARTESIAN_POINT('Ctrl Pts',(-4.13809539255423,-22.2633177913972,
0.));
#227179=CARTESIAN_POINT('Ctrl Pts',(-4.14020318715992,-22.2707656042457,
0.));
#227180=CARTESIAN_POINT('Ctrl Pts',(-4.14240873321985,-22.2784499072027,
0.));
#227181=CARTESIAN_POINT('Ctrl Pts',(-4.14471224859296,-22.2863655389166,
0.));
#227182=CARTESIAN_POINT('Ctrl Pts',(-4.14711394168557,-22.2945075198467,
0.));
#227183=CARTESIAN_POINT('Ctrl Pts',(-4.14961401285523,-22.3028710166933,
0.));
#227184=CARTESIAN_POINT('Ctrl Pts',(-4.15221265396991,-22.3114513545185,
0.));
#227185=CARTESIAN_POINT('Ctrl Pts',(-4.15491004835282,-22.320244018698,
0.));
#227186=CARTESIAN_POINT('Ctrl Pts',(-4.15770637047891,-22.3292446628959,
0.));
#227187=CARTESIAN_POINT('Ctrl Pts',(-4.16060178604165,-22.3384491078602,
0.));
#227188=CARTESIAN_POINT('Ctrl Pts',(-4.16359645263189,-22.3478533253889,
0.));
#227189=CARTESIAN_POINT('Ctrl Pts',(-4.16669052026601,-22.3574534257396,
0.));
#227190=CARTESIAN_POINT('Ctrl Pts',(-4.16988413199458,-22.36724564276,0.));
#227191=CARTESIAN_POINT('Ctrl Pts',(-4.17317742436146,-22.3772263228617,
0.));
#227192=CARTESIAN_POINT('Ctrl Pts',(-4.17657052752826,-22.3873919231334,
0.));
#227193=CARTESIAN_POINT('Ctrl Pts',(-4.18006356544883,-22.3977390078075,
0.));
#227194=CARTESIAN_POINT('Ctrl Pts',(-4.18365665600851,-22.4082642454453,
0.));
#227195=CARTESIAN_POINT('Ctrl Pts',(-4.18734991117722,-22.4189644056115,
0.));
#227196=CARTESIAN_POINT('Ctrl Pts',(-4.19114343726943,-22.4298363535421,
0.));
#227197=CARTESIAN_POINT('Ctrl Pts',(-4.19503733518862,-22.4408770448917,
0.));
#227198=CARTESIAN_POINT('Ctrl Pts',(-4.19903170066356,-22.4520835205419,
0.));
#227199=CARTESIAN_POINT('Ctrl Pts',(-4.20312662448172,-22.4634529011433,
0.));
#227200=CARTESIAN_POINT('Ctrl Pts',(-4.20732219265649,-22.4749823839915,
0.));
#227201=CARTESIAN_POINT('Ctrl Pts',(-4.21161848657429,-22.4866692403147,
0.));
#227202=CARTESIAN_POINT('Ctrl Pts',(-4.21601558313909,-22.4985108124229,
0.));
#227203=CARTESIAN_POINT('Ctrl Pts',(-4.22051355490198,-22.5105045108882,
0.));
#227204=CARTESIAN_POINT('Ctrl Pts',(-4.22511247020041,-22.5226478117885,
0.));
#227205=CARTESIAN_POINT('Ctrl Pts',(-4.22981239330732,-22.5349382540587,
0.));
#227206=CARTESIAN_POINT('Ctrl Pts',(-4.23461338456714,-22.5473734368086,
0.));
#227207=CARTESIAN_POINT('Ctrl Pts',(-4.23951550052527,-22.559951016643,
0.));
#227208=CARTESIAN_POINT('Ctrl Pts',(-4.2445187940486,-22.5726687049922,
0.));
#227209=CARTESIAN_POINT('Ctrl Pts',(-4.24962331444186,-22.5855242662479,
0.));
#227210=CARTESIAN_POINT('Ctrl Pts',(-4.25482910755486,-22.5985155158637,
0.));
#227211=CARTESIAN_POINT('Ctrl Pts',(-4.26013621588304,-22.611640318482,
0.));
#227212=CARTESIAN_POINT('Ctrl Pts',(-4.26554467865572,-22.6248965859975,
0.));
#227213=CARTESIAN_POINT('Ctrl Pts',(-4.27105453193,-22.6382822758171,0.));
#227214=CARTESIAN_POINT('Ctrl Pts',(-4.27666580869118,-22.6517953893303,
0.));
#227215=CARTESIAN_POINT('Ctrl Pts',(-4.2823785389406,-22.665433970311,0.));
#227216=CARTESIAN_POINT('Ctrl Pts',(-4.28819274977767,-22.6791961033536,
0.));
#227217=CARTESIAN_POINT('Ctrl Pts',(-4.29410846547062,-22.6930799122545,
0.));
#227218=CARTESIAN_POINT('Ctrl Pts',(-4.30012570754067,-22.707083558756,
0.));
#227219=CARTESIAN_POINT('Ctrl Pts',(-4.30624449484075,-22.7212052413384,
0.));
#227220=CARTESIAN_POINT('Ctrl Pts',(-4.31246484362551,-22.7354431939926,
0.));
#227221=CARTESIAN_POINT('Ctrl Pts',(-4.31878676761231,-22.7497956849852,
0.));
#227222=CARTESIAN_POINT('Ctrl Pts',(-4.32521027803748,-22.764261015648,
0.));
#227223=CARTESIAN_POINT('Ctrl Pts',(-4.33173538373183,-22.7788375194081,
0.));
#227224=CARTESIAN_POINT('Ctrl Pts',(-4.33836209118444,-22.7935235607807,
0.));
#227225=CARTESIAN_POINT('Ctrl Pts',(-4.34509040460066,-22.808317534379,
0.));
#227226=CARTESIAN_POINT('Ctrl Pts',(-4.35192032594802,-22.8232178638873,
0.));
#227227=CARTESIAN_POINT('Ctrl Pts',(-4.3588518550056,-22.838223001118,0.));
#227228=CARTESIAN_POINT('Ctrl Pts',(-4.36588498943011,-22.8533314252419,
0.));
#227229=CARTESIAN_POINT('Ctrl Pts',(-4.37301972480753,-22.8685416419725,
0.));
#227230=CARTESIAN_POINT('Ctrl Pts',(-4.38025605470091,-22.8838521827702,
0.));
#227231=CARTESIAN_POINT('Ctrl Pts',(-4.38759397068393,-22.8992616040108,
0.));
#227232=CARTESIAN_POINT('Ctrl Pts',(-4.39503346238455,-22.9147684862425,
0.));
#227233=CARTESIAN_POINT('Ctrl Pts',(-4.40257451754308,-22.9303714335549,
0.));
#227234=CARTESIAN_POINT('Ctrl Pts',(-4.41021712205549,-22.9460690729093,
0.));
#227235=CARTESIAN_POINT('Ctrl Pts',(-4.41796126001311,-22.9618600534866,
0.));
#227236=CARTESIAN_POINT('Ctrl Pts',(-4.42580691372772,-22.9777430460021,
0.));
#227237=CARTESIAN_POINT('Ctrl Pts',(-4.43375406376906,-22.9937167421009,
0.));
#227238=CARTESIAN_POINT('Ctrl Pts',(-4.44180268901667,-23.0097798538399,
0.));
#227239=CARTESIAN_POINT('Ctrl Pts',(-4.44995276669699,-23.0259311131395,
0.));
#227240=CARTESIAN_POINT('Ctrl Pts',(-4.45820427241677,-23.0421692712466,
0.));
#227241=CARTESIAN_POINT('Ctrl Pts',(-4.46655718018206,-23.0584930981723,
0.));
#227242=CARTESIAN_POINT('Ctrl Pts',(-4.47501146242822,-23.0749013821867,
0.));
#227243=CARTESIAN_POINT('Ctrl Pts',(-4.48356709006757,-23.0913929293909,
0.));
#227244=CARTESIAN_POINT('Ctrl Pts',(-4.49222403252202,-23.1079665632629,
0.));
#227245=CARTESIAN_POINT('Ctrl Pts',(-4.50098225775179,-23.1246211242117,
0.));
#227246=CARTESIAN_POINT('Ctrl Pts',(-4.50984173227088,-23.1413554691136,
0.));
#227247=CARTESIAN_POINT('Ctrl Pts',(-4.51880242116786,-23.1581684708778,
0.));
#227248=CARTESIAN_POINT('Ctrl Pts',(-4.52786428815049,-23.1750590180923,
0.));
#227249=CARTESIAN_POINT('Ctrl Pts',(-4.53702729557586,-23.1920260146474,
0.));
#227250=CARTESIAN_POINT('Ctrl Pts',(-4.54629140447543,-23.2090683793627,
0.));
#227251=CARTESIAN_POINT('Ctrl Pts',(-4.55565657456957,-23.2261850456055,
0.));
#227252=CARTESIAN_POINT('Ctrl Pts',(-4.56512276427812,-23.2433749609117,
0.));
#227253=CARTESIAN_POINT('Ctrl Pts',(-4.57468993076071,-23.2606370866854,
0.));
#227254=CARTESIAN_POINT('Ctrl Pts',(-4.58435802994675,-23.2779703978868,
0.));
#227255=CARTESIAN_POINT('Ctrl Pts',(-4.5941270165575,-23.295373882719,0.));
#227256=CARTESIAN_POINT('Ctrl Pts',(-4.60399684412176,-23.3128465423119,
0.));
#227257=CARTESIAN_POINT('Ctrl Pts',(-4.61396746497849,-23.3303873903947,
0.));
#227258=CARTESIAN_POINT('Ctrl Pts',(-4.62403883030825,-23.3479954530281,
0.));
#227259=CARTESIAN_POINT('Ctrl Pts',(-4.63421089016555,-23.3656697683496,
0.));
#227260=CARTESIAN_POINT('Ctrl Pts',(-4.64448359349936,-23.383409386307,
0.));
#227261=CARTESIAN_POINT('Ctrl Pts',(-4.65485688816923,-23.4012133683957,
0.));
#227262=CARTESIAN_POINT('Ctrl Pts',(-4.66533072094664,-23.4190807873798,
0.));
#227263=CARTESIAN_POINT('Ctrl Pts',(-4.67590503753051,-23.4370107270444,
0.));
#227264=CARTESIAN_POINT('Ctrl Pts',(-4.68657978258298,-23.4550022819852,
0.));
#227265=CARTESIAN_POINT('Ctrl Pts',(-4.69735489975024,-23.4730545573849,
0.));
#227266=CARTESIAN_POINT('Ctrl Pts',(-4.70823033167821,-23.491166668789,
0.));
#227267=CARTESIAN_POINT('Ctrl Pts',(-4.71920602001905,-23.5093377418784,
0.));
#227268=CARTESIAN_POINT('Ctrl Pts',(-4.73028190543032,-23.5275669122378,
0.));
#227269=CARTESIAN_POINT('Ctrl Pts',(-4.74145792760699,-23.5458533251715,
0.));
#227270=CARTESIAN_POINT('Ctrl Pts',(-4.75273402530616,-23.564196135517,
0.));
#227271=CARTESIAN_POINT('Ctrl Pts',(-4.76411013636252,-23.5825945074535,
0.));
#227272=CARTESIAN_POINT('Ctrl Pts',(-4.77558619769876,-23.6010476143099,
0.));
#227273=CARTESIAN_POINT('Ctrl Pts',(-4.78716214532105,-23.6195546383625,
0.));
#227274=CARTESIAN_POINT('Ctrl Pts',(-4.79883791433231,-23.6381147706581,
0.));
#227275=CARTESIAN_POINT('Ctrl Pts',(-4.81061343896443,-23.6567272108631,
0.));
#227276=CARTESIAN_POINT('Ctrl Pts',(-4.82248865259571,-23.6753911671023,
0.));
#227277=CARTESIAN_POINT('Ctrl Pts',(-4.83446348776268,-23.6941058557971,
0.));
#227278=CARTESIAN_POINT('Ctrl Pts',(-4.84653787616424,-23.7128705015014,
0.));
#227279=CARTESIAN_POINT('Ctrl Pts',(-4.85871174865492,-23.7316843367308,
0.));
#227280=CARTESIAN_POINT('Ctrl Pts',(-4.87098503527144,-23.7505466018239,
0.));
#227281=CARTESIAN_POINT('Ctrl Pts',(-4.88335766525566,-23.7694565448044,
0.));
#227282=CARTESIAN_POINT('Ctrl Pts',(-4.89582956706772,-23.7884134212381,
0.));
#227283=CARTESIAN_POINT('Ctrl Pts',(-4.90840066839348,-23.8074164940897,
0.));
#227284=CARTESIAN_POINT('Ctrl Pts',(-4.92107089613977,-23.8264650335721,
0.));
#227285=CARTESIAN_POINT('Ctrl Pts',(-4.93384017643442,-23.8455583170062,
0.));
#227286=CARTESIAN_POINT('Ctrl Pts',(-4.94670843465869,-23.8646956287172,
0.));
#227287=CARTESIAN_POINT('Ctrl Pts',(-4.95967559546566,-23.883876259922,
0.));
#227288=CARTESIAN_POINT('Ctrl Pts',(-4.9727415827923,-23.9030995086164,
0.));
#227289=CARTESIAN_POINT('Ctrl Pts',(-4.98590631986534,-23.9223646794591,
0.));
#227290=CARTESIAN_POINT('Ctrl Pts',(-4.9991697291931,-23.9416710836529,
0.));
#227291=CARTESIAN_POINT('Ctrl Pts',(-5.01253173257459,-23.9610180388271,
0.));
#227292=CARTESIAN_POINT('Ctrl Pts',(-5.02599225112462,-23.9804048689228,
0.));
#227293=CARTESIAN_POINT('Ctrl Pts',(-5.03955120528528,-23.9998309040747,
0.));
#227294=CARTESIAN_POINT('Ctrl Pts',(-5.05320851483069,-24.0192954804896,
0.));
#227295=CARTESIAN_POINT('Ctrl Pts',(-5.0669640988664,-24.0387979403268,
0.));
#227296=CARTESIAN_POINT('Ctrl Pts',(-5.08081787581271,-24.0583376315636,
0.));
#227297=CARTESIAN_POINT('Ctrl Pts',(-5.09476976342618,-24.0779139079264,
0.));
#227298=CARTESIAN_POINT('Ctrl Pts',(-5.10881967883126,-24.0975261288444,
0.));
#227299=CARTESIAN_POINT('Ctrl Pts',(-5.12296753853858,-24.117173659394,
0.));
#227300=CARTESIAN_POINT('Ctrl Pts',(-5.13721325845746,-24.1368558702443,
0.));
#227301=CARTESIAN_POINT('Ctrl Pts',(-5.1515567539008,-24.1565721375971,
0.));
#227302=CARTESIAN_POINT('Ctrl Pts',(-5.16599793957987,-24.1763218431344,
0.));
#227303=CARTESIAN_POINT('Ctrl Pts',(-5.180536729614,-24.1961043738756,0.));
#227304=CARTESIAN_POINT('Ctrl Pts',(-5.19517303753648,-24.2159191220171,
0.));
#227305=CARTESIAN_POINT('Ctrl Pts',(-5.20990677629177,-24.2357654847766,
0.));
#227306=CARTESIAN_POINT('Ctrl Pts',(-5.22473785822443,-24.2556428642294,
0.));
#227307=CARTESIAN_POINT('Ctrl Pts',(-5.2396661950629,-24.2755506671525,
0.));
#227308=CARTESIAN_POINT('Ctrl Pts',(-5.25469169788857,-24.2954883048447,
0.));
#227309=CARTESIAN_POINT('Ctrl Pts',(-5.269814277188,-24.3154551932221,0.));
#227310=CARTESIAN_POINT('Ctrl Pts',(-5.28503384290649,-24.3354507529414,
0.));
#227311=CARTESIAN_POINT('Ctrl Pts',(-5.30035030449064,-24.3554744095075,
0.));
#227312=CARTESIAN_POINT('Ctrl Pts',(-5.31576357092527,-24.3755255933917,
0.));
#227313=CARTESIAN_POINT('Ctrl Pts',(-5.33127355076035,-24.3956037401293,
0.));
#227314=CARTESIAN_POINT('Ctrl Pts',(-5.34688015213538,-24.4157082904614,
0.));
#227315=CARTESIAN_POINT('Ctrl Pts',(-5.36258328273628,-24.435838689915,
0.));
#227316=CARTESIAN_POINT('Ctrl Pts',(-5.37838284973696,-24.4559943883157,
0.));
#227317=CARTESIAN_POINT('Ctrl Pts',(-5.39427875973825,-24.4761748393321,
0.));
#227318=CARTESIAN_POINT('Ctrl Pts',(-5.41027091869242,-24.496379499983,
0.));
#227319=CARTESIAN_POINT('Ctrl Pts',(-5.4263592318342,-24.5166078302108,
0.));
#227320=CARTESIAN_POINT('Ctrl Pts',(-5.44254360356881,-24.5368592922863,
0.));
#227321=CARTESIAN_POINT('Ctrl Pts',(-5.45882393762262,-24.5571333514842,
0.));
#227322=CARTESIAN_POINT('Ctrl Pts',(-5.4752001372442,-24.5774294770329,
0.));
#227323=CARTESIAN_POINT('Ctrl Pts',(-5.49167210537248,-24.5977471429364,
0.));
#227324=CARTESIAN_POINT('Ctrl Pts',(-5.50823974481963,-24.6180858289179,
0.));
#227325=CARTESIAN_POINT('Ctrl Pts',(-5.52490295840993,-24.6384450211467,
0.));
#227326=CARTESIAN_POINT('Ctrl Pts',(-5.54166164919584,-24.6588242134738,
0.));
#227327=CARTESIAN_POINT('Ctrl Pts',(-5.55851572025377,-24.6792229061794,
0.));
#227328=CARTESIAN_POINT('Ctrl Pts',(-5.57546507427756,-24.6996406035517,
0.));
#227329=CARTESIAN_POINT('Ctrl Pts',(-5.59250961323988,-24.7200768119088,
0.));
#227330=CARTESIAN_POINT('Ctrl Pts',(-5.60964923798492,-24.7405310372739,
0.));
#227331=CARTESIAN_POINT('Ctrl Pts',(-5.62688384790924,-24.7610027835697,
0.));
#227332=CARTESIAN_POINT('Ctrl Pts',(-5.64421334042262,-24.781491549672,
0.));
#227333=CARTESIAN_POINT('Ctrl Pts',(-5.66163761114922,-24.8019968304605,
0.));
#227334=CARTESIAN_POINT('Ctrl Pts',(-5.67915655496543,-24.8225181223845,
0.));
#227335=CARTESIAN_POINT('Ctrl Pts',(-5.69677006679445,-24.8430549277621,
0.));
#227336=CARTESIAN_POINT('Ctrl Pts',(-5.71447804252028,-24.8636067597669,
0.));
#227337=CARTESIAN_POINT('Ctrl Pts',(-5.73228037976928,-24.884173146722,
0.));
#227338=CARTESIAN_POINT('Ctrl Pts',(-5.75017697890805,-24.904753637648,
0.));
#227339=CARTESIAN_POINT('Ctrl Pts',(-5.76816774342221,-24.9253478043656,
0.));
#227340=CARTESIAN_POINT('Ctrl Pts',(-5.78625257775682,-24.945955229334,
0.));
#227341=CARTESIAN_POINT('Ctrl Pts',(-5.80443138549727,-24.9665754954496,
0.));
#227342=CARTESIAN_POINT('Ctrl Pts',(-5.822704067442,-24.9872081752734,0.));
#227343=CARTESIAN_POINT('Ctrl Pts',(-5.84107051963072,-25.0078528200564,
0.));
#227344=CARTESIAN_POINT('Ctrl Pts',(-5.85953063156827,-25.0285089498899,
0.));
#227345=CARTESIAN_POINT('Ctrl Pts',(-5.87808428385367,-25.049176040591,
0.));
#227346=CARTESIAN_POINT('Ctrl Pts',(-5.89673135155515,-25.0698535426514,
0.));
#227347=CARTESIAN_POINT('Ctrl Pts',(-5.91547170844448,-25.0905409050773,
0.));
#227348=CARTESIAN_POINT('Ctrl Pts',(-5.93430523086836,-25.1112375971106,
0.));
#227349=CARTESIAN_POINT('Ctrl Pts',(-5.95323180187379,-25.1319431317237,
0.));
#227350=CARTESIAN_POINT('Ctrl Pts',(-5.97225131495618,-25.1526570863092,
0.));
#227351=CARTESIAN_POINT('Ctrl Pts',(-5.99136367859755,-25.1733791296259,
0.));
#227352=CARTESIAN_POINT('Ctrl Pts',(-6.01056881804614,-25.1941090269819,
0.));
#227353=CARTESIAN_POINT('Ctrl Pts',(-6.02986667389998,-25.21484662016,0.));
#227354=CARTESIAN_POINT('Ctrl Pts',(-6.04925720151219,-25.2355918139032,
0.));
#227355=CARTESIAN_POINT('Ctrl Pts',(-6.06484373634547,-25.2521940105705,
0.));
#227356=CARTESIAN_POINT('Ctrl Pts',(-6.07657531787491,-25.2646490489922,
0.));
#227357=CARTESIAN_POINT('Ctrl Pts',(-6.08441489609794,-25.2729539149517,
0.));
#227358=CARTESIAN_POINT('Ctrl Pts',(-6.088339316177,-25.2771067246846,0.));
#227359=CARTESIAN_POINT('',(-6.088339316177,-25.2771067246846,12.));
#227360=CARTESIAN_POINT('Ctrl Pts',(-6.088339316177,-25.2771067246846,12.));
#227361=CARTESIAN_POINT('Ctrl Pts',(-6.08441489609794,-25.2729539149517,
12.));
#227362=CARTESIAN_POINT('Ctrl Pts',(-6.07657531787491,-25.2646490489922,
12.));
#227363=CARTESIAN_POINT('Ctrl Pts',(-6.06484373634547,-25.2521940105705,
12.));
#227364=CARTESIAN_POINT('Ctrl Pts',(-6.04925720151219,-25.2355918139032,
12.));
#227365=CARTESIAN_POINT('Ctrl Pts',(-6.02986667389998,-25.21484662016,12.));
#227366=CARTESIAN_POINT('Ctrl Pts',(-6.01056881804614,-25.1941090269819,
12.));
#227367=CARTESIAN_POINT('Ctrl Pts',(-5.99136367859755,-25.1733791296259,
12.));
#227368=CARTESIAN_POINT('Ctrl Pts',(-5.97225131495618,-25.1526570863092,
12.));
#227369=CARTESIAN_POINT('Ctrl Pts',(-5.95323180187379,-25.1319431317237,
12.));
#227370=CARTESIAN_POINT('Ctrl Pts',(-5.93430523086836,-25.1112375971106,
12.));
#227371=CARTESIAN_POINT('Ctrl Pts',(-5.91547170844448,-25.0905409050773,
12.));
#227372=CARTESIAN_POINT('Ctrl Pts',(-5.89673135155515,-25.0698535426514,
12.));
#227373=CARTESIAN_POINT('Ctrl Pts',(-5.87808428385367,-25.049176040591,
12.));
#227374=CARTESIAN_POINT('Ctrl Pts',(-5.85953063156827,-25.0285089498899,
12.));
#227375=CARTESIAN_POINT('Ctrl Pts',(-5.84107051963072,-25.0078528200564,
12.));
#227376=CARTESIAN_POINT('Ctrl Pts',(-5.822704067442,-24.9872081752734,12.));
#227377=CARTESIAN_POINT('Ctrl Pts',(-5.80443138549727,-24.9665754954496,
12.));
#227378=CARTESIAN_POINT('Ctrl Pts',(-5.78625257775682,-24.945955229334,
12.));
#227379=CARTESIAN_POINT('Ctrl Pts',(-5.76816774342221,-24.9253478043656,
12.));
#227380=CARTESIAN_POINT('Ctrl Pts',(-5.75017697890805,-24.904753637648,
12.));
#227381=CARTESIAN_POINT('Ctrl Pts',(-5.73228037976928,-24.884173146722,
12.));
#227382=CARTESIAN_POINT('Ctrl Pts',(-5.71447804252028,-24.8636067597669,
12.));
#227383=CARTESIAN_POINT('Ctrl Pts',(-5.69677006679445,-24.8430549277621,
12.));
#227384=CARTESIAN_POINT('Ctrl Pts',(-5.67915655496543,-24.8225181223845,
12.));
#227385=CARTESIAN_POINT('Ctrl Pts',(-5.66163761114922,-24.8019968304605,
12.));
#227386=CARTESIAN_POINT('Ctrl Pts',(-5.64421334042262,-24.781491549672,
12.));
#227387=CARTESIAN_POINT('Ctrl Pts',(-5.62688384790924,-24.7610027835697,
12.));
#227388=CARTESIAN_POINT('Ctrl Pts',(-5.60964923798492,-24.7405310372739,
12.));
#227389=CARTESIAN_POINT('Ctrl Pts',(-5.59250961323988,-24.7200768119088,
12.));
#227390=CARTESIAN_POINT('Ctrl Pts',(-5.57546507427756,-24.6996406035517,
12.));
#227391=CARTESIAN_POINT('Ctrl Pts',(-5.55851572025377,-24.6792229061794,
12.));
#227392=CARTESIAN_POINT('Ctrl Pts',(-5.54166164919584,-24.6588242134738,
12.));
#227393=CARTESIAN_POINT('Ctrl Pts',(-5.52490295840993,-24.6384450211467,
12.));
#227394=CARTESIAN_POINT('Ctrl Pts',(-5.50823974481963,-24.6180858289179,
12.));
#227395=CARTESIAN_POINT('Ctrl Pts',(-5.49167210537248,-24.5977471429364,
12.));
#227396=CARTESIAN_POINT('Ctrl Pts',(-5.4752001372442,-24.5774294770329,
12.));
#227397=CARTESIAN_POINT('Ctrl Pts',(-5.45882393762262,-24.5571333514842,
12.));
#227398=CARTESIAN_POINT('Ctrl Pts',(-5.44254360356881,-24.5368592922863,
12.));
#227399=CARTESIAN_POINT('Ctrl Pts',(-5.4263592318342,-24.5166078302108,
12.));
#227400=CARTESIAN_POINT('Ctrl Pts',(-5.41027091869242,-24.496379499983,
12.));
#227401=CARTESIAN_POINT('Ctrl Pts',(-5.39427875973825,-24.4761748393321,
12.));
#227402=CARTESIAN_POINT('Ctrl Pts',(-5.37838284973696,-24.4559943883157,
12.));
#227403=CARTESIAN_POINT('Ctrl Pts',(-5.36258328273628,-24.435838689915,
12.));
#227404=CARTESIAN_POINT('Ctrl Pts',(-5.34688015213538,-24.4157082904614,
12.));
#227405=CARTESIAN_POINT('Ctrl Pts',(-5.33127355076035,-24.3956037401293,
12.));
#227406=CARTESIAN_POINT('Ctrl Pts',(-5.31576357092527,-24.3755255933917,
12.));
#227407=CARTESIAN_POINT('Ctrl Pts',(-5.30035030449064,-24.3554744095075,
12.));
#227408=CARTESIAN_POINT('Ctrl Pts',(-5.28503384290649,-24.3354507529414,
12.));
#227409=CARTESIAN_POINT('Ctrl Pts',(-5.269814277188,-24.3154551932221,12.));
#227410=CARTESIAN_POINT('Ctrl Pts',(-5.25469169788857,-24.2954883048447,
12.));
#227411=CARTESIAN_POINT('Ctrl Pts',(-5.2396661950629,-24.2755506671525,
12.));
#227412=CARTESIAN_POINT('Ctrl Pts',(-5.22473785822443,-24.2556428642294,
12.));
#227413=CARTESIAN_POINT('Ctrl Pts',(-5.20990677629177,-24.2357654847766,
12.));
#227414=CARTESIAN_POINT('Ctrl Pts',(-5.19517303753648,-24.2159191220171,
12.));
#227415=CARTESIAN_POINT('Ctrl Pts',(-5.180536729614,-24.1961043738756,12.));
#227416=CARTESIAN_POINT('Ctrl Pts',(-5.16599793957987,-24.1763218431344,
12.));
#227417=CARTESIAN_POINT('Ctrl Pts',(-5.1515567539008,-24.1565721375971,
12.));
#227418=CARTESIAN_POINT('Ctrl Pts',(-5.13721325845746,-24.1368558702443,
12.));
#227419=CARTESIAN_POINT('Ctrl Pts',(-5.12296753853858,-24.117173659394,
12.));
#227420=CARTESIAN_POINT('Ctrl Pts',(-5.10881967883126,-24.0975261288444,
12.));
#227421=CARTESIAN_POINT('Ctrl Pts',(-5.09476976342618,-24.0779139079264,
12.));
#227422=CARTESIAN_POINT('Ctrl Pts',(-5.08081787581271,-24.0583376315636,
12.));
#227423=CARTESIAN_POINT('Ctrl Pts',(-5.0669640988664,-24.0387979403268,
12.));
#227424=CARTESIAN_POINT('Ctrl Pts',(-5.05320851483069,-24.0192954804896,
12.));
#227425=CARTESIAN_POINT('Ctrl Pts',(-5.03955120528528,-23.9998309040747,
12.));
#227426=CARTESIAN_POINT('Ctrl Pts',(-5.02599225112462,-23.9804048689228,
12.));
#227427=CARTESIAN_POINT('Ctrl Pts',(-5.01253173257459,-23.9610180388271,
12.));
#227428=CARTESIAN_POINT('Ctrl Pts',(-4.9991697291931,-23.9416710836529,
12.));
#227429=CARTESIAN_POINT('Ctrl Pts',(-4.98590631986534,-23.9223646794591,
12.));
#227430=CARTESIAN_POINT('Ctrl Pts',(-4.9727415827923,-23.9030995086164,
12.));
#227431=CARTESIAN_POINT('Ctrl Pts',(-4.95967559546566,-23.883876259922,
12.));
#227432=CARTESIAN_POINT('Ctrl Pts',(-4.94670843465869,-23.8646956287172,
12.));
#227433=CARTESIAN_POINT('Ctrl Pts',(-4.93384017643442,-23.8455583170062,
12.));
#227434=CARTESIAN_POINT('Ctrl Pts',(-4.92107089613977,-23.8264650335721,
12.));
#227435=CARTESIAN_POINT('Ctrl Pts',(-4.90840066839348,-23.8074164940897,
12.));
#227436=CARTESIAN_POINT('Ctrl Pts',(-4.89582956706772,-23.7884134212381,
12.));
#227437=CARTESIAN_POINT('Ctrl Pts',(-4.88335766525566,-23.7694565448044,
12.));
#227438=CARTESIAN_POINT('Ctrl Pts',(-4.87098503527144,-23.7505466018239,
12.));
#227439=CARTESIAN_POINT('Ctrl Pts',(-4.85871174865492,-23.7316843367308,
12.));
#227440=CARTESIAN_POINT('Ctrl Pts',(-4.84653787616424,-23.7128705015014,
12.));
#227441=CARTESIAN_POINT('Ctrl Pts',(-4.83446348776268,-23.6941058557971,
12.));
#227442=CARTESIAN_POINT('Ctrl Pts',(-4.82248865259571,-23.6753911671023,
12.));
#227443=CARTESIAN_POINT('Ctrl Pts',(-4.81061343896443,-23.6567272108631,
12.));
#227444=CARTESIAN_POINT('Ctrl Pts',(-4.79883791433231,-23.6381147706581,
12.));
#227445=CARTESIAN_POINT('Ctrl Pts',(-4.78716214532105,-23.6195546383625,
12.));
#227446=CARTESIAN_POINT('Ctrl Pts',(-4.77558619769876,-23.6010476143099,
12.));
#227447=CARTESIAN_POINT('Ctrl Pts',(-4.76411013636252,-23.5825945074535,
12.));
#227448=CARTESIAN_POINT('Ctrl Pts',(-4.75273402530616,-23.564196135517,
12.));
#227449=CARTESIAN_POINT('Ctrl Pts',(-4.74145792760699,-23.5458533251715,
12.));
#227450=CARTESIAN_POINT('Ctrl Pts',(-4.73028190543032,-23.5275669122378,
12.));
#227451=CARTESIAN_POINT('Ctrl Pts',(-4.71920602001905,-23.5093377418784,
12.));
#227452=CARTESIAN_POINT('Ctrl Pts',(-4.70823033167821,-23.491166668789,
12.));
#227453=CARTESIAN_POINT('Ctrl Pts',(-4.69735489975024,-23.4730545573849,
12.));
#227454=CARTESIAN_POINT('Ctrl Pts',(-4.68657978258298,-23.4550022819852,
12.));
#227455=CARTESIAN_POINT('Ctrl Pts',(-4.67590503753051,-23.4370107270444,
12.));
#227456=CARTESIAN_POINT('Ctrl Pts',(-4.66533072094664,-23.4190807873798,
12.));
#227457=CARTESIAN_POINT('Ctrl Pts',(-4.65485688816923,-23.4012133683957,
12.));
#227458=CARTESIAN_POINT('Ctrl Pts',(-4.64448359349936,-23.383409386307,
12.));
#227459=CARTESIAN_POINT('Ctrl Pts',(-4.63421089016555,-23.3656697683496,
12.));
#227460=CARTESIAN_POINT('Ctrl Pts',(-4.62403883030825,-23.3479954530281,
12.));
#227461=CARTESIAN_POINT('Ctrl Pts',(-4.61396746497849,-23.3303873903947,
12.));
#227462=CARTESIAN_POINT('Ctrl Pts',(-4.60399684412176,-23.3128465423119,
12.));
#227463=CARTESIAN_POINT('Ctrl Pts',(-4.5941270165575,-23.295373882719,12.));
#227464=CARTESIAN_POINT('Ctrl Pts',(-4.58435802994675,-23.2779703978868,
12.));
#227465=CARTESIAN_POINT('Ctrl Pts',(-4.57468993076071,-23.2606370866854,
12.));
#227466=CARTESIAN_POINT('Ctrl Pts',(-4.56512276427812,-23.2433749609117,
12.));
#227467=CARTESIAN_POINT('Ctrl Pts',(-4.55565657456957,-23.2261850456055,
12.));
#227468=CARTESIAN_POINT('Ctrl Pts',(-4.54629140447543,-23.2090683793627,
12.));
#227469=CARTESIAN_POINT('Ctrl Pts',(-4.53702729557586,-23.1920260146474,
12.));
#227470=CARTESIAN_POINT('Ctrl Pts',(-4.52786428815049,-23.1750590180923,
12.));
#227471=CARTESIAN_POINT('Ctrl Pts',(-4.51880242116786,-23.1581684708778,
12.));
#227472=CARTESIAN_POINT('Ctrl Pts',(-4.50984173227088,-23.1413554691136,
12.));
#227473=CARTESIAN_POINT('Ctrl Pts',(-4.50098225775179,-23.1246211242117,
12.));
#227474=CARTESIAN_POINT('Ctrl Pts',(-4.49222403252202,-23.1079665632629,
12.));
#227475=CARTESIAN_POINT('Ctrl Pts',(-4.48356709006757,-23.0913929293909,
12.));
#227476=CARTESIAN_POINT('Ctrl Pts',(-4.47501146242822,-23.0749013821867,
12.));
#227477=CARTESIAN_POINT('Ctrl Pts',(-4.46655718018206,-23.0584930981723,
12.));
#227478=CARTESIAN_POINT('Ctrl Pts',(-4.45820427241677,-23.0421692712466,
12.));
#227479=CARTESIAN_POINT('Ctrl Pts',(-4.44995276669699,-23.0259311131395,
12.));
#227480=CARTESIAN_POINT('Ctrl Pts',(-4.44180268901667,-23.0097798538399,
12.));
#227481=CARTESIAN_POINT('Ctrl Pts',(-4.43375406376906,-22.9937167421009,
12.));
#227482=CARTESIAN_POINT('Ctrl Pts',(-4.42580691372772,-22.9777430460021,
12.));
#227483=CARTESIAN_POINT('Ctrl Pts',(-4.41796126001311,-22.9618600534866,
12.));
#227484=CARTESIAN_POINT('Ctrl Pts',(-4.41021712205549,-22.9460690729093,
12.));
#227485=CARTESIAN_POINT('Ctrl Pts',(-4.40257451754308,-22.9303714335549,
12.));
#227486=CARTESIAN_POINT('Ctrl Pts',(-4.39503346238455,-22.9147684862425,
12.));
#227487=CARTESIAN_POINT('Ctrl Pts',(-4.38759397068393,-22.8992616040108,
12.));
#227488=CARTESIAN_POINT('Ctrl Pts',(-4.38025605470091,-22.8838521827702,
12.));
#227489=CARTESIAN_POINT('Ctrl Pts',(-4.37301972480753,-22.8685416419725,
12.));
#227490=CARTESIAN_POINT('Ctrl Pts',(-4.36588498943011,-22.8533314252419,
12.));
#227491=CARTESIAN_POINT('Ctrl Pts',(-4.3588518550056,-22.838223001118,12.));
#227492=CARTESIAN_POINT('Ctrl Pts',(-4.35192032594802,-22.8232178638873,
12.));
#227493=CARTESIAN_POINT('Ctrl Pts',(-4.34509040460066,-22.808317534379,
12.));
#227494=CARTESIAN_POINT('Ctrl Pts',(-4.33836209118444,-22.7935235607807,
12.));
#227495=CARTESIAN_POINT('Ctrl Pts',(-4.33173538373183,-22.7788375194081,
12.));
#227496=CARTESIAN_POINT('Ctrl Pts',(-4.32521027803748,-22.764261015648,
12.));
#227497=CARTESIAN_POINT('Ctrl Pts',(-4.31878676761231,-22.7497956849852,
12.));
#227498=CARTESIAN_POINT('Ctrl Pts',(-4.31246484362551,-22.7354431939926,
12.));
#227499=CARTESIAN_POINT('Ctrl Pts',(-4.30624449484075,-22.7212052413384,
12.));
#227500=CARTESIAN_POINT('Ctrl Pts',(-4.30012570754067,-22.707083558756,
12.));
#227501=CARTESIAN_POINT('Ctrl Pts',(-4.29410846547062,-22.6930799122545,
12.));
#227502=CARTESIAN_POINT('Ctrl Pts',(-4.28819274977767,-22.6791961033536,
12.));
#227503=CARTESIAN_POINT('Ctrl Pts',(-4.2823785389406,-22.665433970311,12.));
#227504=CARTESIAN_POINT('Ctrl Pts',(-4.27666580869118,-22.6517953893303,
12.));
#227505=CARTESIAN_POINT('Ctrl Pts',(-4.27105453193,-22.6382822758171,12.));
#227506=CARTESIAN_POINT('Ctrl Pts',(-4.26554467865572,-22.6248965859975,
12.));
#227507=CARTESIAN_POINT('Ctrl Pts',(-4.26013621588304,-22.611640318482,
12.));
#227508=CARTESIAN_POINT('Ctrl Pts',(-4.25482910755486,-22.5985155158637,
12.));
#227509=CARTESIAN_POINT('Ctrl Pts',(-4.24962331444186,-22.5855242662479,
12.));
#227510=CARTESIAN_POINT('Ctrl Pts',(-4.2445187940486,-22.5726687049922,
12.));
#227511=CARTESIAN_POINT('Ctrl Pts',(-4.23951550052527,-22.559951016643,
12.));
#227512=CARTESIAN_POINT('Ctrl Pts',(-4.23461338456714,-22.5473734368086,
12.));
#227513=CARTESIAN_POINT('Ctrl Pts',(-4.22981239330732,-22.5349382540587,
12.));
#227514=CARTESIAN_POINT('Ctrl Pts',(-4.22511247020041,-22.5226478117885,
12.));
#227515=CARTESIAN_POINT('Ctrl Pts',(-4.22051355490198,-22.5105045108882,
12.));
#227516=CARTESIAN_POINT('Ctrl Pts',(-4.21601558313909,-22.4985108124229,
12.));
#227517=CARTESIAN_POINT('Ctrl Pts',(-4.21161848657429,-22.4866692403147,
12.));
#227518=CARTESIAN_POINT('Ctrl Pts',(-4.20732219265649,-22.4749823839915,
12.));
#227519=CARTESIAN_POINT('Ctrl Pts',(-4.20312662448172,-22.4634529011433,
12.));
#227520=CARTESIAN_POINT('Ctrl Pts',(-4.19903170066356,-22.4520835205419,
12.));
#227521=CARTESIAN_POINT('Ctrl Pts',(-4.19503733518862,-22.4408770448917,
12.));
#227522=CARTESIAN_POINT('Ctrl Pts',(-4.19114343726943,-22.4298363535421,
12.));
#227523=CARTESIAN_POINT('Ctrl Pts',(-4.18734991117722,-22.4189644056115,
12.));
#227524=CARTESIAN_POINT('Ctrl Pts',(-4.18365665600851,-22.4082642454453,
12.));
#227525=CARTESIAN_POINT('Ctrl Pts',(-4.18006356544883,-22.3977390078075,
12.));
#227526=CARTESIAN_POINT('Ctrl Pts',(-4.17657052752826,-22.3873919231334,
12.));
#227527=CARTESIAN_POINT('Ctrl Pts',(-4.17317742436146,-22.3772263228617,
12.));
#227528=CARTESIAN_POINT('Ctrl Pts',(-4.16988413199458,-22.36724564276,12.));
#227529=CARTESIAN_POINT('Ctrl Pts',(-4.16669052026601,-22.3574534257396,
12.));
#227530=CARTESIAN_POINT('Ctrl Pts',(-4.16359645263189,-22.3478533253889,
12.));
#227531=CARTESIAN_POINT('Ctrl Pts',(-4.16060178604165,-22.3384491078602,
12.));
#227532=CARTESIAN_POINT('Ctrl Pts',(-4.15770637047891,-22.3292446628959,
12.));
#227533=CARTESIAN_POINT('Ctrl Pts',(-4.15491004835282,-22.320244018698,
12.));
#227534=CARTESIAN_POINT('Ctrl Pts',(-4.15221265396991,-22.3114513545185,
12.));
#227535=CARTESIAN_POINT('Ctrl Pts',(-4.14961401285523,-22.3028710166933,
12.));
#227536=CARTESIAN_POINT('Ctrl Pts',(-4.14711394168557,-22.2945075198467,
12.));
#227537=CARTESIAN_POINT('Ctrl Pts',(-4.14471224859296,-22.2863655389166,
12.));
#227538=CARTESIAN_POINT('Ctrl Pts',(-4.14240873321985,-22.2784499072027,
12.));
#227539=CARTESIAN_POINT('Ctrl Pts',(-4.14020318715992,-22.2707656042457,
12.));
#227540=CARTESIAN_POINT('Ctrl Pts',(-4.13809539255423,-22.2633177913972,
12.));
#227541=CARTESIAN_POINT('Ctrl Pts',(-4.13608511977226,-22.2561118708421,
12.));
#227542=CARTESIAN_POINT('Ctrl Pts',(-4.13417212558811,-22.249153531779,
12.));
#227543=CARTESIAN_POINT('Ctrl Pts',(-4.13235615060161,-22.2424488153523,
12.));
#227544=CARTESIAN_POINT('Ctrl Pts',(-4.13063692157499,-22.2360040565533,
12.));
#227545=CARTESIAN_POINT('Ctrl Pts',(-4.1290141546338,-22.2298258043947,
12.));
#227546=CARTESIAN_POINT('Ctrl Pts',(-4.12748755830105,-22.2239207458781,
12.));
#227547=CARTESIAN_POINT('Ctrl Pts',(-4.12605683613308,-22.2182956401341,
12.));
#227548=CARTESIAN_POINT('Ctrl Pts',(-4.12472167516608,-22.2129576146671,
12.));
#227549=CARTESIAN_POINT('Ctrl Pts',(-4.12348173702024,-22.2079143941719,
12.));
#227550=CARTESIAN_POINT('Ctrl Pts',(-4.12233664408228,-22.2031746532106,
12.));
#227551=CARTESIAN_POINT('Ctrl Pts',(-4.12128598183523,-22.1987479618246,
12.));
#227552=CARTESIAN_POINT('Ctrl Pts',(-4.12032932637737,-22.1946440958098,
12.));
#227553=CARTESIAN_POINT('Ctrl Pts',(-4.11946626228637,-22.1908725908525,
12.));
#227554=CARTESIAN_POINT('Ctrl Pts',(-4.11869641271774,-22.1874419861496,
12.));
#227555=CARTESIAN_POINT('Ctrl Pts',(-4.11801938107481,-22.1843613164855,
12.));
#227556=CARTESIAN_POINT('Ctrl Pts',(-4.11743469691757,-22.1816414985788,
12.));
#227557=CARTESIAN_POINT('Ctrl Pts',(-4.11694173195005,-22.179297473024,
12.));
#227558=CARTESIAN_POINT('Ctrl Pts',(-4.11653973150519,-22.177347426894,
12.));
#227559=CARTESIAN_POINT('Ctrl Pts',(-4.11622797217069,-22.1758088296598,
12.));
#227560=CARTESIAN_POINT('Ctrl Pts',(-4.11600589882846,-22.1746949858775,
12.));
#227561=CARTESIAN_POINT('Ctrl Pts',(-4.11589976826167,-22.1741488021234,
12.));
#227562=CARTESIAN_POINT('Ctrl Pts',(-4.11586035878288,-22.1739341411687,
12.));
#227563=CARTESIAN_POINT('Ctrl Pts',(-4.11585194677443,-22.173877682324,
12.));
#227564=CARTESIAN_POINT('Ctrl Pts',(-4.11585220600463,-22.1738711152697,
12.));
#227565=CARTESIAN_POINT('',(-6.088339316177,-25.2771067246846,0.));
#227566=CARTESIAN_POINT('Origin',(-9.26120677397565,-19.4030938020118,0.));
#227567=CARTESIAN_POINT('',(-9.71462809124917,-20.353053841303,12.));
#227568=CARTESIAN_POINT('',(-4.63060338698782,-9.70154690100589,12.));
#227569=CARTESIAN_POINT('',(-9.71462809124917,-20.353053841303,0.));
#227570=CARTESIAN_POINT('',(-9.71462809124917,-20.353053841303,0.));
#227571=CARTESIAN_POINT('',(-4.63060338698782,-9.70154690100589,0.));
#227572=CARTESIAN_POINT('Ctrl Pts',(-7.36589684767345,-24.9347862158358,
0.));
#227573=CARTESIAN_POINT('Ctrl Pts',(-7.36589684767345,-24.9347862158358,
12.));
#227574=CARTESIAN_POINT('Ctrl Pts',(-7.36721909028843,-24.9292275670674,
0.));
#227575=CARTESIAN_POINT('Ctrl Pts',(-7.36721909028843,-24.9292275670674,
12.));
#227576=CARTESIAN_POINT('Ctrl Pts',(-7.36985593120091,-24.9181155530543,
0.));
#227577=CARTESIAN_POINT('Ctrl Pts',(-7.36985593120091,-24.9181155530543,
12.));
#227578=CARTESIAN_POINT('Ctrl Pts',(-7.37378825961676,-24.901463382605,
0.));
#227579=CARTESIAN_POINT('Ctrl Pts',(-7.37378825961676,-24.901463382605,
12.));
#227580=CARTESIAN_POINT('Ctrl Pts',(-7.3789854964027,-24.8792921911115,
0.));
#227581=CARTESIAN_POINT('Ctrl Pts',(-7.3789854964027,-24.8792921911115,
12.));
#227582=CARTESIAN_POINT('Ctrl Pts',(-7.38540558903621,-24.8516310625176,
0.));
#227583=CARTESIAN_POINT('Ctrl Pts',(-7.38540558903621,-24.8516310625176,
12.));
#227584=CARTESIAN_POINT('Ctrl Pts',(-7.39174922585809,-24.8240228520893,
0.));
#227585=CARTESIAN_POINT('Ctrl Pts',(-7.39174922585809,-24.8240228520893,
12.));
#227586=CARTESIAN_POINT('Ctrl Pts',(-7.39801641583013,-24.7964676646431,
0.));
#227587=CARTESIAN_POINT('Ctrl Pts',(-7.39801641583013,-24.7964676646431,
12.));
#227588=CARTESIAN_POINT('Ctrl Pts',(-7.40420718661603,-24.7689656668983,
0.));
#227589=CARTESIAN_POINT('Ctrl Pts',(-7.40420718661603,-24.7689656668983,
12.));
#227590=CARTESIAN_POINT('Ctrl Pts',(-7.41032159082382,-24.7415170994784,
0.));
#227591=CARTESIAN_POINT('Ctrl Pts',(-7.41032159082382,-24.7415170994784,
12.));
#227592=CARTESIAN_POINT('Ctrl Pts',(-7.41635971481674,-24.7141222950051,
0.));
#227593=CARTESIAN_POINT('Ctrl Pts',(-7.41635971481674,-24.7141222950051,
12.));
#227594=CARTESIAN_POINT('Ctrl Pts',(-7.42232167766266,-24.6867816727192,
0.));
#227595=CARTESIAN_POINT('Ctrl Pts',(-7.42232167766266,-24.6867816727192,
12.));
#227596=CARTESIAN_POINT('Ctrl Pts',(-7.42820762159126,-24.6594957128756,
0.));
#227597=CARTESIAN_POINT('Ctrl Pts',(-7.42820762159126,-24.6594957128756,
12.));
#227598=CARTESIAN_POINT('Ctrl Pts',(-7.43401770489524,-24.6322649369517,
0.));
#227599=CARTESIAN_POINT('Ctrl Pts',(-7.43401770489524,-24.6322649369517,
12.));
#227600=CARTESIAN_POINT('Ctrl Pts',(-7.43975209375504,-24.6050898852368,
0.));
#227601=CARTESIAN_POINT('Ctrl Pts',(-7.43975209375504,-24.6050898852368,
12.));
#227602=CARTESIAN_POINT('Ctrl Pts',(-7.44541095473135,-24.577971096086,
0.));
#227603=CARTESIAN_POINT('Ctrl Pts',(-7.44541095473135,-24.577971096086,
12.));
#227604=CARTESIAN_POINT('Ctrl Pts',(-7.4509944465116,-24.5509090831559,
0.));
#227605=CARTESIAN_POINT('Ctrl Pts',(-7.4509944465116,-24.5509090831559,
12.));
#227606=CARTESIAN_POINT('Ctrl Pts',(-7.45650271335862,-24.5239043173072,
0.));
#227607=CARTESIAN_POINT('Ctrl Pts',(-7.45650271335862,-24.5239043173072,
12.));
#227608=CARTESIAN_POINT('Ctrl Pts',(-7.46193588961464,-24.4969572391483,
0.));
#227609=CARTESIAN_POINT('Ctrl Pts',(-7.46193588961464,-24.4969572391483,
12.));
#227610=CARTESIAN_POINT('Ctrl Pts',(-7.46729410308787,-24.4700682684524,
0.));
#227611=CARTESIAN_POINT('Ctrl Pts',(-7.46729410308787,-24.4700682684524,
12.));
#227612=CARTESIAN_POINT('Ctrl Pts',(-7.47257747883246,-24.443237814649,
0.));
#227613=CARTESIAN_POINT('Ctrl Pts',(-7.47257747883246,-24.443237814649,
12.));
#227614=CARTESIAN_POINT('Ctrl Pts',(-7.47778614286565,-24.4164662871163,
0.));
#227615=CARTESIAN_POINT('Ctrl Pts',(-7.47778614286565,-24.4164662871163,
12.));
#227616=CARTESIAN_POINT('Ctrl Pts',(-7.48292022569301,-24.3897541049254,
0.));
#227617=CARTESIAN_POINT('Ctrl Pts',(-7.48292022569301,-24.3897541049254,
12.));
#227618=CARTESIAN_POINT('Ctrl Pts',(-7.48797986651909,-24.3631017084524,
0.));
#227619=CARTESIAN_POINT('Ctrl Pts',(-7.48797986651909,-24.3631017084524,
12.));
#227620=CARTESIAN_POINT('Ctrl Pts',(-7.49296521252421,-24.3365095573685,
0.));
#227621=CARTESIAN_POINT('Ctrl Pts',(-7.49296521252421,-24.3365095573685,
12.));
#227622=CARTESIAN_POINT('Ctrl Pts',(-7.49787641695439,-24.3099781253355,
0.));
#227623=CARTESIAN_POINT('Ctrl Pts',(-7.49787641695439,-24.3099781253355,
12.));
#227624=CARTESIAN_POINT('Ctrl Pts',(-7.50271363765152,-24.2835078958973,
0.));
#227625=CARTESIAN_POINT('Ctrl Pts',(-7.50271363765152,-24.2835078958973,
12.));
#227626=CARTESIAN_POINT('Ctrl Pts',(-7.50747703535134,-24.2570993577034,
0.));
#227627=CARTESIAN_POINT('Ctrl Pts',(-7.50747703535134,-24.2570993577034,
12.));
#227628=CARTESIAN_POINT('Ctrl Pts',(-7.51216677222181,-24.2307530003887,
0.));
#227629=CARTESIAN_POINT('Ctrl Pts',(-7.51216677222181,-24.2307530003887,
12.));
#227630=CARTESIAN_POINT('Ctrl Pts',(-7.51678300997949,-24.2044693092349,
0.));
#227631=CARTESIAN_POINT('Ctrl Pts',(-7.51678300997949,-24.2044693092349,
12.));
#227632=CARTESIAN_POINT('Ctrl Pts',(-7.52132590953802,-24.1782487641594,
0.));
#227633=CARTESIAN_POINT('Ctrl Pts',(-7.52132590953802,-24.1782487641594,
12.));
#227634=CARTESIAN_POINT('Ctrl Pts',(-7.52579563201424,-24.1520918425364,
0.));
#227635=CARTESIAN_POINT('Ctrl Pts',(-7.52579563201424,-24.1520918425364,
12.));
#227636=CARTESIAN_POINT('Ctrl Pts',(-7.53019233935502,-24.1259990209207,
0.));
#227637=CARTESIAN_POINT('Ctrl Pts',(-7.53019233935502,-24.1259990209207,
12.));
#227638=CARTESIAN_POINT('Ctrl Pts',(-7.53451619514649,-24.0999707772642,
0.));
#227639=CARTESIAN_POINT('Ctrl Pts',(-7.53451619514649,-24.0999707772642,
12.));
#227640=CARTESIAN_POINT('Ctrl Pts',(-7.53876736531014,-24.0740075927985,
0.));
#227641=CARTESIAN_POINT('Ctrl Pts',(-7.53876736531014,-24.0740075927985,
12.));
#227642=CARTESIAN_POINT('Ctrl Pts',(-7.54294601896145,-24.0481099543353,
0.));
#227643=CARTESIAN_POINT('Ctrl Pts',(-7.54294601896145,-24.0481099543353,
12.));
#227644=CARTESIAN_POINT('Ctrl Pts',(-7.5470523288591,-24.022278355453,0.));
#227645=CARTESIAN_POINT('Ctrl Pts',(-7.5470523288591,-24.022278355453,12.));
#227646=CARTESIAN_POINT('Ctrl Pts',(-7.55108647097441,-23.9965132953185,
0.));
#227647=CARTESIAN_POINT('Ctrl Pts',(-7.55108647097441,-23.9965132953185,
12.));
#227648=CARTESIAN_POINT('Ctrl Pts',(-7.55504862424812,-23.9708152779884,
0.));
#227649=CARTESIAN_POINT('Ctrl Pts',(-7.55504862424812,-23.9708152779884,
12.));
#227650=CARTESIAN_POINT('Ctrl Pts',(-7.55893897027683,-23.9451848115,0.));
#227651=CARTESIAN_POINT('Ctrl Pts',(-7.55893897027683,-23.9451848115,12.));
#227652=CARTESIAN_POINT('Ctrl Pts',(-7.56275769304773,-23.9196224070759,
0.));
#227653=CARTESIAN_POINT('Ctrl Pts',(-7.56275769304773,-23.9196224070759,
12.));
#227654=CARTESIAN_POINT('Ctrl Pts',(-7.56650497863792,-23.8941285782003,
0.));
#227655=CARTESIAN_POINT('Ctrl Pts',(-7.56650497863792,-23.8941285782003,
12.));
#227656=CARTESIAN_POINT('Ctrl Pts',(-7.57018101500711,-23.8687038399597,
0.));
#227657=CARTESIAN_POINT('Ctrl Pts',(-7.57018101500711,-23.8687038399597,
12.));
#227658=CARTESIAN_POINT('Ctrl Pts',(-7.57378599219817,-23.8433487096134,
0.));
#227659=CARTESIAN_POINT('Ctrl Pts',(-7.57378599219817,-23.8433487096134,
12.));
#227660=CARTESIAN_POINT('Ctrl Pts',(-7.57732010249066,-23.8180637069977,
0.));
#227661=CARTESIAN_POINT('Ctrl Pts',(-7.57732010249066,-23.8180637069977,
12.));
#227662=CARTESIAN_POINT('Ctrl Pts',(-7.58078354058212,-23.7928493549908,
0.));
#227663=CARTESIAN_POINT('Ctrl Pts',(-7.58078354058212,-23.7928493549908,
12.));
#227664=CARTESIAN_POINT('Ctrl Pts',(-7.58417650376272,-23.7677061799376,
0.));
#227665=CARTESIAN_POINT('Ctrl Pts',(-7.58417650376272,-23.7677061799376,
12.));
#227666=CARTESIAN_POINT('Ctrl Pts',(-7.58749919210832,-23.7426347121006,
0.));
#227667=CARTESIAN_POINT('Ctrl Pts',(-7.58749919210832,-23.7426347121006,
12.));
#227668=CARTESIAN_POINT('Ctrl Pts',(-7.59075180865327,-23.7176354860457,
0.));
#227669=CARTESIAN_POINT('Ctrl Pts',(-7.59075180865327,-23.7176354860457,
12.));
#227670=CARTESIAN_POINT('Ctrl Pts',(-7.59393455934042,-23.6927090405067,
0.));
#227671=CARTESIAN_POINT('Ctrl Pts',(-7.59393455934042,-23.6927090405067,
12.));
#227672=CARTESIAN_POINT('Ctrl Pts',(-7.59704765299572,-23.6678559182876,
0.));
#227673=CARTESIAN_POINT('Ctrl Pts',(-7.59704765299572,-23.6678559182876,
12.));
#227674=CARTESIAN_POINT('Ctrl Pts',(-7.6000913013013,-23.6430766661419,
0.));
#227675=CARTESIAN_POINT('Ctrl Pts',(-7.6000913013013,-23.6430766661419,
12.));
#227676=CARTESIAN_POINT('Ctrl Pts',(-7.60306571877806,-23.6183718346576,
0.));
#227677=CARTESIAN_POINT('Ctrl Pts',(-7.60306571877806,-23.6183718346576,
12.));
#227678=CARTESIAN_POINT('Ctrl Pts',(-7.60597112277094,-23.5937419781244,
0.));
#227679=CARTESIAN_POINT('Ctrl Pts',(-7.60597112277094,-23.5937419781244,
12.));
#227680=CARTESIAN_POINT('Ctrl Pts',(-7.608807733446,-23.5691876544243,0.));
#227681=CARTESIAN_POINT('Ctrl Pts',(-7.608807733446,-23.5691876544243,12.));
#227682=CARTESIAN_POINT('Ctrl Pts',(-7.61157577385372,-23.5447094252028,
0.));
#227683=CARTESIAN_POINT('Ctrl Pts',(-7.61157577385372,-23.5447094252028,
12.));
#227684=CARTESIAN_POINT('Ctrl Pts',(-7.61427546999299,-23.5203078560128,
0.));
#227685=CARTESIAN_POINT('Ctrl Pts',(-7.61427546999299,-23.5203078560128,
12.));
#227686=CARTESIAN_POINT('Ctrl Pts',(-7.61690705088319,-23.4959835164608,
0.));
#227687=CARTESIAN_POINT('Ctrl Pts',(-7.61690705088319,-23.4959835164608,
12.));
#227688=CARTESIAN_POINT('Ctrl Pts',(-7.61947074863978,-23.4717369803438,
0.));
#227689=CARTESIAN_POINT('Ctrl Pts',(-7.61947074863978,-23.4717369803438,
12.));
#227690=CARTESIAN_POINT('Ctrl Pts',(-7.62196679855957,-23.4475688257854,
0.));
#227691=CARTESIAN_POINT('Ctrl Pts',(-7.62196679855957,-23.4475688257854,
12.));
#227692=CARTESIAN_POINT('Ctrl Pts',(-7.62439543920055,-23.4234796353544,
0.));
#227693=CARTESIAN_POINT('Ctrl Pts',(-7.62439543920055,-23.4234796353544,
12.));
#227694=CARTESIAN_POINT('Ctrl Pts',(-7.62675691240335,-23.3994699961122,
0.));
#227695=CARTESIAN_POINT('Ctrl Pts',(-7.62675691240335,-23.3994699961122,
12.));
#227696=CARTESIAN_POINT('Ctrl Pts',(-7.62905146332598,-23.3755404996638,
0.));
#227697=CARTESIAN_POINT('Ctrl Pts',(-7.62905146332598,-23.3755404996638,
12.));
#227698=CARTESIAN_POINT('Ctrl Pts',(-7.63127934048139,-23.3516917421973,
0.));
#227699=CARTESIAN_POINT('Ctrl Pts',(-7.63127934048139,-23.3516917421973,
12.));
#227700=CARTESIAN_POINT('Ctrl Pts',(-7.63344079578163,-23.3279243245241,
0.));
#227701=CARTESIAN_POINT('Ctrl Pts',(-7.63344079578163,-23.3279243245241,
12.));
#227702=CARTESIAN_POINT('Ctrl Pts',(-7.63553608458784,-23.3042388521021,
0.));
#227703=CARTESIAN_POINT('Ctrl Pts',(-7.63553608458784,-23.3042388521021,
12.));
#227704=CARTESIAN_POINT('Ctrl Pts',(-7.63756546576375,-23.2806359350853,
0.));
#227705=CARTESIAN_POINT('Ctrl Pts',(-7.63756546576375,-23.2806359350853,
12.));
#227706=CARTESIAN_POINT('Ctrl Pts',(-7.63952920172837,-23.2571161884487,
0.));
#227707=CARTESIAN_POINT('Ctrl Pts',(-7.63952920172837,-23.2571161884487,
12.));
#227708=CARTESIAN_POINT('Ctrl Pts',(-7.64142755851508,-23.2336802320912,
0.));
#227709=CARTESIAN_POINT('Ctrl Pts',(-7.64142755851508,-23.2336802320912,
12.));
#227710=CARTESIAN_POINT('Ctrl Pts',(-7.64326080583684,-23.2103286909399,
0.));
#227711=CARTESIAN_POINT('Ctrl Pts',(-7.64326080583684,-23.2103286909399,
12.));
#227712=CARTESIAN_POINT('Ctrl Pts',(-7.64502921715483,-23.1870621950452,
0.));
#227713=CARTESIAN_POINT('Ctrl Pts',(-7.64502921715483,-23.1870621950452,
12.));
#227714=CARTESIAN_POINT('Ctrl Pts',(-7.64673306975797,-23.1638813796691,
0.));
#227715=CARTESIAN_POINT('Ctrl Pts',(-7.64673306975797,-23.1638813796691,
12.));
#227716=CARTESIAN_POINT('Ctrl Pts',(-7.64837264482929,-23.1407868853815,
0.));
#227717=CARTESIAN_POINT('Ctrl Pts',(-7.64837264482929,-23.1407868853815,
12.));
#227718=CARTESIAN_POINT('Ctrl Pts',(-7.64994822749845,-23.1177793581674,
0.));
#227719=CARTESIAN_POINT('Ctrl Pts',(-7.64994822749845,-23.1177793581674,
12.));
#227720=CARTESIAN_POINT('Ctrl Pts',(-7.65146010690465,-23.0948594495246,
0.));
#227721=CARTESIAN_POINT('Ctrl Pts',(-7.65146010690465,-23.0948594495246,
12.));
#227722=CARTESIAN_POINT('Ctrl Pts',(-7.65290857626357,-23.072027816555,
0.));
#227723=CARTESIAN_POINT('Ctrl Pts',(-7.65290857626357,-23.072027816555,
12.));
#227724=CARTESIAN_POINT('Ctrl Pts',(-7.65429393293955,-23.049285122053,
0.));
#227725=CARTESIAN_POINT('Ctrl Pts',(-7.65429393293955,-23.049285122053,
12.));
#227726=CARTESIAN_POINT('Ctrl Pts',(-7.65561647852555,-23.0266320345792,
0.));
#227727=CARTESIAN_POINT('Ctrl Pts',(-7.65561647852555,-23.0266320345792,
12.));
#227728=CARTESIAN_POINT('Ctrl Pts',(-7.6568765189133,-23.004069228582,0.));
#227729=CARTESIAN_POINT('Ctrl Pts',(-7.6568765189133,-23.004069228582,12.));
#227730=CARTESIAN_POINT('Ctrl Pts',(-7.65807436436453,-22.9815973845301,
0.));
#227731=CARTESIAN_POINT('Ctrl Pts',(-7.65807436436453,-22.9815973845301,
12.));
#227732=CARTESIAN_POINT('Ctrl Pts',(-7.65921032958912,-22.9592171890332,
0.));
#227733=CARTESIAN_POINT('Ctrl Pts',(-7.65921032958912,-22.9592171890332,
12.));
#227734=CARTESIAN_POINT('Ctrl Pts',(-7.66028473382777,-22.9369293349592,
0.));
#227735=CARTESIAN_POINT('Ctrl Pts',(-7.66028473382777,-22.9369293349592,
12.));
#227736=CARTESIAN_POINT('Ctrl Pts',(-7.661297900941,-22.9147345215418,0.));
#227737=CARTESIAN_POINT('Ctrl Pts',(-7.661297900941,-22.9147345215418,12.));
#227738=CARTESIAN_POINT('Ctrl Pts',(-7.66225015950148,-22.8926334544879,
0.));
#227739=CARTESIAN_POINT('Ctrl Pts',(-7.66225015950148,-22.8926334544879,
12.));
#227740=CARTESIAN_POINT('Ctrl Pts',(-7.66314184287334,-22.870626846128,
0.));
#227741=CARTESIAN_POINT('Ctrl Pts',(-7.66314184287334,-22.870626846128,
12.));
#227742=CARTESIAN_POINT('Ctrl Pts',(-7.66397328929805,-22.8487154155569,
0.));
#227743=CARTESIAN_POINT('Ctrl Pts',(-7.66397328929805,-22.8487154155569,
12.));
#227744=CARTESIAN_POINT('Ctrl Pts',(-7.66474484198553,-22.8268998887678,
0.));
#227745=CARTESIAN_POINT('Ctrl Pts',(-7.66474484198553,-22.8268998887678,
12.));
#227746=CARTESIAN_POINT('Ctrl Pts',(-7.66545684920988,-22.8051809987833,
0.));
#227747=CARTESIAN_POINT('Ctrl Pts',(-7.66545684920988,-22.8051809987833,
12.));
#227748=CARTESIAN_POINT('Ctrl Pts',(-7.66610966441259,-22.7835594857697,
0.));
#227749=CARTESIAN_POINT('Ctrl Pts',(-7.66610966441259,-22.7835594857697,
12.));
#227750=CARTESIAN_POINT('Ctrl Pts',(-7.66670364630273,-22.7620360971839,
0.));
#227751=CARTESIAN_POINT('Ctrl Pts',(-7.66670364630273,-22.7620360971839,
12.));
#227752=CARTESIAN_POINT('Ctrl Pts',(-7.66723915895413,-22.7406115879508,
0.));
#227753=CARTESIAN_POINT('Ctrl Pts',(-7.66723915895413,-22.7406115879508,
12.));
#227754=CARTESIAN_POINT('Ctrl Pts',(-7.6677165719101,-22.7192867206242,
0.));
#227755=CARTESIAN_POINT('Ctrl Pts',(-7.6677165719101,-22.7192867206242,
12.));
#227756=CARTESIAN_POINT('Ctrl Pts',(-7.66813626029277,-22.6980622655446,
0.));
#227757=CARTESIAN_POINT('Ctrl Pts',(-7.66813626029277,-22.6980622655446,
12.));
#227758=CARTESIAN_POINT('Ctrl Pts',(-7.66849860491763,-22.6769390009889,
0.));
#227759=CARTESIAN_POINT('Ctrl Pts',(-7.66849860491763,-22.6769390009889,
12.));
#227760=CARTESIAN_POINT('Ctrl Pts',(-7.66880399241354,-22.6559177133133,
0.));
#227761=CARTESIAN_POINT('Ctrl Pts',(-7.66880399241354,-22.6559177133133,
12.));
#227762=CARTESIAN_POINT('Ctrl Pts',(-7.66905281533745,-22.6349991971547,
0.));
#227763=CARTESIAN_POINT('Ctrl Pts',(-7.66905281533745,-22.6349991971547,
12.));
#227764=CARTESIAN_POINT('Ctrl Pts',(-7.66924547229435,-22.6141842556248,
0.));
#227765=CARTESIAN_POINT('Ctrl Pts',(-7.66924547229435,-22.6141842556248,
12.));
#227766=CARTESIAN_POINT('Ctrl Pts',(-7.66938236806241,-22.5934737004955,
0.));
#227767=CARTESIAN_POINT('Ctrl Pts',(-7.66938236806241,-22.5934737004955,
12.));
#227768=CARTESIAN_POINT('Ctrl Pts',(-7.66946391372299,-22.5728683523828,
0.));
#227769=CARTESIAN_POINT('Ctrl Pts',(-7.66946391372299,-22.5728683523828,
12.));
#227770=CARTESIAN_POINT('Ctrl Pts',(-7.66949052679672,-22.5523690409109,
0.));
#227771=CARTESIAN_POINT('Ctrl Pts',(-7.66949052679672,-22.5523690409109,
12.));
#227772=CARTESIAN_POINT('Ctrl Pts',(-7.66946263138116,-22.5319766049191,
0.));
#227773=CARTESIAN_POINT('Ctrl Pts',(-7.66946263138116,-22.5319766049191,
12.));
#227774=CARTESIAN_POINT('Ctrl Pts',(-7.66938065829083,-22.5116918927023,
0.));
#227775=CARTESIAN_POINT('Ctrl Pts',(-7.66938065829083,-22.5116918927023,
12.));
#227776=CARTESIAN_POINT('Ctrl Pts',(-7.66924504520302,-22.4915157622308,
0.));
#227777=CARTESIAN_POINT('Ctrl Pts',(-7.66924504520302,-22.4915157622308,
12.));
#227778=CARTESIAN_POINT('Ctrl Pts',(-7.66905623680836,-22.47144908137,0.));
#227779=CARTESIAN_POINT('Ctrl Pts',(-7.66905623680836,-22.47144908137,12.));
#227780=CARTESIAN_POINT('Ctrl Pts',(-7.6688146849666,-22.4514927280862,
0.));
#227781=CARTESIAN_POINT('Ctrl Pts',(-7.6688146849666,-22.4514927280862,
12.));
#227782=CARTESIAN_POINT('Ctrl Pts',(-7.66852084886746,-22.4316475906616,
0.));
#227783=CARTESIAN_POINT('Ctrl Pts',(-7.66852084886746,-22.4316475906616,
12.));
#227784=CARTESIAN_POINT('Ctrl Pts',(-7.66817519519682,-22.411914567977,
0.));
#227785=CARTESIAN_POINT('Ctrl Pts',(-7.66817519519682,-22.411914567977,
12.));
#227786=CARTESIAN_POINT('Ctrl Pts',(-7.6677781983082,-22.3922945697782,
0.));
#227787=CARTESIAN_POINT('Ctrl Pts',(-7.6677781983082,-22.3922945697782,
12.));
#227788=CARTESIAN_POINT('Ctrl Pts',(-7.66733034039887,-22.3727885169361,
0.));
#227789=CARTESIAN_POINT('Ctrl Pts',(-7.66733034039887,-22.3727885169361,
12.));
#227790=CARTESIAN_POINT('Ctrl Pts',(-7.66683211169134,-22.3533973417013,
0.));
#227791=CARTESIAN_POINT('Ctrl Pts',(-7.66683211169134,-22.3533973417013,
12.));
#227792=CARTESIAN_POINT('Ctrl Pts',(-7.66628401061906,-22.3341219879454,
0.));
#227793=CARTESIAN_POINT('Ctrl Pts',(-7.66628401061906,-22.3341219879454,
12.));
#227794=CARTESIAN_POINT('Ctrl Pts',(-7.66568654402442,-22.3149634114823,
0.));
#227795=CARTESIAN_POINT('Ctrl Pts',(-7.66568654402442,-22.3149634114823,
12.));
#227796=CARTESIAN_POINT('Ctrl Pts',(-7.66504022736263,-22.2959225803925,
0.));
#227797=CARTESIAN_POINT('Ctrl Pts',(-7.66504022736263,-22.2959225803925,
12.));
#227798=CARTESIAN_POINT('Ctrl Pts',(-7.66434558490973,-22.2770004753332,
0.));
#227799=CARTESIAN_POINT('Ctrl Pts',(-7.66434558490973,-22.2770004753332,
12.));
#227800=CARTESIAN_POINT('Ctrl Pts',(-7.66360314997662,-22.2581980898487,
0.));
#227801=CARTESIAN_POINT('Ctrl Pts',(-7.66360314997662,-22.2581980898487,
12.));
#227802=CARTESIAN_POINT('Ctrl Pts',(-7.66281346512546,-22.239516430656,
0.));
#227803=CARTESIAN_POINT('Ctrl Pts',(-7.66281346512546,-22.239516430656,
12.));
#227804=CARTESIAN_POINT('Ctrl Pts',(-7.66197708240436,-22.2209565180098,
0.));
#227805=CARTESIAN_POINT('Ctrl Pts',(-7.66197708240436,-22.2209565180098,
12.));
#227806=CARTESIAN_POINT('Ctrl Pts',(-7.66109456359292,-22.2025193860972,
0.));
#227807=CARTESIAN_POINT('Ctrl Pts',(-7.66109456359292,-22.2025193860972,
12.));
#227808=CARTESIAN_POINT('Ctrl Pts',(-7.66016648045008,-22.1842060834092,
0.));
#227809=CARTESIAN_POINT('Ctrl Pts',(-7.66016648045008,-22.1842060834092,
12.));
#227810=CARTESIAN_POINT('Ctrl Pts',(-7.65919341496926,-22.1660176731174,
0.));
#227811=CARTESIAN_POINT('Ctrl Pts',(-7.65919341496926,-22.1660176731174,
12.));
#227812=CARTESIAN_POINT('Ctrl Pts',(-7.65817595963351,-22.1479552334206,
0.));
#227813=CARTESIAN_POINT('Ctrl Pts',(-7.65817595963351,-22.1479552334206,
12.));
#227814=CARTESIAN_POINT('Ctrl Pts',(-7.65711471769407,-22.1300198579671,
0.));
#227815=CARTESIAN_POINT('Ctrl Pts',(-7.65711471769407,-22.1300198579671,
12.));
#227816=CARTESIAN_POINT('Ctrl Pts',(-7.65601030346819,-22.1122126563327,
0.));
#227817=CARTESIAN_POINT('Ctrl Pts',(-7.65601030346819,-22.1122126563327,
12.));
#227818=CARTESIAN_POINT('Ctrl Pts',(-7.65486334263651,-22.094534754469,
0.));
#227819=CARTESIAN_POINT('Ctrl Pts',(-7.65486334263651,-22.094534754469,
12.));
#227820=CARTESIAN_POINT('Ctrl Pts',(-7.65367447254945,-22.0769872951596,
0.));
#227821=CARTESIAN_POINT('Ctrl Pts',(-7.65367447254945,-22.0769872951596,
12.));
#227822=CARTESIAN_POINT('Ctrl Pts',(-7.65244434253104,-22.0595714384432,
0.));
#227823=CARTESIAN_POINT('Ctrl Pts',(-7.65244434253104,-22.0595714384432,
12.));
#227824=CARTESIAN_POINT('Ctrl Pts',(-7.65117361421347,-22.0422883621176,
0.));
#227825=CARTESIAN_POINT('Ctrl Pts',(-7.65117361421347,-22.0422883621176,
12.));
#227826=CARTESIAN_POINT('Ctrl Pts',(-7.64986296190157,-22.0251392623209,
0.));
#227827=CARTESIAN_POINT('Ctrl Pts',(-7.64986296190157,-22.0251392623209,
12.));
#227828=CARTESIAN_POINT('Ctrl Pts',(-7.64851307293346,-22.0081253540773,
0.));
#227829=CARTESIAN_POINT('Ctrl Pts',(-7.64851307293346,-22.0081253540773,
12.));
#227830=CARTESIAN_POINT('Ctrl Pts',(-7.64712464805258,-21.9912478718542,
0.));
#227831=CARTESIAN_POINT('Ctrl Pts',(-7.64712464805258,-21.9912478718542,
12.));
#227832=CARTESIAN_POINT('Ctrl Pts',(-7.64569840177359,-21.97450807008,0.));
#227833=CARTESIAN_POINT('Ctrl Pts',(-7.64569840177359,-21.97450807008,12.));
#227834=CARTESIAN_POINT('Ctrl Pts',(-7.64423506279154,-21.9579072237653,
0.));
#227835=CARTESIAN_POINT('Ctrl Pts',(-7.64423506279154,-21.9579072237653,
12.));
#227836=CARTESIAN_POINT('Ctrl Pts',(-7.64273537442707,-21.9414466292074,
0.));
#227837=CARTESIAN_POINT('Ctrl Pts',(-7.64273537442707,-21.9414466292074,
12.));
#227838=CARTESIAN_POINT('Ctrl Pts',(-7.6412000950654,-21.9251276046546,
0.));
#227839=CARTESIAN_POINT('Ctrl Pts',(-7.6412000950654,-21.9251276046546,
12.));
#227840=CARTESIAN_POINT('Ctrl Pts',(-7.63962999860917,-21.9089514909873,
0.));
#227841=CARTESIAN_POINT('Ctrl Pts',(-7.63962999860917,-21.9089514909873,
12.));
#227842=CARTESIAN_POINT('Ctrl Pts',(-7.63802587492008,-21.8929196523511,
0.));
#227843=CARTESIAN_POINT('Ctrl Pts',(-7.63802587492008,-21.8929196523511,
12.));
#227844=CARTESIAN_POINT('Ctrl Pts',(-7.63638853033368,-21.8770334769492,
0.));
#227845=CARTESIAN_POINT('Ctrl Pts',(-7.63638853033368,-21.8770334769492,
12.));
#227846=CARTESIAN_POINT('Ctrl Pts',(-7.63471878821204,-21.8612943779086,
0.));
#227847=CARTESIAN_POINT('Ctrl Pts',(-7.63471878821204,-21.8612943779086,
12.));
#227848=CARTESIAN_POINT('Ctrl Pts',(-7.63301748948936,-21.8457037941084,
0.));
#227849=CARTESIAN_POINT('Ctrl Pts',(-7.63301748948936,-21.8457037941084,
12.));
#227850=CARTESIAN_POINT('Ctrl Pts',(-7.6312854932304,-21.8302631910197,
0.));
#227851=CARTESIAN_POINT('Ctrl Pts',(-7.6312854932304,-21.8302631910197,
12.));
#227852=CARTESIAN_POINT('Ctrl Pts',(-7.62952367718151,-21.8149740615093,
0.));
#227853=CARTESIAN_POINT('Ctrl Pts',(-7.62952367718151,-21.8149740615093,
12.));
#227854=CARTESIAN_POINT('Ctrl Pts',(-7.62773293842409,-21.7998379268583,
0.));
#227855=CARTESIAN_POINT('Ctrl Pts',(-7.62773293842409,-21.7998379268583,
12.));
#227856=CARTESIAN_POINT('Ctrl Pts',(-7.62591419404521,-21.7848563378022,
0.));
#227857=CARTESIAN_POINT('Ctrl Pts',(-7.62591419404521,-21.7848563378022,
12.));
#227858=CARTESIAN_POINT('Ctrl Pts',(-7.62406838181164,-21.7700308755583,
0.));
#227859=CARTESIAN_POINT('Ctrl Pts',(-7.62406838181164,-21.7700308755583,
12.));
#227860=CARTESIAN_POINT('Ctrl Pts',(-7.62219646084226,-21.7553631528329,
0.));
#227861=CARTESIAN_POINT('Ctrl Pts',(-7.62219646084226,-21.7553631528329,
12.));
#227862=CARTESIAN_POINT('Ctrl Pts',(-7.62029941230855,-21.7408548148657,
0.));
#227863=CARTESIAN_POINT('Ctrl Pts',(-7.62029941230855,-21.7408548148657,
12.));
#227864=CARTESIAN_POINT('Ctrl Pts',(-7.61837824030542,-21.7265075407977,
0.));
#227865=CARTESIAN_POINT('Ctrl Pts',(-7.61837824030542,-21.7265075407977,
12.));
#227866=CARTESIAN_POINT('Ctrl Pts',(-7.61643397270425,-21.7123230449835,
0.));
#227867=CARTESIAN_POINT('Ctrl Pts',(-7.61643397270425,-21.7123230449835,
12.));
#227868=CARTESIAN_POINT('Ctrl Pts',(-7.61446766202787,-21.6983030783321,
0.));
#227869=CARTESIAN_POINT('Ctrl Pts',(-7.61446766202787,-21.6983030783321,
12.));
#227870=CARTESIAN_POINT('Ctrl Pts',(-7.61248038630265,-21.6844494295813,
0.));
#227871=CARTESIAN_POINT('Ctrl Pts',(-7.61248038630265,-21.6844494295813,
12.));
#227872=CARTESIAN_POINT('Ctrl Pts',(-7.6104732500095,-21.6707639267573,
0.));
#227873=CARTESIAN_POINT('Ctrl Pts',(-7.6104732500095,-21.6707639267573,
12.));
#227874=CARTESIAN_POINT('Ctrl Pts',(-7.60844738512872,-21.6572484388079,
0.));
#227875=CARTESIAN_POINT('Ctrl Pts',(-7.60844738512872,-21.6572484388079,
12.));
#227876=CARTESIAN_POINT('Ctrl Pts',(-7.60640395216359,-21.6439048771743,
0.));
#227877=CARTESIAN_POINT('Ctrl Pts',(-7.60640395216359,-21.6439048771743,
12.));
#227878=CARTESIAN_POINT('Ctrl Pts',(-7.604344141183,-21.6307351973823,0.));
#227879=CARTESIAN_POINT('Ctrl Pts',(-7.604344141183,-21.6307351973823,12.));
#227880=CARTESIAN_POINT('Ctrl Pts',(-7.60226917285432,-21.6177414005991,
0.));
#227881=CARTESIAN_POINT('Ctrl Pts',(-7.60226917285432,-21.6177414005991,
12.));
#227882=CARTESIAN_POINT('Ctrl Pts',(-7.60018029988238,-21.6049255358842,
0.));
#227883=CARTESIAN_POINT('Ctrl Pts',(-7.60018029988238,-21.6049255358842,
12.));
#227884=CARTESIAN_POINT('Ctrl Pts',(-7.59807880846193,-21.5922897024466,
0.));
#227885=CARTESIAN_POINT('Ctrl Pts',(-7.59807880846193,-21.5922897024466,
12.));
#227886=CARTESIAN_POINT('Ctrl Pts',(-7.59596601973589,-21.5798360518978,
0.));
#227887=CARTESIAN_POINT('Ctrl Pts',(-7.59596601973589,-21.5798360518978,
12.));
#227888=CARTESIAN_POINT('Ctrl Pts',(-7.5938432912493,-21.5675667904728,
0.));
#227889=CARTESIAN_POINT('Ctrl Pts',(-7.5938432912493,-21.5675667904728,
12.));
#227890=CARTESIAN_POINT('Ctrl Pts',(-7.59171201844793,-21.5554841813465,
0.));
#227891=CARTESIAN_POINT('Ctrl Pts',(-7.59171201844793,-21.5554841813465,
12.));
#227892=CARTESIAN_POINT('Ctrl Pts',(-7.58957363620026,-21.5435905470113,
0.));
#227893=CARTESIAN_POINT('Ctrl Pts',(-7.58957363620026,-21.5435905470113,
12.));
#227894=CARTESIAN_POINT('Ctrl Pts',(-7.58742962034834,-21.5318882716735,
0.));
#227895=CARTESIAN_POINT('Ctrl Pts',(-7.58742962034834,-21.5318882716735,
12.));
#227896=CARTESIAN_POINT('Ctrl Pts',(-7.58528148919114,-21.5203798035294,
0.));
#227897=CARTESIAN_POINT('Ctrl Pts',(-7.58528148919114,-21.5203798035294,
12.));
#227898=CARTESIAN_POINT('Ctrl Pts',(-7.58313080519159,-21.5090676573866,
0.));
#227899=CARTESIAN_POINT('Ctrl Pts',(-7.58313080519159,-21.5090676573866,
12.));
#227900=CARTESIAN_POINT('Ctrl Pts',(-7.5809791779073,-21.4979544192739,
0.));
#227901=CARTESIAN_POINT('Ctrl Pts',(-7.5809791779073,-21.4979544192739,
12.));
#227902=CARTESIAN_POINT('Ctrl Pts',(-7.57882826679131,-21.4870427508193,
0.));
#227903=CARTESIAN_POINT('Ctrl Pts',(-7.57882826679131,-21.4870427508193,
12.));
#227904=CARTESIAN_POINT('Ctrl Pts',(-7.57667978403003,-21.4763353936766,
0.));
#227905=CARTESIAN_POINT('Ctrl Pts',(-7.57667978403003,-21.4763353936766,
12.));
#227906=CARTESIAN_POINT('Ctrl Pts',(-7.57453549743435,-21.4658351740135,
0.));
#227907=CARTESIAN_POINT('Ctrl Pts',(-7.57453549743435,-21.4658351740135,
12.));
#227908=CARTESIAN_POINT('Ctrl Pts',(-7.57239723223521,-21.4555450053147,
0.));
#227909=CARTESIAN_POINT('Ctrl Pts',(-7.57239723223521,-21.4555450053147,
12.));
#227910=CARTESIAN_POINT('Ctrl Pts',(-7.5702668726117,-21.445467890751,0.));
#227911=CARTESIAN_POINT('Ctrl Pts',(-7.5702668726117,-21.445467890751,12.));
#227912=CARTESIAN_POINT('Ctrl Pts',(-7.56814636360842,-21.435606926151,
0.));
#227913=CARTESIAN_POINT('Ctrl Pts',(-7.56814636360842,-21.435606926151,
12.));
#227914=CARTESIAN_POINT('Ctrl Pts',(-7.56603771218706,-21.4259653015732,
0.));
#227915=CARTESIAN_POINT('Ctrl Pts',(-7.56603771218706,-21.4259653015732,
12.));
#227916=CARTESIAN_POINT('Ctrl Pts',(-7.56394299313683,-21.4165463106252,
0.));
#227917=CARTESIAN_POINT('Ctrl Pts',(-7.56394299313683,-21.4165463106252,
12.));
#227918=CARTESIAN_POINT('Ctrl Pts',(-7.56186435703622,-21.4073533630364,
0.));
#227919=CARTESIAN_POINT('Ctrl Pts',(-7.56186435703622,-21.4073533630364,
12.));
#227920=CARTESIAN_POINT('Ctrl Pts',(-7.55980403700615,-21.3983899952988,
0.));
#227921=CARTESIAN_POINT('Ctrl Pts',(-7.55980403700615,-21.3983899952988,
12.));
#227922=CARTESIAN_POINT('Ctrl Pts',(-7.55776435731422,-21.3896598842119,
0.));
#227923=CARTESIAN_POINT('Ctrl Pts',(-7.55776435731422,-21.3896598842119,
12.));
#227924=CARTESIAN_POINT('Ctrl Pts',(-7.55574773403508,-21.3811668478933,
0.));
#227925=CARTESIAN_POINT('Ctrl Pts',(-7.55574773403508,-21.3811668478933,
12.));
#227926=CARTESIAN_POINT('Ctrl Pts',(-7.55375667080032,-21.3729148390244,
0.));
#227927=CARTESIAN_POINT('Ctrl Pts',(-7.55375667080032,-21.3729148390244,
12.));
#227928=CARTESIAN_POINT('Ctrl Pts',(-7.55179375777442,-21.3649079431864,
0.));
#227929=CARTESIAN_POINT('Ctrl Pts',(-7.55179375777442,-21.3649079431864,
12.));
#227930=CARTESIAN_POINT('Ctrl Pts',(-7.54986166521307,-21.3571503685853,
0.));
#227931=CARTESIAN_POINT('Ctrl Pts',(-7.54986166521307,-21.3571503685853,
12.));
#227932=CARTESIAN_POINT('Ctrl Pts',(-7.54796316246327,-21.349646476153,
0.));
#227933=CARTESIAN_POINT('Ctrl Pts',(-7.54796316246327,-21.349646476153,
12.));
#227934=CARTESIAN_POINT('Ctrl Pts',(-7.54610114948351,-21.3424008295038,
0.));
#227935=CARTESIAN_POINT('Ctrl Pts',(-7.54610114948351,-21.3424008295038,
12.));
#227936=CARTESIAN_POINT('Ctrl Pts',(-7.54427868151269,-21.3354182340149,
0.));
#227937=CARTESIAN_POINT('Ctrl Pts',(-7.54427868151269,-21.3354182340149,
12.));
#227938=CARTESIAN_POINT('Ctrl Pts',(-7.54249900377032,-21.328703791771,
0.));
#227939=CARTESIAN_POINT('Ctrl Pts',(-7.54249900377032,-21.328703791771,
12.));
#227940=CARTESIAN_POINT('Ctrl Pts',(-7.5407655203828,-21.3222628524165,
0.));
#227941=CARTESIAN_POINT('Ctrl Pts',(-7.5407655203828,-21.3222628524165,
12.));
#227942=CARTESIAN_POINT('Ctrl Pts',(-7.53908175169899,-21.3161009456256,
0.));
#227943=CARTESIAN_POINT('Ctrl Pts',(-7.53908175169899,-21.3161009456256,
12.));
#227944=CARTESIAN_POINT('Ctrl Pts',(-7.5374512936462,-21.3102237167729,
0.));
#227945=CARTESIAN_POINT('Ctrl Pts',(-7.5374512936462,-21.3102237167729,
12.));
#227946=CARTESIAN_POINT('Ctrl Pts',(-7.53587778251743,-21.3046368712156,
0.));
#227947=CARTESIAN_POINT('Ctrl Pts',(-7.53587778251743,-21.3046368712156,
12.));
#227948=CARTESIAN_POINT('Ctrl Pts',(-7.53436505309949,-21.2993464250717,
0.));
#227949=CARTESIAN_POINT('Ctrl Pts',(-7.53436505309949,-21.2993464250717,
12.));
#227950=CARTESIAN_POINT('Ctrl Pts',(-7.53291726078527,-21.2943588989331,
0.));
#227951=CARTESIAN_POINT('Ctrl Pts',(-7.53291726078527,-21.2943588989331,
12.));
#227952=CARTESIAN_POINT('Ctrl Pts',(-7.53153906987847,-21.2896816163843,
0.));
#227953=CARTESIAN_POINT('Ctrl Pts',(-7.53153906987847,-21.2896816163843,
12.));
#227954=CARTESIAN_POINT('Ctrl Pts',(-7.53023562438221,-21.2853226580658,
0.));
#227955=CARTESIAN_POINT('Ctrl Pts',(-7.53023562438221,-21.2853226580658,
12.));
#227956=CARTESIAN_POINT('Ctrl Pts',(-7.52901217930407,-21.2812902781143,
0.));
#227957=CARTESIAN_POINT('Ctrl Pts',(-7.52901217930407,-21.2812902781143,
12.));
#227958=CARTESIAN_POINT('Ctrl Pts',(-7.52787386225344,-21.2775925269651,
0.));
#227959=CARTESIAN_POINT('Ctrl Pts',(-7.52787386225344,-21.2775925269651,
12.));
#227960=CARTESIAN_POINT('Ctrl Pts',(-7.52682526918561,-21.2742366113578,
0.));
#227961=CARTESIAN_POINT('Ctrl Pts',(-7.52682526918561,-21.2742366113578,
12.));
#227962=CARTESIAN_POINT('Ctrl Pts',(-7.52587126095544,-21.2712301573465,
0.));
#227963=CARTESIAN_POINT('Ctrl Pts',(-7.52587126095544,-21.2712301573465,
12.));
#227964=CARTESIAN_POINT('Ctrl Pts',(-7.52501770333522,-21.2685823838672,
0.));
#227965=CARTESIAN_POINT('Ctrl Pts',(-7.52501770333522,-21.2685823838672,
12.));
#227966=CARTESIAN_POINT('Ctrl Pts',(-7.52427261074264,-21.266305915706,
0.));
#227967=CARTESIAN_POINT('Ctrl Pts',(-7.52427261074264,-21.266305915706,
12.));
#227968=CARTESIAN_POINT('Ctrl Pts',(-7.52364573027521,-21.2644161259965,
0.));
#227969=CARTESIAN_POINT('Ctrl Pts',(-7.52364573027521,-21.2644161259965,
12.));
#227970=CARTESIAN_POINT('Ctrl Pts',(-7.52314642316203,-21.262927782038,
0.));
#227971=CARTESIAN_POINT('Ctrl Pts',(-7.52314642316203,-21.262927782038,
12.));
#227972=CARTESIAN_POINT('Ctrl Pts',(-7.52278182242728,-21.261852128355,
0.));
#227973=CARTESIAN_POINT('Ctrl Pts',(-7.52278182242728,-21.261852128355,
12.));
#227974=CARTESIAN_POINT('Ctrl Pts',(-7.52260064231736,-21.2613260540651,
0.));
#227975=CARTESIAN_POINT('Ctrl Pts',(-7.52260064231736,-21.2613260540651,
12.));
#227976=CARTESIAN_POINT('Ctrl Pts',(-7.52252744144958,-21.261120447486,
0.));
#227977=CARTESIAN_POINT('Ctrl Pts',(-7.52252744144958,-21.261120447486,
12.));
#227978=CARTESIAN_POINT('Ctrl Pts',(-7.52250649703992,-21.2610673466883,
0.));
#227979=CARTESIAN_POINT('Ctrl Pts',(-7.52250649703992,-21.2610673466883,
12.));
#227980=CARTESIAN_POINT('Ctrl Pts',(-7.52250298901266,-21.2610617890679,
0.));
#227981=CARTESIAN_POINT('Ctrl Pts',(-7.52250298901266,-21.2610617890679,
12.));
#227982=CARTESIAN_POINT('',(-7.36589684767345,-24.9347862158358,0.));
#227983=CARTESIAN_POINT('Ctrl Pts',(-7.36589684767345,-24.9347862158358,
0.));
#227984=CARTESIAN_POINT('Ctrl Pts',(-7.36721909028843,-24.9292275670674,
0.));
#227985=CARTESIAN_POINT('Ctrl Pts',(-7.36985593120091,-24.9181155530543,
0.));
#227986=CARTESIAN_POINT('Ctrl Pts',(-7.37378825961676,-24.901463382605,
0.));
#227987=CARTESIAN_POINT('Ctrl Pts',(-7.3789854964027,-24.8792921911115,
0.));
#227988=CARTESIAN_POINT('Ctrl Pts',(-7.38540558903621,-24.8516310625176,
0.));
#227989=CARTESIAN_POINT('Ctrl Pts',(-7.39174922585809,-24.8240228520893,
0.));
#227990=CARTESIAN_POINT('Ctrl Pts',(-7.39801641583013,-24.7964676646431,
0.));
#227991=CARTESIAN_POINT('Ctrl Pts',(-7.40420718661603,-24.7689656668983,
0.));
#227992=CARTESIAN_POINT('Ctrl Pts',(-7.41032159082382,-24.7415170994784,
0.));
#227993=CARTESIAN_POINT('Ctrl Pts',(-7.41635971481674,-24.7141222950051,
0.));
#227994=CARTESIAN_POINT('Ctrl Pts',(-7.42232167766266,-24.6867816727192,
0.));
#227995=CARTESIAN_POINT('Ctrl Pts',(-7.42820762159126,-24.6594957128756,
0.));
#227996=CARTESIAN_POINT('Ctrl Pts',(-7.43401770489524,-24.6322649369517,
0.));
#227997=CARTESIAN_POINT('Ctrl Pts',(-7.43975209375504,-24.6050898852368,
0.));
#227998=CARTESIAN_POINT('Ctrl Pts',(-7.44541095473135,-24.577971096086,
0.));
#227999=CARTESIAN_POINT('Ctrl Pts',(-7.4509944465116,-24.5509090831559,
0.));
#228000=CARTESIAN_POINT('Ctrl Pts',(-7.45650271335862,-24.5239043173072,
0.));
#228001=CARTESIAN_POINT('Ctrl Pts',(-7.46193588961464,-24.4969572391483,
0.));
#228002=CARTESIAN_POINT('Ctrl Pts',(-7.46729410308787,-24.4700682684524,
0.));
#228003=CARTESIAN_POINT('Ctrl Pts',(-7.47257747883246,-24.443237814649,
0.));
#228004=CARTESIAN_POINT('Ctrl Pts',(-7.47778614286565,-24.4164662871163,
0.));
#228005=CARTESIAN_POINT('Ctrl Pts',(-7.48292022569301,-24.3897541049254,
0.));
#228006=CARTESIAN_POINT('Ctrl Pts',(-7.48797986651909,-24.3631017084524,
0.));
#228007=CARTESIAN_POINT('Ctrl Pts',(-7.49296521252421,-24.3365095573685,
0.));
#228008=CARTESIAN_POINT('Ctrl Pts',(-7.49787641695439,-24.3099781253355,
0.));
#228009=CARTESIAN_POINT('Ctrl Pts',(-7.50271363765152,-24.2835078958973,
0.));
#228010=CARTESIAN_POINT('Ctrl Pts',(-7.50747703535134,-24.2570993577034,
0.));
#228011=CARTESIAN_POINT('Ctrl Pts',(-7.51216677222181,-24.2307530003887,
0.));
#228012=CARTESIAN_POINT('Ctrl Pts',(-7.51678300997949,-24.2044693092349,
0.));
#228013=CARTESIAN_POINT('Ctrl Pts',(-7.52132590953802,-24.1782487641594,
0.));
#228014=CARTESIAN_POINT('Ctrl Pts',(-7.52579563201424,-24.1520918425364,
0.));
#228015=CARTESIAN_POINT('Ctrl Pts',(-7.53019233935502,-24.1259990209207,
0.));
#228016=CARTESIAN_POINT('Ctrl Pts',(-7.53451619514649,-24.0999707772642,
0.));
#228017=CARTESIAN_POINT('Ctrl Pts',(-7.53876736531014,-24.0740075927985,
0.));
#228018=CARTESIAN_POINT('Ctrl Pts',(-7.54294601896145,-24.0481099543353,
0.));
#228019=CARTESIAN_POINT('Ctrl Pts',(-7.5470523288591,-24.022278355453,0.));
#228020=CARTESIAN_POINT('Ctrl Pts',(-7.55108647097441,-23.9965132953185,
0.));
#228021=CARTESIAN_POINT('Ctrl Pts',(-7.55504862424812,-23.9708152779884,
0.));
#228022=CARTESIAN_POINT('Ctrl Pts',(-7.55893897027683,-23.9451848115,0.));
#228023=CARTESIAN_POINT('Ctrl Pts',(-7.56275769304773,-23.9196224070759,
0.));
#228024=CARTESIAN_POINT('Ctrl Pts',(-7.56650497863792,-23.8941285782003,
0.));
#228025=CARTESIAN_POINT('Ctrl Pts',(-7.57018101500711,-23.8687038399597,
0.));
#228026=CARTESIAN_POINT('Ctrl Pts',(-7.57378599219817,-23.8433487096134,
0.));
#228027=CARTESIAN_POINT('Ctrl Pts',(-7.57732010249066,-23.8180637069977,
0.));
#228028=CARTESIAN_POINT('Ctrl Pts',(-7.58078354058212,-23.7928493549908,
0.));
#228029=CARTESIAN_POINT('Ctrl Pts',(-7.58417650376272,-23.7677061799376,
0.));
#228030=CARTESIAN_POINT('Ctrl Pts',(-7.58749919210832,-23.7426347121006,
0.));
#228031=CARTESIAN_POINT('Ctrl Pts',(-7.59075180865327,-23.7176354860457,
0.));
#228032=CARTESIAN_POINT('Ctrl Pts',(-7.59393455934042,-23.6927090405067,
0.));
#228033=CARTESIAN_POINT('Ctrl Pts',(-7.59704765299572,-23.6678559182876,
0.));
#228034=CARTESIAN_POINT('Ctrl Pts',(-7.6000913013013,-23.6430766661419,
0.));
#228035=CARTESIAN_POINT('Ctrl Pts',(-7.60306571877806,-23.6183718346576,
0.));
#228036=CARTESIAN_POINT('Ctrl Pts',(-7.60597112277094,-23.5937419781244,
0.));
#228037=CARTESIAN_POINT('Ctrl Pts',(-7.608807733446,-23.5691876544243,0.));
#228038=CARTESIAN_POINT('Ctrl Pts',(-7.61157577385372,-23.5447094252028,
0.));
#228039=CARTESIAN_POINT('Ctrl Pts',(-7.61427546999299,-23.5203078560128,
0.));
#228040=CARTESIAN_POINT('Ctrl Pts',(-7.61690705088319,-23.4959835164608,
0.));
#228041=CARTESIAN_POINT('Ctrl Pts',(-7.61947074863978,-23.4717369803438,
0.));
#228042=CARTESIAN_POINT('Ctrl Pts',(-7.62196679855957,-23.4475688257854,
0.));
#228043=CARTESIAN_POINT('Ctrl Pts',(-7.62439543920055,-23.4234796353544,
0.));
#228044=CARTESIAN_POINT('Ctrl Pts',(-7.62675691240335,-23.3994699961122,
0.));
#228045=CARTESIAN_POINT('Ctrl Pts',(-7.62905146332598,-23.3755404996638,
0.));
#228046=CARTESIAN_POINT('Ctrl Pts',(-7.63127934048139,-23.3516917421973,
0.));
#228047=CARTESIAN_POINT('Ctrl Pts',(-7.63344079578163,-23.3279243245241,
0.));
#228048=CARTESIAN_POINT('Ctrl Pts',(-7.63553608458784,-23.3042388521021,
0.));
#228049=CARTESIAN_POINT('Ctrl Pts',(-7.63756546576375,-23.2806359350853,
0.));
#228050=CARTESIAN_POINT('Ctrl Pts',(-7.63952920172837,-23.2571161884487,
0.));
#228051=CARTESIAN_POINT('Ctrl Pts',(-7.64142755851508,-23.2336802320912,
0.));
#228052=CARTESIAN_POINT('Ctrl Pts',(-7.64326080583684,-23.2103286909399,
0.));
#228053=CARTESIAN_POINT('Ctrl Pts',(-7.64502921715483,-23.1870621950452,
0.));
#228054=CARTESIAN_POINT('Ctrl Pts',(-7.64673306975797,-23.1638813796691,
0.));
#228055=CARTESIAN_POINT('Ctrl Pts',(-7.64837264482929,-23.1407868853815,
0.));
#228056=CARTESIAN_POINT('Ctrl Pts',(-7.64994822749845,-23.1177793581674,
0.));
#228057=CARTESIAN_POINT('Ctrl Pts',(-7.65146010690465,-23.0948594495246,
0.));
#228058=CARTESIAN_POINT('Ctrl Pts',(-7.65290857626357,-23.072027816555,
0.));
#228059=CARTESIAN_POINT('Ctrl Pts',(-7.65429393293955,-23.049285122053,
0.));
#228060=CARTESIAN_POINT('Ctrl Pts',(-7.65561647852555,-23.0266320345792,
0.));
#228061=CARTESIAN_POINT('Ctrl Pts',(-7.6568765189133,-23.004069228582,0.));
#228062=CARTESIAN_POINT('Ctrl Pts',(-7.65807436436453,-22.9815973845301,
0.));
#228063=CARTESIAN_POINT('Ctrl Pts',(-7.65921032958912,-22.9592171890332,
0.));
#228064=CARTESIAN_POINT('Ctrl Pts',(-7.66028473382777,-22.9369293349592,
0.));
#228065=CARTESIAN_POINT('Ctrl Pts',(-7.661297900941,-22.9147345215418,0.));
#228066=CARTESIAN_POINT('Ctrl Pts',(-7.66225015950148,-22.8926334544879,
0.));
#228067=CARTESIAN_POINT('Ctrl Pts',(-7.66314184287334,-22.870626846128,
0.));
#228068=CARTESIAN_POINT('Ctrl Pts',(-7.66397328929805,-22.8487154155569,
0.));
#228069=CARTESIAN_POINT('Ctrl Pts',(-7.66474484198553,-22.8268998887678,
0.));
#228070=CARTESIAN_POINT('Ctrl Pts',(-7.66545684920988,-22.8051809987833,
0.));
#228071=CARTESIAN_POINT('Ctrl Pts',(-7.66610966441259,-22.7835594857697,
0.));
#228072=CARTESIAN_POINT('Ctrl Pts',(-7.66670364630273,-22.7620360971839,
0.));
#228073=CARTESIAN_POINT('Ctrl Pts',(-7.66723915895413,-22.7406115879508,
0.));
#228074=CARTESIAN_POINT('Ctrl Pts',(-7.6677165719101,-22.7192867206242,
0.));
#228075=CARTESIAN_POINT('Ctrl Pts',(-7.66813626029277,-22.6980622655446,
0.));
#228076=CARTESIAN_POINT('Ctrl Pts',(-7.66849860491763,-22.6769390009889,
0.));
#228077=CARTESIAN_POINT('Ctrl Pts',(-7.66880399241354,-22.6559177133133,
0.));
#228078=CARTESIAN_POINT('Ctrl Pts',(-7.66905281533745,-22.6349991971547,
0.));
#228079=CARTESIAN_POINT('Ctrl Pts',(-7.66924547229435,-22.6141842556248,
0.));
#228080=CARTESIAN_POINT('Ctrl Pts',(-7.66938236806241,-22.5934737004955,
0.));
#228081=CARTESIAN_POINT('Ctrl Pts',(-7.66946391372299,-22.5728683523828,
0.));
#228082=CARTESIAN_POINT('Ctrl Pts',(-7.66949052679672,-22.5523690409109,
0.));
#228083=CARTESIAN_POINT('Ctrl Pts',(-7.66946263138116,-22.5319766049191,
0.));
#228084=CARTESIAN_POINT('Ctrl Pts',(-7.66938065829083,-22.5116918927023,
0.));
#228085=CARTESIAN_POINT('Ctrl Pts',(-7.66924504520302,-22.4915157622308,
0.));
#228086=CARTESIAN_POINT('Ctrl Pts',(-7.66905623680836,-22.47144908137,0.));
#228087=CARTESIAN_POINT('Ctrl Pts',(-7.6688146849666,-22.4514927280862,
0.));
#228088=CARTESIAN_POINT('Ctrl Pts',(-7.66852084886746,-22.4316475906616,
0.));
#228089=CARTESIAN_POINT('Ctrl Pts',(-7.66817519519682,-22.411914567977,
0.));
#228090=CARTESIAN_POINT('Ctrl Pts',(-7.6677781983082,-22.3922945697782,
0.));
#228091=CARTESIAN_POINT('Ctrl Pts',(-7.66733034039887,-22.3727885169361,
0.));
#228092=CARTESIAN_POINT('Ctrl Pts',(-7.66683211169134,-22.3533973417013,
0.));
#228093=CARTESIAN_POINT('Ctrl Pts',(-7.66628401061906,-22.3341219879454,
0.));
#228094=CARTESIAN_POINT('Ctrl Pts',(-7.66568654402442,-22.3149634114823,
0.));
#228095=CARTESIAN_POINT('Ctrl Pts',(-7.66504022736263,-22.2959225803925,
0.));
#228096=CARTESIAN_POINT('Ctrl Pts',(-7.66434558490973,-22.2770004753332,
0.));
#228097=CARTESIAN_POINT('Ctrl Pts',(-7.66360314997662,-22.2581980898487,
0.));
#228098=CARTESIAN_POINT('Ctrl Pts',(-7.66281346512546,-22.239516430656,
0.));
#228099=CARTESIAN_POINT('Ctrl Pts',(-7.66197708240436,-22.2209565180098,
0.));
#228100=CARTESIAN_POINT('Ctrl Pts',(-7.66109456359292,-22.2025193860972,
0.));
#228101=CARTESIAN_POINT('Ctrl Pts',(-7.66016648045008,-22.1842060834092,
0.));
#228102=CARTESIAN_POINT('Ctrl Pts',(-7.65919341496926,-22.1660176731174,
0.));
#228103=CARTESIAN_POINT('Ctrl Pts',(-7.65817595963351,-22.1479552334206,
0.));
#228104=CARTESIAN_POINT('Ctrl Pts',(-7.65711471769407,-22.1300198579671,
0.));
#228105=CARTESIAN_POINT('Ctrl Pts',(-7.65601030346819,-22.1122126563327,
0.));
#228106=CARTESIAN_POINT('Ctrl Pts',(-7.65486334263651,-22.094534754469,
0.));
#228107=CARTESIAN_POINT('Ctrl Pts',(-7.65367447254945,-22.0769872951596,
0.));
#228108=CARTESIAN_POINT('Ctrl Pts',(-7.65244434253104,-22.0595714384432,
0.));
#228109=CARTESIAN_POINT('Ctrl Pts',(-7.65117361421347,-22.0422883621176,
0.));
#228110=CARTESIAN_POINT('Ctrl Pts',(-7.64986296190157,-22.0251392623209,
0.));
#228111=CARTESIAN_POINT('Ctrl Pts',(-7.64851307293346,-22.0081253540773,
0.));
#228112=CARTESIAN_POINT('Ctrl Pts',(-7.64712464805258,-21.9912478718542,
0.));
#228113=CARTESIAN_POINT('Ctrl Pts',(-7.64569840177359,-21.97450807008,0.));
#228114=CARTESIAN_POINT('Ctrl Pts',(-7.64423506279154,-21.9579072237653,
0.));
#228115=CARTESIAN_POINT('Ctrl Pts',(-7.64273537442707,-21.9414466292074,
0.));
#228116=CARTESIAN_POINT('Ctrl Pts',(-7.6412000950654,-21.9251276046546,
0.));
#228117=CARTESIAN_POINT('Ctrl Pts',(-7.63962999860917,-21.9089514909873,
0.));
#228118=CARTESIAN_POINT('Ctrl Pts',(-7.63802587492008,-21.8929196523511,
0.));
#228119=CARTESIAN_POINT('Ctrl Pts',(-7.63638853033368,-21.8770334769492,
0.));
#228120=CARTESIAN_POINT('Ctrl Pts',(-7.63471878821204,-21.8612943779086,
0.));
#228121=CARTESIAN_POINT('Ctrl Pts',(-7.63301748948936,-21.8457037941084,
0.));
#228122=CARTESIAN_POINT('Ctrl Pts',(-7.6312854932304,-21.8302631910197,
0.));
#228123=CARTESIAN_POINT('Ctrl Pts',(-7.62952367718151,-21.8149740615093,
0.));
#228124=CARTESIAN_POINT('Ctrl Pts',(-7.62773293842409,-21.7998379268583,
0.));
#228125=CARTESIAN_POINT('Ctrl Pts',(-7.62591419404521,-21.7848563378022,
0.));
#228126=CARTESIAN_POINT('Ctrl Pts',(-7.62406838181164,-21.7700308755583,
0.));
#228127=CARTESIAN_POINT('Ctrl Pts',(-7.62219646084226,-21.7553631528329,
0.));
#228128=CARTESIAN_POINT('Ctrl Pts',(-7.62029941230855,-21.7408548148657,
0.));
#228129=CARTESIAN_POINT('Ctrl Pts',(-7.61837824030542,-21.7265075407977,
0.));
#228130=CARTESIAN_POINT('Ctrl Pts',(-7.61643397270425,-21.7123230449835,
0.));
#228131=CARTESIAN_POINT('Ctrl Pts',(-7.61446766202787,-21.6983030783321,
0.));
#228132=CARTESIAN_POINT('Ctrl Pts',(-7.61248038630265,-21.6844494295813,
0.));
#228133=CARTESIAN_POINT('Ctrl Pts',(-7.6104732500095,-21.6707639267573,
0.));
#228134=CARTESIAN_POINT('Ctrl Pts',(-7.60844738512872,-21.6572484388079,
0.));
#228135=CARTESIAN_POINT('Ctrl Pts',(-7.60640395216359,-21.6439048771743,
0.));
#228136=CARTESIAN_POINT('Ctrl Pts',(-7.604344141183,-21.6307351973823,0.));
#228137=CARTESIAN_POINT('Ctrl Pts',(-7.60226917285432,-21.6177414005991,
0.));
#228138=CARTESIAN_POINT('Ctrl Pts',(-7.60018029988238,-21.6049255358842,
0.));
#228139=CARTESIAN_POINT('Ctrl Pts',(-7.59807880846193,-21.5922897024466,
0.));
#228140=CARTESIAN_POINT('Ctrl Pts',(-7.59596601973589,-21.5798360518978,
0.));
#228141=CARTESIAN_POINT('Ctrl Pts',(-7.5938432912493,-21.5675667904728,
0.));
#228142=CARTESIAN_POINT('Ctrl Pts',(-7.59171201844793,-21.5554841813465,
0.));
#228143=CARTESIAN_POINT('Ctrl Pts',(-7.58957363620026,-21.5435905470113,
0.));
#228144=CARTESIAN_POINT('Ctrl Pts',(-7.58742962034834,-21.5318882716735,
0.));
#228145=CARTESIAN_POINT('Ctrl Pts',(-7.58528148919114,-21.5203798035294,
0.));
#228146=CARTESIAN_POINT('Ctrl Pts',(-7.58313080519159,-21.5090676573866,
0.));
#228147=CARTESIAN_POINT('Ctrl Pts',(-7.5809791779073,-21.4979544192739,
0.));
#228148=CARTESIAN_POINT('Ctrl Pts',(-7.57882826679131,-21.4870427508193,
0.));
#228149=CARTESIAN_POINT('Ctrl Pts',(-7.57667978403003,-21.4763353936766,
0.));
#228150=CARTESIAN_POINT('Ctrl Pts',(-7.57453549743435,-21.4658351740135,
0.));
#228151=CARTESIAN_POINT('Ctrl Pts',(-7.57239723223521,-21.4555450053147,
0.));
#228152=CARTESIAN_POINT('Ctrl Pts',(-7.5702668726117,-21.445467890751,0.));
#228153=CARTESIAN_POINT('Ctrl Pts',(-7.56814636360842,-21.435606926151,
0.));
#228154=CARTESIAN_POINT('Ctrl Pts',(-7.56603771218706,-21.4259653015732,
0.));
#228155=CARTESIAN_POINT('Ctrl Pts',(-7.56394299313683,-21.4165463106252,
0.));
#228156=CARTESIAN_POINT('Ctrl Pts',(-7.56186435703622,-21.4073533630364,
0.));
#228157=CARTESIAN_POINT('Ctrl Pts',(-7.55980403700615,-21.3983899952988,
0.));
#228158=CARTESIAN_POINT('Ctrl Pts',(-7.55776435731422,-21.3896598842119,
0.));
#228159=CARTESIAN_POINT('Ctrl Pts',(-7.55574773403508,-21.3811668478933,
0.));
#228160=CARTESIAN_POINT('Ctrl Pts',(-7.55375667080032,-21.3729148390244,
0.));
#228161=CARTESIAN_POINT('Ctrl Pts',(-7.55179375777442,-21.3649079431864,
0.));
#228162=CARTESIAN_POINT('Ctrl Pts',(-7.54986166521307,-21.3571503685853,
0.));
#228163=CARTESIAN_POINT('Ctrl Pts',(-7.54796316246327,-21.349646476153,
0.));
#228164=CARTESIAN_POINT('Ctrl Pts',(-7.54610114948351,-21.3424008295038,
0.));
#228165=CARTESIAN_POINT('Ctrl Pts',(-7.54427868151269,-21.3354182340149,
0.));
#228166=CARTESIAN_POINT('Ctrl Pts',(-7.54249900377032,-21.328703791771,
0.));
#228167=CARTESIAN_POINT('Ctrl Pts',(-7.5407655203828,-21.3222628524165,
0.));
#228168=CARTESIAN_POINT('Ctrl Pts',(-7.53908175169899,-21.3161009456256,
0.));
#228169=CARTESIAN_POINT('Ctrl Pts',(-7.5374512936462,-21.3102237167729,
0.));
#228170=CARTESIAN_POINT('Ctrl Pts',(-7.53587778251743,-21.3046368712156,
0.));
#228171=CARTESIAN_POINT('Ctrl Pts',(-7.53436505309949,-21.2993464250717,
0.));
#228172=CARTESIAN_POINT('Ctrl Pts',(-7.53291726078527,-21.2943588989331,
0.));
#228173=CARTESIAN_POINT('Ctrl Pts',(-7.53153906987847,-21.2896816163843,
0.));
#228174=CARTESIAN_POINT('Ctrl Pts',(-7.53023562438221,-21.2853226580658,
0.));
#228175=CARTESIAN_POINT('Ctrl Pts',(-7.52901217930407,-21.2812902781143,
0.));
#228176=CARTESIAN_POINT('Ctrl Pts',(-7.52787386225344,-21.2775925269651,
0.));
#228177=CARTESIAN_POINT('Ctrl Pts',(-7.52682526918561,-21.2742366113578,
0.));
#228178=CARTESIAN_POINT('Ctrl Pts',(-7.52587126095544,-21.2712301573465,
0.));
#228179=CARTESIAN_POINT('Ctrl Pts',(-7.52501770333522,-21.2685823838672,
0.));
#228180=CARTESIAN_POINT('Ctrl Pts',(-7.52427261074264,-21.266305915706,
0.));
#228181=CARTESIAN_POINT('Ctrl Pts',(-7.52364573027521,-21.2644161259965,
0.));
#228182=CARTESIAN_POINT('Ctrl Pts',(-7.52314642316203,-21.262927782038,
0.));
#228183=CARTESIAN_POINT('Ctrl Pts',(-7.52278182242728,-21.261852128355,
0.));
#228184=CARTESIAN_POINT('Ctrl Pts',(-7.52260064231736,-21.2613260540651,
0.));
#228185=CARTESIAN_POINT('Ctrl Pts',(-7.52252744144958,-21.261120447486,
0.));
#228186=CARTESIAN_POINT('Ctrl Pts',(-7.52250649703992,-21.2610673466883,
0.));
#228187=CARTESIAN_POINT('Ctrl Pts',(-7.52250298901266,-21.2610617890679,
0.));
#228188=CARTESIAN_POINT('',(-7.36589684767345,-24.9347862158358,12.));
#228189=CARTESIAN_POINT('',(-7.36589684767345,-24.9347862158358,0.));
#228190=CARTESIAN_POINT('Ctrl Pts',(-7.52250298901266,-21.2610617890679,
12.));
#228191=CARTESIAN_POINT('Ctrl Pts',(-7.52250649703992,-21.2610673466883,
12.));
#228192=CARTESIAN_POINT('Ctrl Pts',(-7.52252744144958,-21.261120447486,
12.));
#228193=CARTESIAN_POINT('Ctrl Pts',(-7.52260064231736,-21.2613260540651,
12.));
#228194=CARTESIAN_POINT('Ctrl Pts',(-7.52278182242728,-21.261852128355,
12.));
#228195=CARTESIAN_POINT('Ctrl Pts',(-7.52314642316203,-21.262927782038,
12.));
#228196=CARTESIAN_POINT('Ctrl Pts',(-7.52364573027521,-21.2644161259965,
12.));
#228197=CARTESIAN_POINT('Ctrl Pts',(-7.52427261074264,-21.266305915706,
12.));
#228198=CARTESIAN_POINT('Ctrl Pts',(-7.52501770333522,-21.2685823838672,
12.));
#228199=CARTESIAN_POINT('Ctrl Pts',(-7.52587126095544,-21.2712301573465,
12.));
#228200=CARTESIAN_POINT('Ctrl Pts',(-7.52682526918561,-21.2742366113578,
12.));
#228201=CARTESIAN_POINT('Ctrl Pts',(-7.52787386225344,-21.2775925269651,
12.));
#228202=CARTESIAN_POINT('Ctrl Pts',(-7.52901217930407,-21.2812902781143,
12.));
#228203=CARTESIAN_POINT('Ctrl Pts',(-7.53023562438221,-21.2853226580658,
12.));
#228204=CARTESIAN_POINT('Ctrl Pts',(-7.53153906987847,-21.2896816163843,
12.));
#228205=CARTESIAN_POINT('Ctrl Pts',(-7.53291726078527,-21.2943588989331,
12.));
#228206=CARTESIAN_POINT('Ctrl Pts',(-7.53436505309949,-21.2993464250717,
12.));
#228207=CARTESIAN_POINT('Ctrl Pts',(-7.53587778251743,-21.3046368712156,
12.));
#228208=CARTESIAN_POINT('Ctrl Pts',(-7.5374512936462,-21.3102237167729,
12.));
#228209=CARTESIAN_POINT('Ctrl Pts',(-7.53908175169899,-21.3161009456256,
12.));
#228210=CARTESIAN_POINT('Ctrl Pts',(-7.5407655203828,-21.3222628524165,
12.));
#228211=CARTESIAN_POINT('Ctrl Pts',(-7.54249900377032,-21.328703791771,
12.));
#228212=CARTESIAN_POINT('Ctrl Pts',(-7.54427868151269,-21.3354182340149,
12.));
#228213=CARTESIAN_POINT('Ctrl Pts',(-7.54610114948351,-21.3424008295038,
12.));
#228214=CARTESIAN_POINT('Ctrl Pts',(-7.54796316246327,-21.349646476153,
12.));
#228215=CARTESIAN_POINT('Ctrl Pts',(-7.54986166521307,-21.3571503685853,
12.));
#228216=CARTESIAN_POINT('Ctrl Pts',(-7.55179375777442,-21.3649079431864,
12.));
#228217=CARTESIAN_POINT('Ctrl Pts',(-7.55375667080032,-21.3729148390244,
12.));
#228218=CARTESIAN_POINT('Ctrl Pts',(-7.55574773403508,-21.3811668478933,
12.));
#228219=CARTESIAN_POINT('Ctrl Pts',(-7.55776435731422,-21.3896598842119,
12.));
#228220=CARTESIAN_POINT('Ctrl Pts',(-7.55980403700615,-21.3983899952988,
12.));
#228221=CARTESIAN_POINT('Ctrl Pts',(-7.56186435703622,-21.4073533630364,
12.));
#228222=CARTESIAN_POINT('Ctrl Pts',(-7.56394299313683,-21.4165463106252,
12.));
#228223=CARTESIAN_POINT('Ctrl Pts',(-7.56603771218706,-21.4259653015732,
12.));
#228224=CARTESIAN_POINT('Ctrl Pts',(-7.56814636360842,-21.435606926151,
12.));
#228225=CARTESIAN_POINT('Ctrl Pts',(-7.5702668726117,-21.445467890751,12.));
#228226=CARTESIAN_POINT('Ctrl Pts',(-7.57239723223521,-21.4555450053147,
12.));
#228227=CARTESIAN_POINT('Ctrl Pts',(-7.57453549743435,-21.4658351740135,
12.));
#228228=CARTESIAN_POINT('Ctrl Pts',(-7.57667978403003,-21.4763353936766,
12.));
#228229=CARTESIAN_POINT('Ctrl Pts',(-7.57882826679131,-21.4870427508193,
12.));
#228230=CARTESIAN_POINT('Ctrl Pts',(-7.5809791779073,-21.4979544192739,
12.));
#228231=CARTESIAN_POINT('Ctrl Pts',(-7.58313080519159,-21.5090676573866,
12.));
#228232=CARTESIAN_POINT('Ctrl Pts',(-7.58528148919114,-21.5203798035294,
12.));
#228233=CARTESIAN_POINT('Ctrl Pts',(-7.58742962034834,-21.5318882716735,
12.));
#228234=CARTESIAN_POINT('Ctrl Pts',(-7.58957363620026,-21.5435905470113,
12.));
#228235=CARTESIAN_POINT('Ctrl Pts',(-7.59171201844793,-21.5554841813465,
12.));
#228236=CARTESIAN_POINT('Ctrl Pts',(-7.5938432912493,-21.5675667904728,
12.));
#228237=CARTESIAN_POINT('Ctrl Pts',(-7.59596601973589,-21.5798360518978,
12.));
#228238=CARTESIAN_POINT('Ctrl Pts',(-7.59807880846193,-21.5922897024466,
12.));
#228239=CARTESIAN_POINT('Ctrl Pts',(-7.60018029988238,-21.6049255358842,
12.));
#228240=CARTESIAN_POINT('Ctrl Pts',(-7.60226917285432,-21.6177414005991,
12.));
#228241=CARTESIAN_POINT('Ctrl Pts',(-7.604344141183,-21.6307351973823,12.));
#228242=CARTESIAN_POINT('Ctrl Pts',(-7.60640395216359,-21.6439048771743,
12.));
#228243=CARTESIAN_POINT('Ctrl Pts',(-7.60844738512872,-21.6572484388079,
12.));
#228244=CARTESIAN_POINT('Ctrl Pts',(-7.6104732500095,-21.6707639267573,
12.));
#228245=CARTESIAN_POINT('Ctrl Pts',(-7.61248038630265,-21.6844494295813,
12.));
#228246=CARTESIAN_POINT('Ctrl Pts',(-7.61446766202787,-21.6983030783321,
12.));
#228247=CARTESIAN_POINT('Ctrl Pts',(-7.61643397270425,-21.7123230449835,
12.));
#228248=CARTESIAN_POINT('Ctrl Pts',(-7.61837824030542,-21.7265075407977,
12.));
#228249=CARTESIAN_POINT('Ctrl Pts',(-7.62029941230855,-21.7408548148657,
12.));
#228250=CARTESIAN_POINT('Ctrl Pts',(-7.62219646084226,-21.7553631528329,
12.));
#228251=CARTESIAN_POINT('Ctrl Pts',(-7.62406838181164,-21.7700308755583,
12.));
#228252=CARTESIAN_POINT('Ctrl Pts',(-7.62591419404521,-21.7848563378022,
12.));
#228253=CARTESIAN_POINT('Ctrl Pts',(-7.62773293842409,-21.7998379268583,
12.));
#228254=CARTESIAN_POINT('Ctrl Pts',(-7.62952367718151,-21.8149740615093,
12.));
#228255=CARTESIAN_POINT('Ctrl Pts',(-7.6312854932304,-21.8302631910197,
12.));
#228256=CARTESIAN_POINT('Ctrl Pts',(-7.63301748948936,-21.8457037941084,
12.));
#228257=CARTESIAN_POINT('Ctrl Pts',(-7.63471878821204,-21.8612943779086,
12.));
#228258=CARTESIAN_POINT('Ctrl Pts',(-7.63638853033368,-21.8770334769492,
12.));
#228259=CARTESIAN_POINT('Ctrl Pts',(-7.63802587492008,-21.8929196523511,
12.));
#228260=CARTESIAN_POINT('Ctrl Pts',(-7.63962999860917,-21.9089514909873,
12.));
#228261=CARTESIAN_POINT('Ctrl Pts',(-7.6412000950654,-21.9251276046546,
12.));
#228262=CARTESIAN_POINT('Ctrl Pts',(-7.64273537442707,-21.9414466292074,
12.));
#228263=CARTESIAN_POINT('Ctrl Pts',(-7.64423506279154,-21.9579072237653,
12.));
#228264=CARTESIAN_POINT('Ctrl Pts',(-7.64569840177359,-21.97450807008,12.));
#228265=CARTESIAN_POINT('Ctrl Pts',(-7.64712464805258,-21.9912478718542,
12.));
#228266=CARTESIAN_POINT('Ctrl Pts',(-7.64851307293346,-22.0081253540773,
12.));
#228267=CARTESIAN_POINT('Ctrl Pts',(-7.64986296190157,-22.0251392623209,
12.));
#228268=CARTESIAN_POINT('Ctrl Pts',(-7.65117361421347,-22.0422883621176,
12.));
#228269=CARTESIAN_POINT('Ctrl Pts',(-7.65244434253104,-22.0595714384432,
12.));
#228270=CARTESIAN_POINT('Ctrl Pts',(-7.65367447254945,-22.0769872951596,
12.));
#228271=CARTESIAN_POINT('Ctrl Pts',(-7.65486334263651,-22.094534754469,
12.));
#228272=CARTESIAN_POINT('Ctrl Pts',(-7.65601030346819,-22.1122126563327,
12.));
#228273=CARTESIAN_POINT('Ctrl Pts',(-7.65711471769407,-22.1300198579671,
12.));
#228274=CARTESIAN_POINT('Ctrl Pts',(-7.65817595963351,-22.1479552334206,
12.));
#228275=CARTESIAN_POINT('Ctrl Pts',(-7.65919341496926,-22.1660176731174,
12.));
#228276=CARTESIAN_POINT('Ctrl Pts',(-7.66016648045008,-22.1842060834092,
12.));
#228277=CARTESIAN_POINT('Ctrl Pts',(-7.66109456359292,-22.2025193860972,
12.));
#228278=CARTESIAN_POINT('Ctrl Pts',(-7.66197708240436,-22.2209565180098,
12.));
#228279=CARTESIAN_POINT('Ctrl Pts',(-7.66281346512546,-22.239516430656,
12.));
#228280=CARTESIAN_POINT('Ctrl Pts',(-7.66360314997662,-22.2581980898487,
12.));
#228281=CARTESIAN_POINT('Ctrl Pts',(-7.66434558490973,-22.2770004753332,
12.));
#228282=CARTESIAN_POINT('Ctrl Pts',(-7.66504022736263,-22.2959225803925,
12.));
#228283=CARTESIAN_POINT('Ctrl Pts',(-7.66568654402442,-22.3149634114823,
12.));
#228284=CARTESIAN_POINT('Ctrl Pts',(-7.66628401061906,-22.3341219879454,
12.));
#228285=CARTESIAN_POINT('Ctrl Pts',(-7.66683211169134,-22.3533973417013,
12.));
#228286=CARTESIAN_POINT('Ctrl Pts',(-7.66733034039887,-22.3727885169361,
12.));
#228287=CARTESIAN_POINT('Ctrl Pts',(-7.6677781983082,-22.3922945697782,
12.));
#228288=CARTESIAN_POINT('Ctrl Pts',(-7.66817519519682,-22.411914567977,
12.));
#228289=CARTESIAN_POINT('Ctrl Pts',(-7.66852084886746,-22.4316475906616,
12.));
#228290=CARTESIAN_POINT('Ctrl Pts',(-7.6688146849666,-22.4514927280862,
12.));
#228291=CARTESIAN_POINT('Ctrl Pts',(-7.66905623680836,-22.47144908137,12.));
#228292=CARTESIAN_POINT('Ctrl Pts',(-7.66924504520302,-22.4915157622308,
12.));
#228293=CARTESIAN_POINT('Ctrl Pts',(-7.66938065829083,-22.5116918927023,
12.));
#228294=CARTESIAN_POINT('Ctrl Pts',(-7.66946263138116,-22.5319766049191,
12.));
#228295=CARTESIAN_POINT('Ctrl Pts',(-7.66949052679672,-22.5523690409109,
12.));
#228296=CARTESIAN_POINT('Ctrl Pts',(-7.66946391372299,-22.5728683523828,
12.));
#228297=CARTESIAN_POINT('Ctrl Pts',(-7.66938236806241,-22.5934737004955,
12.));
#228298=CARTESIAN_POINT('Ctrl Pts',(-7.66924547229435,-22.6141842556248,
12.));
#228299=CARTESIAN_POINT('Ctrl Pts',(-7.66905281533745,-22.6349991971547,
12.));
#228300=CARTESIAN_POINT('Ctrl Pts',(-7.66880399241354,-22.6559177133133,
12.));
#228301=CARTESIAN_POINT('Ctrl Pts',(-7.66849860491763,-22.6769390009889,
12.));
#228302=CARTESIAN_POINT('Ctrl Pts',(-7.66813626029277,-22.6980622655446,
12.));
#228303=CARTESIAN_POINT('Ctrl Pts',(-7.6677165719101,-22.7192867206242,
12.));
#228304=CARTESIAN_POINT('Ctrl Pts',(-7.66723915895413,-22.7406115879508,
12.));
#228305=CARTESIAN_POINT('Ctrl Pts',(-7.66670364630273,-22.7620360971839,
12.));
#228306=CARTESIAN_POINT('Ctrl Pts',(-7.66610966441259,-22.7835594857697,
12.));
#228307=CARTESIAN_POINT('Ctrl Pts',(-7.66545684920988,-22.8051809987833,
12.));
#228308=CARTESIAN_POINT('Ctrl Pts',(-7.66474484198553,-22.8268998887678,
12.));
#228309=CARTESIAN_POINT('Ctrl Pts',(-7.66397328929805,-22.8487154155569,
12.));
#228310=CARTESIAN_POINT('Ctrl Pts',(-7.66314184287334,-22.870626846128,
12.));
#228311=CARTESIAN_POINT('Ctrl Pts',(-7.66225015950148,-22.8926334544879,
12.));
#228312=CARTESIAN_POINT('Ctrl Pts',(-7.661297900941,-22.9147345215418,12.));
#228313=CARTESIAN_POINT('Ctrl Pts',(-7.66028473382777,-22.9369293349592,
12.));
#228314=CARTESIAN_POINT('Ctrl Pts',(-7.65921032958912,-22.9592171890332,
12.));
#228315=CARTESIAN_POINT('Ctrl Pts',(-7.65807436436453,-22.9815973845301,
12.));
#228316=CARTESIAN_POINT('Ctrl Pts',(-7.6568765189133,-23.004069228582,12.));
#228317=CARTESIAN_POINT('Ctrl Pts',(-7.65561647852555,-23.0266320345792,
12.));
#228318=CARTESIAN_POINT('Ctrl Pts',(-7.65429393293955,-23.049285122053,
12.));
#228319=CARTESIAN_POINT('Ctrl Pts',(-7.65290857626357,-23.072027816555,
12.));
#228320=CARTESIAN_POINT('Ctrl Pts',(-7.65146010690465,-23.0948594495246,
12.));
#228321=CARTESIAN_POINT('Ctrl Pts',(-7.64994822749845,-23.1177793581674,
12.));
#228322=CARTESIAN_POINT('Ctrl Pts',(-7.64837264482929,-23.1407868853815,
12.));
#228323=CARTESIAN_POINT('Ctrl Pts',(-7.64673306975797,-23.1638813796691,
12.));
#228324=CARTESIAN_POINT('Ctrl Pts',(-7.64502921715483,-23.1870621950452,
12.));
#228325=CARTESIAN_POINT('Ctrl Pts',(-7.64326080583684,-23.2103286909399,
12.));
#228326=CARTESIAN_POINT('Ctrl Pts',(-7.64142755851508,-23.2336802320912,
12.));
#228327=CARTESIAN_POINT('Ctrl Pts',(-7.63952920172837,-23.2571161884487,
12.));
#228328=CARTESIAN_POINT('Ctrl Pts',(-7.63756546576375,-23.2806359350853,
12.));
#228329=CARTESIAN_POINT('Ctrl Pts',(-7.63553608458784,-23.3042388521021,
12.));
#228330=CARTESIAN_POINT('Ctrl Pts',(-7.63344079578163,-23.3279243245241,
12.));
#228331=CARTESIAN_POINT('Ctrl Pts',(-7.63127934048139,-23.3516917421973,
12.));
#228332=CARTESIAN_POINT('Ctrl Pts',(-7.62905146332598,-23.3755404996638,
12.));
#228333=CARTESIAN_POINT('Ctrl Pts',(-7.62675691240335,-23.3994699961122,
12.));
#228334=CARTESIAN_POINT('Ctrl Pts',(-7.62439543920055,-23.4234796353544,
12.));
#228335=CARTESIAN_POINT('Ctrl Pts',(-7.62196679855957,-23.4475688257854,
12.));
#228336=CARTESIAN_POINT('Ctrl Pts',(-7.61947074863978,-23.4717369803438,
12.));
#228337=CARTESIAN_POINT('Ctrl Pts',(-7.61690705088319,-23.4959835164608,
12.));
#228338=CARTESIAN_POINT('Ctrl Pts',(-7.61427546999299,-23.5203078560128,
12.));
#228339=CARTESIAN_POINT('Ctrl Pts',(-7.61157577385372,-23.5447094252028,
12.));
#228340=CARTESIAN_POINT('Ctrl Pts',(-7.608807733446,-23.5691876544243,12.));
#228341=CARTESIAN_POINT('Ctrl Pts',(-7.60597112277094,-23.5937419781244,
12.));
#228342=CARTESIAN_POINT('Ctrl Pts',(-7.60306571877806,-23.6183718346576,
12.));
#228343=CARTESIAN_POINT('Ctrl Pts',(-7.6000913013013,-23.6430766661419,
12.));
#228344=CARTESIAN_POINT('Ctrl Pts',(-7.59704765299572,-23.6678559182876,
12.));
#228345=CARTESIAN_POINT('Ctrl Pts',(-7.59393455934042,-23.6927090405067,
12.));
#228346=CARTESIAN_POINT('Ctrl Pts',(-7.59075180865327,-23.7176354860457,
12.));
#228347=CARTESIAN_POINT('Ctrl Pts',(-7.58749919210832,-23.7426347121006,
12.));
#228348=CARTESIAN_POINT('Ctrl Pts',(-7.58417650376272,-23.7677061799376,
12.));
#228349=CARTESIAN_POINT('Ctrl Pts',(-7.58078354058212,-23.7928493549908,
12.));
#228350=CARTESIAN_POINT('Ctrl Pts',(-7.57732010249066,-23.8180637069977,
12.));
#228351=CARTESIAN_POINT('Ctrl Pts',(-7.57378599219817,-23.8433487096134,
12.));
#228352=CARTESIAN_POINT('Ctrl Pts',(-7.57018101500711,-23.8687038399597,
12.));
#228353=CARTESIAN_POINT('Ctrl Pts',(-7.56650497863792,-23.8941285782003,
12.));
#228354=CARTESIAN_POINT('Ctrl Pts',(-7.56275769304773,-23.9196224070759,
12.));
#228355=CARTESIAN_POINT('Ctrl Pts',(-7.55893897027683,-23.9451848115,12.));
#228356=CARTESIAN_POINT('Ctrl Pts',(-7.55504862424812,-23.9708152779884,
12.));
#228357=CARTESIAN_POINT('Ctrl Pts',(-7.55108647097441,-23.9965132953185,
12.));
#228358=CARTESIAN_POINT('Ctrl Pts',(-7.5470523288591,-24.022278355453,12.));
#228359=CARTESIAN_POINT('Ctrl Pts',(-7.54294601896145,-24.0481099543353,
12.));
#228360=CARTESIAN_POINT('Ctrl Pts',(-7.53876736531014,-24.0740075927985,
12.));
#228361=CARTESIAN_POINT('Ctrl Pts',(-7.53451619514649,-24.0999707772642,
12.));
#228362=CARTESIAN_POINT('Ctrl Pts',(-7.53019233935502,-24.1259990209207,
12.));
#228363=CARTESIAN_POINT('Ctrl Pts',(-7.52579563201424,-24.1520918425364,
12.));
#228364=CARTESIAN_POINT('Ctrl Pts',(-7.52132590953802,-24.1782487641594,
12.));
#228365=CARTESIAN_POINT('Ctrl Pts',(-7.51678300997949,-24.2044693092349,
12.));
#228366=CARTESIAN_POINT('Ctrl Pts',(-7.51216677222181,-24.2307530003887,
12.));
#228367=CARTESIAN_POINT('Ctrl Pts',(-7.50747703535134,-24.2570993577034,
12.));
#228368=CARTESIAN_POINT('Ctrl Pts',(-7.50271363765152,-24.2835078958973,
12.));
#228369=CARTESIAN_POINT('Ctrl Pts',(-7.49787641695439,-24.3099781253355,
12.));
#228370=CARTESIAN_POINT('Ctrl Pts',(-7.49296521252421,-24.3365095573685,
12.));
#228371=CARTESIAN_POINT('Ctrl Pts',(-7.48797986651909,-24.3631017084524,
12.));
#228372=CARTESIAN_POINT('Ctrl Pts',(-7.48292022569301,-24.3897541049254,
12.));
#228373=CARTESIAN_POINT('Ctrl Pts',(-7.47778614286565,-24.4164662871163,
12.));
#228374=CARTESIAN_POINT('Ctrl Pts',(-7.47257747883246,-24.443237814649,
12.));
#228375=CARTESIAN_POINT('Ctrl Pts',(-7.46729410308787,-24.4700682684524,
12.));
#228376=CARTESIAN_POINT('Ctrl Pts',(-7.46193588961464,-24.4969572391483,
12.));
#228377=CARTESIAN_POINT('Ctrl Pts',(-7.45650271335862,-24.5239043173072,
12.));
#228378=CARTESIAN_POINT('Ctrl Pts',(-7.4509944465116,-24.5509090831559,
12.));
#228379=CARTESIAN_POINT('Ctrl Pts',(-7.44541095473135,-24.577971096086,
12.));
#228380=CARTESIAN_POINT('Ctrl Pts',(-7.43975209375504,-24.6050898852368,
12.));
#228381=CARTESIAN_POINT('Ctrl Pts',(-7.43401770489524,-24.6322649369517,
12.));
#228382=CARTESIAN_POINT('Ctrl Pts',(-7.42820762159126,-24.6594957128756,
12.));
#228383=CARTESIAN_POINT('Ctrl Pts',(-7.42232167766266,-24.6867816727192,
12.));
#228384=CARTESIAN_POINT('Ctrl Pts',(-7.41635971481674,-24.7141222950051,
12.));
#228385=CARTESIAN_POINT('Ctrl Pts',(-7.41032159082382,-24.7415170994784,
12.));
#228386=CARTESIAN_POINT('Ctrl Pts',(-7.40420718661603,-24.7689656668983,
12.));
#228387=CARTESIAN_POINT('Ctrl Pts',(-7.39801641583013,-24.7964676646431,
12.));
#228388=CARTESIAN_POINT('Ctrl Pts',(-7.39174922585809,-24.8240228520893,
12.));
#228389=CARTESIAN_POINT('Ctrl Pts',(-7.38540558903621,-24.8516310625176,
12.));
#228390=CARTESIAN_POINT('Ctrl Pts',(-7.3789854964027,-24.8792921911115,
12.));
#228391=CARTESIAN_POINT('Ctrl Pts',(-7.37378825961676,-24.901463382605,
12.));
#228392=CARTESIAN_POINT('Ctrl Pts',(-7.36985593120091,-24.9181155530543,
12.));
#228393=CARTESIAN_POINT('Ctrl Pts',(-7.36721909028843,-24.9292275670674,
12.));
#228394=CARTESIAN_POINT('Ctrl Pts',(-7.36589684767345,-24.9347862158358,
12.));
#228395=CARTESIAN_POINT('Ctrl Pts',(-9.71462809124917,-20.353053841303,
0.));
#228396=CARTESIAN_POINT('Ctrl Pts',(-9.71462809124917,-20.353053841303,
12.));
#228397=CARTESIAN_POINT('Ctrl Pts',(-9.71462954053074,-20.353060251684,
0.));
#228398=CARTESIAN_POINT('Ctrl Pts',(-9.71462954053074,-20.353060251684,
12.));
#228399=CARTESIAN_POINT('Ctrl Pts',(-9.71465227853122,-20.3531126095522,
0.));
#228400=CARTESIAN_POINT('Ctrl Pts',(-9.71465227853122,-20.3531126095522,
12.));
#228401=CARTESIAN_POINT('Ctrl Pts',(-9.71474590350792,-20.3533097561886,
0.));
#228402=CARTESIAN_POINT('Ctrl Pts',(-9.71474590350792,-20.3533097561886,
12.));
#228403=CARTESIAN_POINT('Ctrl Pts',(-9.71498978052101,-20.3538098605706,
0.));
#228404=CARTESIAN_POINT('Ctrl Pts',(-9.71498978052101,-20.3538098605706,
12.));
#228405=CARTESIAN_POINT('Ctrl Pts',(-9.71549257088175,-20.3548282742361,
0.));
#228406=CARTESIAN_POINT('Ctrl Pts',(-9.71549257088175,-20.3548282742361,
12.));
#228407=CARTESIAN_POINT('Ctrl Pts',(-9.71619192554147,-20.3562337557875,
0.));
#228408=CARTESIAN_POINT('Ctrl Pts',(-9.71619192554147,-20.3562337557875,
12.));
#228409=CARTESIAN_POINT('Ctrl Pts',(-9.71708493723062,-20.3580133103357,
0.));
#228410=CARTESIAN_POINT('Ctrl Pts',(-9.71708493723062,-20.3580133103357,
12.));
#228411=CARTESIAN_POINT('Ctrl Pts',(-9.71816778327999,-20.3601498764344,
0.));
#228412=CARTESIAN_POINT('Ctrl Pts',(-9.71816778327999,-20.3601498764344,
12.));
#228413=CARTESIAN_POINT('Ctrl Pts',(-9.71943648548115,-20.362625691398,
0.));
#228414=CARTESIAN_POINT('Ctrl Pts',(-9.71943648548115,-20.362625691398,
12.));
#228415=CARTESIAN_POINT('Ctrl Pts',(-9.72088778381102,-20.3654261611055,
0.));
#228416=CARTESIAN_POINT('Ctrl Pts',(-9.72088778381102,-20.3654261611055,
12.));
#228417=CARTESIAN_POINT('Ctrl Pts',(-9.72251930722504,-20.3685406190576,
0.));
#228418=CARTESIAN_POINT('Ctrl Pts',(-9.72251930722504,-20.3685406190576,
12.));
#228419=CARTESIAN_POINT('Ctrl Pts',(-9.72432910043193,-20.371960235676,
0.));
#228420=CARTESIAN_POINT('Ctrl Pts',(-9.72432910043193,-20.371960235676,
12.));
#228421=CARTESIAN_POINT('Ctrl Pts',(-9.72631531732871,-20.3756766651952,
0.));
#228422=CARTESIAN_POINT('Ctrl Pts',(-9.72631531732871,-20.3756766651952,
12.));
#228423=CARTESIAN_POINT('Ctrl Pts',(-9.72847589116533,-20.3796805893304,
0.));
#228424=CARTESIAN_POINT('Ctrl Pts',(-9.72847589116533,-20.3796805893304,
12.));
#228425=CARTESIAN_POINT('Ctrl Pts',(-9.73080870123726,-20.3839624556742,
0.));
#228426=CARTESIAN_POINT('Ctrl Pts',(-9.73080870123726,-20.3839624556742,
12.));
#228427=CARTESIAN_POINT('Ctrl Pts',(-9.73331167102812,-20.3885129129912,
0.));
#228428=CARTESIAN_POINT('Ctrl Pts',(-9.73331167102812,-20.3885129129912,
12.));
#228429=CARTESIAN_POINT('Ctrl Pts',(-9.7359829201425,-20.3933234845646,
0.));
#228430=CARTESIAN_POINT('Ctrl Pts',(-9.7359829201425,-20.3933234845646,
12.));
#228431=CARTESIAN_POINT('Ctrl Pts',(-9.73882077613206,-20.3983866213331,
0.));
#228432=CARTESIAN_POINT('Ctrl Pts',(-9.73882077613206,-20.3983866213331,
12.));
#228433=CARTESIAN_POINT('Ctrl Pts',(-9.74182369656273,-20.4036953576549,
0.));
#228434=CARTESIAN_POINT('Ctrl Pts',(-9.74182369656273,-20.4036953576549,
12.));
#228435=CARTESIAN_POINT('Ctrl Pts',(-9.74499021838537,-20.4092430879861,
0.));
#228436=CARTESIAN_POINT('Ctrl Pts',(-9.74499021838537,-20.4092430879861,
12.));
#228437=CARTESIAN_POINT('Ctrl Pts',(-9.74831889242175,-20.4150232777393,
0.));
#228438=CARTESIAN_POINT('Ctrl Pts',(-9.74831889242175,-20.4150232777393,
12.));
#228439=CARTESIAN_POINT('Ctrl Pts',(-9.75180829786433,-20.4210295275818,
0.));
#228440=CARTESIAN_POINT('Ctrl Pts',(-9.75180829786433,-20.4210295275818,
12.));
#228441=CARTESIAN_POINT('Ctrl Pts',(-9.75545705902416,-20.4272556476629,
0.));
#228442=CARTESIAN_POINT('Ctrl Pts',(-9.75545705902416,-20.4272556476629,
12.));
#228443=CARTESIAN_POINT('Ctrl Pts',(-9.7592638628993,-20.4336957355474,
0.));
#228444=CARTESIAN_POINT('Ctrl Pts',(-9.7592638628993,-20.4336957355474,
12.));
#228445=CARTESIAN_POINT('Ctrl Pts',(-9.76322747195502,-20.4403442329401,
0.));
#228446=CARTESIAN_POINT('Ctrl Pts',(-9.76322747195502,-20.4403442329401,
12.));
#228447=CARTESIAN_POINT('Ctrl Pts',(-9.76734670980897,-20.447195862298,
0.));
#228448=CARTESIAN_POINT('Ctrl Pts',(-9.76734670980897,-20.447195862298,
12.));
#228449=CARTESIAN_POINT('Ctrl Pts',(-9.7716204510407,-20.4542455817527,
0.));
#228450=CARTESIAN_POINT('Ctrl Pts',(-9.7716204510407,-20.4542455817527,
12.));
#228451=CARTESIAN_POINT('Ctrl Pts',(-9.77604760815523,-20.4614885274973,
0.));
#228452=CARTESIAN_POINT('Ctrl Pts',(-9.77604760815523,-20.4614885274973,
12.));
#228453=CARTESIAN_POINT('Ctrl Pts',(-9.78062712373313,-20.4689199790668,
0.));
#228454=CARTESIAN_POINT('Ctrl Pts',(-9.78062712373313,-20.4689199790668,
12.));
#228455=CARTESIAN_POINT('Ctrl Pts',(-9.78535797314162,-20.4765353711585,
0.));
#228456=CARTESIAN_POINT('Ctrl Pts',(-9.78535797314162,-20.4765353711585,
12.));
#228457=CARTESIAN_POINT('Ctrl Pts',(-9.7902391649866,-20.4843302955329,
0.));
#228458=CARTESIAN_POINT('Ctrl Pts',(-9.7902391649866,-20.4843302955329,
12.));
#228459=CARTESIAN_POINT('Ctrl Pts',(-9.79526974288344,-20.4923005087945,
0.));
#228460=CARTESIAN_POINT('Ctrl Pts',(-9.79526974288344,-20.4923005087945,
12.));
#228461=CARTESIAN_POINT('Ctrl Pts',(-9.80044878520968,-20.500441931211,
0.));
#228462=CARTESIAN_POINT('Ctrl Pts',(-9.80044878520968,-20.500441931211,
12.));
#228463=CARTESIAN_POINT('Ctrl Pts',(-9.80577540161103,-20.5087506310507,
0.));
#228464=CARTESIAN_POINT('Ctrl Pts',(-9.80577540161103,-20.5087506310507,
12.));
#228465=CARTESIAN_POINT('Ctrl Pts',(-9.81124873025278,-20.5172228122839,
0.));
#228466=CARTESIAN_POINT('Ctrl Pts',(-9.81124873025278,-20.5172228122839,
12.));
#228467=CARTESIAN_POINT('Ctrl Pts',(-9.81686793455918,-20.5258548000625,
0.));
#228468=CARTESIAN_POINT('Ctrl Pts',(-9.81686793455918,-20.5258548000625,
12.));
#228469=CARTESIAN_POINT('Ctrl Pts',(-9.82263220080328,-20.534643029951,
0.));
#228470=CARTESIAN_POINT('Ctrl Pts',(-9.82263220080328,-20.534643029951,
12.));
#228471=CARTESIAN_POINT('Ctrl Pts',(-9.82854073773858,-20.5435840460717,
0.));
#228472=CARTESIAN_POINT('Ctrl Pts',(-9.82854073773858,-20.5435840460717,
12.));
#228473=CARTESIAN_POINT('Ctrl Pts',(-9.83459277585321,-20.5526744976461,
0.));
#228474=CARTESIAN_POINT('Ctrl Pts',(-9.83459277585321,-20.5526744976461,
12.));
#228475=CARTESIAN_POINT('Ctrl Pts',(-9.84078756677589,-20.5619111362406,
0.));
#228476=CARTESIAN_POINT('Ctrl Pts',(-9.84078756677589,-20.5619111362406,
12.));
#228477=CARTESIAN_POINT('Ctrl Pts',(-9.84712438256308,-20.5712908125145,
0.));
#228478=CARTESIAN_POINT('Ctrl Pts',(-9.84712438256308,-20.5712908125145,
12.));
#228479=CARTESIAN_POINT('Ctrl Pts',(-9.85360251457004,-20.580810471002,
0.));
#228480=CARTESIAN_POINT('Ctrl Pts',(-9.85360251457004,-20.580810471002,
12.));
#228481=CARTESIAN_POINT('Ctrl Pts',(-9.8602212723275,-20.5904671449754,
0.));
#228482=CARTESIAN_POINT('Ctrl Pts',(-9.8602212723275,-20.5904671449754,
12.));
#228483=CARTESIAN_POINT('Ctrl Pts',(-9.86697998242612,-20.6002579513696,
0.));
#228484=CARTESIAN_POINT('Ctrl Pts',(-9.86697998242612,-20.6002579513696,
12.));
#228485=CARTESIAN_POINT('Ctrl Pts',(-9.87387798732944,-20.6101800854491,
0.));
#228486=CARTESIAN_POINT('Ctrl Pts',(-9.87387798732944,-20.6101800854491,
12.));
#228487=CARTESIAN_POINT('Ctrl Pts',(-9.88091464472669,-20.6202308177472,
0.));
#228488=CARTESIAN_POINT('Ctrl Pts',(-9.88091464472669,-20.6202308177472,
12.));
#228489=CARTESIAN_POINT('Ctrl Pts',(-9.88808932697305,-20.6304074914086,
0.));
#228490=CARTESIAN_POINT('Ctrl Pts',(-9.88808932697305,-20.6304074914086,
12.));
#228491=CARTESIAN_POINT('Ctrl Pts',(-9.89540142049124,-20.6407075193977,
0.));
#228492=CARTESIAN_POINT('Ctrl Pts',(-9.89540142049124,-20.6407075193977,
12.));
#228493=CARTESIAN_POINT('Ctrl Pts',(-9.90285032516696,-20.6511283817415,
0.));
#228494=CARTESIAN_POINT('Ctrl Pts',(-9.90285032516696,-20.6511283817415,
12.));
#228495=CARTESIAN_POINT('Ctrl Pts',(-9.91043545377005,-20.6616676228315,
0.));
#228496=CARTESIAN_POINT('Ctrl Pts',(-9.91043545377005,-20.6616676228315,
12.));
#228497=CARTESIAN_POINT('Ctrl Pts',(-9.91815623141285,-20.6723228488261,
0.));
#228498=CARTESIAN_POINT('Ctrl Pts',(-9.91815623141285,-20.6723228488261,
12.));
#228499=CARTESIAN_POINT('Ctrl Pts',(-9.92601209498751,-20.6830917250255,
0.));
#228500=CARTESIAN_POINT('Ctrl Pts',(-9.92601209498751,-20.6830917250255,
12.));
#228501=CARTESIAN_POINT('Ctrl Pts',(-9.93400249259737,-20.6939719732485,
0.));
#228502=CARTESIAN_POINT('Ctrl Pts',(-9.93400249259737,-20.6939719732485,
12.));
#228503=CARTESIAN_POINT('Ctrl Pts',(-9.94212688298251,-20.7049613692237,
0.));
#228504=CARTESIAN_POINT('Ctrl Pts',(-9.94212688298251,-20.7049613692237,
12.));
#228505=CARTESIAN_POINT('Ctrl Pts',(-9.95038473514962,-20.716057740758,
0.));
#228506=CARTESIAN_POINT('Ctrl Pts',(-9.95038473514962,-20.716057740758,
12.));
#228507=CARTESIAN_POINT('Ctrl Pts',(-9.95877552798403,-20.7272589658752,
0.));
#228508=CARTESIAN_POINT('Ctrl Pts',(-9.95877552798403,-20.7272589658752,
12.));
#228509=CARTESIAN_POINT('Ctrl Pts',(-9.96729874986199,-20.7385629709795,
0.));
#228510=CARTESIAN_POINT('Ctrl Pts',(-9.96729874986199,-20.7385629709795,
12.));
#228511=CARTESIAN_POINT('Ctrl Pts',(-9.97595389823461,-20.7499677289625,
0.));
#228512=CARTESIAN_POINT('Ctrl Pts',(-9.97595389823461,-20.7499677289625,
12.));
#228513=CARTESIAN_POINT('Ctrl Pts',(-9.98474047926846,-20.7614712574989,
0.));
#228514=CARTESIAN_POINT('Ctrl Pts',(-9.98474047926846,-20.7614712574989,
12.));
#228515=CARTESIAN_POINT('Ctrl Pts',(-9.99365800754638,-20.7730716175417,
0.));
#228516=CARTESIAN_POINT('Ctrl Pts',(-9.99365800754638,-20.7730716175417,
12.));
#228517=CARTESIAN_POINT('Ctrl Pts',(-10.0027060057389,-20.7847669117568,
0.));
#228518=CARTESIAN_POINT('Ctrl Pts',(-10.0027060057389,-20.7847669117568,
12.));
#228519=CARTESIAN_POINT('Ctrl Pts',(-10.0118840042786,-20.7965552829907,
0.));
#228520=CARTESIAN_POINT('Ctrl Pts',(-10.0118840042786,-20.7965552829907,
12.));
#228521=CARTESIAN_POINT('Ctrl Pts',(-10.0211915410095,-20.8084349126885,
0.));
#228522=CARTESIAN_POINT('Ctrl Pts',(-10.0211915410095,-20.8084349126885,
12.));
#228523=CARTESIAN_POINT('Ctrl Pts',(-10.0306281609435,-20.8204040196599,
0.));
#228524=CARTESIAN_POINT('Ctrl Pts',(-10.0306281609435,-20.8204040196599,
12.));
#228525=CARTESIAN_POINT('Ctrl Pts',(-10.0401934160234,-20.8324608588906,
0.));
#228526=CARTESIAN_POINT('Ctrl Pts',(-10.0401934160234,-20.8324608588906,
12.));
#228527=CARTESIAN_POINT('Ctrl Pts',(-10.0498868648733,-20.8446037203402,
0.));
#228528=CARTESIAN_POINT('Ctrl Pts',(-10.0498868648733,-20.8446037203402,
12.));
#228529=CARTESIAN_POINT('Ctrl Pts',(-10.0597080725375,-20.856830927732,
0.));
#228530=CARTESIAN_POINT('Ctrl Pts',(-10.0597080725375,-20.856830927732,
12.));
#228531=CARTESIAN_POINT('Ctrl Pts',(-10.0696566102219,-20.8691408373705,
0.));
#228532=CARTESIAN_POINT('Ctrl Pts',(-10.0696566102219,-20.8691408373705,
12.));
#228533=CARTESIAN_POINT('Ctrl Pts',(-10.0797320551154,-20.8815318371844,
0.));
#228534=CARTESIAN_POINT('Ctrl Pts',(-10.0797320551154,-20.8815318371844,
12.));
#228535=CARTESIAN_POINT('Ctrl Pts',(-10.0899339901916,-20.8940023457371,
0.));
#228536=CARTESIAN_POINT('Ctrl Pts',(-10.0899339901916,-20.8940023457371,
12.));
#228537=CARTESIAN_POINT('Ctrl Pts',(-10.1002620040076,-20.9065508112556,
0.));
#228538=CARTESIAN_POINT('Ctrl Pts',(-10.1002620040076,-20.9065508112556,
12.));
#228539=CARTESIAN_POINT('Ctrl Pts',(-10.1107156904836,-20.9191757106266,
0.));
#228540=CARTESIAN_POINT('Ctrl Pts',(-10.1107156904836,-20.9191757106266,
12.));
#228541=CARTESIAN_POINT('Ctrl Pts',(-10.1212946487057,-20.931875548473,
0.));
#228542=CARTESIAN_POINT('Ctrl Pts',(-10.1212946487057,-20.931875548473,
12.));
#228543=CARTESIAN_POINT('Ctrl Pts',(-10.1319984827909,-20.944648856393,
0.));
#228544=CARTESIAN_POINT('Ctrl Pts',(-10.1319984827909,-20.944648856393,
12.));
#228545=CARTESIAN_POINT('Ctrl Pts',(-10.1428268017257,-20.9574941921591,
0.));
#228546=CARTESIAN_POINT('Ctrl Pts',(-10.1428268017257,-20.9574941921591,
12.));
#228547=CARTESIAN_POINT('Ctrl Pts',(-10.1537792192065,-20.970410138937,
0.));
#228548=CARTESIAN_POINT('Ctrl Pts',(-10.1537792192065,-20.970410138937,
12.));
#228549=CARTESIAN_POINT('Ctrl Pts',(-10.1648553534567,-20.9833953044736,
0.));
#228550=CARTESIAN_POINT('Ctrl Pts',(-10.1648553534567,-20.9833953044736,
12.));
#228551=CARTESIAN_POINT('Ctrl Pts',(-10.1760548270765,-20.9964483203685,
0.));
#228552=CARTESIAN_POINT('Ctrl Pts',(-10.1760548270765,-20.9964483203685,
12.));
#228553=CARTESIAN_POINT('Ctrl Pts',(-10.1873772669358,-21.0095678414486,
0.));
#228554=CARTESIAN_POINT('Ctrl Pts',(-10.1873772669358,-21.0095678414486,
12.));
#228555=CARTESIAN_POINT('Ctrl Pts',(-10.1988223040425,-21.0227525451107,
0.));
#228556=CARTESIAN_POINT('Ctrl Pts',(-10.1988223040425,-21.0227525451107,
12.));
#228557=CARTESIAN_POINT('Ctrl Pts',(-10.2103895734124,-21.0360011306814,
0.));
#228558=CARTESIAN_POINT('Ctrl Pts',(-10.2103895734124,-21.0360011306814,
12.));
#228559=CARTESIAN_POINT('Ctrl Pts',(-10.2220787139157,-21.0493123187483,
0.));
#228560=CARTESIAN_POINT('Ctrl Pts',(-10.2220787139157,-21.0493123187483,
12.));
#228561=CARTESIAN_POINT('Ctrl Pts',(-10.233889368157,-21.0626848505665,
0.));
#228562=CARTESIAN_POINT('Ctrl Pts',(-10.233889368157,-21.0626848505665,
12.));
#228563=CARTESIAN_POINT('Ctrl Pts',(-10.2458211823915,-21.0761174875448,
0.));
#228564=CARTESIAN_POINT('Ctrl Pts',(-10.2458211823915,-21.0761174875448,
12.));
#228565=CARTESIAN_POINT('Ctrl Pts',(-10.2578738064183,-21.0896090107066,
0.));
#228566=CARTESIAN_POINT('Ctrl Pts',(-10.2578738064183,-21.0896090107066,
12.));
#228567=CARTESIAN_POINT('Ctrl Pts',(-10.2700468934743,-21.1031582201625,
0.));
#228568=CARTESIAN_POINT('Ctrl Pts',(-10.2700468934743,-21.1031582201625,
12.));
#228569=CARTESIAN_POINT('Ctrl Pts',(-10.2823401001067,-21.1167639345623,
0.));
#228570=CARTESIAN_POINT('Ctrl Pts',(-10.2823401001067,-21.1167639345623,
12.));
#228571=CARTESIAN_POINT('Ctrl Pts',(-10.2947530860714,-21.130424990599,
0.));
#228572=CARTESIAN_POINT('Ctrl Pts',(-10.2947530860714,-21.130424990599,
12.));
#228573=CARTESIAN_POINT('Ctrl Pts',(-10.307285514268,-21.1441402425831,
0.));
#228574=CARTESIAN_POINT('Ctrl Pts',(-10.307285514268,-21.1441402425831,
12.));
#228575=CARTESIAN_POINT('Ctrl Pts',(-10.3199370506541,-21.1579085619959,
0.));
#228576=CARTESIAN_POINT('Ctrl Pts',(-10.3199370506541,-21.1579085619959,
12.));
#228577=CARTESIAN_POINT('Ctrl Pts',(-10.3327073641574,-21.1717288370512,
0.));
#228578=CARTESIAN_POINT('Ctrl Pts',(-10.3327073641574,-21.1717288370512,
12.));
#228579=CARTESIAN_POINT('Ctrl Pts',(-10.3455961265706,-21.1855999722427,
0.));
#228580=CARTESIAN_POINT('Ctrl Pts',(-10.3455961265706,-21.1855999722427,
12.));
#228581=CARTESIAN_POINT('Ctrl Pts',(-10.3586030124595,-21.1995208879205,
0.));
#228582=CARTESIAN_POINT('Ctrl Pts',(-10.3586030124595,-21.1995208879205,
12.));
#228583=CARTESIAN_POINT('Ctrl Pts',(-10.3717276991137,-21.2134905199359,
0.));
#228584=CARTESIAN_POINT('Ctrl Pts',(-10.3717276991137,-21.2134905199359,
12.));
#228585=CARTESIAN_POINT('Ctrl Pts',(-10.384969866479,-21.2275078192708,
0.));
#228586=CARTESIAN_POINT('Ctrl Pts',(-10.384969866479,-21.2275078192708,
12.));
#228587=CARTESIAN_POINT('Ctrl Pts',(-10.3983291970846,-21.2415717516713,
0.));
#228588=CARTESIAN_POINT('Ctrl Pts',(-10.3983291970846,-21.2415717516713,
12.));
#228589=CARTESIAN_POINT('Ctrl Pts',(-10.4118053759584,-21.2556812972741,
0.));
#228590=CARTESIAN_POINT('Ctrl Pts',(-10.4118053759584,-21.2556812972741,
12.));
#228591=CARTESIAN_POINT('Ctrl Pts',(-10.4253980905394,-21.2698354502391,
0.));
#228592=CARTESIAN_POINT('Ctrl Pts',(-10.4253980905394,-21.2698354502391,
12.));
#228593=CARTESIAN_POINT('Ctrl Pts',(-10.4391070306385,-21.2840332184471,
0.));
#228594=CARTESIAN_POINT('Ctrl Pts',(-10.4391070306385,-21.2840332184471,
12.));
#228595=CARTESIAN_POINT('Ctrl Pts',(-10.452931888387,-21.2982736231924,
0.));
#228596=CARTESIAN_POINT('Ctrl Pts',(-10.452931888387,-21.2982736231924,
12.));
#228597=CARTESIAN_POINT('Ctrl Pts',(-10.4668723581768,-21.312555698873,
0.));
#228598=CARTESIAN_POINT('Ctrl Pts',(-10.4668723581768,-21.312555698873,
12.));
#228599=CARTESIAN_POINT('Ctrl Pts',(-10.4809281365933,-21.3268784926823,
0.));
#228600=CARTESIAN_POINT('Ctrl Pts',(-10.4809281365933,-21.3268784926823,
12.));
#228601=CARTESIAN_POINT('Ctrl Pts',(-10.4950989223341,-21.3412410642912,
0.));
#228602=CARTESIAN_POINT('Ctrl Pts',(-10.4950989223341,-21.3412410642912,
12.));
#228603=CARTESIAN_POINT('Ctrl Pts',(-10.509384416169,-21.3556424855822,
0.));
#228604=CARTESIAN_POINT('Ctrl Pts',(-10.509384416169,-21.3556424855822,
12.));
#228605=CARTESIAN_POINT('Ctrl Pts',(-10.523784320906,-21.3700818403942,
0.));
#228606=CARTESIAN_POINT('Ctrl Pts',(-10.523784320906,-21.3700818403942,
12.));
#228607=CARTESIAN_POINT('Ctrl Pts',(-10.5382983413422,-21.3845582242604,
0.));
#228608=CARTESIAN_POINT('Ctrl Pts',(-10.5382983413422,-21.3845582242604,
12.));
#228609=CARTESIAN_POINT('Ctrl Pts',(-10.5529261842107,-21.3990707441495,
0.));
#228610=CARTESIAN_POINT('Ctrl Pts',(-10.5529261842107,-21.3990707441495,
12.));
#228611=CARTESIAN_POINT('Ctrl Pts',(-10.5676675581106,-21.4136185181974,
0.));
#228612=CARTESIAN_POINT('Ctrl Pts',(-10.5676675581106,-21.4136185181974,
12.));
#228613=CARTESIAN_POINT('Ctrl Pts',(-10.582522173457,-21.4282006754624,
0.));
#228614=CARTESIAN_POINT('Ctrl Pts',(-10.582522173457,-21.4282006754624,
12.));
#228615=CARTESIAN_POINT('Ctrl Pts',(-10.597489742462,-21.4428163557137,
0.));
#228616=CARTESIAN_POINT('Ctrl Pts',(-10.597489742462,-21.4428163557137,
12.));
#228617=CARTESIAN_POINT('Ctrl Pts',(-10.612569979096,-21.4574647092093,
0.));
#228618=CARTESIAN_POINT('Ctrl Pts',(-10.612569979096,-21.4574647092093,
12.));
#228619=CARTESIAN_POINT('Ctrl Pts',(-10.6277625990457,-21.4721448964766,
0.));
#228620=CARTESIAN_POINT('Ctrl Pts',(-10.6277625990457,-21.4721448964766,
12.));
#228621=CARTESIAN_POINT('Ctrl Pts',(-10.6430673196609,-21.4868560880893,
0.));
#228622=CARTESIAN_POINT('Ctrl Pts',(-10.6430673196609,-21.4868560880893,
12.));
#228623=CARTESIAN_POINT('Ctrl Pts',(-10.6584838598941,-21.5015974644454,
0.));
#228624=CARTESIAN_POINT('Ctrl Pts',(-10.6584838598941,-21.5015974644454,
12.));
#228625=CARTESIAN_POINT('Ctrl Pts',(-10.6740119402835,-21.5163682155805,
0.));
#228626=CARTESIAN_POINT('Ctrl Pts',(-10.6740119402835,-21.5163682155805,
12.));
#228627=CARTESIAN_POINT('Ctrl Pts',(-10.689651282929,-21.531167540981,0.));
#228628=CARTESIAN_POINT('Ctrl Pts',(-10.689651282929,-21.531167540981,12.));
#228629=CARTESIAN_POINT('Ctrl Pts',(-10.7054016114571,-21.5459946493955,
0.));
#228630=CARTESIAN_POINT('Ctrl Pts',(-10.7054016114571,-21.5459946493955,
12.));
#228631=CARTESIAN_POINT('Ctrl Pts',(-10.7212626509816,-21.5608487586467,
0.));
#228632=CARTESIAN_POINT('Ctrl Pts',(-10.7212626509816,-21.5608487586467,
12.));
#228633=CARTESIAN_POINT('Ctrl Pts',(-10.7372341280468,-21.5757290954372,
0.));
#228634=CARTESIAN_POINT('Ctrl Pts',(-10.7372341280468,-21.5757290954372,
12.));
#228635=CARTESIAN_POINT('Ctrl Pts',(-10.7533157705943,-21.5906348951745,
0.));
#228636=CARTESIAN_POINT('Ctrl Pts',(-10.7533157705943,-21.5906348951745,
12.));
#228637=CARTESIAN_POINT('Ctrl Pts',(-10.7695073079554,-21.6055654018179,
0.));
#228638=CARTESIAN_POINT('Ctrl Pts',(-10.7695073079554,-21.6055654018179,
12.));
#228639=CARTESIAN_POINT('Ctrl Pts',(-10.7858084708262,-21.6205198677176,
0.));
#228640=CARTESIAN_POINT('Ctrl Pts',(-10.7858084708262,-21.6205198677176,
12.));
#228641=CARTESIAN_POINT('Ctrl Pts',(-10.802218991237,-21.6354975534557,
0.));
#228642=CARTESIAN_POINT('Ctrl Pts',(-10.802218991237,-21.6354975534557,
12.));
#228643=CARTESIAN_POINT('Ctrl Pts',(-10.8187386025135,-21.6504977276864,
0.));
#228644=CARTESIAN_POINT('Ctrl Pts',(-10.8187386025135,-21.6504977276864,
12.));
#228645=CARTESIAN_POINT('Ctrl Pts',(-10.835367039227,-21.6655196669727,
0.));
#228646=CARTESIAN_POINT('Ctrl Pts',(-10.835367039227,-21.6655196669727,
12.));
#228647=CARTESIAN_POINT('Ctrl Pts',(-10.8521040371832,-21.6805626556461,
0.));
#228648=CARTESIAN_POINT('Ctrl Pts',(-10.8521040371832,-21.6805626556461,
12.));
#228649=CARTESIAN_POINT('Ctrl Pts',(-10.8689493334093,-21.6956259856667,
0.));
#228650=CARTESIAN_POINT('Ctrl Pts',(-10.8689493334093,-21.6956259856667,
12.));
#228651=CARTESIAN_POINT('Ctrl Pts',(-10.8859026661292,-21.7107089564822,
0.));
#228652=CARTESIAN_POINT('Ctrl Pts',(-10.8859026661292,-21.7107089564822,
12.));
#228653=CARTESIAN_POINT('Ctrl Pts',(-10.9029637747341,-21.7258108748874,
0.));
#228654=CARTESIAN_POINT('Ctrl Pts',(-10.9029637747341,-21.7258108748874,
12.));
#228655=CARTESIAN_POINT('Ctrl Pts',(-10.9201323997386,-21.74093105488,0.));
#228656=CARTESIAN_POINT('Ctrl Pts',(-10.9201323997386,-21.74093105488,12.));
#228657=CARTESIAN_POINT('Ctrl Pts',(-10.9374082827446,-21.7560688175252,
0.));
#228658=CARTESIAN_POINT('Ctrl Pts',(-10.9374082827446,-21.7560688175252,
12.));
#228659=CARTESIAN_POINT('Ctrl Pts',(-10.9547911664457,-21.7712234908468,
0.));
#228660=CARTESIAN_POINT('Ctrl Pts',(-10.9547911664457,-21.7712234908468,
12.));
#228661=CARTESIAN_POINT('Ctrl Pts',(-10.9722807946157,-21.7863944097143,
0.));
#228662=CARTESIAN_POINT('Ctrl Pts',(-10.9722807946157,-21.7863944097143,
12.));
#228663=CARTESIAN_POINT('Ctrl Pts',(-10.9898769120913,-21.8015809157302,
0.));
#228664=CARTESIAN_POINT('Ctrl Pts',(-10.9898769120913,-21.8015809157302,
12.));
#228665=CARTESIAN_POINT('Ctrl Pts',(-11.0075792647477,-21.8167823571168,
0.));
#228666=CARTESIAN_POINT('Ctrl Pts',(-11.0075792647477,-21.8167823571168,
12.));
#228667=CARTESIAN_POINT('Ctrl Pts',(-11.0253875994598,-21.8319980886033,
0.));
#228668=CARTESIAN_POINT('Ctrl Pts',(-11.0253875994598,-21.8319980886033,
12.));
#228669=CARTESIAN_POINT('Ctrl Pts',(-11.0433016640808,-21.8472274713103,
0.));
#228670=CARTESIAN_POINT('Ctrl Pts',(-11.0433016640808,-21.8472274713103,
12.));
#228671=CARTESIAN_POINT('Ctrl Pts',(-11.0613212074364,-21.8624698726319,
0.));
#228672=CARTESIAN_POINT('Ctrl Pts',(-11.0613212074364,-21.8624698726319,
12.));
#228673=CARTESIAN_POINT('Ctrl Pts',(-11.0794459793058,-21.8777246661191,
0.));
#228674=CARTESIAN_POINT('Ctrl Pts',(-11.0794459793058,-21.8777246661191,
12.));
#228675=CARTESIAN_POINT('Ctrl Pts',(-11.0976757303944,-21.8929912313608,
0.));
#228676=CARTESIAN_POINT('Ctrl Pts',(-11.0976757303944,-21.8929912313608,
12.));
#228677=CARTESIAN_POINT('Ctrl Pts',(-11.1160102123024,-21.9082689538687,
0.));
#228678=CARTESIAN_POINT('Ctrl Pts',(-11.1160102123024,-21.9082689538687,
12.));
#228679=CARTESIAN_POINT('Ctrl Pts',(-11.134449177474,-21.9235572249518,
0.));
#228680=CARTESIAN_POINT('Ctrl Pts',(-11.134449177474,-21.9235572249518,
12.));
#228681=CARTESIAN_POINT('Ctrl Pts',(-11.1529923792002,-21.9388554416437,
0.));
#228682=CARTESIAN_POINT('Ctrl Pts',(-11.1529923792002,-21.9388554416437,
12.));
#228683=CARTESIAN_POINT('Ctrl Pts',(-11.1716395716375,-21.9541630066504,
0.));
#228684=CARTESIAN_POINT('Ctrl Pts',(-11.1716395716375,-21.9541630066504,
12.));
#228685=CARTESIAN_POINT('Ctrl Pts',(-11.190390509811,-21.9694793282913,
0.));
#228686=CARTESIAN_POINT('Ctrl Pts',(-11.190390509811,-21.9694793282913,
12.));
#228687=CARTESIAN_POINT('Ctrl Pts',(-11.2092449496125,-21.9848038204439,
0.));
#228688=CARTESIAN_POINT('Ctrl Pts',(-11.2092449496125,-21.9848038204439,
12.));
#228689=CARTESIAN_POINT('Ctrl Pts',(-11.2282026477897,-22.0001359024839,
0.));
#228690=CARTESIAN_POINT('Ctrl Pts',(-11.2282026477897,-22.0001359024839,
12.));
#228691=CARTESIAN_POINT('Ctrl Pts',(-11.2472633619276,-22.0154749992364,
0.));
#228692=CARTESIAN_POINT('Ctrl Pts',(-11.2472633619276,-22.0154749992364,
12.));
#228693=CARTESIAN_POINT('Ctrl Pts',(-11.2664268504207,-22.0308205408351,
0.));
#228694=CARTESIAN_POINT('Ctrl Pts',(-11.2664268504207,-22.0308205408351,
12.));
#228695=CARTESIAN_POINT('Ctrl Pts',(-11.2856928724374,-22.046171962566,
0.));
#228696=CARTESIAN_POINT('Ctrl Pts',(-11.2856928724374,-22.046171962566,
12.));
#228697=CARTESIAN_POINT('Ctrl Pts',(-11.3050611878771,-22.0615287047179,
0.));
#228698=CARTESIAN_POINT('Ctrl Pts',(-11.3050611878771,-22.0615287047179,
12.));
#228699=CARTESIAN_POINT('Ctrl Pts',(-11.3245315573168,-22.0768902124267,
0.));
#228700=CARTESIAN_POINT('Ctrl Pts',(-11.3245315573168,-22.0768902124267,
12.));
#228701=CARTESIAN_POINT('Ctrl Pts',(-11.3441037419553,-22.0922559355293,
0.));
#228702=CARTESIAN_POINT('Ctrl Pts',(-11.3441037419553,-22.0922559355293,
12.));
#228703=CARTESIAN_POINT('Ctrl Pts',(-11.3637775035367,-22.1076253283978,
0.));
#228704=CARTESIAN_POINT('Ctrl Pts',(-11.3637775035367,-22.1076253283978,
12.));
#228705=CARTESIAN_POINT('Ctrl Pts',(-11.3835526044256,-22.1229978500185,
0.));
#228706=CARTESIAN_POINT('Ctrl Pts',(-11.3835526044256,-22.1229978500185,
12.));
#228707=CARTESIAN_POINT('Ctrl Pts',(-11.4034288076909,-22.1383729640963,
0.));
#228708=CARTESIAN_POINT('Ctrl Pts',(-11.4034288076909,-22.1383729640963,
12.));
#228709=CARTESIAN_POINT('Ctrl Pts',(-11.4234058771742,-22.1537501391486,
0.));
#228710=CARTESIAN_POINT('Ctrl Pts',(-11.4234058771742,-22.1537501391486,
12.));
#228711=CARTESIAN_POINT('Ctrl Pts',(-11.443483577557,-22.1691288486096,
0.));
#228712=CARTESIAN_POINT('Ctrl Pts',(-11.443483577557,-22.1691288486096,
12.));
#228713=CARTESIAN_POINT('Ctrl Pts',(-11.463661674411,-22.1845085709169,
0.));
#228714=CARTESIAN_POINT('Ctrl Pts',(-11.463661674411,-22.1845085709169,
12.));
#228715=CARTESIAN_POINT('Ctrl Pts',(-11.4839399342589,-22.1998887896435,
0.));
#228716=CARTESIAN_POINT('Ctrl Pts',(-11.4839399342589,-22.1998887896435,
12.));
#228717=CARTESIAN_POINT('Ctrl Pts',(-11.504318124424,-22.215268993102,0.));
#228718=CARTESIAN_POINT('Ctrl Pts',(-11.504318124424,-22.215268993102,12.));
#228719=CARTESIAN_POINT('Ctrl Pts',(-11.5247960128476,-22.2306486738899,
0.));
#228720=CARTESIAN_POINT('Ctrl Pts',(-11.5247960128476,-22.2306486738899,
12.));
#228721=CARTESIAN_POINT('Ctrl Pts',(-11.545373367912,-22.2460273284653,
0.));
#228722=CARTESIAN_POINT('Ctrl Pts',(-11.545373367912,-22.2460273284653,
12.));
#228723=CARTESIAN_POINT('Ctrl Pts',(-11.5660499582403,-22.2614044566898,
0.));
#228724=CARTESIAN_POINT('Ctrl Pts',(-11.5660499582403,-22.2614044566898,
12.));
#228725=CARTESIAN_POINT('Ctrl Pts',(-11.5868255525189,-22.2767795614349,
0.));
#228726=CARTESIAN_POINT('Ctrl Pts',(-11.5868255525189,-22.2767795614349,
12.));
#228727=CARTESIAN_POINT('Ctrl Pts',(-11.6076999192359,-22.2921521480357,
0.));
#228728=CARTESIAN_POINT('Ctrl Pts',(-11.6076999192359,-22.2921521480357,
12.));
#228729=CARTESIAN_POINT('Ctrl Pts',(-11.6286728270011,-22.3075217249049,
0.));
#228730=CARTESIAN_POINT('Ctrl Pts',(-11.6286728270011,-22.3075217249049,
12.));
#228731=CARTESIAN_POINT('Ctrl Pts',(-11.6497440449858,-22.3228878043976,
0.));
#228732=CARTESIAN_POINT('Ctrl Pts',(-11.6497440449858,-22.3228878043976,
12.));
#228733=CARTESIAN_POINT('Ctrl Pts',(-11.6709133432986,-22.3382499035618,
0.));
#228734=CARTESIAN_POINT('Ctrl Pts',(-11.6709133432986,-22.3382499035618,
12.));
#228735=CARTESIAN_POINT('Ctrl Pts',(-11.6921804934056,-22.3536075450028,
0.));
#228736=CARTESIAN_POINT('Ctrl Pts',(-11.6921804934056,-22.3536075450028,
12.));
#228737=CARTESIAN_POINT('Ctrl Pts',(-11.7135452684532,-22.3689602575492,
0.));
#228738=CARTESIAN_POINT('Ctrl Pts',(-11.7135452684532,-22.3689602575492,
12.));
#228739=CARTESIAN_POINT('Ctrl Pts',(-11.7350074437961,-22.3843075773905,
0.));
#228740=CARTESIAN_POINT('Ctrl Pts',(-11.7350074437961,-22.3843075773905,
12.));
#228741=CARTESIAN_POINT('Ctrl Pts',(-11.7565667964765,-22.39964904692,0.));
#228742=CARTESIAN_POINT('Ctrl Pts',(-11.7565667964765,-22.39964904692,12.));
#228743=CARTESIAN_POINT('Ctrl Pts',(-11.7782231042041,-22.4149842125018,
0.));
#228744=CARTESIAN_POINT('Ctrl Pts',(-11.7782231042041,-22.4149842125018,
12.));
#228745=CARTESIAN_POINT('Ctrl Pts',(-11.7999761445175,-22.4303126226468,
0.));
#228746=CARTESIAN_POINT('Ctrl Pts',(-11.7999761445175,-22.4303126226468,
12.));
#228747=CARTESIAN_POINT('Ctrl Pts',(-11.8218256937889,-22.4456338258738,
0.));
#228748=CARTESIAN_POINT('Ctrl Pts',(-11.8218256937889,-22.4456338258738,
12.));
#228749=CARTESIAN_POINT('Ctrl Pts',(-11.8437715264487,-22.4609473690469,
0.));
#228750=CARTESIAN_POINT('Ctrl Pts',(-11.8437715264487,-22.4609473690469,
12.));
#228751=CARTESIAN_POINT('Ctrl Pts',(-11.8658134137018,-22.4762527946694,
0.));
#228752=CARTESIAN_POINT('Ctrl Pts',(-11.8658134137018,-22.4762527946694,
12.));
#228753=CARTESIAN_POINT('Ctrl Pts',(-11.8879511239941,-22.4915496418472,
0.));
#228754=CARTESIAN_POINT('Ctrl Pts',(-11.8879511239941,-22.4915496418472,
12.));
#228755=CARTESIAN_POINT('Ctrl Pts',(-11.9101844254555,-22.5068374513958,
0.));
#228756=CARTESIAN_POINT('Ctrl Pts',(-11.9101844254555,-22.5068374513958,
12.));
#228757=CARTESIAN_POINT('Ctrl Pts',(-11.9325130877801,-22.5221157697869,
0.));
#228758=CARTESIAN_POINT('Ctrl Pts',(-11.9325130877801,-22.5221157697869,
12.));
#228759=CARTESIAN_POINT('Ctrl Pts',(-11.9549368843996,-22.5373841537299,
0.));
#228760=CARTESIAN_POINT('Ctrl Pts',(-11.9549368843996,-22.5373841537299,
12.));
#228761=CARTESIAN_POINT('Ctrl Pts',(-11.9774555943496,-22.5526421741159,
0.));
#228762=CARTESIAN_POINT('Ctrl Pts',(-11.9774555943496,-22.5526421741159,
12.));
#228763=CARTESIAN_POINT('Ctrl Pts',(-12.0000690046697,-22.5678894211194,
0.));
#228764=CARTESIAN_POINT('Ctrl Pts',(-12.0000690046697,-22.5678894211194,
12.));
#228765=CARTESIAN_POINT('Ctrl Pts',(-12.0227769113132,-22.5831255061306,
0.));
#228766=CARTESIAN_POINT('Ctrl Pts',(-12.0227769113132,-22.5831255061306,
12.));
#228767=CARTESIAN_POINT('Ctrl Pts',(-12.0455791139135,-22.5983500505675,
0.));
#228768=CARTESIAN_POINT('Ctrl Pts',(-12.0455791139135,-22.5983500505675,
12.));
#228769=CARTESIAN_POINT('Ctrl Pts',(-12.0684754113869,-22.613562676493,
0.));
#228770=CARTESIAN_POINT('Ctrl Pts',(-12.0684754113869,-22.613562676493,
12.));
#228771=CARTESIAN_POINT('Ctrl Pts',(-12.0914655972828,-22.628762996708,
0.));
#228772=CARTESIAN_POINT('Ctrl Pts',(-12.0914655972828,-22.628762996708,
12.));
#228773=CARTESIAN_POINT('Ctrl Pts',(-12.1145494550384,-22.6439506046611,
0.));
#228774=CARTESIAN_POINT('Ctrl Pts',(-12.1145494550384,-22.6439506046611,
12.));
#228775=CARTESIAN_POINT('Ctrl Pts',(-12.1377267537141,-22.6591250653942,
0.));
#228776=CARTESIAN_POINT('Ctrl Pts',(-12.1377267537141,-22.6591250653942,
12.));
#228777=CARTESIAN_POINT('Ctrl Pts',(-12.1609972423089,-22.6742859034891,
0.));
#228778=CARTESIAN_POINT('Ctrl Pts',(-12.1609972423089,-22.6742859034891,
12.));
#228779=CARTESIAN_POINT('Ctrl Pts',(-12.1843606579246,-22.6894326204959,
0.));
#228780=CARTESIAN_POINT('Ctrl Pts',(-12.1843606579246,-22.6894326204959,
12.));
#228781=CARTESIAN_POINT('Ctrl Pts',(-12.2078167360267,-22.7045647168659,
0.));
#228782=CARTESIAN_POINT('Ctrl Pts',(-12.2078167360267,-22.7045647168659,
12.));
#228783=CARTESIAN_POINT('Ctrl Pts',(-12.2313652198047,-22.7196817119299,
0.));
#228784=CARTESIAN_POINT('Ctrl Pts',(-12.2313652198047,-22.7196817119299,
12.));
#228785=CARTESIAN_POINT('Ctrl Pts',(-12.2550058702389,-22.7347831655251,
0.));
#228786=CARTESIAN_POINT('Ctrl Pts',(-12.2550058702389,-22.7347831655251,
12.));
#228787=CARTESIAN_POINT('Ctrl Pts',(-12.2787384750747,-22.7498686970096,
0.));
#228788=CARTESIAN_POINT('Ctrl Pts',(-12.2787384750747,-22.7498686970096,
12.));
#228789=CARTESIAN_POINT('Ctrl Pts',(-12.3025628601812,-22.7649380101154,
0.));
#228790=CARTESIAN_POINT('Ctrl Pts',(-12.3025628601812,-22.7649380101154,
12.));
#228791=CARTESIAN_POINT('Ctrl Pts',(-12.3264788926108,-22.7799908974947,
0.));
#228792=CARTESIAN_POINT('Ctrl Pts',(-12.3264788926108,-22.7799908974947,
12.));
#228793=CARTESIAN_POINT('Ctrl Pts',(-12.3504864740361,-22.7950272216959,
0.));
#228794=CARTESIAN_POINT('Ctrl Pts',(-12.3504864740361,-22.7950272216959,
12.));
#228795=CARTESIAN_POINT('Ctrl Pts',(-12.3745855366772,-22.8100469022632,
0.));
#228796=CARTESIAN_POINT('Ctrl Pts',(-12.3745855366772,-22.8100469022632,
12.));
#228797=CARTESIAN_POINT('Ctrl Pts',(-12.393937937903,-22.8220493007353,
0.));
#228798=CARTESIAN_POINT('Ctrl Pts',(-12.393937937903,-22.8220493007353,
12.));
#228799=CARTESIAN_POINT('Ctrl Pts',(-12.4084933766366,-22.8310435872852,
0.));
#228800=CARTESIAN_POINT('Ctrl Pts',(-12.4084933766366,-22.8310435872852,
12.));
#228801=CARTESIAN_POINT('Ctrl Pts',(-12.4182152851867,-22.8370364396497,
0.));
#228802=CARTESIAN_POINT('Ctrl Pts',(-12.4182152851867,-22.8370364396497,
12.));
#228803=CARTESIAN_POINT('Ctrl Pts',(-12.4230808101438,-22.8400320311648,
0.));
#228804=CARTESIAN_POINT('Ctrl Pts',(-12.4230808101438,-22.8400320311648,
12.));
#228805=CARTESIAN_POINT('',(-12.4230808101438,-22.8400320311648,0.));
#228806=CARTESIAN_POINT('Ctrl Pts',(-9.71462809124917,-20.353053841303,
0.));
#228807=CARTESIAN_POINT('Ctrl Pts',(-9.71462954053074,-20.353060251684,
0.));
#228808=CARTESIAN_POINT('Ctrl Pts',(-9.71465227853122,-20.3531126095522,
0.));
#228809=CARTESIAN_POINT('Ctrl Pts',(-9.71474590350792,-20.3533097561886,
0.));
#228810=CARTESIAN_POINT('Ctrl Pts',(-9.71498978052101,-20.3538098605706,
0.));
#228811=CARTESIAN_POINT('Ctrl Pts',(-9.71549257088175,-20.3548282742361,
0.));
#228812=CARTESIAN_POINT('Ctrl Pts',(-9.71619192554147,-20.3562337557875,
0.));
#228813=CARTESIAN_POINT('Ctrl Pts',(-9.71708493723062,-20.3580133103357,
0.));
#228814=CARTESIAN_POINT('Ctrl Pts',(-9.71816778327999,-20.3601498764344,
0.));
#228815=CARTESIAN_POINT('Ctrl Pts',(-9.71943648548115,-20.362625691398,
0.));
#228816=CARTESIAN_POINT('Ctrl Pts',(-9.72088778381102,-20.3654261611055,
0.));
#228817=CARTESIAN_POINT('Ctrl Pts',(-9.72251930722504,-20.3685406190576,
0.));
#228818=CARTESIAN_POINT('Ctrl Pts',(-9.72432910043193,-20.371960235676,
0.));
#228819=CARTESIAN_POINT('Ctrl Pts',(-9.72631531732871,-20.3756766651952,
0.));
#228820=CARTESIAN_POINT('Ctrl Pts',(-9.72847589116533,-20.3796805893304,
0.));
#228821=CARTESIAN_POINT('Ctrl Pts',(-9.73080870123726,-20.3839624556742,
0.));
#228822=CARTESIAN_POINT('Ctrl Pts',(-9.73331167102812,-20.3885129129912,
0.));
#228823=CARTESIAN_POINT('Ctrl Pts',(-9.7359829201425,-20.3933234845646,
0.));
#228824=CARTESIAN_POINT('Ctrl Pts',(-9.73882077613206,-20.3983866213331,
0.));
#228825=CARTESIAN_POINT('Ctrl Pts',(-9.74182369656273,-20.4036953576549,
0.));
#228826=CARTESIAN_POINT('Ctrl Pts',(-9.74499021838537,-20.4092430879861,
0.));
#228827=CARTESIAN_POINT('Ctrl Pts',(-9.74831889242175,-20.4150232777393,
0.));
#228828=CARTESIAN_POINT('Ctrl Pts',(-9.75180829786433,-20.4210295275818,
0.));
#228829=CARTESIAN_POINT('Ctrl Pts',(-9.75545705902416,-20.4272556476629,
0.));
#228830=CARTESIAN_POINT('Ctrl Pts',(-9.7592638628993,-20.4336957355474,
0.));
#228831=CARTESIAN_POINT('Ctrl Pts',(-9.76322747195502,-20.4403442329401,
0.));
#228832=CARTESIAN_POINT('Ctrl Pts',(-9.76734670980897,-20.447195862298,
0.));
#228833=CARTESIAN_POINT('Ctrl Pts',(-9.7716204510407,-20.4542455817527,
0.));
#228834=CARTESIAN_POINT('Ctrl Pts',(-9.77604760815523,-20.4614885274973,
0.));
#228835=CARTESIAN_POINT('Ctrl Pts',(-9.78062712373313,-20.4689199790668,
0.));
#228836=CARTESIAN_POINT('Ctrl Pts',(-9.78535797314162,-20.4765353711585,
0.));
#228837=CARTESIAN_POINT('Ctrl Pts',(-9.7902391649866,-20.4843302955329,
0.));
#228838=CARTESIAN_POINT('Ctrl Pts',(-9.79526974288344,-20.4923005087945,
0.));
#228839=CARTESIAN_POINT('Ctrl Pts',(-9.80044878520968,-20.500441931211,
0.));
#228840=CARTESIAN_POINT('Ctrl Pts',(-9.80577540161103,-20.5087506310507,
0.));
#228841=CARTESIAN_POINT('Ctrl Pts',(-9.81124873025278,-20.5172228122839,
0.));
#228842=CARTESIAN_POINT('Ctrl Pts',(-9.81686793455918,-20.5258548000625,
0.));
#228843=CARTESIAN_POINT('Ctrl Pts',(-9.82263220080328,-20.534643029951,
0.));
#228844=CARTESIAN_POINT('Ctrl Pts',(-9.82854073773858,-20.5435840460717,
0.));
#228845=CARTESIAN_POINT('Ctrl Pts',(-9.83459277585321,-20.5526744976461,
0.));
#228846=CARTESIAN_POINT('Ctrl Pts',(-9.84078756677589,-20.5619111362406,
0.));
#228847=CARTESIAN_POINT('Ctrl Pts',(-9.84712438256308,-20.5712908125145,
0.));
#228848=CARTESIAN_POINT('Ctrl Pts',(-9.85360251457004,-20.580810471002,
0.));
#228849=CARTESIAN_POINT('Ctrl Pts',(-9.8602212723275,-20.5904671449754,
0.));
#228850=CARTESIAN_POINT('Ctrl Pts',(-9.86697998242612,-20.6002579513696,
0.));
#228851=CARTESIAN_POINT('Ctrl Pts',(-9.87387798732944,-20.6101800854491,
0.));
#228852=CARTESIAN_POINT('Ctrl Pts',(-9.88091464472669,-20.6202308177472,
0.));
#228853=CARTESIAN_POINT('Ctrl Pts',(-9.88808932697305,-20.6304074914086,
0.));
#228854=CARTESIAN_POINT('Ctrl Pts',(-9.89540142049124,-20.6407075193977,
0.));
#228855=CARTESIAN_POINT('Ctrl Pts',(-9.90285032516696,-20.6511283817415,
0.));
#228856=CARTESIAN_POINT('Ctrl Pts',(-9.91043545377005,-20.6616676228315,
0.));
#228857=CARTESIAN_POINT('Ctrl Pts',(-9.91815623141285,-20.6723228488261,
0.));
#228858=CARTESIAN_POINT('Ctrl Pts',(-9.92601209498751,-20.6830917250255,
0.));
#228859=CARTESIAN_POINT('Ctrl Pts',(-9.93400249259737,-20.6939719732485,
0.));
#228860=CARTESIAN_POINT('Ctrl Pts',(-9.94212688298251,-20.7049613692237,
0.));
#228861=CARTESIAN_POINT('Ctrl Pts',(-9.95038473514962,-20.716057740758,
0.));
#228862=CARTESIAN_POINT('Ctrl Pts',(-9.95877552798403,-20.7272589658752,
0.));
#228863=CARTESIAN_POINT('Ctrl Pts',(-9.96729874986199,-20.7385629709795,
0.));
#228864=CARTESIAN_POINT('Ctrl Pts',(-9.97595389823461,-20.7499677289625,
0.));
#228865=CARTESIAN_POINT('Ctrl Pts',(-9.98474047926846,-20.7614712574989,
0.));
#228866=CARTESIAN_POINT('Ctrl Pts',(-9.99365800754638,-20.7730716175417,
0.));
#228867=CARTESIAN_POINT('Ctrl Pts',(-10.0027060057389,-20.7847669117568,
0.));
#228868=CARTESIAN_POINT('Ctrl Pts',(-10.0118840042786,-20.7965552829907,
0.));
#228869=CARTESIAN_POINT('Ctrl Pts',(-10.0211915410095,-20.8084349126885,
0.));
#228870=CARTESIAN_POINT('Ctrl Pts',(-10.0306281609435,-20.8204040196599,
0.));
#228871=CARTESIAN_POINT('Ctrl Pts',(-10.0401934160234,-20.8324608588906,
0.));
#228872=CARTESIAN_POINT('Ctrl Pts',(-10.0498868648733,-20.8446037203402,
0.));
#228873=CARTESIAN_POINT('Ctrl Pts',(-10.0597080725375,-20.856830927732,
0.));
#228874=CARTESIAN_POINT('Ctrl Pts',(-10.0696566102219,-20.8691408373705,
0.));
#228875=CARTESIAN_POINT('Ctrl Pts',(-10.0797320551154,-20.8815318371844,
0.));
#228876=CARTESIAN_POINT('Ctrl Pts',(-10.0899339901916,-20.8940023457371,
0.));
#228877=CARTESIAN_POINT('Ctrl Pts',(-10.1002620040076,-20.9065508112556,
0.));
#228878=CARTESIAN_POINT('Ctrl Pts',(-10.1107156904836,-20.9191757106266,
0.));
#228879=CARTESIAN_POINT('Ctrl Pts',(-10.1212946487057,-20.931875548473,
0.));
#228880=CARTESIAN_POINT('Ctrl Pts',(-10.1319984827909,-20.944648856393,
0.));
#228881=CARTESIAN_POINT('Ctrl Pts',(-10.1428268017257,-20.9574941921591,
0.));
#228882=CARTESIAN_POINT('Ctrl Pts',(-10.1537792192065,-20.970410138937,
0.));
#228883=CARTESIAN_POINT('Ctrl Pts',(-10.1648553534567,-20.9833953044736,
0.));
#228884=CARTESIAN_POINT('Ctrl Pts',(-10.1760548270765,-20.9964483203685,
0.));
#228885=CARTESIAN_POINT('Ctrl Pts',(-10.1873772669358,-21.0095678414486,
0.));
#228886=CARTESIAN_POINT('Ctrl Pts',(-10.1988223040425,-21.0227525451107,
0.));
#228887=CARTESIAN_POINT('Ctrl Pts',(-10.2103895734124,-21.0360011306814,
0.));
#228888=CARTESIAN_POINT('Ctrl Pts',(-10.2220787139157,-21.0493123187483,
0.));
#228889=CARTESIAN_POINT('Ctrl Pts',(-10.233889368157,-21.0626848505665,
0.));
#228890=CARTESIAN_POINT('Ctrl Pts',(-10.2458211823915,-21.0761174875448,
0.));
#228891=CARTESIAN_POINT('Ctrl Pts',(-10.2578738064183,-21.0896090107066,
0.));
#228892=CARTESIAN_POINT('Ctrl Pts',(-10.2700468934743,-21.1031582201625,
0.));
#228893=CARTESIAN_POINT('Ctrl Pts',(-10.2823401001067,-21.1167639345623,
0.));
#228894=CARTESIAN_POINT('Ctrl Pts',(-10.2947530860714,-21.130424990599,
0.));
#228895=CARTESIAN_POINT('Ctrl Pts',(-10.307285514268,-21.1441402425831,
0.));
#228896=CARTESIAN_POINT('Ctrl Pts',(-10.3199370506541,-21.1579085619959,
0.));
#228897=CARTESIAN_POINT('Ctrl Pts',(-10.3327073641574,-21.1717288370512,
0.));
#228898=CARTESIAN_POINT('Ctrl Pts',(-10.3455961265706,-21.1855999722427,
0.));
#228899=CARTESIAN_POINT('Ctrl Pts',(-10.3586030124595,-21.1995208879205,
0.));
#228900=CARTESIAN_POINT('Ctrl Pts',(-10.3717276991137,-21.2134905199359,
0.));
#228901=CARTESIAN_POINT('Ctrl Pts',(-10.384969866479,-21.2275078192708,
0.));
#228902=CARTESIAN_POINT('Ctrl Pts',(-10.3983291970846,-21.2415717516713,
0.));
#228903=CARTESIAN_POINT('Ctrl Pts',(-10.4118053759584,-21.2556812972741,
0.));
#228904=CARTESIAN_POINT('Ctrl Pts',(-10.4253980905394,-21.2698354502391,
0.));
#228905=CARTESIAN_POINT('Ctrl Pts',(-10.4391070306385,-21.2840332184471,
0.));
#228906=CARTESIAN_POINT('Ctrl Pts',(-10.452931888387,-21.2982736231924,
0.));
#228907=CARTESIAN_POINT('Ctrl Pts',(-10.4668723581768,-21.312555698873,
0.));
#228908=CARTESIAN_POINT('Ctrl Pts',(-10.4809281365933,-21.3268784926823,
0.));
#228909=CARTESIAN_POINT('Ctrl Pts',(-10.4950989223341,-21.3412410642912,
0.));
#228910=CARTESIAN_POINT('Ctrl Pts',(-10.509384416169,-21.3556424855822,
0.));
#228911=CARTESIAN_POINT('Ctrl Pts',(-10.523784320906,-21.3700818403942,
0.));
#228912=CARTESIAN_POINT('Ctrl Pts',(-10.5382983413422,-21.3845582242604,
0.));
#228913=CARTESIAN_POINT('Ctrl Pts',(-10.5529261842107,-21.3990707441495,
0.));
#228914=CARTESIAN_POINT('Ctrl Pts',(-10.5676675581106,-21.4136185181974,
0.));
#228915=CARTESIAN_POINT('Ctrl Pts',(-10.582522173457,-21.4282006754624,
0.));
#228916=CARTESIAN_POINT('Ctrl Pts',(-10.597489742462,-21.4428163557137,
0.));
#228917=CARTESIAN_POINT('Ctrl Pts',(-10.612569979096,-21.4574647092093,
0.));
#228918=CARTESIAN_POINT('Ctrl Pts',(-10.6277625990457,-21.4721448964766,
0.));
#228919=CARTESIAN_POINT('Ctrl Pts',(-10.6430673196609,-21.4868560880893,
0.));
#228920=CARTESIAN_POINT('Ctrl Pts',(-10.6584838598941,-21.5015974644454,
0.));
#228921=CARTESIAN_POINT('Ctrl Pts',(-10.6740119402835,-21.5163682155805,
0.));
#228922=CARTESIAN_POINT('Ctrl Pts',(-10.689651282929,-21.531167540981,0.));
#228923=CARTESIAN_POINT('Ctrl Pts',(-10.7054016114571,-21.5459946493955,
0.));
#228924=CARTESIAN_POINT('Ctrl Pts',(-10.7212626509816,-21.5608487586467,
0.));
#228925=CARTESIAN_POINT('Ctrl Pts',(-10.7372341280468,-21.5757290954372,
0.));
#228926=CARTESIAN_POINT('Ctrl Pts',(-10.7533157705943,-21.5906348951745,
0.));
#228927=CARTESIAN_POINT('Ctrl Pts',(-10.7695073079554,-21.6055654018179,
0.));
#228928=CARTESIAN_POINT('Ctrl Pts',(-10.7858084708262,-21.6205198677176,
0.));
#228929=CARTESIAN_POINT('Ctrl Pts',(-10.802218991237,-21.6354975534557,
0.));
#228930=CARTESIAN_POINT('Ctrl Pts',(-10.8187386025135,-21.6504977276864,
0.));
#228931=CARTESIAN_POINT('Ctrl Pts',(-10.835367039227,-21.6655196669727,
0.));
#228932=CARTESIAN_POINT('Ctrl Pts',(-10.8521040371832,-21.6805626556461,
0.));
#228933=CARTESIAN_POINT('Ctrl Pts',(-10.8689493334093,-21.6956259856667,
0.));
#228934=CARTESIAN_POINT('Ctrl Pts',(-10.8859026661292,-21.7107089564822,
0.));
#228935=CARTESIAN_POINT('Ctrl Pts',(-10.9029637747341,-21.7258108748874,
0.));
#228936=CARTESIAN_POINT('Ctrl Pts',(-10.9201323997386,-21.74093105488,0.));
#228937=CARTESIAN_POINT('Ctrl Pts',(-10.9374082827446,-21.7560688175252,
0.));
#228938=CARTESIAN_POINT('Ctrl Pts',(-10.9547911664457,-21.7712234908468,
0.));
#228939=CARTESIAN_POINT('Ctrl Pts',(-10.9722807946157,-21.7863944097143,
0.));
#228940=CARTESIAN_POINT('Ctrl Pts',(-10.9898769120913,-21.8015809157302,
0.));
#228941=CARTESIAN_POINT('Ctrl Pts',(-11.0075792647477,-21.8167823571168,
0.));
#228942=CARTESIAN_POINT('Ctrl Pts',(-11.0253875994598,-21.8319980886033,
0.));
#228943=CARTESIAN_POINT('Ctrl Pts',(-11.0433016640808,-21.8472274713103,
0.));
#228944=CARTESIAN_POINT('Ctrl Pts',(-11.0613212074364,-21.8624698726319,
0.));
#228945=CARTESIAN_POINT('Ctrl Pts',(-11.0794459793058,-21.8777246661191,
0.));
#228946=CARTESIAN_POINT('Ctrl Pts',(-11.0976757303944,-21.8929912313608,
0.));
#228947=CARTESIAN_POINT('Ctrl Pts',(-11.1160102123024,-21.9082689538687,
0.));
#228948=CARTESIAN_POINT('Ctrl Pts',(-11.134449177474,-21.9235572249518,
0.));
#228949=CARTESIAN_POINT('Ctrl Pts',(-11.1529923792002,-21.9388554416437,
0.));
#228950=CARTESIAN_POINT('Ctrl Pts',(-11.1716395716375,-21.9541630066504,
0.));
#228951=CARTESIAN_POINT('Ctrl Pts',(-11.190390509811,-21.9694793282913,
0.));
#228952=CARTESIAN_POINT('Ctrl Pts',(-11.2092449496125,-21.9848038204439,
0.));
#228953=CARTESIAN_POINT('Ctrl Pts',(-11.2282026477897,-22.0001359024839,
0.));
#228954=CARTESIAN_POINT('Ctrl Pts',(-11.2472633619276,-22.0154749992364,
0.));
#228955=CARTESIAN_POINT('Ctrl Pts',(-11.2664268504207,-22.0308205408351,
0.));
#228956=CARTESIAN_POINT('Ctrl Pts',(-11.2856928724374,-22.046171962566,
0.));
#228957=CARTESIAN_POINT('Ctrl Pts',(-11.3050611878771,-22.0615287047179,
0.));
#228958=CARTESIAN_POINT('Ctrl Pts',(-11.3245315573168,-22.0768902124267,
0.));
#228959=CARTESIAN_POINT('Ctrl Pts',(-11.3441037419553,-22.0922559355293,
0.));
#228960=CARTESIAN_POINT('Ctrl Pts',(-11.3637775035367,-22.1076253283978,
0.));
#228961=CARTESIAN_POINT('Ctrl Pts',(-11.3835526044256,-22.1229978500185,
0.));
#228962=CARTESIAN_POINT('Ctrl Pts',(-11.4034288076909,-22.1383729640963,
0.));
#228963=CARTESIAN_POINT('Ctrl Pts',(-11.4234058771742,-22.1537501391486,
0.));
#228964=CARTESIAN_POINT('Ctrl Pts',(-11.443483577557,-22.1691288486096,
0.));
#228965=CARTESIAN_POINT('Ctrl Pts',(-11.463661674411,-22.1845085709169,
0.));
#228966=CARTESIAN_POINT('Ctrl Pts',(-11.4839399342589,-22.1998887896435,
0.));
#228967=CARTESIAN_POINT('Ctrl Pts',(-11.504318124424,-22.215268993102,0.));
#228968=CARTESIAN_POINT('Ctrl Pts',(-11.5247960128476,-22.2306486738899,
0.));
#228969=CARTESIAN_POINT('Ctrl Pts',(-11.545373367912,-22.2460273284653,
0.));
#228970=CARTESIAN_POINT('Ctrl Pts',(-11.5660499582403,-22.2614044566898,
0.));
#228971=CARTESIAN_POINT('Ctrl Pts',(-11.5868255525189,-22.2767795614349,
0.));
#228972=CARTESIAN_POINT('Ctrl Pts',(-11.6076999192359,-22.2921521480357,
0.));
#228973=CARTESIAN_POINT('Ctrl Pts',(-11.6286728270011,-22.3075217249049,
0.));
#228974=CARTESIAN_POINT('Ctrl Pts',(-11.6497440449858,-22.3228878043976,
0.));
#228975=CARTESIAN_POINT('Ctrl Pts',(-11.6709133432986,-22.3382499035618,
0.));
#228976=CARTESIAN_POINT('Ctrl Pts',(-11.6921804934056,-22.3536075450028,
0.));
#228977=CARTESIAN_POINT('Ctrl Pts',(-11.7135452684532,-22.3689602575492,
0.));
#228978=CARTESIAN_POINT('Ctrl Pts',(-11.7350074437961,-22.3843075773905,
0.));
#228979=CARTESIAN_POINT('Ctrl Pts',(-11.7565667964765,-22.39964904692,0.));
#228980=CARTESIAN_POINT('Ctrl Pts',(-11.7782231042041,-22.4149842125018,
0.));
#228981=CARTESIAN_POINT('Ctrl Pts',(-11.7999761445175,-22.4303126226468,
0.));
#228982=CARTESIAN_POINT('Ctrl Pts',(-11.8218256937889,-22.4456338258738,
0.));
#228983=CARTESIAN_POINT('Ctrl Pts',(-11.8437715264487,-22.4609473690469,
0.));
#228984=CARTESIAN_POINT('Ctrl Pts',(-11.8658134137018,-22.4762527946694,
0.));
#228985=CARTESIAN_POINT('Ctrl Pts',(-11.8879511239941,-22.4915496418472,
0.));
#228986=CARTESIAN_POINT('Ctrl Pts',(-11.9101844254555,-22.5068374513958,
0.));
#228987=CARTESIAN_POINT('Ctrl Pts',(-11.9325130877801,-22.5221157697869,
0.));
#228988=CARTESIAN_POINT('Ctrl Pts',(-11.9549368843996,-22.5373841537299,
0.));
#228989=CARTESIAN_POINT('Ctrl Pts',(-11.9774555943496,-22.5526421741159,
0.));
#228990=CARTESIAN_POINT('Ctrl Pts',(-12.0000690046697,-22.5678894211194,
0.));
#228991=CARTESIAN_POINT('Ctrl Pts',(-12.0227769113132,-22.5831255061306,
0.));
#228992=CARTESIAN_POINT('Ctrl Pts',(-12.0455791139135,-22.5983500505675,
0.));
#228993=CARTESIAN_POINT('Ctrl Pts',(-12.0684754113869,-22.613562676493,
0.));
#228994=CARTESIAN_POINT('Ctrl Pts',(-12.0914655972828,-22.628762996708,
0.));
#228995=CARTESIAN_POINT('Ctrl Pts',(-12.1145494550384,-22.6439506046611,
0.));
#228996=CARTESIAN_POINT('Ctrl Pts',(-12.1377267537141,-22.6591250653942,
0.));
#228997=CARTESIAN_POINT('Ctrl Pts',(-12.1609972423089,-22.6742859034891,
0.));
#228998=CARTESIAN_POINT('Ctrl Pts',(-12.1843606579246,-22.6894326204959,
0.));
#228999=CARTESIAN_POINT('Ctrl Pts',(-12.2078167360267,-22.7045647168659,
0.));
#229000=CARTESIAN_POINT('Ctrl Pts',(-12.2313652198047,-22.7196817119299,
0.));
#229001=CARTESIAN_POINT('Ctrl Pts',(-12.2550058702389,-22.7347831655251,
0.));
#229002=CARTESIAN_POINT('Ctrl Pts',(-12.2787384750747,-22.7498686970096,
0.));
#229003=CARTESIAN_POINT('Ctrl Pts',(-12.3025628601812,-22.7649380101154,
0.));
#229004=CARTESIAN_POINT('Ctrl Pts',(-12.3264788926108,-22.7799908974947,
0.));
#229005=CARTESIAN_POINT('Ctrl Pts',(-12.3504864740361,-22.7950272216959,
0.));
#229006=CARTESIAN_POINT('Ctrl Pts',(-12.3745855366772,-22.8100469022632,
0.));
#229007=CARTESIAN_POINT('Ctrl Pts',(-12.393937937903,-22.8220493007353,
0.));
#229008=CARTESIAN_POINT('Ctrl Pts',(-12.4084933766366,-22.8310435872852,
0.));
#229009=CARTESIAN_POINT('Ctrl Pts',(-12.4182152851867,-22.8370364396497,
0.));
#229010=CARTESIAN_POINT('Ctrl Pts',(-12.4230808101438,-22.8400320311648,
0.));
#229011=CARTESIAN_POINT('',(-12.4230808101438,-22.8400320311648,12.));
#229012=CARTESIAN_POINT('Ctrl Pts',(-12.4230808101438,-22.8400320311648,
12.));
#229013=CARTESIAN_POINT('Ctrl Pts',(-12.4182152851867,-22.8370364396497,
12.));
#229014=CARTESIAN_POINT('Ctrl Pts',(-12.4084933766366,-22.8310435872852,
12.));
#229015=CARTESIAN_POINT('Ctrl Pts',(-12.393937937903,-22.8220493007353,
12.));
#229016=CARTESIAN_POINT('Ctrl Pts',(-12.3745855366772,-22.8100469022632,
12.));
#229017=CARTESIAN_POINT('Ctrl Pts',(-12.3504864740361,-22.7950272216959,
12.));
#229018=CARTESIAN_POINT('Ctrl Pts',(-12.3264788926108,-22.7799908974947,
12.));
#229019=CARTESIAN_POINT('Ctrl Pts',(-12.3025628601812,-22.7649380101154,
12.));
#229020=CARTESIAN_POINT('Ctrl Pts',(-12.2787384750747,-22.7498686970096,
12.));
#229021=CARTESIAN_POINT('Ctrl Pts',(-12.2550058702389,-22.7347831655251,
12.));
#229022=CARTESIAN_POINT('Ctrl Pts',(-12.2313652198047,-22.7196817119299,
12.));
#229023=CARTESIAN_POINT('Ctrl Pts',(-12.2078167360267,-22.7045647168659,
12.));
#229024=CARTESIAN_POINT('Ctrl Pts',(-12.1843606579246,-22.6894326204959,
12.));
#229025=CARTESIAN_POINT('Ctrl Pts',(-12.1609972423089,-22.6742859034891,
12.));
#229026=CARTESIAN_POINT('Ctrl Pts',(-12.1377267537141,-22.6591250653942,
12.));
#229027=CARTESIAN_POINT('Ctrl Pts',(-12.1145494550384,-22.6439506046611,
12.));
#229028=CARTESIAN_POINT('Ctrl Pts',(-12.0914655972828,-22.628762996708,
12.));
#229029=CARTESIAN_POINT('Ctrl Pts',(-12.0684754113869,-22.613562676493,
12.));
#229030=CARTESIAN_POINT('Ctrl Pts',(-12.0455791139135,-22.5983500505675,
12.));
#229031=CARTESIAN_POINT('Ctrl Pts',(-12.0227769113132,-22.5831255061306,
12.));
#229032=CARTESIAN_POINT('Ctrl Pts',(-12.0000690046697,-22.5678894211194,
12.));
#229033=CARTESIAN_POINT('Ctrl Pts',(-11.9774555943496,-22.5526421741159,
12.));
#229034=CARTESIAN_POINT('Ctrl Pts',(-11.9549368843996,-22.5373841537299,
12.));
#229035=CARTESIAN_POINT('Ctrl Pts',(-11.9325130877801,-22.5221157697869,
12.));
#229036=CARTESIAN_POINT('Ctrl Pts',(-11.9101844254555,-22.5068374513958,
12.));
#229037=CARTESIAN_POINT('Ctrl Pts',(-11.8879511239941,-22.4915496418472,
12.));
#229038=CARTESIAN_POINT('Ctrl Pts',(-11.8658134137018,-22.4762527946694,
12.));
#229039=CARTESIAN_POINT('Ctrl Pts',(-11.8437715264487,-22.4609473690469,
12.));
#229040=CARTESIAN_POINT('Ctrl Pts',(-11.8218256937889,-22.4456338258738,
12.));
#229041=CARTESIAN_POINT('Ctrl Pts',(-11.7999761445175,-22.4303126226468,
12.));
#229042=CARTESIAN_POINT('Ctrl Pts',(-11.7782231042041,-22.4149842125018,
12.));
#229043=CARTESIAN_POINT('Ctrl Pts',(-11.7565667964765,-22.39964904692,12.));
#229044=CARTESIAN_POINT('Ctrl Pts',(-11.7350074437961,-22.3843075773905,
12.));
#229045=CARTESIAN_POINT('Ctrl Pts',(-11.7135452684532,-22.3689602575492,
12.));
#229046=CARTESIAN_POINT('Ctrl Pts',(-11.6921804934056,-22.3536075450028,
12.));
#229047=CARTESIAN_POINT('Ctrl Pts',(-11.6709133432986,-22.3382499035618,
12.));
#229048=CARTESIAN_POINT('Ctrl Pts',(-11.6497440449858,-22.3228878043976,
12.));
#229049=CARTESIAN_POINT('Ctrl Pts',(-11.6286728270011,-22.3075217249049,
12.));
#229050=CARTESIAN_POINT('Ctrl Pts',(-11.6076999192359,-22.2921521480357,
12.));
#229051=CARTESIAN_POINT('Ctrl Pts',(-11.5868255525189,-22.2767795614349,
12.));
#229052=CARTESIAN_POINT('Ctrl Pts',(-11.5660499582403,-22.2614044566898,
12.));
#229053=CARTESIAN_POINT('Ctrl Pts',(-11.545373367912,-22.2460273284653,
12.));
#229054=CARTESIAN_POINT('Ctrl Pts',(-11.5247960128476,-22.2306486738899,
12.));
#229055=CARTESIAN_POINT('Ctrl Pts',(-11.504318124424,-22.215268993102,12.));
#229056=CARTESIAN_POINT('Ctrl Pts',(-11.4839399342589,-22.1998887896435,
12.));
#229057=CARTESIAN_POINT('Ctrl Pts',(-11.463661674411,-22.1845085709169,
12.));
#229058=CARTESIAN_POINT('Ctrl Pts',(-11.443483577557,-22.1691288486096,
12.));
#229059=CARTESIAN_POINT('Ctrl Pts',(-11.4234058771742,-22.1537501391486,
12.));
#229060=CARTESIAN_POINT('Ctrl Pts',(-11.4034288076909,-22.1383729640963,
12.));
#229061=CARTESIAN_POINT('Ctrl Pts',(-11.3835526044256,-22.1229978500185,
12.));
#229062=CARTESIAN_POINT('Ctrl Pts',(-11.3637775035367,-22.1076253283978,
12.));
#229063=CARTESIAN_POINT('Ctrl Pts',(-11.3441037419553,-22.0922559355293,
12.));
#229064=CARTESIAN_POINT('Ctrl Pts',(-11.3245315573168,-22.0768902124267,
12.));
#229065=CARTESIAN_POINT('Ctrl Pts',(-11.3050611878771,-22.0615287047179,
12.));
#229066=CARTESIAN_POINT('Ctrl Pts',(-11.2856928724374,-22.046171962566,
12.));
#229067=CARTESIAN_POINT('Ctrl Pts',(-11.2664268504207,-22.0308205408351,
12.));
#229068=CARTESIAN_POINT('Ctrl Pts',(-11.2472633619276,-22.0154749992364,
12.));
#229069=CARTESIAN_POINT('Ctrl Pts',(-11.2282026477897,-22.0001359024839,
12.));
#229070=CARTESIAN_POINT('Ctrl Pts',(-11.2092449496125,-21.9848038204439,
12.));
#229071=CARTESIAN_POINT('Ctrl Pts',(-11.190390509811,-21.9694793282913,
12.));
#229072=CARTESIAN_POINT('Ctrl Pts',(-11.1716395716375,-21.9541630066504,
12.));
#229073=CARTESIAN_POINT('Ctrl Pts',(-11.1529923792002,-21.9388554416437,
12.));
#229074=CARTESIAN_POINT('Ctrl Pts',(-11.134449177474,-21.9235572249518,
12.));
#229075=CARTESIAN_POINT('Ctrl Pts',(-11.1160102123024,-21.9082689538687,
12.));
#229076=CARTESIAN_POINT('Ctrl Pts',(-11.0976757303944,-21.8929912313608,
12.));
#229077=CARTESIAN_POINT('Ctrl Pts',(-11.0794459793058,-21.8777246661191,
12.));
#229078=CARTESIAN_POINT('Ctrl Pts',(-11.0613212074364,-21.8624698726319,
12.));
#229079=CARTESIAN_POINT('Ctrl Pts',(-11.0433016640808,-21.8472274713103,
12.));
#229080=CARTESIAN_POINT('Ctrl Pts',(-11.0253875994598,-21.8319980886033,
12.));
#229081=CARTESIAN_POINT('Ctrl Pts',(-11.0075792647477,-21.8167823571168,
12.));
#229082=CARTESIAN_POINT('Ctrl Pts',(-10.9898769120913,-21.8015809157302,
12.));
#229083=CARTESIAN_POINT('Ctrl Pts',(-10.9722807946157,-21.7863944097143,
12.));
#229084=CARTESIAN_POINT('Ctrl Pts',(-10.9547911664457,-21.7712234908468,
12.));
#229085=CARTESIAN_POINT('Ctrl Pts',(-10.9374082827446,-21.7560688175252,
12.));
#229086=CARTESIAN_POINT('Ctrl Pts',(-10.9201323997386,-21.74093105488,12.));
#229087=CARTESIAN_POINT('Ctrl Pts',(-10.9029637747341,-21.7258108748874,
12.));
#229088=CARTESIAN_POINT('Ctrl Pts',(-10.8859026661292,-21.7107089564822,
12.));
#229089=CARTESIAN_POINT('Ctrl Pts',(-10.8689493334093,-21.6956259856667,
12.));
#229090=CARTESIAN_POINT('Ctrl Pts',(-10.8521040371832,-21.6805626556461,
12.));
#229091=CARTESIAN_POINT('Ctrl Pts',(-10.835367039227,-21.6655196669727,
12.));
#229092=CARTESIAN_POINT('Ctrl Pts',(-10.8187386025135,-21.6504977276864,
12.));
#229093=CARTESIAN_POINT('Ctrl Pts',(-10.802218991237,-21.6354975534557,
12.));
#229094=CARTESIAN_POINT('Ctrl Pts',(-10.7858084708262,-21.6205198677176,
12.));
#229095=CARTESIAN_POINT('Ctrl Pts',(-10.7695073079554,-21.6055654018179,
12.));
#229096=CARTESIAN_POINT('Ctrl Pts',(-10.7533157705943,-21.5906348951745,
12.));
#229097=CARTESIAN_POINT('Ctrl Pts',(-10.7372341280468,-21.5757290954372,
12.));
#229098=CARTESIAN_POINT('Ctrl Pts',(-10.7212626509816,-21.5608487586467,
12.));
#229099=CARTESIAN_POINT('Ctrl Pts',(-10.7054016114571,-21.5459946493955,
12.));
#229100=CARTESIAN_POINT('Ctrl Pts',(-10.689651282929,-21.531167540981,12.));
#229101=CARTESIAN_POINT('Ctrl Pts',(-10.6740119402835,-21.5163682155805,
12.));
#229102=CARTESIAN_POINT('Ctrl Pts',(-10.6584838598941,-21.5015974644454,
12.));
#229103=CARTESIAN_POINT('Ctrl Pts',(-10.6430673196609,-21.4868560880893,
12.));
#229104=CARTESIAN_POINT('Ctrl Pts',(-10.6277625990457,-21.4721448964766,
12.));
#229105=CARTESIAN_POINT('Ctrl Pts',(-10.612569979096,-21.4574647092093,
12.));
#229106=CARTESIAN_POINT('Ctrl Pts',(-10.597489742462,-21.4428163557137,
12.));
#229107=CARTESIAN_POINT('Ctrl Pts',(-10.582522173457,-21.4282006754624,
12.));
#229108=CARTESIAN_POINT('Ctrl Pts',(-10.5676675581106,-21.4136185181974,
12.));
#229109=CARTESIAN_POINT('Ctrl Pts',(-10.5529261842107,-21.3990707441495,
12.));
#229110=CARTESIAN_POINT('Ctrl Pts',(-10.5382983413422,-21.3845582242604,
12.));
#229111=CARTESIAN_POINT('Ctrl Pts',(-10.523784320906,-21.3700818403942,
12.));
#229112=CARTESIAN_POINT('Ctrl Pts',(-10.509384416169,-21.3556424855822,
12.));
#229113=CARTESIAN_POINT('Ctrl Pts',(-10.4950989223341,-21.3412410642912,
12.));
#229114=CARTESIAN_POINT('Ctrl Pts',(-10.4809281365933,-21.3268784926823,
12.));
#229115=CARTESIAN_POINT('Ctrl Pts',(-10.4668723581768,-21.312555698873,
12.));
#229116=CARTESIAN_POINT('Ctrl Pts',(-10.452931888387,-21.2982736231924,
12.));
#229117=CARTESIAN_POINT('Ctrl Pts',(-10.4391070306385,-21.2840332184471,
12.));
#229118=CARTESIAN_POINT('Ctrl Pts',(-10.4253980905394,-21.2698354502391,
12.));
#229119=CARTESIAN_POINT('Ctrl Pts',(-10.4118053759584,-21.2556812972741,
12.));
#229120=CARTESIAN_POINT('Ctrl Pts',(-10.3983291970846,-21.2415717516713,
12.));
#229121=CARTESIAN_POINT('Ctrl Pts',(-10.384969866479,-21.2275078192708,
12.));
#229122=CARTESIAN_POINT('Ctrl Pts',(-10.3717276991137,-21.2134905199359,
12.));
#229123=CARTESIAN_POINT('Ctrl Pts',(-10.3586030124595,-21.1995208879205,
12.));
#229124=CARTESIAN_POINT('Ctrl Pts',(-10.3455961265706,-21.1855999722427,
12.));
#229125=CARTESIAN_POINT('Ctrl Pts',(-10.3327073641574,-21.1717288370512,
12.));
#229126=CARTESIAN_POINT('Ctrl Pts',(-10.3199370506541,-21.1579085619959,
12.));
#229127=CARTESIAN_POINT('Ctrl Pts',(-10.307285514268,-21.1441402425831,
12.));
#229128=CARTESIAN_POINT('Ctrl Pts',(-10.2947530860714,-21.130424990599,
12.));
#229129=CARTESIAN_POINT('Ctrl Pts',(-10.2823401001067,-21.1167639345623,
12.));
#229130=CARTESIAN_POINT('Ctrl Pts',(-10.2700468934743,-21.1031582201625,
12.));
#229131=CARTESIAN_POINT('Ctrl Pts',(-10.2578738064183,-21.0896090107066,
12.));
#229132=CARTESIAN_POINT('Ctrl Pts',(-10.2458211823915,-21.0761174875448,
12.));
#229133=CARTESIAN_POINT('Ctrl Pts',(-10.233889368157,-21.0626848505665,
12.));
#229134=CARTESIAN_POINT('Ctrl Pts',(-10.2220787139157,-21.0493123187483,
12.));
#229135=CARTESIAN_POINT('Ctrl Pts',(-10.2103895734124,-21.0360011306814,
12.));
#229136=CARTESIAN_POINT('Ctrl Pts',(-10.1988223040425,-21.0227525451107,
12.));
#229137=CARTESIAN_POINT('Ctrl Pts',(-10.1873772669358,-21.0095678414486,
12.));
#229138=CARTESIAN_POINT('Ctrl Pts',(-10.1760548270765,-20.9964483203685,
12.));
#229139=CARTESIAN_POINT('Ctrl Pts',(-10.1648553534567,-20.9833953044736,
12.));
#229140=CARTESIAN_POINT('Ctrl Pts',(-10.1537792192065,-20.970410138937,
12.));
#229141=CARTESIAN_POINT('Ctrl Pts',(-10.1428268017257,-20.9574941921591,
12.));
#229142=CARTESIAN_POINT('Ctrl Pts',(-10.1319984827909,-20.944648856393,
12.));
#229143=CARTESIAN_POINT('Ctrl Pts',(-10.1212946487057,-20.931875548473,
12.));
#229144=CARTESIAN_POINT('Ctrl Pts',(-10.1107156904836,-20.9191757106266,
12.));
#229145=CARTESIAN_POINT('Ctrl Pts',(-10.1002620040076,-20.9065508112556,
12.));
#229146=CARTESIAN_POINT('Ctrl Pts',(-10.0899339901916,-20.8940023457371,
12.));
#229147=CARTESIAN_POINT('Ctrl Pts',(-10.0797320551154,-20.8815318371844,
12.));
#229148=CARTESIAN_POINT('Ctrl Pts',(-10.0696566102219,-20.8691408373705,
12.));
#229149=CARTESIAN_POINT('Ctrl Pts',(-10.0597080725375,-20.856830927732,
12.));
#229150=CARTESIAN_POINT('Ctrl Pts',(-10.0498868648733,-20.8446037203402,
12.));
#229151=CARTESIAN_POINT('Ctrl Pts',(-10.0401934160234,-20.8324608588906,
12.));
#229152=CARTESIAN_POINT('Ctrl Pts',(-10.0306281609435,-20.8204040196599,
12.));
#229153=CARTESIAN_POINT('Ctrl Pts',(-10.0211915410095,-20.8084349126885,
12.));
#229154=CARTESIAN_POINT('Ctrl Pts',(-10.0118840042786,-20.7965552829907,
12.));
#229155=CARTESIAN_POINT('Ctrl Pts',(-10.0027060057389,-20.7847669117568,
12.));
#229156=CARTESIAN_POINT('Ctrl Pts',(-9.99365800754638,-20.7730716175417,
12.));
#229157=CARTESIAN_POINT('Ctrl Pts',(-9.98474047926846,-20.7614712574989,
12.));
#229158=CARTESIAN_POINT('Ctrl Pts',(-9.97595389823461,-20.7499677289625,
12.));
#229159=CARTESIAN_POINT('Ctrl Pts',(-9.96729874986199,-20.7385629709795,
12.));
#229160=CARTESIAN_POINT('Ctrl Pts',(-9.95877552798403,-20.7272589658752,
12.));
#229161=CARTESIAN_POINT('Ctrl Pts',(-9.95038473514962,-20.716057740758,
12.));
#229162=CARTESIAN_POINT('Ctrl Pts',(-9.94212688298251,-20.7049613692237,
12.));
#229163=CARTESIAN_POINT('Ctrl Pts',(-9.93400249259737,-20.6939719732485,
12.));
#229164=CARTESIAN_POINT('Ctrl Pts',(-9.92601209498751,-20.6830917250255,
12.));
#229165=CARTESIAN_POINT('Ctrl Pts',(-9.91815623141285,-20.6723228488261,
12.));
#229166=CARTESIAN_POINT('Ctrl Pts',(-9.91043545377005,-20.6616676228315,
12.));
#229167=CARTESIAN_POINT('Ctrl Pts',(-9.90285032516696,-20.6511283817415,
12.));
#229168=CARTESIAN_POINT('Ctrl Pts',(-9.89540142049124,-20.6407075193977,
12.));
#229169=CARTESIAN_POINT('Ctrl Pts',(-9.88808932697305,-20.6304074914086,
12.));
#229170=CARTESIAN_POINT('Ctrl Pts',(-9.88091464472669,-20.6202308177472,
12.));
#229171=CARTESIAN_POINT('Ctrl Pts',(-9.87387798732944,-20.6101800854491,
12.));
#229172=CARTESIAN_POINT('Ctrl Pts',(-9.86697998242612,-20.6002579513696,
12.));
#229173=CARTESIAN_POINT('Ctrl Pts',(-9.8602212723275,-20.5904671449754,
12.));
#229174=CARTESIAN_POINT('Ctrl Pts',(-9.85360251457004,-20.580810471002,
12.));
#229175=CARTESIAN_POINT('Ctrl Pts',(-9.84712438256308,-20.5712908125145,
12.));
#229176=CARTESIAN_POINT('Ctrl Pts',(-9.84078756677589,-20.5619111362406,
12.));
#229177=CARTESIAN_POINT('Ctrl Pts',(-9.83459277585321,-20.5526744976461,
12.));
#229178=CARTESIAN_POINT('Ctrl Pts',(-9.82854073773858,-20.5435840460717,
12.));
#229179=CARTESIAN_POINT('Ctrl Pts',(-9.82263220080328,-20.534643029951,
12.));
#229180=CARTESIAN_POINT('Ctrl Pts',(-9.81686793455918,-20.5258548000625,
12.));
#229181=CARTESIAN_POINT('Ctrl Pts',(-9.81124873025278,-20.5172228122839,
12.));
#229182=CARTESIAN_POINT('Ctrl Pts',(-9.80577540161103,-20.5087506310507,
12.));
#229183=CARTESIAN_POINT('Ctrl Pts',(-9.80044878520968,-20.500441931211,
12.));
#229184=CARTESIAN_POINT('Ctrl Pts',(-9.79526974288344,-20.4923005087945,
12.));
#229185=CARTESIAN_POINT('Ctrl Pts',(-9.7902391649866,-20.4843302955329,
12.));
#229186=CARTESIAN_POINT('Ctrl Pts',(-9.78535797314162,-20.4765353711585,
12.));
#229187=CARTESIAN_POINT('Ctrl Pts',(-9.78062712373313,-20.4689199790668,
12.));
#229188=CARTESIAN_POINT('Ctrl Pts',(-9.77604760815523,-20.4614885274973,
12.));
#229189=CARTESIAN_POINT('Ctrl Pts',(-9.7716204510407,-20.4542455817527,
12.));
#229190=CARTESIAN_POINT('Ctrl Pts',(-9.76734670980897,-20.447195862298,
12.));
#229191=CARTESIAN_POINT('Ctrl Pts',(-9.76322747195502,-20.4403442329401,
12.));
#229192=CARTESIAN_POINT('Ctrl Pts',(-9.7592638628993,-20.4336957355474,
12.));
#229193=CARTESIAN_POINT('Ctrl Pts',(-9.75545705902416,-20.4272556476629,
12.));
#229194=CARTESIAN_POINT('Ctrl Pts',(-9.75180829786433,-20.4210295275818,
12.));
#229195=CARTESIAN_POINT('Ctrl Pts',(-9.74831889242175,-20.4150232777393,
12.));
#229196=CARTESIAN_POINT('Ctrl Pts',(-9.74499021838537,-20.4092430879861,
12.));
#229197=CARTESIAN_POINT('Ctrl Pts',(-9.74182369656273,-20.4036953576549,
12.));
#229198=CARTESIAN_POINT('Ctrl Pts',(-9.73882077613206,-20.3983866213331,
12.));
#229199=CARTESIAN_POINT('Ctrl Pts',(-9.7359829201425,-20.3933234845646,
12.));
#229200=CARTESIAN_POINT('Ctrl Pts',(-9.73331167102812,-20.3885129129912,
12.));
#229201=CARTESIAN_POINT('Ctrl Pts',(-9.73080870123726,-20.3839624556742,
12.));
#229202=CARTESIAN_POINT('Ctrl Pts',(-9.72847589116533,-20.3796805893304,
12.));
#229203=CARTESIAN_POINT('Ctrl Pts',(-9.72631531732871,-20.3756766651952,
12.));
#229204=CARTESIAN_POINT('Ctrl Pts',(-9.72432910043193,-20.371960235676,
12.));
#229205=CARTESIAN_POINT('Ctrl Pts',(-9.72251930722504,-20.3685406190576,
12.));
#229206=CARTESIAN_POINT('Ctrl Pts',(-9.72088778381102,-20.3654261611055,
12.));
#229207=CARTESIAN_POINT('Ctrl Pts',(-9.71943648548115,-20.362625691398,
12.));
#229208=CARTESIAN_POINT('Ctrl Pts',(-9.71816778327999,-20.3601498764344,
12.));
#229209=CARTESIAN_POINT('Ctrl Pts',(-9.71708493723062,-20.3580133103357,
12.));
#229210=CARTESIAN_POINT('Ctrl Pts',(-9.71619192554147,-20.3562337557875,
12.));
#229211=CARTESIAN_POINT('Ctrl Pts',(-9.71549257088175,-20.3548282742361,
12.));
#229212=CARTESIAN_POINT('Ctrl Pts',(-9.71498978052101,-20.3538098605706,
12.));
#229213=CARTESIAN_POINT('Ctrl Pts',(-9.71474590350792,-20.3533097561886,
12.));
#229214=CARTESIAN_POINT('Ctrl Pts',(-9.71465227853122,-20.3531126095522,
12.));
#229215=CARTESIAN_POINT('Ctrl Pts',(-9.71462954053074,-20.353060251684,
12.));
#229216=CARTESIAN_POINT('Ctrl Pts',(-9.71462809124917,-20.353053841303,
12.));
#229217=CARTESIAN_POINT('',(-12.4230808101438,-22.8400320311648,0.));
#229218=CARTESIAN_POINT('Origin',(-13.9675290154577,-16.3449727195351,0.));
#229219=CARTESIAN_POINT('',(-14.6513681262571,-17.1452095830632,12.));
#229220=CARTESIAN_POINT('',(-6.98376450772884,-8.17248635976757,12.));
#229221=CARTESIAN_POINT('',(-14.6513681262571,-17.1452095830632,0.));
#229222=CARTESIAN_POINT('',(-14.6513681262571,-17.1452095830632,0.));
#229223=CARTESIAN_POINT('',(-6.98376450772884,-8.17248635976757,0.));
#229224=CARTESIAN_POINT('Ctrl Pts',(-13.5685075571671,-22.1787195904339,
0.));
#229225=CARTESIAN_POINT('Ctrl Pts',(-13.5685075571671,-22.1787195904339,
12.));
#229226=CARTESIAN_POINT('Ctrl Pts',(-13.5683460612913,-22.1730081264583,
0.));
#229227=CARTESIAN_POINT('Ctrl Pts',(-13.5683460612913,-22.1730081264583,
12.));
#229228=CARTESIAN_POINT('Ctrl Pts',(-13.5680170531724,-22.1615922804939,
0.));
#229229=CARTESIAN_POINT('Ctrl Pts',(-13.5680170531724,-22.1615922804939,
12.));
#229230=CARTESIAN_POINT('Ctrl Pts',(-13.5675054918922,-22.1444897575076,
0.));
#229231=CARTESIAN_POINT('Ctrl Pts',(-13.5675054918922,-22.1444897575076,
12.));
#229232=CARTESIAN_POINT('Ctrl Pts',(-13.5667873105179,-22.1217288871823,
0.));
#229233=CARTESIAN_POINT('Ctrl Pts',(-13.5667873105179,-22.1217288871823,
12.));
#229234=CARTESIAN_POINT('Ctrl Pts',(-13.5658294169107,-22.0933486464442,
0.));
#229235=CARTESIAN_POINT('Ctrl Pts',(-13.5658294169107,-22.0933486464442,
12.));
#229236=CARTESIAN_POINT('Ctrl Pts',(-13.5648113688895,-22.0650393089492,
0.));
#229237=CARTESIAN_POINT('Ctrl Pts',(-13.5648113688895,-22.0650393089492,
12.));
#229238=CARTESIAN_POINT('Ctrl Pts',(-13.5637332022393,-22.0368009736227,
0.));
#229239=CARTESIAN_POINT('Ctrl Pts',(-13.5637332022393,-22.0368009736227,
12.));
#229240=CARTESIAN_POINT('Ctrl Pts',(-13.5625949868313,-22.0086337943431,
0.));
#229241=CARTESIAN_POINT('Ctrl Pts',(-13.5625949868313,-22.0086337943431,
12.));
#229242=CARTESIAN_POINT('Ctrl Pts',(-13.5613968357589,-21.9805379899192,
0.));
#229243=CARTESIAN_POINT('Ctrl Pts',(-13.5613968357589,-21.9805379899192,
12.));
#229244=CARTESIAN_POINT('Ctrl Pts',(-13.5601389185315,-21.9525138592862,
0.));
#229245=CARTESIAN_POINT('Ctrl Pts',(-13.5601389185315,-21.9525138592862,
12.));
#229246=CARTESIAN_POINT('Ctrl Pts',(-13.5588214586672,-21.9245617765827,
0.));
#229247=CARTESIAN_POINT('Ctrl Pts',(-13.5588214586672,-21.9245617765827,
12.));
#229248=CARTESIAN_POINT('Ctrl Pts',(-13.5574447178485,-21.8966821688876,
0.));
#229249=CARTESIAN_POINT('Ctrl Pts',(-13.5574447178485,-21.8966821688876,
12.));
#229250=CARTESIAN_POINT('Ctrl Pts',(-13.5560089839426,-21.8688754989401,
0.));
#229251=CARTESIAN_POINT('Ctrl Pts',(-13.5560089839426,-21.8688754989401,
12.));
#229252=CARTESIAN_POINT('Ctrl Pts',(-13.5545145573049,-21.841142245609,
0.));
#229253=CARTESIAN_POINT('Ctrl Pts',(-13.5545145573049,-21.841142245609,
12.));
#229254=CARTESIAN_POINT('Ctrl Pts',(-13.5529617381569,-21.8134828857963,
0.));
#229255=CARTESIAN_POINT('Ctrl Pts',(-13.5529617381569,-21.8134828857963,
12.));
#229256=CARTESIAN_POINT('Ctrl Pts',(-13.5513508127232,-21.7858978745848,
0.));
#229257=CARTESIAN_POINT('Ctrl Pts',(-13.5513508127232,-21.7858978745848,
12.));
#229258=CARTESIAN_POINT('Ctrl Pts',(-13.5496820422187,-21.7583876294532,
0.));
#229259=CARTESIAN_POINT('Ctrl Pts',(-13.5496820422187,-21.7583876294532,
12.));
#229260=CARTESIAN_POINT('Ctrl Pts',(-13.5479556704457,-21.730952541226,
0.));
#229261=CARTESIAN_POINT('Ctrl Pts',(-13.5479556704457,-21.730952541226,
12.));
#229262=CARTESIAN_POINT('Ctrl Pts',(-13.546171929503,-21.7035929822939,
0.));
#229263=CARTESIAN_POINT('Ctrl Pts',(-13.546171929503,-21.7035929822939,
12.));
#229264=CARTESIAN_POINT('Ctrl Pts',(-13.5443310461516,-21.676309315769,
0.));
#229265=CARTESIAN_POINT('Ctrl Pts',(-13.5443310461516,-21.676309315769,
12.));
#229266=CARTESIAN_POINT('Ctrl Pts',(-13.5424332480698,-21.6491019044647,
0.));
#229267=CARTESIAN_POINT('Ctrl Pts',(-13.5424332480698,-21.6491019044647,
12.));
#229268=CARTESIAN_POINT('Ctrl Pts',(-13.5404787697798,-21.6219711193951,
0.));
#229269=CARTESIAN_POINT('Ctrl Pts',(-13.5404787697798,-21.6219711193951,
12.));
#229270=CARTESIAN_POINT('Ctrl Pts',(-13.5384678597206,-21.5949173499022,
0.));
#229271=CARTESIAN_POINT('Ctrl Pts',(-13.5384678597206,-21.5949173499022,
12.));
#229272=CARTESIAN_POINT('Ctrl Pts',(-13.5364007790292,-21.5679410019011,
0.));
#229273=CARTESIAN_POINT('Ctrl Pts',(-13.5364007790292,-21.5679410019011,
12.));
#229274=CARTESIAN_POINT('Ctrl Pts',(-13.5342777983225,-21.5410424932511,
0.));
#229275=CARTESIAN_POINT('Ctrl Pts',(-13.5342777983225,-21.5410424932511,
12.));
#229276=CARTESIAN_POINT('Ctrl Pts',(-13.5320991952145,-21.5142222501671,
0.));
#229277=CARTESIAN_POINT('Ctrl Pts',(-13.5320991952145,-21.5142222501671,
12.));
#229278=CARTESIAN_POINT('Ctrl Pts',(-13.5298652514357,-21.487480703047,
0.));
#229279=CARTESIAN_POINT('Ctrl Pts',(-13.5298652514357,-21.487480703047,
12.));
#229280=CARTESIAN_POINT('Ctrl Pts',(-13.5275762503553,-21.4608182828695,
0.));
#229281=CARTESIAN_POINT('Ctrl Pts',(-13.5275762503553,-21.4608182828695,
12.));
#229282=CARTESIAN_POINT('Ctrl Pts',(-13.5252324737795,-21.4342354165253,
0.));
#229283=CARTESIAN_POINT('Ctrl Pts',(-13.5252324737795,-21.4342354165253,
12.));
#229284=CARTESIAN_POINT('Ctrl Pts',(-13.5228342013508,-21.4077325259318,
0.));
#229285=CARTESIAN_POINT('Ctrl Pts',(-13.5228342013508,-21.4077325259318,
12.));
#229286=CARTESIAN_POINT('Ctrl Pts',(-13.5203817122497,-21.3813100304967,
0.));
#229287=CARTESIAN_POINT('Ctrl Pts',(-13.5203817122497,-21.3813100304967,
12.));
#229288=CARTESIAN_POINT('Ctrl Pts',(-13.5178752862461,-21.3549683486219,
0.));
#229289=CARTESIAN_POINT('Ctrl Pts',(-13.5178752862461,-21.3549683486219,
12.));
#229290=CARTESIAN_POINT('Ctrl Pts',(-13.5153152050554,-21.328707899634,
0.));
#229291=CARTESIAN_POINT('Ctrl Pts',(-13.5153152050554,-21.328707899634,
12.));
#229292=CARTESIAN_POINT('Ctrl Pts',(-13.5127017534972,-21.3025291054236,
0.));
#229293=CARTESIAN_POINT('Ctrl Pts',(-13.5127017534972,-21.3025291054236,
12.));
#229294=CARTESIAN_POINT('Ctrl Pts',(-13.5100352209207,-21.2764323924442,
0.));
#229295=CARTESIAN_POINT('Ctrl Pts',(-13.5100352209207,-21.2764323924442,
12.));
#229296=CARTESIAN_POINT('Ctrl Pts',(-13.5073159019454,-21.2504181927429,
0.));
#229297=CARTESIAN_POINT('Ctrl Pts',(-13.5073159019454,-21.2504181927429,
12.));
#229298=CARTESIAN_POINT('Ctrl Pts',(-13.5045440957404,-21.224486942933,
0.));
#229299=CARTESIAN_POINT('Ctrl Pts',(-13.5045440957404,-21.224486942933,
12.));
#229300=CARTESIAN_POINT('Ctrl Pts',(-13.5017201056088,-21.1986390835825,
0.));
#229301=CARTESIAN_POINT('Ctrl Pts',(-13.5017201056088,-21.1986390835825,
12.));
#229302=CARTESIAN_POINT('Ctrl Pts',(-13.4988442384491,-21.1728750584173,
0.));
#229303=CARTESIAN_POINT('Ctrl Pts',(-13.4988442384491,-21.1728750584173,
12.));
#229304=CARTESIAN_POINT('Ctrl Pts',(-13.4959168042934,-21.1471953136209,
0.));
#229305=CARTESIAN_POINT('Ctrl Pts',(-13.4959168042934,-21.1471953136209,
12.));
#229306=CARTESIAN_POINT('Ctrl Pts',(-13.4929381157778,-21.1216002970209,
0.));
#229307=CARTESIAN_POINT('Ctrl Pts',(-13.4929381157778,-21.1216002970209,
12.));
#229308=CARTESIAN_POINT('Ctrl Pts',(-13.4899084877718,-21.0960904575048,
0.));
#229309=CARTESIAN_POINT('Ctrl Pts',(-13.4899084877718,-21.0960904575048,
12.));
#229310=CARTESIAN_POINT('Ctrl Pts',(-13.4868282377192,-21.0706662455202,
0.));
#229311=CARTESIAN_POINT('Ctrl Pts',(-13.4868282377192,-21.0706662455202,
12.));
#229312=CARTESIAN_POINT('Ctrl Pts',(-13.4836976858912,-21.0453281134247,
0.));
#229313=CARTESIAN_POINT('Ctrl Pts',(-13.4836976858912,-21.0453281134247,
12.));
#229314=CARTESIAN_POINT('Ctrl Pts',(-13.4805171556822,-21.0200765158885,
0.));
#229315=CARTESIAN_POINT('Ctrl Pts',(-13.4805171556822,-21.0200765158885,
12.));
#229316=CARTESIAN_POINT('Ctrl Pts',(-13.4772869738879,-20.9949119102592,
0.));
#229317=CARTESIAN_POINT('Ctrl Pts',(-13.4772869738879,-20.9949119102592,
12.));
#229318=CARTESIAN_POINT('Ctrl Pts',(-13.4740074710087,-20.9698347569476,
0.));
#229319=CARTESIAN_POINT('Ctrl Pts',(-13.4740074710087,-20.9698347569476,
12.));
#229320=CARTESIAN_POINT('Ctrl Pts',(-13.4706789815167,-20.9448455197557,
0.));
#229321=CARTESIAN_POINT('Ctrl Pts',(-13.4706789815167,-20.9448455197557,
12.));
#229322=CARTESIAN_POINT('Ctrl Pts',(-13.4673018437718,-20.9199446657584,
0.));
#229323=CARTESIAN_POINT('Ctrl Pts',(-13.4673018437718,-20.9199446657584,
12.));
#229324=CARTESIAN_POINT('Ctrl Pts',(-13.4638763999726,-20.8951326652158,
0.));
#229325=CARTESIAN_POINT('Ctrl Pts',(-13.4638763999726,-20.8951326652158,
12.));
#229326=CARTESIAN_POINT('Ctrl Pts',(-13.4604029960983,-20.8704099914641,
0.));
#229327=CARTESIAN_POINT('Ctrl Pts',(-13.4604029960983,-20.8704099914641,
12.));
#229328=CARTESIAN_POINT('Ctrl Pts',(-13.4568819818631,-20.8457771208082,
0.));
#229329=CARTESIAN_POINT('Ctrl Pts',(-13.4568819818631,-20.8457771208082,
12.));
#229330=CARTESIAN_POINT('Ctrl Pts',(-13.4533137106667,-20.821234532398,
0.));
#229331=CARTESIAN_POINT('Ctrl Pts',(-13.4533137106667,-20.821234532398,
12.));
#229332=CARTESIAN_POINT('Ctrl Pts',(-13.4496985395637,-20.7967827081227,
0.));
#229333=CARTESIAN_POINT('Ctrl Pts',(-13.4496985395637,-20.7967827081227,
12.));
#229334=CARTESIAN_POINT('Ctrl Pts',(-13.4460368293688,-20.7724221327608,
0.));
#229335=CARTESIAN_POINT('Ctrl Pts',(-13.4460368293688,-20.7724221327608,
12.));
#229336=CARTESIAN_POINT('Ctrl Pts',(-13.4423289447561,-20.7481532941013,
0.));
#229337=CARTESIAN_POINT('Ctrl Pts',(-13.4423289447561,-20.7481532941013,
12.));
#229338=CARTESIAN_POINT('Ctrl Pts',(-13.4385752543663,-20.7239766830675,
0.));
#229339=CARTESIAN_POINT('Ctrl Pts',(-13.4385752543663,-20.7239766830675,
12.));
#229340=CARTESIAN_POINT('Ctrl Pts',(-13.4347761309154,-20.6998927938288,
0.));
#229341=CARTESIAN_POINT('Ctrl Pts',(-13.4347761309154,-20.6998927938288,
12.));
#229342=CARTESIAN_POINT('Ctrl Pts',(-13.4309319513119,-20.6759021239103,
0.));
#229343=CARTESIAN_POINT('Ctrl Pts',(-13.4309319513119,-20.6759021239103,
12.));
#229344=CARTESIAN_POINT('Ctrl Pts',(-13.4270430967652,-20.6520051742869,
0.));
#229345=CARTESIAN_POINT('Ctrl Pts',(-13.4270430967652,-20.6520051742869,
12.));
#229346=CARTESIAN_POINT('Ctrl Pts',(-13.4231099528179,-20.6282024494237,
0.));
#229347=CARTESIAN_POINT('Ctrl Pts',(-13.4231099528179,-20.6282024494237,
12.));
#229348=CARTESIAN_POINT('Ctrl Pts',(-13.4191329093933,-20.6044944573153,
0.));
#229349=CARTESIAN_POINT('Ctrl Pts',(-13.4191329093933,-20.6044944573153,
12.));
#229350=CARTESIAN_POINT('Ctrl Pts',(-13.4151123608411,-20.5808817095155,
0.));
#229351=CARTESIAN_POINT('Ctrl Pts',(-13.4151123608411,-20.5808817095155,
12.));
#229352=CARTESIAN_POINT('Ctrl Pts',(-13.4110487059912,-20.5573647211639,
0.));
#229353=CARTESIAN_POINT('Ctrl Pts',(-13.4110487059912,-20.5573647211639,
12.));
#229354=CARTESIAN_POINT('Ctrl Pts',(-13.4069423482076,-20.5339440109956,
0.));
#229355=CARTESIAN_POINT('Ctrl Pts',(-13.4069423482076,-20.5339440109956,
12.));
#229356=CARTESIAN_POINT('Ctrl Pts',(-13.4027936954529,-20.5106201013753,
0.));
#229357=CARTESIAN_POINT('Ctrl Pts',(-13.4027936954529,-20.5106201013753,
12.));
#229358=CARTESIAN_POINT('Ctrl Pts',(-13.3986031603716,-20.487393518404,
0.));
#229359=CARTESIAN_POINT('Ctrl Pts',(-13.3986031603716,-20.487393518404,
12.));
#229360=CARTESIAN_POINT('Ctrl Pts',(-13.3943711603739,-20.4642647920037,
0.));
#229361=CARTESIAN_POINT('Ctrl Pts',(-13.3943711603739,-20.4642647920037,
12.));
#229362=CARTESIAN_POINT('Ctrl Pts',(-13.3900981177255,-20.4412344560007,
0.));
#229363=CARTESIAN_POINT('Ctrl Pts',(-13.3900981177255,-20.4412344560007,
12.));
#229364=CARTESIAN_POINT('Ctrl Pts',(-13.3857844596387,-20.4183030482002,
0.));
#229365=CARTESIAN_POINT('Ctrl Pts',(-13.3857844596387,-20.4183030482002,
12.));
#229366=CARTESIAN_POINT('Ctrl Pts',(-13.3814306183719,-20.3954711104502,
0.));
#229367=CARTESIAN_POINT('Ctrl Pts',(-13.3814306183719,-20.3954711104502,
12.));
#229368=CARTESIAN_POINT('Ctrl Pts',(-13.3770370313188,-20.3727391887184,
0.));
#229369=CARTESIAN_POINT('Ctrl Pts',(-13.3770370313188,-20.3727391887184,
12.));
#229370=CARTESIAN_POINT('Ctrl Pts',(-13.3726041410867,-20.3501078331814,
0.));
#229371=CARTESIAN_POINT('Ctrl Pts',(-13.3726041410867,-20.3501078331814,
12.));
#229372=CARTESIAN_POINT('Ctrl Pts',(-13.3681323955826,-20.3275775983029,
0.));
#229373=CARTESIAN_POINT('Ctrl Pts',(-13.3681323955826,-20.3275775983029,
12.));
#229374=CARTESIAN_POINT('Ctrl Pts',(-13.3636222481016,-20.3051490429048,
0.));
#229375=CARTESIAN_POINT('Ctrl Pts',(-13.3636222481016,-20.3051490429048,
12.));
#229376=CARTESIAN_POINT('Ctrl Pts',(-13.3590741574195,-20.2828227302339,
0.));
#229377=CARTESIAN_POINT('Ctrl Pts',(-13.3590741574195,-20.2828227302339,
12.));
#229378=CARTESIAN_POINT('Ctrl Pts',(-13.3544885878889,-20.2605992280122,
0.));
#229379=CARTESIAN_POINT('Ctrl Pts',(-13.3544885878889,-20.2605992280122,
12.));
#229380=CARTESIAN_POINT('Ctrl Pts',(-13.3498660095386,-20.2384791085359,
0.));
#229381=CARTESIAN_POINT('Ctrl Pts',(-13.3498660095386,-20.2384791085359,
12.));
#229382=CARTESIAN_POINT('Ctrl Pts',(-13.3452068981766,-20.216462948786,
0.));
#229383=CARTESIAN_POINT('Ctrl Pts',(-13.3452068981766,-20.216462948786,
12.));
#229384=CARTESIAN_POINT('Ctrl Pts',(-13.3405117354971,-20.1945513305235,
0.));
#229385=CARTESIAN_POINT('Ctrl Pts',(-13.3405117354971,-20.1945513305235,
12.));
#229386=CARTESIAN_POINT('Ctrl Pts',(-13.3357810091903,-20.1727448403817,
0.));
#229387=CARTESIAN_POINT('Ctrl Pts',(-13.3357810091903,-20.1727448403817,
12.));
#229388=CARTESIAN_POINT('Ctrl Pts',(-13.3310152130564,-20.1510440699474,
0.));
#229389=CARTESIAN_POINT('Ctrl Pts',(-13.3310152130564,-20.1510440699474,
12.));
#229390=CARTESIAN_POINT('Ctrl Pts',(-13.3262148471226,-20.1294496158402,
0.));
#229391=CARTESIAN_POINT('Ctrl Pts',(-13.3262148471226,-20.1294496158402,
12.));
#229392=CARTESIAN_POINT('Ctrl Pts',(-13.3213804177587,-20.1079620798375,
0.));
#229393=CARTESIAN_POINT('Ctrl Pts',(-13.3213804177587,-20.1079620798375,
12.));
#229394=CARTESIAN_POINT('Ctrl Pts',(-13.3165124377963,-20.0865820689882,
0.));
#229395=CARTESIAN_POINT('Ctrl Pts',(-13.3165124377963,-20.0865820689882,
12.));
#229396=CARTESIAN_POINT('Ctrl Pts',(-13.3116114266515,-20.0653101957188,
0.));
#229397=CARTESIAN_POINT('Ctrl Pts',(-13.3116114266515,-20.0653101957188,
12.));
#229398=CARTESIAN_POINT('Ctrl Pts',(-13.3066779104515,-20.0441470779345,
0.));
#229399=CARTESIAN_POINT('Ctrl Pts',(-13.3066779104515,-20.0441470779345,
12.));
#229400=CARTESIAN_POINT('Ctrl Pts',(-13.3017124221637,-20.0230933391038,
0.));
#229401=CARTESIAN_POINT('Ctrl Pts',(-13.3017124221637,-20.0230933391038,
12.));
#229402=CARTESIAN_POINT('Ctrl Pts',(-13.2967155017306,-20.0021496083738,
0.));
#229403=CARTESIAN_POINT('Ctrl Pts',(-13.2967155017306,-20.0021496083738,
12.));
#229404=CARTESIAN_POINT('Ctrl Pts',(-13.2916876962094,-19.981316520717,
0.));
#229405=CARTESIAN_POINT('Ctrl Pts',(-13.2916876962094,-19.981316520717,
12.));
#229406=CARTESIAN_POINT('Ctrl Pts',(-13.286629559915,-19.9605947170586,
0.));
#229407=CARTESIAN_POINT('Ctrl Pts',(-13.286629559915,-19.9605947170586,
12.));
#229408=CARTESIAN_POINT('Ctrl Pts',(-13.2815416545663,-19.9399848444019,
0.));
#229409=CARTESIAN_POINT('Ctrl Pts',(-13.2815416545663,-19.9399848444019,
12.));
#229410=CARTESIAN_POINT('Ctrl Pts',(-13.2764245494357,-19.9194875559422,
0.));
#229411=CARTESIAN_POINT('Ctrl Pts',(-13.2764245494357,-19.9194875559422,
12.));
#229412=CARTESIAN_POINT('Ctrl Pts',(-13.271278821502,-19.8991035111745,
0.));
#229413=CARTESIAN_POINT('Ctrl Pts',(-13.271278821502,-19.8991035111745,
12.));
#229414=CARTESIAN_POINT('Ctrl Pts',(-13.2661050556132,-19.8788333760577,
0.));
#229415=CARTESIAN_POINT('Ctrl Pts',(-13.2661050556132,-19.8788333760577,
12.));
#229416=CARTESIAN_POINT('Ctrl Pts',(-13.2609038446529,-19.8586778231715,
0.));
#229417=CARTESIAN_POINT('Ctrl Pts',(-13.2609038446529,-19.8586778231715,
12.));
#229418=CARTESIAN_POINT('Ctrl Pts',(-13.2556757897086,-19.8386375318634,
0.));
#229419=CARTESIAN_POINT('Ctrl Pts',(-13.2556757897086,-19.8386375318634,
12.));
#229420=CARTESIAN_POINT('Ctrl Pts',(-13.2504215002457,-19.8187131883917,
0.));
#229421=CARTESIAN_POINT('Ctrl Pts',(-13.2504215002457,-19.8187131883917,
12.));
#229422=CARTESIAN_POINT('Ctrl Pts',(-13.2451415942805,-19.7989054860495,
0.));
#229423=CARTESIAN_POINT('Ctrl Pts',(-13.2451415942805,-19.7989054860495,
12.));
#229424=CARTESIAN_POINT('Ctrl Pts',(-13.2398366985675,-19.7792151253289,
0.));
#229425=CARTESIAN_POINT('Ctrl Pts',(-13.2398366985675,-19.7792151253289,
12.));
#229426=CARTESIAN_POINT('Ctrl Pts',(-13.2345074487963,-19.7596428141168,
0.));
#229427=CARTESIAN_POINT('Ctrl Pts',(-13.2345074487963,-19.7596428141168,
12.));
#229428=CARTESIAN_POINT('Ctrl Pts',(-13.2291544897899,-19.7401892678697,
0.));
#229429=CARTESIAN_POINT('Ctrl Pts',(-13.2291544897899,-19.7401892678697,
12.));
#229430=CARTESIAN_POINT('Ctrl Pts',(-13.2237784757066,-19.7208552097868,
0.));
#229431=CARTESIAN_POINT('Ctrl Pts',(-13.2237784757066,-19.7208552097868,
12.));
#229432=CARTESIAN_POINT('Ctrl Pts',(-13.2183800702436,-19.7016413709685,
0.));
#229433=CARTESIAN_POINT('Ctrl Pts',(-13.2183800702436,-19.7016413709685,
12.));
#229434=CARTESIAN_POINT('Ctrl Pts',(-13.2129599468485,-19.6825484905823,
0.));
#229435=CARTESIAN_POINT('Ctrl Pts',(-13.2129599468485,-19.6825484905823,
12.));
#229436=CARTESIAN_POINT('Ctrl Pts',(-13.2075187889529,-19.6635773160936,
0.));
#229437=CARTESIAN_POINT('Ctrl Pts',(-13.2075187889529,-19.6635773160936,
12.));
#229438=CARTESIAN_POINT('Ctrl Pts',(-13.2020572902065,-19.6447286034772,
0.));
#229439=CARTESIAN_POINT('Ctrl Pts',(-13.2020572902065,-19.6447286034772,
12.));
#229440=CARTESIAN_POINT('Ctrl Pts',(-13.1965761547151,-19.6260031174244,
0.));
#229441=CARTESIAN_POINT('Ctrl Pts',(-13.1965761547151,-19.6260031174244,
12.));
#229442=CARTESIAN_POINT('Ctrl Pts',(-13.1910760972814,-19.6074016315414,
0.));
#229443=CARTESIAN_POINT('Ctrl Pts',(-13.1910760972814,-19.6074016315414,
12.));
#229444=CARTESIAN_POINT('Ctrl Pts',(-13.1855578436471,-19.5889249285338,
0.));
#229445=CARTESIAN_POINT('Ctrl Pts',(-13.1855578436471,-19.5889249285338,
12.));
#229446=CARTESIAN_POINT('Ctrl Pts',(-13.1800221307673,-19.5705738004667,
0.));
#229447=CARTESIAN_POINT('Ctrl Pts',(-13.1800221307673,-19.5705738004667,
12.));
#229448=CARTESIAN_POINT('Ctrl Pts',(-13.1744697070911,-19.5523490490244,
0.));
#229449=CARTESIAN_POINT('Ctrl Pts',(-13.1744697070911,-19.5523490490244,
12.));
#229450=CARTESIAN_POINT('Ctrl Pts',(-13.1689013328431,-19.5342514857562,
0.));
#229451=CARTESIAN_POINT('Ctrl Pts',(-13.1689013328431,-19.5342514857562,
12.));
#229452=CARTESIAN_POINT('Ctrl Pts',(-13.1633177803101,-19.5162819323213,
0.));
#229453=CARTESIAN_POINT('Ctrl Pts',(-13.1633177803101,-19.5162819323213,
12.));
#229454=CARTESIAN_POINT('Ctrl Pts',(-13.1577198341245,-19.4984412207081,
0.));
#229455=CARTESIAN_POINT('Ctrl Pts',(-13.1577198341245,-19.4984412207081,
12.));
#229456=CARTESIAN_POINT('Ctrl Pts',(-13.1521082915853,-19.4807301935268,
0.));
#229457=CARTESIAN_POINT('Ctrl Pts',(-13.1521082915853,-19.4807301935268,
12.));
#229458=CARTESIAN_POINT('Ctrl Pts',(-13.1464839629971,-19.4631497043258,
0.));
#229459=CARTESIAN_POINT('Ctrl Pts',(-13.1464839629971,-19.4631497043258,
12.));
#229460=CARTESIAN_POINT('Ctrl Pts',(-13.1408476720061,-19.4457006178876,
0.));
#229461=CARTESIAN_POINT('Ctrl Pts',(-13.1408476720061,-19.4457006178876,
12.));
#229462=CARTESIAN_POINT('Ctrl Pts',(-13.1352002559438,-19.4283838105262,
0.));
#229463=CARTESIAN_POINT('Ctrl Pts',(-13.1352002559438,-19.4283838105262,
12.));
#229464=CARTESIAN_POINT('Ctrl Pts',(-13.1295425661634,-19.4112001703557,
0.));
#229465=CARTESIAN_POINT('Ctrl Pts',(-13.1295425661634,-19.4112001703557,
12.));
#229466=CARTESIAN_POINT('Ctrl Pts',(-13.1238754684177,-19.3941505976263,
0.));
#229467=CARTESIAN_POINT('Ctrl Pts',(-13.1238754684177,-19.3941505976263,
12.));
#229468=CARTESIAN_POINT('Ctrl Pts',(-13.118199843271,-19.3772360051091,
0.));
#229469=CARTESIAN_POINT('Ctrl Pts',(-13.118199843271,-19.3772360051091,
12.));
#229470=CARTESIAN_POINT('Ctrl Pts',(-13.1125165865022,-19.3604573184515,
0.));
#229471=CARTESIAN_POINT('Ctrl Pts',(-13.1125165865022,-19.3604573184515,
12.));
#229472=CARTESIAN_POINT('Ctrl Pts',(-13.1068266095186,-19.3438154765395,
0.));
#229473=CARTESIAN_POINT('Ctrl Pts',(-13.1068266095186,-19.3438154765395,
12.));
#229474=CARTESIAN_POINT('Ctrl Pts',(-13.1011308397591,-19.3273114318269,
0.));
#229475=CARTESIAN_POINT('Ctrl Pts',(-13.1011308397591,-19.3273114318269,
12.));
#229476=CARTESIAN_POINT('Ctrl Pts',(-13.0954302211479,-19.310946150736,
0.));
#229477=CARTESIAN_POINT('Ctrl Pts',(-13.0954302211479,-19.310946150736,
12.));
#229478=CARTESIAN_POINT('Ctrl Pts',(-13.0897257145969,-19.2947206141247,
0.));
#229479=CARTESIAN_POINT('Ctrl Pts',(-13.0897257145969,-19.2947206141247,
12.));
#229480=CARTESIAN_POINT('Ctrl Pts',(-13.0840182984949,-19.2786358177198,
0.));
#229481=CARTESIAN_POINT('Ctrl Pts',(-13.0840182984949,-19.2786358177198,
12.));
#229482=CARTESIAN_POINT('Ctrl Pts',(-13.0783089692118,-19.2626927725596,
0.));
#229483=CARTESIAN_POINT('Ctrl Pts',(-13.0783089692118,-19.2626927725596,
12.));
#229484=CARTESIAN_POINT('Ctrl Pts',(-13.0725987415859,-19.2468925053989,
0.));
#229485=CARTESIAN_POINT('Ctrl Pts',(-13.0725987415859,-19.2468925053989,
12.));
#229486=CARTESIAN_POINT('Ctrl Pts',(-13.0668886494795,-19.2312360592033,
0.));
#229487=CARTESIAN_POINT('Ctrl Pts',(-13.0668886494795,-19.2312360592033,
12.));
#229488=CARTESIAN_POINT('Ctrl Pts',(-13.0611797463915,-19.2157244937142,
0.));
#229489=CARTESIAN_POINT('Ctrl Pts',(-13.0611797463915,-19.2157244937142,
12.));
#229490=CARTESIAN_POINT('Ctrl Pts',(-13.0554731060538,-19.2003588859772,
0.));
#229491=CARTESIAN_POINT('Ctrl Pts',(-13.0554731060538,-19.2003588859772,
12.));
#229492=CARTESIAN_POINT('Ctrl Pts',(-13.0497698230441,-19.1851403308825,
0.));
#229493=CARTESIAN_POINT('Ctrl Pts',(-13.0497698230441,-19.1851403308825,
12.));
#229494=CARTESIAN_POINT('Ctrl Pts',(-13.0440710133772,-19.1700699416622,
0.));
#229495=CARTESIAN_POINT('Ctrl Pts',(-13.0440710133772,-19.1700699416622,
12.));
#229496=CARTESIAN_POINT('Ctrl Pts',(-13.0383778152068,-19.155148850523,
0.));
#229497=CARTESIAN_POINT('Ctrl Pts',(-13.0383778152068,-19.155148850523,
12.));
#229498=CARTESIAN_POINT('Ctrl Pts',(-13.0326913895838,-19.1403782093386,
0.));
#229499=CARTESIAN_POINT('Ctrl Pts',(-13.0326913895838,-19.1403782093386,
12.));
#229500=CARTESIAN_POINT('Ctrl Pts',(-13.0270129211976,-19.1257591903099,
0.));
#229501=CARTESIAN_POINT('Ctrl Pts',(-13.0270129211976,-19.1257591903099,
12.));
#229502=CARTESIAN_POINT('Ctrl Pts',(-13.0213436191328,-19.111292986631,
0.));
#229503=CARTESIAN_POINT('Ctrl Pts',(-13.0213436191328,-19.111292986631,
12.));
#229504=CARTESIAN_POINT('Ctrl Pts',(-13.0156847176097,-19.0969808131228,
0.));
#229505=CARTESIAN_POINT('Ctrl Pts',(-13.0156847176097,-19.0969808131228,
12.));
#229506=CARTESIAN_POINT('Ctrl Pts',(-13.0100374768788,-19.0828239070484,
0.));
#229507=CARTESIAN_POINT('Ctrl Pts',(-13.0100374768788,-19.0828239070484,
12.));
#229508=CARTESIAN_POINT('Ctrl Pts',(-13.0044031841382,-19.0688235289437,
0.));
#229509=CARTESIAN_POINT('Ctrl Pts',(-13.0044031841382,-19.0688235289437,
12.));
#229510=CARTESIAN_POINT('Ctrl Pts',(-12.9987831544502,-19.0549809634354,
0.));
#229511=CARTESIAN_POINT('Ctrl Pts',(-12.9987831544502,-19.0549809634354,
12.));
#229512=CARTESIAN_POINT('Ctrl Pts',(-12.9931787316514,-19.0412975200398,
0.));
#229513=CARTESIAN_POINT('Ctrl Pts',(-12.9931787316514,-19.0412975200398,
12.));
#229514=CARTESIAN_POINT('Ctrl Pts',(-12.9875912893003,-19.0277745339908,
0.));
#229515=CARTESIAN_POINT('Ctrl Pts',(-12.9875912893003,-19.0277745339908,
12.));
#229516=CARTESIAN_POINT('Ctrl Pts',(-12.9820222318716,-19.014413367335,
0.));
#229517=CARTESIAN_POINT('Ctrl Pts',(-12.9820222318716,-19.014413367335,
12.));
#229518=CARTESIAN_POINT('Ctrl Pts',(-12.9764729959206,-19.0012154099792,
0.));
#229519=CARTESIAN_POINT('Ctrl Pts',(-12.9764729959206,-19.0012154099792,
12.));
#229520=CARTESIAN_POINT('Ctrl Pts',(-12.9709450512747,-18.9881820807585,
0.));
#229521=CARTESIAN_POINT('Ctrl Pts',(-12.9709450512747,-18.9881820807585,
12.));
#229522=CARTESIAN_POINT('Ctrl Pts',(-12.9654399021868,-18.9753148284473,
0.));
#229523=CARTESIAN_POINT('Ctrl Pts',(-12.9654399021868,-18.9753148284473,
12.));
#229524=CARTESIAN_POINT('Ctrl Pts',(-12.9599590886318,-18.9626151329226,
0.));
#229525=CARTESIAN_POINT('Ctrl Pts',(-12.9599590886318,-18.9626151329226,
12.));
#229526=CARTESIAN_POINT('Ctrl Pts',(-12.9545041877377,-18.9500845064714,
0.));
#229527=CARTESIAN_POINT('Ctrl Pts',(-12.9545041877377,-18.9500845064714,
12.));
#229528=CARTESIAN_POINT('Ctrl Pts',(-12.9490768151821,-18.9377244950435,
0.));
#229529=CARTESIAN_POINT('Ctrl Pts',(-12.9490768151821,-18.9377244950435,
12.));
#229530=CARTESIAN_POINT('Ctrl Pts',(-12.9436786266106,-18.9255366795196,
0.));
#229531=CARTESIAN_POINT('Ctrl Pts',(-12.9436786266106,-18.9255366795196,
12.));
#229532=CARTESIAN_POINT('Ctrl Pts',(-12.9383113190375,-18.9135226769466,
0.));
#229533=CARTESIAN_POINT('Ctrl Pts',(-12.9383113190375,-18.9135226769466,
12.));
#229534=CARTESIAN_POINT('Ctrl Pts',(-12.9329766328184,-18.9016841423402,
0.));
#229535=CARTESIAN_POINT('Ctrl Pts',(-12.9329766328184,-18.9016841423402,
12.));
#229536=CARTESIAN_POINT('Ctrl Pts',(-12.9276763536373,-18.8900227704888,
0.));
#229537=CARTESIAN_POINT('Ctrl Pts',(-12.9276763536373,-18.8900227704888,
12.));
#229538=CARTESIAN_POINT('Ctrl Pts',(-12.9224123144982,-18.8785402977528,
0.));
#229539=CARTESIAN_POINT('Ctrl Pts',(-12.9224123144982,-18.8785402977528,
12.));
#229540=CARTESIAN_POINT('Ctrl Pts',(-12.9171863977047,-18.8672385038328,
0.));
#229541=CARTESIAN_POINT('Ctrl Pts',(-12.9171863977047,-18.8672385038328,
12.));
#229542=CARTESIAN_POINT('Ctrl Pts',(-12.9120005369066,-18.8561192136201,
0.));
#229543=CARTESIAN_POINT('Ctrl Pts',(-12.9120005369066,-18.8561192136201,
12.));
#229544=CARTESIAN_POINT('Ctrl Pts',(-12.9068567191856,-18.8451842990986,
0.));
#229545=CARTESIAN_POINT('Ctrl Pts',(-12.9068567191856,-18.8451842990986,
12.));
#229546=CARTESIAN_POINT('Ctrl Pts',(-12.9017569871738,-18.834435681259,
0.));
#229547=CARTESIAN_POINT('Ctrl Pts',(-12.9017569871738,-18.834435681259,
12.));
#229548=CARTESIAN_POINT('Ctrl Pts',(-12.8967034410752,-18.8238753319124,
0.));
#229549=CARTESIAN_POINT('Ctrl Pts',(-12.8967034410752,-18.8238753319124,
12.));
#229550=CARTESIAN_POINT('Ctrl Pts',(-12.8916982409931,-18.8135052757815,
0.));
#229551=CARTESIAN_POINT('Ctrl Pts',(-12.8916982409931,-18.8135052757815,
12.));
#229552=CARTESIAN_POINT('Ctrl Pts',(-12.8867436109543,-18.8033275941939,
0.));
#229553=CARTESIAN_POINT('Ctrl Pts',(-12.8867436109543,-18.8033275941939,
12.));
#229554=CARTESIAN_POINT('Ctrl Pts',(-12.8818418427474,-18.7933444285867,
0.));
#229555=CARTESIAN_POINT('Ctrl Pts',(-12.8818418427474,-18.7933444285867,
12.));
#229556=CARTESIAN_POINT('Ctrl Pts',(-12.8769952998097,-18.7835579840481,
0.));
#229557=CARTESIAN_POINT('Ctrl Pts',(-12.8769952998097,-18.7835579840481,
12.));
#229558=CARTESIAN_POINT('Ctrl Pts',(-12.8722064211814,-18.7739705329028,
0.));
#229559=CARTESIAN_POINT('Ctrl Pts',(-12.8722064211814,-18.7739705329028,
12.));
#229560=CARTESIAN_POINT('Ctrl Pts',(-12.8674777239656,-18.7645844169568,
0.));
#229561=CARTESIAN_POINT('Ctrl Pts',(-12.8674777239656,-18.7645844169568,
12.));
#229562=CARTESIAN_POINT('Ctrl Pts',(-12.8628118054172,-18.7554020493888,
0.));
#229563=CARTESIAN_POINT('Ctrl Pts',(-12.8628118054172,-18.7554020493888,
12.));
#229564=CARTESIAN_POINT('Ctrl Pts',(-12.8582113455645,-18.7464259171248,
0.));
#229565=CARTESIAN_POINT('Ctrl Pts',(-12.8582113455645,-18.7464259171248,
12.));
#229566=CARTESIAN_POINT('Ctrl Pts',(-12.8536791086315,-18.7376585820851,
0.));
#229567=CARTESIAN_POINT('Ctrl Pts',(-12.8536791086315,-18.7376585820851,
12.));
#229568=CARTESIAN_POINT('Ctrl Pts',(-12.849217951159,-18.7291026886552,
0.));
#229569=CARTESIAN_POINT('Ctrl Pts',(-12.849217951159,-18.7291026886552,
12.));
#229570=CARTESIAN_POINT('Ctrl Pts',(-12.8448308329494,-18.7207609737701,
0.));
#229571=CARTESIAN_POINT('Ctrl Pts',(-12.8448308329494,-18.7207609737701,
12.));
#229572=CARTESIAN_POINT('Ctrl Pts',(-12.8405208263432,-18.7126362754446,
0.));
#229573=CARTESIAN_POINT('Ctrl Pts',(-12.8405208263432,-18.7126362754446,
12.));
#229574=CARTESIAN_POINT('Ctrl Pts',(-12.8362911280362,-18.7047315436296,
0.));
#229575=CARTESIAN_POINT('Ctrl Pts',(-12.8362911280362,-18.7047315436296,
12.));
#229576=CARTESIAN_POINT('Ctrl Pts',(-12.832145059979,-18.6970498410173,
0.));
#229577=CARTESIAN_POINT('Ctrl Pts',(-12.832145059979,-18.6970498410173,
12.));
#229578=CARTESIAN_POINT('Ctrl Pts',(-12.8280860635231,-18.6895943376172,
0.));
#229579=CARTESIAN_POINT('Ctrl Pts',(-12.8280860635231,-18.6895943376172,
12.));
#229580=CARTESIAN_POINT('Ctrl Pts',(-12.8241176980016,-18.6823683094138,
0.));
#229581=CARTESIAN_POINT('Ctrl Pts',(-12.8241176980016,-18.6823683094138,
12.));
#229582=CARTESIAN_POINT('Ctrl Pts',(-12.8202436318473,-18.6753751301091,
0.));
#229583=CARTESIAN_POINT('Ctrl Pts',(-12.8202436318473,-18.6753751301091,
12.));
#229584=CARTESIAN_POINT('Ctrl Pts',(-12.8164676687361,-18.6686182952798,
0.));
#229585=CARTESIAN_POINT('Ctrl Pts',(-12.8164676687361,-18.6686182952798,
12.));
#229586=CARTESIAN_POINT('Ctrl Pts',(-12.8127937909632,-18.6621014624746,
0.));
#229587=CARTESIAN_POINT('Ctrl Pts',(-12.8127937909632,-18.6621014624746,
12.));
#229588=CARTESIAN_POINT('Ctrl Pts',(-12.8092261933858,-18.6558284825772,
0.));
#229589=CARTESIAN_POINT('Ctrl Pts',(-12.8092261933858,-18.6558284825772,
12.));
#229590=CARTESIAN_POINT('Ctrl Pts',(-12.805769331162,-18.6498034438986,
0.));
#229591=CARTESIAN_POINT('Ctrl Pts',(-12.805769331162,-18.6498034438986,
12.));
#229592=CARTESIAN_POINT('Ctrl Pts',(-12.8024278770153,-18.6440306327457,
0.));
#229593=CARTESIAN_POINT('Ctrl Pts',(-12.8024278770153,-18.6440306327457,
12.));
#229594=CARTESIAN_POINT('Ctrl Pts',(-12.7992066625264,-18.63851447924,0.));
#229595=CARTESIAN_POINT('Ctrl Pts',(-12.7992066625264,-18.63851447924,12.));
#229596=CARTESIAN_POINT('Ctrl Pts',(-12.7961106222251,-18.6332595057005,
0.));
#229597=CARTESIAN_POINT('Ctrl Pts',(-12.7961106222251,-18.6332595057005,
12.));
#229598=CARTESIAN_POINT('Ctrl Pts',(-12.7931447451556,-18.6282702819371,
0.));
#229599=CARTESIAN_POINT('Ctrl Pts',(-12.7931447451556,-18.6282702819371,
12.));
#229600=CARTESIAN_POINT('Ctrl Pts',(-12.7903142925235,-18.6235516265575,
0.));
#229601=CARTESIAN_POINT('Ctrl Pts',(-12.7903142925235,-18.6235516265575,
12.));
#229602=CARTESIAN_POINT('Ctrl Pts',(-12.7876249657834,-18.6191087624752,
0.));
#229603=CARTESIAN_POINT('Ctrl Pts',(-12.7876249657834,-18.6191087624752,
12.));
#229604=CARTESIAN_POINT('Ctrl Pts',(-12.78508316579,-18.6149475565189,0.));
#229605=CARTESIAN_POINT('Ctrl Pts',(-12.78508316579,-18.6149475565189,12.));
#229606=CARTESIAN_POINT('Ctrl Pts',(-12.7826959526924,-18.611074482622,
0.));
#229607=CARTESIAN_POINT('Ctrl Pts',(-12.7826959526924,-18.611074482622,
12.));
#229608=CARTESIAN_POINT('Ctrl Pts',(-12.7804705387658,-18.6074961535723,
0.));
#229609=CARTESIAN_POINT('Ctrl Pts',(-12.7804705387658,-18.6074961535723,
12.));
#229610=CARTESIAN_POINT('Ctrl Pts',(-12.7784139605067,-18.6042190183703,
0.));
#229611=CARTESIAN_POINT('Ctrl Pts',(-12.7784139605067,-18.6042190183703,
12.));
#229612=CARTESIAN_POINT('Ctrl Pts',(-12.7765325225083,-18.6012488486708,
0.));
#229613=CARTESIAN_POINT('Ctrl Pts',(-12.7765325225083,-18.6012488486708,
12.));
#229614=CARTESIAN_POINT('Ctrl Pts',(-12.7748328937639,-18.5985917525949,
0.));
#229615=CARTESIAN_POINT('Ctrl Pts',(-12.7748328937639,-18.5985917525949,
12.));
#229616=CARTESIAN_POINT('Ctrl Pts',(-12.7733231262107,-18.5962551167772,
0.));
#229617=CARTESIAN_POINT('Ctrl Pts',(-12.7733231262107,-18.5962551167772,
12.));
#229618=CARTESIAN_POINT('Ctrl Pts',(-12.7720142287169,-18.5942490615409,
0.));
#229619=CARTESIAN_POINT('Ctrl Pts',(-12.7720142287169,-18.5942490615409,
12.));
#229620=CARTESIAN_POINT('Ctrl Pts',(-12.7709195951154,-18.5925859134582,
0.));
#229621=CARTESIAN_POINT('Ctrl Pts',(-12.7709195951154,-18.5925859134582,
12.));
#229622=CARTESIAN_POINT('Ctrl Pts',(-12.7700520897174,-18.5912775137806,
0.));
#229623=CARTESIAN_POINT('Ctrl Pts',(-12.7700520897174,-18.5912775137806,
12.));
#229624=CARTESIAN_POINT('Ctrl Pts',(-12.7694215127923,-18.590332877722,
0.));
#229625=CARTESIAN_POINT('Ctrl Pts',(-12.7694215127923,-18.590332877722,
12.));
#229626=CARTESIAN_POINT('Ctrl Pts',(-12.7691103481996,-18.589871621842,
0.));
#229627=CARTESIAN_POINT('Ctrl Pts',(-12.7691103481996,-18.589871621842,
12.));
#229628=CARTESIAN_POINT('Ctrl Pts',(-12.7689864266924,-18.5896919669158,
0.));
#229629=CARTESIAN_POINT('Ctrl Pts',(-12.7689864266924,-18.5896919669158,
12.));
#229630=CARTESIAN_POINT('Ctrl Pts',(-12.7689524524484,-18.5896460962961,
0.));
#229631=CARTESIAN_POINT('Ctrl Pts',(-12.7689524524484,-18.5896460962961,
12.));
#229632=CARTESIAN_POINT('Ctrl Pts',(-12.7689476255363,-18.5896416359912,
0.));
#229633=CARTESIAN_POINT('Ctrl Pts',(-12.7689476255363,-18.5896416359912,
12.));
#229634=CARTESIAN_POINT('',(-13.5685075571671,-22.1787195904339,0.));
#229635=CARTESIAN_POINT('Ctrl Pts',(-13.5685075571671,-22.1787195904339,
0.));
#229636=CARTESIAN_POINT('Ctrl Pts',(-13.5683460612913,-22.1730081264583,
0.));
#229637=CARTESIAN_POINT('Ctrl Pts',(-13.5680170531724,-22.1615922804939,
0.));
#229638=CARTESIAN_POINT('Ctrl Pts',(-13.5675054918922,-22.1444897575076,
0.));
#229639=CARTESIAN_POINT('Ctrl Pts',(-13.5667873105179,-22.1217288871823,
0.));
#229640=CARTESIAN_POINT('Ctrl Pts',(-13.5658294169107,-22.0933486464442,
0.));
#229641=CARTESIAN_POINT('Ctrl Pts',(-13.5648113688895,-22.0650393089492,
0.));
#229642=CARTESIAN_POINT('Ctrl Pts',(-13.5637332022393,-22.0368009736227,
0.));
#229643=CARTESIAN_POINT('Ctrl Pts',(-13.5625949868313,-22.0086337943431,
0.));
#229644=CARTESIAN_POINT('Ctrl Pts',(-13.5613968357589,-21.9805379899192,
0.));
#229645=CARTESIAN_POINT('Ctrl Pts',(-13.5601389185315,-21.9525138592862,
0.));
#229646=CARTESIAN_POINT('Ctrl Pts',(-13.5588214586672,-21.9245617765827,
0.));
#229647=CARTESIAN_POINT('Ctrl Pts',(-13.5574447178485,-21.8966821688876,
0.));
#229648=CARTESIAN_POINT('Ctrl Pts',(-13.5560089839426,-21.8688754989401,
0.));
#229649=CARTESIAN_POINT('Ctrl Pts',(-13.5545145573049,-21.841142245609,
0.));
#229650=CARTESIAN_POINT('Ctrl Pts',(-13.5529617381569,-21.8134828857963,
0.));
#229651=CARTESIAN_POINT('Ctrl Pts',(-13.5513508127232,-21.7858978745848,
0.));
#229652=CARTESIAN_POINT('Ctrl Pts',(-13.5496820422187,-21.7583876294532,
0.));
#229653=CARTESIAN_POINT('Ctrl Pts',(-13.5479556704457,-21.730952541226,
0.));
#229654=CARTESIAN_POINT('Ctrl Pts',(-13.546171929503,-21.7035929822939,
0.));
#229655=CARTESIAN_POINT('Ctrl Pts',(-13.5443310461516,-21.676309315769,
0.));
#229656=CARTESIAN_POINT('Ctrl Pts',(-13.5424332480698,-21.6491019044647,
0.));
#229657=CARTESIAN_POINT('Ctrl Pts',(-13.5404787697798,-21.6219711193951,
0.));
#229658=CARTESIAN_POINT('Ctrl Pts',(-13.5384678597206,-21.5949173499022,
0.));
#229659=CARTESIAN_POINT('Ctrl Pts',(-13.5364007790292,-21.5679410019011,
0.));
#229660=CARTESIAN_POINT('Ctrl Pts',(-13.5342777983225,-21.5410424932511,
0.));
#229661=CARTESIAN_POINT('Ctrl Pts',(-13.5320991952145,-21.5142222501671,
0.));
#229662=CARTESIAN_POINT('Ctrl Pts',(-13.5298652514357,-21.487480703047,
0.));
#229663=CARTESIAN_POINT('Ctrl Pts',(-13.5275762503553,-21.4608182828695,
0.));
#229664=CARTESIAN_POINT('Ctrl Pts',(-13.5252324737795,-21.4342354165253,
0.));
#229665=CARTESIAN_POINT('Ctrl Pts',(-13.5228342013508,-21.4077325259318,
0.));
#229666=CARTESIAN_POINT('Ctrl Pts',(-13.5203817122497,-21.3813100304967,
0.));
#229667=CARTESIAN_POINT('Ctrl Pts',(-13.5178752862461,-21.3549683486219,
0.));
#229668=CARTESIAN_POINT('Ctrl Pts',(-13.5153152050554,-21.328707899634,
0.));
#229669=CARTESIAN_POINT('Ctrl Pts',(-13.5127017534972,-21.3025291054236,
0.));
#229670=CARTESIAN_POINT('Ctrl Pts',(-13.5100352209207,-21.2764323924442,
0.));
#229671=CARTESIAN_POINT('Ctrl Pts',(-13.5073159019454,-21.2504181927429,
0.));
#229672=CARTESIAN_POINT('Ctrl Pts',(-13.5045440957404,-21.224486942933,
0.));
#229673=CARTESIAN_POINT('Ctrl Pts',(-13.5017201056088,-21.1986390835825,
0.));
#229674=CARTESIAN_POINT('Ctrl Pts',(-13.4988442384491,-21.1728750584173,
0.));
#229675=CARTESIAN_POINT('Ctrl Pts',(-13.4959168042934,-21.1471953136209,
0.));
#229676=CARTESIAN_POINT('Ctrl Pts',(-13.4929381157778,-21.1216002970209,
0.));
#229677=CARTESIAN_POINT('Ctrl Pts',(-13.4899084877718,-21.0960904575048,
0.));
#229678=CARTESIAN_POINT('Ctrl Pts',(-13.4868282377192,-21.0706662455202,
0.));
#229679=CARTESIAN_POINT('Ctrl Pts',(-13.4836976858912,-21.0453281134247,
0.));
#229680=CARTESIAN_POINT('Ctrl Pts',(-13.4805171556822,-21.0200765158885,
0.));
#229681=CARTESIAN_POINT('Ctrl Pts',(-13.4772869738879,-20.9949119102592,
0.));
#229682=CARTESIAN_POINT('Ctrl Pts',(-13.4740074710087,-20.9698347569476,
0.));
#229683=CARTESIAN_POINT('Ctrl Pts',(-13.4706789815167,-20.9448455197557,
0.));
#229684=CARTESIAN_POINT('Ctrl Pts',(-13.4673018437718,-20.9199446657584,
0.));
#229685=CARTESIAN_POINT('Ctrl Pts',(-13.4638763999726,-20.8951326652158,
0.));
#229686=CARTESIAN_POINT('Ctrl Pts',(-13.4604029960983,-20.8704099914641,
0.));
#229687=CARTESIAN_POINT('Ctrl Pts',(-13.4568819818631,-20.8457771208082,
0.));
#229688=CARTESIAN_POINT('Ctrl Pts',(-13.4533137106667,-20.821234532398,
0.));
#229689=CARTESIAN_POINT('Ctrl Pts',(-13.4496985395637,-20.7967827081227,
0.));
#229690=CARTESIAN_POINT('Ctrl Pts',(-13.4460368293688,-20.7724221327608,
0.));
#229691=CARTESIAN_POINT('Ctrl Pts',(-13.4423289447561,-20.7481532941013,
0.));
#229692=CARTESIAN_POINT('Ctrl Pts',(-13.4385752543663,-20.7239766830675,
0.));
#229693=CARTESIAN_POINT('Ctrl Pts',(-13.4347761309154,-20.6998927938288,
0.));
#229694=CARTESIAN_POINT('Ctrl Pts',(-13.4309319513119,-20.6759021239103,
0.));
#229695=CARTESIAN_POINT('Ctrl Pts',(-13.4270430967652,-20.6520051742869,
0.));
#229696=CARTESIAN_POINT('Ctrl Pts',(-13.4231099528179,-20.6282024494237,
0.));
#229697=CARTESIAN_POINT('Ctrl Pts',(-13.4191329093933,-20.6044944573153,
0.));
#229698=CARTESIAN_POINT('Ctrl Pts',(-13.4151123608411,-20.5808817095155,
0.));
#229699=CARTESIAN_POINT('Ctrl Pts',(-13.4110487059912,-20.5573647211639,
0.));
#229700=CARTESIAN_POINT('Ctrl Pts',(-13.4069423482076,-20.5339440109956,
0.));
#229701=CARTESIAN_POINT('Ctrl Pts',(-13.4027936954529,-20.5106201013753,
0.));
#229702=CARTESIAN_POINT('Ctrl Pts',(-13.3986031603716,-20.487393518404,
0.));
#229703=CARTESIAN_POINT('Ctrl Pts',(-13.3943711603739,-20.4642647920037,
0.));
#229704=CARTESIAN_POINT('Ctrl Pts',(-13.3900981177255,-20.4412344560007,
0.));
#229705=CARTESIAN_POINT('Ctrl Pts',(-13.3857844596387,-20.4183030482002,
0.));
#229706=CARTESIAN_POINT('Ctrl Pts',(-13.3814306183719,-20.3954711104502,
0.));
#229707=CARTESIAN_POINT('Ctrl Pts',(-13.3770370313188,-20.3727391887184,
0.));
#229708=CARTESIAN_POINT('Ctrl Pts',(-13.3726041410867,-20.3501078331814,
0.));
#229709=CARTESIAN_POINT('Ctrl Pts',(-13.3681323955826,-20.3275775983029,
0.));
#229710=CARTESIAN_POINT('Ctrl Pts',(-13.3636222481016,-20.3051490429048,
0.));
#229711=CARTESIAN_POINT('Ctrl Pts',(-13.3590741574195,-20.2828227302339,
0.));
#229712=CARTESIAN_POINT('Ctrl Pts',(-13.3544885878889,-20.2605992280122,
0.));
#229713=CARTESIAN_POINT('Ctrl Pts',(-13.3498660095386,-20.2384791085359,
0.));
#229714=CARTESIAN_POINT('Ctrl Pts',(-13.3452068981766,-20.216462948786,
0.));
#229715=CARTESIAN_POINT('Ctrl Pts',(-13.3405117354971,-20.1945513305235,
0.));
#229716=CARTESIAN_POINT('Ctrl Pts',(-13.3357810091903,-20.1727448403817,
0.));
#229717=CARTESIAN_POINT('Ctrl Pts',(-13.3310152130564,-20.1510440699474,
0.));
#229718=CARTESIAN_POINT('Ctrl Pts',(-13.3262148471226,-20.1294496158402,
0.));
#229719=CARTESIAN_POINT('Ctrl Pts',(-13.3213804177587,-20.1079620798375,
0.));
#229720=CARTESIAN_POINT('Ctrl Pts',(-13.3165124377963,-20.0865820689882,
0.));
#229721=CARTESIAN_POINT('Ctrl Pts',(-13.3116114266515,-20.0653101957188,
0.));
#229722=CARTESIAN_POINT('Ctrl Pts',(-13.3066779104515,-20.0441470779345,
0.));
#229723=CARTESIAN_POINT('Ctrl Pts',(-13.3017124221637,-20.0230933391038,
0.));
#229724=CARTESIAN_POINT('Ctrl Pts',(-13.2967155017306,-20.0021496083738,
0.));
#229725=CARTESIAN_POINT('Ctrl Pts',(-13.2916876962094,-19.981316520717,
0.));
#229726=CARTESIAN_POINT('Ctrl Pts',(-13.286629559915,-19.9605947170586,
0.));
#229727=CARTESIAN_POINT('Ctrl Pts',(-13.2815416545663,-19.9399848444019,
0.));
#229728=CARTESIAN_POINT('Ctrl Pts',(-13.2764245494357,-19.9194875559422,
0.));
#229729=CARTESIAN_POINT('Ctrl Pts',(-13.271278821502,-19.8991035111745,
0.));
#229730=CARTESIAN_POINT('Ctrl Pts',(-13.2661050556132,-19.8788333760577,
0.));
#229731=CARTESIAN_POINT('Ctrl Pts',(-13.2609038446529,-19.8586778231715,
0.));
#229732=CARTESIAN_POINT('Ctrl Pts',(-13.2556757897086,-19.8386375318634,
0.));
#229733=CARTESIAN_POINT('Ctrl Pts',(-13.2504215002457,-19.8187131883917,
0.));
#229734=CARTESIAN_POINT('Ctrl Pts',(-13.2451415942805,-19.7989054860495,
0.));
#229735=CARTESIAN_POINT('Ctrl Pts',(-13.2398366985675,-19.7792151253289,
0.));
#229736=CARTESIAN_POINT('Ctrl Pts',(-13.2345074487963,-19.7596428141168,
0.));
#229737=CARTESIAN_POINT('Ctrl Pts',(-13.2291544897899,-19.7401892678697,
0.));
#229738=CARTESIAN_POINT('Ctrl Pts',(-13.2237784757066,-19.7208552097868,
0.));
#229739=CARTESIAN_POINT('Ctrl Pts',(-13.2183800702436,-19.7016413709685,
0.));
#229740=CARTESIAN_POINT('Ctrl Pts',(-13.2129599468485,-19.6825484905823,
0.));
#229741=CARTESIAN_POINT('Ctrl Pts',(-13.2075187889529,-19.6635773160936,
0.));
#229742=CARTESIAN_POINT('Ctrl Pts',(-13.2020572902065,-19.6447286034772,
0.));
#229743=CARTESIAN_POINT('Ctrl Pts',(-13.1965761547151,-19.6260031174244,
0.));
#229744=CARTESIAN_POINT('Ctrl Pts',(-13.1910760972814,-19.6074016315414,
0.));
#229745=CARTESIAN_POINT('Ctrl Pts',(-13.1855578436471,-19.5889249285338,
0.));
#229746=CARTESIAN_POINT('Ctrl Pts',(-13.1800221307673,-19.5705738004667,
0.));
#229747=CARTESIAN_POINT('Ctrl Pts',(-13.1744697070911,-19.5523490490244,
0.));
#229748=CARTESIAN_POINT('Ctrl Pts',(-13.1689013328431,-19.5342514857562,
0.));
#229749=CARTESIAN_POINT('Ctrl Pts',(-13.1633177803101,-19.5162819323213,
0.));
#229750=CARTESIAN_POINT('Ctrl Pts',(-13.1577198341245,-19.4984412207081,
0.));
#229751=CARTESIAN_POINT('Ctrl Pts',(-13.1521082915853,-19.4807301935268,
0.));
#229752=CARTESIAN_POINT('Ctrl Pts',(-13.1464839629971,-19.4631497043258,
0.));
#229753=CARTESIAN_POINT('Ctrl Pts',(-13.1408476720061,-19.4457006178876,
0.));
#229754=CARTESIAN_POINT('Ctrl Pts',(-13.1352002559438,-19.4283838105262,
0.));
#229755=CARTESIAN_POINT('Ctrl Pts',(-13.1295425661634,-19.4112001703557,
0.));
#229756=CARTESIAN_POINT('Ctrl Pts',(-13.1238754684177,-19.3941505976263,
0.));
#229757=CARTESIAN_POINT('Ctrl Pts',(-13.118199843271,-19.3772360051091,
0.));
#229758=CARTESIAN_POINT('Ctrl Pts',(-13.1125165865022,-19.3604573184515,
0.));
#229759=CARTESIAN_POINT('Ctrl Pts',(-13.1068266095186,-19.3438154765395,
0.));
#229760=CARTESIAN_POINT('Ctrl Pts',(-13.1011308397591,-19.3273114318269,
0.));
#229761=CARTESIAN_POINT('Ctrl Pts',(-13.0954302211479,-19.310946150736,
0.));
#229762=CARTESIAN_POINT('Ctrl Pts',(-13.0897257145969,-19.2947206141247,
0.));
#229763=CARTESIAN_POINT('Ctrl Pts',(-13.0840182984949,-19.2786358177198,
0.));
#229764=CARTESIAN_POINT('Ctrl Pts',(-13.0783089692118,-19.2626927725596,
0.));
#229765=CARTESIAN_POINT('Ctrl Pts',(-13.0725987415859,-19.2468925053989,
0.));
#229766=CARTESIAN_POINT('Ctrl Pts',(-13.0668886494795,-19.2312360592033,
0.));
#229767=CARTESIAN_POINT('Ctrl Pts',(-13.0611797463915,-19.2157244937142,
0.));
#229768=CARTESIAN_POINT('Ctrl Pts',(-13.0554731060538,-19.2003588859772,
0.));
#229769=CARTESIAN_POINT('Ctrl Pts',(-13.0497698230441,-19.1851403308825,
0.));
#229770=CARTESIAN_POINT('Ctrl Pts',(-13.0440710133772,-19.1700699416622,
0.));
#229771=CARTESIAN_POINT('Ctrl Pts',(-13.0383778152068,-19.155148850523,
0.));
#229772=CARTESIAN_POINT('Ctrl Pts',(-13.0326913895838,-19.1403782093386,
0.));
#229773=CARTESIAN_POINT('Ctrl Pts',(-13.0270129211976,-19.1257591903099,
0.));
#229774=CARTESIAN_POINT('Ctrl Pts',(-13.0213436191328,-19.111292986631,
0.));
#229775=CARTESIAN_POINT('Ctrl Pts',(-13.0156847176097,-19.0969808131228,
0.));
#229776=CARTESIAN_POINT('Ctrl Pts',(-13.0100374768788,-19.0828239070484,
0.));
#229777=CARTESIAN_POINT('Ctrl Pts',(-13.0044031841382,-19.0688235289437,
0.));
#229778=CARTESIAN_POINT('Ctrl Pts',(-12.9987831544502,-19.0549809634354,
0.));
#229779=CARTESIAN_POINT('Ctrl Pts',(-12.9931787316514,-19.0412975200398,
0.));
#229780=CARTESIAN_POINT('Ctrl Pts',(-12.9875912893003,-19.0277745339908,
0.));
#229781=CARTESIAN_POINT('Ctrl Pts',(-12.9820222318716,-19.014413367335,
0.));
#229782=CARTESIAN_POINT('Ctrl Pts',(-12.9764729959206,-19.0012154099792,
0.));
#229783=CARTESIAN_POINT('Ctrl Pts',(-12.9709450512747,-18.9881820807585,
0.));
#229784=CARTESIAN_POINT('Ctrl Pts',(-12.9654399021868,-18.9753148284473,
0.));
#229785=CARTESIAN_POINT('Ctrl Pts',(-12.9599590886318,-18.9626151329226,
0.));
#229786=CARTESIAN_POINT('Ctrl Pts',(-12.9545041877377,-18.9500845064714,
0.));
#229787=CARTESIAN_POINT('Ctrl Pts',(-12.9490768151821,-18.9377244950435,
0.));
#229788=CARTESIAN_POINT('Ctrl Pts',(-12.9436786266106,-18.9255366795196,
0.));
#229789=CARTESIAN_POINT('Ctrl Pts',(-12.9383113190375,-18.9135226769466,
0.));
#229790=CARTESIAN_POINT('Ctrl Pts',(-12.9329766328184,-18.9016841423402,
0.));
#229791=CARTESIAN_POINT('Ctrl Pts',(-12.9276763536373,-18.8900227704888,
0.));
#229792=CARTESIAN_POINT('Ctrl Pts',(-12.9224123144982,-18.8785402977528,
0.));
#229793=CARTESIAN_POINT('Ctrl Pts',(-12.9171863977047,-18.8672385038328,
0.));
#229794=CARTESIAN_POINT('Ctrl Pts',(-12.9120005369066,-18.8561192136201,
0.));
#229795=CARTESIAN_POINT('Ctrl Pts',(-12.9068567191856,-18.8451842990986,
0.));
#229796=CARTESIAN_POINT('Ctrl Pts',(-12.9017569871738,-18.834435681259,
0.));
#229797=CARTESIAN_POINT('Ctrl Pts',(-12.8967034410752,-18.8238753319124,
0.));
#229798=CARTESIAN_POINT('Ctrl Pts',(-12.8916982409931,-18.8135052757815,
0.));
#229799=CARTESIAN_POINT('Ctrl Pts',(-12.8867436109543,-18.8033275941939,
0.));
#229800=CARTESIAN_POINT('Ctrl Pts',(-12.8818418427474,-18.7933444285867,
0.));
#229801=CARTESIAN_POINT('Ctrl Pts',(-12.8769952998097,-18.7835579840481,
0.));
#229802=CARTESIAN_POINT('Ctrl Pts',(-12.8722064211814,-18.7739705329028,
0.));
#229803=CARTESIAN_POINT('Ctrl Pts',(-12.8674777239656,-18.7645844169568,
0.));
#229804=CARTESIAN_POINT('Ctrl Pts',(-12.8628118054172,-18.7554020493888,
0.));
#229805=CARTESIAN_POINT('Ctrl Pts',(-12.8582113455645,-18.7464259171248,
0.));
#229806=CARTESIAN_POINT('Ctrl Pts',(-12.8536791086315,-18.7376585820851,
0.));
#229807=CARTESIAN_POINT('Ctrl Pts',(-12.849217951159,-18.7291026886552,
0.));
#229808=CARTESIAN_POINT('Ctrl Pts',(-12.8448308329494,-18.7207609737701,
0.));
#229809=CARTESIAN_POINT('Ctrl Pts',(-12.8405208263432,-18.7126362754446,
0.));
#229810=CARTESIAN_POINT('Ctrl Pts',(-12.8362911280362,-18.7047315436296,
0.));
#229811=CARTESIAN_POINT('Ctrl Pts',(-12.832145059979,-18.6970498410173,
0.));
#229812=CARTESIAN_POINT('Ctrl Pts',(-12.8280860635231,-18.6895943376172,
0.));
#229813=CARTESIAN_POINT('Ctrl Pts',(-12.8241176980016,-18.6823683094138,
0.));
#229814=CARTESIAN_POINT('Ctrl Pts',(-12.8202436318473,-18.6753751301091,
0.));
#229815=CARTESIAN_POINT('Ctrl Pts',(-12.8164676687361,-18.6686182952798,
0.));
#229816=CARTESIAN_POINT('Ctrl Pts',(-12.8127937909632,-18.6621014624746,
0.));
#229817=CARTESIAN_POINT('Ctrl Pts',(-12.8092261933858,-18.6558284825772,
0.));
#229818=CARTESIAN_POINT('Ctrl Pts',(-12.805769331162,-18.6498034438986,
0.));
#229819=CARTESIAN_POINT('Ctrl Pts',(-12.8024278770153,-18.6440306327457,
0.));
#229820=CARTESIAN_POINT('Ctrl Pts',(-12.7992066625264,-18.63851447924,0.));
#229821=CARTESIAN_POINT('Ctrl Pts',(-12.7961106222251,-18.6332595057005,
0.));
#229822=CARTESIAN_POINT('Ctrl Pts',(-12.7931447451556,-18.6282702819371,
0.));
#229823=CARTESIAN_POINT('Ctrl Pts',(-12.7903142925235,-18.6235516265575,
0.));
#229824=CARTESIAN_POINT('Ctrl Pts',(-12.7876249657834,-18.6191087624752,
0.));
#229825=CARTESIAN_POINT('Ctrl Pts',(-12.78508316579,-18.6149475565189,0.));
#229826=CARTESIAN_POINT('Ctrl Pts',(-12.7826959526924,-18.611074482622,
0.));
#229827=CARTESIAN_POINT('Ctrl Pts',(-12.7804705387658,-18.6074961535723,
0.));
#229828=CARTESIAN_POINT('Ctrl Pts',(-12.7784139605067,-18.6042190183703,
0.));
#229829=CARTESIAN_POINT('Ctrl Pts',(-12.7765325225083,-18.6012488486708,
0.));
#229830=CARTESIAN_POINT('Ctrl Pts',(-12.7748328937639,-18.5985917525949,
0.));
#229831=CARTESIAN_POINT('Ctrl Pts',(-12.7733231262107,-18.5962551167772,
0.));
#229832=CARTESIAN_POINT('Ctrl Pts',(-12.7720142287169,-18.5942490615409,
0.));
#229833=CARTESIAN_POINT('Ctrl Pts',(-12.7709195951154,-18.5925859134582,
0.));
#229834=CARTESIAN_POINT('Ctrl Pts',(-12.7700520897174,-18.5912775137806,
0.));
#229835=CARTESIAN_POINT('Ctrl Pts',(-12.7694215127923,-18.590332877722,
0.));
#229836=CARTESIAN_POINT('Ctrl Pts',(-12.7691103481996,-18.589871621842,
0.));
#229837=CARTESIAN_POINT('Ctrl Pts',(-12.7689864266924,-18.5896919669158,
0.));
#229838=CARTESIAN_POINT('Ctrl Pts',(-12.7689524524484,-18.5896460962961,
0.));
#229839=CARTESIAN_POINT('Ctrl Pts',(-12.7689476255363,-18.5896416359912,
0.));
#229840=CARTESIAN_POINT('',(-13.5685075571671,-22.1787195904339,12.));
#229841=CARTESIAN_POINT('',(-13.5685075571671,-22.1787195904339,0.));
#229842=CARTESIAN_POINT('Ctrl Pts',(-12.7689476255363,-18.5896416359912,
12.));
#229843=CARTESIAN_POINT('Ctrl Pts',(-12.7689524524484,-18.5896460962961,
12.));
#229844=CARTESIAN_POINT('Ctrl Pts',(-12.7689864266924,-18.5896919669158,
12.));
#229845=CARTESIAN_POINT('Ctrl Pts',(-12.7691103481996,-18.589871621842,
12.));
#229846=CARTESIAN_POINT('Ctrl Pts',(-12.7694215127923,-18.590332877722,
12.));
#229847=CARTESIAN_POINT('Ctrl Pts',(-12.7700520897174,-18.5912775137806,
12.));
#229848=CARTESIAN_POINT('Ctrl Pts',(-12.7709195951154,-18.5925859134582,
12.));
#229849=CARTESIAN_POINT('Ctrl Pts',(-12.7720142287169,-18.5942490615409,
12.));
#229850=CARTESIAN_POINT('Ctrl Pts',(-12.7733231262107,-18.5962551167772,
12.));
#229851=CARTESIAN_POINT('Ctrl Pts',(-12.7748328937639,-18.5985917525949,
12.));
#229852=CARTESIAN_POINT('Ctrl Pts',(-12.7765325225083,-18.6012488486708,
12.));
#229853=CARTESIAN_POINT('Ctrl Pts',(-12.7784139605067,-18.6042190183703,
12.));
#229854=CARTESIAN_POINT('Ctrl Pts',(-12.7804705387658,-18.6074961535723,
12.));
#229855=CARTESIAN_POINT('Ctrl Pts',(-12.7826959526924,-18.611074482622,
12.));
#229856=CARTESIAN_POINT('Ctrl Pts',(-12.78508316579,-18.6149475565189,12.));
#229857=CARTESIAN_POINT('Ctrl Pts',(-12.7876249657834,-18.6191087624752,
12.));
#229858=CARTESIAN_POINT('Ctrl Pts',(-12.7903142925235,-18.6235516265575,
12.));
#229859=CARTESIAN_POINT('Ctrl Pts',(-12.7931447451556,-18.6282702819371,
12.));
#229860=CARTESIAN_POINT('Ctrl Pts',(-12.7961106222251,-18.6332595057005,
12.));
#229861=CARTESIAN_POINT('Ctrl Pts',(-12.7992066625264,-18.63851447924,12.));
#229862=CARTESIAN_POINT('Ctrl Pts',(-12.8024278770153,-18.6440306327457,
12.));
#229863=CARTESIAN_POINT('Ctrl Pts',(-12.805769331162,-18.6498034438986,
12.));
#229864=CARTESIAN_POINT('Ctrl Pts',(-12.8092261933858,-18.6558284825772,
12.));
#229865=CARTESIAN_POINT('Ctrl Pts',(-12.8127937909632,-18.6621014624746,
12.));
#229866=CARTESIAN_POINT('Ctrl Pts',(-12.8164676687361,-18.6686182952798,
12.));
#229867=CARTESIAN_POINT('Ctrl Pts',(-12.8202436318473,-18.6753751301091,
12.));
#229868=CARTESIAN_POINT('Ctrl Pts',(-12.8241176980016,-18.6823683094138,
12.));
#229869=CARTESIAN_POINT('Ctrl Pts',(-12.8280860635231,-18.6895943376172,
12.));
#229870=CARTESIAN_POINT('Ctrl Pts',(-12.832145059979,-18.6970498410173,
12.));
#229871=CARTESIAN_POINT('Ctrl Pts',(-12.8362911280362,-18.7047315436296,
12.));
#229872=CARTESIAN_POINT('Ctrl Pts',(-12.8405208263432,-18.7126362754446,
12.));
#229873=CARTESIAN_POINT('Ctrl Pts',(-12.8448308329494,-18.7207609737701,
12.));
#229874=CARTESIAN_POINT('Ctrl Pts',(-12.849217951159,-18.7291026886552,
12.));
#229875=CARTESIAN_POINT('Ctrl Pts',(-12.8536791086315,-18.7376585820851,
12.));
#229876=CARTESIAN_POINT('Ctrl Pts',(-12.8582113455645,-18.7464259171248,
12.));
#229877=CARTESIAN_POINT('Ctrl Pts',(-12.8628118054172,-18.7554020493888,
12.));
#229878=CARTESIAN_POINT('Ctrl Pts',(-12.8674777239656,-18.7645844169568,
12.));
#229879=CARTESIAN_POINT('Ctrl Pts',(-12.8722064211814,-18.7739705329028,
12.));
#229880=CARTESIAN_POINT('Ctrl Pts',(-12.8769952998097,-18.7835579840481,
12.));
#229881=CARTESIAN_POINT('Ctrl Pts',(-12.8818418427474,-18.7933444285867,
12.));
#229882=CARTESIAN_POINT('Ctrl Pts',(-12.8867436109543,-18.8033275941939,
12.));
#229883=CARTESIAN_POINT('Ctrl Pts',(-12.8916982409931,-18.8135052757815,
12.));
#229884=CARTESIAN_POINT('Ctrl Pts',(-12.8967034410752,-18.8238753319124,
12.));
#229885=CARTESIAN_POINT('Ctrl Pts',(-12.9017569871738,-18.834435681259,
12.));
#229886=CARTESIAN_POINT('Ctrl Pts',(-12.9068567191856,-18.8451842990986,
12.));
#229887=CARTESIAN_POINT('Ctrl Pts',(-12.9120005369066,-18.8561192136201,
12.));
#229888=CARTESIAN_POINT('Ctrl Pts',(-12.9171863977047,-18.8672385038328,
12.));
#229889=CARTESIAN_POINT('Ctrl Pts',(-12.9224123144982,-18.8785402977528,
12.));
#229890=CARTESIAN_POINT('Ctrl Pts',(-12.9276763536373,-18.8900227704888,
12.));
#229891=CARTESIAN_POINT('Ctrl Pts',(-12.9329766328184,-18.9016841423402,
12.));
#229892=CARTESIAN_POINT('Ctrl Pts',(-12.9383113190375,-18.9135226769466,
12.));
#229893=CARTESIAN_POINT('Ctrl Pts',(-12.9436786266106,-18.9255366795196,
12.));
#229894=CARTESIAN_POINT('Ctrl Pts',(-12.9490768151821,-18.9377244950435,
12.));
#229895=CARTESIAN_POINT('Ctrl Pts',(-12.9545041877377,-18.9500845064714,
12.));
#229896=CARTESIAN_POINT('Ctrl Pts',(-12.9599590886318,-18.9626151329226,
12.));
#229897=CARTESIAN_POINT('Ctrl Pts',(-12.9654399021868,-18.9753148284473,
12.));
#229898=CARTESIAN_POINT('Ctrl Pts',(-12.9709450512747,-18.9881820807585,
12.));
#229899=CARTESIAN_POINT('Ctrl Pts',(-12.9764729959206,-19.0012154099792,
12.));
#229900=CARTESIAN_POINT('Ctrl Pts',(-12.9820222318716,-19.014413367335,
12.));
#229901=CARTESIAN_POINT('Ctrl Pts',(-12.9875912893003,-19.0277745339908,
12.));
#229902=CARTESIAN_POINT('Ctrl Pts',(-12.9931787316514,-19.0412975200398,
12.));
#229903=CARTESIAN_POINT('Ctrl Pts',(-12.9987831544502,-19.0549809634354,
12.));
#229904=CARTESIAN_POINT('Ctrl Pts',(-13.0044031841382,-19.0688235289437,
12.));
#229905=CARTESIAN_POINT('Ctrl Pts',(-13.0100374768788,-19.0828239070484,
12.));
#229906=CARTESIAN_POINT('Ctrl Pts',(-13.0156847176097,-19.0969808131228,
12.));
#229907=CARTESIAN_POINT('Ctrl Pts',(-13.0213436191328,-19.111292986631,
12.));
#229908=CARTESIAN_POINT('Ctrl Pts',(-13.0270129211976,-19.1257591903099,
12.));
#229909=CARTESIAN_POINT('Ctrl Pts',(-13.0326913895838,-19.1403782093386,
12.));
#229910=CARTESIAN_POINT('Ctrl Pts',(-13.0383778152068,-19.155148850523,
12.));
#229911=CARTESIAN_POINT('Ctrl Pts',(-13.0440710133772,-19.1700699416622,
12.));
#229912=CARTESIAN_POINT('Ctrl Pts',(-13.0497698230441,-19.1851403308825,
12.));
#229913=CARTESIAN_POINT('Ctrl Pts',(-13.0554731060538,-19.2003588859772,
12.));
#229914=CARTESIAN_POINT('Ctrl Pts',(-13.0611797463915,-19.2157244937142,
12.));
#229915=CARTESIAN_POINT('Ctrl Pts',(-13.0668886494795,-19.2312360592033,
12.));
#229916=CARTESIAN_POINT('Ctrl Pts',(-13.0725987415859,-19.2468925053989,
12.));
#229917=CARTESIAN_POINT('Ctrl Pts',(-13.0783089692118,-19.2626927725596,
12.));
#229918=CARTESIAN_POINT('Ctrl Pts',(-13.0840182984949,-19.2786358177198,
12.));
#229919=CARTESIAN_POINT('Ctrl Pts',(-13.0897257145969,-19.2947206141247,
12.));
#229920=CARTESIAN_POINT('Ctrl Pts',(-13.0954302211479,-19.310946150736,
12.));
#229921=CARTESIAN_POINT('Ctrl Pts',(-13.1011308397591,-19.3273114318269,
12.));
#229922=CARTESIAN_POINT('Ctrl Pts',(-13.1068266095186,-19.3438154765395,
12.));
#229923=CARTESIAN_POINT('Ctrl Pts',(-13.1125165865022,-19.3604573184515,
12.));
#229924=CARTESIAN_POINT('Ctrl Pts',(-13.118199843271,-19.3772360051091,
12.));
#229925=CARTESIAN_POINT('Ctrl Pts',(-13.1238754684177,-19.3941505976263,
12.));
#229926=CARTESIAN_POINT('Ctrl Pts',(-13.1295425661634,-19.4112001703557,
12.));
#229927=CARTESIAN_POINT('Ctrl Pts',(-13.1352002559438,-19.4283838105262,
12.));
#229928=CARTESIAN_POINT('Ctrl Pts',(-13.1408476720061,-19.4457006178876,
12.));
#229929=CARTESIAN_POINT('Ctrl Pts',(-13.1464839629971,-19.4631497043258,
12.));
#229930=CARTESIAN_POINT('Ctrl Pts',(-13.1521082915853,-19.4807301935268,
12.));
#229931=CARTESIAN_POINT('Ctrl Pts',(-13.1577198341245,-19.4984412207081,
12.));
#229932=CARTESIAN_POINT('Ctrl Pts',(-13.1633177803101,-19.5162819323213,
12.));
#229933=CARTESIAN_POINT('Ctrl Pts',(-13.1689013328431,-19.5342514857562,
12.));
#229934=CARTESIAN_POINT('Ctrl Pts',(-13.1744697070911,-19.5523490490244,
12.));
#229935=CARTESIAN_POINT('Ctrl Pts',(-13.1800221307673,-19.5705738004667,
12.));
#229936=CARTESIAN_POINT('Ctrl Pts',(-13.1855578436471,-19.5889249285338,
12.));
#229937=CARTESIAN_POINT('Ctrl Pts',(-13.1910760972814,-19.6074016315414,
12.));
#229938=CARTESIAN_POINT('Ctrl Pts',(-13.1965761547151,-19.6260031174244,
12.));
#229939=CARTESIAN_POINT('Ctrl Pts',(-13.2020572902065,-19.6447286034772,
12.));
#229940=CARTESIAN_POINT('Ctrl Pts',(-13.2075187889529,-19.6635773160936,
12.));
#229941=CARTESIAN_POINT('Ctrl Pts',(-13.2129599468485,-19.6825484905823,
12.));
#229942=CARTESIAN_POINT('Ctrl Pts',(-13.2183800702436,-19.7016413709685,
12.));
#229943=CARTESIAN_POINT('Ctrl Pts',(-13.2237784757066,-19.7208552097868,
12.));
#229944=CARTESIAN_POINT('Ctrl Pts',(-13.2291544897899,-19.7401892678697,
12.));
#229945=CARTESIAN_POINT('Ctrl Pts',(-13.2345074487963,-19.7596428141168,
12.));
#229946=CARTESIAN_POINT('Ctrl Pts',(-13.2398366985675,-19.7792151253289,
12.));
#229947=CARTESIAN_POINT('Ctrl Pts',(-13.2451415942805,-19.7989054860495,
12.));
#229948=CARTESIAN_POINT('Ctrl Pts',(-13.2504215002457,-19.8187131883917,
12.));
#229949=CARTESIAN_POINT('Ctrl Pts',(-13.2556757897086,-19.8386375318634,
12.));
#229950=CARTESIAN_POINT('Ctrl Pts',(-13.2609038446529,-19.8586778231715,
12.));
#229951=CARTESIAN_POINT('Ctrl Pts',(-13.2661050556132,-19.8788333760577,
12.));
#229952=CARTESIAN_POINT('Ctrl Pts',(-13.271278821502,-19.8991035111745,
12.));
#229953=CARTESIAN_POINT('Ctrl Pts',(-13.2764245494357,-19.9194875559422,
12.));
#229954=CARTESIAN_POINT('Ctrl Pts',(-13.2815416545663,-19.9399848444019,
12.));
#229955=CARTESIAN_POINT('Ctrl Pts',(-13.286629559915,-19.9605947170586,
12.));
#229956=CARTESIAN_POINT('Ctrl Pts',(-13.2916876962094,-19.981316520717,
12.));
#229957=CARTESIAN_POINT('Ctrl Pts',(-13.2967155017306,-20.0021496083738,
12.));
#229958=CARTESIAN_POINT('Ctrl Pts',(-13.3017124221637,-20.0230933391038,
12.));
#229959=CARTESIAN_POINT('Ctrl Pts',(-13.3066779104515,-20.0441470779345,
12.));
#229960=CARTESIAN_POINT('Ctrl Pts',(-13.3116114266515,-20.0653101957188,
12.));
#229961=CARTESIAN_POINT('Ctrl Pts',(-13.3165124377963,-20.0865820689882,
12.));
#229962=CARTESIAN_POINT('Ctrl Pts',(-13.3213804177587,-20.1079620798375,
12.));
#229963=CARTESIAN_POINT('Ctrl Pts',(-13.3262148471226,-20.1294496158402,
12.));
#229964=CARTESIAN_POINT('Ctrl Pts',(-13.3310152130564,-20.1510440699474,
12.));
#229965=CARTESIAN_POINT('Ctrl Pts',(-13.3357810091903,-20.1727448403817,
12.));
#229966=CARTESIAN_POINT('Ctrl Pts',(-13.3405117354971,-20.1945513305235,
12.));
#229967=CARTESIAN_POINT('Ctrl Pts',(-13.3452068981766,-20.216462948786,
12.));
#229968=CARTESIAN_POINT('Ctrl Pts',(-13.3498660095386,-20.2384791085359,
12.));
#229969=CARTESIAN_POINT('Ctrl Pts',(-13.3544885878889,-20.2605992280122,
12.));
#229970=CARTESIAN_POINT('Ctrl Pts',(-13.3590741574195,-20.2828227302339,
12.));
#229971=CARTESIAN_POINT('Ctrl Pts',(-13.3636222481016,-20.3051490429048,
12.));
#229972=CARTESIAN_POINT('Ctrl Pts',(-13.3681323955826,-20.3275775983029,
12.));
#229973=CARTESIAN_POINT('Ctrl Pts',(-13.3726041410867,-20.3501078331814,
12.));
#229974=CARTESIAN_POINT('Ctrl Pts',(-13.3770370313188,-20.3727391887184,
12.));
#229975=CARTESIAN_POINT('Ctrl Pts',(-13.3814306183719,-20.3954711104502,
12.));
#229976=CARTESIAN_POINT('Ctrl Pts',(-13.3857844596387,-20.4183030482002,
12.));
#229977=CARTESIAN_POINT('Ctrl Pts',(-13.3900981177255,-20.4412344560007,
12.));
#229978=CARTESIAN_POINT('Ctrl Pts',(-13.3943711603739,-20.4642647920037,
12.));
#229979=CARTESIAN_POINT('Ctrl Pts',(-13.3986031603716,-20.487393518404,
12.));
#229980=CARTESIAN_POINT('Ctrl Pts',(-13.4027936954529,-20.5106201013753,
12.));
#229981=CARTESIAN_POINT('Ctrl Pts',(-13.4069423482076,-20.5339440109956,
12.));
#229982=CARTESIAN_POINT('Ctrl Pts',(-13.4110487059912,-20.5573647211639,
12.));
#229983=CARTESIAN_POINT('Ctrl Pts',(-13.4151123608411,-20.5808817095155,
12.));
#229984=CARTESIAN_POINT('Ctrl Pts',(-13.4191329093933,-20.6044944573153,
12.));
#229985=CARTESIAN_POINT('Ctrl Pts',(-13.4231099528179,-20.6282024494237,
12.));
#229986=CARTESIAN_POINT('Ctrl Pts',(-13.4270430967652,-20.6520051742869,
12.));
#229987=CARTESIAN_POINT('Ctrl Pts',(-13.4309319513119,-20.6759021239103,
12.));
#229988=CARTESIAN_POINT('Ctrl Pts',(-13.4347761309154,-20.6998927938288,
12.));
#229989=CARTESIAN_POINT('Ctrl Pts',(-13.4385752543663,-20.7239766830675,
12.));
#229990=CARTESIAN_POINT('Ctrl Pts',(-13.4423289447561,-20.7481532941013,
12.));
#229991=CARTESIAN_POINT('Ctrl Pts',(-13.4460368293688,-20.7724221327608,
12.));
#229992=CARTESIAN_POINT('Ctrl Pts',(-13.4496985395637,-20.7967827081227,
12.));
#229993=CARTESIAN_POINT('Ctrl Pts',(-13.4533137106667,-20.821234532398,
12.));
#229994=CARTESIAN_POINT('Ctrl Pts',(-13.4568819818631,-20.8457771208082,
12.));
#229995=CARTESIAN_POINT('Ctrl Pts',(-13.4604029960983,-20.8704099914641,
12.));
#229996=CARTESIAN_POINT('Ctrl Pts',(-13.4638763999726,-20.8951326652158,
12.));
#229997=CARTESIAN_POINT('Ctrl Pts',(-13.4673018437718,-20.9199446657584,
12.));
#229998=CARTESIAN_POINT('Ctrl Pts',(-13.4706789815167,-20.9448455197557,
12.));
#229999=CARTESIAN_POINT('Ctrl Pts',(-13.4740074710087,-20.9698347569476,
12.));
#230000=CARTESIAN_POINT('Ctrl Pts',(-13.4772869738879,-20.9949119102592,
12.));
#230001=CARTESIAN_POINT('Ctrl Pts',(-13.4805171556822,-21.0200765158885,
12.));
#230002=CARTESIAN_POINT('Ctrl Pts',(-13.4836976858912,-21.0453281134247,
12.));
#230003=CARTESIAN_POINT('Ctrl Pts',(-13.4868282377192,-21.0706662455202,
12.));
#230004=CARTESIAN_POINT('Ctrl Pts',(-13.4899084877718,-21.0960904575048,
12.));
#230005=CARTESIAN_POINT('Ctrl Pts',(-13.4929381157778,-21.1216002970209,
12.));
#230006=CARTESIAN_POINT('Ctrl Pts',(-13.4959168042934,-21.1471953136209,
12.));
#230007=CARTESIAN_POINT('Ctrl Pts',(-13.4988442384491,-21.1728750584173,
12.));
#230008=CARTESIAN_POINT('Ctrl Pts',(-13.5017201056088,-21.1986390835825,
12.));
#230009=CARTESIAN_POINT('Ctrl Pts',(-13.5045440957404,-21.224486942933,
12.));
#230010=CARTESIAN_POINT('Ctrl Pts',(-13.5073159019454,-21.2504181927429,
12.));
#230011=CARTESIAN_POINT('Ctrl Pts',(-13.5100352209207,-21.2764323924442,
12.));
#230012=CARTESIAN_POINT('Ctrl Pts',(-13.5127017534972,-21.3025291054236,
12.));
#230013=CARTESIAN_POINT('Ctrl Pts',(-13.5153152050554,-21.328707899634,
12.));
#230014=CARTESIAN_POINT('Ctrl Pts',(-13.5178752862461,-21.3549683486219,
12.));
#230015=CARTESIAN_POINT('Ctrl Pts',(-13.5203817122497,-21.3813100304967,
12.));
#230016=CARTESIAN_POINT('Ctrl Pts',(-13.5228342013508,-21.4077325259318,
12.));
#230017=CARTESIAN_POINT('Ctrl Pts',(-13.5252324737795,-21.4342354165253,
12.));
#230018=CARTESIAN_POINT('Ctrl Pts',(-13.5275762503553,-21.4608182828695,
12.));
#230019=CARTESIAN_POINT('Ctrl Pts',(-13.5298652514357,-21.487480703047,
12.));
#230020=CARTESIAN_POINT('Ctrl Pts',(-13.5320991952145,-21.5142222501671,
12.));
#230021=CARTESIAN_POINT('Ctrl Pts',(-13.5342777983225,-21.5410424932511,
12.));
#230022=CARTESIAN_POINT('Ctrl Pts',(-13.5364007790292,-21.5679410019011,
12.));
#230023=CARTESIAN_POINT('Ctrl Pts',(-13.5384678597206,-21.5949173499022,
12.));
#230024=CARTESIAN_POINT('Ctrl Pts',(-13.5404787697798,-21.6219711193951,
12.));
#230025=CARTESIAN_POINT('Ctrl Pts',(-13.5424332480698,-21.6491019044647,
12.));
#230026=CARTESIAN_POINT('Ctrl Pts',(-13.5443310461516,-21.676309315769,
12.));
#230027=CARTESIAN_POINT('Ctrl Pts',(-13.546171929503,-21.7035929822939,
12.));
#230028=CARTESIAN_POINT('Ctrl Pts',(-13.5479556704457,-21.730952541226,
12.));
#230029=CARTESIAN_POINT('Ctrl Pts',(-13.5496820422187,-21.7583876294532,
12.));
#230030=CARTESIAN_POINT('Ctrl Pts',(-13.5513508127232,-21.7858978745848,
12.));
#230031=CARTESIAN_POINT('Ctrl Pts',(-13.5529617381569,-21.8134828857963,
12.));
#230032=CARTESIAN_POINT('Ctrl Pts',(-13.5545145573049,-21.841142245609,
12.));
#230033=CARTESIAN_POINT('Ctrl Pts',(-13.5560089839426,-21.8688754989401,
12.));
#230034=CARTESIAN_POINT('Ctrl Pts',(-13.5574447178485,-21.8966821688876,
12.));
#230035=CARTESIAN_POINT('Ctrl Pts',(-13.5588214586672,-21.9245617765827,
12.));
#230036=CARTESIAN_POINT('Ctrl Pts',(-13.5601389185315,-21.9525138592862,
12.));
#230037=CARTESIAN_POINT('Ctrl Pts',(-13.5613968357589,-21.9805379899192,
12.));
#230038=CARTESIAN_POINT('Ctrl Pts',(-13.5625949868313,-22.0086337943431,
12.));
#230039=CARTESIAN_POINT('Ctrl Pts',(-13.5637332022393,-22.0368009736227,
12.));
#230040=CARTESIAN_POINT('Ctrl Pts',(-13.5648113688895,-22.0650393089492,
12.));
#230041=CARTESIAN_POINT('Ctrl Pts',(-13.5658294169107,-22.0933486464442,
12.));
#230042=CARTESIAN_POINT('Ctrl Pts',(-13.5667873105179,-22.1217288871823,
12.));
#230043=CARTESIAN_POINT('Ctrl Pts',(-13.5675054918922,-22.1444897575076,
12.));
#230044=CARTESIAN_POINT('Ctrl Pts',(-13.5680170531724,-22.1615922804939,
12.));
#230045=CARTESIAN_POINT('Ctrl Pts',(-13.5683460612913,-22.1730081264583,
12.));
#230046=CARTESIAN_POINT('Ctrl Pts',(-13.5685075571671,-22.1787195904339,
12.));
#230047=CARTESIAN_POINT('Ctrl Pts',(-14.6513681262571,-17.1452095830632,
0.));
#230048=CARTESIAN_POINT('Ctrl Pts',(-14.6513681262571,-17.1452095830632,
12.));
#230049=CARTESIAN_POINT('Ctrl Pts',(-14.6513711852843,-17.1452153999142,
0.));
#230050=CARTESIAN_POINT('Ctrl Pts',(-14.6513711852843,-17.1452153999142,
12.));
#230051=CARTESIAN_POINT('Ctrl Pts',(-14.6514066997196,-17.1452600887037,
0.));
#230052=CARTESIAN_POINT('Ctrl Pts',(-14.6514066997196,-17.1452600887037,
12.));
#230053=CARTESIAN_POINT('Ctrl Pts',(-14.6515481598068,-17.1454262858043,
0.));
#230054=CARTESIAN_POINT('Ctrl Pts',(-14.6515481598068,-17.1454262858043,
12.));
#230055=CARTESIAN_POINT('Ctrl Pts',(-14.6519131634508,-17.1458462295271,
0.));
#230056=CARTESIAN_POINT('Ctrl Pts',(-14.6519131634508,-17.1458462295271,
12.));
#230057=CARTESIAN_POINT('Ctrl Pts',(-14.6526624064978,-17.1466998098673,
0.));
#230058=CARTESIAN_POINT('Ctrl Pts',(-14.6526624064978,-17.1466998098673,
12.));
#230059=CARTESIAN_POINT('Ctrl Pts',(-14.6537016966184,-17.147876394491,
0.));
#230060=CARTESIAN_POINT('Ctrl Pts',(-14.6537016966184,-17.147876394491,
12.));
#230061=CARTESIAN_POINT('Ctrl Pts',(-14.655024862281,-17.1493641837558,
0.));
#230062=CARTESIAN_POINT('Ctrl Pts',(-14.655024862281,-17.1493641837558,
12.));
#230063=CARTESIAN_POINT('Ctrl Pts',(-14.6566237952435,-17.1511476869496,
0.));
#230064=CARTESIAN_POINT('Ctrl Pts',(-14.6566237952435,-17.1511476869496,
12.));
#230065=CARTESIAN_POINT('Ctrl Pts',(-14.6584900555302,-17.1532107762718,
0.));
#230066=CARTESIAN_POINT('Ctrl Pts',(-14.6584900555302,-17.1532107762718,
12.));
#230067=CARTESIAN_POINT('Ctrl Pts',(-14.6606167169642,-17.1555401986401,
0.));
#230068=CARTESIAN_POINT('Ctrl Pts',(-14.6606167169642,-17.1555401986401,
12.));
#230069=CARTESIAN_POINT('Ctrl Pts',(-14.6629987285992,-17.1581262646789,
0.));
#230070=CARTESIAN_POINT('Ctrl Pts',(-14.6629987285992,-17.1581262646789,
12.));
#230071=CARTESIAN_POINT('Ctrl Pts',(-14.6656319165057,-17.1609609517369,
0.));
#230072=CARTESIAN_POINT('Ctrl Pts',(-14.6656319165057,-17.1609609517369,
12.));
#230073=CARTESIAN_POINT('Ctrl Pts',(-14.6685123374423,-17.1640366762305,
0.));
#230074=CARTESIAN_POINT('Ctrl Pts',(-14.6685123374423,-17.1640366762305,
12.));
#230075=CARTESIAN_POINT('Ctrl Pts',(-14.671635583332,-17.167344972302,0.));
#230076=CARTESIAN_POINT('Ctrl Pts',(-14.671635583332,-17.167344972302,12.));
#230077=CARTESIAN_POINT('Ctrl Pts',(-14.6749971333867,-17.1708771619129,
0.));
#230078=CARTESIAN_POINT('Ctrl Pts',(-14.6749971333867,-17.1708771619129,
12.));
#230079=CARTESIAN_POINT('Ctrl Pts',(-14.6785925615677,-17.1746247499056,
0.));
#230080=CARTESIAN_POINT('Ctrl Pts',(-14.6785925615677,-17.1746247499056,
12.));
#230081=CARTESIAN_POINT('Ctrl Pts',(-14.6824178576167,-17.1785800350826,
0.));
#230082=CARTESIAN_POINT('Ctrl Pts',(-14.6824178576167,-17.1785800350826,
12.));
#230083=CARTESIAN_POINT('Ctrl Pts',(-14.686469452232,-17.1827361584719,
0.));
#230084=CARTESIAN_POINT('Ctrl Pts',(-14.686469452232,-17.1827361584719,
12.));
#230085=CARTESIAN_POINT('Ctrl Pts',(-14.6907440526958,-17.1870867909918,
0.));
#230086=CARTESIAN_POINT('Ctrl Pts',(-14.6907440526958,-17.1870867909918,
12.));
#230087=CARTESIAN_POINT('Ctrl Pts',(-14.6952385361706,-17.1916259308415,
0.));
#230088=CARTESIAN_POINT('Ctrl Pts',(-14.6952385361706,-17.1916259308415,
12.));
#230089=CARTESIAN_POINT('Ctrl Pts',(-14.699949811582,-17.1963476411694,
0.));
#230090=CARTESIAN_POINT('Ctrl Pts',(-14.699949811582,-17.1963476411694,
12.));
#230091=CARTESIAN_POINT('Ctrl Pts',(-14.7048748502663,-17.2012461084268,
0.));
#230092=CARTESIAN_POINT('Ctrl Pts',(-14.7048748502663,-17.2012461084268,
12.));
#230093=CARTESIAN_POINT('Ctrl Pts',(-14.7100107213586,-17.2063157097315,
0.));
#230094=CARTESIAN_POINT('Ctrl Pts',(-14.7100107213586,-17.2063157097315,
12.));
#230095=CARTESIAN_POINT('Ctrl Pts',(-14.7153546289339,-17.2115510835989,
0.));
#230096=CARTESIAN_POINT('Ctrl Pts',(-14.7153546289339,-17.2115510835989,
12.));
#230097=CARTESIAN_POINT('Ctrl Pts',(-14.7209039390327,-17.2169471814256,
0.));
#230098=CARTESIAN_POINT('Ctrl Pts',(-14.7209039390327,-17.2169471814256,
12.));
#230099=CARTESIAN_POINT('Ctrl Pts',(-14.7266561494282,-17.2224992099666,
0.));
#230100=CARTESIAN_POINT('Ctrl Pts',(-14.7266561494282,-17.2224992099666,
12.));
#230101=CARTESIAN_POINT('Ctrl Pts',(-14.7326088681163,-17.2282025904314,
0.));
#230102=CARTESIAN_POINT('Ctrl Pts',(-14.7326088681163,-17.2282025904314,
12.));
#230103=CARTESIAN_POINT('Ctrl Pts',(-14.7387597858117,-17.2340529062076,
0.));
#230104=CARTESIAN_POINT('Ctrl Pts',(-14.7387597858117,-17.2340529062076,
12.));
#230105=CARTESIAN_POINT('Ctrl Pts',(-14.7451066593792,-17.2400458713565,
0.));
#230106=CARTESIAN_POINT('Ctrl Pts',(-14.7451066593792,-17.2400458713565,
12.));
#230107=CARTESIAN_POINT('Ctrl Pts',(-14.7516473175124,-17.2461773413288,
0.));
#230108=CARTESIAN_POINT('Ctrl Pts',(-14.7516473175124,-17.2461773413288,
12.));
#230109=CARTESIAN_POINT('Ctrl Pts',(-14.7583796616617,-17.2524433146837,
0.));
#230110=CARTESIAN_POINT('Ctrl Pts',(-14.7583796616617,-17.2524433146837,
12.));
#230111=CARTESIAN_POINT('Ctrl Pts',(-14.7653016697591,-17.2588399401465,
0.));
#230112=CARTESIAN_POINT('Ctrl Pts',(-14.7653016697591,-17.2588399401465,
12.));
#230113=CARTESIAN_POINT('Ctrl Pts',(-14.7724113956731,-17.2653635155319,
0.));
#230114=CARTESIAN_POINT('Ctrl Pts',(-14.7724113956731,-17.2653635155319,
12.));
#230115=CARTESIAN_POINT('Ctrl Pts',(-14.7797069617804,-17.2720104735194,
0.));
#230116=CARTESIAN_POINT('Ctrl Pts',(-14.7797069617804,-17.2720104735194,
12.));
#230117=CARTESIAN_POINT('Ctrl Pts',(-14.787186553128,-17.2787773704849,
0.));
#230118=CARTESIAN_POINT('Ctrl Pts',(-14.787186553128,-17.2787773704849,
12.));
#230119=CARTESIAN_POINT('Ctrl Pts',(-14.7948484105249,-17.2856608733196,
0.));
#230120=CARTESIAN_POINT('Ctrl Pts',(-14.7948484105249,-17.2856608733196,
12.));
#230121=CARTESIAN_POINT('Ctrl Pts',(-14.8026908254276,-17.2926577496513,
0.));
#230122=CARTESIAN_POINT('Ctrl Pts',(-14.8026908254276,-17.2926577496513,
12.));
#230123=CARTESIAN_POINT('Ctrl Pts',(-14.8107121391036,-17.299764866148,
0.));
#230124=CARTESIAN_POINT('Ctrl Pts',(-14.8107121391036,-17.299764866148,
12.));
#230125=CARTESIAN_POINT('Ctrl Pts',(-14.8189107410162,-17.3069791853706,
0.));
#230126=CARTESIAN_POINT('Ctrl Pts',(-14.8189107410162,-17.3069791853706,
12.));
#230127=CARTESIAN_POINT('Ctrl Pts',(-14.8272850675379,-17.3142977632659,
0.));
#230128=CARTESIAN_POINT('Ctrl Pts',(-14.8272850675379,-17.3142977632659,
12.));
#230129=CARTESIAN_POINT('Ctrl Pts',(-14.8358336004197,-17.3217177462101,
0.));
#230130=CARTESIAN_POINT('Ctrl Pts',(-14.8358336004197,-17.3217177462101,
12.));
#230131=CARTESIAN_POINT('Ctrl Pts',(-14.8445548643508,-17.3292363662605,
0.));
#230132=CARTESIAN_POINT('Ctrl Pts',(-14.8445548643508,-17.3292363662605,
12.));
#230133=CARTESIAN_POINT('Ctrl Pts',(-14.8534474245434,-17.336850936485,
0.));
#230134=CARTESIAN_POINT('Ctrl Pts',(-14.8534474245434,-17.336850936485,
12.));
#230135=CARTESIAN_POINT('Ctrl Pts',(-14.8625098843417,-17.3445588463474,
0.));
#230136=CARTESIAN_POINT('Ctrl Pts',(-14.8625098843417,-17.3445588463474,
12.));
#230137=CARTESIAN_POINT('Ctrl Pts',(-14.8717408826956,-17.3523575568645,
0.));
#230138=CARTESIAN_POINT('Ctrl Pts',(-14.8717408826956,-17.3523575568645,
12.));
#230139=CARTESIAN_POINT('Ctrl Pts',(-14.8811390927423,-17.3602445978161,
0.));
#230140=CARTESIAN_POINT('Ctrl Pts',(-14.8811390927423,-17.3602445978161,
12.));
#230141=CARTESIAN_POINT('Ctrl Pts',(-14.8907032205788,-17.3682175653235,
0.));
#230142=CARTESIAN_POINT('Ctrl Pts',(-14.8907032205788,-17.3682175653235,
12.));
#230143=CARTESIAN_POINT('Ctrl Pts',(-14.900432003961,-17.3762741193076,
0.));
#230144=CARTESIAN_POINT('Ctrl Pts',(-14.900432003961,-17.3762741193076,
12.));
#230145=CARTESIAN_POINT('Ctrl Pts',(-14.9103242110058,-17.3844119809824,
0.));
#230146=CARTESIAN_POINT('Ctrl Pts',(-14.9103242110058,-17.3844119809824,
12.));
#230147=CARTESIAN_POINT('Ctrl Pts',(-14.9203786389342,-17.3926289303986,
0.));
#230148=CARTESIAN_POINT('Ctrl Pts',(-14.9203786389342,-17.3926289303986,
12.));
#230149=CARTESIAN_POINT('Ctrl Pts',(-14.9305941128757,-17.4009228040749,
0.));
#230150=CARTESIAN_POINT('Ctrl Pts',(-14.9305941128757,-17.4009228040749,
12.));
#230151=CARTESIAN_POINT('Ctrl Pts',(-14.940969484645,-17.4092914926071,
0.));
#230152=CARTESIAN_POINT('Ctrl Pts',(-14.940969484645,-17.4092914926071,
12.));
#230153=CARTESIAN_POINT('Ctrl Pts',(-14.9515036315143,-17.4177329382828,
0.));
#230154=CARTESIAN_POINT('Ctrl Pts',(-14.9515036315143,-17.4177329382828,
12.));
#230155=CARTESIAN_POINT('Ctrl Pts',(-14.9621954549827,-17.426245132709,
0.));
#230156=CARTESIAN_POINT('Ctrl Pts',(-14.9621954549827,-17.426245132709,
12.));
#230157=CARTESIAN_POINT('Ctrl Pts',(-14.9730438799452,-17.4348261151396,
0.));
#230158=CARTESIAN_POINT('Ctrl Pts',(-14.9730438799452,-17.4348261151396,
12.));
#230159=CARTESIAN_POINT('Ctrl Pts',(-14.9840478538358,-17.4434739707773,
0.));
#230160=CARTESIAN_POINT('Ctrl Pts',(-14.9840478538358,-17.4434739707773,
12.));
#230161=CARTESIAN_POINT('Ctrl Pts',(-14.9952063457778,-17.4521868291004,
0.));
#230162=CARTESIAN_POINT('Ctrl Pts',(-14.9952063457778,-17.4521868291004,
12.));
#230163=CARTESIAN_POINT('Ctrl Pts',(-15.0065183456921,-17.4609628621418,
0.));
#230164=CARTESIAN_POINT('Ctrl Pts',(-15.0065183456921,-17.4609628621418,
12.));
#230165=CARTESIAN_POINT('Ctrl Pts',(-15.0179828635086,-17.4698002829356,
0.));
#230166=CARTESIAN_POINT('Ctrl Pts',(-15.0179828635086,-17.4698002829356,
12.));
#230167=CARTESIAN_POINT('Ctrl Pts',(-15.029598928488,-17.4786973441417,
0.));
#230168=CARTESIAN_POINT('Ctrl Pts',(-15.029598928488,-17.4786973441417,
12.));
#230169=CARTESIAN_POINT('Ctrl Pts',(-15.0413655884993,-17.4876523366178,
0.));
#230170=CARTESIAN_POINT('Ctrl Pts',(-15.0413655884993,-17.4876523366178,
12.));
#230171=CARTESIAN_POINT('Ctrl Pts',(-15.0532819093085,-17.4966635880245,
0.));
#230172=CARTESIAN_POINT('Ctrl Pts',(-15.0532819093085,-17.4966635880245,
12.));
#230173=CARTESIAN_POINT('Ctrl Pts',(-15.0653469738306,-17.5057294613874,
0.));
#230174=CARTESIAN_POINT('Ctrl Pts',(-15.0653469738306,-17.5057294613874,
12.));
#230175=CARTESIAN_POINT('Ctrl Pts',(-15.0775598815748,-17.5148483539683,
0.));
#230176=CARTESIAN_POINT('Ctrl Pts',(-15.0775598815748,-17.5148483539683,
12.));
#230177=CARTESIAN_POINT('Ctrl Pts',(-15.0899197481082,-17.5240186961788,
0.));
#230178=CARTESIAN_POINT('Ctrl Pts',(-15.0899197481082,-17.5240186961788,
12.));
#230179=CARTESIAN_POINT('Ctrl Pts',(-15.1024257045033,-17.5332389504829,
0.));
#230180=CARTESIAN_POINT('Ctrl Pts',(-15.1024257045033,-17.5332389504829,
12.));
#230181=CARTESIAN_POINT('Ctrl Pts',(-15.1150768967729,-17.5425076102966,
0.));
#230182=CARTESIAN_POINT('Ctrl Pts',(-15.1150768967729,-17.5425076102966,
12.));
#230183=CARTESIAN_POINT('Ctrl Pts',(-15.127872485314,-17.5518231989122,
0.));
#230184=CARTESIAN_POINT('Ctrl Pts',(-15.127872485314,-17.5518231989122,
12.));
#230185=CARTESIAN_POINT('Ctrl Pts',(-15.1408116444877,-17.5611842686196,
0.));
#230186=CARTESIAN_POINT('Ctrl Pts',(-15.1408116444877,-17.5611842686196,
12.));
#230187=CARTESIAN_POINT('Ctrl Pts',(-15.1538935621715,-17.570589399803,
0.));
#230188=CARTESIAN_POINT('Ctrl Pts',(-15.1538935621715,-17.570589399803,
12.));
#230189=CARTESIAN_POINT('Ctrl Pts',(-15.1671174393137,-17.5800372000539,
0.));
#230190=CARTESIAN_POINT('Ctrl Pts',(-15.1671174393137,-17.5800372000539,
12.));
#230191=CARTESIAN_POINT('Ctrl Pts',(-15.1804824894605,-17.5895263032592,
0.));
#230192=CARTESIAN_POINT('Ctrl Pts',(-15.1804824894605,-17.5895263032592,
12.));
#230193=CARTESIAN_POINT('Ctrl Pts',(-15.1939879383268,-17.5990553687595,
0.));
#230194=CARTESIAN_POINT('Ctrl Pts',(-15.1939879383268,-17.5990553687595,
12.));
#230195=CARTESIAN_POINT('Ctrl Pts',(-15.2076330234686,-17.6086230806497,
0.));
#230196=CARTESIAN_POINT('Ctrl Pts',(-15.2076330234686,-17.6086230806497,
12.));
#230197=CARTESIAN_POINT('Ctrl Pts',(-15.22141699392,-17.6182281470467,0.));
#230198=CARTESIAN_POINT('Ctrl Pts',(-15.22141699392,-17.6182281470467,12.));
#230199=CARTESIAN_POINT('Ctrl Pts',(-15.2353391098367,-17.6278692993765,
0.));
#230200=CARTESIAN_POINT('Ctrl Pts',(-15.2353391098367,-17.6278692993765,
12.));
#230201=CARTESIAN_POINT('Ctrl Pts',(-15.2493986421091,-17.637545291637,
0.));
#230202=CARTESIAN_POINT('Ctrl Pts',(-15.2493986421091,-17.637545291637,
12.));
#230203=CARTESIAN_POINT('Ctrl Pts',(-15.263594872029,-17.6472548997329,
0.));
#230204=CARTESIAN_POINT('Ctrl Pts',(-15.263594872029,-17.6472548997329,
12.));
#230205=CARTESIAN_POINT('Ctrl Pts',(-15.2779270910238,-17.6569969209,0.));
#230206=CARTESIAN_POINT('Ctrl Pts',(-15.2779270910238,-17.6569969209,12.));
#230207=CARTESIAN_POINT('Ctrl Pts',(-15.2923946003598,-17.6667701731041,
0.));
#230208=CARTESIAN_POINT('Ctrl Pts',(-15.2923946003598,-17.6667701731041,
12.));
#230209=CARTESIAN_POINT('Ctrl Pts',(-15.3069967108501,-17.6765734944559,
0.));
#230210=CARTESIAN_POINT('Ctrl Pts',(-15.3069967108501,-17.6765734944559,
12.));
#230211=CARTESIAN_POINT('Ctrl Pts',(-15.3217327425341,-17.6864057426052,
0.));
#230212=CARTESIAN_POINT('Ctrl Pts',(-15.3217327425341,-17.6864057426052,
12.));
#230213=CARTESIAN_POINT('Ctrl Pts',(-15.3366020244069,-17.6962657941984,
0.));
#230214=CARTESIAN_POINT('Ctrl Pts',(-15.3366020244069,-17.6962657941984,
12.));
#230215=CARTESIAN_POINT('Ctrl Pts',(-15.3516038942064,-17.7061525444044,
0.));
#230216=CARTESIAN_POINT('Ctrl Pts',(-15.3516038942064,-17.7061525444044,
12.));
#230217=CARTESIAN_POINT('Ctrl Pts',(-15.3667376981702,-17.7160649064208,
0.));
#230218=CARTESIAN_POINT('Ctrl Pts',(-15.3667376981702,-17.7160649064208,
12.));
#230219=CARTESIAN_POINT('Ctrl Pts',(-15.3820027907965,-17.7260018109923,
0.));
#230220=CARTESIAN_POINT('Ctrl Pts',(-15.3820027907965,-17.7260018109923,
12.));
#230221=CARTESIAN_POINT('Ctrl Pts',(-15.3973985345796,-17.7359622059143,
0.));
#230222=CARTESIAN_POINT('Ctrl Pts',(-15.3973985345796,-17.7359622059143,
12.));
#230223=CARTESIAN_POINT('Ctrl Pts',(-15.4129242997828,-17.7459450555803,
0.));
#230224=CARTESIAN_POINT('Ctrl Pts',(-15.4129242997828,-17.7459450555803,
12.));
#230225=CARTESIAN_POINT('Ctrl Pts',(-15.4285794642658,-17.7559493405871,
0.));
#230226=CARTESIAN_POINT('Ctrl Pts',(-15.4285794642658,-17.7559493405871,
12.));
#230227=CARTESIAN_POINT('Ctrl Pts',(-15.4443634132865,-17.765974057326,
0.));
#230228=CARTESIAN_POINT('Ctrl Pts',(-15.4443634132865,-17.765974057326,
12.));
#230229=CARTESIAN_POINT('Ctrl Pts',(-15.460275539302,-17.7760182175817,
0.));
#230230=CARTESIAN_POINT('Ctrl Pts',(-15.460275539302,-17.7760182175817,
12.));
#230231=CARTESIAN_POINT('Ctrl Pts',(-15.4763152417506,-17.7860808481229,
0.));
#230232=CARTESIAN_POINT('Ctrl Pts',(-15.4763152417506,-17.7860808481229,
12.));
#230233=CARTESIAN_POINT('Ctrl Pts',(-15.4924819268529,-17.7961609903161,
0.));
#230234=CARTESIAN_POINT('Ctrl Pts',(-15.4924819268529,-17.7961609903161,
12.));
#230235=CARTESIAN_POINT('Ctrl Pts',(-15.5087750074728,-17.8062576997964,
0.));
#230236=CARTESIAN_POINT('Ctrl Pts',(-15.5087750074728,-17.8062576997964,
12.));
#230237=CARTESIAN_POINT('Ctrl Pts',(-15.5251939029558,-17.8163700461262,
0.));
#230238=CARTESIAN_POINT('Ctrl Pts',(-15.5251939029558,-17.8163700461262,
12.));
#230239=CARTESIAN_POINT('Ctrl Pts',(-15.5417380389639,-17.8264971124606,
0.));
#230240=CARTESIAN_POINT('Ctrl Pts',(-15.5417380389639,-17.8264971124606,
12.));
#230241=CARTESIAN_POINT('Ctrl Pts',(-15.5584068472976,-17.8366379952078,
0.));
#230242=CARTESIAN_POINT('Ctrl Pts',(-15.5584068472976,-17.8366379952078,
12.));
#230243=CARTESIAN_POINT('Ctrl Pts',(-15.5751997657154,-17.8467918036976,
0.));
#230244=CARTESIAN_POINT('Ctrl Pts',(-15.5751997657154,-17.8467918036976,
12.));
#230245=CARTESIAN_POINT('Ctrl Pts',(-15.5921162378183,-17.8569576598996,
0.));
#230246=CARTESIAN_POINT('Ctrl Pts',(-15.5921162378183,-17.8569576598996,
12.));
#230247=CARTESIAN_POINT('Ctrl Pts',(-15.6091557129205,-17.8671346981388,
0.));
#230248=CARTESIAN_POINT('Ctrl Pts',(-15.6091557129205,-17.8671346981388,
12.));
#230249=CARTESIAN_POINT('Ctrl Pts',(-15.6263176459107,-17.8773220648125,
0.));
#230250=CARTESIAN_POINT('Ctrl Pts',(-15.6263176459107,-17.8773220648125,
12.));
#230251=CARTESIAN_POINT('Ctrl Pts',(-15.6436014971088,-17.8875189181095,
0.));
#230252=CARTESIAN_POINT('Ctrl Pts',(-15.6436014971088,-17.8875189181095,
12.));
#230253=CARTESIAN_POINT('Ctrl Pts',(-15.6610067321036,-17.8977244277247,
0.));
#230254=CARTESIAN_POINT('Ctrl Pts',(-15.6610067321036,-17.8977244277247,
12.));
#230255=CARTESIAN_POINT('Ctrl Pts',(-15.6785328216467,-17.9079377746118,
0.));
#230256=CARTESIAN_POINT('Ctrl Pts',(-15.6785328216467,-17.9079377746118,
12.));
#230257=CARTESIAN_POINT('Ctrl Pts',(-15.6961792415526,-17.918158150746,
0.));
#230258=CARTESIAN_POINT('Ctrl Pts',(-15.6961792415526,-17.918158150746,
12.));
#230259=CARTESIAN_POINT('Ctrl Pts',(-15.713945472584,-17.9283847588837,
0.));
#230260=CARTESIAN_POINT('Ctrl Pts',(-15.713945472584,-17.9283847588837,
12.));
#230261=CARTESIAN_POINT('Ctrl Pts',(-15.7318310003334,-17.9386168123261,
0.));
#230262=CARTESIAN_POINT('Ctrl Pts',(-15.7318310003334,-17.9386168123261,
12.));
#230263=CARTESIAN_POINT('Ctrl Pts',(-15.7498353150856,-17.9488535346776,
0.));
#230264=CARTESIAN_POINT('Ctrl Pts',(-15.7498353150856,-17.9488535346776,
12.));
#230265=CARTESIAN_POINT('Ctrl Pts',(-15.7679579117072,-17.9590941596236,
0.));
#230266=CARTESIAN_POINT('Ctrl Pts',(-15.7679579117072,-17.9590941596236,
12.));
#230267=CARTESIAN_POINT('Ctrl Pts',(-15.786198289572,-17.9693379307297,
0.));
#230268=CARTESIAN_POINT('Ctrl Pts',(-15.786198289572,-17.9693379307297,
12.));
#230269=CARTESIAN_POINT('Ctrl Pts',(-15.8045559524674,-17.9795841012383,
0.));
#230270=CARTESIAN_POINT('Ctrl Pts',(-15.8045559524674,-17.9795841012383,
12.));
#230271=CARTESIAN_POINT('Ctrl Pts',(-15.8230304084963,-17.9898319338664,
0.));
#230272=CARTESIAN_POINT('Ctrl Pts',(-15.8230304084963,-17.9898319338664,
12.));
#230273=CARTESIAN_POINT('Ctrl Pts',(-15.8416211699682,-18.0000807006055,
0.));
#230274=CARTESIAN_POINT('Ctrl Pts',(-15.8416211699682,-18.0000807006055,
12.));
#230275=CARTESIAN_POINT('Ctrl Pts',(-15.8603277532834,-18.010329682521,
0.));
#230276=CARTESIAN_POINT('Ctrl Pts',(-15.8603277532834,-18.010329682521,
12.));
#230277=CARTESIAN_POINT('Ctrl Pts',(-15.8791496788685,-18.0205781695773,
0.));
#230278=CARTESIAN_POINT('Ctrl Pts',(-15.8791496788685,-18.0205781695773,
12.));
#230279=CARTESIAN_POINT('Ctrl Pts',(-15.8980864711043,-18.0308254604638,
0.));
#230280=CARTESIAN_POINT('Ctrl Pts',(-15.8980864711043,-18.0308254604638,
12.));
#230281=CARTESIAN_POINT('Ctrl Pts',(-15.9171376582436,-18.0410708624208,
0.));
#230282=CARTESIAN_POINT('Ctrl Pts',(-15.9171376582436,-18.0410708624208,
12.));
#230283=CARTESIAN_POINT('Ctrl Pts',(-15.9363027723244,-18.0513136910691,
0.));
#230284=CARTESIAN_POINT('Ctrl Pts',(-15.9363027723244,-18.0513136910691,
12.));
#230285=CARTESIAN_POINT('Ctrl Pts',(-15.9555813490645,-18.061553270236,
0.));
#230286=CARTESIAN_POINT('Ctrl Pts',(-15.9555813490645,-18.061553270236,
12.));
#230287=CARTESIAN_POINT('Ctrl Pts',(-15.9749729277848,-18.071788931796,
0.));
#230288=CARTESIAN_POINT('Ctrl Pts',(-15.9749729277848,-18.071788931796,
12.));
#230289=CARTESIAN_POINT('Ctrl Pts',(-15.9944770513616,-18.0820200155238,
0.));
#230290=CARTESIAN_POINT('Ctrl Pts',(-15.9944770513616,-18.0820200155238,
12.));
#230291=CARTESIAN_POINT('Ctrl Pts',(-16.0140932661612,-18.0922458689464,
0.));
#230292=CARTESIAN_POINT('Ctrl Pts',(-16.0140932661612,-18.0922458689464,
12.));
#230293=CARTESIAN_POINT('Ctrl Pts',(-16.0338211219694,-18.1024658471966,
0.));
#230294=CARTESIAN_POINT('Ctrl Pts',(-16.0338211219694,-18.1024658471966,
12.));
#230295=CARTESIAN_POINT('Ctrl Pts',(-16.0536601719124,-18.1126793128688,
0.));
#230296=CARTESIAN_POINT('Ctrl Pts',(-16.0536601719124,-18.1126793128688,
12.));
#230297=CARTESIAN_POINT('Ctrl Pts',(-16.0736099723665,-18.1228856358746,
0.));
#230298=CARTESIAN_POINT('Ctrl Pts',(-16.0736099723665,-18.1228856358746,
12.));
#230299=CARTESIAN_POINT('Ctrl Pts',(-16.0936700829108,-18.1330841933099,
0.));
#230300=CARTESIAN_POINT('Ctrl Pts',(-16.0936700829108,-18.1330841933099,
12.));
#230301=CARTESIAN_POINT('Ctrl Pts',(-16.1138400662791,-18.1432743693231,
0.));
#230302=CARTESIAN_POINT('Ctrl Pts',(-16.1138400662791,-18.1432743693231,
12.));
#230303=CARTESIAN_POINT('Ctrl Pts',(-16.1341194882987,-18.153455554985,
0.));
#230304=CARTESIAN_POINT('Ctrl Pts',(-16.1341194882987,-18.153455554985,
12.));
#230305=CARTESIAN_POINT('Ctrl Pts',(-16.1545079178261,-18.1636271481616,
0.));
#230306=CARTESIAN_POINT('Ctrl Pts',(-16.1545079178261,-18.1636271481616,
12.));
#230307=CARTESIAN_POINT('Ctrl Pts',(-16.1750049266673,-18.1737885533852,
0.));
#230308=CARTESIAN_POINT('Ctrl Pts',(-16.1750049266673,-18.1737885533852,
12.));
#230309=CARTESIAN_POINT('Ctrl Pts',(-16.1956100895076,-18.1839391817335,
0.));
#230310=CARTESIAN_POINT('Ctrl Pts',(-16.1956100895076,-18.1839391817335,
12.));
#230311=CARTESIAN_POINT('Ctrl Pts',(-16.2163229838878,-18.1940784507232,
0.));
#230312=CARTESIAN_POINT('Ctrl Pts',(-16.2163229838878,-18.1940784507232,
12.));
#230313=CARTESIAN_POINT('Ctrl Pts',(-16.237143190164,-18.2042057842037,
0.));
#230314=CARTESIAN_POINT('Ctrl Pts',(-16.237143190164,-18.2042057842037,
12.));
#230315=CARTESIAN_POINT('Ctrl Pts',(-16.2580702914615,-18.214320612253,
0.));
#230316=CARTESIAN_POINT('Ctrl Pts',(-16.2580702914615,-18.214320612253,
12.));
#230317=CARTESIAN_POINT('Ctrl Pts',(-16.2791038736223,-18.2244223710745,
0.));
#230318=CARTESIAN_POINT('Ctrl Pts',(-16.2791038736223,-18.2244223710745,
12.));
#230319=CARTESIAN_POINT('Ctrl Pts',(-16.3002435251378,-18.2345105028981,
0.));
#230320=CARTESIAN_POINT('Ctrl Pts',(-16.3002435251378,-18.2345105028981,
12.));
#230321=CARTESIAN_POINT('Ctrl Pts',(-16.3214888370988,-18.2445844558742,
0.));
#230322=CARTESIAN_POINT('Ctrl Pts',(-16.3214888370988,-18.2445844558742,
12.));
#230323=CARTESIAN_POINT('Ctrl Pts',(-16.342839403159,-18.2546436839609,
0.));
#230324=CARTESIAN_POINT('Ctrl Pts',(-16.342839403159,-18.2546436839609,
12.));
#230325=CARTESIAN_POINT('Ctrl Pts',(-16.3642948194869,-18.2646876468169,
0.));
#230326=CARTESIAN_POINT('Ctrl Pts',(-16.3642948194869,-18.2646876468169,
12.));
#230327=CARTESIAN_POINT('Ctrl Pts',(-16.385854684708,-18.2747158096934,
0.));
#230328=CARTESIAN_POINT('Ctrl Pts',(-16.385854684708,-18.2747158096934,
12.));
#230329=CARTESIAN_POINT('Ctrl Pts',(-16.4075185998454,-18.2847276433308,
0.));
#230330=CARTESIAN_POINT('Ctrl Pts',(-16.4075185998454,-18.2847276433308,
12.));
#230331=CARTESIAN_POINT('Ctrl Pts',(-16.4292861682377,-18.2947226238509,
0.));
#230332=CARTESIAN_POINT('Ctrl Pts',(-16.4292861682377,-18.2947226238509,
12.));
#230333=CARTESIAN_POINT('Ctrl Pts',(-16.4511569955231,-18.3047002326858,
0.));
#230334=CARTESIAN_POINT('Ctrl Pts',(-16.4511569955231,-18.3047002326858,
12.));
#230335=CARTESIAN_POINT('Ctrl Pts',(-16.4731306896439,-18.3146599565229,
0.));
#230336=CARTESIAN_POINT('Ctrl Pts',(-16.4731306896439,-18.3146599565229,
12.));
#230337=CARTESIAN_POINT('Ctrl Pts',(-16.4952068608344,-18.3246012872468,
0.));
#230338=CARTESIAN_POINT('Ctrl Pts',(-16.4952068608344,-18.3246012872468,
12.));
#230339=CARTESIAN_POINT('Ctrl Pts',(-16.5173851216045,-18.3345237218864,
0.));
#230340=CARTESIAN_POINT('Ctrl Pts',(-16.5173851216045,-18.3345237218864,
12.));
#230341=CARTESIAN_POINT('Ctrl Pts',(-16.539665086714,-18.3444267625601,
0.));
#230342=CARTESIAN_POINT('Ctrl Pts',(-16.539665086714,-18.3444267625601,
12.));
#230343=CARTESIAN_POINT('Ctrl Pts',(-16.5620463731414,-18.3543099164331,
0.));
#230344=CARTESIAN_POINT('Ctrl Pts',(-16.5620463731414,-18.3543099164331,
12.));
#230345=CARTESIAN_POINT('Ctrl Pts',(-16.5845286000219,-18.364172695589,
0.));
#230346=CARTESIAN_POINT('Ctrl Pts',(-16.5845286000219,-18.364172695589,
12.));
#230347=CARTESIAN_POINT('Ctrl Pts',(-16.6071113885711,-18.3740146168879,
0.));
#230348=CARTESIAN_POINT('Ctrl Pts',(-16.6071113885711,-18.3740146168879,
12.));
#230349=CARTESIAN_POINT('Ctrl Pts',(-16.6297943620056,-18.3838352018327,
0.));
#230350=CARTESIAN_POINT('Ctrl Pts',(-16.6297943620056,-18.3838352018327,
12.));
#230351=CARTESIAN_POINT('Ctrl Pts',(-16.6525771454513,-18.3936339764332,
0.));
#230352=CARTESIAN_POINT('Ctrl Pts',(-16.6525771454513,-18.3936339764332,
12.));
#230353=CARTESIAN_POINT('Ctrl Pts',(-16.6754593658513,-18.4034104710789,
0.));
#230354=CARTESIAN_POINT('Ctrl Pts',(-16.6754593658513,-18.4034104710789,
12.));
#230355=CARTESIAN_POINT('Ctrl Pts',(-16.698440651849,-18.4131642203989,
0.));
#230356=CARTESIAN_POINT('Ctrl Pts',(-16.698440651849,-18.4131642203989,
12.));
#230357=CARTESIAN_POINT('Ctrl Pts',(-16.7215206338818,-18.4228947633186,
0.));
#230358=CARTESIAN_POINT('Ctrl Pts',(-16.7215206338818,-18.4228947633186,
12.));
#230359=CARTESIAN_POINT('Ctrl Pts',(-16.7446989442882,-18.4326016431392,
0.));
#230360=CARTESIAN_POINT('Ctrl Pts',(-16.7446989442882,-18.4326016431392,
12.));
#230361=CARTESIAN_POINT('Ctrl Pts',(-16.7679752173992,-18.4422844076099,
0.));
#230362=CARTESIAN_POINT('Ctrl Pts',(-16.7679752173992,-18.4422844076099,
12.));
#230363=CARTESIAN_POINT('Ctrl Pts',(-16.791349089629,-18.4519426090124,
0.));
#230364=CARTESIAN_POINT('Ctrl Pts',(-16.791349089629,-18.4519426090124,
12.));
#230365=CARTESIAN_POINT('Ctrl Pts',(-16.8148201995472,-18.4615758042305,
0.));
#230366=CARTESIAN_POINT('Ctrl Pts',(-16.8148201995472,-18.4615758042305,
12.));
#230367=CARTESIAN_POINT('Ctrl Pts',(-16.8383881879707,-18.4711835548622,
0.));
#230368=CARTESIAN_POINT('Ctrl Pts',(-16.8383881879707,-18.4711835548622,
12.));
#230369=CARTESIAN_POINT('Ctrl Pts',(-16.8620526977169,-18.4807654268769,
0.));
#230370=CARTESIAN_POINT('Ctrl Pts',(-16.8620526977169,-18.4807654268769,
12.));
#230371=CARTESIAN_POINT('Ctrl Pts',(-16.8858133733086,-18.4903209902226,
0.));
#230372=CARTESIAN_POINT('Ctrl Pts',(-16.8858133733086,-18.4903209902226,
12.));
#230373=CARTESIAN_POINT('Ctrl Pts',(-16.9096698606942,-18.4998498184619,
0.));
#230374=CARTESIAN_POINT('Ctrl Pts',(-16.9096698606942,-18.4998498184619,
12.));
#230375=CARTESIAN_POINT('Ctrl Pts',(-16.9336218069353,-18.5093514883835,
0.));
#230376=CARTESIAN_POINT('Ctrl Pts',(-16.9336218069353,-18.5093514883835,
12.));
#230377=CARTESIAN_POINT('Ctrl Pts',(-16.957668859934,-18.518825579666,0.));
#230378=CARTESIAN_POINT('Ctrl Pts',(-16.957668859934,-18.518825579666,12.));
#230379=CARTESIAN_POINT('Ctrl Pts',(-16.9818106680382,-18.5282716744198,
0.));
#230380=CARTESIAN_POINT('Ctrl Pts',(-16.9818106680382,-18.5282716744198,
12.));
#230381=CARTESIAN_POINT('Ctrl Pts',(-17.0060468805099,-18.5376893576961,
0.));
#230382=CARTESIAN_POINT('Ctrl Pts',(-17.0060468805099,-18.5376893576961,
12.));
#230383=CARTESIAN_POINT('Ctrl Pts',(-17.030377148174,-18.5470782182089,
0.));
#230384=CARTESIAN_POINT('Ctrl Pts',(-17.030377148174,-18.5470782182089,
12.));
#230385=CARTESIAN_POINT('Ctrl Pts',(-17.0548011239751,-18.5564378489628,
0.));
#230386=CARTESIAN_POINT('Ctrl Pts',(-17.0548011239751,-18.5564378489628,
12.));
#230387=CARTESIAN_POINT('Ctrl Pts',(-17.0793184636079,-18.5657678479788,
0.));
#230388=CARTESIAN_POINT('Ctrl Pts',(-17.0793184636079,-18.5657678479788,
12.));
#230389=CARTESIAN_POINT('Ctrl Pts',(-17.1039288260002,-18.5750678188543,
0.));
#230390=CARTESIAN_POINT('Ctrl Pts',(-17.1039288260002,-18.5750678188543,
12.));
#230391=CARTESIAN_POINT('Ctrl Pts',(-17.1286318741185,-18.5843373717253,
0.));
#230392=CARTESIAN_POINT('Ctrl Pts',(-17.1286318741185,-18.5843373717253,
12.));
#230393=CARTESIAN_POINT('Ctrl Pts',(-17.1534272741646,-18.5935761222833,
0.));
#230394=CARTESIAN_POINT('Ctrl Pts',(-17.1534272741646,-18.5935761222833,
12.));
#230395=CARTESIAN_POINT('Ctrl Pts',(-17.1783146940131,-18.6027836898826,
0.));
#230396=CARTESIAN_POINT('Ctrl Pts',(-17.1783146940131,-18.6027836898826,
12.));
#230397=CARTESIAN_POINT('Ctrl Pts',(-17.2032938019288,-18.6119596959957,
0.));
#230398=CARTESIAN_POINT('Ctrl Pts',(-17.2032938019288,-18.6119596959957,
12.));
#230399=CARTESIAN_POINT('Ctrl Pts',(-17.2283642650519,-18.6211037624041,
0.));
#230400=CARTESIAN_POINT('Ctrl Pts',(-17.2283642650519,-18.6211037624041,
12.));
#230401=CARTESIAN_POINT('Ctrl Pts',(-17.2535257482186,-18.630215509794,
0.));
#230402=CARTESIAN_POINT('Ctrl Pts',(-17.2535257482186,-18.630215509794,
12.));
#230403=CARTESIAN_POINT('Ctrl Pts',(-17.278777912021,-18.639294555474,0.));
#230404=CARTESIAN_POINT('Ctrl Pts',(-17.278777912021,-18.639294555474,12.));
#230405=CARTESIAN_POINT('Ctrl Pts',(-17.3041204135069,-18.6483405141853,
0.));
#230406=CARTESIAN_POINT('Ctrl Pts',(-17.3041204135069,-18.6483405141853,
12.));
#230407=CARTESIAN_POINT('Ctrl Pts',(-17.3295529098612,-18.6573530024019,
0.));
#230408=CARTESIAN_POINT('Ctrl Pts',(-17.3295529098612,-18.6573530024019,
12.));
#230409=CARTESIAN_POINT('Ctrl Pts',(-17.3550750612438,-18.6663316416569,
0.));
#230410=CARTESIAN_POINT('Ctrl Pts',(-17.3550750612438,-18.6663316416569,
12.));
#230411=CARTESIAN_POINT('Ctrl Pts',(-17.3806865340744,-18.6752760624045,
0.));
#230412=CARTESIAN_POINT('Ctrl Pts',(-17.3806865340744,-18.6752760624045,
12.));
#230413=CARTESIAN_POINT('Ctrl Pts',(-17.4063870038563,-18.6841859073472,
0.));
#230414=CARTESIAN_POINT('Ctrl Pts',(-17.4063870038563,-18.6841859073472,
12.));
#230415=CARTESIAN_POINT('Ctrl Pts',(-17.4321761588148,-18.6930608357421,
0.));
#230416=CARTESIAN_POINT('Ctrl Pts',(-17.4321761588148,-18.6930608357421,
12.));
#230417=CARTESIAN_POINT('Ctrl Pts',(-17.4580537012764,-18.7019005250322,
0.));
#230418=CARTESIAN_POINT('Ctrl Pts',(-17.4580537012764,-18.7019005250322,
12.));
#230419=CARTESIAN_POINT('Ctrl Pts',(-17.4840193397176,-18.7107046613941,
0.));
#230420=CARTESIAN_POINT('Ctrl Pts',(-17.4840193397176,-18.7107046613941,
12.));
#230421=CARTESIAN_POINT('Ctrl Pts',(-17.5100727820891,-18.7194729318127,
0.));
#230422=CARTESIAN_POINT('Ctrl Pts',(-17.5100727820891,-18.7194729318127,
12.));
#230423=CARTESIAN_POINT('Ctrl Pts',(-17.5362137287604,-18.728205015716,
0.));
#230424=CARTESIAN_POINT('Ctrl Pts',(-17.5362137287604,-18.728205015716,
12.));
#230425=CARTESIAN_POINT('Ctrl Pts',(-17.5624418653248,-18.7369005764558,
0.));
#230426=CARTESIAN_POINT('Ctrl Pts',(-17.5624418653248,-18.7369005764558,
12.));
#230427=CARTESIAN_POINT('Ctrl Pts',(-17.5887568561361,-18.7455592536667,
0.));
#230428=CARTESIAN_POINT('Ctrl Pts',(-17.5887568561361,-18.7455592536667,
12.));
#230429=CARTESIAN_POINT('Ctrl Pts',(-17.6151583356989,-18.7541806530935,
0.));
#230430=CARTESIAN_POINT('Ctrl Pts',(-17.6151583356989,-18.7541806530935,
12.));
#230431=CARTESIAN_POINT('Ctrl Pts',(-17.6416459210646,-18.7627643613138,
0.));
#230432=CARTESIAN_POINT('Ctrl Pts',(-17.6416459210646,-18.7627643613138,
12.));
#230433=CARTESIAN_POINT('Ctrl Pts',(-17.6682192274197,-18.7713099642673,
0.));
#230434=CARTESIAN_POINT('Ctrl Pts',(-17.6682192274197,-18.7713099642673,
12.));
#230435=CARTESIAN_POINT('Ctrl Pts',(-17.6948778822982,-18.7798170641305,
0.));
#230436=CARTESIAN_POINT('Ctrl Pts',(-17.6948778822982,-18.7798170641305,
12.));
#230437=CARTESIAN_POINT('Ctrl Pts',(-17.7216215409019,-18.7882852976016,
0.));
#230438=CARTESIAN_POINT('Ctrl Pts',(-17.7216215409019,-18.7882852976016,
12.));
#230439=CARTESIAN_POINT('Ctrl Pts',(-17.7484498996917,-18.7967143519444,
0.));
#230440=CARTESIAN_POINT('Ctrl Pts',(-17.7484498996917,-18.7967143519444,
12.));
#230441=CARTESIAN_POINT('Ctrl Pts',(-17.7753627137898,-18.8051039860543,
0.));
#230442=CARTESIAN_POINT('Ctrl Pts',(-17.7753627137898,-18.8051039860543,
12.));
#230443=CARTESIAN_POINT('Ctrl Pts',(-17.8023598011135,-18.8134540340581,
0.));
#230444=CARTESIAN_POINT('Ctrl Pts',(-17.8023598011135,-18.8134540340581,
12.));
#230445=CARTESIAN_POINT('Ctrl Pts',(-17.8294410311105,-18.8217643886368,
0.));
#230446=CARTESIAN_POINT('Ctrl Pts',(-17.8294410311105,-18.8217643886368,
12.));
#230447=CARTESIAN_POINT('Ctrl Pts',(-17.8566063174871,-18.8300349896187,
0.));
#230448=CARTESIAN_POINT('Ctrl Pts',(-17.8566063174871,-18.8300349896187,
12.));
#230449=CARTESIAN_POINT('Ctrl Pts',(-17.8784057509434,-18.8366196462746,
0.));
#230450=CARTESIAN_POINT('Ctrl Pts',(-17.8784057509434,-18.8366196462746,
12.));
#230451=CARTESIAN_POINT('Ctrl Pts',(-17.8947931177853,-18.8415402351882,
0.));
#230452=CARTESIAN_POINT('Ctrl Pts',(-17.8947931177853,-18.8415402351882,
12.));
#230453=CARTESIAN_POINT('Ctrl Pts',(-17.9057348246611,-18.8448126709726,
0.));
#230454=CARTESIAN_POINT('Ctrl Pts',(-17.9057348246611,-18.8448126709726,
12.));
#230455=CARTESIAN_POINT('Ctrl Pts',(-17.9112098770111,-18.8464468996588,
0.));
#230456=CARTESIAN_POINT('Ctrl Pts',(-17.9112098770111,-18.8464468996588,
12.));
#230457=CARTESIAN_POINT('',(-17.9112098770111,-18.8464468996588,0.));
#230458=CARTESIAN_POINT('Ctrl Pts',(-14.6513681262571,-17.1452095830632,
0.));
#230459=CARTESIAN_POINT('Ctrl Pts',(-14.6513711852843,-17.1452153999142,
0.));
#230460=CARTESIAN_POINT('Ctrl Pts',(-14.6514066997196,-17.1452600887037,
0.));
#230461=CARTESIAN_POINT('Ctrl Pts',(-14.6515481598068,-17.1454262858043,
0.));
#230462=CARTESIAN_POINT('Ctrl Pts',(-14.6519131634508,-17.1458462295271,
0.));
#230463=CARTESIAN_POINT('Ctrl Pts',(-14.6526624064978,-17.1466998098673,
0.));
#230464=CARTESIAN_POINT('Ctrl Pts',(-14.6537016966184,-17.147876394491,
0.));
#230465=CARTESIAN_POINT('Ctrl Pts',(-14.655024862281,-17.1493641837558,
0.));
#230466=CARTESIAN_POINT('Ctrl Pts',(-14.6566237952435,-17.1511476869496,
0.));
#230467=CARTESIAN_POINT('Ctrl Pts',(-14.6584900555302,-17.1532107762718,
0.));
#230468=CARTESIAN_POINT('Ctrl Pts',(-14.6606167169642,-17.1555401986401,
0.));
#230469=CARTESIAN_POINT('Ctrl Pts',(-14.6629987285992,-17.1581262646789,
0.));
#230470=CARTESIAN_POINT('Ctrl Pts',(-14.6656319165057,-17.1609609517369,
0.));
#230471=CARTESIAN_POINT('Ctrl Pts',(-14.6685123374423,-17.1640366762305,
0.));
#230472=CARTESIAN_POINT('Ctrl Pts',(-14.671635583332,-17.167344972302,0.));
#230473=CARTESIAN_POINT('Ctrl Pts',(-14.6749971333867,-17.1708771619129,
0.));
#230474=CARTESIAN_POINT('Ctrl Pts',(-14.6785925615677,-17.1746247499056,
0.));
#230475=CARTESIAN_POINT('Ctrl Pts',(-14.6824178576167,-17.1785800350826,
0.));
#230476=CARTESIAN_POINT('Ctrl Pts',(-14.686469452232,-17.1827361584719,
0.));
#230477=CARTESIAN_POINT('Ctrl Pts',(-14.6907440526958,-17.1870867909918,
0.));
#230478=CARTESIAN_POINT('Ctrl Pts',(-14.6952385361706,-17.1916259308415,
0.));
#230479=CARTESIAN_POINT('Ctrl Pts',(-14.699949811582,-17.1963476411694,
0.));
#230480=CARTESIAN_POINT('Ctrl Pts',(-14.7048748502663,-17.2012461084268,
0.));
#230481=CARTESIAN_POINT('Ctrl Pts',(-14.7100107213586,-17.2063157097315,
0.));
#230482=CARTESIAN_POINT('Ctrl Pts',(-14.7153546289339,-17.2115510835989,
0.));
#230483=CARTESIAN_POINT('Ctrl Pts',(-14.7209039390327,-17.2169471814256,
0.));
#230484=CARTESIAN_POINT('Ctrl Pts',(-14.7266561494282,-17.2224992099666,
0.));
#230485=CARTESIAN_POINT('Ctrl Pts',(-14.7326088681163,-17.2282025904314,
0.));
#230486=CARTESIAN_POINT('Ctrl Pts',(-14.7387597858117,-17.2340529062076,
0.));
#230487=CARTESIAN_POINT('Ctrl Pts',(-14.7451066593792,-17.2400458713565,
0.));
#230488=CARTESIAN_POINT('Ctrl Pts',(-14.7516473175124,-17.2461773413288,
0.));
#230489=CARTESIAN_POINT('Ctrl Pts',(-14.7583796616617,-17.2524433146837,
0.));
#230490=CARTESIAN_POINT('Ctrl Pts',(-14.7653016697591,-17.2588399401465,
0.));
#230491=CARTESIAN_POINT('Ctrl Pts',(-14.7724113956731,-17.2653635155319,
0.));
#230492=CARTESIAN_POINT('Ctrl Pts',(-14.7797069617804,-17.2720104735194,
0.));
#230493=CARTESIAN_POINT('Ctrl Pts',(-14.787186553128,-17.2787773704849,
0.));
#230494=CARTESIAN_POINT('Ctrl Pts',(-14.7948484105249,-17.2856608733196,
0.));
#230495=CARTESIAN_POINT('Ctrl Pts',(-14.8026908254276,-17.2926577496513,
0.));
#230496=CARTESIAN_POINT('Ctrl Pts',(-14.8107121391036,-17.299764866148,
0.));
#230497=CARTESIAN_POINT('Ctrl Pts',(-14.8189107410162,-17.3069791853706,
0.));
#230498=CARTESIAN_POINT('Ctrl Pts',(-14.8272850675379,-17.3142977632659,
0.));
#230499=CARTESIAN_POINT('Ctrl Pts',(-14.8358336004197,-17.3217177462101,
0.));
#230500=CARTESIAN_POINT('Ctrl Pts',(-14.8445548643508,-17.3292363662605,
0.));
#230501=CARTESIAN_POINT('Ctrl Pts',(-14.8534474245434,-17.336850936485,
0.));
#230502=CARTESIAN_POINT('Ctrl Pts',(-14.8625098843417,-17.3445588463474,
0.));
#230503=CARTESIAN_POINT('Ctrl Pts',(-14.8717408826956,-17.3523575568645,
0.));
#230504=CARTESIAN_POINT('Ctrl Pts',(-14.8811390927423,-17.3602445978161,
0.));
#230505=CARTESIAN_POINT('Ctrl Pts',(-14.8907032205788,-17.3682175653235,
0.));
#230506=CARTESIAN_POINT('Ctrl Pts',(-14.900432003961,-17.3762741193076,
0.));
#230507=CARTESIAN_POINT('Ctrl Pts',(-14.9103242110058,-17.3844119809824,
0.));
#230508=CARTESIAN_POINT('Ctrl Pts',(-14.9203786389342,-17.3926289303986,
0.));
#230509=CARTESIAN_POINT('Ctrl Pts',(-14.9305941128757,-17.4009228040749,
0.));
#230510=CARTESIAN_POINT('Ctrl Pts',(-14.940969484645,-17.4092914926071,
0.));
#230511=CARTESIAN_POINT('Ctrl Pts',(-14.9515036315143,-17.4177329382828,
0.));
#230512=CARTESIAN_POINT('Ctrl Pts',(-14.9621954549827,-17.426245132709,
0.));
#230513=CARTESIAN_POINT('Ctrl Pts',(-14.9730438799452,-17.4348261151396,
0.));
#230514=CARTESIAN_POINT('Ctrl Pts',(-14.9840478538358,-17.4434739707773,
0.));
#230515=CARTESIAN_POINT('Ctrl Pts',(-14.9952063457778,-17.4521868291004,
0.));
#230516=CARTESIAN_POINT('Ctrl Pts',(-15.0065183456921,-17.4609628621418,
0.));
#230517=CARTESIAN_POINT('Ctrl Pts',(-15.0179828635086,-17.4698002829356,
0.));
#230518=CARTESIAN_POINT('Ctrl Pts',(-15.029598928488,-17.4786973441417,
0.));
#230519=CARTESIAN_POINT('Ctrl Pts',(-15.0413655884993,-17.4876523366178,
0.));
#230520=CARTESIAN_POINT('Ctrl Pts',(-15.0532819093085,-17.4966635880245,
0.));
#230521=CARTESIAN_POINT('Ctrl Pts',(-15.0653469738306,-17.5057294613874,
0.));
#230522=CARTESIAN_POINT('Ctrl Pts',(-15.0775598815748,-17.5148483539683,
0.));
#230523=CARTESIAN_POINT('Ctrl Pts',(-15.0899197481082,-17.5240186961788,
0.));
#230524=CARTESIAN_POINT('Ctrl Pts',(-15.1024257045033,-17.5332389504829,
0.));
#230525=CARTESIAN_POINT('Ctrl Pts',(-15.1150768967729,-17.5425076102966,
0.));
#230526=CARTESIAN_POINT('Ctrl Pts',(-15.127872485314,-17.5518231989122,
0.));
#230527=CARTESIAN_POINT('Ctrl Pts',(-15.1408116444877,-17.5611842686196,
0.));
#230528=CARTESIAN_POINT('Ctrl Pts',(-15.1538935621715,-17.570589399803,
0.));
#230529=CARTESIAN_POINT('Ctrl Pts',(-15.1671174393137,-17.5800372000539,
0.));
#230530=CARTESIAN_POINT('Ctrl Pts',(-15.1804824894605,-17.5895263032592,
0.));
#230531=CARTESIAN_POINT('Ctrl Pts',(-15.1939879383268,-17.5990553687595,
0.));
#230532=CARTESIAN_POINT('Ctrl Pts',(-15.2076330234686,-17.6086230806497,
0.));
#230533=CARTESIAN_POINT('Ctrl Pts',(-15.22141699392,-17.6182281470467,0.));
#230534=CARTESIAN_POINT('Ctrl Pts',(-15.2353391098367,-17.6278692993765,
0.));
#230535=CARTESIAN_POINT('Ctrl Pts',(-15.2493986421091,-17.637545291637,
0.));
#230536=CARTESIAN_POINT('Ctrl Pts',(-15.263594872029,-17.6472548997329,
0.));
#230537=CARTESIAN_POINT('Ctrl Pts',(-15.2779270910238,-17.6569969209,0.));
#230538=CARTESIAN_POINT('Ctrl Pts',(-15.2923946003598,-17.6667701731041,
0.));
#230539=CARTESIAN_POINT('Ctrl Pts',(-15.3069967108501,-17.6765734944559,
0.));
#230540=CARTESIAN_POINT('Ctrl Pts',(-15.3217327425341,-17.6864057426052,
0.));
#230541=CARTESIAN_POINT('Ctrl Pts',(-15.3366020244069,-17.6962657941984,
0.));
#230542=CARTESIAN_POINT('Ctrl Pts',(-15.3516038942064,-17.7061525444044,
0.));
#230543=CARTESIAN_POINT('Ctrl Pts',(-15.3667376981702,-17.7160649064208,
0.));
#230544=CARTESIAN_POINT('Ctrl Pts',(-15.3820027907965,-17.7260018109923,
0.));
#230545=CARTESIAN_POINT('Ctrl Pts',(-15.3973985345796,-17.7359622059143,
0.));
#230546=CARTESIAN_POINT('Ctrl Pts',(-15.4129242997828,-17.7459450555803,
0.));
#230547=CARTESIAN_POINT('Ctrl Pts',(-15.4285794642658,-17.7559493405871,
0.));
#230548=CARTESIAN_POINT('Ctrl Pts',(-15.4443634132865,-17.765974057326,
0.));
#230549=CARTESIAN_POINT('Ctrl Pts',(-15.460275539302,-17.7760182175817,
0.));
#230550=CARTESIAN_POINT('Ctrl Pts',(-15.4763152417506,-17.7860808481229,
0.));
#230551=CARTESIAN_POINT('Ctrl Pts',(-15.4924819268529,-17.7961609903161,
0.));
#230552=CARTESIAN_POINT('Ctrl Pts',(-15.5087750074728,-17.8062576997964,
0.));
#230553=CARTESIAN_POINT('Ctrl Pts',(-15.5251939029558,-17.8163700461262,
0.));
#230554=CARTESIAN_POINT('Ctrl Pts',(-15.5417380389639,-17.8264971124606,
0.));
#230555=CARTESIAN_POINT('Ctrl Pts',(-15.5584068472976,-17.8366379952078,
0.));
#230556=CARTESIAN_POINT('Ctrl Pts',(-15.5751997657154,-17.8467918036976,
0.));
#230557=CARTESIAN_POINT('Ctrl Pts',(-15.5921162378183,-17.8569576598996,
0.));
#230558=CARTESIAN_POINT('Ctrl Pts',(-15.6091557129205,-17.8671346981388,
0.));
#230559=CARTESIAN_POINT('Ctrl Pts',(-15.6263176459107,-17.8773220648125,
0.));
#230560=CARTESIAN_POINT('Ctrl Pts',(-15.6436014971088,-17.8875189181095,
0.));
#230561=CARTESIAN_POINT('Ctrl Pts',(-15.6610067321036,-17.8977244277247,
0.));
#230562=CARTESIAN_POINT('Ctrl Pts',(-15.6785328216467,-17.9079377746118,
0.));
#230563=CARTESIAN_POINT('Ctrl Pts',(-15.6961792415526,-17.918158150746,
0.));
#230564=CARTESIAN_POINT('Ctrl Pts',(-15.713945472584,-17.9283847588837,
0.));
#230565=CARTESIAN_POINT('Ctrl Pts',(-15.7318310003334,-17.9386168123261,
0.));
#230566=CARTESIAN_POINT('Ctrl Pts',(-15.7498353150856,-17.9488535346776,
0.));
#230567=CARTESIAN_POINT('Ctrl Pts',(-15.7679579117072,-17.9590941596236,
0.));
#230568=CARTESIAN_POINT('Ctrl Pts',(-15.786198289572,-17.9693379307297,
0.));
#230569=CARTESIAN_POINT('Ctrl Pts',(-15.8045559524674,-17.9795841012383,
0.));
#230570=CARTESIAN_POINT('Ctrl Pts',(-15.8230304084963,-17.9898319338664,
0.));
#230571=CARTESIAN_POINT('Ctrl Pts',(-15.8416211699682,-18.0000807006055,
0.));
#230572=CARTESIAN_POINT('Ctrl Pts',(-15.8603277532834,-18.010329682521,
0.));
#230573=CARTESIAN_POINT('Ctrl Pts',(-15.8791496788685,-18.0205781695773,
0.));
#230574=CARTESIAN_POINT('Ctrl Pts',(-15.8980864711043,-18.0308254604638,
0.));
#230575=CARTESIAN_POINT('Ctrl Pts',(-15.9171376582436,-18.0410708624208,
0.));
#230576=CARTESIAN_POINT('Ctrl Pts',(-15.9363027723244,-18.0513136910691,
0.));
#230577=CARTESIAN_POINT('Ctrl Pts',(-15.9555813490645,-18.061553270236,
0.));
#230578=CARTESIAN_POINT('Ctrl Pts',(-15.9749729277848,-18.071788931796,
0.));
#230579=CARTESIAN_POINT('Ctrl Pts',(-15.9944770513616,-18.0820200155238,
0.));
#230580=CARTESIAN_POINT('Ctrl Pts',(-16.0140932661612,-18.0922458689464,
0.));
#230581=CARTESIAN_POINT('Ctrl Pts',(-16.0338211219694,-18.1024658471966,
0.));
#230582=CARTESIAN_POINT('Ctrl Pts',(-16.0536601719124,-18.1126793128688,
0.));
#230583=CARTESIAN_POINT('Ctrl Pts',(-16.0736099723665,-18.1228856358746,
0.));
#230584=CARTESIAN_POINT('Ctrl Pts',(-16.0936700829108,-18.1330841933099,
0.));
#230585=CARTESIAN_POINT('Ctrl Pts',(-16.1138400662791,-18.1432743693231,
0.));
#230586=CARTESIAN_POINT('Ctrl Pts',(-16.1341194882987,-18.153455554985,
0.));
#230587=CARTESIAN_POINT('Ctrl Pts',(-16.1545079178261,-18.1636271481616,
0.));
#230588=CARTESIAN_POINT('Ctrl Pts',(-16.1750049266673,-18.1737885533852,
0.));
#230589=CARTESIAN_POINT('Ctrl Pts',(-16.1956100895076,-18.1839391817335,
0.));
#230590=CARTESIAN_POINT('Ctrl Pts',(-16.2163229838878,-18.1940784507232,
0.));
#230591=CARTESIAN_POINT('Ctrl Pts',(-16.237143190164,-18.2042057842037,
0.));
#230592=CARTESIAN_POINT('Ctrl Pts',(-16.2580702914615,-18.214320612253,
0.));
#230593=CARTESIAN_POINT('Ctrl Pts',(-16.2791038736223,-18.2244223710745,
0.));
#230594=CARTESIAN_POINT('Ctrl Pts',(-16.3002435251378,-18.2345105028981,
0.));
#230595=CARTESIAN_POINT('Ctrl Pts',(-16.3214888370988,-18.2445844558742,
0.));
#230596=CARTESIAN_POINT('Ctrl Pts',(-16.342839403159,-18.2546436839609,
0.));
#230597=CARTESIAN_POINT('Ctrl Pts',(-16.3642948194869,-18.2646876468169,
0.));
#230598=CARTESIAN_POINT('Ctrl Pts',(-16.385854684708,-18.2747158096934,
0.));
#230599=CARTESIAN_POINT('Ctrl Pts',(-16.4075185998454,-18.2847276433308,
0.));
#230600=CARTESIAN_POINT('Ctrl Pts',(-16.4292861682377,-18.2947226238509,
0.));
#230601=CARTESIAN_POINT('Ctrl Pts',(-16.4511569955231,-18.3047002326858,
0.));
#230602=CARTESIAN_POINT('Ctrl Pts',(-16.4731306896439,-18.3146599565229,
0.));
#230603=CARTESIAN_POINT('Ctrl Pts',(-16.4952068608344,-18.3246012872468,
0.));
#230604=CARTESIAN_POINT('Ctrl Pts',(-16.5173851216045,-18.3345237218864,
0.));
#230605=CARTESIAN_POINT('Ctrl Pts',(-16.539665086714,-18.3444267625601,
0.));
#230606=CARTESIAN_POINT('Ctrl Pts',(-16.5620463731414,-18.3543099164331,
0.));
#230607=CARTESIAN_POINT('Ctrl Pts',(-16.5845286000219,-18.364172695589,
0.));
#230608=CARTESIAN_POINT('Ctrl Pts',(-16.6071113885711,-18.3740146168879,
0.));
#230609=CARTESIAN_POINT('Ctrl Pts',(-16.6297943620056,-18.3838352018327,
0.));
#230610=CARTESIAN_POINT('Ctrl Pts',(-16.6525771454513,-18.3936339764332,
0.));
#230611=CARTESIAN_POINT('Ctrl Pts',(-16.6754593658513,-18.4034104710789,
0.));
#230612=CARTESIAN_POINT('Ctrl Pts',(-16.698440651849,-18.4131642203989,
0.));
#230613=CARTESIAN_POINT('Ctrl Pts',(-16.7215206338818,-18.4228947633186,
0.));
#230614=CARTESIAN_POINT('Ctrl Pts',(-16.7446989442882,-18.4326016431392,
0.));
#230615=CARTESIAN_POINT('Ctrl Pts',(-16.7679752173992,-18.4422844076099,
0.));
#230616=CARTESIAN_POINT('Ctrl Pts',(-16.791349089629,-18.4519426090124,
0.));
#230617=CARTESIAN_POINT('Ctrl Pts',(-16.8148201995472,-18.4615758042305,
0.));
#230618=CARTESIAN_POINT('Ctrl Pts',(-16.8383881879707,-18.4711835548622,
0.));
#230619=CARTESIAN_POINT('Ctrl Pts',(-16.8620526977169,-18.4807654268769,
0.));
#230620=CARTESIAN_POINT('Ctrl Pts',(-16.8858133733086,-18.4903209902226,
0.));
#230621=CARTESIAN_POINT('Ctrl Pts',(-16.9096698606942,-18.4998498184619,
0.));
#230622=CARTESIAN_POINT('Ctrl Pts',(-16.9336218069353,-18.5093514883835,
0.));
#230623=CARTESIAN_POINT('Ctrl Pts',(-16.957668859934,-18.518825579666,0.));
#230624=CARTESIAN_POINT('Ctrl Pts',(-16.9818106680382,-18.5282716744198,
0.));
#230625=CARTESIAN_POINT('Ctrl Pts',(-17.0060468805099,-18.5376893576961,
0.));
#230626=CARTESIAN_POINT('Ctrl Pts',(-17.030377148174,-18.5470782182089,
0.));
#230627=CARTESIAN_POINT('Ctrl Pts',(-17.0548011239751,-18.5564378489628,
0.));
#230628=CARTESIAN_POINT('Ctrl Pts',(-17.0793184636079,-18.5657678479788,
0.));
#230629=CARTESIAN_POINT('Ctrl Pts',(-17.1039288260002,-18.5750678188543,
0.));
#230630=CARTESIAN_POINT('Ctrl Pts',(-17.1286318741185,-18.5843373717253,
0.));
#230631=CARTESIAN_POINT('Ctrl Pts',(-17.1534272741646,-18.5935761222833,
0.));
#230632=CARTESIAN_POINT('Ctrl Pts',(-17.1783146940131,-18.6027836898826,
0.));
#230633=CARTESIAN_POINT('Ctrl Pts',(-17.2032938019288,-18.6119596959957,
0.));
#230634=CARTESIAN_POINT('Ctrl Pts',(-17.2283642650519,-18.6211037624041,
0.));
#230635=CARTESIAN_POINT('Ctrl Pts',(-17.2535257482186,-18.630215509794,
0.));
#230636=CARTESIAN_POINT('Ctrl Pts',(-17.278777912021,-18.639294555474,0.));
#230637=CARTESIAN_POINT('Ctrl Pts',(-17.3041204135069,-18.6483405141853,
0.));
#230638=CARTESIAN_POINT('Ctrl Pts',(-17.3295529098612,-18.6573530024019,
0.));
#230639=CARTESIAN_POINT('Ctrl Pts',(-17.3550750612438,-18.6663316416569,
0.));
#230640=CARTESIAN_POINT('Ctrl Pts',(-17.3806865340744,-18.6752760624045,
0.));
#230641=CARTESIAN_POINT('Ctrl Pts',(-17.4063870038563,-18.6841859073472,
0.));
#230642=CARTESIAN_POINT('Ctrl Pts',(-17.4321761588148,-18.6930608357421,
0.));
#230643=CARTESIAN_POINT('Ctrl Pts',(-17.4580537012764,-18.7019005250322,
0.));
#230644=CARTESIAN_POINT('Ctrl Pts',(-17.4840193397176,-18.7107046613941,
0.));
#230645=CARTESIAN_POINT('Ctrl Pts',(-17.5100727820891,-18.7194729318127,
0.));
#230646=CARTESIAN_POINT('Ctrl Pts',(-17.5362137287604,-18.728205015716,
0.));
#230647=CARTESIAN_POINT('Ctrl Pts',(-17.5624418653248,-18.7369005764558,
0.));
#230648=CARTESIAN_POINT('Ctrl Pts',(-17.5887568561361,-18.7455592536667,
0.));
#230649=CARTESIAN_POINT('Ctrl Pts',(-17.6151583356989,-18.7541806530935,
0.));
#230650=CARTESIAN_POINT('Ctrl Pts',(-17.6416459210646,-18.7627643613138,
0.));
#230651=CARTESIAN_POINT('Ctrl Pts',(-17.6682192274197,-18.7713099642673,
0.));
#230652=CARTESIAN_POINT('Ctrl Pts',(-17.6948778822982,-18.7798170641305,
0.));
#230653=CARTESIAN_POINT('Ctrl Pts',(-17.7216215409019,-18.7882852976016,
0.));
#230654=CARTESIAN_POINT('Ctrl Pts',(-17.7484498996917,-18.7967143519444,
0.));
#230655=CARTESIAN_POINT('Ctrl Pts',(-17.7753627137898,-18.8051039860543,
0.));
#230656=CARTESIAN_POINT('Ctrl Pts',(-17.8023598011135,-18.8134540340581,
0.));
#230657=CARTESIAN_POINT('Ctrl Pts',(-17.8294410311105,-18.8217643886368,
0.));
#230658=CARTESIAN_POINT('Ctrl Pts',(-17.8566063174871,-18.8300349896187,
0.));
#230659=CARTESIAN_POINT('Ctrl Pts',(-17.8784057509434,-18.8366196462746,
0.));
#230660=CARTESIAN_POINT('Ctrl Pts',(-17.8947931177853,-18.8415402351882,
0.));
#230661=CARTESIAN_POINT('Ctrl Pts',(-17.9057348246611,-18.8448126709726,
0.));
#230662=CARTESIAN_POINT('Ctrl Pts',(-17.9112098770111,-18.8464468996588,
0.));
#230663=CARTESIAN_POINT('',(-17.9112098770111,-18.8464468996588,12.));
#230664=CARTESIAN_POINT('Ctrl Pts',(-17.9112098770111,-18.8464468996588,
12.));
#230665=CARTESIAN_POINT('Ctrl Pts',(-17.9057348246611,-18.8448126709726,
12.));
#230666=CARTESIAN_POINT('Ctrl Pts',(-17.8947931177853,-18.8415402351882,
12.));
#230667=CARTESIAN_POINT('Ctrl Pts',(-17.8784057509434,-18.8366196462746,
12.));
#230668=CARTESIAN_POINT('Ctrl Pts',(-17.8566063174871,-18.8300349896187,
12.));
#230669=CARTESIAN_POINT('Ctrl Pts',(-17.8294410311105,-18.8217643886368,
12.));
#230670=CARTESIAN_POINT('Ctrl Pts',(-17.8023598011135,-18.8134540340581,
12.));
#230671=CARTESIAN_POINT('Ctrl Pts',(-17.7753627137898,-18.8051039860543,
12.));
#230672=CARTESIAN_POINT('Ctrl Pts',(-17.7484498996917,-18.7967143519444,
12.));
#230673=CARTESIAN_POINT('Ctrl Pts',(-17.7216215409019,-18.7882852976016,
12.));
#230674=CARTESIAN_POINT('Ctrl Pts',(-17.6948778822982,-18.7798170641305,
12.));
#230675=CARTESIAN_POINT('Ctrl Pts',(-17.6682192274197,-18.7713099642673,
12.));
#230676=CARTESIAN_POINT('Ctrl Pts',(-17.6416459210646,-18.7627643613138,
12.));
#230677=CARTESIAN_POINT('Ctrl Pts',(-17.6151583356989,-18.7541806530935,
12.));
#230678=CARTESIAN_POINT('Ctrl Pts',(-17.5887568561361,-18.7455592536667,
12.));
#230679=CARTESIAN_POINT('Ctrl Pts',(-17.5624418653248,-18.7369005764558,
12.));
#230680=CARTESIAN_POINT('Ctrl Pts',(-17.5362137287604,-18.728205015716,
12.));
#230681=CARTESIAN_POINT('Ctrl Pts',(-17.5100727820891,-18.7194729318127,
12.));
#230682=CARTESIAN_POINT('Ctrl Pts',(-17.4840193397176,-18.7107046613941,
12.));
#230683=CARTESIAN_POINT('Ctrl Pts',(-17.4580537012764,-18.7019005250322,
12.));
#230684=CARTESIAN_POINT('Ctrl Pts',(-17.4321761588148,-18.6930608357421,
12.));
#230685=CARTESIAN_POINT('Ctrl Pts',(-17.4063870038563,-18.6841859073472,
12.));
#230686=CARTESIAN_POINT('Ctrl Pts',(-17.3806865340744,-18.6752760624045,
12.));
#230687=CARTESIAN_POINT('Ctrl Pts',(-17.3550750612438,-18.6663316416569,
12.));
#230688=CARTESIAN_POINT('Ctrl Pts',(-17.3295529098612,-18.6573530024019,
12.));
#230689=CARTESIAN_POINT('Ctrl Pts',(-17.3041204135069,-18.6483405141853,
12.));
#230690=CARTESIAN_POINT('Ctrl Pts',(-17.278777912021,-18.639294555474,12.));
#230691=CARTESIAN_POINT('Ctrl Pts',(-17.2535257482186,-18.630215509794,
12.));
#230692=CARTESIAN_POINT('Ctrl Pts',(-17.2283642650519,-18.6211037624041,
12.));
#230693=CARTESIAN_POINT('Ctrl Pts',(-17.2032938019288,-18.6119596959957,
12.));
#230694=CARTESIAN_POINT('Ctrl Pts',(-17.1783146940131,-18.6027836898826,
12.));
#230695=CARTESIAN_POINT('Ctrl Pts',(-17.1534272741646,-18.5935761222833,
12.));
#230696=CARTESIAN_POINT('Ctrl Pts',(-17.1286318741185,-18.5843373717253,
12.));
#230697=CARTESIAN_POINT('Ctrl Pts',(-17.1039288260002,-18.5750678188543,
12.));
#230698=CARTESIAN_POINT('Ctrl Pts',(-17.0793184636079,-18.5657678479788,
12.));
#230699=CARTESIAN_POINT('Ctrl Pts',(-17.0548011239751,-18.5564378489628,
12.));
#230700=CARTESIAN_POINT('Ctrl Pts',(-17.030377148174,-18.5470782182089,
12.));
#230701=CARTESIAN_POINT('Ctrl Pts',(-17.0060468805099,-18.5376893576961,
12.));
#230702=CARTESIAN_POINT('Ctrl Pts',(-16.9818106680382,-18.5282716744198,
12.));
#230703=CARTESIAN_POINT('Ctrl Pts',(-16.957668859934,-18.518825579666,12.));
#230704=CARTESIAN_POINT('Ctrl Pts',(-16.9336218069353,-18.5093514883835,
12.));
#230705=CARTESIAN_POINT('Ctrl Pts',(-16.9096698606942,-18.4998498184619,
12.));
#230706=CARTESIAN_POINT('Ctrl Pts',(-16.8858133733086,-18.4903209902226,
12.));
#230707=CARTESIAN_POINT('Ctrl Pts',(-16.8620526977169,-18.4807654268769,
12.));
#230708=CARTESIAN_POINT('Ctrl Pts',(-16.8383881879707,-18.4711835548622,
12.));
#230709=CARTESIAN_POINT('Ctrl Pts',(-16.8148201995472,-18.4615758042305,
12.));
#230710=CARTESIAN_POINT('Ctrl Pts',(-16.791349089629,-18.4519426090124,
12.));
#230711=CARTESIAN_POINT('Ctrl Pts',(-16.7679752173992,-18.4422844076099,
12.));
#230712=CARTESIAN_POINT('Ctrl Pts',(-16.7446989442882,-18.4326016431392,
12.));
#230713=CARTESIAN_POINT('Ctrl Pts',(-16.7215206338818,-18.4228947633186,
12.));
#230714=CARTESIAN_POINT('Ctrl Pts',(-16.698440651849,-18.4131642203989,
12.));
#230715=CARTESIAN_POINT('Ctrl Pts',(-16.6754593658513,-18.4034104710789,
12.));
#230716=CARTESIAN_POINT('Ctrl Pts',(-16.6525771454513,-18.3936339764332,
12.));
#230717=CARTESIAN_POINT('Ctrl Pts',(-16.6297943620056,-18.3838352018327,
12.));
#230718=CARTESIAN_POINT('Ctrl Pts',(-16.6071113885711,-18.3740146168879,
12.));
#230719=CARTESIAN_POINT('Ctrl Pts',(-16.5845286000219,-18.364172695589,
12.));
#230720=CARTESIAN_POINT('Ctrl Pts',(-16.5620463731414,-18.3543099164331,
12.));
#230721=CARTESIAN_POINT('Ctrl Pts',(-16.539665086714,-18.3444267625601,
12.));
#230722=CARTESIAN_POINT('Ctrl Pts',(-16.5173851216045,-18.3345237218864,
12.));
#230723=CARTESIAN_POINT('Ctrl Pts',(-16.4952068608344,-18.3246012872468,
12.));
#230724=CARTESIAN_POINT('Ctrl Pts',(-16.4731306896439,-18.3146599565229,
12.));
#230725=CARTESIAN_POINT('Ctrl Pts',(-16.4511569955231,-18.3047002326858,
12.));
#230726=CARTESIAN_POINT('Ctrl Pts',(-16.4292861682377,-18.2947226238509,
12.));
#230727=CARTESIAN_POINT('Ctrl Pts',(-16.4075185998454,-18.2847276433308,
12.));
#230728=CARTESIAN_POINT('Ctrl Pts',(-16.385854684708,-18.2747158096934,
12.));
#230729=CARTESIAN_POINT('Ctrl Pts',(-16.3642948194869,-18.2646876468169,
12.));
#230730=CARTESIAN_POINT('Ctrl Pts',(-16.342839403159,-18.2546436839609,
12.));
#230731=CARTESIAN_POINT('Ctrl Pts',(-16.3214888370988,-18.2445844558742,
12.));
#230732=CARTESIAN_POINT('Ctrl Pts',(-16.3002435251378,-18.2345105028981,
12.));
#230733=CARTESIAN_POINT('Ctrl Pts',(-16.2791038736223,-18.2244223710745,
12.));
#230734=CARTESIAN_POINT('Ctrl Pts',(-16.2580702914615,-18.214320612253,
12.));
#230735=CARTESIAN_POINT('Ctrl Pts',(-16.237143190164,-18.2042057842037,
12.));
#230736=CARTESIAN_POINT('Ctrl Pts',(-16.2163229838878,-18.1940784507232,
12.));
#230737=CARTESIAN_POINT('Ctrl Pts',(-16.1956100895076,-18.1839391817335,
12.));
#230738=CARTESIAN_POINT('Ctrl Pts',(-16.1750049266673,-18.1737885533852,
12.));
#230739=CARTESIAN_POINT('Ctrl Pts',(-16.1545079178261,-18.1636271481616,
12.));
#230740=CARTESIAN_POINT('Ctrl Pts',(-16.1341194882987,-18.153455554985,
12.));
#230741=CARTESIAN_POINT('Ctrl Pts',(-16.1138400662791,-18.1432743693231,
12.));
#230742=CARTESIAN_POINT('Ctrl Pts',(-16.0936700829108,-18.1330841933099,
12.));
#230743=CARTESIAN_POINT('Ctrl Pts',(-16.0736099723665,-18.1228856358746,
12.));
#230744=CARTESIAN_POINT('Ctrl Pts',(-16.0536601719124,-18.1126793128688,
12.));
#230745=CARTESIAN_POINT('Ctrl Pts',(-16.0338211219694,-18.1024658471966,
12.));
#230746=CARTESIAN_POINT('Ctrl Pts',(-16.0140932661612,-18.0922458689464,
12.));
#230747=CARTESIAN_POINT('Ctrl Pts',(-15.9944770513616,-18.0820200155238,
12.));
#230748=CARTESIAN_POINT('Ctrl Pts',(-15.9749729277848,-18.071788931796,
12.));
#230749=CARTESIAN_POINT('Ctrl Pts',(-15.9555813490645,-18.061553270236,
12.));
#230750=CARTESIAN_POINT('Ctrl Pts',(-15.9363027723244,-18.0513136910691,
12.));
#230751=CARTESIAN_POINT('Ctrl Pts',(-15.9171376582436,-18.0410708624208,
12.));
#230752=CARTESIAN_POINT('Ctrl Pts',(-15.8980864711043,-18.0308254604638,
12.));
#230753=CARTESIAN_POINT('Ctrl Pts',(-15.8791496788685,-18.0205781695773,
12.));
#230754=CARTESIAN_POINT('Ctrl Pts',(-15.8603277532834,-18.010329682521,
12.));
#230755=CARTESIAN_POINT('Ctrl Pts',(-15.8416211699682,-18.0000807006055,
12.));
#230756=CARTESIAN_POINT('Ctrl Pts',(-15.8230304084963,-17.9898319338664,
12.));
#230757=CARTESIAN_POINT('Ctrl Pts',(-15.8045559524674,-17.9795841012383,
12.));
#230758=CARTESIAN_POINT('Ctrl Pts',(-15.786198289572,-17.9693379307297,
12.));
#230759=CARTESIAN_POINT('Ctrl Pts',(-15.7679579117072,-17.9590941596236,
12.));
#230760=CARTESIAN_POINT('Ctrl Pts',(-15.7498353150856,-17.9488535346776,
12.));
#230761=CARTESIAN_POINT('Ctrl Pts',(-15.7318310003334,-17.9386168123261,
12.));
#230762=CARTESIAN_POINT('Ctrl Pts',(-15.713945472584,-17.9283847588837,
12.));
#230763=CARTESIAN_POINT('Ctrl Pts',(-15.6961792415526,-17.918158150746,
12.));
#230764=CARTESIAN_POINT('Ctrl Pts',(-15.6785328216467,-17.9079377746118,
12.));
#230765=CARTESIAN_POINT('Ctrl Pts',(-15.6610067321036,-17.8977244277247,
12.));
#230766=CARTESIAN_POINT('Ctrl Pts',(-15.6436014971088,-17.8875189181095,
12.));
#230767=CARTESIAN_POINT('Ctrl Pts',(-15.6263176459107,-17.8773220648125,
12.));
#230768=CARTESIAN_POINT('Ctrl Pts',(-15.6091557129205,-17.8671346981388,
12.));
#230769=CARTESIAN_POINT('Ctrl Pts',(-15.5921162378183,-17.8569576598996,
12.));
#230770=CARTESIAN_POINT('Ctrl Pts',(-15.5751997657154,-17.8467918036976,
12.));
#230771=CARTESIAN_POINT('Ctrl Pts',(-15.5584068472976,-17.8366379952078,
12.));
#230772=CARTESIAN_POINT('Ctrl Pts',(-15.5417380389639,-17.8264971124606,
12.));
#230773=CARTESIAN_POINT('Ctrl Pts',(-15.5251939029558,-17.8163700461262,
12.));
#230774=CARTESIAN_POINT('Ctrl Pts',(-15.5087750074728,-17.8062576997964,
12.));
#230775=CARTESIAN_POINT('Ctrl Pts',(-15.4924819268529,-17.7961609903161,
12.));
#230776=CARTESIAN_POINT('Ctrl Pts',(-15.4763152417506,-17.7860808481229,
12.));
#230777=CARTESIAN_POINT('Ctrl Pts',(-15.460275539302,-17.7760182175817,
12.));
#230778=CARTESIAN_POINT('Ctrl Pts',(-15.4443634132865,-17.765974057326,
12.));
#230779=CARTESIAN_POINT('Ctrl Pts',(-15.4285794642658,-17.7559493405871,
12.));
#230780=CARTESIAN_POINT('Ctrl Pts',(-15.4129242997828,-17.7459450555803,
12.));
#230781=CARTESIAN_POINT('Ctrl Pts',(-15.3973985345796,-17.7359622059143,
12.));
#230782=CARTESIAN_POINT('Ctrl Pts',(-15.3820027907965,-17.7260018109923,
12.));
#230783=CARTESIAN_POINT('Ctrl Pts',(-15.3667376981702,-17.7160649064208,
12.));
#230784=CARTESIAN_POINT('Ctrl Pts',(-15.3516038942064,-17.7061525444044,
12.));
#230785=CARTESIAN_POINT('Ctrl Pts',(-15.3366020244069,-17.6962657941984,
12.));
#230786=CARTESIAN_POINT('Ctrl Pts',(-15.3217327425341,-17.6864057426052,
12.));
#230787=CARTESIAN_POINT('Ctrl Pts',(-15.3069967108501,-17.6765734944559,
12.));
#230788=CARTESIAN_POINT('Ctrl Pts',(-15.2923946003598,-17.6667701731041,
12.));
#230789=CARTESIAN_POINT('Ctrl Pts',(-15.2779270910238,-17.6569969209,12.));
#230790=CARTESIAN_POINT('Ctrl Pts',(-15.263594872029,-17.6472548997329,
12.));
#230791=CARTESIAN_POINT('Ctrl Pts',(-15.2493986421091,-17.637545291637,
12.));
#230792=CARTESIAN_POINT('Ctrl Pts',(-15.2353391098367,-17.6278692993765,
12.));
#230793=CARTESIAN_POINT('Ctrl Pts',(-15.22141699392,-17.6182281470467,12.));
#230794=CARTESIAN_POINT('Ctrl Pts',(-15.2076330234686,-17.6086230806497,
12.));
#230795=CARTESIAN_POINT('Ctrl Pts',(-15.1939879383268,-17.5990553687595,
12.));
#230796=CARTESIAN_POINT('Ctrl Pts',(-15.1804824894605,-17.5895263032592,
12.));
#230797=CARTESIAN_POINT('Ctrl Pts',(-15.1671174393137,-17.5800372000539,
12.));
#230798=CARTESIAN_POINT('Ctrl Pts',(-15.1538935621715,-17.570589399803,
12.));
#230799=CARTESIAN_POINT('Ctrl Pts',(-15.1408116444877,-17.5611842686196,
12.));
#230800=CARTESIAN_POINT('Ctrl Pts',(-15.127872485314,-17.5518231989122,
12.));
#230801=CARTESIAN_POINT('Ctrl Pts',(-15.1150768967729,-17.5425076102966,
12.));
#230802=CARTESIAN_POINT('Ctrl Pts',(-15.1024257045033,-17.5332389504829,
12.));
#230803=CARTESIAN_POINT('Ctrl Pts',(-15.0899197481082,-17.5240186961788,
12.));
#230804=CARTESIAN_POINT('Ctrl Pts',(-15.0775598815748,-17.5148483539683,
12.));
#230805=CARTESIAN_POINT('Ctrl Pts',(-15.0653469738306,-17.5057294613874,
12.));
#230806=CARTESIAN_POINT('Ctrl Pts',(-15.0532819093085,-17.4966635880245,
12.));
#230807=CARTESIAN_POINT('Ctrl Pts',(-15.0413655884993,-17.4876523366178,
12.));
#230808=CARTESIAN_POINT('Ctrl Pts',(-15.029598928488,-17.4786973441417,
12.));
#230809=CARTESIAN_POINT('Ctrl Pts',(-15.0179828635086,-17.4698002829356,
12.));
#230810=CARTESIAN_POINT('Ctrl Pts',(-15.0065183456921,-17.4609628621418,
12.));
#230811=CARTESIAN_POINT('Ctrl Pts',(-14.9952063457778,-17.4521868291004,
12.));
#230812=CARTESIAN_POINT('Ctrl Pts',(-14.9840478538358,-17.4434739707773,
12.));
#230813=CARTESIAN_POINT('Ctrl Pts',(-14.9730438799452,-17.4348261151396,
12.));
#230814=CARTESIAN_POINT('Ctrl Pts',(-14.9621954549827,-17.426245132709,
12.));
#230815=CARTESIAN_POINT('Ctrl Pts',(-14.9515036315143,-17.4177329382828,
12.));
#230816=CARTESIAN_POINT('Ctrl Pts',(-14.940969484645,-17.4092914926071,
12.));
#230817=CARTESIAN_POINT('Ctrl Pts',(-14.9305941128757,-17.4009228040749,
12.));
#230818=CARTESIAN_POINT('Ctrl Pts',(-14.9203786389342,-17.3926289303986,
12.));
#230819=CARTESIAN_POINT('Ctrl Pts',(-14.9103242110058,-17.3844119809824,
12.));
#230820=CARTESIAN_POINT('Ctrl Pts',(-14.900432003961,-17.3762741193076,
12.));
#230821=CARTESIAN_POINT('Ctrl Pts',(-14.8907032205788,-17.3682175653235,
12.));
#230822=CARTESIAN_POINT('Ctrl Pts',(-14.8811390927423,-17.3602445978161,
12.));
#230823=CARTESIAN_POINT('Ctrl Pts',(-14.8717408826956,-17.3523575568645,
12.));
#230824=CARTESIAN_POINT('Ctrl Pts',(-14.8625098843417,-17.3445588463474,
12.));
#230825=CARTESIAN_POINT('Ctrl Pts',(-14.8534474245434,-17.336850936485,
12.));
#230826=CARTESIAN_POINT('Ctrl Pts',(-14.8445548643508,-17.3292363662605,
12.));
#230827=CARTESIAN_POINT('Ctrl Pts',(-14.8358336004197,-17.3217177462101,
12.));
#230828=CARTESIAN_POINT('Ctrl Pts',(-14.8272850675379,-17.3142977632659,
12.));
#230829=CARTESIAN_POINT('Ctrl Pts',(-14.8189107410162,-17.3069791853706,
12.));
#230830=CARTESIAN_POINT('Ctrl Pts',(-14.8107121391036,-17.299764866148,
12.));
#230831=CARTESIAN_POINT('Ctrl Pts',(-14.8026908254276,-17.2926577496513,
12.));
#230832=CARTESIAN_POINT('Ctrl Pts',(-14.7948484105249,-17.2856608733196,
12.));
#230833=CARTESIAN_POINT('Ctrl Pts',(-14.787186553128,-17.2787773704849,
12.));
#230834=CARTESIAN_POINT('Ctrl Pts',(-14.7797069617804,-17.2720104735194,
12.));
#230835=CARTESIAN_POINT('Ctrl Pts',(-14.7724113956731,-17.2653635155319,
12.));
#230836=CARTESIAN_POINT('Ctrl Pts',(-14.7653016697591,-17.2588399401465,
12.));
#230837=CARTESIAN_POINT('Ctrl Pts',(-14.7583796616617,-17.2524433146837,
12.));
#230838=CARTESIAN_POINT('Ctrl Pts',(-14.7516473175124,-17.2461773413288,
12.));
#230839=CARTESIAN_POINT('Ctrl Pts',(-14.7451066593792,-17.2400458713565,
12.));
#230840=CARTESIAN_POINT('Ctrl Pts',(-14.7387597858117,-17.2340529062076,
12.));
#230841=CARTESIAN_POINT('Ctrl Pts',(-14.7326088681163,-17.2282025904314,
12.));
#230842=CARTESIAN_POINT('Ctrl Pts',(-14.7266561494282,-17.2224992099666,
12.));
#230843=CARTESIAN_POINT('Ctrl Pts',(-14.7209039390327,-17.2169471814256,
12.));
#230844=CARTESIAN_POINT('Ctrl Pts',(-14.7153546289339,-17.2115510835989,
12.));
#230845=CARTESIAN_POINT('Ctrl Pts',(-14.7100107213586,-17.2063157097315,
12.));
#230846=CARTESIAN_POINT('Ctrl Pts',(-14.7048748502663,-17.2012461084268,
12.));
#230847=CARTESIAN_POINT('Ctrl Pts',(-14.699949811582,-17.1963476411694,
12.));
#230848=CARTESIAN_POINT('Ctrl Pts',(-14.6952385361706,-17.1916259308415,
12.));
#230849=CARTESIAN_POINT('Ctrl Pts',(-14.6907440526958,-17.1870867909918,
12.));
#230850=CARTESIAN_POINT('Ctrl Pts',(-14.686469452232,-17.1827361584719,
12.));
#230851=CARTESIAN_POINT('Ctrl Pts',(-14.6824178576167,-17.1785800350826,
12.));
#230852=CARTESIAN_POINT('Ctrl Pts',(-14.6785925615677,-17.1746247499056,
12.));
#230853=CARTESIAN_POINT('Ctrl Pts',(-14.6749971333867,-17.1708771619129,
12.));
#230854=CARTESIAN_POINT('Ctrl Pts',(-14.671635583332,-17.167344972302,12.));
#230855=CARTESIAN_POINT('Ctrl Pts',(-14.6685123374423,-17.1640366762305,
12.));
#230856=CARTESIAN_POINT('Ctrl Pts',(-14.6656319165057,-17.1609609517369,
12.));
#230857=CARTESIAN_POINT('Ctrl Pts',(-14.6629987285992,-17.1581262646789,
12.));
#230858=CARTESIAN_POINT('Ctrl Pts',(-14.6606167169642,-17.1555401986401,
12.));
#230859=CARTESIAN_POINT('Ctrl Pts',(-14.6584900555302,-17.1532107762718,
12.));
#230860=CARTESIAN_POINT('Ctrl Pts',(-14.6566237952435,-17.1511476869496,
12.));
#230861=CARTESIAN_POINT('Ctrl Pts',(-14.655024862281,-17.1493641837558,
12.));
#230862=CARTESIAN_POINT('Ctrl Pts',(-14.6537016966184,-17.147876394491,
12.));
#230863=CARTESIAN_POINT('Ctrl Pts',(-14.6526624064978,-17.1466998098673,
12.));
#230864=CARTESIAN_POINT('Ctrl Pts',(-14.6519131634508,-17.1458462295271,
12.));
#230865=CARTESIAN_POINT('Ctrl Pts',(-14.6515481598068,-17.1454262858043,
12.));
#230866=CARTESIAN_POINT('Ctrl Pts',(-14.6514066997196,-17.1452600887037,
12.));
#230867=CARTESIAN_POINT('Ctrl Pts',(-14.6513711852843,-17.1452153999142,
12.));
#230868=CARTESIAN_POINT('Ctrl Pts',(-14.6513681262571,-17.1452095830632,
12.));
#230869=CARTESIAN_POINT('',(-17.9112098770111,-18.8464468996588,0.));
#230870=CARTESIAN_POINT('Origin',(-17.7219872369693,-12.1729687575668,0.));
#230871=CARTESIAN_POINT('',(-18.5896416359912,-12.7689476255363,12.));
#230872=CARTESIAN_POINT('',(-8.86099361848466,-6.08648437878338,12.));
#230873=CARTESIAN_POINT('',(-18.5896416359912,-12.7689476255363,0.));
#230874=CARTESIAN_POINT('',(-18.5896416359912,-12.7689476255363,0.));
#230875=CARTESIAN_POINT('',(-8.86099361848466,-6.08648437878338,0.));
#230876=CARTESIAN_POINT('Ctrl Pts',(-18.8464468996588,-17.9112098770111,
0.));
#230877=CARTESIAN_POINT('Ctrl Pts',(-18.8464468996588,-17.9112098770111,
12.));
#230878=CARTESIAN_POINT('Ctrl Pts',(-18.8448126709692,-17.9057348246595,
0.));
#230879=CARTESIAN_POINT('Ctrl Pts',(-18.8448126709692,-17.9057348246595,
12.));
#230880=CARTESIAN_POINT('Ctrl Pts',(-18.8415402351786,-17.8947931177807,
0.));
#230881=CARTESIAN_POINT('Ctrl Pts',(-18.8415402351786,-17.8947931177807,
12.));
#230882=CARTESIAN_POINT('Ctrl Pts',(-18.8366196462581,-17.8784057509356,
0.));
#230883=CARTESIAN_POINT('Ctrl Pts',(-18.8366196462581,-17.8784057509356,
12.));
#230884=CARTESIAN_POINT('Ctrl Pts',(-18.8300349895974,-17.8566063174771,
0.));
#230885=CARTESIAN_POINT('Ctrl Pts',(-18.8300349895974,-17.8566063174771,
12.));
#230886=CARTESIAN_POINT('Ctrl Pts',(-18.8217643886157,-17.8294410311006,
0.));
#230887=CARTESIAN_POINT('Ctrl Pts',(-18.8217643886157,-17.8294410311006,
12.));
#230888=CARTESIAN_POINT('Ctrl Pts',(-18.8134540340417,-17.8023598011057,
0.));
#230889=CARTESIAN_POINT('Ctrl Pts',(-18.8134540340417,-17.8023598011057,
12.));
#230890=CARTESIAN_POINT('Ctrl Pts',(-18.8051039860448,-17.7753627137853,
0.));
#230891=CARTESIAN_POINT('Ctrl Pts',(-18.8051039860448,-17.7753627137853,
12.));
#230892=CARTESIAN_POINT('Ctrl Pts',(-18.7967143519419,-17.7484498996905,
0.));
#230893=CARTESIAN_POINT('Ctrl Pts',(-18.7967143519419,-17.7484498996905,
12.));
#230894=CARTESIAN_POINT('Ctrl Pts',(-18.788285297605,-17.7216215409035,
0.));
#230895=CARTESIAN_POINT('Ctrl Pts',(-18.788285297605,-17.7216215409035,
12.));
#230896=CARTESIAN_POINT('Ctrl Pts',(-18.7798170641374,-17.6948778823014,
0.));
#230897=CARTESIAN_POINT('Ctrl Pts',(-18.7798170641374,-17.6948778823014,
12.));
#230898=CARTESIAN_POINT('Ctrl Pts',(-18.7713099642754,-17.6682192274236,
0.));
#230899=CARTESIAN_POINT('Ctrl Pts',(-18.7713099642754,-17.6682192274236,
12.));
#230900=CARTESIAN_POINT('Ctrl Pts',(-18.762764361321,-17.6416459210681,
0.));
#230901=CARTESIAN_POINT('Ctrl Pts',(-18.762764361321,-17.6416459210681,
12.));
#230902=CARTESIAN_POINT('Ctrl Pts',(-18.7541806530984,-17.6151583357012,
0.));
#230903=CARTESIAN_POINT('Ctrl Pts',(-18.7541806530984,-17.6151583357012,
12.));
#230904=CARTESIAN_POINT('Ctrl Pts',(-18.7455592536687,-17.5887568561371,
0.));
#230905=CARTESIAN_POINT('Ctrl Pts',(-18.7455592536687,-17.5887568561371,
12.));
#230906=CARTESIAN_POINT('Ctrl Pts',(-18.7369005764553,-17.5624418653245,
0.));
#230907=CARTESIAN_POINT('Ctrl Pts',(-18.7369005764553,-17.5624418653245,
12.));
#230908=CARTESIAN_POINT('Ctrl Pts',(-18.7282050157138,-17.5362137287593,
0.));
#230909=CARTESIAN_POINT('Ctrl Pts',(-18.7282050157138,-17.5362137287593,
12.));
#230910=CARTESIAN_POINT('Ctrl Pts',(-18.7194729318098,-17.5100727820876,
0.));
#230911=CARTESIAN_POINT('Ctrl Pts',(-18.7194729318098,-17.5100727820876,
12.));
#230912=CARTESIAN_POINT('Ctrl Pts',(-18.7107046613912,-17.4840193397162,
0.));
#230913=CARTESIAN_POINT('Ctrl Pts',(-18.7107046613912,-17.4840193397162,
12.));
#230914=CARTESIAN_POINT('Ctrl Pts',(-18.70190052503,-17.4580537012753,0.));
#230915=CARTESIAN_POINT('Ctrl Pts',(-18.70190052503,-17.4580537012753,12.));
#230916=CARTESIAN_POINT('Ctrl Pts',(-18.6930608357409,-17.4321761588142,
0.));
#230917=CARTESIAN_POINT('Ctrl Pts',(-18.6930608357409,-17.4321761588142,
12.));
#230918=CARTESIAN_POINT('Ctrl Pts',(-18.6841859073471,-17.4063870038562,
0.));
#230919=CARTESIAN_POINT('Ctrl Pts',(-18.6841859073471,-17.4063870038562,
12.));
#230920=CARTESIAN_POINT('Ctrl Pts',(-18.6752760624052,-17.3806865340747,
0.));
#230921=CARTESIAN_POINT('Ctrl Pts',(-18.6752760624052,-17.3806865340747,
12.));
#230922=CARTESIAN_POINT('Ctrl Pts',(-18.6663316416582,-17.3550750612443,
0.));
#230923=CARTESIAN_POINT('Ctrl Pts',(-18.6663316416582,-17.3550750612443,
12.));
#230924=CARTESIAN_POINT('Ctrl Pts',(-18.6573530024033,-17.3295529098618,
0.));
#230925=CARTESIAN_POINT('Ctrl Pts',(-18.6573530024033,-17.3295529098618,
12.));
#230926=CARTESIAN_POINT('Ctrl Pts',(-18.6483405141865,-17.3041204135074,
0.));
#230927=CARTESIAN_POINT('Ctrl Pts',(-18.6483405141865,-17.3041204135074,
12.));
#230928=CARTESIAN_POINT('Ctrl Pts',(-18.6392945554748,-17.2787779120213,
0.));
#230929=CARTESIAN_POINT('Ctrl Pts',(-18.6392945554748,-17.2787779120213,
12.));
#230930=CARTESIAN_POINT('Ctrl Pts',(-18.6302155097943,-17.2535257482187,
0.));
#230931=CARTESIAN_POINT('Ctrl Pts',(-18.6302155097943,-17.2535257482187,
12.));
#230932=CARTESIAN_POINT('Ctrl Pts',(-18.6211037624038,-17.2283642650518,
0.));
#230933=CARTESIAN_POINT('Ctrl Pts',(-18.6211037624038,-17.2283642650518,
12.));
#230934=CARTESIAN_POINT('Ctrl Pts',(-18.6119596959949,-17.2032938019284,
0.));
#230935=CARTESIAN_POINT('Ctrl Pts',(-18.6119596959949,-17.2032938019284,
12.));
#230936=CARTESIAN_POINT('Ctrl Pts',(-18.6027836898817,-17.1783146940127,
0.));
#230937=CARTESIAN_POINT('Ctrl Pts',(-18.6027836898817,-17.1783146940127,
12.));
#230938=CARTESIAN_POINT('Ctrl Pts',(-18.5935761222825,-17.1534272741643,
0.));
#230939=CARTESIAN_POINT('Ctrl Pts',(-18.5935761222825,-17.1534272741643,
12.));
#230940=CARTESIAN_POINT('Ctrl Pts',(-18.5843373717247,-17.1286318741183,
0.));
#230941=CARTESIAN_POINT('Ctrl Pts',(-18.5843373717247,-17.1286318741183,
12.));
#230942=CARTESIAN_POINT('Ctrl Pts',(-18.5750678188542,-17.1039288260001,
0.));
#230943=CARTESIAN_POINT('Ctrl Pts',(-18.5750678188542,-17.1039288260001,
12.));
#230944=CARTESIAN_POINT('Ctrl Pts',(-18.5657678479789,-17.0793184636079,
0.));
#230945=CARTESIAN_POINT('Ctrl Pts',(-18.5657678479789,-17.0793184636079,
12.));
#230946=CARTESIAN_POINT('Ctrl Pts',(-18.556437848963,-17.0548011239751,
0.));
#230947=CARTESIAN_POINT('Ctrl Pts',(-18.556437848963,-17.0548011239751,
12.));
#230948=CARTESIAN_POINT('Ctrl Pts',(-18.547078218209,-17.0303771481738,
0.));
#230949=CARTESIAN_POINT('Ctrl Pts',(-18.547078218209,-17.0303771481738,
12.));
#230950=CARTESIAN_POINT('Ctrl Pts',(-18.5376893576961,-17.0060468805097,
0.));
#230951=CARTESIAN_POINT('Ctrl Pts',(-18.5376893576961,-17.0060468805097,
12.));
#230952=CARTESIAN_POINT('Ctrl Pts',(-18.5282716744197,-16.981810668038,
0.));
#230953=CARTESIAN_POINT('Ctrl Pts',(-18.5282716744197,-16.981810668038,
12.));
#230954=CARTESIAN_POINT('Ctrl Pts',(-18.5188255796659,-16.9576688599339,
0.));
#230955=CARTESIAN_POINT('Ctrl Pts',(-18.5188255796659,-16.9576688599339,
12.));
#230956=CARTESIAN_POINT('Ctrl Pts',(-18.5093514883835,-16.9336218069353,
0.));
#230957=CARTESIAN_POINT('Ctrl Pts',(-18.5093514883835,-16.9336218069353,
12.));
#230958=CARTESIAN_POINT('Ctrl Pts',(-18.499849818462,-16.9096698606943,
0.));
#230959=CARTESIAN_POINT('Ctrl Pts',(-18.499849818462,-16.9096698606943,
12.));
#230960=CARTESIAN_POINT('Ctrl Pts',(-18.4903209902227,-16.8858133733088,
0.));
#230961=CARTESIAN_POINT('Ctrl Pts',(-18.4903209902227,-16.8858133733088,
12.));
#230962=CARTESIAN_POINT('Ctrl Pts',(-18.4807654268771,-16.8620526977171,
0.));
#230963=CARTESIAN_POINT('Ctrl Pts',(-18.4807654268771,-16.8620526977171,
12.));
#230964=CARTESIAN_POINT('Ctrl Pts',(-18.4711835548623,-16.8383881879709,
0.));
#230965=CARTESIAN_POINT('Ctrl Pts',(-18.4711835548623,-16.8383881879709,
12.));
#230966=CARTESIAN_POINT('Ctrl Pts',(-18.4615758042305,-16.8148201995472,
0.));
#230967=CARTESIAN_POINT('Ctrl Pts',(-18.4615758042305,-16.8148201995472,
12.));
#230968=CARTESIAN_POINT('Ctrl Pts',(-18.4519426090124,-16.791349089629,
0.));
#230969=CARTESIAN_POINT('Ctrl Pts',(-18.4519426090124,-16.791349089629,
12.));
#230970=CARTESIAN_POINT('Ctrl Pts',(-18.44228440761,-16.7679752173992,0.));
#230971=CARTESIAN_POINT('Ctrl Pts',(-18.44228440761,-16.7679752173992,12.));
#230972=CARTESIAN_POINT('Ctrl Pts',(-18.4326016431392,-16.7446989442882,
0.));
#230973=CARTESIAN_POINT('Ctrl Pts',(-18.4326016431392,-16.7446989442882,
12.));
#230974=CARTESIAN_POINT('Ctrl Pts',(-18.4228947633187,-16.7215206338818,
0.));
#230975=CARTESIAN_POINT('Ctrl Pts',(-18.4228947633187,-16.7215206338818,
12.));
#230976=CARTESIAN_POINT('Ctrl Pts',(-18.413164220399,-16.6984406518491,
0.));
#230977=CARTESIAN_POINT('Ctrl Pts',(-18.413164220399,-16.6984406518491,
12.));
#230978=CARTESIAN_POINT('Ctrl Pts',(-18.403410471079,-16.6754593658513,
0.));
#230979=CARTESIAN_POINT('Ctrl Pts',(-18.403410471079,-16.6754593658513,
12.));
#230980=CARTESIAN_POINT('Ctrl Pts',(-18.3936339764332,-16.6525771454513,
0.));
#230981=CARTESIAN_POINT('Ctrl Pts',(-18.3936339764332,-16.6525771454513,
12.));
#230982=CARTESIAN_POINT('Ctrl Pts',(-18.3838352018327,-16.6297943620056,
0.));
#230983=CARTESIAN_POINT('Ctrl Pts',(-18.3838352018327,-16.6297943620056,
12.));
#230984=CARTESIAN_POINT('Ctrl Pts',(-18.3740146168879,-16.607111388571,
0.));
#230985=CARTESIAN_POINT('Ctrl Pts',(-18.3740146168879,-16.607111388571,
12.));
#230986=CARTESIAN_POINT('Ctrl Pts',(-18.3641726955889,-16.5845286000217,
0.));
#230987=CARTESIAN_POINT('Ctrl Pts',(-18.3641726955889,-16.5845286000217,
12.));
#230988=CARTESIAN_POINT('Ctrl Pts',(-18.354309916433,-16.5620463731413,
0.));
#230989=CARTESIAN_POINT('Ctrl Pts',(-18.354309916433,-16.5620463731413,
12.));
#230990=CARTESIAN_POINT('Ctrl Pts',(-18.34442676256,-16.5396650867139,0.));
#230991=CARTESIAN_POINT('Ctrl Pts',(-18.34442676256,-16.5396650867139,12.));
#230992=CARTESIAN_POINT('Ctrl Pts',(-18.3345237218864,-16.5173851216045,
0.));
#230993=CARTESIAN_POINT('Ctrl Pts',(-18.3345237218864,-16.5173851216045,
12.));
#230994=CARTESIAN_POINT('Ctrl Pts',(-18.3246012872469,-16.4952068608345,
0.));
#230995=CARTESIAN_POINT('Ctrl Pts',(-18.3246012872469,-16.4952068608345,
12.));
#230996=CARTESIAN_POINT('Ctrl Pts',(-18.3146599565231,-16.4731306896441,
0.));
#230997=CARTESIAN_POINT('Ctrl Pts',(-18.3146599565231,-16.4731306896441,
12.));
#230998=CARTESIAN_POINT('Ctrl Pts',(-18.304700232686,-16.4511569955233,
0.));
#230999=CARTESIAN_POINT('Ctrl Pts',(-18.304700232686,-16.4511569955233,
12.));
#231000=CARTESIAN_POINT('Ctrl Pts',(-18.294722623851,-16.4292861682379,
0.));
#231001=CARTESIAN_POINT('Ctrl Pts',(-18.294722623851,-16.4292861682379,
12.));
#231002=CARTESIAN_POINT('Ctrl Pts',(-18.2847276433309,-16.4075185998455,
0.));
#231003=CARTESIAN_POINT('Ctrl Pts',(-18.2847276433309,-16.4075185998455,
12.));
#231004=CARTESIAN_POINT('Ctrl Pts',(-18.2747158096934,-16.385854684708,
0.));
#231005=CARTESIAN_POINT('Ctrl Pts',(-18.2747158096934,-16.385854684708,
12.));
#231006=CARTESIAN_POINT('Ctrl Pts',(-18.2646876468169,-16.3642948194868,
0.));
#231007=CARTESIAN_POINT('Ctrl Pts',(-18.2646876468169,-16.3642948194868,
12.));
#231008=CARTESIAN_POINT('Ctrl Pts',(-18.2546436839608,-16.3428394031589,
0.));
#231009=CARTESIAN_POINT('Ctrl Pts',(-18.2546436839608,-16.3428394031589,
12.));
#231010=CARTESIAN_POINT('Ctrl Pts',(-18.2445844558742,-16.3214888370987,
0.));
#231011=CARTESIAN_POINT('Ctrl Pts',(-18.2445844558742,-16.3214888370987,
12.));
#231012=CARTESIAN_POINT('Ctrl Pts',(-18.2345105028982,-16.3002435251378,
0.));
#231013=CARTESIAN_POINT('Ctrl Pts',(-18.2345105028982,-16.3002435251378,
12.));
#231014=CARTESIAN_POINT('Ctrl Pts',(-18.2244223710746,-16.2791038736223,
0.));
#231015=CARTESIAN_POINT('Ctrl Pts',(-18.2244223710746,-16.2791038736223,
12.));
#231016=CARTESIAN_POINT('Ctrl Pts',(-18.2143206122529,-16.2580702914615,
0.));
#231017=CARTESIAN_POINT('Ctrl Pts',(-18.2143206122529,-16.2580702914615,
12.));
#231018=CARTESIAN_POINT('Ctrl Pts',(-18.2042057842035,-16.2371431901638,
0.));
#231019=CARTESIAN_POINT('Ctrl Pts',(-18.2042057842035,-16.2371431901638,
12.));
#231020=CARTESIAN_POINT('Ctrl Pts',(-18.1940784507229,-16.2163229838875,
0.));
#231021=CARTESIAN_POINT('Ctrl Pts',(-18.1940784507229,-16.2163229838875,
12.));
#231022=CARTESIAN_POINT('Ctrl Pts',(-18.1839391817331,-16.1956100895073,
0.));
#231023=CARTESIAN_POINT('Ctrl Pts',(-18.1839391817331,-16.1956100895073,
12.));
#231024=CARTESIAN_POINT('Ctrl Pts',(-18.1737885533849,-16.1750049266671,
0.));
#231025=CARTESIAN_POINT('Ctrl Pts',(-18.1737885533849,-16.1750049266671,
12.));
#231026=CARTESIAN_POINT('Ctrl Pts',(-18.1636271481615,-16.154507917826,
0.));
#231027=CARTESIAN_POINT('Ctrl Pts',(-18.1636271481615,-16.154507917826,
12.));
#231028=CARTESIAN_POINT('Ctrl Pts',(-18.1534555549852,-16.1341194882988,
0.));
#231029=CARTESIAN_POINT('Ctrl Pts',(-18.1534555549852,-16.1341194882988,
12.));
#231030=CARTESIAN_POINT('Ctrl Pts',(-18.1432743693235,-16.1138400662794,
0.));
#231031=CARTESIAN_POINT('Ctrl Pts',(-18.1432743693235,-16.1138400662794,
12.));
#231032=CARTESIAN_POINT('Ctrl Pts',(-18.1330841933105,-16.0936700829112,
0.));
#231033=CARTESIAN_POINT('Ctrl Pts',(-18.1330841933105,-16.0936700829112,
12.));
#231034=CARTESIAN_POINT('Ctrl Pts',(-18.1228856358751,-16.0736099723668,
0.));
#231035=CARTESIAN_POINT('Ctrl Pts',(-18.1228856358751,-16.0736099723668,
12.));
#231036=CARTESIAN_POINT('Ctrl Pts',(-18.112679312869,-16.0536601719126,
0.));
#231037=CARTESIAN_POINT('Ctrl Pts',(-18.112679312869,-16.0536601719126,
12.));
#231038=CARTESIAN_POINT('Ctrl Pts',(-18.1024658471966,-16.0338211219693,
0.));
#231039=CARTESIAN_POINT('Ctrl Pts',(-18.1024658471966,-16.0338211219693,
12.));
#231040=CARTESIAN_POINT('Ctrl Pts',(-18.0922458689462,-16.014093266161,
0.));
#231041=CARTESIAN_POINT('Ctrl Pts',(-18.0922458689462,-16.014093266161,
12.));
#231042=CARTESIAN_POINT('Ctrl Pts',(-18.0820200155236,-15.9944770513613,
0.));
#231043=CARTESIAN_POINT('Ctrl Pts',(-18.0820200155236,-15.9944770513613,
12.));
#231044=CARTESIAN_POINT('Ctrl Pts',(-18.0717889317958,-15.9749729277846,
0.));
#231045=CARTESIAN_POINT('Ctrl Pts',(-18.0717889317958,-15.9749729277846,
12.));
#231046=CARTESIAN_POINT('Ctrl Pts',(-18.061553270236,-15.9555813490644,
0.));
#231047=CARTESIAN_POINT('Ctrl Pts',(-18.061553270236,-15.9555813490644,
12.));
#231048=CARTESIAN_POINT('Ctrl Pts',(-18.0513136910691,-15.9363027723244,
0.));
#231049=CARTESIAN_POINT('Ctrl Pts',(-18.0513136910691,-15.9363027723244,
12.));
#231050=CARTESIAN_POINT('Ctrl Pts',(-18.0410708624208,-15.9171376582436,
0.));
#231051=CARTESIAN_POINT('Ctrl Pts',(-18.0410708624208,-15.9171376582436,
12.));
#231052=CARTESIAN_POINT('Ctrl Pts',(-18.0308254604636,-15.8980864711042,
0.));
#231053=CARTESIAN_POINT('Ctrl Pts',(-18.0308254604636,-15.8980864711042,
12.));
#231054=CARTESIAN_POINT('Ctrl Pts',(-18.0205781695769,-15.8791496788682,
0.));
#231055=CARTESIAN_POINT('Ctrl Pts',(-18.0205781695769,-15.8791496788682,
12.));
#231056=CARTESIAN_POINT('Ctrl Pts',(-18.0103296825205,-15.8603277532831,
0.));
#231057=CARTESIAN_POINT('Ctrl Pts',(-18.0103296825205,-15.8603277532831,
12.));
#231058=CARTESIAN_POINT('Ctrl Pts',(-18.0000807006052,-15.8416211699679,
0.));
#231059=CARTESIAN_POINT('Ctrl Pts',(-18.0000807006052,-15.8416211699679,
12.));
#231060=CARTESIAN_POINT('Ctrl Pts',(-17.9898319338664,-15.8230304084962,
0.));
#231061=CARTESIAN_POINT('Ctrl Pts',(-17.9898319338664,-15.8230304084962,
12.));
#231062=CARTESIAN_POINT('Ctrl Pts',(-17.9795841012386,-15.8045559524676,
0.));
#231063=CARTESIAN_POINT('Ctrl Pts',(-17.9795841012386,-15.8045559524676,
12.));
#231064=CARTESIAN_POINT('Ctrl Pts',(-17.9693379307303,-15.7861982895724,
0.));
#231065=CARTESIAN_POINT('Ctrl Pts',(-17.9693379307303,-15.7861982895724,
12.));
#231066=CARTESIAN_POINT('Ctrl Pts',(-17.9590941596242,-15.7679579117077,
0.));
#231067=CARTESIAN_POINT('Ctrl Pts',(-17.9590941596242,-15.7679579117077,
12.));
#231068=CARTESIAN_POINT('Ctrl Pts',(-17.9488535346781,-15.749835315086,
0.));
#231069=CARTESIAN_POINT('Ctrl Pts',(-17.9488535346781,-15.749835315086,
12.));
#231070=CARTESIAN_POINT('Ctrl Pts',(-17.9386168123262,-15.7318310003335,
0.));
#231071=CARTESIAN_POINT('Ctrl Pts',(-17.9386168123262,-15.7318310003335,
12.));
#231072=CARTESIAN_POINT('Ctrl Pts',(-17.9283847588836,-15.7139454725838,
0.));
#231073=CARTESIAN_POINT('Ctrl Pts',(-17.9283847588836,-15.7139454725838,
12.));
#231074=CARTESIAN_POINT('Ctrl Pts',(-17.9181581507455,-15.6961792415522,
0.));
#231075=CARTESIAN_POINT('Ctrl Pts',(-17.9181581507455,-15.6961792415522,
12.));
#231076=CARTESIAN_POINT('Ctrl Pts',(-17.9079377746111,-15.678532821646,
0.));
#231077=CARTESIAN_POINT('Ctrl Pts',(-17.9079377746111,-15.678532821646,
12.));
#231078=CARTESIAN_POINT('Ctrl Pts',(-17.897724427724,-15.661006732103,0.));
#231079=CARTESIAN_POINT('Ctrl Pts',(-17.897724427724,-15.661006732103,12.));
#231080=CARTESIAN_POINT('Ctrl Pts',(-17.8875189181091,-15.6436014971084,
0.));
#231081=CARTESIAN_POINT('Ctrl Pts',(-17.8875189181091,-15.6436014971084,
12.));
#231082=CARTESIAN_POINT('Ctrl Pts',(-17.8773220648125,-15.6263176459108,
0.));
#231083=CARTESIAN_POINT('Ctrl Pts',(-17.8773220648125,-15.6263176459108,
12.));
#231084=CARTESIAN_POINT('Ctrl Pts',(-17.8671346981394,-15.609155712921,
0.));
#231085=CARTESIAN_POINT('Ctrl Pts',(-17.8671346981394,-15.609155712921,
12.));
#231086=CARTESIAN_POINT('Ctrl Pts',(-17.8569576599006,-15.5921162378192,
0.));
#231087=CARTESIAN_POINT('Ctrl Pts',(-17.8569576599006,-15.5921162378192,
12.));
#231088=CARTESIAN_POINT('Ctrl Pts',(-17.8467918036987,-15.5751997657163,
0.));
#231089=CARTESIAN_POINT('Ctrl Pts',(-17.8467918036987,-15.5751997657163,
12.));
#231090=CARTESIAN_POINT('Ctrl Pts',(-17.8366379952085,-15.5584068472982,
0.));
#231091=CARTESIAN_POINT('Ctrl Pts',(-17.8366379952085,-15.5584068472982,
12.));
#231092=CARTESIAN_POINT('Ctrl Pts',(-17.8264971124607,-15.541738038964,
0.));
#231093=CARTESIAN_POINT('Ctrl Pts',(-17.8264971124607,-15.541738038964,
12.));
#231094=CARTESIAN_POINT('Ctrl Pts',(-17.8163700461256,-15.5251939029552,
0.));
#231095=CARTESIAN_POINT('Ctrl Pts',(-17.8163700461256,-15.5251939029552,
12.));
#231096=CARTESIAN_POINT('Ctrl Pts',(-17.8062576997952,-15.5087750074718,
0.));
#231097=CARTESIAN_POINT('Ctrl Pts',(-17.8062576997952,-15.5087750074718,
12.));
#231098=CARTESIAN_POINT('Ctrl Pts',(-17.7961609903148,-15.4924819268517,
0.));
#231099=CARTESIAN_POINT('Ctrl Pts',(-17.7961609903148,-15.4924819268517,
12.));
#231100=CARTESIAN_POINT('Ctrl Pts',(-17.786080848122,-15.4763152417497,
0.));
#231101=CARTESIAN_POINT('Ctrl Pts',(-17.786080848122,-15.4763152417497,
12.));
#231102=CARTESIAN_POINT('Ctrl Pts',(-17.7760182175815,-15.4602755393017,
0.));
#231103=CARTESIAN_POINT('Ctrl Pts',(-17.7760182175815,-15.4602755393017,
12.));
#231104=CARTESIAN_POINT('Ctrl Pts',(-17.7659740573265,-15.4443634132869,
0.));
#231105=CARTESIAN_POINT('Ctrl Pts',(-17.7659740573265,-15.4443634132869,
12.));
#231106=CARTESIAN_POINT('Ctrl Pts',(-17.7559493405881,-15.4285794642668,
0.));
#231107=CARTESIAN_POINT('Ctrl Pts',(-17.7559493405881,-15.4285794642668,
12.));
#231108=CARTESIAN_POINT('Ctrl Pts',(-17.7459450555812,-15.4129242997837,
0.));
#231109=CARTESIAN_POINT('Ctrl Pts',(-17.7459450555812,-15.4129242997837,
12.));
#231110=CARTESIAN_POINT('Ctrl Pts',(-17.735962205915,-15.3973985345802,
0.));
#231111=CARTESIAN_POINT('Ctrl Pts',(-17.735962205915,-15.3973985345802,
12.));
#231112=CARTESIAN_POINT('Ctrl Pts',(-17.7260018109924,-15.3820027907967,
0.));
#231113=CARTESIAN_POINT('Ctrl Pts',(-17.7260018109924,-15.3820027907967,
12.));
#231114=CARTESIAN_POINT('Ctrl Pts',(-17.7160649064206,-15.3667376981699,
0.));
#231115=CARTESIAN_POINT('Ctrl Pts',(-17.7160649064206,-15.3667376981699,
12.));
#231116=CARTESIAN_POINT('Ctrl Pts',(-17.7061525444042,-15.351603894206,
0.));
#231117=CARTESIAN_POINT('Ctrl Pts',(-17.7061525444042,-15.351603894206,
12.));
#231118=CARTESIAN_POINT('Ctrl Pts',(-17.6962657941983,-15.3366020244066,
0.));
#231119=CARTESIAN_POINT('Ctrl Pts',(-17.6962657941983,-15.3366020244066,
12.));
#231120=CARTESIAN_POINT('Ctrl Pts',(-17.6864057426052,-15.3217327425338,
0.));
#231121=CARTESIAN_POINT('Ctrl Pts',(-17.6864057426052,-15.3217327425338,
12.));
#231122=CARTESIAN_POINT('Ctrl Pts',(-17.676573494456,-15.3069967108501,
0.));
#231123=CARTESIAN_POINT('Ctrl Pts',(-17.676573494456,-15.3069967108501,
12.));
#231124=CARTESIAN_POINT('Ctrl Pts',(-17.6667701731041,-15.2923946003598,
0.));
#231125=CARTESIAN_POINT('Ctrl Pts',(-17.6667701731041,-15.2923946003598,
12.));
#231126=CARTESIAN_POINT('Ctrl Pts',(-17.6569969209,-15.2779270910239,0.));
#231127=CARTESIAN_POINT('Ctrl Pts',(-17.6569969209,-15.2779270910239,12.));
#231128=CARTESIAN_POINT('Ctrl Pts',(-17.6472548997328,-15.2635948720292,
0.));
#231129=CARTESIAN_POINT('Ctrl Pts',(-17.6472548997328,-15.2635948720292,
12.));
#231130=CARTESIAN_POINT('Ctrl Pts',(-17.6375452916369,-15.2493986421092,
0.));
#231131=CARTESIAN_POINT('Ctrl Pts',(-17.6375452916369,-15.2493986421092,
12.));
#231132=CARTESIAN_POINT('Ctrl Pts',(-17.6278692993764,-15.2353391098366,
0.));
#231133=CARTESIAN_POINT('Ctrl Pts',(-17.6278692993764,-15.2353391098366,
12.));
#231134=CARTESIAN_POINT('Ctrl Pts',(-17.6182281470468,-15.2214169939199,
0.));
#231135=CARTESIAN_POINT('Ctrl Pts',(-17.6182281470468,-15.2214169939199,
12.));
#231136=CARTESIAN_POINT('Ctrl Pts',(-17.60862308065,-15.2076330234686,0.));
#231137=CARTESIAN_POINT('Ctrl Pts',(-17.60862308065,-15.2076330234686,12.));
#231138=CARTESIAN_POINT('Ctrl Pts',(-17.5990553687599,-15.1939879383268,
0.));
#231139=CARTESIAN_POINT('Ctrl Pts',(-17.5990553687599,-15.1939879383268,
12.));
#231140=CARTESIAN_POINT('Ctrl Pts',(-17.5895263032595,-15.1804824894605,
0.));
#231141=CARTESIAN_POINT('Ctrl Pts',(-17.5895263032595,-15.1804824894605,
12.));
#231142=CARTESIAN_POINT('Ctrl Pts',(-17.580037200054,-15.1671174393137,
0.));
#231143=CARTESIAN_POINT('Ctrl Pts',(-17.580037200054,-15.1671174393137,
12.));
#231144=CARTESIAN_POINT('Ctrl Pts',(-17.5705893998029,-15.1538935621714,
0.));
#231145=CARTESIAN_POINT('Ctrl Pts',(-17.5705893998029,-15.1538935621714,
12.));
#231146=CARTESIAN_POINT('Ctrl Pts',(-17.5611842686192,-15.1408116444876,
0.));
#231147=CARTESIAN_POINT('Ctrl Pts',(-17.5611842686192,-15.1408116444876,
12.));
#231148=CARTESIAN_POINT('Ctrl Pts',(-17.5518231989117,-15.1278724853138,
0.));
#231149=CARTESIAN_POINT('Ctrl Pts',(-17.5518231989117,-15.1278724853138,
12.));
#231150=CARTESIAN_POINT('Ctrl Pts',(-17.5425076102963,-15.1150768967728,
0.));
#231151=CARTESIAN_POINT('Ctrl Pts',(-17.5425076102963,-15.1150768967728,
12.));
#231152=CARTESIAN_POINT('Ctrl Pts',(-17.5332389504829,-15.1024257045033,
0.));
#231153=CARTESIAN_POINT('Ctrl Pts',(-17.5332389504829,-15.1024257045033,
12.));
#231154=CARTESIAN_POINT('Ctrl Pts',(-17.5240186961791,-15.0899197481082,
0.));
#231155=CARTESIAN_POINT('Ctrl Pts',(-17.5240186961791,-15.0899197481082,
12.));
#231156=CARTESIAN_POINT('Ctrl Pts',(-17.5148483539687,-15.0775598815749,
0.));
#231157=CARTESIAN_POINT('Ctrl Pts',(-17.5148483539687,-15.0775598815749,
12.));
#231158=CARTESIAN_POINT('Ctrl Pts',(-17.5057294613877,-15.0653469738307,
0.));
#231159=CARTESIAN_POINT('Ctrl Pts',(-17.5057294613877,-15.0653469738307,
12.));
#231160=CARTESIAN_POINT('Ctrl Pts',(-17.4966635880246,-15.0532819093085,
0.));
#231161=CARTESIAN_POINT('Ctrl Pts',(-17.4966635880246,-15.0532819093085,
12.));
#231162=CARTESIAN_POINT('Ctrl Pts',(-17.4876523366178,-15.0413655884993,
0.));
#231163=CARTESIAN_POINT('Ctrl Pts',(-17.4876523366178,-15.0413655884993,
12.));
#231164=CARTESIAN_POINT('Ctrl Pts',(-17.4786973441417,-15.029598928488,
0.));
#231165=CARTESIAN_POINT('Ctrl Pts',(-17.4786973441417,-15.029598928488,
12.));
#231166=CARTESIAN_POINT('Ctrl Pts',(-17.4698002829357,-15.0179828635087,
0.));
#231167=CARTESIAN_POINT('Ctrl Pts',(-17.4698002829357,-15.0179828635087,
12.));
#231168=CARTESIAN_POINT('Ctrl Pts',(-17.4609628621419,-15.0065183456922,
0.));
#231169=CARTESIAN_POINT('Ctrl Pts',(-17.4609628621419,-15.0065183456922,
12.));
#231170=CARTESIAN_POINT('Ctrl Pts',(-17.4521868291005,-14.9952063457779,
0.));
#231171=CARTESIAN_POINT('Ctrl Pts',(-17.4521868291005,-14.9952063457779,
12.));
#231172=CARTESIAN_POINT('Ctrl Pts',(-17.4434739707773,-14.9840478538357,
0.));
#231173=CARTESIAN_POINT('Ctrl Pts',(-17.4434739707773,-14.9840478538357,
12.));
#231174=CARTESIAN_POINT('Ctrl Pts',(-17.4348261151395,-14.973043879945,
0.));
#231175=CARTESIAN_POINT('Ctrl Pts',(-17.4348261151395,-14.973043879945,
12.));
#231176=CARTESIAN_POINT('Ctrl Pts',(-17.4262451327088,-14.9621954549825,
0.));
#231177=CARTESIAN_POINT('Ctrl Pts',(-17.4262451327088,-14.9621954549825,
12.));
#231178=CARTESIAN_POINT('Ctrl Pts',(-17.4177329382827,-14.9515036315142,
0.));
#231179=CARTESIAN_POINT('Ctrl Pts',(-17.4177329382827,-14.9515036315142,
12.));
#231180=CARTESIAN_POINT('Ctrl Pts',(-17.4092914926071,-14.940969484645,
0.));
#231181=CARTESIAN_POINT('Ctrl Pts',(-17.4092914926071,-14.940969484645,
12.));
#231182=CARTESIAN_POINT('Ctrl Pts',(-17.400922804075,-14.9305941128758,
0.));
#231183=CARTESIAN_POINT('Ctrl Pts',(-17.400922804075,-14.9305941128758,
12.));
#231184=CARTESIAN_POINT('Ctrl Pts',(-17.3926289303987,-14.9203786389343,
0.));
#231185=CARTESIAN_POINT('Ctrl Pts',(-17.3926289303987,-14.9203786389343,
12.));
#231186=CARTESIAN_POINT('Ctrl Pts',(-17.3844119809823,-14.9103242110057,
0.));
#231187=CARTESIAN_POINT('Ctrl Pts',(-17.3844119809823,-14.9103242110057,
12.));
#231188=CARTESIAN_POINT('Ctrl Pts',(-17.3762741193075,-14.9004320039609,
0.));
#231189=CARTESIAN_POINT('Ctrl Pts',(-17.3762741193075,-14.9004320039609,
12.));
#231190=CARTESIAN_POINT('Ctrl Pts',(-17.3682175653236,-14.8907032205789,
0.));
#231191=CARTESIAN_POINT('Ctrl Pts',(-17.3682175653236,-14.8907032205789,
12.));
#231192=CARTESIAN_POINT('Ctrl Pts',(-17.3602445978163,-14.8811390927424,
0.));
#231193=CARTESIAN_POINT('Ctrl Pts',(-17.3602445978163,-14.8811390927424,
12.));
#231194=CARTESIAN_POINT('Ctrl Pts',(-17.3523575568648,-14.8717408826958,
0.));
#231195=CARTESIAN_POINT('Ctrl Pts',(-17.3523575568648,-14.8717408826958,
12.));
#231196=CARTESIAN_POINT('Ctrl Pts',(-17.3445588463477,-14.8625098843419,
0.));
#231197=CARTESIAN_POINT('Ctrl Pts',(-17.3445588463477,-14.8625098843419,
12.));
#231198=CARTESIAN_POINT('Ctrl Pts',(-17.336850936485,-14.8534474245433,
0.));
#231199=CARTESIAN_POINT('Ctrl Pts',(-17.336850936485,-14.8534474245433,
12.));
#231200=CARTESIAN_POINT('Ctrl Pts',(-17.3292363662601,-14.8445548643505,
0.));
#231201=CARTESIAN_POINT('Ctrl Pts',(-17.3292363662601,-14.8445548643505,
12.));
#231202=CARTESIAN_POINT('Ctrl Pts',(-17.3217177462096,-14.8358336004193,
0.));
#231203=CARTESIAN_POINT('Ctrl Pts',(-17.3217177462096,-14.8358336004193,
12.));
#231204=CARTESIAN_POINT('Ctrl Pts',(-17.3142977632656,-14.8272850675375,
0.));
#231205=CARTESIAN_POINT('Ctrl Pts',(-17.3142977632656,-14.8272850675375,
12.));
#231206=CARTESIAN_POINT('Ctrl Pts',(-17.3069791853705,-14.8189107410161,
0.));
#231207=CARTESIAN_POINT('Ctrl Pts',(-17.3069791853705,-14.8189107410161,
12.));
#231208=CARTESIAN_POINT('Ctrl Pts',(-17.2997648661483,-14.8107121391038,
0.));
#231209=CARTESIAN_POINT('Ctrl Pts',(-17.2997648661483,-14.8107121391038,
12.));
#231210=CARTESIAN_POINT('Ctrl Pts',(-17.2926577496519,-14.8026908254281,
0.));
#231211=CARTESIAN_POINT('Ctrl Pts',(-17.2926577496519,-14.8026908254281,
12.));
#231212=CARTESIAN_POINT('Ctrl Pts',(-17.28566087332,-14.7948484105253,0.));
#231213=CARTESIAN_POINT('Ctrl Pts',(-17.28566087332,-14.7948484105253,12.));
#231214=CARTESIAN_POINT('Ctrl Pts',(-17.278777370485,-14.787186553128,0.));
#231215=CARTESIAN_POINT('Ctrl Pts',(-17.278777370485,-14.787186553128,12.));
#231216=CARTESIAN_POINT('Ctrl Pts',(-17.2720104735192,-14.7797069617802,
0.));
#231217=CARTESIAN_POINT('Ctrl Pts',(-17.2720104735192,-14.7797069617802,
12.));
#231218=CARTESIAN_POINT('Ctrl Pts',(-17.2653635155317,-14.7724113956728,
0.));
#231219=CARTESIAN_POINT('Ctrl Pts',(-17.2653635155317,-14.7724113956728,
12.));
#231220=CARTESIAN_POINT('Ctrl Pts',(-17.2588399401464,-14.7653016697589,
0.));
#231221=CARTESIAN_POINT('Ctrl Pts',(-17.2588399401464,-14.7653016697589,
12.));
#231222=CARTESIAN_POINT('Ctrl Pts',(-17.2524433146837,-14.7583796616617,
0.));
#231223=CARTESIAN_POINT('Ctrl Pts',(-17.2524433146837,-14.7583796616617,
12.));
#231224=CARTESIAN_POINT('Ctrl Pts',(-17.2461773413289,-14.7516473175125,
0.));
#231225=CARTESIAN_POINT('Ctrl Pts',(-17.2461773413289,-14.7516473175125,
12.));
#231226=CARTESIAN_POINT('Ctrl Pts',(-17.2400458713566,-14.7451066593793,
0.));
#231227=CARTESIAN_POINT('Ctrl Pts',(-17.2400458713566,-14.7451066593793,
12.));
#231228=CARTESIAN_POINT('Ctrl Pts',(-17.2340529062077,-14.7387597858117,
0.));
#231229=CARTESIAN_POINT('Ctrl Pts',(-17.2340529062077,-14.7387597858117,
12.));
#231230=CARTESIAN_POINT('Ctrl Pts',(-17.2282025904314,-14.7326088681163,
0.));
#231231=CARTESIAN_POINT('Ctrl Pts',(-17.2282025904314,-14.7326088681163,
12.));
#231232=CARTESIAN_POINT('Ctrl Pts',(-17.2224992099666,-14.7266561494282,
0.));
#231233=CARTESIAN_POINT('Ctrl Pts',(-17.2224992099666,-14.7266561494282,
12.));
#231234=CARTESIAN_POINT('Ctrl Pts',(-17.2169471814255,-14.7209039390326,
0.));
#231235=CARTESIAN_POINT('Ctrl Pts',(-17.2169471814255,-14.7209039390326,
12.));
#231236=CARTESIAN_POINT('Ctrl Pts',(-17.2115510835988,-14.7153546289338,
0.));
#231237=CARTESIAN_POINT('Ctrl Pts',(-17.2115510835988,-14.7153546289338,
12.));
#231238=CARTESIAN_POINT('Ctrl Pts',(-17.2063157097316,-14.7100107213586,
0.));
#231239=CARTESIAN_POINT('Ctrl Pts',(-17.2063157097316,-14.7100107213586,
12.));
#231240=CARTESIAN_POINT('Ctrl Pts',(-17.2012461084268,-14.7048748502663,
0.));
#231241=CARTESIAN_POINT('Ctrl Pts',(-17.2012461084268,-14.7048748502663,
12.));
#231242=CARTESIAN_POINT('Ctrl Pts',(-17.1963476411694,-14.699949811582,
0.));
#231243=CARTESIAN_POINT('Ctrl Pts',(-17.1963476411694,-14.699949811582,
12.));
#231244=CARTESIAN_POINT('Ctrl Pts',(-17.1916259308416,-14.6952385361706,
0.));
#231245=CARTESIAN_POINT('Ctrl Pts',(-17.1916259308416,-14.6952385361706,
12.));
#231246=CARTESIAN_POINT('Ctrl Pts',(-17.1870867909918,-14.6907440526958,
0.));
#231247=CARTESIAN_POINT('Ctrl Pts',(-17.1870867909918,-14.6907440526958,
12.));
#231248=CARTESIAN_POINT('Ctrl Pts',(-17.182736158472,-14.6864694522319,
0.));
#231249=CARTESIAN_POINT('Ctrl Pts',(-17.182736158472,-14.6864694522319,
12.));
#231250=CARTESIAN_POINT('Ctrl Pts',(-17.1785800350827,-14.6824178576167,
0.));
#231251=CARTESIAN_POINT('Ctrl Pts',(-17.1785800350827,-14.6824178576167,
12.));
#231252=CARTESIAN_POINT('Ctrl Pts',(-17.1746247499057,-14.6785925615676,
0.));
#231253=CARTESIAN_POINT('Ctrl Pts',(-17.1746247499057,-14.6785925615676,
12.));
#231254=CARTESIAN_POINT('Ctrl Pts',(-17.1708771619129,-14.6749971333867,
0.));
#231255=CARTESIAN_POINT('Ctrl Pts',(-17.1708771619129,-14.6749971333867,
12.));
#231256=CARTESIAN_POINT('Ctrl Pts',(-17.1673449723019,-14.6716355833321,
0.));
#231257=CARTESIAN_POINT('Ctrl Pts',(-17.1673449723019,-14.6716355833321,
12.));
#231258=CARTESIAN_POINT('Ctrl Pts',(-17.1640366762304,-14.6685123374424,
0.));
#231259=CARTESIAN_POINT('Ctrl Pts',(-17.1640366762304,-14.6685123374424,
12.));
#231260=CARTESIAN_POINT('Ctrl Pts',(-17.1609609517369,-14.6656319165057,
0.));
#231261=CARTESIAN_POINT('Ctrl Pts',(-17.1609609517369,-14.6656319165057,
12.));
#231262=CARTESIAN_POINT('Ctrl Pts',(-17.1581262646789,-14.662998728599,
0.));
#231263=CARTESIAN_POINT('Ctrl Pts',(-17.1581262646789,-14.662998728599,
12.));
#231264=CARTESIAN_POINT('Ctrl Pts',(-17.1555401986403,-14.660616716964,
0.));
#231265=CARTESIAN_POINT('Ctrl Pts',(-17.1555401986403,-14.660616716964,
12.));
#231266=CARTESIAN_POINT('Ctrl Pts',(-17.1532107762719,-14.6584900555301,
0.));
#231267=CARTESIAN_POINT('Ctrl Pts',(-17.1532107762719,-14.6584900555301,
12.));
#231268=CARTESIAN_POINT('Ctrl Pts',(-17.1511476869495,-14.6566237952435,
0.));
#231269=CARTESIAN_POINT('Ctrl Pts',(-17.1511476869495,-14.6566237952435,
12.));
#231270=CARTESIAN_POINT('Ctrl Pts',(-17.1493641837556,-14.6550248622813,
0.));
#231271=CARTESIAN_POINT('Ctrl Pts',(-17.1493641837556,-14.6550248622813,
12.));
#231272=CARTESIAN_POINT('Ctrl Pts',(-17.1478763944909,-14.6537016966188,
0.));
#231273=CARTESIAN_POINT('Ctrl Pts',(-17.1478763944909,-14.6537016966188,
12.));
#231274=CARTESIAN_POINT('Ctrl Pts',(-17.1466998098673,-14.6526624064978,
0.));
#231275=CARTESIAN_POINT('Ctrl Pts',(-17.1466998098673,-14.6526624064978,
12.));
#231276=CARTESIAN_POINT('Ctrl Pts',(-17.1458462295273,-14.65191316345,0.));
#231277=CARTESIAN_POINT('Ctrl Pts',(-17.1458462295273,-14.65191316345,12.));
#231278=CARTESIAN_POINT('Ctrl Pts',(-17.1454262858045,-14.6515481598057,
0.));
#231279=CARTESIAN_POINT('Ctrl Pts',(-17.1454262858045,-14.6515481598057,
12.));
#231280=CARTESIAN_POINT('Ctrl Pts',(-17.1452600887039,-14.6514066997188,
0.));
#231281=CARTESIAN_POINT('Ctrl Pts',(-17.1452600887039,-14.6514066997188,
12.));
#231282=CARTESIAN_POINT('Ctrl Pts',(-17.1452153999142,-14.651371185284,
0.));
#231283=CARTESIAN_POINT('Ctrl Pts',(-17.1452153999142,-14.651371185284,
12.));
#231284=CARTESIAN_POINT('Ctrl Pts',(-17.1452095830633,-14.6513681262571,
0.));
#231285=CARTESIAN_POINT('Ctrl Pts',(-17.1452095830633,-14.6513681262571,
12.));
#231286=CARTESIAN_POINT('',(-18.8464468996588,-17.9112098770111,0.));
#231287=CARTESIAN_POINT('Ctrl Pts',(-18.8464468996588,-17.9112098770111,
0.));
#231288=CARTESIAN_POINT('Ctrl Pts',(-18.8448126709692,-17.9057348246595,
0.));
#231289=CARTESIAN_POINT('Ctrl Pts',(-18.8415402351786,-17.8947931177807,
0.));
#231290=CARTESIAN_POINT('Ctrl Pts',(-18.8366196462581,-17.8784057509356,
0.));
#231291=CARTESIAN_POINT('Ctrl Pts',(-18.8300349895974,-17.8566063174771,
0.));
#231292=CARTESIAN_POINT('Ctrl Pts',(-18.8217643886157,-17.8294410311006,
0.));
#231293=CARTESIAN_POINT('Ctrl Pts',(-18.8134540340417,-17.8023598011057,
0.));
#231294=CARTESIAN_POINT('Ctrl Pts',(-18.8051039860448,-17.7753627137853,
0.));
#231295=CARTESIAN_POINT('Ctrl Pts',(-18.7967143519419,-17.7484498996905,
0.));
#231296=CARTESIAN_POINT('Ctrl Pts',(-18.788285297605,-17.7216215409035,
0.));
#231297=CARTESIAN_POINT('Ctrl Pts',(-18.7798170641374,-17.6948778823014,
0.));
#231298=CARTESIAN_POINT('Ctrl Pts',(-18.7713099642754,-17.6682192274236,
0.));
#231299=CARTESIAN_POINT('Ctrl Pts',(-18.762764361321,-17.6416459210681,
0.));
#231300=CARTESIAN_POINT('Ctrl Pts',(-18.7541806530984,-17.6151583357012,
0.));
#231301=CARTESIAN_POINT('Ctrl Pts',(-18.7455592536687,-17.5887568561371,
0.));
#231302=CARTESIAN_POINT('Ctrl Pts',(-18.7369005764553,-17.5624418653245,
0.));
#231303=CARTESIAN_POINT('Ctrl Pts',(-18.7282050157138,-17.5362137287593,
0.));
#231304=CARTESIAN_POINT('Ctrl Pts',(-18.7194729318098,-17.5100727820876,
0.));
#231305=CARTESIAN_POINT('Ctrl Pts',(-18.7107046613912,-17.4840193397162,
0.));
#231306=CARTESIAN_POINT('Ctrl Pts',(-18.70190052503,-17.4580537012753,0.));
#231307=CARTESIAN_POINT('Ctrl Pts',(-18.6930608357409,-17.4321761588142,
0.));
#231308=CARTESIAN_POINT('Ctrl Pts',(-18.6841859073471,-17.4063870038562,
0.));
#231309=CARTESIAN_POINT('Ctrl Pts',(-18.6752760624052,-17.3806865340747,
0.));
#231310=CARTESIAN_POINT('Ctrl Pts',(-18.6663316416582,-17.3550750612443,
0.));
#231311=CARTESIAN_POINT('Ctrl Pts',(-18.6573530024033,-17.3295529098618,
0.));
#231312=CARTESIAN_POINT('Ctrl Pts',(-18.6483405141865,-17.3041204135074,
0.));
#231313=CARTESIAN_POINT('Ctrl Pts',(-18.6392945554748,-17.2787779120213,
0.));
#231314=CARTESIAN_POINT('Ctrl Pts',(-18.6302155097943,-17.2535257482187,
0.));
#231315=CARTESIAN_POINT('Ctrl Pts',(-18.6211037624038,-17.2283642650518,
0.));
#231316=CARTESIAN_POINT('Ctrl Pts',(-18.6119596959949,-17.2032938019284,
0.));
#231317=CARTESIAN_POINT('Ctrl Pts',(-18.6027836898817,-17.1783146940127,
0.));
#231318=CARTESIAN_POINT('Ctrl Pts',(-18.5935761222825,-17.1534272741643,
0.));
#231319=CARTESIAN_POINT('Ctrl Pts',(-18.5843373717247,-17.1286318741183,
0.));
#231320=CARTESIAN_POINT('Ctrl Pts',(-18.5750678188542,-17.1039288260001,
0.));
#231321=CARTESIAN_POINT('Ctrl Pts',(-18.5657678479789,-17.0793184636079,
0.));
#231322=CARTESIAN_POINT('Ctrl Pts',(-18.556437848963,-17.0548011239751,
0.));
#231323=CARTESIAN_POINT('Ctrl Pts',(-18.547078218209,-17.0303771481738,
0.));
#231324=CARTESIAN_POINT('Ctrl Pts',(-18.5376893576961,-17.0060468805097,
0.));
#231325=CARTESIAN_POINT('Ctrl Pts',(-18.5282716744197,-16.981810668038,
0.));
#231326=CARTESIAN_POINT('Ctrl Pts',(-18.5188255796659,-16.9576688599339,
0.));
#231327=CARTESIAN_POINT('Ctrl Pts',(-18.5093514883835,-16.9336218069353,
0.));
#231328=CARTESIAN_POINT('Ctrl Pts',(-18.499849818462,-16.9096698606943,
0.));
#231329=CARTESIAN_POINT('Ctrl Pts',(-18.4903209902227,-16.8858133733088,
0.));
#231330=CARTESIAN_POINT('Ctrl Pts',(-18.4807654268771,-16.8620526977171,
0.));
#231331=CARTESIAN_POINT('Ctrl Pts',(-18.4711835548623,-16.8383881879709,
0.));
#231332=CARTESIAN_POINT('Ctrl Pts',(-18.4615758042305,-16.8148201995472,
0.));
#231333=CARTESIAN_POINT('Ctrl Pts',(-18.4519426090124,-16.791349089629,
0.));
#231334=CARTESIAN_POINT('Ctrl Pts',(-18.44228440761,-16.7679752173992,0.));
#231335=CARTESIAN_POINT('Ctrl Pts',(-18.4326016431392,-16.7446989442882,
0.));
#231336=CARTESIAN_POINT('Ctrl Pts',(-18.4228947633187,-16.7215206338818,
0.));
#231337=CARTESIAN_POINT('Ctrl Pts',(-18.413164220399,-16.6984406518491,
0.));
#231338=CARTESIAN_POINT('Ctrl Pts',(-18.403410471079,-16.6754593658513,
0.));
#231339=CARTESIAN_POINT('Ctrl Pts',(-18.3936339764332,-16.6525771454513,
0.));
#231340=CARTESIAN_POINT('Ctrl Pts',(-18.3838352018327,-16.6297943620056,
0.));
#231341=CARTESIAN_POINT('Ctrl Pts',(-18.3740146168879,-16.607111388571,
0.));
#231342=CARTESIAN_POINT('Ctrl Pts',(-18.3641726955889,-16.5845286000217,
0.));
#231343=CARTESIAN_POINT('Ctrl Pts',(-18.354309916433,-16.5620463731413,
0.));
#231344=CARTESIAN_POINT('Ctrl Pts',(-18.34442676256,-16.5396650867139,0.));
#231345=CARTESIAN_POINT('Ctrl Pts',(-18.3345237218864,-16.5173851216045,
0.));
#231346=CARTESIAN_POINT('Ctrl Pts',(-18.3246012872469,-16.4952068608345,
0.));
#231347=CARTESIAN_POINT('Ctrl Pts',(-18.3146599565231,-16.4731306896441,
0.));
#231348=CARTESIAN_POINT('Ctrl Pts',(-18.304700232686,-16.4511569955233,
0.));
#231349=CARTESIAN_POINT('Ctrl Pts',(-18.294722623851,-16.4292861682379,
0.));
#231350=CARTESIAN_POINT('Ctrl Pts',(-18.2847276433309,-16.4075185998455,
0.));
#231351=CARTESIAN_POINT('Ctrl Pts',(-18.2747158096934,-16.385854684708,
0.));
#231352=CARTESIAN_POINT('Ctrl Pts',(-18.2646876468169,-16.3642948194868,
0.));
#231353=CARTESIAN_POINT('Ctrl Pts',(-18.2546436839608,-16.3428394031589,
0.));
#231354=CARTESIAN_POINT('Ctrl Pts',(-18.2445844558742,-16.3214888370987,
0.));
#231355=CARTESIAN_POINT('Ctrl Pts',(-18.2345105028982,-16.3002435251378,
0.));
#231356=CARTESIAN_POINT('Ctrl Pts',(-18.2244223710746,-16.2791038736223,
0.));
#231357=CARTESIAN_POINT('Ctrl Pts',(-18.2143206122529,-16.2580702914615,
0.));
#231358=CARTESIAN_POINT('Ctrl Pts',(-18.2042057842035,-16.2371431901638,
0.));
#231359=CARTESIAN_POINT('Ctrl Pts',(-18.1940784507229,-16.2163229838875,
0.));
#231360=CARTESIAN_POINT('Ctrl Pts',(-18.1839391817331,-16.1956100895073,
0.));
#231361=CARTESIAN_POINT('Ctrl Pts',(-18.1737885533849,-16.1750049266671,
0.));
#231362=CARTESIAN_POINT('Ctrl Pts',(-18.1636271481615,-16.154507917826,
0.));
#231363=CARTESIAN_POINT('Ctrl Pts',(-18.1534555549852,-16.1341194882988,
0.));
#231364=CARTESIAN_POINT('Ctrl Pts',(-18.1432743693235,-16.1138400662794,
0.));
#231365=CARTESIAN_POINT('Ctrl Pts',(-18.1330841933105,-16.0936700829112,
0.));
#231366=CARTESIAN_POINT('Ctrl Pts',(-18.1228856358751,-16.0736099723668,
0.));
#231367=CARTESIAN_POINT('Ctrl Pts',(-18.112679312869,-16.0536601719126,
0.));
#231368=CARTESIAN_POINT('Ctrl Pts',(-18.1024658471966,-16.0338211219693,
0.));
#231369=CARTESIAN_POINT('Ctrl Pts',(-18.0922458689462,-16.014093266161,
0.));
#231370=CARTESIAN_POINT('Ctrl Pts',(-18.0820200155236,-15.9944770513613,
0.));
#231371=CARTESIAN_POINT('Ctrl Pts',(-18.0717889317958,-15.9749729277846,
0.));
#231372=CARTESIAN_POINT('Ctrl Pts',(-18.061553270236,-15.9555813490644,
0.));
#231373=CARTESIAN_POINT('Ctrl Pts',(-18.0513136910691,-15.9363027723244,
0.));
#231374=CARTESIAN_POINT('Ctrl Pts',(-18.0410708624208,-15.9171376582436,
0.));
#231375=CARTESIAN_POINT('Ctrl Pts',(-18.0308254604636,-15.8980864711042,
0.));
#231376=CARTESIAN_POINT('Ctrl Pts',(-18.0205781695769,-15.8791496788682,
0.));
#231377=CARTESIAN_POINT('Ctrl Pts',(-18.0103296825205,-15.8603277532831,
0.));
#231378=CARTESIAN_POINT('Ctrl Pts',(-18.0000807006052,-15.8416211699679,
0.));
#231379=CARTESIAN_POINT('Ctrl Pts',(-17.9898319338664,-15.8230304084962,
0.));
#231380=CARTESIAN_POINT('Ctrl Pts',(-17.9795841012386,-15.8045559524676,
0.));
#231381=CARTESIAN_POINT('Ctrl Pts',(-17.9693379307303,-15.7861982895724,
0.));
#231382=CARTESIAN_POINT('Ctrl Pts',(-17.9590941596242,-15.7679579117077,
0.));
#231383=CARTESIAN_POINT('Ctrl Pts',(-17.9488535346781,-15.749835315086,
0.));
#231384=CARTESIAN_POINT('Ctrl Pts',(-17.9386168123262,-15.7318310003335,
0.));
#231385=CARTESIAN_POINT('Ctrl Pts',(-17.9283847588836,-15.7139454725838,
0.));
#231386=CARTESIAN_POINT('Ctrl Pts',(-17.9181581507455,-15.6961792415522,
0.));
#231387=CARTESIAN_POINT('Ctrl Pts',(-17.9079377746111,-15.678532821646,
0.));
#231388=CARTESIAN_POINT('Ctrl Pts',(-17.897724427724,-15.661006732103,0.));
#231389=CARTESIAN_POINT('Ctrl Pts',(-17.8875189181091,-15.6436014971084,
0.));
#231390=CARTESIAN_POINT('Ctrl Pts',(-17.8773220648125,-15.6263176459108,
0.));
#231391=CARTESIAN_POINT('Ctrl Pts',(-17.8671346981394,-15.609155712921,
0.));
#231392=CARTESIAN_POINT('Ctrl Pts',(-17.8569576599006,-15.5921162378192,
0.));
#231393=CARTESIAN_POINT('Ctrl Pts',(-17.8467918036987,-15.5751997657163,
0.));
#231394=CARTESIAN_POINT('Ctrl Pts',(-17.8366379952085,-15.5584068472982,
0.));
#231395=CARTESIAN_POINT('Ctrl Pts',(-17.8264971124607,-15.541738038964,
0.));
#231396=CARTESIAN_POINT('Ctrl Pts',(-17.8163700461256,-15.5251939029552,
0.));
#231397=CARTESIAN_POINT('Ctrl Pts',(-17.8062576997952,-15.5087750074718,
0.));
#231398=CARTESIAN_POINT('Ctrl Pts',(-17.7961609903148,-15.4924819268517,
0.));
#231399=CARTESIAN_POINT('Ctrl Pts',(-17.786080848122,-15.4763152417497,
0.));
#231400=CARTESIAN_POINT('Ctrl Pts',(-17.7760182175815,-15.4602755393017,
0.));
#231401=CARTESIAN_POINT('Ctrl Pts',(-17.7659740573265,-15.4443634132869,
0.));
#231402=CARTESIAN_POINT('Ctrl Pts',(-17.7559493405881,-15.4285794642668,
0.));
#231403=CARTESIAN_POINT('Ctrl Pts',(-17.7459450555812,-15.4129242997837,
0.));
#231404=CARTESIAN_POINT('Ctrl Pts',(-17.735962205915,-15.3973985345802,
0.));
#231405=CARTESIAN_POINT('Ctrl Pts',(-17.7260018109924,-15.3820027907967,
0.));
#231406=CARTESIAN_POINT('Ctrl Pts',(-17.7160649064206,-15.3667376981699,
0.));
#231407=CARTESIAN_POINT('Ctrl Pts',(-17.7061525444042,-15.351603894206,
0.));
#231408=CARTESIAN_POINT('Ctrl Pts',(-17.6962657941983,-15.3366020244066,
0.));
#231409=CARTESIAN_POINT('Ctrl Pts',(-17.6864057426052,-15.3217327425338,
0.));
#231410=CARTESIAN_POINT('Ctrl Pts',(-17.676573494456,-15.3069967108501,
0.));
#231411=CARTESIAN_POINT('Ctrl Pts',(-17.6667701731041,-15.2923946003598,
0.));
#231412=CARTESIAN_POINT('Ctrl Pts',(-17.6569969209,-15.2779270910239,0.));
#231413=CARTESIAN_POINT('Ctrl Pts',(-17.6472548997328,-15.2635948720292,
0.));
#231414=CARTESIAN_POINT('Ctrl Pts',(-17.6375452916369,-15.2493986421092,
0.));
#231415=CARTESIAN_POINT('Ctrl Pts',(-17.6278692993764,-15.2353391098366,
0.));
#231416=CARTESIAN_POINT('Ctrl Pts',(-17.6182281470468,-15.2214169939199,
0.));
#231417=CARTESIAN_POINT('Ctrl Pts',(-17.60862308065,-15.2076330234686,0.));
#231418=CARTESIAN_POINT('Ctrl Pts',(-17.5990553687599,-15.1939879383268,
0.));
#231419=CARTESIAN_POINT('Ctrl Pts',(-17.5895263032595,-15.1804824894605,
0.));
#231420=CARTESIAN_POINT('Ctrl Pts',(-17.580037200054,-15.1671174393137,
0.));
#231421=CARTESIAN_POINT('Ctrl Pts',(-17.5705893998029,-15.1538935621714,
0.));
#231422=CARTESIAN_POINT('Ctrl Pts',(-17.5611842686192,-15.1408116444876,
0.));
#231423=CARTESIAN_POINT('Ctrl Pts',(-17.5518231989117,-15.1278724853138,
0.));
#231424=CARTESIAN_POINT('Ctrl Pts',(-17.5425076102963,-15.1150768967728,
0.));
#231425=CARTESIAN_POINT('Ctrl Pts',(-17.5332389504829,-15.1024257045033,
0.));
#231426=CARTESIAN_POINT('Ctrl Pts',(-17.5240186961791,-15.0899197481082,
0.));
#231427=CARTESIAN_POINT('Ctrl Pts',(-17.5148483539687,-15.0775598815749,
0.));
#231428=CARTESIAN_POINT('Ctrl Pts',(-17.5057294613877,-15.0653469738307,
0.));
#231429=CARTESIAN_POINT('Ctrl Pts',(-17.4966635880246,-15.0532819093085,
0.));
#231430=CARTESIAN_POINT('Ctrl Pts',(-17.4876523366178,-15.0413655884993,
0.));
#231431=CARTESIAN_POINT('Ctrl Pts',(-17.4786973441417,-15.029598928488,
0.));
#231432=CARTESIAN_POINT('Ctrl Pts',(-17.4698002829357,-15.0179828635087,
0.));
#231433=CARTESIAN_POINT('Ctrl Pts',(-17.4609628621419,-15.0065183456922,
0.));
#231434=CARTESIAN_POINT('Ctrl Pts',(-17.4521868291005,-14.9952063457779,
0.));
#231435=CARTESIAN_POINT('Ctrl Pts',(-17.4434739707773,-14.9840478538357,
0.));
#231436=CARTESIAN_POINT('Ctrl Pts',(-17.4348261151395,-14.973043879945,
0.));
#231437=CARTESIAN_POINT('Ctrl Pts',(-17.4262451327088,-14.9621954549825,
0.));
#231438=CARTESIAN_POINT('Ctrl Pts',(-17.4177329382827,-14.9515036315142,
0.));
#231439=CARTESIAN_POINT('Ctrl Pts',(-17.4092914926071,-14.940969484645,
0.));
#231440=CARTESIAN_POINT('Ctrl Pts',(-17.400922804075,-14.9305941128758,
0.));
#231441=CARTESIAN_POINT('Ctrl Pts',(-17.3926289303987,-14.9203786389343,
0.));
#231442=CARTESIAN_POINT('Ctrl Pts',(-17.3844119809823,-14.9103242110057,
0.));
#231443=CARTESIAN_POINT('Ctrl Pts',(-17.3762741193075,-14.9004320039609,
0.));
#231444=CARTESIAN_POINT('Ctrl Pts',(-17.3682175653236,-14.8907032205789,
0.));
#231445=CARTESIAN_POINT('Ctrl Pts',(-17.3602445978163,-14.8811390927424,
0.));
#231446=CARTESIAN_POINT('Ctrl Pts',(-17.3523575568648,-14.8717408826958,
0.));
#231447=CARTESIAN_POINT('Ctrl Pts',(-17.3445588463477,-14.8625098843419,
0.));
#231448=CARTESIAN_POINT('Ctrl Pts',(-17.336850936485,-14.8534474245433,
0.));
#231449=CARTESIAN_POINT('Ctrl Pts',(-17.3292363662601,-14.8445548643505,
0.));
#231450=CARTESIAN_POINT('Ctrl Pts',(-17.3217177462096,-14.8358336004193,
0.));
#231451=CARTESIAN_POINT('Ctrl Pts',(-17.3142977632656,-14.8272850675375,
0.));
#231452=CARTESIAN_POINT('Ctrl Pts',(-17.3069791853705,-14.8189107410161,
0.));
#231453=CARTESIAN_POINT('Ctrl Pts',(-17.2997648661483,-14.8107121391038,
0.));
#231454=CARTESIAN_POINT('Ctrl Pts',(-17.2926577496519,-14.8026908254281,
0.));
#231455=CARTESIAN_POINT('Ctrl Pts',(-17.28566087332,-14.7948484105253,0.));
#231456=CARTESIAN_POINT('Ctrl Pts',(-17.278777370485,-14.787186553128,0.));
#231457=CARTESIAN_POINT('Ctrl Pts',(-17.2720104735192,-14.7797069617802,
0.));
#231458=CARTESIAN_POINT('Ctrl Pts',(-17.2653635155317,-14.7724113956728,
0.));
#231459=CARTESIAN_POINT('Ctrl Pts',(-17.2588399401464,-14.7653016697589,
0.));
#231460=CARTESIAN_POINT('Ctrl Pts',(-17.2524433146837,-14.7583796616617,
0.));
#231461=CARTESIAN_POINT('Ctrl Pts',(-17.2461773413289,-14.7516473175125,
0.));
#231462=CARTESIAN_POINT('Ctrl Pts',(-17.2400458713566,-14.7451066593793,
0.));
#231463=CARTESIAN_POINT('Ctrl Pts',(-17.2340529062077,-14.7387597858117,
0.));
#231464=CARTESIAN_POINT('Ctrl Pts',(-17.2282025904314,-14.7326088681163,
0.));
#231465=CARTESIAN_POINT('Ctrl Pts',(-17.2224992099666,-14.7266561494282,
0.));
#231466=CARTESIAN_POINT('Ctrl Pts',(-17.2169471814255,-14.7209039390326,
0.));
#231467=CARTESIAN_POINT('Ctrl Pts',(-17.2115510835988,-14.7153546289338,
0.));
#231468=CARTESIAN_POINT('Ctrl Pts',(-17.2063157097316,-14.7100107213586,
0.));
#231469=CARTESIAN_POINT('Ctrl Pts',(-17.2012461084268,-14.7048748502663,
0.));
#231470=CARTESIAN_POINT('Ctrl Pts',(-17.1963476411694,-14.699949811582,
0.));
#231471=CARTESIAN_POINT('Ctrl Pts',(-17.1916259308416,-14.6952385361706,
0.));
#231472=CARTESIAN_POINT('Ctrl Pts',(-17.1870867909918,-14.6907440526958,
0.));
#231473=CARTESIAN_POINT('Ctrl Pts',(-17.182736158472,-14.6864694522319,
0.));
#231474=CARTESIAN_POINT('Ctrl Pts',(-17.1785800350827,-14.6824178576167,
0.));
#231475=CARTESIAN_POINT('Ctrl Pts',(-17.1746247499057,-14.6785925615676,
0.));
#231476=CARTESIAN_POINT('Ctrl Pts',(-17.1708771619129,-14.6749971333867,
0.));
#231477=CARTESIAN_POINT('Ctrl Pts',(-17.1673449723019,-14.6716355833321,
0.));
#231478=CARTESIAN_POINT('Ctrl Pts',(-17.1640366762304,-14.6685123374424,
0.));
#231479=CARTESIAN_POINT('Ctrl Pts',(-17.1609609517369,-14.6656319165057,
0.));
#231480=CARTESIAN_POINT('Ctrl Pts',(-17.1581262646789,-14.662998728599,
0.));
#231481=CARTESIAN_POINT('Ctrl Pts',(-17.1555401986403,-14.660616716964,
0.));
#231482=CARTESIAN_POINT('Ctrl Pts',(-17.1532107762719,-14.6584900555301,
0.));
#231483=CARTESIAN_POINT('Ctrl Pts',(-17.1511476869495,-14.6566237952435,
0.));
#231484=CARTESIAN_POINT('Ctrl Pts',(-17.1493641837556,-14.6550248622813,
0.));
#231485=CARTESIAN_POINT('Ctrl Pts',(-17.1478763944909,-14.6537016966188,
0.));
#231486=CARTESIAN_POINT('Ctrl Pts',(-17.1466998098673,-14.6526624064978,
0.));
#231487=CARTESIAN_POINT('Ctrl Pts',(-17.1458462295273,-14.65191316345,0.));
#231488=CARTESIAN_POINT('Ctrl Pts',(-17.1454262858045,-14.6515481598057,
0.));
#231489=CARTESIAN_POINT('Ctrl Pts',(-17.1452600887039,-14.6514066997188,
0.));
#231490=CARTESIAN_POINT('Ctrl Pts',(-17.1452153999142,-14.651371185284,
0.));
#231491=CARTESIAN_POINT('Ctrl Pts',(-17.1452095830633,-14.6513681262571,
0.));
#231492=CARTESIAN_POINT('',(-18.8464468996588,-17.9112098770111,12.));
#231493=CARTESIAN_POINT('',(-18.8464468996588,-17.9112098770111,0.));
#231494=CARTESIAN_POINT('Ctrl Pts',(-17.1452095830633,-14.6513681262571,
12.));
#231495=CARTESIAN_POINT('Ctrl Pts',(-17.1452153999142,-14.651371185284,
12.));
#231496=CARTESIAN_POINT('Ctrl Pts',(-17.1452600887039,-14.6514066997188,
12.));
#231497=CARTESIAN_POINT('Ctrl Pts',(-17.1454262858045,-14.6515481598057,
12.));
#231498=CARTESIAN_POINT('Ctrl Pts',(-17.1458462295273,-14.65191316345,12.));
#231499=CARTESIAN_POINT('Ctrl Pts',(-17.1466998098673,-14.6526624064978,
12.));
#231500=CARTESIAN_POINT('Ctrl Pts',(-17.1478763944909,-14.6537016966188,
12.));
#231501=CARTESIAN_POINT('Ctrl Pts',(-17.1493641837556,-14.6550248622813,
12.));
#231502=CARTESIAN_POINT('Ctrl Pts',(-17.1511476869495,-14.6566237952435,
12.));
#231503=CARTESIAN_POINT('Ctrl Pts',(-17.1532107762719,-14.6584900555301,
12.));
#231504=CARTESIAN_POINT('Ctrl Pts',(-17.1555401986403,-14.660616716964,
12.));
#231505=CARTESIAN_POINT('Ctrl Pts',(-17.1581262646789,-14.662998728599,
12.));
#231506=CARTESIAN_POINT('Ctrl Pts',(-17.1609609517369,-14.6656319165057,
12.));
#231507=CARTESIAN_POINT('Ctrl Pts',(-17.1640366762304,-14.6685123374424,
12.));
#231508=CARTESIAN_POINT('Ctrl Pts',(-17.1673449723019,-14.6716355833321,
12.));
#231509=CARTESIAN_POINT('Ctrl Pts',(-17.1708771619129,-14.6749971333867,
12.));
#231510=CARTESIAN_POINT('Ctrl Pts',(-17.1746247499057,-14.6785925615676,
12.));
#231511=CARTESIAN_POINT('Ctrl Pts',(-17.1785800350827,-14.6824178576167,
12.));
#231512=CARTESIAN_POINT('Ctrl Pts',(-17.182736158472,-14.6864694522319,
12.));
#231513=CARTESIAN_POINT('Ctrl Pts',(-17.1870867909918,-14.6907440526958,
12.));
#231514=CARTESIAN_POINT('Ctrl Pts',(-17.1916259308416,-14.6952385361706,
12.));
#231515=CARTESIAN_POINT('Ctrl Pts',(-17.1963476411694,-14.699949811582,
12.));
#231516=CARTESIAN_POINT('Ctrl Pts',(-17.2012461084268,-14.7048748502663,
12.));
#231517=CARTESIAN_POINT('Ctrl Pts',(-17.2063157097316,-14.7100107213586,
12.));
#231518=CARTESIAN_POINT('Ctrl Pts',(-17.2115510835988,-14.7153546289338,
12.));
#231519=CARTESIAN_POINT('Ctrl Pts',(-17.2169471814255,-14.7209039390326,
12.));
#231520=CARTESIAN_POINT('Ctrl Pts',(-17.2224992099666,-14.7266561494282,
12.));
#231521=CARTESIAN_POINT('Ctrl Pts',(-17.2282025904314,-14.7326088681163,
12.));
#231522=CARTESIAN_POINT('Ctrl Pts',(-17.2340529062077,-14.7387597858117,
12.));
#231523=CARTESIAN_POINT('Ctrl Pts',(-17.2400458713566,-14.7451066593793,
12.));
#231524=CARTESIAN_POINT('Ctrl Pts',(-17.2461773413289,-14.7516473175125,
12.));
#231525=CARTESIAN_POINT('Ctrl Pts',(-17.2524433146837,-14.7583796616617,
12.));
#231526=CARTESIAN_POINT('Ctrl Pts',(-17.2588399401464,-14.7653016697589,
12.));
#231527=CARTESIAN_POINT('Ctrl Pts',(-17.2653635155317,-14.7724113956728,
12.));
#231528=CARTESIAN_POINT('Ctrl Pts',(-17.2720104735192,-14.7797069617802,
12.));
#231529=CARTESIAN_POINT('Ctrl Pts',(-17.278777370485,-14.787186553128,12.));
#231530=CARTESIAN_POINT('Ctrl Pts',(-17.28566087332,-14.7948484105253,12.));
#231531=CARTESIAN_POINT('Ctrl Pts',(-17.2926577496519,-14.8026908254281,
12.));
#231532=CARTESIAN_POINT('Ctrl Pts',(-17.2997648661483,-14.8107121391038,
12.));
#231533=CARTESIAN_POINT('Ctrl Pts',(-17.3069791853705,-14.8189107410161,
12.));
#231534=CARTESIAN_POINT('Ctrl Pts',(-17.3142977632656,-14.8272850675375,
12.));
#231535=CARTESIAN_POINT('Ctrl Pts',(-17.3217177462096,-14.8358336004193,
12.));
#231536=CARTESIAN_POINT('Ctrl Pts',(-17.3292363662601,-14.8445548643505,
12.));
#231537=CARTESIAN_POINT('Ctrl Pts',(-17.336850936485,-14.8534474245433,
12.));
#231538=CARTESIAN_POINT('Ctrl Pts',(-17.3445588463477,-14.8625098843419,
12.));
#231539=CARTESIAN_POINT('Ctrl Pts',(-17.3523575568648,-14.8717408826958,
12.));
#231540=CARTESIAN_POINT('Ctrl Pts',(-17.3602445978163,-14.8811390927424,
12.));
#231541=CARTESIAN_POINT('Ctrl Pts',(-17.3682175653236,-14.8907032205789,
12.));
#231542=CARTESIAN_POINT('Ctrl Pts',(-17.3762741193075,-14.9004320039609,
12.));
#231543=CARTESIAN_POINT('Ctrl Pts',(-17.3844119809823,-14.9103242110057,
12.));
#231544=CARTESIAN_POINT('Ctrl Pts',(-17.3926289303987,-14.9203786389343,
12.));
#231545=CARTESIAN_POINT('Ctrl Pts',(-17.400922804075,-14.9305941128758,
12.));
#231546=CARTESIAN_POINT('Ctrl Pts',(-17.4092914926071,-14.940969484645,
12.));
#231547=CARTESIAN_POINT('Ctrl Pts',(-17.4177329382827,-14.9515036315142,
12.));
#231548=CARTESIAN_POINT('Ctrl Pts',(-17.4262451327088,-14.9621954549825,
12.));
#231549=CARTESIAN_POINT('Ctrl Pts',(-17.4348261151395,-14.973043879945,
12.));
#231550=CARTESIAN_POINT('Ctrl Pts',(-17.4434739707773,-14.9840478538357,
12.));
#231551=CARTESIAN_POINT('Ctrl Pts',(-17.4521868291005,-14.9952063457779,
12.));
#231552=CARTESIAN_POINT('Ctrl Pts',(-17.4609628621419,-15.0065183456922,
12.));
#231553=CARTESIAN_POINT('Ctrl Pts',(-17.4698002829357,-15.0179828635087,
12.));
#231554=CARTESIAN_POINT('Ctrl Pts',(-17.4786973441417,-15.029598928488,
12.));
#231555=CARTESIAN_POINT('Ctrl Pts',(-17.4876523366178,-15.0413655884993,
12.));
#231556=CARTESIAN_POINT('Ctrl Pts',(-17.4966635880246,-15.0532819093085,
12.));
#231557=CARTESIAN_POINT('Ctrl Pts',(-17.5057294613877,-15.0653469738307,
12.));
#231558=CARTESIAN_POINT('Ctrl Pts',(-17.5148483539687,-15.0775598815749,
12.));
#231559=CARTESIAN_POINT('Ctrl Pts',(-17.5240186961791,-15.0899197481082,
12.));
#231560=CARTESIAN_POINT('Ctrl Pts',(-17.5332389504829,-15.1024257045033,
12.));
#231561=CARTESIAN_POINT('Ctrl Pts',(-17.5425076102963,-15.1150768967728,
12.));
#231562=CARTESIAN_POINT('Ctrl Pts',(-17.5518231989117,-15.1278724853138,
12.));
#231563=CARTESIAN_POINT('Ctrl Pts',(-17.5611842686192,-15.1408116444876,
12.));
#231564=CARTESIAN_POINT('Ctrl Pts',(-17.5705893998029,-15.1538935621714,
12.));
#231565=CARTESIAN_POINT('Ctrl Pts',(-17.580037200054,-15.1671174393137,
12.));
#231566=CARTESIAN_POINT('Ctrl Pts',(-17.5895263032595,-15.1804824894605,
12.));
#231567=CARTESIAN_POINT('Ctrl Pts',(-17.5990553687599,-15.1939879383268,
12.));
#231568=CARTESIAN_POINT('Ctrl Pts',(-17.60862308065,-15.2076330234686,12.));
#231569=CARTESIAN_POINT('Ctrl Pts',(-17.6182281470468,-15.2214169939199,
12.));
#231570=CARTESIAN_POINT('Ctrl Pts',(-17.6278692993764,-15.2353391098366,
12.));
#231571=CARTESIAN_POINT('Ctrl Pts',(-17.6375452916369,-15.2493986421092,
12.));
#231572=CARTESIAN_POINT('Ctrl Pts',(-17.6472548997328,-15.2635948720292,
12.));
#231573=CARTESIAN_POINT('Ctrl Pts',(-17.6569969209,-15.2779270910239,12.));
#231574=CARTESIAN_POINT('Ctrl Pts',(-17.6667701731041,-15.2923946003598,
12.));
#231575=CARTESIAN_POINT('Ctrl Pts',(-17.676573494456,-15.3069967108501,
12.));
#231576=CARTESIAN_POINT('Ctrl Pts',(-17.6864057426052,-15.3217327425338,
12.));
#231577=CARTESIAN_POINT('Ctrl Pts',(-17.6962657941983,-15.3366020244066,
12.));
#231578=CARTESIAN_POINT('Ctrl Pts',(-17.7061525444042,-15.351603894206,
12.));
#231579=CARTESIAN_POINT('Ctrl Pts',(-17.7160649064206,-15.3667376981699,
12.));
#231580=CARTESIAN_POINT('Ctrl Pts',(-17.7260018109924,-15.3820027907967,
12.));
#231581=CARTESIAN_POINT('Ctrl Pts',(-17.735962205915,-15.3973985345802,
12.));
#231582=CARTESIAN_POINT('Ctrl Pts',(-17.7459450555812,-15.4129242997837,
12.));
#231583=CARTESIAN_POINT('Ctrl Pts',(-17.7559493405881,-15.4285794642668,
12.));
#231584=CARTESIAN_POINT('Ctrl Pts',(-17.7659740573265,-15.4443634132869,
12.));
#231585=CARTESIAN_POINT('Ctrl Pts',(-17.7760182175815,-15.4602755393017,
12.));
#231586=CARTESIAN_POINT('Ctrl Pts',(-17.786080848122,-15.4763152417497,
12.));
#231587=CARTESIAN_POINT('Ctrl Pts',(-17.7961609903148,-15.4924819268517,
12.));
#231588=CARTESIAN_POINT('Ctrl Pts',(-17.8062576997952,-15.5087750074718,
12.));
#231589=CARTESIAN_POINT('Ctrl Pts',(-17.8163700461256,-15.5251939029552,
12.));
#231590=CARTESIAN_POINT('Ctrl Pts',(-17.8264971124607,-15.541738038964,
12.));
#231591=CARTESIAN_POINT('Ctrl Pts',(-17.8366379952085,-15.5584068472982,
12.));
#231592=CARTESIAN_POINT('Ctrl Pts',(-17.8467918036987,-15.5751997657163,
12.));
#231593=CARTESIAN_POINT('Ctrl Pts',(-17.8569576599006,-15.5921162378192,
12.));
#231594=CARTESIAN_POINT('Ctrl Pts',(-17.8671346981394,-15.609155712921,
12.));
#231595=CARTESIAN_POINT('Ctrl Pts',(-17.8773220648125,-15.6263176459108,
12.));
#231596=CARTESIAN_POINT('Ctrl Pts',(-17.8875189181091,-15.6436014971084,
12.));
#231597=CARTESIAN_POINT('Ctrl Pts',(-17.897724427724,-15.661006732103,12.));
#231598=CARTESIAN_POINT('Ctrl Pts',(-17.9079377746111,-15.678532821646,
12.));
#231599=CARTESIAN_POINT('Ctrl Pts',(-17.9181581507455,-15.6961792415522,
12.));
#231600=CARTESIAN_POINT('Ctrl Pts',(-17.9283847588836,-15.7139454725838,
12.));
#231601=CARTESIAN_POINT('Ctrl Pts',(-17.9386168123262,-15.7318310003335,
12.));
#231602=CARTESIAN_POINT('Ctrl Pts',(-17.9488535346781,-15.749835315086,
12.));
#231603=CARTESIAN_POINT('Ctrl Pts',(-17.9590941596242,-15.7679579117077,
12.));
#231604=CARTESIAN_POINT('Ctrl Pts',(-17.9693379307303,-15.7861982895724,
12.));
#231605=CARTESIAN_POINT('Ctrl Pts',(-17.9795841012386,-15.8045559524676,
12.));
#231606=CARTESIAN_POINT('Ctrl Pts',(-17.9898319338664,-15.8230304084962,
12.));
#231607=CARTESIAN_POINT('Ctrl Pts',(-18.0000807006052,-15.8416211699679,
12.));
#231608=CARTESIAN_POINT('Ctrl Pts',(-18.0103296825205,-15.8603277532831,
12.));
#231609=CARTESIAN_POINT('Ctrl Pts',(-18.0205781695769,-15.8791496788682,
12.));
#231610=CARTESIAN_POINT('Ctrl Pts',(-18.0308254604636,-15.8980864711042,
12.));
#231611=CARTESIAN_POINT('Ctrl Pts',(-18.0410708624208,-15.9171376582436,
12.));
#231612=CARTESIAN_POINT('Ctrl Pts',(-18.0513136910691,-15.9363027723244,
12.));
#231613=CARTESIAN_POINT('Ctrl Pts',(-18.061553270236,-15.9555813490644,
12.));
#231614=CARTESIAN_POINT('Ctrl Pts',(-18.0717889317958,-15.9749729277846,
12.));
#231615=CARTESIAN_POINT('Ctrl Pts',(-18.0820200155236,-15.9944770513613,
12.));
#231616=CARTESIAN_POINT('Ctrl Pts',(-18.0922458689462,-16.014093266161,
12.));
#231617=CARTESIAN_POINT('Ctrl Pts',(-18.1024658471966,-16.0338211219693,
12.));
#231618=CARTESIAN_POINT('Ctrl Pts',(-18.112679312869,-16.0536601719126,
12.));
#231619=CARTESIAN_POINT('Ctrl Pts',(-18.1228856358751,-16.0736099723668,
12.));
#231620=CARTESIAN_POINT('Ctrl Pts',(-18.1330841933105,-16.0936700829112,
12.));
#231621=CARTESIAN_POINT('Ctrl Pts',(-18.1432743693235,-16.1138400662794,
12.));
#231622=CARTESIAN_POINT('Ctrl Pts',(-18.1534555549852,-16.1341194882988,
12.));
#231623=CARTESIAN_POINT('Ctrl Pts',(-18.1636271481615,-16.154507917826,
12.));
#231624=CARTESIAN_POINT('Ctrl Pts',(-18.1737885533849,-16.1750049266671,
12.));
#231625=CARTESIAN_POINT('Ctrl Pts',(-18.1839391817331,-16.1956100895073,
12.));
#231626=CARTESIAN_POINT('Ctrl Pts',(-18.1940784507229,-16.2163229838875,
12.));
#231627=CARTESIAN_POINT('Ctrl Pts',(-18.2042057842035,-16.2371431901638,
12.));
#231628=CARTESIAN_POINT('Ctrl Pts',(-18.2143206122529,-16.2580702914615,
12.));
#231629=CARTESIAN_POINT('Ctrl Pts',(-18.2244223710746,-16.2791038736223,
12.));
#231630=CARTESIAN_POINT('Ctrl Pts',(-18.2345105028982,-16.3002435251378,
12.));
#231631=CARTESIAN_POINT('Ctrl Pts',(-18.2445844558742,-16.3214888370987,
12.));
#231632=CARTESIAN_POINT('Ctrl Pts',(-18.2546436839608,-16.3428394031589,
12.));
#231633=CARTESIAN_POINT('Ctrl Pts',(-18.2646876468169,-16.3642948194868,
12.));
#231634=CARTESIAN_POINT('Ctrl Pts',(-18.2747158096934,-16.385854684708,
12.));
#231635=CARTESIAN_POINT('Ctrl Pts',(-18.2847276433309,-16.4075185998455,
12.));
#231636=CARTESIAN_POINT('Ctrl Pts',(-18.294722623851,-16.4292861682379,
12.));
#231637=CARTESIAN_POINT('Ctrl Pts',(-18.304700232686,-16.4511569955233,
12.));
#231638=CARTESIAN_POINT('Ctrl Pts',(-18.3146599565231,-16.4731306896441,
12.));
#231639=CARTESIAN_POINT('Ctrl Pts',(-18.3246012872469,-16.4952068608345,
12.));
#231640=CARTESIAN_POINT('Ctrl Pts',(-18.3345237218864,-16.5173851216045,
12.));
#231641=CARTESIAN_POINT('Ctrl Pts',(-18.34442676256,-16.5396650867139,12.));
#231642=CARTESIAN_POINT('Ctrl Pts',(-18.354309916433,-16.5620463731413,
12.));
#231643=CARTESIAN_POINT('Ctrl Pts',(-18.3641726955889,-16.5845286000217,
12.));
#231644=CARTESIAN_POINT('Ctrl Pts',(-18.3740146168879,-16.607111388571,
12.));
#231645=CARTESIAN_POINT('Ctrl Pts',(-18.3838352018327,-16.6297943620056,
12.));
#231646=CARTESIAN_POINT('Ctrl Pts',(-18.3936339764332,-16.6525771454513,
12.));
#231647=CARTESIAN_POINT('Ctrl Pts',(-18.403410471079,-16.6754593658513,
12.));
#231648=CARTESIAN_POINT('Ctrl Pts',(-18.413164220399,-16.6984406518491,
12.));
#231649=CARTESIAN_POINT('Ctrl Pts',(-18.4228947633187,-16.7215206338818,
12.));
#231650=CARTESIAN_POINT('Ctrl Pts',(-18.4326016431392,-16.7446989442882,
12.));
#231651=CARTESIAN_POINT('Ctrl Pts',(-18.44228440761,-16.7679752173992,12.));
#231652=CARTESIAN_POINT('Ctrl Pts',(-18.4519426090124,-16.791349089629,
12.));
#231653=CARTESIAN_POINT('Ctrl Pts',(-18.4615758042305,-16.8148201995472,
12.));
#231654=CARTESIAN_POINT('Ctrl Pts',(-18.4711835548623,-16.8383881879709,
12.));
#231655=CARTESIAN_POINT('Ctrl Pts',(-18.4807654268771,-16.8620526977171,
12.));
#231656=CARTESIAN_POINT('Ctrl Pts',(-18.4903209902227,-16.8858133733088,
12.));
#231657=CARTESIAN_POINT('Ctrl Pts',(-18.499849818462,-16.9096698606943,
12.));
#231658=CARTESIAN_POINT('Ctrl Pts',(-18.5093514883835,-16.9336218069353,
12.));
#231659=CARTESIAN_POINT('Ctrl Pts',(-18.5188255796659,-16.9576688599339,
12.));
#231660=CARTESIAN_POINT('Ctrl Pts',(-18.5282716744197,-16.981810668038,
12.));
#231661=CARTESIAN_POINT('Ctrl Pts',(-18.5376893576961,-17.0060468805097,
12.));
#231662=CARTESIAN_POINT('Ctrl Pts',(-18.547078218209,-17.0303771481738,
12.));
#231663=CARTESIAN_POINT('Ctrl Pts',(-18.556437848963,-17.0548011239751,
12.));
#231664=CARTESIAN_POINT('Ctrl Pts',(-18.5657678479789,-17.0793184636079,
12.));
#231665=CARTESIAN_POINT('Ctrl Pts',(-18.5750678188542,-17.1039288260001,
12.));
#231666=CARTESIAN_POINT('Ctrl Pts',(-18.5843373717247,-17.1286318741183,
12.));
#231667=CARTESIAN_POINT('Ctrl Pts',(-18.5935761222825,-17.1534272741643,
12.));
#231668=CARTESIAN_POINT('Ctrl Pts',(-18.6027836898817,-17.1783146940127,
12.));
#231669=CARTESIAN_POINT('Ctrl Pts',(-18.6119596959949,-17.2032938019284,
12.));
#231670=CARTESIAN_POINT('Ctrl Pts',(-18.6211037624038,-17.2283642650518,
12.));
#231671=CARTESIAN_POINT('Ctrl Pts',(-18.6302155097943,-17.2535257482187,
12.));
#231672=CARTESIAN_POINT('Ctrl Pts',(-18.6392945554748,-17.2787779120213,
12.));
#231673=CARTESIAN_POINT('Ctrl Pts',(-18.6483405141865,-17.3041204135074,
12.));
#231674=CARTESIAN_POINT('Ctrl Pts',(-18.6573530024033,-17.3295529098618,
12.));
#231675=CARTESIAN_POINT('Ctrl Pts',(-18.6663316416582,-17.3550750612443,
12.));
#231676=CARTESIAN_POINT('Ctrl Pts',(-18.6752760624052,-17.3806865340747,
12.));
#231677=CARTESIAN_POINT('Ctrl Pts',(-18.6841859073471,-17.4063870038562,
12.));
#231678=CARTESIAN_POINT('Ctrl Pts',(-18.6930608357409,-17.4321761588142,
12.));
#231679=CARTESIAN_POINT('Ctrl Pts',(-18.70190052503,-17.4580537012753,12.));
#231680=CARTESIAN_POINT('Ctrl Pts',(-18.7107046613912,-17.4840193397162,
12.));
#231681=CARTESIAN_POINT('Ctrl Pts',(-18.7194729318098,-17.5100727820876,
12.));
#231682=CARTESIAN_POINT('Ctrl Pts',(-18.7282050157138,-17.5362137287593,
12.));
#231683=CARTESIAN_POINT('Ctrl Pts',(-18.7369005764553,-17.5624418653245,
12.));
#231684=CARTESIAN_POINT('Ctrl Pts',(-18.7455592536687,-17.5887568561371,
12.));
#231685=CARTESIAN_POINT('Ctrl Pts',(-18.7541806530984,-17.6151583357012,
12.));
#231686=CARTESIAN_POINT('Ctrl Pts',(-18.762764361321,-17.6416459210681,
12.));
#231687=CARTESIAN_POINT('Ctrl Pts',(-18.7713099642754,-17.6682192274236,
12.));
#231688=CARTESIAN_POINT('Ctrl Pts',(-18.7798170641374,-17.6948778823014,
12.));
#231689=CARTESIAN_POINT('Ctrl Pts',(-18.788285297605,-17.7216215409035,
12.));
#231690=CARTESIAN_POINT('Ctrl Pts',(-18.7967143519419,-17.7484498996905,
12.));
#231691=CARTESIAN_POINT('Ctrl Pts',(-18.8051039860448,-17.7753627137853,
12.));
#231692=CARTESIAN_POINT('Ctrl Pts',(-18.8134540340417,-17.8023598011057,
12.));
#231693=CARTESIAN_POINT('Ctrl Pts',(-18.8217643886157,-17.8294410311006,
12.));
#231694=CARTESIAN_POINT('Ctrl Pts',(-18.8300349895974,-17.8566063174771,
12.));
#231695=CARTESIAN_POINT('Ctrl Pts',(-18.8366196462581,-17.8784057509356,
12.));
#231696=CARTESIAN_POINT('Ctrl Pts',(-18.8415402351786,-17.8947931177807,
12.));
#231697=CARTESIAN_POINT('Ctrl Pts',(-18.8448126709692,-17.9057348246595,
12.));
#231698=CARTESIAN_POINT('Ctrl Pts',(-18.8464468996588,-17.9112098770111,
12.));
#231699=CARTESIAN_POINT('Ctrl Pts',(-18.5896416359912,-12.7689476255363,
0.));
#231700=CARTESIAN_POINT('Ctrl Pts',(-18.5896416359912,-12.7689476255363,
12.));
#231701=CARTESIAN_POINT('Ctrl Pts',(-18.5896460962964,-12.7689524524483,
0.));
#231702=CARTESIAN_POINT('Ctrl Pts',(-18.5896460962964,-12.7689524524483,
12.));
#231703=CARTESIAN_POINT('Ctrl Pts',(-18.5896919669165,-12.768986426692,
0.));
#231704=CARTESIAN_POINT('Ctrl Pts',(-18.5896919669165,-12.768986426692,
12.));
#231705=CARTESIAN_POINT('Ctrl Pts',(-18.589871621843,-12.769110348199,0.));
#231706=CARTESIAN_POINT('Ctrl Pts',(-18.589871621843,-12.769110348199,12.));
#231707=CARTESIAN_POINT('Ctrl Pts',(-18.5903328777227,-12.7694215127919,
0.));
#231708=CARTESIAN_POINT('Ctrl Pts',(-18.5903328777227,-12.7694215127919,
12.));
#231709=CARTESIAN_POINT('Ctrl Pts',(-18.5912775137806,-12.7700520897173,
0.));
#231710=CARTESIAN_POINT('Ctrl Pts',(-18.5912775137806,-12.7700520897173,
12.));
#231711=CARTESIAN_POINT('Ctrl Pts',(-18.5925859134579,-12.7709195951156,
0.));
#231712=CARTESIAN_POINT('Ctrl Pts',(-18.5925859134579,-12.7709195951156,
12.));
#231713=CARTESIAN_POINT('Ctrl Pts',(-18.5942490615407,-12.7720142287172,
0.));
#231714=CARTESIAN_POINT('Ctrl Pts',(-18.5942490615407,-12.7720142287172,
12.));
#231715=CARTESIAN_POINT('Ctrl Pts',(-18.5962551167772,-12.7733231262108,
0.));
#231716=CARTESIAN_POINT('Ctrl Pts',(-18.5962551167772,-12.7733231262108,
12.));
#231717=CARTESIAN_POINT('Ctrl Pts',(-18.598591752595,-12.7748328937638,
0.));
#231718=CARTESIAN_POINT('Ctrl Pts',(-18.598591752595,-12.7748328937638,
12.));
#231719=CARTESIAN_POINT('Ctrl Pts',(-18.6012488486709,-12.7765325225081,
0.));
#231720=CARTESIAN_POINT('Ctrl Pts',(-18.6012488486709,-12.7765325225081,
12.));
#231721=CARTESIAN_POINT('Ctrl Pts',(-18.6042190183704,-12.7784139605066,
0.));
#231722=CARTESIAN_POINT('Ctrl Pts',(-18.6042190183704,-12.7784139605066,
12.));
#231723=CARTESIAN_POINT('Ctrl Pts',(-18.6074961535723,-12.7804705387658,
0.));
#231724=CARTESIAN_POINT('Ctrl Pts',(-18.6074961535723,-12.7804705387658,
12.));
#231725=CARTESIAN_POINT('Ctrl Pts',(-18.6110744826219,-12.7826959526925,
0.));
#231726=CARTESIAN_POINT('Ctrl Pts',(-18.6110744826219,-12.7826959526925,
12.));
#231727=CARTESIAN_POINT('Ctrl Pts',(-18.6149475565188,-12.7850831657901,
0.));
#231728=CARTESIAN_POINT('Ctrl Pts',(-18.6149475565188,-12.7850831657901,
12.));
#231729=CARTESIAN_POINT('Ctrl Pts',(-18.6191087624752,-12.7876249657834,
0.));
#231730=CARTESIAN_POINT('Ctrl Pts',(-18.6191087624752,-12.7876249657834,
12.));
#231731=CARTESIAN_POINT('Ctrl Pts',(-18.6235516265575,-12.7903142925234,
0.));
#231732=CARTESIAN_POINT('Ctrl Pts',(-18.6235516265575,-12.7903142925234,
12.));
#231733=CARTESIAN_POINT('Ctrl Pts',(-18.6282702819371,-12.7931447451555,
0.));
#231734=CARTESIAN_POINT('Ctrl Pts',(-18.6282702819371,-12.7931447451555,
12.));
#231735=CARTESIAN_POINT('Ctrl Pts',(-18.6332595057006,-12.7961106222251,
0.));
#231736=CARTESIAN_POINT('Ctrl Pts',(-18.6332595057006,-12.7961106222251,
12.));
#231737=CARTESIAN_POINT('Ctrl Pts',(-18.63851447924,-12.7992066625264,0.));
#231738=CARTESIAN_POINT('Ctrl Pts',(-18.63851447924,-12.7992066625264,12.));
#231739=CARTESIAN_POINT('Ctrl Pts',(-18.6440306327456,-12.8024278770152,
0.));
#231740=CARTESIAN_POINT('Ctrl Pts',(-18.6440306327456,-12.8024278770152,
12.));
#231741=CARTESIAN_POINT('Ctrl Pts',(-18.6498034438987,-12.805769331162,
0.));
#231742=CARTESIAN_POINT('Ctrl Pts',(-18.6498034438987,-12.805769331162,
12.));
#231743=CARTESIAN_POINT('Ctrl Pts',(-18.6558284825773,-12.8092261933858,
0.));
#231744=CARTESIAN_POINT('Ctrl Pts',(-18.6558284825773,-12.8092261933858,
12.));
#231745=CARTESIAN_POINT('Ctrl Pts',(-18.6621014624746,-12.8127937909631,
0.));
#231746=CARTESIAN_POINT('Ctrl Pts',(-18.6621014624746,-12.8127937909631,
12.));
#231747=CARTESIAN_POINT('Ctrl Pts',(-18.6686182952799,-12.8164676687362,
0.));
#231748=CARTESIAN_POINT('Ctrl Pts',(-18.6686182952799,-12.8164676687362,
12.));
#231749=CARTESIAN_POINT('Ctrl Pts',(-18.6753751301092,-12.8202436318474,
0.));
#231750=CARTESIAN_POINT('Ctrl Pts',(-18.6753751301092,-12.8202436318474,
12.));
#231751=CARTESIAN_POINT('Ctrl Pts',(-18.6823683094139,-12.8241176980017,
0.));
#231752=CARTESIAN_POINT('Ctrl Pts',(-18.6823683094139,-12.8241176980017,
12.));
#231753=CARTESIAN_POINT('Ctrl Pts',(-18.6895943376171,-12.8280860635231,
0.));
#231754=CARTESIAN_POINT('Ctrl Pts',(-18.6895943376171,-12.8280860635231,
12.));
#231755=CARTESIAN_POINT('Ctrl Pts',(-18.6970498410172,-12.8321450599789,
0.));
#231756=CARTESIAN_POINT('Ctrl Pts',(-18.6970498410172,-12.8321450599789,
12.));
#231757=CARTESIAN_POINT('Ctrl Pts',(-18.7047315436294,-12.8362911280361,
0.));
#231758=CARTESIAN_POINT('Ctrl Pts',(-18.7047315436294,-12.8362911280361,
12.));
#231759=CARTESIAN_POINT('Ctrl Pts',(-18.7126362754445,-12.8405208263431,
0.));
#231760=CARTESIAN_POINT('Ctrl Pts',(-18.7126362754445,-12.8405208263431,
12.));
#231761=CARTESIAN_POINT('Ctrl Pts',(-18.7207609737702,-12.8448308329494,
0.));
#231762=CARTESIAN_POINT('Ctrl Pts',(-18.7207609737702,-12.8448308329494,
12.));
#231763=CARTESIAN_POINT('Ctrl Pts',(-18.7291026886554,-12.8492179511591,
0.));
#231764=CARTESIAN_POINT('Ctrl Pts',(-18.7291026886554,-12.8492179511591,
12.));
#231765=CARTESIAN_POINT('Ctrl Pts',(-18.7376585820854,-12.8536791086316,
0.));
#231766=CARTESIAN_POINT('Ctrl Pts',(-18.7376585820854,-12.8536791086316,
12.));
#231767=CARTESIAN_POINT('Ctrl Pts',(-18.7464259171251,-12.8582113455646,
0.));
#231768=CARTESIAN_POINT('Ctrl Pts',(-18.7464259171251,-12.8582113455646,
12.));
#231769=CARTESIAN_POINT('Ctrl Pts',(-18.7554020493887,-12.8628118054171,
0.));
#231770=CARTESIAN_POINT('Ctrl Pts',(-18.7554020493887,-12.8628118054171,
12.));
#231771=CARTESIAN_POINT('Ctrl Pts',(-18.7645844169564,-12.8674777239653,
0.));
#231772=CARTESIAN_POINT('Ctrl Pts',(-18.7645844169564,-12.8674777239653,
12.));
#231773=CARTESIAN_POINT('Ctrl Pts',(-18.7739705329022,-12.872206421181,
0.));
#231774=CARTESIAN_POINT('Ctrl Pts',(-18.7739705329022,-12.872206421181,
12.));
#231775=CARTESIAN_POINT('Ctrl Pts',(-18.7835579840477,-12.8769952998095,
0.));
#231776=CARTESIAN_POINT('Ctrl Pts',(-18.7835579840477,-12.8769952998095,
12.));
#231777=CARTESIAN_POINT('Ctrl Pts',(-18.7933444285868,-12.8818418427475,
0.));
#231778=CARTESIAN_POINT('Ctrl Pts',(-18.7933444285868,-12.8818418427475,
12.));
#231779=CARTESIAN_POINT('Ctrl Pts',(-18.8033275941943,-12.8867436109546,
0.));
#231780=CARTESIAN_POINT('Ctrl Pts',(-18.8033275941943,-12.8867436109546,
12.));
#231781=CARTESIAN_POINT('Ctrl Pts',(-18.813505275782,-12.8916982409935,
0.));
#231782=CARTESIAN_POINT('Ctrl Pts',(-18.813505275782,-12.8916982409935,
12.));
#231783=CARTESIAN_POINT('Ctrl Pts',(-18.8238753319129,-12.8967034410755,
0.));
#231784=CARTESIAN_POINT('Ctrl Pts',(-18.8238753319129,-12.8967034410755,
12.));
#231785=CARTESIAN_POINT('Ctrl Pts',(-18.834435681259,-12.9017569871738,
0.));
#231786=CARTESIAN_POINT('Ctrl Pts',(-18.834435681259,-12.9017569871738,
12.));
#231787=CARTESIAN_POINT('Ctrl Pts',(-18.8451842990984,-12.9068567191854,
0.));
#231788=CARTESIAN_POINT('Ctrl Pts',(-18.8451842990984,-12.9068567191854,
12.));
#231789=CARTESIAN_POINT('Ctrl Pts',(-18.8561192136198,-12.9120005369063,
0.));
#231790=CARTESIAN_POINT('Ctrl Pts',(-18.8561192136198,-12.9120005369063,
12.));
#231791=CARTESIAN_POINT('Ctrl Pts',(-18.8672385038326,-12.9171863977045,
0.));
#231792=CARTESIAN_POINT('Ctrl Pts',(-18.8672385038326,-12.9171863977045,
12.));
#231793=CARTESIAN_POINT('Ctrl Pts',(-18.8785402977527,-12.9224123144982,
0.));
#231794=CARTESIAN_POINT('Ctrl Pts',(-18.8785402977527,-12.9224123144982,
12.));
#231795=CARTESIAN_POINT('Ctrl Pts',(-18.8900227704889,-12.9276763536373,
0.));
#231796=CARTESIAN_POINT('Ctrl Pts',(-18.8900227704889,-12.9276763536373,
12.));
#231797=CARTESIAN_POINT('Ctrl Pts',(-18.9016841423403,-12.9329766328185,
0.));
#231798=CARTESIAN_POINT('Ctrl Pts',(-18.9016841423403,-12.9329766328185,
12.));
#231799=CARTESIAN_POINT('Ctrl Pts',(-18.9135226769465,-12.9383113190375,
0.));
#231800=CARTESIAN_POINT('Ctrl Pts',(-18.9135226769465,-12.9383113190375,
12.));
#231801=CARTESIAN_POINT('Ctrl Pts',(-18.9255366795195,-12.9436786266105,
0.));
#231802=CARTESIAN_POINT('Ctrl Pts',(-18.9255366795195,-12.9436786266105,
12.));
#231803=CARTESIAN_POINT('Ctrl Pts',(-18.9377244950435,-12.9490768151821,
0.));
#231804=CARTESIAN_POINT('Ctrl Pts',(-18.9377244950435,-12.9490768151821,
12.));
#231805=CARTESIAN_POINT('Ctrl Pts',(-18.9500845064715,-12.9545041877377,
0.));
#231806=CARTESIAN_POINT('Ctrl Pts',(-18.9500845064715,-12.9545041877377,
12.));
#231807=CARTESIAN_POINT('Ctrl Pts',(-18.9626151329229,-12.9599590886319,
0.));
#231808=CARTESIAN_POINT('Ctrl Pts',(-18.9626151329229,-12.9599590886319,
12.));
#231809=CARTESIAN_POINT('Ctrl Pts',(-18.9753148284475,-12.9654399021869,
0.));
#231810=CARTESIAN_POINT('Ctrl Pts',(-18.9753148284475,-12.9654399021869,
12.));
#231811=CARTESIAN_POINT('Ctrl Pts',(-18.9881820807586,-12.9709450512747,
0.));
#231812=CARTESIAN_POINT('Ctrl Pts',(-18.9881820807586,-12.9709450512747,
12.));
#231813=CARTESIAN_POINT('Ctrl Pts',(-19.0012154099791,-12.9764729959205,
0.));
#231814=CARTESIAN_POINT('Ctrl Pts',(-19.0012154099791,-12.9764729959205,
12.));
#231815=CARTESIAN_POINT('Ctrl Pts',(-19.0144133673348,-12.9820222318716,
0.));
#231816=CARTESIAN_POINT('Ctrl Pts',(-19.0144133673348,-12.9820222318716,
12.));
#231817=CARTESIAN_POINT('Ctrl Pts',(-19.0277745339908,-12.9875912893003,
0.));
#231818=CARTESIAN_POINT('Ctrl Pts',(-19.0277745339908,-12.9875912893003,
12.));
#231819=CARTESIAN_POINT('Ctrl Pts',(-19.0412975200398,-12.9931787316515,
0.));
#231820=CARTESIAN_POINT('Ctrl Pts',(-19.0412975200398,-12.9931787316515,
12.));
#231821=CARTESIAN_POINT('Ctrl Pts',(-19.0549809634355,-12.9987831544502,
0.));
#231822=CARTESIAN_POINT('Ctrl Pts',(-19.0549809634355,-12.9987831544502,
12.));
#231823=CARTESIAN_POINT('Ctrl Pts',(-19.0688235289437,-13.0044031841381,
0.));
#231824=CARTESIAN_POINT('Ctrl Pts',(-19.0688235289437,-13.0044031841381,
12.));
#231825=CARTESIAN_POINT('Ctrl Pts',(-19.0828239070482,-13.0100374768785,
0.));
#231826=CARTESIAN_POINT('Ctrl Pts',(-19.0828239070482,-13.0100374768785,
12.));
#231827=CARTESIAN_POINT('Ctrl Pts',(-19.0969808131226,-13.0156847176093,
0.));
#231828=CARTESIAN_POINT('Ctrl Pts',(-19.0969808131226,-13.0156847176093,
12.));
#231829=CARTESIAN_POINT('Ctrl Pts',(-19.1112929866308,-13.0213436191326,
0.));
#231830=CARTESIAN_POINT('Ctrl Pts',(-19.1112929866308,-13.0213436191326,
12.));
#231831=CARTESIAN_POINT('Ctrl Pts',(-19.1257591903099,-13.0270129211976,
0.));
#231832=CARTESIAN_POINT('Ctrl Pts',(-19.1257591903099,-13.0270129211976,
12.));
#231833=CARTESIAN_POINT('Ctrl Pts',(-19.1403782093389,-13.0326913895841,
0.));
#231834=CARTESIAN_POINT('Ctrl Pts',(-19.1403782093389,-13.0326913895841,
12.));
#231835=CARTESIAN_POINT('Ctrl Pts',(-19.1551488505233,-13.0383778152072,
0.));
#231836=CARTESIAN_POINT('Ctrl Pts',(-19.1551488505233,-13.0383778152072,
12.));
#231837=CARTESIAN_POINT('Ctrl Pts',(-19.1700699416625,-13.0440710133775,
0.));
#231838=CARTESIAN_POINT('Ctrl Pts',(-19.1700699416625,-13.0440710133775,
12.));
#231839=CARTESIAN_POINT('Ctrl Pts',(-19.1851403308825,-13.0497698230442,
0.));
#231840=CARTESIAN_POINT('Ctrl Pts',(-19.1851403308825,-13.0497698230442,
12.));
#231841=CARTESIAN_POINT('Ctrl Pts',(-19.2003588859771,-13.0554731060537,
0.));
#231842=CARTESIAN_POINT('Ctrl Pts',(-19.2003588859771,-13.0554731060537,
12.));
#231843=CARTESIAN_POINT('Ctrl Pts',(-19.2157244937141,-13.0611797463913,
0.));
#231844=CARTESIAN_POINT('Ctrl Pts',(-19.2157244937141,-13.0611797463913,
12.));
#231845=CARTESIAN_POINT('Ctrl Pts',(-19.2312360592031,-13.0668886494791,
0.));
#231846=CARTESIAN_POINT('Ctrl Pts',(-19.2312360592031,-13.0668886494791,
12.));
#231847=CARTESIAN_POINT('Ctrl Pts',(-19.2468925053988,-13.0725987415856,
0.));
#231848=CARTESIAN_POINT('Ctrl Pts',(-19.2468925053988,-13.0725987415856,
12.));
#231849=CARTESIAN_POINT('Ctrl Pts',(-19.2626927725596,-13.0783089692118,
0.));
#231850=CARTESIAN_POINT('Ctrl Pts',(-19.2626927725596,-13.0783089692118,
12.));
#231851=CARTESIAN_POINT('Ctrl Pts',(-19.2786358177198,-13.0840182984949,
0.));
#231852=CARTESIAN_POINT('Ctrl Pts',(-19.2786358177198,-13.0840182984949,
12.));
#231853=CARTESIAN_POINT('Ctrl Pts',(-19.2947206141246,-13.0897257145969,
0.));
#231854=CARTESIAN_POINT('Ctrl Pts',(-19.2947206141246,-13.0897257145969,
12.));
#231855=CARTESIAN_POINT('Ctrl Pts',(-19.3109461507358,-13.095430221148,
0.));
#231856=CARTESIAN_POINT('Ctrl Pts',(-19.3109461507358,-13.095430221148,
12.));
#231857=CARTESIAN_POINT('Ctrl Pts',(-19.3273114318268,-13.1011308397592,
0.));
#231858=CARTESIAN_POINT('Ctrl Pts',(-19.3273114318268,-13.1011308397592,
12.));
#231859=CARTESIAN_POINT('Ctrl Pts',(-19.3438154765395,-13.1068266095186,
0.));
#231860=CARTESIAN_POINT('Ctrl Pts',(-19.3438154765395,-13.1068266095186,
12.));
#231861=CARTESIAN_POINT('Ctrl Pts',(-19.3604573184516,-13.1125165865021,
0.));
#231862=CARTESIAN_POINT('Ctrl Pts',(-19.3604573184516,-13.1125165865021,
12.));
#231863=CARTESIAN_POINT('Ctrl Pts',(-19.3772360051093,-13.118199843271,
0.));
#231864=CARTESIAN_POINT('Ctrl Pts',(-19.3772360051093,-13.118199843271,
12.));
#231865=CARTESIAN_POINT('Ctrl Pts',(-19.3941505976267,-13.1238754684177,
0.));
#231866=CARTESIAN_POINT('Ctrl Pts',(-19.3941505976267,-13.1238754684177,
12.));
#231867=CARTESIAN_POINT('Ctrl Pts',(-19.4112001703561,-13.1295425661635,
0.));
#231868=CARTESIAN_POINT('Ctrl Pts',(-19.4112001703561,-13.1295425661635,
12.));
#231869=CARTESIAN_POINT('Ctrl Pts',(-19.4283838105265,-13.1352002559439,
0.));
#231870=CARTESIAN_POINT('Ctrl Pts',(-19.4283838105265,-13.1352002559439,
12.));
#231871=CARTESIAN_POINT('Ctrl Pts',(-19.4457006178875,-13.140847672006,
0.));
#231872=CARTESIAN_POINT('Ctrl Pts',(-19.4457006178875,-13.140847672006,
12.));
#231873=CARTESIAN_POINT('Ctrl Pts',(-19.463149704325,-13.1464839629966,
0.));
#231874=CARTESIAN_POINT('Ctrl Pts',(-19.463149704325,-13.1464839629966,
12.));
#231875=CARTESIAN_POINT('Ctrl Pts',(-19.4807301935256,-13.1521082915846,
0.));
#231876=CARTESIAN_POINT('Ctrl Pts',(-19.4807301935256,-13.1521082915846,
12.));
#231877=CARTESIAN_POINT('Ctrl Pts',(-19.498441220707,-13.1577198341238,
0.));
#231878=CARTESIAN_POINT('Ctrl Pts',(-19.498441220707,-13.1577198341238,
12.));
#231879=CARTESIAN_POINT('Ctrl Pts',(-19.5162819323207,-13.1633177803097,
0.));
#231880=CARTESIAN_POINT('Ctrl Pts',(-19.5162819323207,-13.1633177803097,
12.));
#231881=CARTESIAN_POINT('Ctrl Pts',(-19.5342514857564,-13.1689013328432,
0.));
#231882=CARTESIAN_POINT('Ctrl Pts',(-19.5342514857564,-13.1689013328432,
12.));
#231883=CARTESIAN_POINT('Ctrl Pts',(-19.5523490490254,-13.1744697070918,
0.));
#231884=CARTESIAN_POINT('Ctrl Pts',(-19.5523490490254,-13.1744697070918,
12.));
#231885=CARTESIAN_POINT('Ctrl Pts',(-19.5705738004682,-13.1800221307682,
0.));
#231886=CARTESIAN_POINT('Ctrl Pts',(-19.5705738004682,-13.1800221307682,
12.));
#231887=CARTESIAN_POINT('Ctrl Pts',(-19.5889249285352,-13.1855578436479,
0.));
#231888=CARTESIAN_POINT('Ctrl Pts',(-19.5889249285352,-13.1855578436479,
12.));
#231889=CARTESIAN_POINT('Ctrl Pts',(-19.6074016315421,-13.1910760972818,
0.));
#231890=CARTESIAN_POINT('Ctrl Pts',(-19.6074016315421,-13.1910760972818,
12.));
#231891=CARTESIAN_POINT('Ctrl Pts',(-19.6260031174244,-13.196576154715,
0.));
#231892=CARTESIAN_POINT('Ctrl Pts',(-19.6260031174244,-13.196576154715,
12.));
#231893=CARTESIAN_POINT('Ctrl Pts',(-19.6447286034764,-13.202057290206,
0.));
#231894=CARTESIAN_POINT('Ctrl Pts',(-19.6447286034764,-13.202057290206,
12.));
#231895=CARTESIAN_POINT('Ctrl Pts',(-19.6635773160924,-13.2075187889522,
0.));
#231896=CARTESIAN_POINT('Ctrl Pts',(-19.6635773160924,-13.2075187889522,
12.));
#231897=CARTESIAN_POINT('Ctrl Pts',(-19.6825484905812,-13.2129599468478,
0.));
#231898=CARTESIAN_POINT('Ctrl Pts',(-19.6825484905812,-13.2129599468478,
12.));
#231899=CARTESIAN_POINT('Ctrl Pts',(-19.7016413709678,-13.2183800702431,
0.));
#231900=CARTESIAN_POINT('Ctrl Pts',(-19.7016413709678,-13.2183800702431,
12.));
#231901=CARTESIAN_POINT('Ctrl Pts',(-19.7208552097867,-13.2237784757065,
0.));
#231902=CARTESIAN_POINT('Ctrl Pts',(-19.7208552097867,-13.2237784757065,
12.));
#231903=CARTESIAN_POINT('Ctrl Pts',(-19.7401892678701,-13.2291544897902,
0.));
#231904=CARTESIAN_POINT('Ctrl Pts',(-19.7401892678701,-13.2291544897902,
12.));
#231905=CARTESIAN_POINT('Ctrl Pts',(-19.7596428141176,-13.2345074487968,
0.));
#231906=CARTESIAN_POINT('Ctrl Pts',(-19.7596428141176,-13.2345074487968,
12.));
#231907=CARTESIAN_POINT('Ctrl Pts',(-19.7792151253297,-13.239836698568,
0.));
#231908=CARTESIAN_POINT('Ctrl Pts',(-19.7792151253297,-13.239836698568,
12.));
#231909=CARTESIAN_POINT('Ctrl Pts',(-19.7989054860501,-13.2451415942809,
0.));
#231910=CARTESIAN_POINT('Ctrl Pts',(-19.7989054860501,-13.2451415942809,
12.));
#231911=CARTESIAN_POINT('Ctrl Pts',(-19.8187131883919,-13.2504215002458,
0.));
#231912=CARTESIAN_POINT('Ctrl Pts',(-19.8187131883919,-13.2504215002458,
12.));
#231913=CARTESIAN_POINT('Ctrl Pts',(-19.8386375318632,-13.2556757897085,
0.));
#231914=CARTESIAN_POINT('Ctrl Pts',(-19.8386375318632,-13.2556757897085,
12.));
#231915=CARTESIAN_POINT('Ctrl Pts',(-19.8586778231711,-13.2609038446525,
0.));
#231916=CARTESIAN_POINT('Ctrl Pts',(-19.8586778231711,-13.2609038446525,
12.));
#231917=CARTESIAN_POINT('Ctrl Pts',(-19.8788333760571,-13.2661050556128,
0.));
#231918=CARTESIAN_POINT('Ctrl Pts',(-19.8788333760571,-13.2661050556128,
12.));
#231919=CARTESIAN_POINT('Ctrl Pts',(-19.8991035111739,-13.2712788215015,
0.));
#231920=CARTESIAN_POINT('Ctrl Pts',(-19.8991035111739,-13.2712788215015,
12.));
#231921=CARTESIAN_POINT('Ctrl Pts',(-19.9194875559419,-13.2764245494354,
0.));
#231922=CARTESIAN_POINT('Ctrl Pts',(-19.9194875559419,-13.2764245494354,
12.));
#231923=CARTESIAN_POINT('Ctrl Pts',(-19.9399848444019,-13.2815416545663,
0.));
#231924=CARTESIAN_POINT('Ctrl Pts',(-19.9399848444019,-13.2815416545663,
12.));
#231925=CARTESIAN_POINT('Ctrl Pts',(-19.9605947170589,-13.2866295599152,
0.));
#231926=CARTESIAN_POINT('Ctrl Pts',(-19.9605947170589,-13.2866295599152,
12.));
#231927=CARTESIAN_POINT('Ctrl Pts',(-19.9813165207174,-13.2916876962098,
0.));
#231928=CARTESIAN_POINT('Ctrl Pts',(-19.9813165207174,-13.2916876962098,
12.));
#231929=CARTESIAN_POINT('Ctrl Pts',(-20.0021496083742,-13.296715501731,
0.));
#231930=CARTESIAN_POINT('Ctrl Pts',(-20.0021496083742,-13.296715501731,
12.));
#231931=CARTESIAN_POINT('Ctrl Pts',(-20.023093339104,-13.3017124221639,
0.));
#231932=CARTESIAN_POINT('Ctrl Pts',(-20.023093339104,-13.3017124221639,
12.));
#231933=CARTESIAN_POINT('Ctrl Pts',(-20.0441470779345,-13.3066779104515,
0.));
#231934=CARTESIAN_POINT('Ctrl Pts',(-20.0441470779345,-13.3066779104515,
12.));
#231935=CARTESIAN_POINT('Ctrl Pts',(-20.0653101957188,-13.3116114266514,
0.));
#231936=CARTESIAN_POINT('Ctrl Pts',(-20.0653101957188,-13.3116114266514,
12.));
#231937=CARTESIAN_POINT('Ctrl Pts',(-20.0865820689883,-13.3165124377963,
0.));
#231938=CARTESIAN_POINT('Ctrl Pts',(-20.0865820689883,-13.3165124377963,
12.));
#231939=CARTESIAN_POINT('Ctrl Pts',(-20.1079620798377,-13.3213804177588,
0.));
#231940=CARTESIAN_POINT('Ctrl Pts',(-20.1079620798377,-13.3213804177588,
12.));
#231941=CARTESIAN_POINT('Ctrl Pts',(-20.1294496158405,-13.3262148471228,
0.));
#231942=CARTESIAN_POINT('Ctrl Pts',(-20.1294496158405,-13.3262148471228,
12.));
#231943=CARTESIAN_POINT('Ctrl Pts',(-20.1510440699477,-13.3310152130565,
0.));
#231944=CARTESIAN_POINT('Ctrl Pts',(-20.1510440699477,-13.3310152130565,
12.));
#231945=CARTESIAN_POINT('Ctrl Pts',(-20.1727448403818,-13.3357810091903,
0.));
#231946=CARTESIAN_POINT('Ctrl Pts',(-20.1727448403818,-13.3357810091903,
12.));
#231947=CARTESIAN_POINT('Ctrl Pts',(-20.1945513305233,-13.3405117354969,
0.));
#231948=CARTESIAN_POINT('Ctrl Pts',(-20.1945513305233,-13.3405117354969,
12.));
#231949=CARTESIAN_POINT('Ctrl Pts',(-20.2164629487855,-13.3452068981763,
0.));
#231950=CARTESIAN_POINT('Ctrl Pts',(-20.2164629487855,-13.3452068981763,
12.));
#231951=CARTESIAN_POINT('Ctrl Pts',(-20.2384791085354,-13.3498660095382,
0.));
#231952=CARTESIAN_POINT('Ctrl Pts',(-20.2384791085354,-13.3498660095382,
12.));
#231953=CARTESIAN_POINT('Ctrl Pts',(-20.2605992280117,-13.3544885878886,
0.));
#231954=CARTESIAN_POINT('Ctrl Pts',(-20.2605992280117,-13.3544885878886,
12.));
#231955=CARTESIAN_POINT('Ctrl Pts',(-20.2828227302337,-13.3590741574194,
0.));
#231956=CARTESIAN_POINT('Ctrl Pts',(-20.2828227302337,-13.3590741574194,
12.));
#231957=CARTESIAN_POINT('Ctrl Pts',(-20.3051490429049,-13.3636222481017,
0.));
#231958=CARTESIAN_POINT('Ctrl Pts',(-20.3051490429049,-13.3636222481017,
12.));
#231959=CARTESIAN_POINT('Ctrl Pts',(-20.3275775983032,-13.3681323955828,
0.));
#231960=CARTESIAN_POINT('Ctrl Pts',(-20.3275775983032,-13.3681323955828,
12.));
#231961=CARTESIAN_POINT('Ctrl Pts',(-20.3501078331818,-13.3726041410869,
0.));
#231962=CARTESIAN_POINT('Ctrl Pts',(-20.3501078331818,-13.3726041410869,
12.));
#231963=CARTESIAN_POINT('Ctrl Pts',(-20.3727391887187,-13.377037031319,
0.));
#231964=CARTESIAN_POINT('Ctrl Pts',(-20.3727391887187,-13.377037031319,
12.));
#231965=CARTESIAN_POINT('Ctrl Pts',(-20.3954711104505,-13.3814306183721,
0.));
#231966=CARTESIAN_POINT('Ctrl Pts',(-20.3954711104505,-13.3814306183721,
12.));
#231967=CARTESIAN_POINT('Ctrl Pts',(-20.4183030482002,-13.3857844596387,
0.));
#231968=CARTESIAN_POINT('Ctrl Pts',(-20.4183030482002,-13.3857844596387,
12.));
#231969=CARTESIAN_POINT('Ctrl Pts',(-20.4412344560007,-13.3900981177254,
0.));
#231970=CARTESIAN_POINT('Ctrl Pts',(-20.4412344560007,-13.3900981177254,
12.));
#231971=CARTESIAN_POINT('Ctrl Pts',(-20.4642647920038,-13.3943711603739,
0.));
#231972=CARTESIAN_POINT('Ctrl Pts',(-20.4642647920038,-13.3943711603739,
12.));
#231973=CARTESIAN_POINT('Ctrl Pts',(-20.4873935184041,-13.3986031603716,
0.));
#231974=CARTESIAN_POINT('Ctrl Pts',(-20.4873935184041,-13.3986031603716,
12.));
#231975=CARTESIAN_POINT('Ctrl Pts',(-20.5106201013755,-13.4027936954529,
0.));
#231976=CARTESIAN_POINT('Ctrl Pts',(-20.5106201013755,-13.4027936954529,
12.));
#231977=CARTESIAN_POINT('Ctrl Pts',(-20.5339440109958,-13.4069423482076,
0.));
#231978=CARTESIAN_POINT('Ctrl Pts',(-20.5339440109958,-13.4069423482076,
12.));
#231979=CARTESIAN_POINT('Ctrl Pts',(-20.557364721164,-13.4110487059912,
0.));
#231980=CARTESIAN_POINT('Ctrl Pts',(-20.557364721164,-13.4110487059912,
12.));
#231981=CARTESIAN_POINT('Ctrl Pts',(-20.5808817095155,-13.4151123608411,
0.));
#231982=CARTESIAN_POINT('Ctrl Pts',(-20.5808817095155,-13.4151123608411,
12.));
#231983=CARTESIAN_POINT('Ctrl Pts',(-20.6044944573151,-13.4191329093932,
0.));
#231984=CARTESIAN_POINT('Ctrl Pts',(-20.6044944573151,-13.4191329093932,
12.));
#231985=CARTESIAN_POINT('Ctrl Pts',(-20.6282024494234,-13.4231099528178,
0.));
#231986=CARTESIAN_POINT('Ctrl Pts',(-20.6282024494234,-13.4231099528178,
12.));
#231987=CARTESIAN_POINT('Ctrl Pts',(-20.6520051742868,-13.427043096765,
0.));
#231988=CARTESIAN_POINT('Ctrl Pts',(-20.6520051742868,-13.427043096765,
12.));
#231989=CARTESIAN_POINT('Ctrl Pts',(-20.6759021239102,-13.4309319513119,
0.));
#231990=CARTESIAN_POINT('Ctrl Pts',(-20.6759021239102,-13.4309319513119,
12.));
#231991=CARTESIAN_POINT('Ctrl Pts',(-20.6998927938288,-13.4347761309154,
0.));
#231992=CARTESIAN_POINT('Ctrl Pts',(-20.6998927938288,-13.4347761309154,
12.));
#231993=CARTESIAN_POINT('Ctrl Pts',(-20.7239766830675,-13.4385752543663,
0.));
#231994=CARTESIAN_POINT('Ctrl Pts',(-20.7239766830675,-13.4385752543663,
12.));
#231995=CARTESIAN_POINT('Ctrl Pts',(-20.7481532941014,-13.4423289447561,
0.));
#231996=CARTESIAN_POINT('Ctrl Pts',(-20.7481532941014,-13.4423289447561,
12.));
#231997=CARTESIAN_POINT('Ctrl Pts',(-20.7724221327609,-13.4460368293689,
0.));
#231998=CARTESIAN_POINT('Ctrl Pts',(-20.7724221327609,-13.4460368293689,
12.));
#231999=CARTESIAN_POINT('Ctrl Pts',(-20.7967827081228,-13.4496985395637,
0.));
#232000=CARTESIAN_POINT('Ctrl Pts',(-20.7967827081228,-13.4496985395637,
12.));
#232001=CARTESIAN_POINT('Ctrl Pts',(-20.821234532398,-13.4533137106667,
0.));
#232002=CARTESIAN_POINT('Ctrl Pts',(-20.821234532398,-13.4533137106667,
12.));
#232003=CARTESIAN_POINT('Ctrl Pts',(-20.8457771208083,-13.4568819818631,
0.));
#232004=CARTESIAN_POINT('Ctrl Pts',(-20.8457771208083,-13.4568819818631,
12.));
#232005=CARTESIAN_POINT('Ctrl Pts',(-20.8704099914641,-13.4604029960983,
0.));
#232006=CARTESIAN_POINT('Ctrl Pts',(-20.8704099914641,-13.4604029960983,
12.));
#232007=CARTESIAN_POINT('Ctrl Pts',(-20.8951326652158,-13.4638763999725,
0.));
#232008=CARTESIAN_POINT('Ctrl Pts',(-20.8951326652158,-13.4638763999725,
12.));
#232009=CARTESIAN_POINT('Ctrl Pts',(-20.9199446657583,-13.4673018437717,
0.));
#232010=CARTESIAN_POINT('Ctrl Pts',(-20.9199446657583,-13.4673018437717,
12.));
#232011=CARTESIAN_POINT('Ctrl Pts',(-20.9448455197557,-13.4706789815166,
0.));
#232012=CARTESIAN_POINT('Ctrl Pts',(-20.9448455197557,-13.4706789815166,
12.));
#232013=CARTESIAN_POINT('Ctrl Pts',(-20.9698347569477,-13.4740074710086,
0.));
#232014=CARTESIAN_POINT('Ctrl Pts',(-20.9698347569477,-13.4740074710086,
12.));
#232015=CARTESIAN_POINT('Ctrl Pts',(-20.9949119102592,-13.4772869738879,
0.));
#232016=CARTESIAN_POINT('Ctrl Pts',(-20.9949119102592,-13.4772869738879,
12.));
#232017=CARTESIAN_POINT('Ctrl Pts',(-21.0200765158884,-13.4805171556822,
0.));
#232018=CARTESIAN_POINT('Ctrl Pts',(-21.0200765158884,-13.4805171556822,
12.));
#232019=CARTESIAN_POINT('Ctrl Pts',(-21.0453281134245,-13.4836976858912,
0.));
#232020=CARTESIAN_POINT('Ctrl Pts',(-21.0453281134245,-13.4836976858912,
12.));
#232021=CARTESIAN_POINT('Ctrl Pts',(-21.0706662455199,-13.4868282377191,
0.));
#232022=CARTESIAN_POINT('Ctrl Pts',(-21.0706662455199,-13.4868282377191,
12.));
#232023=CARTESIAN_POINT('Ctrl Pts',(-21.0960904575046,-13.4899084877717,
0.));
#232024=CARTESIAN_POINT('Ctrl Pts',(-21.0960904575046,-13.4899084877717,
12.));
#232025=CARTESIAN_POINT('Ctrl Pts',(-21.1216002970207,-13.4929381157778,
0.));
#232026=CARTESIAN_POINT('Ctrl Pts',(-21.1216002970207,-13.4929381157778,
12.));
#232027=CARTESIAN_POINT('Ctrl Pts',(-21.1471953136209,-13.4959168042934,
0.));
#232028=CARTESIAN_POINT('Ctrl Pts',(-21.1471953136209,-13.4959168042934,
12.));
#232029=CARTESIAN_POINT('Ctrl Pts',(-21.1728750584175,-13.4988442384491,
0.));
#232030=CARTESIAN_POINT('Ctrl Pts',(-21.1728750584175,-13.4988442384491,
12.));
#232031=CARTESIAN_POINT('Ctrl Pts',(-21.1986390835828,-13.5017201056088,
0.));
#232032=CARTESIAN_POINT('Ctrl Pts',(-21.1986390835828,-13.5017201056088,
12.));
#232033=CARTESIAN_POINT('Ctrl Pts',(-21.2244869429332,-13.5045440957404,
0.));
#232034=CARTESIAN_POINT('Ctrl Pts',(-21.2244869429332,-13.5045440957404,
12.));
#232035=CARTESIAN_POINT('Ctrl Pts',(-21.250418192743,-13.5073159019452,
0.));
#232036=CARTESIAN_POINT('Ctrl Pts',(-21.250418192743,-13.5073159019452,
12.));
#232037=CARTESIAN_POINT('Ctrl Pts',(-21.2764323924442,-13.5100352209205,
0.));
#232038=CARTESIAN_POINT('Ctrl Pts',(-21.2764323924442,-13.5100352209205,
12.));
#232039=CARTESIAN_POINT('Ctrl Pts',(-21.3025291054235,-13.5127017534971,
0.));
#232040=CARTESIAN_POINT('Ctrl Pts',(-21.3025291054235,-13.5127017534971,
12.));
#232041=CARTESIAN_POINT('Ctrl Pts',(-21.3287078996341,-13.5153152050555,
0.));
#232042=CARTESIAN_POINT('Ctrl Pts',(-21.3287078996341,-13.5153152050555,
12.));
#232043=CARTESIAN_POINT('Ctrl Pts',(-21.3549683486222,-13.5178752862466,
0.));
#232044=CARTESIAN_POINT('Ctrl Pts',(-21.3549683486222,-13.5178752862466,
12.));
#232045=CARTESIAN_POINT('Ctrl Pts',(-21.3813100304973,-13.5203817122504,
0.));
#232046=CARTESIAN_POINT('Ctrl Pts',(-21.3813100304973,-13.5203817122504,
12.));
#232047=CARTESIAN_POINT('Ctrl Pts',(-21.4077325259324,-13.5228342013516,
0.));
#232048=CARTESIAN_POINT('Ctrl Pts',(-21.4077325259324,-13.5228342013516,
12.));
#232049=CARTESIAN_POINT('Ctrl Pts',(-21.4342354165259,-13.5252324737802,
0.));
#232050=CARTESIAN_POINT('Ctrl Pts',(-21.4342354165259,-13.5252324737802,
12.));
#232051=CARTESIAN_POINT('Ctrl Pts',(-21.4608182828697,-13.5275762503555,
0.));
#232052=CARTESIAN_POINT('Ctrl Pts',(-21.4608182828697,-13.5275762503555,
12.));
#232053=CARTESIAN_POINT('Ctrl Pts',(-21.4874807030468,-13.5298652514355,
0.));
#232054=CARTESIAN_POINT('Ctrl Pts',(-21.4874807030468,-13.5298652514355,
12.));
#232055=CARTESIAN_POINT('Ctrl Pts',(-21.5142222501666,-13.5320991952138,
0.));
#232056=CARTESIAN_POINT('Ctrl Pts',(-21.5142222501666,-13.5320991952138,
12.));
#232057=CARTESIAN_POINT('Ctrl Pts',(-21.5410424932503,-13.5342777983215,
0.));
#232058=CARTESIAN_POINT('Ctrl Pts',(-21.5410424932503,-13.5342777983215,
12.));
#232059=CARTESIAN_POINT('Ctrl Pts',(-21.5679410019001,-13.536400779028,
0.));
#232060=CARTESIAN_POINT('Ctrl Pts',(-21.5679410019001,-13.536400779028,
12.));
#232061=CARTESIAN_POINT('Ctrl Pts',(-21.5949173499013,-13.5384678597195,
0.));
#232062=CARTESIAN_POINT('Ctrl Pts',(-21.5949173499013,-13.5384678597195,
12.));
#232063=CARTESIAN_POINT('Ctrl Pts',(-21.6219711193946,-13.5404787697792,
0.));
#232064=CARTESIAN_POINT('Ctrl Pts',(-21.6219711193946,-13.5404787697792,
12.));
#232065=CARTESIAN_POINT('Ctrl Pts',(-21.6491019044648,-13.5424332480699,
0.));
#232066=CARTESIAN_POINT('Ctrl Pts',(-21.6491019044648,-13.5424332480699,
12.));
#232067=CARTESIAN_POINT('Ctrl Pts',(-21.6763093157699,-13.5443310461526,
0.));
#232068=CARTESIAN_POINT('Ctrl Pts',(-21.6763093157699,-13.5443310461526,
12.));
#232069=CARTESIAN_POINT('Ctrl Pts',(-21.7035929822955,-13.5461719295048,
0.));
#232070=CARTESIAN_POINT('Ctrl Pts',(-21.7035929822955,-13.5461719295048,
12.));
#232071=CARTESIAN_POINT('Ctrl Pts',(-21.7309525412281,-13.5479556704481,
0.));
#232072=CARTESIAN_POINT('Ctrl Pts',(-21.7309525412281,-13.5479556704481,
12.));
#232073=CARTESIAN_POINT('Ctrl Pts',(-21.7583876294554,-13.5496820422211,
0.));
#232074=CARTESIAN_POINT('Ctrl Pts',(-21.7583876294554,-13.5496820422211,
12.));
#232075=CARTESIAN_POINT('Ctrl Pts',(-21.7858978745865,-13.551350812725,
0.));
#232076=CARTESIAN_POINT('Ctrl Pts',(-21.7858978745865,-13.551350812725,
12.));
#232077=CARTESIAN_POINT('Ctrl Pts',(-21.8134828857967,-13.5529617381573,
0.));
#232078=CARTESIAN_POINT('Ctrl Pts',(-21.8134828857967,-13.5529617381573,
12.));
#232079=CARTESIAN_POINT('Ctrl Pts',(-21.8411422456075,-13.5545145573031,
0.));
#232080=CARTESIAN_POINT('Ctrl Pts',(-21.8411422456075,-13.5545145573031,
12.));
#232081=CARTESIAN_POINT('Ctrl Pts',(-21.8688754989365,-13.5560089839385,
0.));
#232082=CARTESIAN_POINT('Ctrl Pts',(-21.8688754989365,-13.5560089839385,
12.));
#232083=CARTESIAN_POINT('Ctrl Pts',(-21.8966821688824,-13.5574447178424,
0.));
#232084=CARTESIAN_POINT('Ctrl Pts',(-21.8966821688824,-13.5574447178424,
12.));
#232085=CARTESIAN_POINT('Ctrl Pts',(-21.9245617765769,-13.5588214586604,
0.));
#232086=CARTESIAN_POINT('Ctrl Pts',(-21.9245617765769,-13.5588214586604,
12.));
#232087=CARTESIAN_POINT('Ctrl Pts',(-21.9525138592813,-13.5601389185257,
0.));
#232088=CARTESIAN_POINT('Ctrl Pts',(-21.9525138592813,-13.5601389185257,
12.));
#232089=CARTESIAN_POINT('Ctrl Pts',(-21.9805379899168,-13.5613968357561,
0.));
#232090=CARTESIAN_POINT('Ctrl Pts',(-21.9805379899168,-13.5613968357561,
12.));
#232091=CARTESIAN_POINT('Ctrl Pts',(-22.0086337943449,-13.5625949868333,
0.));
#232092=CARTESIAN_POINT('Ctrl Pts',(-22.0086337943449,-13.5625949868333,
12.));
#232093=CARTESIAN_POINT('Ctrl Pts',(-22.0368009736295,-13.5637332022473,
0.));
#232094=CARTESIAN_POINT('Ctrl Pts',(-22.0368009736295,-13.5637332022473,
12.));
#232095=CARTESIAN_POINT('Ctrl Pts',(-22.0650393089609,-13.5648113689033,
0.));
#232096=CARTESIAN_POINT('Ctrl Pts',(-22.0650393089609,-13.5648113689033,
12.));
#232097=CARTESIAN_POINT('Ctrl Pts',(-22.0933486464593,-13.5658294169284,
0.));
#232098=CARTESIAN_POINT('Ctrl Pts',(-22.0933486464593,-13.5658294169284,
12.));
#232099=CARTESIAN_POINT('Ctrl Pts',(-22.1217288871975,-13.5667873105359,
0.));
#232100=CARTESIAN_POINT('Ctrl Pts',(-22.1217288871975,-13.5667873105359,
12.));
#232101=CARTESIAN_POINT('Ctrl Pts',(-22.1444897575194,-13.5675054919061,
0.));
#232102=CARTESIAN_POINT('Ctrl Pts',(-22.1444897575194,-13.5675054919061,
12.));
#232103=CARTESIAN_POINT('Ctrl Pts',(-22.1615922805008,-13.5680170531805,
0.));
#232104=CARTESIAN_POINT('Ctrl Pts',(-22.1615922805008,-13.5680170531805,
12.));
#232105=CARTESIAN_POINT('Ctrl Pts',(-22.1730081264608,-13.5683460612942,
0.));
#232106=CARTESIAN_POINT('Ctrl Pts',(-22.1730081264608,-13.5683460612942,
12.));
#232107=CARTESIAN_POINT('Ctrl Pts',(-22.1787195904339,-13.5685075571671,
0.));
#232108=CARTESIAN_POINT('Ctrl Pts',(-22.1787195904339,-13.5685075571671,
12.));
#232109=CARTESIAN_POINT('',(-22.1787195904339,-13.5685075571671,0.));
#232110=CARTESIAN_POINT('Ctrl Pts',(-18.5896416359912,-12.7689476255363,
0.));
#232111=CARTESIAN_POINT('Ctrl Pts',(-18.5896460962964,-12.7689524524483,
0.));
#232112=CARTESIAN_POINT('Ctrl Pts',(-18.5896919669165,-12.768986426692,
0.));
#232113=CARTESIAN_POINT('Ctrl Pts',(-18.589871621843,-12.769110348199,0.));
#232114=CARTESIAN_POINT('Ctrl Pts',(-18.5903328777227,-12.7694215127919,
0.));
#232115=CARTESIAN_POINT('Ctrl Pts',(-18.5912775137806,-12.7700520897173,
0.));
#232116=CARTESIAN_POINT('Ctrl Pts',(-18.5925859134579,-12.7709195951156,
0.));
#232117=CARTESIAN_POINT('Ctrl Pts',(-18.5942490615407,-12.7720142287172,
0.));
#232118=CARTESIAN_POINT('Ctrl Pts',(-18.5962551167772,-12.7733231262108,
0.));
#232119=CARTESIAN_POINT('Ctrl Pts',(-18.598591752595,-12.7748328937638,
0.));
#232120=CARTESIAN_POINT('Ctrl Pts',(-18.6012488486709,-12.7765325225081,
0.));
#232121=CARTESIAN_POINT('Ctrl Pts',(-18.6042190183704,-12.7784139605066,
0.));
#232122=CARTESIAN_POINT('Ctrl Pts',(-18.6074961535723,-12.7804705387658,
0.));
#232123=CARTESIAN_POINT('Ctrl Pts',(-18.6110744826219,-12.7826959526925,
0.));
#232124=CARTESIAN_POINT('Ctrl Pts',(-18.6149475565188,-12.7850831657901,
0.));
#232125=CARTESIAN_POINT('Ctrl Pts',(-18.6191087624752,-12.7876249657834,
0.));
#232126=CARTESIAN_POINT('Ctrl Pts',(-18.6235516265575,-12.7903142925234,
0.));
#232127=CARTESIAN_POINT('Ctrl Pts',(-18.6282702819371,-12.7931447451555,
0.));
#232128=CARTESIAN_POINT('Ctrl Pts',(-18.6332595057006,-12.7961106222251,
0.));
#232129=CARTESIAN_POINT('Ctrl Pts',(-18.63851447924,-12.7992066625264,0.));
#232130=CARTESIAN_POINT('Ctrl Pts',(-18.6440306327456,-12.8024278770152,
0.));
#232131=CARTESIAN_POINT('Ctrl Pts',(-18.6498034438987,-12.805769331162,
0.));
#232132=CARTESIAN_POINT('Ctrl Pts',(-18.6558284825773,-12.8092261933858,
0.));
#232133=CARTESIAN_POINT('Ctrl Pts',(-18.6621014624746,-12.8127937909631,
0.));
#232134=CARTESIAN_POINT('Ctrl Pts',(-18.6686182952799,-12.8164676687362,
0.));
#232135=CARTESIAN_POINT('Ctrl Pts',(-18.6753751301092,-12.8202436318474,
0.));
#232136=CARTESIAN_POINT('Ctrl Pts',(-18.6823683094139,-12.8241176980017,
0.));
#232137=CARTESIAN_POINT('Ctrl Pts',(-18.6895943376171,-12.8280860635231,
0.));
#232138=CARTESIAN_POINT('Ctrl Pts',(-18.6970498410172,-12.8321450599789,
0.));
#232139=CARTESIAN_POINT('Ctrl Pts',(-18.7047315436294,-12.8362911280361,
0.));
#232140=CARTESIAN_POINT('Ctrl Pts',(-18.7126362754445,-12.8405208263431,
0.));
#232141=CARTESIAN_POINT('Ctrl Pts',(-18.7207609737702,-12.8448308329494,
0.));
#232142=CARTESIAN_POINT('Ctrl Pts',(-18.7291026886554,-12.8492179511591,
0.));
#232143=CARTESIAN_POINT('Ctrl Pts',(-18.7376585820854,-12.8536791086316,
0.));
#232144=CARTESIAN_POINT('Ctrl Pts',(-18.7464259171251,-12.8582113455646,
0.));
#232145=CARTESIAN_POINT('Ctrl Pts',(-18.7554020493887,-12.8628118054171,
0.));
#232146=CARTESIAN_POINT('Ctrl Pts',(-18.7645844169564,-12.8674777239653,
0.));
#232147=CARTESIAN_POINT('Ctrl Pts',(-18.7739705329022,-12.872206421181,
0.));
#232148=CARTESIAN_POINT('Ctrl Pts',(-18.7835579840477,-12.8769952998095,
0.));
#232149=CARTESIAN_POINT('Ctrl Pts',(-18.7933444285868,-12.8818418427475,
0.));
#232150=CARTESIAN_POINT('Ctrl Pts',(-18.8033275941943,-12.8867436109546,
0.));
#232151=CARTESIAN_POINT('Ctrl Pts',(-18.813505275782,-12.8916982409935,
0.));
#232152=CARTESIAN_POINT('Ctrl Pts',(-18.8238753319129,-12.8967034410755,
0.));
#232153=CARTESIAN_POINT('Ctrl Pts',(-18.834435681259,-12.9017569871738,
0.));
#232154=CARTESIAN_POINT('Ctrl Pts',(-18.8451842990984,-12.9068567191854,
0.));
#232155=CARTESIAN_POINT('Ctrl Pts',(-18.8561192136198,-12.9120005369063,
0.));
#232156=CARTESIAN_POINT('Ctrl Pts',(-18.8672385038326,-12.9171863977045,
0.));
#232157=CARTESIAN_POINT('Ctrl Pts',(-18.8785402977527,-12.9224123144982,
0.));
#232158=CARTESIAN_POINT('Ctrl Pts',(-18.8900227704889,-12.9276763536373,
0.));
#232159=CARTESIAN_POINT('Ctrl Pts',(-18.9016841423403,-12.9329766328185,
0.));
#232160=CARTESIAN_POINT('Ctrl Pts',(-18.9135226769465,-12.9383113190375,
0.));
#232161=CARTESIAN_POINT('Ctrl Pts',(-18.9255366795195,-12.9436786266105,
0.));
#232162=CARTESIAN_POINT('Ctrl Pts',(-18.9377244950435,-12.9490768151821,
0.));
#232163=CARTESIAN_POINT('Ctrl Pts',(-18.9500845064715,-12.9545041877377,
0.));
#232164=CARTESIAN_POINT('Ctrl Pts',(-18.9626151329229,-12.9599590886319,
0.));
#232165=CARTESIAN_POINT('Ctrl Pts',(-18.9753148284475,-12.9654399021869,
0.));
#232166=CARTESIAN_POINT('Ctrl Pts',(-18.9881820807586,-12.9709450512747,
0.));
#232167=CARTESIAN_POINT('Ctrl Pts',(-19.0012154099791,-12.9764729959205,
0.));
#232168=CARTESIAN_POINT('Ctrl Pts',(-19.0144133673348,-12.9820222318716,
0.));
#232169=CARTESIAN_POINT('Ctrl Pts',(-19.0277745339908,-12.9875912893003,
0.));
#232170=CARTESIAN_POINT('Ctrl Pts',(-19.0412975200398,-12.9931787316515,
0.));
#232171=CARTESIAN_POINT('Ctrl Pts',(-19.0549809634355,-12.9987831544502,
0.));
#232172=CARTESIAN_POINT('Ctrl Pts',(-19.0688235289437,-13.0044031841381,
0.));
#232173=CARTESIAN_POINT('Ctrl Pts',(-19.0828239070482,-13.0100374768785,
0.));
#232174=CARTESIAN_POINT('Ctrl Pts',(-19.0969808131226,-13.0156847176093,
0.));
#232175=CARTESIAN_POINT('Ctrl Pts',(-19.1112929866308,-13.0213436191326,
0.));
#232176=CARTESIAN_POINT('Ctrl Pts',(-19.1257591903099,-13.0270129211976,
0.));
#232177=CARTESIAN_POINT('Ctrl Pts',(-19.1403782093389,-13.0326913895841,
0.));
#232178=CARTESIAN_POINT('Ctrl Pts',(-19.1551488505233,-13.0383778152072,
0.));
#232179=CARTESIAN_POINT('Ctrl Pts',(-19.1700699416625,-13.0440710133775,
0.));
#232180=CARTESIAN_POINT('Ctrl Pts',(-19.1851403308825,-13.0497698230442,
0.));
#232181=CARTESIAN_POINT('Ctrl Pts',(-19.2003588859771,-13.0554731060537,
0.));
#232182=CARTESIAN_POINT('Ctrl Pts',(-19.2157244937141,-13.0611797463913,
0.));
#232183=CARTESIAN_POINT('Ctrl Pts',(-19.2312360592031,-13.0668886494791,
0.));
#232184=CARTESIAN_POINT('Ctrl Pts',(-19.2468925053988,-13.0725987415856,
0.));
#232185=CARTESIAN_POINT('Ctrl Pts',(-19.2626927725596,-13.0783089692118,
0.));
#232186=CARTESIAN_POINT('Ctrl Pts',(-19.2786358177198,-13.0840182984949,
0.));
#232187=CARTESIAN_POINT('Ctrl Pts',(-19.2947206141246,-13.0897257145969,
0.));
#232188=CARTESIAN_POINT('Ctrl Pts',(-19.3109461507358,-13.095430221148,
0.));
#232189=CARTESIAN_POINT('Ctrl Pts',(-19.3273114318268,-13.1011308397592,
0.));
#232190=CARTESIAN_POINT('Ctrl Pts',(-19.3438154765395,-13.1068266095186,
0.));
#232191=CARTESIAN_POINT('Ctrl Pts',(-19.3604573184516,-13.1125165865021,
0.));
#232192=CARTESIAN_POINT('Ctrl Pts',(-19.3772360051093,-13.118199843271,
0.));
#232193=CARTESIAN_POINT('Ctrl Pts',(-19.3941505976267,-13.1238754684177,
0.));
#232194=CARTESIAN_POINT('Ctrl Pts',(-19.4112001703561,-13.1295425661635,
0.));
#232195=CARTESIAN_POINT('Ctrl Pts',(-19.4283838105265,-13.1352002559439,
0.));
#232196=CARTESIAN_POINT('Ctrl Pts',(-19.4457006178875,-13.140847672006,
0.));
#232197=CARTESIAN_POINT('Ctrl Pts',(-19.463149704325,-13.1464839629966,
0.));
#232198=CARTESIAN_POINT('Ctrl Pts',(-19.4807301935256,-13.1521082915846,
0.));
#232199=CARTESIAN_POINT('Ctrl Pts',(-19.498441220707,-13.1577198341238,
0.));
#232200=CARTESIAN_POINT('Ctrl Pts',(-19.5162819323207,-13.1633177803097,
0.));
#232201=CARTESIAN_POINT('Ctrl Pts',(-19.5342514857564,-13.1689013328432,
0.));
#232202=CARTESIAN_POINT('Ctrl Pts',(-19.5523490490254,-13.1744697070918,
0.));
#232203=CARTESIAN_POINT('Ctrl Pts',(-19.5705738004682,-13.1800221307682,
0.));
#232204=CARTESIAN_POINT('Ctrl Pts',(-19.5889249285352,-13.1855578436479,
0.));
#232205=CARTESIAN_POINT('Ctrl Pts',(-19.6074016315421,-13.1910760972818,
0.));
#232206=CARTESIAN_POINT('Ctrl Pts',(-19.6260031174244,-13.196576154715,
0.));
#232207=CARTESIAN_POINT('Ctrl Pts',(-19.6447286034764,-13.202057290206,
0.));
#232208=CARTESIAN_POINT('Ctrl Pts',(-19.6635773160924,-13.2075187889522,
0.));
#232209=CARTESIAN_POINT('Ctrl Pts',(-19.6825484905812,-13.2129599468478,
0.));
#232210=CARTESIAN_POINT('Ctrl Pts',(-19.7016413709678,-13.2183800702431,
0.));
#232211=CARTESIAN_POINT('Ctrl Pts',(-19.7208552097867,-13.2237784757065,
0.));
#232212=CARTESIAN_POINT('Ctrl Pts',(-19.7401892678701,-13.2291544897902,
0.));
#232213=CARTESIAN_POINT('Ctrl Pts',(-19.7596428141176,-13.2345074487968,
0.));
#232214=CARTESIAN_POINT('Ctrl Pts',(-19.7792151253297,-13.239836698568,
0.));
#232215=CARTESIAN_POINT('Ctrl Pts',(-19.7989054860501,-13.2451415942809,
0.));
#232216=CARTESIAN_POINT('Ctrl Pts',(-19.8187131883919,-13.2504215002458,
0.));
#232217=CARTESIAN_POINT('Ctrl Pts',(-19.8386375318632,-13.2556757897085,
0.));
#232218=CARTESIAN_POINT('Ctrl Pts',(-19.8586778231711,-13.2609038446525,
0.));
#232219=CARTESIAN_POINT('Ctrl Pts',(-19.8788333760571,-13.2661050556128,
0.));
#232220=CARTESIAN_POINT('Ctrl Pts',(-19.8991035111739,-13.2712788215015,
0.));
#232221=CARTESIAN_POINT('Ctrl Pts',(-19.9194875559419,-13.2764245494354,
0.));
#232222=CARTESIAN_POINT('Ctrl Pts',(-19.9399848444019,-13.2815416545663,
0.));
#232223=CARTESIAN_POINT('Ctrl Pts',(-19.9605947170589,-13.2866295599152,
0.));
#232224=CARTESIAN_POINT('Ctrl Pts',(-19.9813165207174,-13.2916876962098,
0.));
#232225=CARTESIAN_POINT('Ctrl Pts',(-20.0021496083742,-13.296715501731,
0.));
#232226=CARTESIAN_POINT('Ctrl Pts',(-20.023093339104,-13.3017124221639,
0.));
#232227=CARTESIAN_POINT('Ctrl Pts',(-20.0441470779345,-13.3066779104515,
0.));
#232228=CARTESIAN_POINT('Ctrl Pts',(-20.0653101957188,-13.3116114266514,
0.));
#232229=CARTESIAN_POINT('Ctrl Pts',(-20.0865820689883,-13.3165124377963,
0.));
#232230=CARTESIAN_POINT('Ctrl Pts',(-20.1079620798377,-13.3213804177588,
0.));
#232231=CARTESIAN_POINT('Ctrl Pts',(-20.1294496158405,-13.3262148471228,
0.));
#232232=CARTESIAN_POINT('Ctrl Pts',(-20.1510440699477,-13.3310152130565,
0.));
#232233=CARTESIAN_POINT('Ctrl Pts',(-20.1727448403818,-13.3357810091903,
0.));
#232234=CARTESIAN_POINT('Ctrl Pts',(-20.1945513305233,-13.3405117354969,
0.));
#232235=CARTESIAN_POINT('Ctrl Pts',(-20.2164629487855,-13.3452068981763,
0.));
#232236=CARTESIAN_POINT('Ctrl Pts',(-20.2384791085354,-13.3498660095382,
0.));
#232237=CARTESIAN_POINT('Ctrl Pts',(-20.2605992280117,-13.3544885878886,
0.));
#232238=CARTESIAN_POINT('Ctrl Pts',(-20.2828227302337,-13.3590741574194,
0.));
#232239=CARTESIAN_POINT('Ctrl Pts',(-20.3051490429049,-13.3636222481017,
0.));
#232240=CARTESIAN_POINT('Ctrl Pts',(-20.3275775983032,-13.3681323955828,
0.));
#232241=CARTESIAN_POINT('Ctrl Pts',(-20.3501078331818,-13.3726041410869,
0.));
#232242=CARTESIAN_POINT('Ctrl Pts',(-20.3727391887187,-13.377037031319,
0.));
#232243=CARTESIAN_POINT('Ctrl Pts',(-20.3954711104505,-13.3814306183721,
0.));
#232244=CARTESIAN_POINT('Ctrl Pts',(-20.4183030482002,-13.3857844596387,
0.));
#232245=CARTESIAN_POINT('Ctrl Pts',(-20.4412344560007,-13.3900981177254,
0.));
#232246=CARTESIAN_POINT('Ctrl Pts',(-20.4642647920038,-13.3943711603739,
0.));
#232247=CARTESIAN_POINT('Ctrl Pts',(-20.4873935184041,-13.3986031603716,
0.));
#232248=CARTESIAN_POINT('Ctrl Pts',(-20.5106201013755,-13.4027936954529,
0.));
#232249=CARTESIAN_POINT('Ctrl Pts',(-20.5339440109958,-13.4069423482076,
0.));
#232250=CARTESIAN_POINT('Ctrl Pts',(-20.557364721164,-13.4110487059912,
0.));
#232251=CARTESIAN_POINT('Ctrl Pts',(-20.5808817095155,-13.4151123608411,
0.));
#232252=CARTESIAN_POINT('Ctrl Pts',(-20.6044944573151,-13.4191329093932,
0.));
#232253=CARTESIAN_POINT('Ctrl Pts',(-20.6282024494234,-13.4231099528178,
0.));
#232254=CARTESIAN_POINT('Ctrl Pts',(-20.6520051742868,-13.427043096765,
0.));
#232255=CARTESIAN_POINT('Ctrl Pts',(-20.6759021239102,-13.4309319513119,
0.));
#232256=CARTESIAN_POINT('Ctrl Pts',(-20.6998927938288,-13.4347761309154,
0.));
#232257=CARTESIAN_POINT('Ctrl Pts',(-20.7239766830675,-13.4385752543663,
0.));
#232258=CARTESIAN_POINT('Ctrl Pts',(-20.7481532941014,-13.4423289447561,
0.));
#232259=CARTESIAN_POINT('Ctrl Pts',(-20.7724221327609,-13.4460368293689,
0.));
#232260=CARTESIAN_POINT('Ctrl Pts',(-20.7967827081228,-13.4496985395637,
0.));
#232261=CARTESIAN_POINT('Ctrl Pts',(-20.821234532398,-13.4533137106667,
0.));
#232262=CARTESIAN_POINT('Ctrl Pts',(-20.8457771208083,-13.4568819818631,
0.));
#232263=CARTESIAN_POINT('Ctrl Pts',(-20.8704099914641,-13.4604029960983,
0.));
#232264=CARTESIAN_POINT('Ctrl Pts',(-20.8951326652158,-13.4638763999725,
0.));
#232265=CARTESIAN_POINT('Ctrl Pts',(-20.9199446657583,-13.4673018437717,
0.));
#232266=CARTESIAN_POINT('Ctrl Pts',(-20.9448455197557,-13.4706789815166,
0.));
#232267=CARTESIAN_POINT('Ctrl Pts',(-20.9698347569477,-13.4740074710086,
0.));
#232268=CARTESIAN_POINT('Ctrl Pts',(-20.9949119102592,-13.4772869738879,
0.));
#232269=CARTESIAN_POINT('Ctrl Pts',(-21.0200765158884,-13.4805171556822,
0.));
#232270=CARTESIAN_POINT('Ctrl Pts',(-21.0453281134245,-13.4836976858912,
0.));
#232271=CARTESIAN_POINT('Ctrl Pts',(-21.0706662455199,-13.4868282377191,
0.));
#232272=CARTESIAN_POINT('Ctrl Pts',(-21.0960904575046,-13.4899084877717,
0.));
#232273=CARTESIAN_POINT('Ctrl Pts',(-21.1216002970207,-13.4929381157778,
0.));
#232274=CARTESIAN_POINT('Ctrl Pts',(-21.1471953136209,-13.4959168042934,
0.));
#232275=CARTESIAN_POINT('Ctrl Pts',(-21.1728750584175,-13.4988442384491,
0.));
#232276=CARTESIAN_POINT('Ctrl Pts',(-21.1986390835828,-13.5017201056088,
0.));
#232277=CARTESIAN_POINT('Ctrl Pts',(-21.2244869429332,-13.5045440957404,
0.));
#232278=CARTESIAN_POINT('Ctrl Pts',(-21.250418192743,-13.5073159019452,
0.));
#232279=CARTESIAN_POINT('Ctrl Pts',(-21.2764323924442,-13.5100352209205,
0.));
#232280=CARTESIAN_POINT('Ctrl Pts',(-21.3025291054235,-13.5127017534971,
0.));
#232281=CARTESIAN_POINT('Ctrl Pts',(-21.3287078996341,-13.5153152050555,
0.));
#232282=CARTESIAN_POINT('Ctrl Pts',(-21.3549683486222,-13.5178752862466,
0.));
#232283=CARTESIAN_POINT('Ctrl Pts',(-21.3813100304973,-13.5203817122504,
0.));
#232284=CARTESIAN_POINT('Ctrl Pts',(-21.4077325259324,-13.5228342013516,
0.));
#232285=CARTESIAN_POINT('Ctrl Pts',(-21.4342354165259,-13.5252324737802,
0.));
#232286=CARTESIAN_POINT('Ctrl Pts',(-21.4608182828697,-13.5275762503555,
0.));
#232287=CARTESIAN_POINT('Ctrl Pts',(-21.4874807030468,-13.5298652514355,
0.));
#232288=CARTESIAN_POINT('Ctrl Pts',(-21.5142222501666,-13.5320991952138,
0.));
#232289=CARTESIAN_POINT('Ctrl Pts',(-21.5410424932503,-13.5342777983215,
0.));
#232290=CARTESIAN_POINT('Ctrl Pts',(-21.5679410019001,-13.536400779028,
0.));
#232291=CARTESIAN_POINT('Ctrl Pts',(-21.5949173499013,-13.5384678597195,
0.));
#232292=CARTESIAN_POINT('Ctrl Pts',(-21.6219711193946,-13.5404787697792,
0.));
#232293=CARTESIAN_POINT('Ctrl Pts',(-21.6491019044648,-13.5424332480699,
0.));
#232294=CARTESIAN_POINT('Ctrl Pts',(-21.6763093157699,-13.5443310461526,
0.));
#232295=CARTESIAN_POINT('Ctrl Pts',(-21.7035929822955,-13.5461719295048,
0.));
#232296=CARTESIAN_POINT('Ctrl Pts',(-21.7309525412281,-13.5479556704481,
0.));
#232297=CARTESIAN_POINT('Ctrl Pts',(-21.7583876294554,-13.5496820422211,
0.));
#232298=CARTESIAN_POINT('Ctrl Pts',(-21.7858978745865,-13.551350812725,
0.));
#232299=CARTESIAN_POINT('Ctrl Pts',(-21.8134828857967,-13.5529617381573,
0.));
#232300=CARTESIAN_POINT('Ctrl Pts',(-21.8411422456075,-13.5545145573031,
0.));
#232301=CARTESIAN_POINT('Ctrl Pts',(-21.8688754989365,-13.5560089839385,
0.));
#232302=CARTESIAN_POINT('Ctrl Pts',(-21.8966821688824,-13.5574447178424,
0.));
#232303=CARTESIAN_POINT('Ctrl Pts',(-21.9245617765769,-13.5588214586604,
0.));
#232304=CARTESIAN_POINT('Ctrl Pts',(-21.9525138592813,-13.5601389185257,
0.));
#232305=CARTESIAN_POINT('Ctrl Pts',(-21.9805379899168,-13.5613968357561,
0.));
#232306=CARTESIAN_POINT('Ctrl Pts',(-22.0086337943449,-13.5625949868333,
0.));
#232307=CARTESIAN_POINT('Ctrl Pts',(-22.0368009736295,-13.5637332022473,
0.));
#232308=CARTESIAN_POINT('Ctrl Pts',(-22.0650393089609,-13.5648113689033,
0.));
#232309=CARTESIAN_POINT('Ctrl Pts',(-22.0933486464593,-13.5658294169284,
0.));
#232310=CARTESIAN_POINT('Ctrl Pts',(-22.1217288871975,-13.5667873105359,
0.));
#232311=CARTESIAN_POINT('Ctrl Pts',(-22.1444897575194,-13.5675054919061,
0.));
#232312=CARTESIAN_POINT('Ctrl Pts',(-22.1615922805008,-13.5680170531805,
0.));
#232313=CARTESIAN_POINT('Ctrl Pts',(-22.1730081264608,-13.5683460612942,
0.));
#232314=CARTESIAN_POINT('Ctrl Pts',(-22.1787195904339,-13.5685075571671,
0.));
#232315=CARTESIAN_POINT('',(-22.1787195904339,-13.5685075571671,12.));
#232316=CARTESIAN_POINT('Ctrl Pts',(-22.1787195904339,-13.5685075571671,
12.));
#232317=CARTESIAN_POINT('Ctrl Pts',(-22.1730081264608,-13.5683460612942,
12.));
#232318=CARTESIAN_POINT('Ctrl Pts',(-22.1615922805008,-13.5680170531805,
12.));
#232319=CARTESIAN_POINT('Ctrl Pts',(-22.1444897575194,-13.5675054919061,
12.));
#232320=CARTESIAN_POINT('Ctrl Pts',(-22.1217288871975,-13.5667873105359,
12.));
#232321=CARTESIAN_POINT('Ctrl Pts',(-22.0933486464593,-13.5658294169284,
12.));
#232322=CARTESIAN_POINT('Ctrl Pts',(-22.0650393089609,-13.5648113689033,
12.));
#232323=CARTESIAN_POINT('Ctrl Pts',(-22.0368009736295,-13.5637332022473,
12.));
#232324=CARTESIAN_POINT('Ctrl Pts',(-22.0086337943449,-13.5625949868333,
12.));
#232325=CARTESIAN_POINT('Ctrl Pts',(-21.9805379899168,-13.5613968357561,
12.));
#232326=CARTESIAN_POINT('Ctrl Pts',(-21.9525138592813,-13.5601389185257,
12.));
#232327=CARTESIAN_POINT('Ctrl Pts',(-21.9245617765769,-13.5588214586604,
12.));
#232328=CARTESIAN_POINT('Ctrl Pts',(-21.8966821688824,-13.5574447178424,
12.));
#232329=CARTESIAN_POINT('Ctrl Pts',(-21.8688754989365,-13.5560089839385,
12.));
#232330=CARTESIAN_POINT('Ctrl Pts',(-21.8411422456075,-13.5545145573031,
12.));
#232331=CARTESIAN_POINT('Ctrl Pts',(-21.8134828857967,-13.5529617381573,
12.));
#232332=CARTESIAN_POINT('Ctrl Pts',(-21.7858978745865,-13.551350812725,
12.));
#232333=CARTESIAN_POINT('Ctrl Pts',(-21.7583876294554,-13.5496820422211,
12.));
#232334=CARTESIAN_POINT('Ctrl Pts',(-21.7309525412281,-13.5479556704481,
12.));
#232335=CARTESIAN_POINT('Ctrl Pts',(-21.7035929822955,-13.5461719295048,
12.));
#232336=CARTESIAN_POINT('Ctrl Pts',(-21.6763093157699,-13.5443310461526,
12.));
#232337=CARTESIAN_POINT('Ctrl Pts',(-21.6491019044648,-13.5424332480699,
12.));
#232338=CARTESIAN_POINT('Ctrl Pts',(-21.6219711193946,-13.5404787697792,
12.));
#232339=CARTESIAN_POINT('Ctrl Pts',(-21.5949173499013,-13.5384678597195,
12.));
#232340=CARTESIAN_POINT('Ctrl Pts',(-21.5679410019001,-13.536400779028,
12.));
#232341=CARTESIAN_POINT('Ctrl Pts',(-21.5410424932503,-13.5342777983215,
12.));
#232342=CARTESIAN_POINT('Ctrl Pts',(-21.5142222501666,-13.5320991952138,
12.));
#232343=CARTESIAN_POINT('Ctrl Pts',(-21.4874807030468,-13.5298652514355,
12.));
#232344=CARTESIAN_POINT('Ctrl Pts',(-21.4608182828697,-13.5275762503555,
12.));
#232345=CARTESIAN_POINT('Ctrl Pts',(-21.4342354165259,-13.5252324737802,
12.));
#232346=CARTESIAN_POINT('Ctrl Pts',(-21.4077325259324,-13.5228342013516,
12.));
#232347=CARTESIAN_POINT('Ctrl Pts',(-21.3813100304973,-13.5203817122504,
12.));
#232348=CARTESIAN_POINT('Ctrl Pts',(-21.3549683486222,-13.5178752862466,
12.));
#232349=CARTESIAN_POINT('Ctrl Pts',(-21.3287078996341,-13.5153152050555,
12.));
#232350=CARTESIAN_POINT('Ctrl Pts',(-21.3025291054235,-13.5127017534971,
12.));
#232351=CARTESIAN_POINT('Ctrl Pts',(-21.2764323924442,-13.5100352209205,
12.));
#232352=CARTESIAN_POINT('Ctrl Pts',(-21.250418192743,-13.5073159019452,
12.));
#232353=CARTESIAN_POINT('Ctrl Pts',(-21.2244869429332,-13.5045440957404,
12.));
#232354=CARTESIAN_POINT('Ctrl Pts',(-21.1986390835828,-13.5017201056088,
12.));
#232355=CARTESIAN_POINT('Ctrl Pts',(-21.1728750584175,-13.4988442384491,
12.));
#232356=CARTESIAN_POINT('Ctrl Pts',(-21.1471953136209,-13.4959168042934,
12.));
#232357=CARTESIAN_POINT('Ctrl Pts',(-21.1216002970207,-13.4929381157778,
12.));
#232358=CARTESIAN_POINT('Ctrl Pts',(-21.0960904575046,-13.4899084877717,
12.));
#232359=CARTESIAN_POINT('Ctrl Pts',(-21.0706662455199,-13.4868282377191,
12.));
#232360=CARTESIAN_POINT('Ctrl Pts',(-21.0453281134245,-13.4836976858912,
12.));
#232361=CARTESIAN_POINT('Ctrl Pts',(-21.0200765158884,-13.4805171556822,
12.));
#232362=CARTESIAN_POINT('Ctrl Pts',(-20.9949119102592,-13.4772869738879,
12.));
#232363=CARTESIAN_POINT('Ctrl Pts',(-20.9698347569477,-13.4740074710086,
12.));
#232364=CARTESIAN_POINT('Ctrl Pts',(-20.9448455197557,-13.4706789815166,
12.));
#232365=CARTESIAN_POINT('Ctrl Pts',(-20.9199446657583,-13.4673018437717,
12.));
#232366=CARTESIAN_POINT('Ctrl Pts',(-20.8951326652158,-13.4638763999725,
12.));
#232367=CARTESIAN_POINT('Ctrl Pts',(-20.8704099914641,-13.4604029960983,
12.));
#232368=CARTESIAN_POINT('Ctrl Pts',(-20.8457771208083,-13.4568819818631,
12.));
#232369=CARTESIAN_POINT('Ctrl Pts',(-20.821234532398,-13.4533137106667,
12.));
#232370=CARTESIAN_POINT('Ctrl Pts',(-20.7967827081228,-13.4496985395637,
12.));
#232371=CARTESIAN_POINT('Ctrl Pts',(-20.7724221327609,-13.4460368293689,
12.));
#232372=CARTESIAN_POINT('Ctrl Pts',(-20.7481532941014,-13.4423289447561,
12.));
#232373=CARTESIAN_POINT('Ctrl Pts',(-20.7239766830675,-13.4385752543663,
12.));
#232374=CARTESIAN_POINT('Ctrl Pts',(-20.6998927938288,-13.4347761309154,
12.));
#232375=CARTESIAN_POINT('Ctrl Pts',(-20.6759021239102,-13.4309319513119,
12.));
#232376=CARTESIAN_POINT('Ctrl Pts',(-20.6520051742868,-13.427043096765,
12.));
#232377=CARTESIAN_POINT('Ctrl Pts',(-20.6282024494234,-13.4231099528178,
12.));
#232378=CARTESIAN_POINT('Ctrl Pts',(-20.6044944573151,-13.4191329093932,
12.));
#232379=CARTESIAN_POINT('Ctrl Pts',(-20.5808817095155,-13.4151123608411,
12.));
#232380=CARTESIAN_POINT('Ctrl Pts',(-20.557364721164,-13.4110487059912,
12.));
#232381=CARTESIAN_POINT('Ctrl Pts',(-20.5339440109958,-13.4069423482076,
12.));
#232382=CARTESIAN_POINT('Ctrl Pts',(-20.5106201013755,-13.4027936954529,
12.));
#232383=CARTESIAN_POINT('Ctrl Pts',(-20.4873935184041,-13.3986031603716,
12.));
#232384=CARTESIAN_POINT('Ctrl Pts',(-20.4642647920038,-13.3943711603739,
12.));
#232385=CARTESIAN_POINT('Ctrl Pts',(-20.4412344560007,-13.3900981177254,
12.));
#232386=CARTESIAN_POINT('Ctrl Pts',(-20.4183030482002,-13.3857844596387,
12.));
#232387=CARTESIAN_POINT('Ctrl Pts',(-20.3954711104505,-13.3814306183721,
12.));
#232388=CARTESIAN_POINT('Ctrl Pts',(-20.3727391887187,-13.377037031319,
12.));
#232389=CARTESIAN_POINT('Ctrl Pts',(-20.3501078331818,-13.3726041410869,
12.));
#232390=CARTESIAN_POINT('Ctrl Pts',(-20.3275775983032,-13.3681323955828,
12.));
#232391=CARTESIAN_POINT('Ctrl Pts',(-20.3051490429049,-13.3636222481017,
12.));
#232392=CARTESIAN_POINT('Ctrl Pts',(-20.2828227302337,-13.3590741574194,
12.));
#232393=CARTESIAN_POINT('Ctrl Pts',(-20.2605992280117,-13.3544885878886,
12.));
#232394=CARTESIAN_POINT('Ctrl Pts',(-20.2384791085354,-13.3498660095382,
12.));
#232395=CARTESIAN_POINT('Ctrl Pts',(-20.2164629487855,-13.3452068981763,
12.));
#232396=CARTESIAN_POINT('Ctrl Pts',(-20.1945513305233,-13.3405117354969,
12.));
#232397=CARTESIAN_POINT('Ctrl Pts',(-20.1727448403818,-13.3357810091903,
12.));
#232398=CARTESIAN_POINT('Ctrl Pts',(-20.1510440699477,-13.3310152130565,
12.));
#232399=CARTESIAN_POINT('Ctrl Pts',(-20.1294496158405,-13.3262148471228,
12.));
#232400=CARTESIAN_POINT('Ctrl Pts',(-20.1079620798377,-13.3213804177588,
12.));
#232401=CARTESIAN_POINT('Ctrl Pts',(-20.0865820689883,-13.3165124377963,
12.));
#232402=CARTESIAN_POINT('Ctrl Pts',(-20.0653101957188,-13.3116114266514,
12.));
#232403=CARTESIAN_POINT('Ctrl Pts',(-20.0441470779345,-13.3066779104515,
12.));
#232404=CARTESIAN_POINT('Ctrl Pts',(-20.023093339104,-13.3017124221639,
12.));
#232405=CARTESIAN_POINT('Ctrl Pts',(-20.0021496083742,-13.296715501731,
12.));
#232406=CARTESIAN_POINT('Ctrl Pts',(-19.9813165207174,-13.2916876962098,
12.));
#232407=CARTESIAN_POINT('Ctrl Pts',(-19.9605947170589,-13.2866295599152,
12.));
#232408=CARTESIAN_POINT('Ctrl Pts',(-19.9399848444019,-13.2815416545663,
12.));
#232409=CARTESIAN_POINT('Ctrl Pts',(-19.9194875559419,-13.2764245494354,
12.));
#232410=CARTESIAN_POINT('Ctrl Pts',(-19.8991035111739,-13.2712788215015,
12.));
#232411=CARTESIAN_POINT('Ctrl Pts',(-19.8788333760571,-13.2661050556128,
12.));
#232412=CARTESIAN_POINT('Ctrl Pts',(-19.8586778231711,-13.2609038446525,
12.));
#232413=CARTESIAN_POINT('Ctrl Pts',(-19.8386375318632,-13.2556757897085,
12.));
#232414=CARTESIAN_POINT('Ctrl Pts',(-19.8187131883919,-13.2504215002458,
12.));
#232415=CARTESIAN_POINT('Ctrl Pts',(-19.7989054860501,-13.2451415942809,
12.));
#232416=CARTESIAN_POINT('Ctrl Pts',(-19.7792151253297,-13.239836698568,
12.));
#232417=CARTESIAN_POINT('Ctrl Pts',(-19.7596428141176,-13.2345074487968,
12.));
#232418=CARTESIAN_POINT('Ctrl Pts',(-19.7401892678701,-13.2291544897902,
12.));
#232419=CARTESIAN_POINT('Ctrl Pts',(-19.7208552097867,-13.2237784757065,
12.));
#232420=CARTESIAN_POINT('Ctrl Pts',(-19.7016413709678,-13.2183800702431,
12.));
#232421=CARTESIAN_POINT('Ctrl Pts',(-19.6825484905812,-13.2129599468478,
12.));
#232422=CARTESIAN_POINT('Ctrl Pts',(-19.6635773160924,-13.2075187889522,
12.));
#232423=CARTESIAN_POINT('Ctrl Pts',(-19.6447286034764,-13.202057290206,
12.));
#232424=CARTESIAN_POINT('Ctrl Pts',(-19.6260031174244,-13.196576154715,
12.));
#232425=CARTESIAN_POINT('Ctrl Pts',(-19.6074016315421,-13.1910760972818,
12.));
#232426=CARTESIAN_POINT('Ctrl Pts',(-19.5889249285352,-13.1855578436479,
12.));
#232427=CARTESIAN_POINT('Ctrl Pts',(-19.5705738004682,-13.1800221307682,
12.));
#232428=CARTESIAN_POINT('Ctrl Pts',(-19.5523490490254,-13.1744697070918,
12.));
#232429=CARTESIAN_POINT('Ctrl Pts',(-19.5342514857564,-13.1689013328432,
12.));
#232430=CARTESIAN_POINT('Ctrl Pts',(-19.5162819323207,-13.1633177803097,
12.));
#232431=CARTESIAN_POINT('Ctrl Pts',(-19.498441220707,-13.1577198341238,
12.));
#232432=CARTESIAN_POINT('Ctrl Pts',(-19.4807301935256,-13.1521082915846,
12.));
#232433=CARTESIAN_POINT('Ctrl Pts',(-19.463149704325,-13.1464839629966,
12.));
#232434=CARTESIAN_POINT('Ctrl Pts',(-19.4457006178875,-13.140847672006,
12.));
#232435=CARTESIAN_POINT('Ctrl Pts',(-19.4283838105265,-13.1352002559439,
12.));
#232436=CARTESIAN_POINT('Ctrl Pts',(-19.4112001703561,-13.1295425661635,
12.));
#232437=CARTESIAN_POINT('Ctrl Pts',(-19.3941505976267,-13.1238754684177,
12.));
#232438=CARTESIAN_POINT('Ctrl Pts',(-19.3772360051093,-13.118199843271,
12.));
#232439=CARTESIAN_POINT('Ctrl Pts',(-19.3604573184516,-13.1125165865021,
12.));
#232440=CARTESIAN_POINT('Ctrl Pts',(-19.3438154765395,-13.1068266095186,
12.));
#232441=CARTESIAN_POINT('Ctrl Pts',(-19.3273114318268,-13.1011308397592,
12.));
#232442=CARTESIAN_POINT('Ctrl Pts',(-19.3109461507358,-13.095430221148,
12.));
#232443=CARTESIAN_POINT('Ctrl Pts',(-19.2947206141246,-13.0897257145969,
12.));
#232444=CARTESIAN_POINT('Ctrl Pts',(-19.2786358177198,-13.0840182984949,
12.));
#232445=CARTESIAN_POINT('Ctrl Pts',(-19.2626927725596,-13.0783089692118,
12.));
#232446=CARTESIAN_POINT('Ctrl Pts',(-19.2468925053988,-13.0725987415856,
12.));
#232447=CARTESIAN_POINT('Ctrl Pts',(-19.2312360592031,-13.0668886494791,
12.));
#232448=CARTESIAN_POINT('Ctrl Pts',(-19.2157244937141,-13.0611797463913,
12.));
#232449=CARTESIAN_POINT('Ctrl Pts',(-19.2003588859771,-13.0554731060537,
12.));
#232450=CARTESIAN_POINT('Ctrl Pts',(-19.1851403308825,-13.0497698230442,
12.));
#232451=CARTESIAN_POINT('Ctrl Pts',(-19.1700699416625,-13.0440710133775,
12.));
#232452=CARTESIAN_POINT('Ctrl Pts',(-19.1551488505233,-13.0383778152072,
12.));
#232453=CARTESIAN_POINT('Ctrl Pts',(-19.1403782093389,-13.0326913895841,
12.));
#232454=CARTESIAN_POINT('Ctrl Pts',(-19.1257591903099,-13.0270129211976,
12.));
#232455=CARTESIAN_POINT('Ctrl Pts',(-19.1112929866308,-13.0213436191326,
12.));
#232456=CARTESIAN_POINT('Ctrl Pts',(-19.0969808131226,-13.0156847176093,
12.));
#232457=CARTESIAN_POINT('Ctrl Pts',(-19.0828239070482,-13.0100374768785,
12.));
#232458=CARTESIAN_POINT('Ctrl Pts',(-19.0688235289437,-13.0044031841381,
12.));
#232459=CARTESIAN_POINT('Ctrl Pts',(-19.0549809634355,-12.9987831544502,
12.));
#232460=CARTESIAN_POINT('Ctrl Pts',(-19.0412975200398,-12.9931787316515,
12.));
#232461=CARTESIAN_POINT('Ctrl Pts',(-19.0277745339908,-12.9875912893003,
12.));
#232462=CARTESIAN_POINT('Ctrl Pts',(-19.0144133673348,-12.9820222318716,
12.));
#232463=CARTESIAN_POINT('Ctrl Pts',(-19.0012154099791,-12.9764729959205,
12.));
#232464=CARTESIAN_POINT('Ctrl Pts',(-18.9881820807586,-12.9709450512747,
12.));
#232465=CARTESIAN_POINT('Ctrl Pts',(-18.9753148284475,-12.9654399021869,
12.));
#232466=CARTESIAN_POINT('Ctrl Pts',(-18.9626151329229,-12.9599590886319,
12.));
#232467=CARTESIAN_POINT('Ctrl Pts',(-18.9500845064715,-12.9545041877377,
12.));
#232468=CARTESIAN_POINT('Ctrl Pts',(-18.9377244950435,-12.9490768151821,
12.));
#232469=CARTESIAN_POINT('Ctrl Pts',(-18.9255366795195,-12.9436786266105,
12.));
#232470=CARTESIAN_POINT('Ctrl Pts',(-18.9135226769465,-12.9383113190375,
12.));
#232471=CARTESIAN_POINT('Ctrl Pts',(-18.9016841423403,-12.9329766328185,
12.));
#232472=CARTESIAN_POINT('Ctrl Pts',(-18.8900227704889,-12.9276763536373,
12.));
#232473=CARTESIAN_POINT('Ctrl Pts',(-18.8785402977527,-12.9224123144982,
12.));
#232474=CARTESIAN_POINT('Ctrl Pts',(-18.8672385038326,-12.9171863977045,
12.));
#232475=CARTESIAN_POINT('Ctrl Pts',(-18.8561192136198,-12.9120005369063,
12.));
#232476=CARTESIAN_POINT('Ctrl Pts',(-18.8451842990984,-12.9068567191854,
12.));
#232477=CARTESIAN_POINT('Ctrl Pts',(-18.834435681259,-12.9017569871738,
12.));
#232478=CARTESIAN_POINT('Ctrl Pts',(-18.8238753319129,-12.8967034410755,
12.));
#232479=CARTESIAN_POINT('Ctrl Pts',(-18.813505275782,-12.8916982409935,
12.));
#232480=CARTESIAN_POINT('Ctrl Pts',(-18.8033275941943,-12.8867436109546,
12.));
#232481=CARTESIAN_POINT('Ctrl Pts',(-18.7933444285868,-12.8818418427475,
12.));
#232482=CARTESIAN_POINT('Ctrl Pts',(-18.7835579840477,-12.8769952998095,
12.));
#232483=CARTESIAN_POINT('Ctrl Pts',(-18.7739705329022,-12.872206421181,
12.));
#232484=CARTESIAN_POINT('Ctrl Pts',(-18.7645844169564,-12.8674777239653,
12.));
#232485=CARTESIAN_POINT('Ctrl Pts',(-18.7554020493887,-12.8628118054171,
12.));
#232486=CARTESIAN_POINT('Ctrl Pts',(-18.7464259171251,-12.8582113455646,
12.));
#232487=CARTESIAN_POINT('Ctrl Pts',(-18.7376585820854,-12.8536791086316,
12.));
#232488=CARTESIAN_POINT('Ctrl Pts',(-18.7291026886554,-12.8492179511591,
12.));
#232489=CARTESIAN_POINT('Ctrl Pts',(-18.7207609737702,-12.8448308329494,
12.));
#232490=CARTESIAN_POINT('Ctrl Pts',(-18.7126362754445,-12.8405208263431,
12.));
#232491=CARTESIAN_POINT('Ctrl Pts',(-18.7047315436294,-12.8362911280361,
12.));
#232492=CARTESIAN_POINT('Ctrl Pts',(-18.6970498410172,-12.8321450599789,
12.));
#232493=CARTESIAN_POINT('Ctrl Pts',(-18.6895943376171,-12.8280860635231,
12.));
#232494=CARTESIAN_POINT('Ctrl Pts',(-18.6823683094139,-12.8241176980017,
12.));
#232495=CARTESIAN_POINT('Ctrl Pts',(-18.6753751301092,-12.8202436318474,
12.));
#232496=CARTESIAN_POINT('Ctrl Pts',(-18.6686182952799,-12.8164676687362,
12.));
#232497=CARTESIAN_POINT('Ctrl Pts',(-18.6621014624746,-12.8127937909631,
12.));
#232498=CARTESIAN_POINT('Ctrl Pts',(-18.6558284825773,-12.8092261933858,
12.));
#232499=CARTESIAN_POINT('Ctrl Pts',(-18.6498034438987,-12.805769331162,
12.));
#232500=CARTESIAN_POINT('Ctrl Pts',(-18.6440306327456,-12.8024278770152,
12.));
#232501=CARTESIAN_POINT('Ctrl Pts',(-18.63851447924,-12.7992066625264,12.));
#232502=CARTESIAN_POINT('Ctrl Pts',(-18.6332595057006,-12.7961106222251,
12.));
#232503=CARTESIAN_POINT('Ctrl Pts',(-18.6282702819371,-12.7931447451555,
12.));
#232504=CARTESIAN_POINT('Ctrl Pts',(-18.6235516265575,-12.7903142925234,
12.));
#232505=CARTESIAN_POINT('Ctrl Pts',(-18.6191087624752,-12.7876249657834,
12.));
#232506=CARTESIAN_POINT('Ctrl Pts',(-18.6149475565188,-12.7850831657901,
12.));
#232507=CARTESIAN_POINT('Ctrl Pts',(-18.6110744826219,-12.7826959526925,
12.));
#232508=CARTESIAN_POINT('Ctrl Pts',(-18.6074961535723,-12.7804705387658,
12.));
#232509=CARTESIAN_POINT('Ctrl Pts',(-18.6042190183704,-12.7784139605066,
12.));
#232510=CARTESIAN_POINT('Ctrl Pts',(-18.6012488486709,-12.7765325225081,
12.));
#232511=CARTESIAN_POINT('Ctrl Pts',(-18.598591752595,-12.7748328937638,
12.));
#232512=CARTESIAN_POINT('Ctrl Pts',(-18.5962551167772,-12.7733231262108,
12.));
#232513=CARTESIAN_POINT('Ctrl Pts',(-18.5942490615407,-12.7720142287172,
12.));
#232514=CARTESIAN_POINT('Ctrl Pts',(-18.5925859134579,-12.7709195951156,
12.));
#232515=CARTESIAN_POINT('Ctrl Pts',(-18.5912775137806,-12.7700520897173,
12.));
#232516=CARTESIAN_POINT('Ctrl Pts',(-18.5903328777227,-12.7694215127919,
12.));
#232517=CARTESIAN_POINT('Ctrl Pts',(-18.589871621843,-12.769110348199,12.));
#232518=CARTESIAN_POINT('Ctrl Pts',(-18.5896919669165,-12.768986426692,
12.));
#232519=CARTESIAN_POINT('Ctrl Pts',(-18.5896460962964,-12.7689524524483,
12.));
#232520=CARTESIAN_POINT('Ctrl Pts',(-18.5896416359912,-12.7689476255363,
12.));
#232521=CARTESIAN_POINT('',(-22.178719590434,-13.5685075571671,0.));
#232522=CARTESIAN_POINT('Origin',(-20.2687213152502,-7.17139709155223,0.));
#232523=CARTESIAN_POINT('',(-21.2610617890679,-7.52250298901264,12.));
#232524=CARTESIAN_POINT('',(-10.1343606576251,-3.58569854577611,12.));
#232525=CARTESIAN_POINT('',(-21.2610617890679,-7.52250298901264,0.));
#232526=CARTESIAN_POINT('',(-21.2610617890679,-7.52250298901264,0.));
#232527=CARTESIAN_POINT('',(-10.1343606576251,-3.58569854577611,0.));
#232528=CARTESIAN_POINT('Ctrl Pts',(-22.8400320311649,-12.4230808101438,
0.));
#232529=CARTESIAN_POINT('Ctrl Pts',(-22.8400320311649,-12.4230808101438,
12.));
#232530=CARTESIAN_POINT('Ctrl Pts',(-22.8370364396459,-12.418215285186,
0.));
#232531=CARTESIAN_POINT('Ctrl Pts',(-22.8370364396459,-12.418215285186,
12.));
#232532=CARTESIAN_POINT('Ctrl Pts',(-22.8310435872748,-12.4084933766346,
0.));
#232533=CARTESIAN_POINT('Ctrl Pts',(-22.8310435872748,-12.4084933766346,
12.));
#232534=CARTESIAN_POINT('Ctrl Pts',(-22.8220493007173,-12.3939379378998,
0.));
#232535=CARTESIAN_POINT('Ctrl Pts',(-22.8220493007173,-12.3939379378998,
12.));
#232536=CARTESIAN_POINT('Ctrl Pts',(-22.81004690224,-12.374585536673,0.));
#232537=CARTESIAN_POINT('Ctrl Pts',(-22.81004690224,-12.374585536673,12.));
#232538=CARTESIAN_POINT('Ctrl Pts',(-22.795027221673,-12.3504864740319,
0.));
#232539=CARTESIAN_POINT('Ctrl Pts',(-22.795027221673,-12.3504864740319,
12.));
#232540=CARTESIAN_POINT('Ctrl Pts',(-22.7799908974768,-12.3264788926075,
0.));
#232541=CARTESIAN_POINT('Ctrl Pts',(-22.7799908974768,-12.3264788926075,
12.));
#232542=CARTESIAN_POINT('Ctrl Pts',(-22.764938010105,-12.3025628601792,
0.));
#232543=CARTESIAN_POINT('Ctrl Pts',(-22.764938010105,-12.3025628601792,
12.));
#232544=CARTESIAN_POINT('Ctrl Pts',(-22.7498686970069,-12.2787384750742,
0.));
#232545=CARTESIAN_POINT('Ctrl Pts',(-22.7498686970069,-12.2787384750742,
12.));
#232546=CARTESIAN_POINT('Ctrl Pts',(-22.7347831655287,-12.2550058702395,
0.));
#232547=CARTESIAN_POINT('Ctrl Pts',(-22.7347831655287,-12.2550058702395,
12.));
#232548=CARTESIAN_POINT('Ctrl Pts',(-22.7196817119374,-12.2313652198061,
0.));
#232549=CARTESIAN_POINT('Ctrl Pts',(-22.7196817119374,-12.2313652198061,
12.));
#232550=CARTESIAN_POINT('Ctrl Pts',(-22.7045647168747,-12.2078167360284,
0.));
#232551=CARTESIAN_POINT('Ctrl Pts',(-22.7045647168747,-12.2078167360284,
12.));
#232552=CARTESIAN_POINT('Ctrl Pts',(-22.6894326205037,-12.1843606579261,
0.));
#232553=CARTESIAN_POINT('Ctrl Pts',(-22.6894326205037,-12.1843606579261,
12.));
#232554=CARTESIAN_POINT('Ctrl Pts',(-22.6742859034944,-12.1609972423099,
0.));
#232555=CARTESIAN_POINT('Ctrl Pts',(-22.6742859034944,-12.1609972423099,
12.));
#232556=CARTESIAN_POINT('Ctrl Pts',(-22.6591250653965,-12.1377267537145,
0.));
#232557=CARTESIAN_POINT('Ctrl Pts',(-22.6591250653965,-12.1377267537145,
12.));
#232558=CARTESIAN_POINT('Ctrl Pts',(-22.6439506046605,-12.1145494550383,
0.));
#232559=CARTESIAN_POINT('Ctrl Pts',(-22.6439506046605,-12.1145494550383,
12.));
#232560=CARTESIAN_POINT('Ctrl Pts',(-22.6287629967056,-12.0914655972823,
0.));
#232561=CARTESIAN_POINT('Ctrl Pts',(-22.6287629967056,-12.0914655972823,
12.));
#232562=CARTESIAN_POINT('Ctrl Pts',(-22.6135626764898,-12.0684754113862,
0.));
#232563=CARTESIAN_POINT('Ctrl Pts',(-22.6135626764898,-12.0684754113862,
12.));
#232564=CARTESIAN_POINT('Ctrl Pts',(-22.5983500505644,-12.0455791139128,
0.));
#232565=CARTESIAN_POINT('Ctrl Pts',(-22.5983500505644,-12.0455791139128,
12.));
#232566=CARTESIAN_POINT('Ctrl Pts',(-22.5831255061282,-12.0227769113127,
0.));
#232567=CARTESIAN_POINT('Ctrl Pts',(-22.5831255061282,-12.0227769113127,
12.));
#232568=CARTESIAN_POINT('Ctrl Pts',(-22.5678894211181,-12.0000690046695,
0.));
#232569=CARTESIAN_POINT('Ctrl Pts',(-22.5678894211181,-12.0000690046695,
12.));
#232570=CARTESIAN_POINT('Ctrl Pts',(-22.5526421741158,-11.9774555943496,
0.));
#232571=CARTESIAN_POINT('Ctrl Pts',(-22.5526421741158,-11.9774555943496,
12.));
#232572=CARTESIAN_POINT('Ctrl Pts',(-22.5373841537307,-11.9549368843997,
0.));
#232573=CARTESIAN_POINT('Ctrl Pts',(-22.5373841537307,-11.9549368843997,
12.));
#232574=CARTESIAN_POINT('Ctrl Pts',(-22.5221157697883,-11.9325130877803,
0.));
#232575=CARTESIAN_POINT('Ctrl Pts',(-22.5221157697883,-11.9325130877803,
12.));
#232576=CARTESIAN_POINT('Ctrl Pts',(-22.5068374513973,-11.9101844254557,
0.));
#232577=CARTESIAN_POINT('Ctrl Pts',(-22.5068374513973,-11.9101844254557,
12.));
#232578=CARTESIAN_POINT('Ctrl Pts',(-22.4915496418485,-11.8879511239942,
0.));
#232579=CARTESIAN_POINT('Ctrl Pts',(-22.4915496418485,-11.8879511239942,
12.));
#232580=CARTESIAN_POINT('Ctrl Pts',(-22.4762527946702,-11.8658134137019,
0.));
#232581=CARTESIAN_POINT('Ctrl Pts',(-22.4762527946702,-11.8658134137019,
12.));
#232582=CARTESIAN_POINT('Ctrl Pts',(-22.4609473690471,-11.8437715264487,
0.));
#232583=CARTESIAN_POINT('Ctrl Pts',(-22.4609473690471,-11.8437715264487,
12.));
#232584=CARTESIAN_POINT('Ctrl Pts',(-22.4456338258735,-11.8218256937889,
0.));
#232585=CARTESIAN_POINT('Ctrl Pts',(-22.4456338258735,-11.8218256937889,
12.));
#232586=CARTESIAN_POINT('Ctrl Pts',(-22.430312622646,-11.7999761445173,
0.));
#232587=CARTESIAN_POINT('Ctrl Pts',(-22.430312622646,-11.7999761445173,
12.));
#232588=CARTESIAN_POINT('Ctrl Pts',(-22.4149842125008,-11.7782231042039,
0.));
#232589=CARTESIAN_POINT('Ctrl Pts',(-22.4149842125008,-11.7782231042039,
12.));
#232590=CARTESIAN_POINT('Ctrl Pts',(-22.3996490469191,-11.7565667964764,
0.));
#232591=CARTESIAN_POINT('Ctrl Pts',(-22.3996490469191,-11.7565667964764,
12.));
#232592=CARTESIAN_POINT('Ctrl Pts',(-22.3843075773899,-11.7350074437961,
0.));
#232593=CARTESIAN_POINT('Ctrl Pts',(-22.3843075773899,-11.7350074437961,
12.));
#232594=CARTESIAN_POINT('Ctrl Pts',(-22.3689602575491,-11.7135452684532,
0.));
#232595=CARTESIAN_POINT('Ctrl Pts',(-22.3689602575491,-11.7135452684532,
12.));
#232596=CARTESIAN_POINT('Ctrl Pts',(-22.3536075450029,-11.6921804934056,
0.));
#232597=CARTESIAN_POINT('Ctrl Pts',(-22.3536075450029,-11.6921804934056,
12.));
#232598=CARTESIAN_POINT('Ctrl Pts',(-22.3382499035619,-11.6709133432985,
0.));
#232599=CARTESIAN_POINT('Ctrl Pts',(-22.3382499035619,-11.6709133432985,
12.));
#232600=CARTESIAN_POINT('Ctrl Pts',(-22.3228878043976,-11.6497440449857,
0.));
#232601=CARTESIAN_POINT('Ctrl Pts',(-22.3228878043976,-11.6497440449857,
12.));
#232602=CARTESIAN_POINT('Ctrl Pts',(-22.3075217249049,-11.6286728270009,
0.));
#232603=CARTESIAN_POINT('Ctrl Pts',(-22.3075217249049,-11.6286728270009,
12.));
#232604=CARTESIAN_POINT('Ctrl Pts',(-22.2921521480356,-11.6076999192357,
0.));
#232605=CARTESIAN_POINT('Ctrl Pts',(-22.2921521480356,-11.6076999192357,
12.));
#232606=CARTESIAN_POINT('Ctrl Pts',(-22.2767795614348,-11.5868255525188,
0.));
#232607=CARTESIAN_POINT('Ctrl Pts',(-22.2767795614348,-11.5868255525188,
12.));
#232608=CARTESIAN_POINT('Ctrl Pts',(-22.2614044566898,-11.5660499582403,
0.));
#232609=CARTESIAN_POINT('Ctrl Pts',(-22.2614044566898,-11.5660499582403,
12.));
#232610=CARTESIAN_POINT('Ctrl Pts',(-22.2460273284654,-11.5453733679121,
0.));
#232611=CARTESIAN_POINT('Ctrl Pts',(-22.2460273284654,-11.5453733679121,
12.));
#232612=CARTESIAN_POINT('Ctrl Pts',(-22.2306486738901,-11.5247960128477,
0.));
#232613=CARTESIAN_POINT('Ctrl Pts',(-22.2306486738901,-11.5247960128477,
12.));
#232614=CARTESIAN_POINT('Ctrl Pts',(-22.2152689931022,-11.5043181244242,
0.));
#232615=CARTESIAN_POINT('Ctrl Pts',(-22.2152689931022,-11.5043181244242,
12.));
#232616=CARTESIAN_POINT('Ctrl Pts',(-22.1998887896436,-11.483939934259,
0.));
#232617=CARTESIAN_POINT('Ctrl Pts',(-22.1998887896436,-11.483939934259,
12.));
#232618=CARTESIAN_POINT('Ctrl Pts',(-22.184508570917,-11.463661674411,0.));
#232619=CARTESIAN_POINT('Ctrl Pts',(-22.184508570917,-11.463661674411,12.));
#232620=CARTESIAN_POINT('Ctrl Pts',(-22.1691288486096,-11.443483577557,
0.));
#232621=CARTESIAN_POINT('Ctrl Pts',(-22.1691288486096,-11.443483577557,
12.));
#232622=CARTESIAN_POINT('Ctrl Pts',(-22.1537501391487,-11.4234058771742,
0.));
#232623=CARTESIAN_POINT('Ctrl Pts',(-22.1537501391487,-11.4234058771742,
12.));
#232624=CARTESIAN_POINT('Ctrl Pts',(-22.1383729640964,-11.4034288076908,
0.));
#232625=CARTESIAN_POINT('Ctrl Pts',(-22.1383729640964,-11.4034288076908,
12.));
#232626=CARTESIAN_POINT('Ctrl Pts',(-22.1229978500186,-11.3835526044256,
0.));
#232627=CARTESIAN_POINT('Ctrl Pts',(-22.1229978500186,-11.3835526044256,
12.));
#232628=CARTESIAN_POINT('Ctrl Pts',(-22.1076253283979,-11.3637775035367,
0.));
#232629=CARTESIAN_POINT('Ctrl Pts',(-22.1076253283979,-11.3637775035367,
12.));
#232630=CARTESIAN_POINT('Ctrl Pts',(-22.0922559355294,-11.3441037419553,
0.));
#232631=CARTESIAN_POINT('Ctrl Pts',(-22.0922559355294,-11.3441037419553,
12.));
#232632=CARTESIAN_POINT('Ctrl Pts',(-22.0768902124267,-11.3245315573168,
0.));
#232633=CARTESIAN_POINT('Ctrl Pts',(-22.0768902124267,-11.3245315573168,
12.));
#232634=CARTESIAN_POINT('Ctrl Pts',(-22.0615287047179,-11.3050611878771,
0.));
#232635=CARTESIAN_POINT('Ctrl Pts',(-22.0615287047179,-11.3050611878771,
12.));
#232636=CARTESIAN_POINT('Ctrl Pts',(-22.046171962566,-11.2856928724374,
0.));
#232637=CARTESIAN_POINT('Ctrl Pts',(-22.046171962566,-11.2856928724374,
12.));
#232638=CARTESIAN_POINT('Ctrl Pts',(-22.030820540835,-11.2664268504206,
0.));
#232639=CARTESIAN_POINT('Ctrl Pts',(-22.030820540835,-11.2664268504206,
12.));
#232640=CARTESIAN_POINT('Ctrl Pts',(-22.0154749992363,-11.2472633619275,
0.));
#232641=CARTESIAN_POINT('Ctrl Pts',(-22.0154749992363,-11.2472633619275,
12.));
#232642=CARTESIAN_POINT('Ctrl Pts',(-22.0001359024839,-11.2282026477896,
0.));
#232643=CARTESIAN_POINT('Ctrl Pts',(-22.0001359024839,-11.2282026477896,
12.));
#232644=CARTESIAN_POINT('Ctrl Pts',(-21.9848038204439,-11.2092449496125,
0.));
#232645=CARTESIAN_POINT('Ctrl Pts',(-21.9848038204439,-11.2092449496125,
12.));
#232646=CARTESIAN_POINT('Ctrl Pts',(-21.9694793282914,-11.190390509811,
0.));
#232647=CARTESIAN_POINT('Ctrl Pts',(-21.9694793282914,-11.190390509811,
12.));
#232648=CARTESIAN_POINT('Ctrl Pts',(-21.9541630066506,-11.1716395716376,
0.));
#232649=CARTESIAN_POINT('Ctrl Pts',(-21.9541630066506,-11.1716395716376,
12.));
#232650=CARTESIAN_POINT('Ctrl Pts',(-21.9388554416439,-11.1529923792003,
0.));
#232651=CARTESIAN_POINT('Ctrl Pts',(-21.9388554416439,-11.1529923792003,
12.));
#232652=CARTESIAN_POINT('Ctrl Pts',(-21.923557224952,-11.1344491774741,
0.));
#232653=CARTESIAN_POINT('Ctrl Pts',(-21.923557224952,-11.1344491774741,
12.));
#232654=CARTESIAN_POINT('Ctrl Pts',(-21.9082689538688,-11.1160102123024,
0.));
#232655=CARTESIAN_POINT('Ctrl Pts',(-21.9082689538688,-11.1160102123024,
12.));
#232656=CARTESIAN_POINT('Ctrl Pts',(-21.8929912313608,-11.0976757303944,
0.));
#232657=CARTESIAN_POINT('Ctrl Pts',(-21.8929912313608,-11.0976757303944,
12.));
#232658=CARTESIAN_POINT('Ctrl Pts',(-21.877724666119,-11.0794459793057,
0.));
#232659=CARTESIAN_POINT('Ctrl Pts',(-21.877724666119,-11.0794459793057,
12.));
#232660=CARTESIAN_POINT('Ctrl Pts',(-21.8624698726318,-11.0613212074363,
0.));
#232661=CARTESIAN_POINT('Ctrl Pts',(-21.8624698726318,-11.0613212074363,
12.));
#232662=CARTESIAN_POINT('Ctrl Pts',(-21.8472274713103,-11.0433016640807,
0.));
#232663=CARTESIAN_POINT('Ctrl Pts',(-21.8472274713103,-11.0433016640807,
12.));
#232664=CARTESIAN_POINT('Ctrl Pts',(-21.8319980886033,-11.0253875994598,
0.));
#232665=CARTESIAN_POINT('Ctrl Pts',(-21.8319980886033,-11.0253875994598,
12.));
#232666=CARTESIAN_POINT('Ctrl Pts',(-21.8167823571168,-11.0075792647477,
0.));
#232667=CARTESIAN_POINT('Ctrl Pts',(-21.8167823571168,-11.0075792647477,
12.));
#232668=CARTESIAN_POINT('Ctrl Pts',(-21.8015809157301,-10.9898769120912,
0.));
#232669=CARTESIAN_POINT('Ctrl Pts',(-21.8015809157301,-10.9898769120912,
12.));
#232670=CARTESIAN_POINT('Ctrl Pts',(-21.7863944097141,-10.9722807946155,
0.));
#232671=CARTESIAN_POINT('Ctrl Pts',(-21.7863944097141,-10.9722807946155,
12.));
#232672=CARTESIAN_POINT('Ctrl Pts',(-21.7712234908464,-10.9547911664455,
0.));
#232673=CARTESIAN_POINT('Ctrl Pts',(-21.7712234908464,-10.9547911664455,
12.));
#232674=CARTESIAN_POINT('Ctrl Pts',(-21.7560688175247,-10.9374082827444,
0.));
#232675=CARTESIAN_POINT('Ctrl Pts',(-21.7560688175247,-10.9374082827444,
12.));
#232676=CARTESIAN_POINT('Ctrl Pts',(-21.7409310548797,-10.9201323997384,
0.));
#232677=CARTESIAN_POINT('Ctrl Pts',(-21.7409310548797,-10.9201323997384,
12.));
#232678=CARTESIAN_POINT('Ctrl Pts',(-21.7258108748873,-10.902963774734,
0.));
#232679=CARTESIAN_POINT('Ctrl Pts',(-21.7258108748873,-10.902963774734,
12.));
#232680=CARTESIAN_POINT('Ctrl Pts',(-21.7107089564825,-10.8859026661293,
0.));
#232681=CARTESIAN_POINT('Ctrl Pts',(-21.7107089564825,-10.8859026661293,
12.));
#232682=CARTESIAN_POINT('Ctrl Pts',(-21.6956259856672,-10.8689493334095,
0.));
#232683=CARTESIAN_POINT('Ctrl Pts',(-21.6956259856672,-10.8689493334095,
12.));
#232684=CARTESIAN_POINT('Ctrl Pts',(-21.6805626556467,-10.8521040371835,
0.));
#232685=CARTESIAN_POINT('Ctrl Pts',(-21.6805626556467,-10.8521040371835,
12.));
#232686=CARTESIAN_POINT('Ctrl Pts',(-21.6655196669732,-10.8353670392272,
0.));
#232687=CARTESIAN_POINT('Ctrl Pts',(-21.6655196669732,-10.8353670392272,
12.));
#232688=CARTESIAN_POINT('Ctrl Pts',(-21.6504977276866,-10.8187386025136,
0.));
#232689=CARTESIAN_POINT('Ctrl Pts',(-21.6504977276866,-10.8187386025136,
12.));
#232690=CARTESIAN_POINT('Ctrl Pts',(-21.6354975534557,-10.8022189912369,
0.));
#232691=CARTESIAN_POINT('Ctrl Pts',(-21.6354975534557,-10.8022189912369,
12.));
#232692=CARTESIAN_POINT('Ctrl Pts',(-21.6205198677173,-10.7858084708261,
0.));
#232693=CARTESIAN_POINT('Ctrl Pts',(-21.6205198677173,-10.7858084708261,
12.));
#232694=CARTESIAN_POINT('Ctrl Pts',(-21.6055654018176,-10.7695073079552,
0.));
#232695=CARTESIAN_POINT('Ctrl Pts',(-21.6055654018176,-10.7695073079552,
12.));
#232696=CARTESIAN_POINT('Ctrl Pts',(-21.5906348951743,-10.7533157705941,
0.));
#232697=CARTESIAN_POINT('Ctrl Pts',(-21.5906348951743,-10.7533157705941,
12.));
#232698=CARTESIAN_POINT('Ctrl Pts',(-21.5757290954371,-10.7372341280467,
0.));
#232699=CARTESIAN_POINT('Ctrl Pts',(-21.5757290954371,-10.7372341280467,
12.));
#232700=CARTESIAN_POINT('Ctrl Pts',(-21.5608487586468,-10.7212626509816,
0.));
#232701=CARTESIAN_POINT('Ctrl Pts',(-21.5608487586468,-10.7212626509816,
12.));
#232702=CARTESIAN_POINT('Ctrl Pts',(-21.5459946493955,-10.7054016114571,
0.));
#232703=CARTESIAN_POINT('Ctrl Pts',(-21.5459946493955,-10.7054016114571,
12.));
#232704=CARTESIAN_POINT('Ctrl Pts',(-21.5311675409807,-10.689651282929,
0.));
#232705=CARTESIAN_POINT('Ctrl Pts',(-21.5311675409807,-10.689651282929,
12.));
#232706=CARTESIAN_POINT('Ctrl Pts',(-21.51636821558,-10.6740119402834,0.));
#232707=CARTESIAN_POINT('Ctrl Pts',(-21.51636821558,-10.6740119402834,12.));
#232708=CARTESIAN_POINT('Ctrl Pts',(-21.5015974644449,-10.6584838598939,
0.));
#232709=CARTESIAN_POINT('Ctrl Pts',(-21.5015974644449,-10.6584838598939,
12.));
#232710=CARTESIAN_POINT('Ctrl Pts',(-21.4868560880889,-10.6430673196607,
0.));
#232711=CARTESIAN_POINT('Ctrl Pts',(-21.4868560880889,-10.6430673196607,
12.));
#232712=CARTESIAN_POINT('Ctrl Pts',(-21.4721448964766,-10.6277625990456,
0.));
#232713=CARTESIAN_POINT('Ctrl Pts',(-21.4721448964766,-10.6277625990456,
12.));
#232714=CARTESIAN_POINT('Ctrl Pts',(-21.4574647092097,-10.6125699790961,
0.));
#232715=CARTESIAN_POINT('Ctrl Pts',(-21.4574647092097,-10.6125699790961,
12.));
#232716=CARTESIAN_POINT('Ctrl Pts',(-21.4428163557144,-10.5974897424622,
0.));
#232717=CARTESIAN_POINT('Ctrl Pts',(-21.4428163557144,-10.5974897424622,
12.));
#232718=CARTESIAN_POINT('Ctrl Pts',(-21.4282006754631,-10.5825221734573,
0.));
#232719=CARTESIAN_POINT('Ctrl Pts',(-21.4282006754631,-10.5825221734573,
12.));
#232720=CARTESIAN_POINT('Ctrl Pts',(-21.4136185181979,-10.5676675581108,
0.));
#232721=CARTESIAN_POINT('Ctrl Pts',(-21.4136185181979,-10.5676675581108,
12.));
#232722=CARTESIAN_POINT('Ctrl Pts',(-21.3990707441497,-10.5529261842108,
0.));
#232723=CARTESIAN_POINT('Ctrl Pts',(-21.3990707441497,-10.5529261842108,
12.));
#232724=CARTESIAN_POINT('Ctrl Pts',(-21.3845582242602,-10.5382983413421,
0.));
#232725=CARTESIAN_POINT('Ctrl Pts',(-21.3845582242602,-10.5382983413421,
12.));
#232726=CARTESIAN_POINT('Ctrl Pts',(-21.3700818403936,-10.5237843209057,
0.));
#232727=CARTESIAN_POINT('Ctrl Pts',(-21.3700818403936,-10.5237843209057,
12.));
#232728=CARTESIAN_POINT('Ctrl Pts',(-21.3556424855814,-10.5093844161685,
0.));
#232729=CARTESIAN_POINT('Ctrl Pts',(-21.3556424855814,-10.5093844161685,
12.));
#232730=CARTESIAN_POINT('Ctrl Pts',(-21.3412410642904,-10.4950989223337,
0.));
#232731=CARTESIAN_POINT('Ctrl Pts',(-21.3412410642904,-10.4950989223337,
12.));
#232732=CARTESIAN_POINT('Ctrl Pts',(-21.3268784926819,-10.4809281365931,
0.));
#232733=CARTESIAN_POINT('Ctrl Pts',(-21.3268784926819,-10.4809281365931,
12.));
#232734=CARTESIAN_POINT('Ctrl Pts',(-21.3125556988731,-10.4668723581768,
0.));
#232735=CARTESIAN_POINT('Ctrl Pts',(-21.3125556988731,-10.4668723581768,
12.));
#232736=CARTESIAN_POINT('Ctrl Pts',(-21.2982736231931,-10.4529318883874,
0.));
#232737=CARTESIAN_POINT('Ctrl Pts',(-21.2982736231931,-10.4529318883874,
12.));
#232738=CARTESIAN_POINT('Ctrl Pts',(-21.2840332184483,-10.4391070306391,
0.));
#232739=CARTESIAN_POINT('Ctrl Pts',(-21.2840332184483,-10.4391070306391,
12.));
#232740=CARTESIAN_POINT('Ctrl Pts',(-21.2698354502403,-10.42539809054,0.));
#232741=CARTESIAN_POINT('Ctrl Pts',(-21.2698354502403,-10.42539809054,12.));
#232742=CARTESIAN_POINT('Ctrl Pts',(-21.255681297275,-10.4118053759588,
0.));
#232743=CARTESIAN_POINT('Ctrl Pts',(-21.255681297275,-10.4118053759588,
12.));
#232744=CARTESIAN_POINT('Ctrl Pts',(-21.2415717516714,-10.3983291970846,
0.));
#232745=CARTESIAN_POINT('Ctrl Pts',(-21.2415717516714,-10.3983291970846,
12.));
#232746=CARTESIAN_POINT('Ctrl Pts',(-21.22750781927,-10.3849698664786,0.));
#232747=CARTESIAN_POINT('Ctrl Pts',(-21.22750781927,-10.3849698664786,12.));
#232748=CARTESIAN_POINT('Ctrl Pts',(-21.2134905199345,-10.371727699113,
0.));
#232749=CARTESIAN_POINT('Ctrl Pts',(-21.2134905199345,-10.371727699113,
12.));
#232750=CARTESIAN_POINT('Ctrl Pts',(-21.199520887919,-10.3586030124587,
0.));
#232751=CARTESIAN_POINT('Ctrl Pts',(-21.199520887919,-10.3586030124587,
12.));
#232752=CARTESIAN_POINT('Ctrl Pts',(-21.1855999722416,-10.34559612657,0.));
#232753=CARTESIAN_POINT('Ctrl Pts',(-21.1855999722416,-10.34559612657,12.));
#232754=CARTESIAN_POINT('Ctrl Pts',(-21.1717288370509,-10.3327073641572,
0.));
#232755=CARTESIAN_POINT('Ctrl Pts',(-21.1717288370509,-10.3327073641572,
12.));
#232756=CARTESIAN_POINT('Ctrl Pts',(-21.1579085619965,-10.3199370506544,
0.));
#232757=CARTESIAN_POINT('Ctrl Pts',(-21.1579085619965,-10.3199370506544,
12.));
#232758=CARTESIAN_POINT('Ctrl Pts',(-21.1441402425843,-10.3072855142687,
0.));
#232759=CARTESIAN_POINT('Ctrl Pts',(-21.1441402425843,-10.3072855142687,
12.));
#232760=CARTESIAN_POINT('Ctrl Pts',(-21.1304249906002,-10.2947530860721,
0.));
#232761=CARTESIAN_POINT('Ctrl Pts',(-21.1304249906002,-10.2947530860721,
12.));
#232762=CARTESIAN_POINT('Ctrl Pts',(-21.1167639345631,-10.2823401001072,
0.));
#232763=CARTESIAN_POINT('Ctrl Pts',(-21.1167639345631,-10.2823401001072,
12.));
#232764=CARTESIAN_POINT('Ctrl Pts',(-21.1031582201627,-10.2700468934744,
0.));
#232765=CARTESIAN_POINT('Ctrl Pts',(-21.1031582201627,-10.2700468934744,
12.));
#232766=CARTESIAN_POINT('Ctrl Pts',(-21.0896090107063,-10.2578738064181,
0.));
#232767=CARTESIAN_POINT('Ctrl Pts',(-21.0896090107063,-10.2578738064181,
12.));
#232768=CARTESIAN_POINT('Ctrl Pts',(-21.0761174875445,-10.2458211823912,
0.));
#232769=CARTESIAN_POINT('Ctrl Pts',(-21.0761174875445,-10.2458211823912,
12.));
#232770=CARTESIAN_POINT('Ctrl Pts',(-21.0626848505663,-10.2338893681567,
0.));
#232771=CARTESIAN_POINT('Ctrl Pts',(-21.0626848505663,-10.2338893681567,
12.));
#232772=CARTESIAN_POINT('Ctrl Pts',(-21.0493123187483,-10.2220787139154,
0.));
#232773=CARTESIAN_POINT('Ctrl Pts',(-21.0493123187483,-10.2220787139154,
12.));
#232774=CARTESIAN_POINT('Ctrl Pts',(-21.0360011306815,-10.2103895734123,
0.));
#232775=CARTESIAN_POINT('Ctrl Pts',(-21.0360011306815,-10.2103895734123,
12.));
#232776=CARTESIAN_POINT('Ctrl Pts',(-21.0227525451107,-10.1988223040425,
0.));
#232777=CARTESIAN_POINT('Ctrl Pts',(-21.0227525451107,-10.1988223040425,
12.));
#232778=CARTESIAN_POINT('Ctrl Pts',(-21.0095678414486,-10.187377266936,
0.));
#232779=CARTESIAN_POINT('Ctrl Pts',(-21.0095678414486,-10.187377266936,
12.));
#232780=CARTESIAN_POINT('Ctrl Pts',(-20.9964483203686,-10.1760548270767,
0.));
#232781=CARTESIAN_POINT('Ctrl Pts',(-20.9964483203686,-10.1760548270767,
12.));
#232782=CARTESIAN_POINT('Ctrl Pts',(-20.9833953044736,-10.1648553534568,
0.));
#232783=CARTESIAN_POINT('Ctrl Pts',(-20.9833953044736,-10.1648553534568,
12.));
#232784=CARTESIAN_POINT('Ctrl Pts',(-20.9704101389369,-10.1537792192065,
0.));
#232785=CARTESIAN_POINT('Ctrl Pts',(-20.9704101389369,-10.1537792192065,
12.));
#232786=CARTESIAN_POINT('Ctrl Pts',(-20.9574941921591,-10.1428268017256,
0.));
#232787=CARTESIAN_POINT('Ctrl Pts',(-20.9574941921591,-10.1428268017256,
12.));
#232788=CARTESIAN_POINT('Ctrl Pts',(-20.9446488563933,-10.1319984827908,
0.));
#232789=CARTESIAN_POINT('Ctrl Pts',(-20.9446488563933,-10.1319984827908,
12.));
#232790=CARTESIAN_POINT('Ctrl Pts',(-20.9318755484734,-10.1212946487057,
0.));
#232791=CARTESIAN_POINT('Ctrl Pts',(-20.9318755484734,-10.1212946487057,
12.));
#232792=CARTESIAN_POINT('Ctrl Pts',(-20.919175710627,-10.1107156904836,
0.));
#232793=CARTESIAN_POINT('Ctrl Pts',(-20.919175710627,-10.1107156904836,
12.));
#232794=CARTESIAN_POINT('Ctrl Pts',(-20.9065508112557,-10.1002620040076,
0.));
#232795=CARTESIAN_POINT('Ctrl Pts',(-20.9065508112557,-10.1002620040076,
12.));
#232796=CARTESIAN_POINT('Ctrl Pts',(-20.894002345737,-10.0899339901915,
0.));
#232797=CARTESIAN_POINT('Ctrl Pts',(-20.894002345737,-10.0899339901915,
12.));
#232798=CARTESIAN_POINT('Ctrl Pts',(-20.881531837184,-10.0797320551154,
0.));
#232799=CARTESIAN_POINT('Ctrl Pts',(-20.881531837184,-10.0797320551154,
12.));
#232800=CARTESIAN_POINT('Ctrl Pts',(-20.86914083737,-10.0696566102218,0.));
#232801=CARTESIAN_POINT('Ctrl Pts',(-20.86914083737,-10.0696566102218,12.));
#232802=CARTESIAN_POINT('Ctrl Pts',(-20.8568309277316,-10.0597080725375,
0.));
#232803=CARTESIAN_POINT('Ctrl Pts',(-20.8568309277316,-10.0597080725375,
12.));
#232804=CARTESIAN_POINT('Ctrl Pts',(-20.8446037203402,-10.0498868648733,
0.));
#232805=CARTESIAN_POINT('Ctrl Pts',(-20.8446037203402,-10.0498868648733,
12.));
#232806=CARTESIAN_POINT('Ctrl Pts',(-20.8324608588909,-10.0401934160234,
0.));
#232807=CARTESIAN_POINT('Ctrl Pts',(-20.8324608588909,-10.0401934160234,
12.));
#232808=CARTESIAN_POINT('Ctrl Pts',(-20.8204040196602,-10.0306281609435,
0.));
#232809=CARTESIAN_POINT('Ctrl Pts',(-20.8204040196602,-10.0306281609435,
12.));
#232810=CARTESIAN_POINT('Ctrl Pts',(-20.8084349126888,-10.0211915410095,
0.));
#232811=CARTESIAN_POINT('Ctrl Pts',(-20.8084349126888,-10.0211915410095,
12.));
#232812=CARTESIAN_POINT('Ctrl Pts',(-20.7965552829908,-10.0118840042786,
0.));
#232813=CARTESIAN_POINT('Ctrl Pts',(-20.7965552829908,-10.0118840042786,
12.));
#232814=CARTESIAN_POINT('Ctrl Pts',(-20.7847669117568,-10.0027060057389,
0.));
#232815=CARTESIAN_POINT('Ctrl Pts',(-20.7847669117568,-10.0027060057389,
12.));
#232816=CARTESIAN_POINT('Ctrl Pts',(-20.7730716175417,-9.9936580075464,
0.));
#232817=CARTESIAN_POINT('Ctrl Pts',(-20.7730716175417,-9.9936580075464,
12.));
#232818=CARTESIAN_POINT('Ctrl Pts',(-20.761471257499,-9.98474047926852,
0.));
#232819=CARTESIAN_POINT('Ctrl Pts',(-20.761471257499,-9.98474047926852,
12.));
#232820=CARTESIAN_POINT('Ctrl Pts',(-20.7499677289627,-9.9759538982347,
0.));
#232821=CARTESIAN_POINT('Ctrl Pts',(-20.7499677289627,-9.9759538982347,
12.));
#232822=CARTESIAN_POINT('Ctrl Pts',(-20.7385629709795,-9.96729874986201,
0.));
#232823=CARTESIAN_POINT('Ctrl Pts',(-20.7385629709795,-9.96729874986201,
12.));
#232824=CARTESIAN_POINT('Ctrl Pts',(-20.7272589658751,-9.95877552798397,
0.));
#232825=CARTESIAN_POINT('Ctrl Pts',(-20.7272589658751,-9.95877552798397,
12.));
#232826=CARTESIAN_POINT('Ctrl Pts',(-20.7160577407579,-9.95038473514948,
0.));
#232827=CARTESIAN_POINT('Ctrl Pts',(-20.7160577407579,-9.95038473514948,
12.));
#232828=CARTESIAN_POINT('Ctrl Pts',(-20.7049613692234,-9.94212688298236,
0.));
#232829=CARTESIAN_POINT('Ctrl Pts',(-20.7049613692234,-9.94212688298236,
12.));
#232830=CARTESIAN_POINT('Ctrl Pts',(-20.6939719732484,-9.93400249259729,
0.));
#232831=CARTESIAN_POINT('Ctrl Pts',(-20.6939719732484,-9.93400249259729,
12.));
#232832=CARTESIAN_POINT('Ctrl Pts',(-20.6830917250255,-9.92601209498748,
0.));
#232833=CARTESIAN_POINT('Ctrl Pts',(-20.6830917250255,-9.92601209498748,
12.));
#232834=CARTESIAN_POINT('Ctrl Pts',(-20.6723228488263,-9.91815623141288,
0.));
#232835=CARTESIAN_POINT('Ctrl Pts',(-20.6723228488263,-9.91815623141288,
12.));
#232836=CARTESIAN_POINT('Ctrl Pts',(-20.6616676228315,-9.91043545377007,
0.));
#232837=CARTESIAN_POINT('Ctrl Pts',(-20.6616676228315,-9.91043545377007,
12.));
#232838=CARTESIAN_POINT('Ctrl Pts',(-20.6511283817414,-9.90285032516692,
0.));
#232839=CARTESIAN_POINT('Ctrl Pts',(-20.6511283817414,-9.90285032516692,
12.));
#232840=CARTESIAN_POINT('Ctrl Pts',(-20.6407075193976,-9.89540142049119,
0.));
#232841=CARTESIAN_POINT('Ctrl Pts',(-20.6407075193976,-9.89540142049119,
12.));
#232842=CARTESIAN_POINT('Ctrl Pts',(-20.6304074914087,-9.88808932697306,
0.));
#232843=CARTESIAN_POINT('Ctrl Pts',(-20.6304074914087,-9.88808932697306,
12.));
#232844=CARTESIAN_POINT('Ctrl Pts',(-20.6202308177474,-9.88091464472675,
0.));
#232845=CARTESIAN_POINT('Ctrl Pts',(-20.6202308177474,-9.88091464472675,
12.));
#232846=CARTESIAN_POINT('Ctrl Pts',(-20.6101800854494,-9.87387798732956,
0.));
#232847=CARTESIAN_POINT('Ctrl Pts',(-20.6101800854494,-9.87387798732956,
12.));
#232848=CARTESIAN_POINT('Ctrl Pts',(-20.6002579513699,-9.86697998242622,
0.));
#232849=CARTESIAN_POINT('Ctrl Pts',(-20.6002579513699,-9.86697998242622,
12.));
#232850=CARTESIAN_POINT('Ctrl Pts',(-20.5904671449754,-9.86022127232747,
0.));
#232851=CARTESIAN_POINT('Ctrl Pts',(-20.5904671449754,-9.86022127232747,
12.));
#232852=CARTESIAN_POINT('Ctrl Pts',(-20.5808104710015,-9.8536025145698,
0.));
#232853=CARTESIAN_POINT('Ctrl Pts',(-20.5808104710015,-9.8536025145698,
12.));
#232854=CARTESIAN_POINT('Ctrl Pts',(-20.5712908125139,-9.84712438256277,
0.));
#232855=CARTESIAN_POINT('Ctrl Pts',(-20.5712908125139,-9.84712438256277,
12.));
#232856=CARTESIAN_POINT('Ctrl Pts',(-20.5619111362402,-9.84078756677565,
0.));
#232857=CARTESIAN_POINT('Ctrl Pts',(-20.5619111362402,-9.84078756677565,
12.));
#232858=CARTESIAN_POINT('Ctrl Pts',(-20.552674497646,-9.83459277585315,
0.));
#232859=CARTESIAN_POINT('Ctrl Pts',(-20.552674497646,-9.83459277585315,
12.));
#232860=CARTESIAN_POINT('Ctrl Pts',(-20.5435840460721,-9.82854073773877,
0.));
#232861=CARTESIAN_POINT('Ctrl Pts',(-20.5435840460721,-9.82854073773877,
12.));
#232862=CARTESIAN_POINT('Ctrl Pts',(-20.5346430299517,-9.82263220080362,
0.));
#232863=CARTESIAN_POINT('Ctrl Pts',(-20.5346430299517,-9.82263220080362,
12.));
#232864=CARTESIAN_POINT('Ctrl Pts',(-20.5258548000629,-9.81686793455942,
0.));
#232865=CARTESIAN_POINT('Ctrl Pts',(-20.5258548000629,-9.81686793455942,
12.));
#232866=CARTESIAN_POINT('Ctrl Pts',(-20.517222812284,-9.81124873025281,
0.));
#232867=CARTESIAN_POINT('Ctrl Pts',(-20.517222812284,-9.81124873025281,
12.));
#232868=CARTESIAN_POINT('Ctrl Pts',(-20.5087506310505,-9.80577540161087,
0.));
#232869=CARTESIAN_POINT('Ctrl Pts',(-20.5087506310505,-9.80577540161087,
12.));
#232870=CARTESIAN_POINT('Ctrl Pts',(-20.5004419312107,-9.80044878520948,
0.));
#232871=CARTESIAN_POINT('Ctrl Pts',(-20.5004419312107,-9.80044878520948,
12.));
#232872=CARTESIAN_POINT('Ctrl Pts',(-20.4923005087943,-9.7952697428833,
0.));
#232873=CARTESIAN_POINT('Ctrl Pts',(-20.4923005087943,-9.7952697428833,
12.));
#232874=CARTESIAN_POINT('Ctrl Pts',(-20.4843302955329,-9.79023916498655,
0.));
#232875=CARTESIAN_POINT('Ctrl Pts',(-20.4843302955329,-9.79023916498655,
12.));
#232876=CARTESIAN_POINT('Ctrl Pts',(-20.4765353711586,-9.78535797314166,
0.));
#232877=CARTESIAN_POINT('Ctrl Pts',(-20.4765353711586,-9.78535797314166,
12.));
#232878=CARTESIAN_POINT('Ctrl Pts',(-20.4689199790669,-9.7806271237332,
0.));
#232879=CARTESIAN_POINT('Ctrl Pts',(-20.4689199790669,-9.7806271237332,
12.));
#232880=CARTESIAN_POINT('Ctrl Pts',(-20.4614885274975,-9.77604760815528,
0.));
#232881=CARTESIAN_POINT('Ctrl Pts',(-20.4614885274975,-9.77604760815528,
12.));
#232882=CARTESIAN_POINT('Ctrl Pts',(-20.4542455817527,-9.77162045104069,
0.));
#232883=CARTESIAN_POINT('Ctrl Pts',(-20.4542455817527,-9.77162045104069,
12.));
#232884=CARTESIAN_POINT('Ctrl Pts',(-20.447195862298,-9.76734670980891,
0.));
#232885=CARTESIAN_POINT('Ctrl Pts',(-20.447195862298,-9.76734670980891,
12.));
#232886=CARTESIAN_POINT('Ctrl Pts',(-20.44034423294,-9.76322747195494,0.));
#232887=CARTESIAN_POINT('Ctrl Pts',(-20.44034423294,-9.76322747195494,12.));
#232888=CARTESIAN_POINT('Ctrl Pts',(-20.4336957355473,-9.75926386289922,
0.));
#232889=CARTESIAN_POINT('Ctrl Pts',(-20.4336957355473,-9.75926386289922,
12.));
#232890=CARTESIAN_POINT('Ctrl Pts',(-20.4272556476629,-9.75545705902417,
0.));
#232891=CARTESIAN_POINT('Ctrl Pts',(-20.4272556476629,-9.75545705902417,
12.));
#232892=CARTESIAN_POINT('Ctrl Pts',(-20.4210295275817,-9.7518082978643,
0.));
#232893=CARTESIAN_POINT('Ctrl Pts',(-20.4210295275817,-9.7518082978643,
12.));
#232894=CARTESIAN_POINT('Ctrl Pts',(-20.4150232777393,-9.74831889242174,
0.));
#232895=CARTESIAN_POINT('Ctrl Pts',(-20.4150232777393,-9.74831889242174,
12.));
#232896=CARTESIAN_POINT('Ctrl Pts',(-20.4092430879861,-9.74499021838537,
0.));
#232897=CARTESIAN_POINT('Ctrl Pts',(-20.4092430879861,-9.74499021838537,
12.));
#232898=CARTESIAN_POINT('Ctrl Pts',(-20.4036953576549,-9.74182369656271,
0.));
#232899=CARTESIAN_POINT('Ctrl Pts',(-20.4036953576549,-9.74182369656271,
12.));
#232900=CARTESIAN_POINT('Ctrl Pts',(-20.3983866213331,-9.738820776132,0.));
#232901=CARTESIAN_POINT('Ctrl Pts',(-20.3983866213331,-9.738820776132,12.));
#232902=CARTESIAN_POINT('Ctrl Pts',(-20.3933234845647,-9.73598292014242,
0.));
#232903=CARTESIAN_POINT('Ctrl Pts',(-20.3933234845647,-9.73598292014242,
12.));
#232904=CARTESIAN_POINT('Ctrl Pts',(-20.3885129129912,-9.73331167102807,
0.));
#232905=CARTESIAN_POINT('Ctrl Pts',(-20.3885129129912,-9.73331167102807,
12.));
#232906=CARTESIAN_POINT('Ctrl Pts',(-20.3839624556742,-9.73080870123727,
0.));
#232907=CARTESIAN_POINT('Ctrl Pts',(-20.3839624556742,-9.73080870123727,
12.));
#232908=CARTESIAN_POINT('Ctrl Pts',(-20.3796805893304,-9.72847589116541,
0.));
#232909=CARTESIAN_POINT('Ctrl Pts',(-20.3796805893304,-9.72847589116541,
12.));
#232910=CARTESIAN_POINT('Ctrl Pts',(-20.3756766651951,-9.7263153173288,
0.));
#232911=CARTESIAN_POINT('Ctrl Pts',(-20.3756766651951,-9.7263153173288,
12.));
#232912=CARTESIAN_POINT('Ctrl Pts',(-20.371960235676,-9.72432910043194,
0.));
#232913=CARTESIAN_POINT('Ctrl Pts',(-20.371960235676,-9.72432910043194,
12.));
#232914=CARTESIAN_POINT('Ctrl Pts',(-20.3685406190576,-9.72251930722489,
0.));
#232915=CARTESIAN_POINT('Ctrl Pts',(-20.3685406190576,-9.72251930722489,
12.));
#232916=CARTESIAN_POINT('Ctrl Pts',(-20.3654261611056,-9.7208877838108,
0.));
#232917=CARTESIAN_POINT('Ctrl Pts',(-20.3654261611056,-9.7208877838108,
12.));
#232918=CARTESIAN_POINT('Ctrl Pts',(-20.3626256913981,-9.71943648548099,
0.));
#232919=CARTESIAN_POINT('Ctrl Pts',(-20.3626256913981,-9.71943648548099,
12.));
#232920=CARTESIAN_POINT('Ctrl Pts',(-20.3601498764344,-9.71816778328006,
0.));
#232921=CARTESIAN_POINT('Ctrl Pts',(-20.3601498764344,-9.71816778328006,
12.));
#232922=CARTESIAN_POINT('Ctrl Pts',(-20.3580133103356,-9.71708493723096,
0.));
#232923=CARTESIAN_POINT('Ctrl Pts',(-20.3580133103356,-9.71708493723096,
12.));
#232924=CARTESIAN_POINT('Ctrl Pts',(-20.3562337557875,-9.71619192554185,
0.));
#232925=CARTESIAN_POINT('Ctrl Pts',(-20.3562337557875,-9.71619192554185,
12.));
#232926=CARTESIAN_POINT('Ctrl Pts',(-20.3548282742361,-9.71549257088172,
0.));
#232927=CARTESIAN_POINT('Ctrl Pts',(-20.3548282742361,-9.71549257088172,
12.));
#232928=CARTESIAN_POINT('Ctrl Pts',(-20.3538098605706,-9.7149897805202,
0.));
#232929=CARTESIAN_POINT('Ctrl Pts',(-20.3538098605706,-9.7149897805202,
12.));
#232930=CARTESIAN_POINT('Ctrl Pts',(-20.3533097561886,-9.7147459035068,
0.));
#232931=CARTESIAN_POINT('Ctrl Pts',(-20.3533097561886,-9.7147459035068,
12.));
#232932=CARTESIAN_POINT('Ctrl Pts',(-20.3531126095522,-9.71465227853041,
0.));
#232933=CARTESIAN_POINT('Ctrl Pts',(-20.3531126095522,-9.71465227853041,
12.));
#232934=CARTESIAN_POINT('Ctrl Pts',(-20.353060251684,-9.71462954053041,
0.));
#232935=CARTESIAN_POINT('Ctrl Pts',(-20.353060251684,-9.71462954053041,
12.));
#232936=CARTESIAN_POINT('Ctrl Pts',(-20.353053841303,-9.71462809124915,
0.));
#232937=CARTESIAN_POINT('Ctrl Pts',(-20.353053841303,-9.71462809124915,
12.));
#232938=CARTESIAN_POINT('',(-22.8400320311649,-12.4230808101438,0.));
#232939=CARTESIAN_POINT('Ctrl Pts',(-22.8400320311649,-12.4230808101438,
0.));
#232940=CARTESIAN_POINT('Ctrl Pts',(-22.8370364396459,-12.418215285186,
0.));
#232941=CARTESIAN_POINT('Ctrl Pts',(-22.8310435872748,-12.4084933766346,
0.));
#232942=CARTESIAN_POINT('Ctrl Pts',(-22.8220493007173,-12.3939379378998,
0.));
#232943=CARTESIAN_POINT('Ctrl Pts',(-22.81004690224,-12.374585536673,0.));
#232944=CARTESIAN_POINT('Ctrl Pts',(-22.795027221673,-12.3504864740319,
0.));
#232945=CARTESIAN_POINT('Ctrl Pts',(-22.7799908974768,-12.3264788926075,
0.));
#232946=CARTESIAN_POINT('Ctrl Pts',(-22.764938010105,-12.3025628601792,
0.));
#232947=CARTESIAN_POINT('Ctrl Pts',(-22.7498686970069,-12.2787384750742,
0.));
#232948=CARTESIAN_POINT('Ctrl Pts',(-22.7347831655287,-12.2550058702395,
0.));
#232949=CARTESIAN_POINT('Ctrl Pts',(-22.7196817119374,-12.2313652198061,
0.));
#232950=CARTESIAN_POINT('Ctrl Pts',(-22.7045647168747,-12.2078167360284,
0.));
#232951=CARTESIAN_POINT('Ctrl Pts',(-22.6894326205037,-12.1843606579261,
0.));
#232952=CARTESIAN_POINT('Ctrl Pts',(-22.6742859034944,-12.1609972423099,
0.));
#232953=CARTESIAN_POINT('Ctrl Pts',(-22.6591250653965,-12.1377267537145,
0.));
#232954=CARTESIAN_POINT('Ctrl Pts',(-22.6439506046605,-12.1145494550383,
0.));
#232955=CARTESIAN_POINT('Ctrl Pts',(-22.6287629967056,-12.0914655972823,
0.));
#232956=CARTESIAN_POINT('Ctrl Pts',(-22.6135626764898,-12.0684754113862,
0.));
#232957=CARTESIAN_POINT('Ctrl Pts',(-22.5983500505644,-12.0455791139128,
0.));
#232958=CARTESIAN_POINT('Ctrl Pts',(-22.5831255061282,-12.0227769113127,
0.));
#232959=CARTESIAN_POINT('Ctrl Pts',(-22.5678894211181,-12.0000690046695,
0.));
#232960=CARTESIAN_POINT('Ctrl Pts',(-22.5526421741158,-11.9774555943496,
0.));
#232961=CARTESIAN_POINT('Ctrl Pts',(-22.5373841537307,-11.9549368843997,
0.));
#232962=CARTESIAN_POINT('Ctrl Pts',(-22.5221157697883,-11.9325130877803,
0.));
#232963=CARTESIAN_POINT('Ctrl Pts',(-22.5068374513973,-11.9101844254557,
0.));
#232964=CARTESIAN_POINT('Ctrl Pts',(-22.4915496418485,-11.8879511239942,
0.));
#232965=CARTESIAN_POINT('Ctrl Pts',(-22.4762527946702,-11.8658134137019,
0.));
#232966=CARTESIAN_POINT('Ctrl Pts',(-22.4609473690471,-11.8437715264487,
0.));
#232967=CARTESIAN_POINT('Ctrl Pts',(-22.4456338258735,-11.8218256937889,
0.));
#232968=CARTESIAN_POINT('Ctrl Pts',(-22.430312622646,-11.7999761445173,
0.));
#232969=CARTESIAN_POINT('Ctrl Pts',(-22.4149842125008,-11.7782231042039,
0.));
#232970=CARTESIAN_POINT('Ctrl Pts',(-22.3996490469191,-11.7565667964764,
0.));
#232971=CARTESIAN_POINT('Ctrl Pts',(-22.3843075773899,-11.7350074437961,
0.));
#232972=CARTESIAN_POINT('Ctrl Pts',(-22.3689602575491,-11.7135452684532,
0.));
#232973=CARTESIAN_POINT('Ctrl Pts',(-22.3536075450029,-11.6921804934056,
0.));
#232974=CARTESIAN_POINT('Ctrl Pts',(-22.3382499035619,-11.6709133432985,
0.));
#232975=CARTESIAN_POINT('Ctrl Pts',(-22.3228878043976,-11.6497440449857,
0.));
#232976=CARTESIAN_POINT('Ctrl Pts',(-22.3075217249049,-11.6286728270009,
0.));
#232977=CARTESIAN_POINT('Ctrl Pts',(-22.2921521480356,-11.6076999192357,
0.));
#232978=CARTESIAN_POINT('Ctrl Pts',(-22.2767795614348,-11.5868255525188,
0.));
#232979=CARTESIAN_POINT('Ctrl Pts',(-22.2614044566898,-11.5660499582403,
0.));
#232980=CARTESIAN_POINT('Ctrl Pts',(-22.2460273284654,-11.5453733679121,
0.));
#232981=CARTESIAN_POINT('Ctrl Pts',(-22.2306486738901,-11.5247960128477,
0.));
#232982=CARTESIAN_POINT('Ctrl Pts',(-22.2152689931022,-11.5043181244242,
0.));
#232983=CARTESIAN_POINT('Ctrl Pts',(-22.1998887896436,-11.483939934259,
0.));
#232984=CARTESIAN_POINT('Ctrl Pts',(-22.184508570917,-11.463661674411,0.));
#232985=CARTESIAN_POINT('Ctrl Pts',(-22.1691288486096,-11.443483577557,
0.));
#232986=CARTESIAN_POINT('Ctrl Pts',(-22.1537501391487,-11.4234058771742,
0.));
#232987=CARTESIAN_POINT('Ctrl Pts',(-22.1383729640964,-11.4034288076908,
0.));
#232988=CARTESIAN_POINT('Ctrl Pts',(-22.1229978500186,-11.3835526044256,
0.));
#232989=CARTESIAN_POINT('Ctrl Pts',(-22.1076253283979,-11.3637775035367,
0.));
#232990=CARTESIAN_POINT('Ctrl Pts',(-22.0922559355294,-11.3441037419553,
0.));
#232991=CARTESIAN_POINT('Ctrl Pts',(-22.0768902124267,-11.3245315573168,
0.));
#232992=CARTESIAN_POINT('Ctrl Pts',(-22.0615287047179,-11.3050611878771,
0.));
#232993=CARTESIAN_POINT('Ctrl Pts',(-22.046171962566,-11.2856928724374,
0.));
#232994=CARTESIAN_POINT('Ctrl Pts',(-22.030820540835,-11.2664268504206,
0.));
#232995=CARTESIAN_POINT('Ctrl Pts',(-22.0154749992363,-11.2472633619275,
0.));
#232996=CARTESIAN_POINT('Ctrl Pts',(-22.0001359024839,-11.2282026477896,
0.));
#232997=CARTESIAN_POINT('Ctrl Pts',(-21.9848038204439,-11.2092449496125,
0.));
#232998=CARTESIAN_POINT('Ctrl Pts',(-21.9694793282914,-11.190390509811,
0.));
#232999=CARTESIAN_POINT('Ctrl Pts',(-21.9541630066506,-11.1716395716376,
0.));
#233000=CARTESIAN_POINT('Ctrl Pts',(-21.9388554416439,-11.1529923792003,
0.));
#233001=CARTESIAN_POINT('Ctrl Pts',(-21.923557224952,-11.1344491774741,
0.));
#233002=CARTESIAN_POINT('Ctrl Pts',(-21.9082689538688,-11.1160102123024,
0.));
#233003=CARTESIAN_POINT('Ctrl Pts',(-21.8929912313608,-11.0976757303944,
0.));
#233004=CARTESIAN_POINT('Ctrl Pts',(-21.877724666119,-11.0794459793057,
0.));
#233005=CARTESIAN_POINT('Ctrl Pts',(-21.8624698726318,-11.0613212074363,
0.));
#233006=CARTESIAN_POINT('Ctrl Pts',(-21.8472274713103,-11.0433016640807,
0.));
#233007=CARTESIAN_POINT('Ctrl Pts',(-21.8319980886033,-11.0253875994598,
0.));
#233008=CARTESIAN_POINT('Ctrl Pts',(-21.8167823571168,-11.0075792647477,
0.));
#233009=CARTESIAN_POINT('Ctrl Pts',(-21.8015809157301,-10.9898769120912,
0.));
#233010=CARTESIAN_POINT('Ctrl Pts',(-21.7863944097141,-10.9722807946155,
0.));
#233011=CARTESIAN_POINT('Ctrl Pts',(-21.7712234908464,-10.9547911664455,
0.));
#233012=CARTESIAN_POINT('Ctrl Pts',(-21.7560688175247,-10.9374082827444,
0.));
#233013=CARTESIAN_POINT('Ctrl Pts',(-21.7409310548797,-10.9201323997384,
0.));
#233014=CARTESIAN_POINT('Ctrl Pts',(-21.7258108748873,-10.902963774734,
0.));
#233015=CARTESIAN_POINT('Ctrl Pts',(-21.7107089564825,-10.8859026661293,
0.));
#233016=CARTESIAN_POINT('Ctrl Pts',(-21.6956259856672,-10.8689493334095,
0.));
#233017=CARTESIAN_POINT('Ctrl Pts',(-21.6805626556467,-10.8521040371835,
0.));
#233018=CARTESIAN_POINT('Ctrl Pts',(-21.6655196669732,-10.8353670392272,
0.));
#233019=CARTESIAN_POINT('Ctrl Pts',(-21.6504977276866,-10.8187386025136,
0.));
#233020=CARTESIAN_POINT('Ctrl Pts',(-21.6354975534557,-10.8022189912369,
0.));
#233021=CARTESIAN_POINT('Ctrl Pts',(-21.6205198677173,-10.7858084708261,
0.));
#233022=CARTESIAN_POINT('Ctrl Pts',(-21.6055654018176,-10.7695073079552,
0.));
#233023=CARTESIAN_POINT('Ctrl Pts',(-21.5906348951743,-10.7533157705941,
0.));
#233024=CARTESIAN_POINT('Ctrl Pts',(-21.5757290954371,-10.7372341280467,
0.));
#233025=CARTESIAN_POINT('Ctrl Pts',(-21.5608487586468,-10.7212626509816,
0.));
#233026=CARTESIAN_POINT('Ctrl Pts',(-21.5459946493955,-10.7054016114571,
0.));
#233027=CARTESIAN_POINT('Ctrl Pts',(-21.5311675409807,-10.689651282929,
0.));
#233028=CARTESIAN_POINT('Ctrl Pts',(-21.51636821558,-10.6740119402834,0.));
#233029=CARTESIAN_POINT('Ctrl Pts',(-21.5015974644449,-10.6584838598939,
0.));
#233030=CARTESIAN_POINT('Ctrl Pts',(-21.4868560880889,-10.6430673196607,
0.));
#233031=CARTESIAN_POINT('Ctrl Pts',(-21.4721448964766,-10.6277625990456,
0.));
#233032=CARTESIAN_POINT('Ctrl Pts',(-21.4574647092097,-10.6125699790961,
0.));
#233033=CARTESIAN_POINT('Ctrl Pts',(-21.4428163557144,-10.5974897424622,
0.));
#233034=CARTESIAN_POINT('Ctrl Pts',(-21.4282006754631,-10.5825221734573,
0.));
#233035=CARTESIAN_POINT('Ctrl Pts',(-21.4136185181979,-10.5676675581108,
0.));
#233036=CARTESIAN_POINT('Ctrl Pts',(-21.3990707441497,-10.5529261842108,
0.));
#233037=CARTESIAN_POINT('Ctrl Pts',(-21.3845582242602,-10.5382983413421,
0.));
#233038=CARTESIAN_POINT('Ctrl Pts',(-21.3700818403936,-10.5237843209057,
0.));
#233039=CARTESIAN_POINT('Ctrl Pts',(-21.3556424855814,-10.5093844161685,
0.));
#233040=CARTESIAN_POINT('Ctrl Pts',(-21.3412410642904,-10.4950989223337,
0.));
#233041=CARTESIAN_POINT('Ctrl Pts',(-21.3268784926819,-10.4809281365931,
0.));
#233042=CARTESIAN_POINT('Ctrl Pts',(-21.3125556988731,-10.4668723581768,
0.));
#233043=CARTESIAN_POINT('Ctrl Pts',(-21.2982736231931,-10.4529318883874,
0.));
#233044=CARTESIAN_POINT('Ctrl Pts',(-21.2840332184483,-10.4391070306391,
0.));
#233045=CARTESIAN_POINT('Ctrl Pts',(-21.2698354502403,-10.42539809054,0.));
#233046=CARTESIAN_POINT('Ctrl Pts',(-21.255681297275,-10.4118053759588,
0.));
#233047=CARTESIAN_POINT('Ctrl Pts',(-21.2415717516714,-10.3983291970846,
0.));
#233048=CARTESIAN_POINT('Ctrl Pts',(-21.22750781927,-10.3849698664786,0.));
#233049=CARTESIAN_POINT('Ctrl Pts',(-21.2134905199345,-10.371727699113,
0.));
#233050=CARTESIAN_POINT('Ctrl Pts',(-21.199520887919,-10.3586030124587,
0.));
#233051=CARTESIAN_POINT('Ctrl Pts',(-21.1855999722416,-10.34559612657,0.));
#233052=CARTESIAN_POINT('Ctrl Pts',(-21.1717288370509,-10.3327073641572,
0.));
#233053=CARTESIAN_POINT('Ctrl Pts',(-21.1579085619965,-10.3199370506544,
0.));
#233054=CARTESIAN_POINT('Ctrl Pts',(-21.1441402425843,-10.3072855142687,
0.));
#233055=CARTESIAN_POINT('Ctrl Pts',(-21.1304249906002,-10.2947530860721,
0.));
#233056=CARTESIAN_POINT('Ctrl Pts',(-21.1167639345631,-10.2823401001072,
0.));
#233057=CARTESIAN_POINT('Ctrl Pts',(-21.1031582201627,-10.2700468934744,
0.));
#233058=CARTESIAN_POINT('Ctrl Pts',(-21.0896090107063,-10.2578738064181,
0.));
#233059=CARTESIAN_POINT('Ctrl Pts',(-21.0761174875445,-10.2458211823912,
0.));
#233060=CARTESIAN_POINT('Ctrl Pts',(-21.0626848505663,-10.2338893681567,
0.));
#233061=CARTESIAN_POINT('Ctrl Pts',(-21.0493123187483,-10.2220787139154,
0.));
#233062=CARTESIAN_POINT('Ctrl Pts',(-21.0360011306815,-10.2103895734123,
0.));
#233063=CARTESIAN_POINT('Ctrl Pts',(-21.0227525451107,-10.1988223040425,
0.));
#233064=CARTESIAN_POINT('Ctrl Pts',(-21.0095678414486,-10.187377266936,
0.));
#233065=CARTESIAN_POINT('Ctrl Pts',(-20.9964483203686,-10.1760548270767,
0.));
#233066=CARTESIAN_POINT('Ctrl Pts',(-20.9833953044736,-10.1648553534568,
0.));
#233067=CARTESIAN_POINT('Ctrl Pts',(-20.9704101389369,-10.1537792192065,
0.));
#233068=CARTESIAN_POINT('Ctrl Pts',(-20.9574941921591,-10.1428268017256,
0.));
#233069=CARTESIAN_POINT('Ctrl Pts',(-20.9446488563933,-10.1319984827908,
0.));
#233070=CARTESIAN_POINT('Ctrl Pts',(-20.9318755484734,-10.1212946487057,
0.));
#233071=CARTESIAN_POINT('Ctrl Pts',(-20.919175710627,-10.1107156904836,
0.));
#233072=CARTESIAN_POINT('Ctrl Pts',(-20.9065508112557,-10.1002620040076,
0.));
#233073=CARTESIAN_POINT('Ctrl Pts',(-20.894002345737,-10.0899339901915,
0.));
#233074=CARTESIAN_POINT('Ctrl Pts',(-20.881531837184,-10.0797320551154,
0.));
#233075=CARTESIAN_POINT('Ctrl Pts',(-20.86914083737,-10.0696566102218,0.));
#233076=CARTESIAN_POINT('Ctrl Pts',(-20.8568309277316,-10.0597080725375,
0.));
#233077=CARTESIAN_POINT('Ctrl Pts',(-20.8446037203402,-10.0498868648733,
0.));
#233078=CARTESIAN_POINT('Ctrl Pts',(-20.8324608588909,-10.0401934160234,
0.));
#233079=CARTESIAN_POINT('Ctrl Pts',(-20.8204040196602,-10.0306281609435,
0.));
#233080=CARTESIAN_POINT('Ctrl Pts',(-20.8084349126888,-10.0211915410095,
0.));
#233081=CARTESIAN_POINT('Ctrl Pts',(-20.7965552829908,-10.0118840042786,
0.));
#233082=CARTESIAN_POINT('Ctrl Pts',(-20.7847669117568,-10.0027060057389,
0.));
#233083=CARTESIAN_POINT('Ctrl Pts',(-20.7730716175417,-9.9936580075464,
0.));
#233084=CARTESIAN_POINT('Ctrl Pts',(-20.761471257499,-9.98474047926852,
0.));
#233085=CARTESIAN_POINT('Ctrl Pts',(-20.7499677289627,-9.9759538982347,
0.));
#233086=CARTESIAN_POINT('Ctrl Pts',(-20.7385629709795,-9.96729874986201,
0.));
#233087=CARTESIAN_POINT('Ctrl Pts',(-20.7272589658751,-9.95877552798397,
0.));
#233088=CARTESIAN_POINT('Ctrl Pts',(-20.7160577407579,-9.95038473514948,
0.));
#233089=CARTESIAN_POINT('Ctrl Pts',(-20.7049613692234,-9.94212688298236,
0.));
#233090=CARTESIAN_POINT('Ctrl Pts',(-20.6939719732484,-9.93400249259729,
0.));
#233091=CARTESIAN_POINT('Ctrl Pts',(-20.6830917250255,-9.92601209498748,
0.));
#233092=CARTESIAN_POINT('Ctrl Pts',(-20.6723228488263,-9.91815623141288,
0.));
#233093=CARTESIAN_POINT('Ctrl Pts',(-20.6616676228315,-9.91043545377007,
0.));
#233094=CARTESIAN_POINT('Ctrl Pts',(-20.6511283817414,-9.90285032516692,
0.));
#233095=CARTESIAN_POINT('Ctrl Pts',(-20.6407075193976,-9.89540142049119,
0.));
#233096=CARTESIAN_POINT('Ctrl Pts',(-20.6304074914087,-9.88808932697306,
0.));
#233097=CARTESIAN_POINT('Ctrl Pts',(-20.6202308177474,-9.88091464472675,
0.));
#233098=CARTESIAN_POINT('Ctrl Pts',(-20.6101800854494,-9.87387798732956,
0.));
#233099=CARTESIAN_POINT('Ctrl Pts',(-20.6002579513699,-9.86697998242622,
0.));
#233100=CARTESIAN_POINT('Ctrl Pts',(-20.5904671449754,-9.86022127232747,
0.));
#233101=CARTESIAN_POINT('Ctrl Pts',(-20.5808104710015,-9.8536025145698,
0.));
#233102=CARTESIAN_POINT('Ctrl Pts',(-20.5712908125139,-9.84712438256277,
0.));
#233103=CARTESIAN_POINT('Ctrl Pts',(-20.5619111362402,-9.84078756677565,
0.));
#233104=CARTESIAN_POINT('Ctrl Pts',(-20.552674497646,-9.83459277585315,
0.));
#233105=CARTESIAN_POINT('Ctrl Pts',(-20.5435840460721,-9.82854073773877,
0.));
#233106=CARTESIAN_POINT('Ctrl Pts',(-20.5346430299517,-9.82263220080362,
0.));
#233107=CARTESIAN_POINT('Ctrl Pts',(-20.5258548000629,-9.81686793455942,
0.));
#233108=CARTESIAN_POINT('Ctrl Pts',(-20.517222812284,-9.81124873025281,
0.));
#233109=CARTESIAN_POINT('Ctrl Pts',(-20.5087506310505,-9.80577540161087,
0.));
#233110=CARTESIAN_POINT('Ctrl Pts',(-20.5004419312107,-9.80044878520948,
0.));
#233111=CARTESIAN_POINT('Ctrl Pts',(-20.4923005087943,-9.7952697428833,
0.));
#233112=CARTESIAN_POINT('Ctrl Pts',(-20.4843302955329,-9.79023916498655,
0.));
#233113=CARTESIAN_POINT('Ctrl Pts',(-20.4765353711586,-9.78535797314166,
0.));
#233114=CARTESIAN_POINT('Ctrl Pts',(-20.4689199790669,-9.7806271237332,
0.));
#233115=CARTESIAN_POINT('Ctrl Pts',(-20.4614885274975,-9.77604760815528,
0.));
#233116=CARTESIAN_POINT('Ctrl Pts',(-20.4542455817527,-9.77162045104069,
0.));
#233117=CARTESIAN_POINT('Ctrl Pts',(-20.447195862298,-9.76734670980891,
0.));
#233118=CARTESIAN_POINT('Ctrl Pts',(-20.44034423294,-9.76322747195494,0.));
#233119=CARTESIAN_POINT('Ctrl Pts',(-20.4336957355473,-9.75926386289922,
0.));
#233120=CARTESIAN_POINT('Ctrl Pts',(-20.4272556476629,-9.75545705902417,
0.));
#233121=CARTESIAN_POINT('Ctrl Pts',(-20.4210295275817,-9.7518082978643,
0.));
#233122=CARTESIAN_POINT('Ctrl Pts',(-20.4150232777393,-9.74831889242174,
0.));
#233123=CARTESIAN_POINT('Ctrl Pts',(-20.4092430879861,-9.74499021838537,
0.));
#233124=CARTESIAN_POINT('Ctrl Pts',(-20.4036953576549,-9.74182369656271,
0.));
#233125=CARTESIAN_POINT('Ctrl Pts',(-20.3983866213331,-9.738820776132,0.));
#233126=CARTESIAN_POINT('Ctrl Pts',(-20.3933234845647,-9.73598292014242,
0.));
#233127=CARTESIAN_POINT('Ctrl Pts',(-20.3885129129912,-9.73331167102807,
0.));
#233128=CARTESIAN_POINT('Ctrl Pts',(-20.3839624556742,-9.73080870123727,
0.));
#233129=CARTESIAN_POINT('Ctrl Pts',(-20.3796805893304,-9.72847589116541,
0.));
#233130=CARTESIAN_POINT('Ctrl Pts',(-20.3756766651951,-9.7263153173288,
0.));
#233131=CARTESIAN_POINT('Ctrl Pts',(-20.371960235676,-9.72432910043194,
0.));
#233132=CARTESIAN_POINT('Ctrl Pts',(-20.3685406190576,-9.72251930722489,
0.));
#233133=CARTESIAN_POINT('Ctrl Pts',(-20.3654261611056,-9.7208877838108,
0.));
#233134=CARTESIAN_POINT('Ctrl Pts',(-20.3626256913981,-9.71943648548099,
0.));
#233135=CARTESIAN_POINT('Ctrl Pts',(-20.3601498764344,-9.71816778328006,
0.));
#233136=CARTESIAN_POINT('Ctrl Pts',(-20.3580133103356,-9.71708493723096,
0.));
#233137=CARTESIAN_POINT('Ctrl Pts',(-20.3562337557875,-9.71619192554185,
0.));
#233138=CARTESIAN_POINT('Ctrl Pts',(-20.3548282742361,-9.71549257088172,
0.));
#233139=CARTESIAN_POINT('Ctrl Pts',(-20.3538098605706,-9.7149897805202,
0.));
#233140=CARTESIAN_POINT('Ctrl Pts',(-20.3533097561886,-9.7147459035068,
0.));
#233141=CARTESIAN_POINT('Ctrl Pts',(-20.3531126095522,-9.71465227853041,
0.));
#233142=CARTESIAN_POINT('Ctrl Pts',(-20.353060251684,-9.71462954053041,
0.));
#233143=CARTESIAN_POINT('Ctrl Pts',(-20.353053841303,-9.71462809124915,
0.));
#233144=CARTESIAN_POINT('',(-22.8400320311649,-12.4230808101438,12.));
#233145=CARTESIAN_POINT('',(-22.8400320311649,-12.4230808101438,0.));
#233146=CARTESIAN_POINT('Ctrl Pts',(-20.353053841303,-9.71462809124915,
12.));
#233147=CARTESIAN_POINT('Ctrl Pts',(-20.353060251684,-9.71462954053041,
12.));
#233148=CARTESIAN_POINT('Ctrl Pts',(-20.3531126095522,-9.71465227853041,
12.));
#233149=CARTESIAN_POINT('Ctrl Pts',(-20.3533097561886,-9.7147459035068,
12.));
#233150=CARTESIAN_POINT('Ctrl Pts',(-20.3538098605706,-9.7149897805202,
12.));
#233151=CARTESIAN_POINT('Ctrl Pts',(-20.3548282742361,-9.71549257088172,
12.));
#233152=CARTESIAN_POINT('Ctrl Pts',(-20.3562337557875,-9.71619192554185,
12.));
#233153=CARTESIAN_POINT('Ctrl Pts',(-20.3580133103356,-9.71708493723096,
12.));
#233154=CARTESIAN_POINT('Ctrl Pts',(-20.3601498764344,-9.71816778328006,
12.));
#233155=CARTESIAN_POINT('Ctrl Pts',(-20.3626256913981,-9.71943648548099,
12.));
#233156=CARTESIAN_POINT('Ctrl Pts',(-20.3654261611056,-9.7208877838108,
12.));
#233157=CARTESIAN_POINT('Ctrl Pts',(-20.3685406190576,-9.72251930722489,
12.));
#233158=CARTESIAN_POINT('Ctrl Pts',(-20.371960235676,-9.72432910043194,
12.));
#233159=CARTESIAN_POINT('Ctrl Pts',(-20.3756766651951,-9.7263153173288,
12.));
#233160=CARTESIAN_POINT('Ctrl Pts',(-20.3796805893304,-9.72847589116541,
12.));
#233161=CARTESIAN_POINT('Ctrl Pts',(-20.3839624556742,-9.73080870123727,
12.));
#233162=CARTESIAN_POINT('Ctrl Pts',(-20.3885129129912,-9.73331167102807,
12.));
#233163=CARTESIAN_POINT('Ctrl Pts',(-20.3933234845647,-9.73598292014242,
12.));
#233164=CARTESIAN_POINT('Ctrl Pts',(-20.3983866213331,-9.738820776132,12.));
#233165=CARTESIAN_POINT('Ctrl Pts',(-20.4036953576549,-9.74182369656271,
12.));
#233166=CARTESIAN_POINT('Ctrl Pts',(-20.4092430879861,-9.74499021838537,
12.));
#233167=CARTESIAN_POINT('Ctrl Pts',(-20.4150232777393,-9.74831889242174,
12.));
#233168=CARTESIAN_POINT('Ctrl Pts',(-20.4210295275817,-9.7518082978643,
12.));
#233169=CARTESIAN_POINT('Ctrl Pts',(-20.4272556476629,-9.75545705902417,
12.));
#233170=CARTESIAN_POINT('Ctrl Pts',(-20.4336957355473,-9.75926386289922,
12.));
#233171=CARTESIAN_POINT('Ctrl Pts',(-20.44034423294,-9.76322747195494,12.));
#233172=CARTESIAN_POINT('Ctrl Pts',(-20.447195862298,-9.76734670980891,
12.));
#233173=CARTESIAN_POINT('Ctrl Pts',(-20.4542455817527,-9.77162045104069,
12.));
#233174=CARTESIAN_POINT('Ctrl Pts',(-20.4614885274975,-9.77604760815528,
12.));
#233175=CARTESIAN_POINT('Ctrl Pts',(-20.4689199790669,-9.7806271237332,
12.));
#233176=CARTESIAN_POINT('Ctrl Pts',(-20.4765353711586,-9.78535797314166,
12.));
#233177=CARTESIAN_POINT('Ctrl Pts',(-20.4843302955329,-9.79023916498655,
12.));
#233178=CARTESIAN_POINT('Ctrl Pts',(-20.4923005087943,-9.7952697428833,
12.));
#233179=CARTESIAN_POINT('Ctrl Pts',(-20.5004419312107,-9.80044878520948,
12.));
#233180=CARTESIAN_POINT('Ctrl Pts',(-20.5087506310505,-9.80577540161087,
12.));
#233181=CARTESIAN_POINT('Ctrl Pts',(-20.517222812284,-9.81124873025281,
12.));
#233182=CARTESIAN_POINT('Ctrl Pts',(-20.5258548000629,-9.81686793455942,
12.));
#233183=CARTESIAN_POINT('Ctrl Pts',(-20.5346430299517,-9.82263220080362,
12.));
#233184=CARTESIAN_POINT('Ctrl Pts',(-20.5435840460721,-9.82854073773877,
12.));
#233185=CARTESIAN_POINT('Ctrl Pts',(-20.552674497646,-9.83459277585315,
12.));
#233186=CARTESIAN_POINT('Ctrl Pts',(-20.5619111362402,-9.84078756677565,
12.));
#233187=CARTESIAN_POINT('Ctrl Pts',(-20.5712908125139,-9.84712438256277,
12.));
#233188=CARTESIAN_POINT('Ctrl Pts',(-20.5808104710015,-9.8536025145698,
12.));
#233189=CARTESIAN_POINT('Ctrl Pts',(-20.5904671449754,-9.86022127232747,
12.));
#233190=CARTESIAN_POINT('Ctrl Pts',(-20.6002579513699,-9.86697998242622,
12.));
#233191=CARTESIAN_POINT('Ctrl Pts',(-20.6101800854494,-9.87387798732956,
12.));
#233192=CARTESIAN_POINT('Ctrl Pts',(-20.6202308177474,-9.88091464472675,
12.));
#233193=CARTESIAN_POINT('Ctrl Pts',(-20.6304074914087,-9.88808932697306,
12.));
#233194=CARTESIAN_POINT('Ctrl Pts',(-20.6407075193976,-9.89540142049119,
12.));
#233195=CARTESIAN_POINT('Ctrl Pts',(-20.6511283817414,-9.90285032516692,
12.));
#233196=CARTESIAN_POINT('Ctrl Pts',(-20.6616676228315,-9.91043545377007,
12.));
#233197=CARTESIAN_POINT('Ctrl Pts',(-20.6723228488263,-9.91815623141288,
12.));
#233198=CARTESIAN_POINT('Ctrl Pts',(-20.6830917250255,-9.92601209498748,
12.));
#233199=CARTESIAN_POINT('Ctrl Pts',(-20.6939719732484,-9.93400249259729,
12.));
#233200=CARTESIAN_POINT('Ctrl Pts',(-20.7049613692234,-9.94212688298236,
12.));
#233201=CARTESIAN_POINT('Ctrl Pts',(-20.7160577407579,-9.95038473514948,
12.));
#233202=CARTESIAN_POINT('Ctrl Pts',(-20.7272589658751,-9.95877552798397,
12.));
#233203=CARTESIAN_POINT('Ctrl Pts',(-20.7385629709795,-9.96729874986201,
12.));
#233204=CARTESIAN_POINT('Ctrl Pts',(-20.7499677289627,-9.9759538982347,
12.));
#233205=CARTESIAN_POINT('Ctrl Pts',(-20.761471257499,-9.98474047926852,
12.));
#233206=CARTESIAN_POINT('Ctrl Pts',(-20.7730716175417,-9.9936580075464,
12.));
#233207=CARTESIAN_POINT('Ctrl Pts',(-20.7847669117568,-10.0027060057389,
12.));
#233208=CARTESIAN_POINT('Ctrl Pts',(-20.7965552829908,-10.0118840042786,
12.));
#233209=CARTESIAN_POINT('Ctrl Pts',(-20.8084349126888,-10.0211915410095,
12.));
#233210=CARTESIAN_POINT('Ctrl Pts',(-20.8204040196602,-10.0306281609435,
12.));
#233211=CARTESIAN_POINT('Ctrl Pts',(-20.8324608588909,-10.0401934160234,
12.));
#233212=CARTESIAN_POINT('Ctrl Pts',(-20.8446037203402,-10.0498868648733,
12.));
#233213=CARTESIAN_POINT('Ctrl Pts',(-20.8568309277316,-10.0597080725375,
12.));
#233214=CARTESIAN_POINT('Ctrl Pts',(-20.86914083737,-10.0696566102218,12.));
#233215=CARTESIAN_POINT('Ctrl Pts',(-20.881531837184,-10.0797320551154,
12.));
#233216=CARTESIAN_POINT('Ctrl Pts',(-20.894002345737,-10.0899339901915,
12.));
#233217=CARTESIAN_POINT('Ctrl Pts',(-20.9065508112557,-10.1002620040076,
12.));
#233218=CARTESIAN_POINT('Ctrl Pts',(-20.919175710627,-10.1107156904836,
12.));
#233219=CARTESIAN_POINT('Ctrl Pts',(-20.9318755484734,-10.1212946487057,
12.));
#233220=CARTESIAN_POINT('Ctrl Pts',(-20.9446488563933,-10.1319984827908,
12.));
#233221=CARTESIAN_POINT('Ctrl Pts',(-20.9574941921591,-10.1428268017256,
12.));
#233222=CARTESIAN_POINT('Ctrl Pts',(-20.9704101389369,-10.1537792192065,
12.));
#233223=CARTESIAN_POINT('Ctrl Pts',(-20.9833953044736,-10.1648553534568,
12.));
#233224=CARTESIAN_POINT('Ctrl Pts',(-20.9964483203686,-10.1760548270767,
12.));
#233225=CARTESIAN_POINT('Ctrl Pts',(-21.0095678414486,-10.187377266936,
12.));
#233226=CARTESIAN_POINT('Ctrl Pts',(-21.0227525451107,-10.1988223040425,
12.));
#233227=CARTESIAN_POINT('Ctrl Pts',(-21.0360011306815,-10.2103895734123,
12.));
#233228=CARTESIAN_POINT('Ctrl Pts',(-21.0493123187483,-10.2220787139154,
12.));
#233229=CARTESIAN_POINT('Ctrl Pts',(-21.0626848505663,-10.2338893681567,
12.));
#233230=CARTESIAN_POINT('Ctrl Pts',(-21.0761174875445,-10.2458211823912,
12.));
#233231=CARTESIAN_POINT('Ctrl Pts',(-21.0896090107063,-10.2578738064181,
12.));
#233232=CARTESIAN_POINT('Ctrl Pts',(-21.1031582201627,-10.2700468934744,
12.));
#233233=CARTESIAN_POINT('Ctrl Pts',(-21.1167639345631,-10.2823401001072,
12.));
#233234=CARTESIAN_POINT('Ctrl Pts',(-21.1304249906002,-10.2947530860721,
12.));
#233235=CARTESIAN_POINT('Ctrl Pts',(-21.1441402425843,-10.3072855142687,
12.));
#233236=CARTESIAN_POINT('Ctrl Pts',(-21.1579085619965,-10.3199370506544,
12.));
#233237=CARTESIAN_POINT('Ctrl Pts',(-21.1717288370509,-10.3327073641572,
12.));
#233238=CARTESIAN_POINT('Ctrl Pts',(-21.1855999722416,-10.34559612657,12.));
#233239=CARTESIAN_POINT('Ctrl Pts',(-21.199520887919,-10.3586030124587,
12.));
#233240=CARTESIAN_POINT('Ctrl Pts',(-21.2134905199345,-10.371727699113,
12.));
#233241=CARTESIAN_POINT('Ctrl Pts',(-21.22750781927,-10.3849698664786,12.));
#233242=CARTESIAN_POINT('Ctrl Pts',(-21.2415717516714,-10.3983291970846,
12.));
#233243=CARTESIAN_POINT('Ctrl Pts',(-21.255681297275,-10.4118053759588,
12.));
#233244=CARTESIAN_POINT('Ctrl Pts',(-21.2698354502403,-10.42539809054,12.));
#233245=CARTESIAN_POINT('Ctrl Pts',(-21.2840332184483,-10.4391070306391,
12.));
#233246=CARTESIAN_POINT('Ctrl Pts',(-21.2982736231931,-10.4529318883874,
12.));
#233247=CARTESIAN_POINT('Ctrl Pts',(-21.3125556988731,-10.4668723581768,
12.));
#233248=CARTESIAN_POINT('Ctrl Pts',(-21.3268784926819,-10.4809281365931,
12.));
#233249=CARTESIAN_POINT('Ctrl Pts',(-21.3412410642904,-10.4950989223337,
12.));
#233250=CARTESIAN_POINT('Ctrl Pts',(-21.3556424855814,-10.5093844161685,
12.));
#233251=CARTESIAN_POINT('Ctrl Pts',(-21.3700818403936,-10.5237843209057,
12.));
#233252=CARTESIAN_POINT('Ctrl Pts',(-21.3845582242602,-10.5382983413421,
12.));
#233253=CARTESIAN_POINT('Ctrl Pts',(-21.3990707441497,-10.5529261842108,
12.));
#233254=CARTESIAN_POINT('Ctrl Pts',(-21.4136185181979,-10.5676675581108,
12.));
#233255=CARTESIAN_POINT('Ctrl Pts',(-21.4282006754631,-10.5825221734573,
12.));
#233256=CARTESIAN_POINT('Ctrl Pts',(-21.4428163557144,-10.5974897424622,
12.));
#233257=CARTESIAN_POINT('Ctrl Pts',(-21.4574647092097,-10.6125699790961,
12.));
#233258=CARTESIAN_POINT('Ctrl Pts',(-21.4721448964766,-10.6277625990456,
12.));
#233259=CARTESIAN_POINT('Ctrl Pts',(-21.4868560880889,-10.6430673196607,
12.));
#233260=CARTESIAN_POINT('Ctrl Pts',(-21.5015974644449,-10.6584838598939,
12.));
#233261=CARTESIAN_POINT('Ctrl Pts',(-21.51636821558,-10.6740119402834,12.));
#233262=CARTESIAN_POINT('Ctrl Pts',(-21.5311675409807,-10.689651282929,
12.));
#233263=CARTESIAN_POINT('Ctrl Pts',(-21.5459946493955,-10.7054016114571,
12.));
#233264=CARTESIAN_POINT('Ctrl Pts',(-21.5608487586468,-10.7212626509816,
12.));
#233265=CARTESIAN_POINT('Ctrl Pts',(-21.5757290954371,-10.7372341280467,
12.));
#233266=CARTESIAN_POINT('Ctrl Pts',(-21.5906348951743,-10.7533157705941,
12.));
#233267=CARTESIAN_POINT('Ctrl Pts',(-21.6055654018176,-10.7695073079552,
12.));
#233268=CARTESIAN_POINT('Ctrl Pts',(-21.6205198677173,-10.7858084708261,
12.));
#233269=CARTESIAN_POINT('Ctrl Pts',(-21.6354975534557,-10.8022189912369,
12.));
#233270=CARTESIAN_POINT('Ctrl Pts',(-21.6504977276866,-10.8187386025136,
12.));
#233271=CARTESIAN_POINT('Ctrl Pts',(-21.6655196669732,-10.8353670392272,
12.));
#233272=CARTESIAN_POINT('Ctrl Pts',(-21.6805626556467,-10.8521040371835,
12.));
#233273=CARTESIAN_POINT('Ctrl Pts',(-21.6956259856672,-10.8689493334095,
12.));
#233274=CARTESIAN_POINT('Ctrl Pts',(-21.7107089564825,-10.8859026661293,
12.));
#233275=CARTESIAN_POINT('Ctrl Pts',(-21.7258108748873,-10.902963774734,
12.));
#233276=CARTESIAN_POINT('Ctrl Pts',(-21.7409310548797,-10.9201323997384,
12.));
#233277=CARTESIAN_POINT('Ctrl Pts',(-21.7560688175247,-10.9374082827444,
12.));
#233278=CARTESIAN_POINT('Ctrl Pts',(-21.7712234908464,-10.9547911664455,
12.));
#233279=CARTESIAN_POINT('Ctrl Pts',(-21.7863944097141,-10.9722807946155,
12.));
#233280=CARTESIAN_POINT('Ctrl Pts',(-21.8015809157301,-10.9898769120912,
12.));
#233281=CARTESIAN_POINT('Ctrl Pts',(-21.8167823571168,-11.0075792647477,
12.));
#233282=CARTESIAN_POINT('Ctrl Pts',(-21.8319980886033,-11.0253875994598,
12.));
#233283=CARTESIAN_POINT('Ctrl Pts',(-21.8472274713103,-11.0433016640807,
12.));
#233284=CARTESIAN_POINT('Ctrl Pts',(-21.8624698726318,-11.0613212074363,
12.));
#233285=CARTESIAN_POINT('Ctrl Pts',(-21.877724666119,-11.0794459793057,
12.));
#233286=CARTESIAN_POINT('Ctrl Pts',(-21.8929912313608,-11.0976757303944,
12.));
#233287=CARTESIAN_POINT('Ctrl Pts',(-21.9082689538688,-11.1160102123024,
12.));
#233288=CARTESIAN_POINT('Ctrl Pts',(-21.923557224952,-11.1344491774741,
12.));
#233289=CARTESIAN_POINT('Ctrl Pts',(-21.9388554416439,-11.1529923792003,
12.));
#233290=CARTESIAN_POINT('Ctrl Pts',(-21.9541630066506,-11.1716395716376,
12.));
#233291=CARTESIAN_POINT('Ctrl Pts',(-21.9694793282914,-11.190390509811,
12.));
#233292=CARTESIAN_POINT('Ctrl Pts',(-21.9848038204439,-11.2092449496125,
12.));
#233293=CARTESIAN_POINT('Ctrl Pts',(-22.0001359024839,-11.2282026477896,
12.));
#233294=CARTESIAN_POINT('Ctrl Pts',(-22.0154749992363,-11.2472633619275,
12.));
#233295=CARTESIAN_POINT('Ctrl Pts',(-22.030820540835,-11.2664268504206,
12.));
#233296=CARTESIAN_POINT('Ctrl Pts',(-22.046171962566,-11.2856928724374,
12.));
#233297=CARTESIAN_POINT('Ctrl Pts',(-22.0615287047179,-11.3050611878771,
12.));
#233298=CARTESIAN_POINT('Ctrl Pts',(-22.0768902124267,-11.3245315573168,
12.));
#233299=CARTESIAN_POINT('Ctrl Pts',(-22.0922559355294,-11.3441037419553,
12.));
#233300=CARTESIAN_POINT('Ctrl Pts',(-22.1076253283979,-11.3637775035367,
12.));
#233301=CARTESIAN_POINT('Ctrl Pts',(-22.1229978500186,-11.3835526044256,
12.));
#233302=CARTESIAN_POINT('Ctrl Pts',(-22.1383729640964,-11.4034288076908,
12.));
#233303=CARTESIAN_POINT('Ctrl Pts',(-22.1537501391487,-11.4234058771742,
12.));
#233304=CARTESIAN_POINT('Ctrl Pts',(-22.1691288486096,-11.443483577557,
12.));
#233305=CARTESIAN_POINT('Ctrl Pts',(-22.184508570917,-11.463661674411,12.));
#233306=CARTESIAN_POINT('Ctrl Pts',(-22.1998887896436,-11.483939934259,
12.));
#233307=CARTESIAN_POINT('Ctrl Pts',(-22.2152689931022,-11.5043181244242,
12.));
#233308=CARTESIAN_POINT('Ctrl Pts',(-22.2306486738901,-11.5247960128477,
12.));
#233309=CARTESIAN_POINT('Ctrl Pts',(-22.2460273284654,-11.5453733679121,
12.));
#233310=CARTESIAN_POINT('Ctrl Pts',(-22.2614044566898,-11.5660499582403,
12.));
#233311=CARTESIAN_POINT('Ctrl Pts',(-22.2767795614348,-11.5868255525188,
12.));
#233312=CARTESIAN_POINT('Ctrl Pts',(-22.2921521480356,-11.6076999192357,
12.));
#233313=CARTESIAN_POINT('Ctrl Pts',(-22.3075217249049,-11.6286728270009,
12.));
#233314=CARTESIAN_POINT('Ctrl Pts',(-22.3228878043976,-11.6497440449857,
12.));
#233315=CARTESIAN_POINT('Ctrl Pts',(-22.3382499035619,-11.6709133432985,
12.));
#233316=CARTESIAN_POINT('Ctrl Pts',(-22.3536075450029,-11.6921804934056,
12.));
#233317=CARTESIAN_POINT('Ctrl Pts',(-22.3689602575491,-11.7135452684532,
12.));
#233318=CARTESIAN_POINT('Ctrl Pts',(-22.3843075773899,-11.7350074437961,
12.));
#233319=CARTESIAN_POINT('Ctrl Pts',(-22.3996490469191,-11.7565667964764,
12.));
#233320=CARTESIAN_POINT('Ctrl Pts',(-22.4149842125008,-11.7782231042039,
12.));
#233321=CARTESIAN_POINT('Ctrl Pts',(-22.430312622646,-11.7999761445173,
12.));
#233322=CARTESIAN_POINT('Ctrl Pts',(-22.4456338258735,-11.8218256937889,
12.));
#233323=CARTESIAN_POINT('Ctrl Pts',(-22.4609473690471,-11.8437715264487,
12.));
#233324=CARTESIAN_POINT('Ctrl Pts',(-22.4762527946702,-11.8658134137019,
12.));
#233325=CARTESIAN_POINT('Ctrl Pts',(-22.4915496418485,-11.8879511239942,
12.));
#233326=CARTESIAN_POINT('Ctrl Pts',(-22.5068374513973,-11.9101844254557,
12.));
#233327=CARTESIAN_POINT('Ctrl Pts',(-22.5221157697883,-11.9325130877803,
12.));
#233328=CARTESIAN_POINT('Ctrl Pts',(-22.5373841537307,-11.9549368843997,
12.));
#233329=CARTESIAN_POINT('Ctrl Pts',(-22.5526421741158,-11.9774555943496,
12.));
#233330=CARTESIAN_POINT('Ctrl Pts',(-22.5678894211181,-12.0000690046695,
12.));
#233331=CARTESIAN_POINT('Ctrl Pts',(-22.5831255061282,-12.0227769113127,
12.));
#233332=CARTESIAN_POINT('Ctrl Pts',(-22.5983500505644,-12.0455791139128,
12.));
#233333=CARTESIAN_POINT('Ctrl Pts',(-22.6135626764898,-12.0684754113862,
12.));
#233334=CARTESIAN_POINT('Ctrl Pts',(-22.6287629967056,-12.0914655972823,
12.));
#233335=CARTESIAN_POINT('Ctrl Pts',(-22.6439506046605,-12.1145494550383,
12.));
#233336=CARTESIAN_POINT('Ctrl Pts',(-22.6591250653965,-12.1377267537145,
12.));
#233337=CARTESIAN_POINT('Ctrl Pts',(-22.6742859034944,-12.1609972423099,
12.));
#233338=CARTESIAN_POINT('Ctrl Pts',(-22.6894326205037,-12.1843606579261,
12.));
#233339=CARTESIAN_POINT('Ctrl Pts',(-22.7045647168747,-12.2078167360284,
12.));
#233340=CARTESIAN_POINT('Ctrl Pts',(-22.7196817119374,-12.2313652198061,
12.));
#233341=CARTESIAN_POINT('Ctrl Pts',(-22.7347831655287,-12.2550058702395,
12.));
#233342=CARTESIAN_POINT('Ctrl Pts',(-22.7498686970069,-12.2787384750742,
12.));
#233343=CARTESIAN_POINT('Ctrl Pts',(-22.764938010105,-12.3025628601792,
12.));
#233344=CARTESIAN_POINT('Ctrl Pts',(-22.7799908974768,-12.3264788926075,
12.));
#233345=CARTESIAN_POINT('Ctrl Pts',(-22.795027221673,-12.3504864740319,
12.));
#233346=CARTESIAN_POINT('Ctrl Pts',(-22.81004690224,-12.374585536673,12.));
#233347=CARTESIAN_POINT('Ctrl Pts',(-22.8220493007173,-12.3939379378998,
12.));
#233348=CARTESIAN_POINT('Ctrl Pts',(-22.8310435872748,-12.4084933766346,
12.));
#233349=CARTESIAN_POINT('Ctrl Pts',(-22.8370364396459,-12.418215285186,
12.));
#233350=CARTESIAN_POINT('Ctrl Pts',(-22.8400320311649,-12.4230808101438,
12.));
#233351=CARTESIAN_POINT('Ctrl Pts',(-21.2610617890679,-7.52250298901264,
0.));
#233352=CARTESIAN_POINT('Ctrl Pts',(-21.2610617890679,-7.52250298901264,
12.));
#233353=CARTESIAN_POINT('Ctrl Pts',(-21.2610673466886,-7.5225064970397,
0.));
#233354=CARTESIAN_POINT('Ctrl Pts',(-21.2610673466886,-7.5225064970397,
12.));
#233355=CARTESIAN_POINT('Ctrl Pts',(-21.2611204474866,-7.52252744144903,
0.));
#233356=CARTESIAN_POINT('Ctrl Pts',(-21.2611204474866,-7.52252744144903,
12.));
#233357=CARTESIAN_POINT('Ctrl Pts',(-21.261326054066,-7.5226006423166,0.));
#233358=CARTESIAN_POINT('Ctrl Pts',(-21.261326054066,-7.5226006423166,12.));
#233359=CARTESIAN_POINT('Ctrl Pts',(-21.2618521283555,-7.52278182242669,
0.));
#233360=CARTESIAN_POINT('Ctrl Pts',(-21.2618521283555,-7.52278182242669,
12.));
#233361=CARTESIAN_POINT('Ctrl Pts',(-21.262927782038,-7.52314642316199,
0.));
#233362=CARTESIAN_POINT('Ctrl Pts',(-21.262927782038,-7.52314642316199,
12.));
#233363=CARTESIAN_POINT('Ctrl Pts',(-21.2644161259962,-7.52364573027552,
0.));
#233364=CARTESIAN_POINT('Ctrl Pts',(-21.2644161259962,-7.52364573027552,
12.));
#233365=CARTESIAN_POINT('Ctrl Pts',(-21.2663059157058,-7.52427261074297,
0.));
#233366=CARTESIAN_POINT('Ctrl Pts',(-21.2663059157058,-7.52427261074297,
12.));
#233367=CARTESIAN_POINT('Ctrl Pts',(-21.2685823838671,-7.5250177033353,
0.));
#233368=CARTESIAN_POINT('Ctrl Pts',(-21.2685823838671,-7.5250177033353,
12.));
#233369=CARTESIAN_POINT('Ctrl Pts',(-21.2712301573466,-7.52587126095529,
0.));
#233370=CARTESIAN_POINT('Ctrl Pts',(-21.2712301573466,-7.52587126095529,
12.));
#233371=CARTESIAN_POINT('Ctrl Pts',(-21.2742366113579,-7.5268252691854,
0.));
#233372=CARTESIAN_POINT('Ctrl Pts',(-21.2742366113579,-7.5268252691854,
12.));
#233373=CARTESIAN_POINT('Ctrl Pts',(-21.2775925269652,-7.52787386225332,
0.));
#233374=CARTESIAN_POINT('Ctrl Pts',(-21.2775925269652,-7.52787386225332,
12.));
#233375=CARTESIAN_POINT('Ctrl Pts',(-21.2812902781143,-7.52901217930407,
0.));
#233376=CARTESIAN_POINT('Ctrl Pts',(-21.2812902781143,-7.52901217930407,
12.));
#233377=CARTESIAN_POINT('Ctrl Pts',(-21.2853226580657,-7.53023562438229,
0.));
#233378=CARTESIAN_POINT('Ctrl Pts',(-21.2853226580657,-7.53023562438229,
12.));
#233379=CARTESIAN_POINT('Ctrl Pts',(-21.2896816163842,-7.53153906987855,
0.));
#233380=CARTESIAN_POINT('Ctrl Pts',(-21.2896816163842,-7.53153906987855,
12.));
#233381=CARTESIAN_POINT('Ctrl Pts',(-21.2943588989331,-7.53291726078526,
0.));
#233382=CARTESIAN_POINT('Ctrl Pts',(-21.2943588989331,-7.53291726078526,
12.));
#233383=CARTESIAN_POINT('Ctrl Pts',(-21.2993464250717,-7.53436505309942,
0.));
#233384=CARTESIAN_POINT('Ctrl Pts',(-21.2993464250717,-7.53436505309942,
12.));
#233385=CARTESIAN_POINT('Ctrl Pts',(-21.3046368712157,-7.53587778251735,
0.));
#233386=CARTESIAN_POINT('Ctrl Pts',(-21.3046368712157,-7.53587778251735,
12.));
#233387=CARTESIAN_POINT('Ctrl Pts',(-21.310223716773,-7.53745129364616,
0.));
#233388=CARTESIAN_POINT('Ctrl Pts',(-21.310223716773,-7.53745129364616,
12.));
#233389=CARTESIAN_POINT('Ctrl Pts',(-21.3161009456256,-7.53908175169898,
0.));
#233390=CARTESIAN_POINT('Ctrl Pts',(-21.3161009456256,-7.53908175169898,
12.));
#233391=CARTESIAN_POINT('Ctrl Pts',(-21.3222628524165,-7.54076552038278,
0.));
#233392=CARTESIAN_POINT('Ctrl Pts',(-21.3222628524165,-7.54076552038278,
12.));
#233393=CARTESIAN_POINT('Ctrl Pts',(-21.328703791771,-7.5424990037703,0.));
#233394=CARTESIAN_POINT('Ctrl Pts',(-21.328703791771,-7.5424990037703,12.));
#233395=CARTESIAN_POINT('Ctrl Pts',(-21.3354182340149,-7.54427868151267,
0.));
#233396=CARTESIAN_POINT('Ctrl Pts',(-21.3354182340149,-7.54427868151267,
12.));
#233397=CARTESIAN_POINT('Ctrl Pts',(-21.3424008295038,-7.54610114948346,
0.));
#233398=CARTESIAN_POINT('Ctrl Pts',(-21.3424008295038,-7.54610114948346,
12.));
#233399=CARTESIAN_POINT('Ctrl Pts',(-21.3496464761531,-7.5479631624633,
0.));
#233400=CARTESIAN_POINT('Ctrl Pts',(-21.3496464761531,-7.5479631624633,
12.));
#233401=CARTESIAN_POINT('Ctrl Pts',(-21.3571503685855,-7.54986166521309,
0.));
#233402=CARTESIAN_POINT('Ctrl Pts',(-21.3571503685855,-7.54986166521309,
12.));
#233403=CARTESIAN_POINT('Ctrl Pts',(-21.3649079431865,-7.55179375777443,
0.));
#233404=CARTESIAN_POINT('Ctrl Pts',(-21.3649079431865,-7.55179375777443,
12.));
#233405=CARTESIAN_POINT('Ctrl Pts',(-21.3729148390243,-7.55375667080028,
0.));
#233406=CARTESIAN_POINT('Ctrl Pts',(-21.3729148390243,-7.55375667080028,
12.));
#233407=CARTESIAN_POINT('Ctrl Pts',(-21.3811668478932,-7.55574773403502,
0.));
#233408=CARTESIAN_POINT('Ctrl Pts',(-21.3811668478932,-7.55574773403502,
12.));
#233409=CARTESIAN_POINT('Ctrl Pts',(-21.3896598842117,-7.55776435731416,
0.));
#233410=CARTESIAN_POINT('Ctrl Pts',(-21.3896598842117,-7.55776435731416,
12.));
#233411=CARTESIAN_POINT('Ctrl Pts',(-21.3983899952987,-7.5598040370061,
0.));
#233412=CARTESIAN_POINT('Ctrl Pts',(-21.3983899952987,-7.5598040370061,
12.));
#233413=CARTESIAN_POINT('Ctrl Pts',(-21.4073533630365,-7.56186435703621,
0.));
#233414=CARTESIAN_POINT('Ctrl Pts',(-21.4073533630365,-7.56186435703621,
12.));
#233415=CARTESIAN_POINT('Ctrl Pts',(-21.4165463106254,-7.56394299313684,
0.));
#233416=CARTESIAN_POINT('Ctrl Pts',(-21.4165463106254,-7.56394299313684,
12.));
#233417=CARTESIAN_POINT('Ctrl Pts',(-21.4259653015736,-7.56603771218712,
0.));
#233418=CARTESIAN_POINT('Ctrl Pts',(-21.4259653015736,-7.56603771218712,
12.));
#233419=CARTESIAN_POINT('Ctrl Pts',(-21.4356069261513,-7.56814636360847,
0.));
#233420=CARTESIAN_POINT('Ctrl Pts',(-21.4356069261513,-7.56814636360847,
12.));
#233421=CARTESIAN_POINT('Ctrl Pts',(-21.4454678907509,-7.57026687261165,
0.));
#233422=CARTESIAN_POINT('Ctrl Pts',(-21.4454678907509,-7.57026687261165,
12.));
#233423=CARTESIAN_POINT('Ctrl Pts',(-21.4555450053142,-7.57239723223505,
0.));
#233424=CARTESIAN_POINT('Ctrl Pts',(-21.4555450053142,-7.57239723223505,
12.));
#233425=CARTESIAN_POINT('Ctrl Pts',(-21.4658351740128,-7.57453549743411,
0.));
#233426=CARTESIAN_POINT('Ctrl Pts',(-21.4658351740128,-7.57453549743411,
12.));
#233427=CARTESIAN_POINT('Ctrl Pts',(-21.4763353936762,-7.57667978402987,
0.));
#233428=CARTESIAN_POINT('Ctrl Pts',(-21.4763353936762,-7.57667978402987,
12.));
#233429=CARTESIAN_POINT('Ctrl Pts',(-21.4870427508194,-7.57882826679131,
0.));
#233430=CARTESIAN_POINT('Ctrl Pts',(-21.4870427508194,-7.57882826679131,
12.));
#233431=CARTESIAN_POINT('Ctrl Pts',(-21.4979544192744,-7.58097917790744,
0.));
#233432=CARTESIAN_POINT('Ctrl Pts',(-21.4979544192744,-7.58097917790744,
12.));
#233433=CARTESIAN_POINT('Ctrl Pts',(-21.5090676573873,-7.58313080519179,
0.));
#233434=CARTESIAN_POINT('Ctrl Pts',(-21.5090676573873,-7.58313080519179,
12.));
#233435=CARTESIAN_POINT('Ctrl Pts',(-21.5203798035299,-7.58528148919129,
0.));
#233436=CARTESIAN_POINT('Ctrl Pts',(-21.5203798035299,-7.58528148919129,
12.));
#233437=CARTESIAN_POINT('Ctrl Pts',(-21.5318882716736,-7.58742962034833,
0.));
#233438=CARTESIAN_POINT('Ctrl Pts',(-21.5318882716736,-7.58742962034833,
12.));
#233439=CARTESIAN_POINT('Ctrl Pts',(-21.543590547011,-7.58957363620013,
0.));
#233440=CARTESIAN_POINT('Ctrl Pts',(-21.543590547011,-7.58957363620013,
12.));
#233441=CARTESIAN_POINT('Ctrl Pts',(-21.5554841813462,-7.59171201844776,
0.));
#233442=CARTESIAN_POINT('Ctrl Pts',(-21.5554841813462,-7.59171201844776,
12.));
#233443=CARTESIAN_POINT('Ctrl Pts',(-21.5675667904726,-7.59384329124918,
0.));
#233444=CARTESIAN_POINT('Ctrl Pts',(-21.5675667904726,-7.59384329124918,
12.));
#233445=CARTESIAN_POINT('Ctrl Pts',(-21.5798360518978,-7.59596601973583,
0.));
#233446=CARTESIAN_POINT('Ctrl Pts',(-21.5798360518978,-7.59596601973583,
12.));
#233447=CARTESIAN_POINT('Ctrl Pts',(-21.5922897024466,-7.59807880846194,
0.));
#233448=CARTESIAN_POINT('Ctrl Pts',(-21.5922897024466,-7.59807880846194,
12.));
#233449=CARTESIAN_POINT('Ctrl Pts',(-21.6049255358843,-7.6001802998824,
0.));
#233450=CARTESIAN_POINT('Ctrl Pts',(-21.6049255358843,-7.6001802998824,
12.));
#233451=CARTESIAN_POINT('Ctrl Pts',(-21.617741400599,-7.60226917285428,
0.));
#233452=CARTESIAN_POINT('Ctrl Pts',(-21.617741400599,-7.60226917285428,
12.));
#233453=CARTESIAN_POINT('Ctrl Pts',(-21.6307351973822,-7.60434414118295,
0.));
#233454=CARTESIAN_POINT('Ctrl Pts',(-21.6307351973822,-7.60434414118295,
12.));
#233455=CARTESIAN_POINT('Ctrl Pts',(-21.6439048771743,-7.60640395216356,
0.));
#233456=CARTESIAN_POINT('Ctrl Pts',(-21.6439048771743,-7.60640395216356,
12.));
#233457=CARTESIAN_POINT('Ctrl Pts',(-21.6572484388081,-7.60844738512873,
0.));
#233458=CARTESIAN_POINT('Ctrl Pts',(-21.6572484388081,-7.60844738512873,
12.));
#233459=CARTESIAN_POINT('Ctrl Pts',(-21.6707639267576,-7.61047325000955,
0.));
#233460=CARTESIAN_POINT('Ctrl Pts',(-21.6707639267576,-7.61047325000955,
12.));
#233461=CARTESIAN_POINT('Ctrl Pts',(-21.6844494295815,-7.61248038630268,
0.));
#233462=CARTESIAN_POINT('Ctrl Pts',(-21.6844494295815,-7.61248038630268,
12.));
#233463=CARTESIAN_POINT('Ctrl Pts',(-21.6983030783322,-7.61446766202786,
0.));
#233464=CARTESIAN_POINT('Ctrl Pts',(-21.6983030783322,-7.61446766202786,
12.));
#233465=CARTESIAN_POINT('Ctrl Pts',(-21.7123230449834,-7.6164339727042,
0.));
#233466=CARTESIAN_POINT('Ctrl Pts',(-21.7123230449834,-7.6164339727042,
12.));
#233467=CARTESIAN_POINT('Ctrl Pts',(-21.7265075407975,-7.61837824030537,
0.));
#233468=CARTESIAN_POINT('Ctrl Pts',(-21.7265075407975,-7.61837824030537,
12.));
#233469=CARTESIAN_POINT('Ctrl Pts',(-21.7408548148656,-7.62029941230854,
0.));
#233470=CARTESIAN_POINT('Ctrl Pts',(-21.7408548148656,-7.62029941230854,
12.));
#233471=CARTESIAN_POINT('Ctrl Pts',(-21.7553631528328,-7.62219646084228,
0.));
#233472=CARTESIAN_POINT('Ctrl Pts',(-21.7553631528328,-7.62219646084228,
12.));
#233473=CARTESIAN_POINT('Ctrl Pts',(-21.7700308755584,-7.62406838181166,
0.));
#233474=CARTESIAN_POINT('Ctrl Pts',(-21.7700308755584,-7.62406838181166,
12.));
#233475=CARTESIAN_POINT('Ctrl Pts',(-21.7848563378021,-7.62591419404512,
0.));
#233476=CARTESIAN_POINT('Ctrl Pts',(-21.7848563378021,-7.62591419404512,
12.));
#233477=CARTESIAN_POINT('Ctrl Pts',(-21.799837926858,-7.62773293842389,
0.));
#233478=CARTESIAN_POINT('Ctrl Pts',(-21.799837926858,-7.62773293842389,
12.));
#233479=CARTESIAN_POINT('Ctrl Pts',(-21.814974061509,-7.62952367718126,
0.));
#233480=CARTESIAN_POINT('Ctrl Pts',(-21.814974061509,-7.62952367718126,
12.));
#233481=CARTESIAN_POINT('Ctrl Pts',(-21.8302631910195,-7.63128549323022,
0.));
#233482=CARTESIAN_POINT('Ctrl Pts',(-21.8302631910195,-7.63128549323022,
12.));
#233483=CARTESIAN_POINT('Ctrl Pts',(-21.8457037941084,-7.63301748948935,
0.));
#233484=CARTESIAN_POINT('Ctrl Pts',(-21.8457037941084,-7.63301748948935,
12.));
#233485=CARTESIAN_POINT('Ctrl Pts',(-21.8612943779089,-7.63471878821225,
0.));
#233486=CARTESIAN_POINT('Ctrl Pts',(-21.8612943779089,-7.63471878821225,
12.));
#233487=CARTESIAN_POINT('Ctrl Pts',(-21.8770334769496,-7.63638853033399,
0.));
#233488=CARTESIAN_POINT('Ctrl Pts',(-21.8770334769496,-7.63638853033399,
12.));
#233489=CARTESIAN_POINT('Ctrl Pts',(-21.8929196523514,-7.63802587492034,
0.));
#233490=CARTESIAN_POINT('Ctrl Pts',(-21.8929196523514,-7.63802587492034,
12.));
#233491=CARTESIAN_POINT('Ctrl Pts',(-21.9089514909874,-7.63962999860927,
0.));
#233492=CARTESIAN_POINT('Ctrl Pts',(-21.9089514909874,-7.63962999860927,
12.));
#233493=CARTESIAN_POINT('Ctrl Pts',(-21.9251276046546,-7.64120009506531,
0.));
#233494=CARTESIAN_POINT('Ctrl Pts',(-21.9251276046546,-7.64120009506531,
12.));
#233495=CARTESIAN_POINT('Ctrl Pts',(-21.9414466292072,-7.64273537442682,
0.));
#233496=CARTESIAN_POINT('Ctrl Pts',(-21.9414466292072,-7.64273537442682,
12.));
#233497=CARTESIAN_POINT('Ctrl Pts',(-21.9579072237651,-7.64423506279122,
0.));
#233498=CARTESIAN_POINT('Ctrl Pts',(-21.9579072237651,-7.64423506279122,
12.));
#233499=CARTESIAN_POINT('Ctrl Pts',(-21.9745080700798,-7.64569840177335,
0.));
#233500=CARTESIAN_POINT('Ctrl Pts',(-21.9745080700798,-7.64569840177335,
12.));
#233501=CARTESIAN_POINT('Ctrl Pts',(-21.9912478718542,-7.64712464805249,
0.));
#233502=CARTESIAN_POINT('Ctrl Pts',(-21.9912478718542,-7.64712464805249,
12.));
#233503=CARTESIAN_POINT('Ctrl Pts',(-22.0081253540774,-7.64851307293351,
0.));
#233504=CARTESIAN_POINT('Ctrl Pts',(-22.0081253540774,-7.64851307293351,
12.));
#233505=CARTESIAN_POINT('Ctrl Pts',(-22.0251392623209,-7.64986296190168,
0.));
#233506=CARTESIAN_POINT('Ctrl Pts',(-22.0251392623209,-7.64986296190168,
12.));
#233507=CARTESIAN_POINT('Ctrl Pts',(-22.0422883621174,-7.65117361421358,
0.));
#233508=CARTESIAN_POINT('Ctrl Pts',(-22.0422883621174,-7.65117361421358,
12.));
#233509=CARTESIAN_POINT('Ctrl Pts',(-22.0595714384431,-7.65244434253112,
0.));
#233510=CARTESIAN_POINT('Ctrl Pts',(-22.0595714384431,-7.65244434253112,
12.));
#233511=CARTESIAN_POINT('Ctrl Pts',(-22.0769872951596,-7.65367447254949,
0.));
#233512=CARTESIAN_POINT('Ctrl Pts',(-22.0769872951596,-7.65367447254949,
12.));
#233513=CARTESIAN_POINT('Ctrl Pts',(-22.094534754469,-7.65486334263643,
0.));
#233514=CARTESIAN_POINT('Ctrl Pts',(-22.094534754469,-7.65486334263643,
12.));
#233515=CARTESIAN_POINT('Ctrl Pts',(-22.1122126563329,-7.65601030346806,
0.));
#233516=CARTESIAN_POINT('Ctrl Pts',(-22.1122126563329,-7.65601030346806,
12.));
#233517=CARTESIAN_POINT('Ctrl Pts',(-22.1300198579675,-7.65711471769396,
0.));
#233518=CARTESIAN_POINT('Ctrl Pts',(-22.1300198579675,-7.65711471769396,
12.));
#233519=CARTESIAN_POINT('Ctrl Pts',(-22.1479552334211,-7.65817595963349,
0.));
#233520=CARTESIAN_POINT('Ctrl Pts',(-22.1479552334211,-7.65817595963349,
12.));
#233521=CARTESIAN_POINT('Ctrl Pts',(-22.1660176731178,-7.6591934149693,
0.));
#233522=CARTESIAN_POINT('Ctrl Pts',(-22.1660176731178,-7.6591934149693,
12.));
#233523=CARTESIAN_POINT('Ctrl Pts',(-22.1842060834091,-7.66016648045004,
0.));
#233524=CARTESIAN_POINT('Ctrl Pts',(-22.1842060834091,-7.66016648045004,
12.));
#233525=CARTESIAN_POINT('Ctrl Pts',(-22.2025193860964,-7.6610945635927,
0.));
#233526=CARTESIAN_POINT('Ctrl Pts',(-22.2025193860964,-7.6610945635927,
12.));
#233527=CARTESIAN_POINT('Ctrl Pts',(-22.2209565180085,-7.66197708240399,
0.));
#233528=CARTESIAN_POINT('Ctrl Pts',(-22.2209565180085,-7.66197708240399,
12.));
#233529=CARTESIAN_POINT('Ctrl Pts',(-22.2395164306547,-7.66281346512508,
0.));
#233530=CARTESIAN_POINT('Ctrl Pts',(-22.2395164306547,-7.66281346512508,
12.));
#233531=CARTESIAN_POINT('Ctrl Pts',(-22.258198089848,-7.6636031499764,0.));
#233532=CARTESIAN_POINT('Ctrl Pts',(-22.258198089848,-7.6636031499764,12.));
#233533=CARTESIAN_POINT('Ctrl Pts',(-22.2770004753335,-7.66434558490978,
0.));
#233534=CARTESIAN_POINT('Ctrl Pts',(-22.2770004753335,-7.66434558490978,
12.));
#233535=CARTESIAN_POINT('Ctrl Pts',(-22.2959225803937,-7.66504022736298,
0.));
#233536=CARTESIAN_POINT('Ctrl Pts',(-22.2959225803937,-7.66504022736298,
12.));
#233537=CARTESIAN_POINT('Ctrl Pts',(-22.314963411484,-7.66568654402493,
0.));
#233538=CARTESIAN_POINT('Ctrl Pts',(-22.314963411484,-7.66568654402493,
12.));
#233539=CARTESIAN_POINT('Ctrl Pts',(-22.3341219879469,-7.66628401061952,
0.));
#233540=CARTESIAN_POINT('Ctrl Pts',(-22.3341219879469,-7.66628401061952,
12.));
#233541=CARTESIAN_POINT('Ctrl Pts',(-22.3533973417021,-7.66683211169158,
0.));
#233542=CARTESIAN_POINT('Ctrl Pts',(-22.3533973417021,-7.66683211169158,
12.));
#233543=CARTESIAN_POINT('Ctrl Pts',(-22.372788516936,-7.66733034039882,
0.));
#233544=CARTESIAN_POINT('Ctrl Pts',(-22.372788516936,-7.66733034039882,
12.));
#233545=CARTESIAN_POINT('Ctrl Pts',(-22.3922945697773,-7.66777819830789,
0.));
#233546=CARTESIAN_POINT('Ctrl Pts',(-22.3922945697773,-7.66777819830789,
12.));
#233547=CARTESIAN_POINT('Ctrl Pts',(-22.4119145679758,-7.66817519519639,
0.));
#233548=CARTESIAN_POINT('Ctrl Pts',(-22.4119145679758,-7.66817519519639,
12.));
#233549=CARTESIAN_POINT('Ctrl Pts',(-22.4316475906603,-7.66852084886704,
0.));
#233550=CARTESIAN_POINT('Ctrl Pts',(-22.4316475906603,-7.66852084886704,
12.));
#233551=CARTESIAN_POINT('Ctrl Pts',(-22.4514927280855,-7.66881468496634,
0.));
#233552=CARTESIAN_POINT('Ctrl Pts',(-22.4514927280855,-7.66881468496634,
12.));
#233553=CARTESIAN_POINT('Ctrl Pts',(-22.47144908137,-7.6690562368083,0.));
#233554=CARTESIAN_POINT('Ctrl Pts',(-22.47144908137,-7.6690562368083,12.));
#233555=CARTESIAN_POINT('Ctrl Pts',(-22.4915157622312,-7.66924504520314,
0.));
#233556=CARTESIAN_POINT('Ctrl Pts',(-22.4915157622312,-7.66924504520314,
12.));
#233557=CARTESIAN_POINT('Ctrl Pts',(-22.5116918927032,-7.66938065829107,
0.));
#233558=CARTESIAN_POINT('Ctrl Pts',(-22.5116918927032,-7.66938065829107,
12.));
#233559=CARTESIAN_POINT('Ctrl Pts',(-22.53197660492,-7.66946263138143,0.));
#233560=CARTESIAN_POINT('Ctrl Pts',(-22.53197660492,-7.66946263138143,12.));
#233561=CARTESIAN_POINT('Ctrl Pts',(-22.5523690409116,-7.66949052679692,
0.));
#233562=CARTESIAN_POINT('Ctrl Pts',(-22.5523690409116,-7.66949052679692,
12.));
#233563=CARTESIAN_POINT('Ctrl Pts',(-22.5728683523831,-7.66946391372305,
0.));
#233564=CARTESIAN_POINT('Ctrl Pts',(-22.5728683523831,-7.66946391372305,
12.));
#233565=CARTESIAN_POINT('Ctrl Pts',(-22.5934737004953,-7.66938236806232,
0.));
#233566=CARTESIAN_POINT('Ctrl Pts',(-22.5934737004953,-7.66938236806232,
12.));
#233567=CARTESIAN_POINT('Ctrl Pts',(-22.6141842556243,-7.66924547229413,
0.));
#233568=CARTESIAN_POINT('Ctrl Pts',(-22.6141842556243,-7.66924547229413,
12.));
#233569=CARTESIAN_POINT('Ctrl Pts',(-22.6349991971541,-7.66905281533714,
0.));
#233570=CARTESIAN_POINT('Ctrl Pts',(-22.6349991971541,-7.66905281533714,
12.));
#233571=CARTESIAN_POINT('Ctrl Pts',(-22.6559177133127,-7.66880399241322,
0.));
#233572=CARTESIAN_POINT('Ctrl Pts',(-22.6559177133127,-7.66880399241322,
12.));
#233573=CARTESIAN_POINT('Ctrl Pts',(-22.6769390009885,-7.66849860491742,
0.));
#233574=CARTESIAN_POINT('Ctrl Pts',(-22.6769390009885,-7.66849860491742,
12.));
#233575=CARTESIAN_POINT('Ctrl Pts',(-22.6980622655446,-7.66813626029274,
0.));
#233576=CARTESIAN_POINT('Ctrl Pts',(-22.6980622655446,-7.66813626029274,
12.));
#233577=CARTESIAN_POINT('Ctrl Pts',(-22.7192867206245,-7.66771657191027,
0.));
#233578=CARTESIAN_POINT('Ctrl Pts',(-22.7192867206245,-7.66771657191027,
12.));
#233579=CARTESIAN_POINT('Ctrl Pts',(-22.7406115879513,-7.66723915895439,
0.));
#233580=CARTESIAN_POINT('Ctrl Pts',(-22.7406115879513,-7.66723915895439,
12.));
#233581=CARTESIAN_POINT('Ctrl Pts',(-22.7620360971843,-7.66670364630298,
0.));
#233582=CARTESIAN_POINT('Ctrl Pts',(-22.7620360971843,-7.66670364630298,
12.));
#233583=CARTESIAN_POINT('Ctrl Pts',(-22.7835594857699,-7.66610966441272,
0.));
#233584=CARTESIAN_POINT('Ctrl Pts',(-22.7835594857699,-7.66610966441272,
12.));
#233585=CARTESIAN_POINT('Ctrl Pts',(-22.8051809987833,-7.66545684920987,
0.));
#233586=CARTESIAN_POINT('Ctrl Pts',(-22.8051809987833,-7.66545684920987,
12.));
#233587=CARTESIAN_POINT('Ctrl Pts',(-22.8268998887678,-7.66474484198548,
0.));
#233588=CARTESIAN_POINT('Ctrl Pts',(-22.8268998887678,-7.66474484198548,
12.));
#233589=CARTESIAN_POINT('Ctrl Pts',(-22.848715415557,-7.66397328929802,
0.));
#233590=CARTESIAN_POINT('Ctrl Pts',(-22.848715415557,-7.66397328929802,
12.));
#233591=CARTESIAN_POINT('Ctrl Pts',(-22.8706268461283,-7.66314184287336,
0.));
#233592=CARTESIAN_POINT('Ctrl Pts',(-22.8706268461283,-7.66314184287336,
12.));
#233593=CARTESIAN_POINT('Ctrl Pts',(-22.8926334544883,-7.66225015950155,
0.));
#233594=CARTESIAN_POINT('Ctrl Pts',(-22.8926334544883,-7.66225015950155,
12.));
#233595=CARTESIAN_POINT('Ctrl Pts',(-22.9147345215421,-7.66129790094107,
0.));
#233596=CARTESIAN_POINT('Ctrl Pts',(-22.9147345215421,-7.66129790094107,
12.));
#233597=CARTESIAN_POINT('Ctrl Pts',(-22.9369293349593,-7.66028473382777,
0.));
#233598=CARTESIAN_POINT('Ctrl Pts',(-22.9369293349593,-7.66028473382777,
12.));
#233599=CARTESIAN_POINT('Ctrl Pts',(-22.959217189033,-7.65921032958901,
0.));
#233600=CARTESIAN_POINT('Ctrl Pts',(-22.959217189033,-7.65921032958901,
12.));
#233601=CARTESIAN_POINT('Ctrl Pts',(-22.9815973845296,-7.65807436436431,
0.));
#233602=CARTESIAN_POINT('Ctrl Pts',(-22.9815973845296,-7.65807436436431,
12.));
#233603=CARTESIAN_POINT('Ctrl Pts',(-23.0040692285814,-7.65687651891304,
0.));
#233604=CARTESIAN_POINT('Ctrl Pts',(-23.0040692285814,-7.65687651891304,
12.));
#233605=CARTESIAN_POINT('Ctrl Pts',(-23.0266320345787,-7.65561647852533,
0.));
#233606=CARTESIAN_POINT('Ctrl Pts',(-23.0266320345787,-7.65561647852533,
12.));
#233607=CARTESIAN_POINT('Ctrl Pts',(-23.0492851220528,-7.65429393293945,
0.));
#233608=CARTESIAN_POINT('Ctrl Pts',(-23.0492851220528,-7.65429393293945,
12.));
#233609=CARTESIAN_POINT('Ctrl Pts',(-23.072027816555,-7.65290857626357,
0.));
#233610=CARTESIAN_POINT('Ctrl Pts',(-23.072027816555,-7.65290857626357,
12.));
#233611=CARTESIAN_POINT('Ctrl Pts',(-23.094859449525,-7.65146010690475,
0.));
#233612=CARTESIAN_POINT('Ctrl Pts',(-23.094859449525,-7.65146010690475,
12.));
#233613=CARTESIAN_POINT('Ctrl Pts',(-23.1177793581679,-7.64994822749859,
0.));
#233614=CARTESIAN_POINT('Ctrl Pts',(-23.1177793581679,-7.64994822749859,
12.));
#233615=CARTESIAN_POINT('Ctrl Pts',(-23.1407868853819,-7.64837264482942,
0.));
#233616=CARTESIAN_POINT('Ctrl Pts',(-23.1407868853819,-7.64837264482942,
12.));
#233617=CARTESIAN_POINT('Ctrl Pts',(-23.1638813796694,-7.64673306975804,
0.));
#233618=CARTESIAN_POINT('Ctrl Pts',(-23.1638813796694,-7.64673306975804,
12.));
#233619=CARTESIAN_POINT('Ctrl Pts',(-23.1870621950452,-7.64502921715482,
0.));
#233620=CARTESIAN_POINT('Ctrl Pts',(-23.1870621950452,-7.64502921715482,
12.));
#233621=CARTESIAN_POINT('Ctrl Pts',(-23.2103286909398,-7.64326080583679,
0.));
#233622=CARTESIAN_POINT('Ctrl Pts',(-23.2103286909398,-7.64326080583679,
12.));
#233623=CARTESIAN_POINT('Ctrl Pts',(-23.2336802320912,-7.64142755851504,
0.));
#233624=CARTESIAN_POINT('Ctrl Pts',(-23.2336802320912,-7.64142755851504,
12.));
#233625=CARTESIAN_POINT('Ctrl Pts',(-23.2571161884488,-7.63952920172835,
0.));
#233626=CARTESIAN_POINT('Ctrl Pts',(-23.2571161884488,-7.63952920172835,
12.));
#233627=CARTESIAN_POINT('Ctrl Pts',(-23.2806359350855,-7.63756546576374,
0.));
#233628=CARTESIAN_POINT('Ctrl Pts',(-23.2806359350855,-7.63756546576374,
12.));
#233629=CARTESIAN_POINT('Ctrl Pts',(-23.3042388521022,-7.63553608458782,
0.));
#233630=CARTESIAN_POINT('Ctrl Pts',(-23.3042388521022,-7.63553608458782,
12.));
#233631=CARTESIAN_POINT('Ctrl Pts',(-23.3279243245241,-7.63344079578161,
0.));
#233632=CARTESIAN_POINT('Ctrl Pts',(-23.3279243245241,-7.63344079578161,
12.));
#233633=CARTESIAN_POINT('Ctrl Pts',(-23.3516917421972,-7.63127934048136,
0.));
#233634=CARTESIAN_POINT('Ctrl Pts',(-23.3516917421972,-7.63127934048136,
12.));
#233635=CARTESIAN_POINT('Ctrl Pts',(-23.3755404996636,-7.62905146332592,
0.));
#233636=CARTESIAN_POINT('Ctrl Pts',(-23.3755404996636,-7.62905146332592,
12.));
#233637=CARTESIAN_POINT('Ctrl Pts',(-23.399469996112,-7.62675691240328,
0.));
#233638=CARTESIAN_POINT('Ctrl Pts',(-23.399469996112,-7.62675691240328,
12.));
#233639=CARTESIAN_POINT('Ctrl Pts',(-23.4234796353542,-7.62439543920049,
0.));
#233640=CARTESIAN_POINT('Ctrl Pts',(-23.4234796353542,-7.62439543920049,
12.));
#233641=CARTESIAN_POINT('Ctrl Pts',(-23.4475688257854,-7.62196679855954,
0.));
#233642=CARTESIAN_POINT('Ctrl Pts',(-23.4475688257854,-7.62196679855954,
12.));
#233643=CARTESIAN_POINT('Ctrl Pts',(-23.4717369803438,-7.61947074863976,
0.));
#233644=CARTESIAN_POINT('Ctrl Pts',(-23.4717369803438,-7.61947074863976,
12.));
#233645=CARTESIAN_POINT('Ctrl Pts',(-23.4959835164609,-7.61690705088318,
0.));
#233646=CARTESIAN_POINT('Ctrl Pts',(-23.4959835164609,-7.61690705088318,
12.));
#233647=CARTESIAN_POINT('Ctrl Pts',(-23.5203078560129,-7.61427546999297,
0.));
#233648=CARTESIAN_POINT('Ctrl Pts',(-23.5203078560129,-7.61427546999297,
12.));
#233649=CARTESIAN_POINT('Ctrl Pts',(-23.544709425203,-7.61157577385371,
0.));
#233650=CARTESIAN_POINT('Ctrl Pts',(-23.544709425203,-7.61157577385371,
12.));
#233651=CARTESIAN_POINT('Ctrl Pts',(-23.5691876544244,-7.60880773344599,
0.));
#233652=CARTESIAN_POINT('Ctrl Pts',(-23.5691876544244,-7.60880773344599,
12.));
#233653=CARTESIAN_POINT('Ctrl Pts',(-23.5937419781245,-7.60597112277093,
0.));
#233654=CARTESIAN_POINT('Ctrl Pts',(-23.5937419781245,-7.60597112277093,
12.));
#233655=CARTESIAN_POINT('Ctrl Pts',(-23.6183718346576,-7.60306571877805,
0.));
#233656=CARTESIAN_POINT('Ctrl Pts',(-23.6183718346576,-7.60306571877805,
12.));
#233657=CARTESIAN_POINT('Ctrl Pts',(-23.6430766661418,-7.60009130130125,
0.));
#233658=CARTESIAN_POINT('Ctrl Pts',(-23.6430766661418,-7.60009130130125,
12.));
#233659=CARTESIAN_POINT('Ctrl Pts',(-23.6678559182875,-7.59704765299566,
0.));
#233660=CARTESIAN_POINT('Ctrl Pts',(-23.6678559182875,-7.59704765299566,
12.));
#233661=CARTESIAN_POINT('Ctrl Pts',(-23.6927090405066,-7.59393455934034,
0.));
#233662=CARTESIAN_POINT('Ctrl Pts',(-23.6927090405066,-7.59393455934034,
12.));
#233663=CARTESIAN_POINT('Ctrl Pts',(-23.7176354860457,-7.5907518086532,
0.));
#233664=CARTESIAN_POINT('Ctrl Pts',(-23.7176354860457,-7.5907518086532,
12.));
#233665=CARTESIAN_POINT('Ctrl Pts',(-23.7426347121006,-7.58749919210825,
0.));
#233666=CARTESIAN_POINT('Ctrl Pts',(-23.7426347121006,-7.58749919210825,
12.));
#233667=CARTESIAN_POINT('Ctrl Pts',(-23.7677061799376,-7.5841765037627,
0.));
#233668=CARTESIAN_POINT('Ctrl Pts',(-23.7677061799376,-7.5841765037627,
12.));
#233669=CARTESIAN_POINT('Ctrl Pts',(-23.7928493549908,-7.58078354058212,
0.));
#233670=CARTESIAN_POINT('Ctrl Pts',(-23.7928493549908,-7.58078354058212,
12.));
#233671=CARTESIAN_POINT('Ctrl Pts',(-23.8180637069976,-7.57732010249065,
0.));
#233672=CARTESIAN_POINT('Ctrl Pts',(-23.8180637069976,-7.57732010249065,
12.));
#233673=CARTESIAN_POINT('Ctrl Pts',(-23.8433487096132,-7.57378599219814,
0.));
#233674=CARTESIAN_POINT('Ctrl Pts',(-23.8433487096132,-7.57378599219814,
12.));
#233675=CARTESIAN_POINT('Ctrl Pts',(-23.8687038399595,-7.57018101500709,
0.));
#233676=CARTESIAN_POINT('Ctrl Pts',(-23.8687038399595,-7.57018101500709,
12.));
#233677=CARTESIAN_POINT('Ctrl Pts',(-23.8941285782002,-7.5665049786379,
0.));
#233678=CARTESIAN_POINT('Ctrl Pts',(-23.8941285782002,-7.5665049786379,
12.));
#233679=CARTESIAN_POINT('Ctrl Pts',(-23.9196224070759,-7.56275769304772,
0.));
#233680=CARTESIAN_POINT('Ctrl Pts',(-23.9196224070759,-7.56275769304772,
12.));
#233681=CARTESIAN_POINT('Ctrl Pts',(-23.9451848115002,-7.55893897027679,
0.));
#233682=CARTESIAN_POINT('Ctrl Pts',(-23.9451848115002,-7.55893897027679,
12.));
#233683=CARTESIAN_POINT('Ctrl Pts',(-23.9708152779886,-7.55504862424807,
0.));
#233684=CARTESIAN_POINT('Ctrl Pts',(-23.9708152779886,-7.55504862424807,
12.));
#233685=CARTESIAN_POINT('Ctrl Pts',(-23.9965132953187,-7.55108647097431,
0.));
#233686=CARTESIAN_POINT('Ctrl Pts',(-23.9965132953187,-7.55108647097431,
12.));
#233687=CARTESIAN_POINT('Ctrl Pts',(-24.0222783554531,-7.54705232885894,
0.));
#233688=CARTESIAN_POINT('Ctrl Pts',(-24.0222783554531,-7.54705232885894,
12.));
#233689=CARTESIAN_POINT('Ctrl Pts',(-24.0481099543353,-7.54294601896127,
0.));
#233690=CARTESIAN_POINT('Ctrl Pts',(-24.0481099543353,-7.54294601896127,
12.));
#233691=CARTESIAN_POINT('Ctrl Pts',(-24.0740075927984,-7.53876736531004,
0.));
#233692=CARTESIAN_POINT('Ctrl Pts',(-24.0740075927984,-7.53876736531004,
12.));
#233693=CARTESIAN_POINT('Ctrl Pts',(-24.0999707772643,-7.53451619514658,
0.));
#233694=CARTESIAN_POINT('Ctrl Pts',(-24.0999707772643,-7.53451619514658,
12.));
#233695=CARTESIAN_POINT('Ctrl Pts',(-24.1259990209211,-7.53019233935536,
0.));
#233696=CARTESIAN_POINT('Ctrl Pts',(-24.1259990209211,-7.53019233935536,
12.));
#233697=CARTESIAN_POINT('Ctrl Pts',(-24.152091842537,-7.52579563201478,
0.));
#233698=CARTESIAN_POINT('Ctrl Pts',(-24.152091842537,-7.52579563201478,
12.));
#233699=CARTESIAN_POINT('Ctrl Pts',(-24.1782487641602,-7.52132590953862,
0.));
#233700=CARTESIAN_POINT('Ctrl Pts',(-24.1782487641602,-7.52132590953862,
12.));
#233701=CARTESIAN_POINT('Ctrl Pts',(-24.2044693092356,-7.51678300997997,
0.));
#233702=CARTESIAN_POINT('Ctrl Pts',(-24.2044693092356,-7.51678300997997,
12.));
#233703=CARTESIAN_POINT('Ctrl Pts',(-24.230753000389,-7.51216677222198,
0.));
#233704=CARTESIAN_POINT('Ctrl Pts',(-24.230753000389,-7.51216677222198,
12.));
#233705=CARTESIAN_POINT('Ctrl Pts',(-24.2570993577032,-7.50747703535114,
0.));
#233706=CARTESIAN_POINT('Ctrl Pts',(-24.2570993577032,-7.50747703535114,
12.));
#233707=CARTESIAN_POINT('Ctrl Pts',(-24.2835078958966,-7.50271363765098,
0.));
#233708=CARTESIAN_POINT('Ctrl Pts',(-24.2835078958966,-7.50271363765098,
12.));
#233709=CARTESIAN_POINT('Ctrl Pts',(-24.3099781253345,-7.49787641695358,
0.));
#233710=CARTESIAN_POINT('Ctrl Pts',(-24.3099781253345,-7.49787641695358,
12.));
#233711=CARTESIAN_POINT('Ctrl Pts',(-24.3365095573673,-7.49296521252329,
0.));
#233712=CARTESIAN_POINT('Ctrl Pts',(-24.3365095573673,-7.49296521252329,
12.));
#233713=CARTESIAN_POINT('Ctrl Pts',(-24.3631017084513,-7.48797986651827,
0.));
#233714=CARTESIAN_POINT('Ctrl Pts',(-24.3631017084513,-7.48797986651827,
12.));
#233715=CARTESIAN_POINT('Ctrl Pts',(-24.3897541049248,-7.48292022569253,
0.));
#233716=CARTESIAN_POINT('Ctrl Pts',(-24.3897541049248,-7.48292022569253,
12.));
#233717=CARTESIAN_POINT('Ctrl Pts',(-24.4164662871165,-7.47778614286573,
0.));
#233718=CARTESIAN_POINT('Ctrl Pts',(-24.4164662871165,-7.47778614286573,
12.));
#233719=CARTESIAN_POINT('Ctrl Pts',(-24.4432378146501,-7.47257747883318,
0.));
#233720=CARTESIAN_POINT('Ctrl Pts',(-24.4432378146501,-7.47257747883318,
12.));
#233721=CARTESIAN_POINT('Ctrl Pts',(-24.4700682684544,-7.46729410308922,
0.));
#233722=CARTESIAN_POINT('Ctrl Pts',(-24.4700682684544,-7.46729410308922,
12.));
#233723=CARTESIAN_POINT('Ctrl Pts',(-24.4969572391509,-7.46193588961641,
0.));
#233724=CARTESIAN_POINT('Ctrl Pts',(-24.4969572391509,-7.46193588961641,
12.));
#233725=CARTESIAN_POINT('Ctrl Pts',(-24.52390431731,-7.45650271336045,0.));
#233726=CARTESIAN_POINT('Ctrl Pts',(-24.52390431731,-7.45650271336045,12.));
#233727=CARTESIAN_POINT('Ctrl Pts',(-24.5509090831579,-7.45099444651295,
0.));
#233728=CARTESIAN_POINT('Ctrl Pts',(-24.5509090831579,-7.45099444651295,
12.));
#233729=CARTESIAN_POINT('Ctrl Pts',(-24.5779710960865,-7.44541095473162,
0.));
#233730=CARTESIAN_POINT('Ctrl Pts',(-24.5779710960865,-7.44541095473162,
12.));
#233731=CARTESIAN_POINT('Ctrl Pts',(-24.6050898852349,-7.43975209375374,
0.));
#233732=CARTESIAN_POINT('Ctrl Pts',(-24.6050898852349,-7.43975209375374,
12.));
#233733=CARTESIAN_POINT('Ctrl Pts',(-24.6322649369472,-7.4340177048922,
0.));
#233734=CARTESIAN_POINT('Ctrl Pts',(-24.6322649369472,-7.4340177048922,
12.));
#233735=CARTESIAN_POINT('Ctrl Pts',(-24.659495712869,-7.4282076215868,0.));
#233736=CARTESIAN_POINT('Ctrl Pts',(-24.659495712869,-7.4282076215868,12.));
#233737=CARTESIAN_POINT('Ctrl Pts',(-24.6867816727118,-7.42232167765762,
0.));
#233738=CARTESIAN_POINT('Ctrl Pts',(-24.6867816727118,-7.42232167765762,
12.));
#233739=CARTESIAN_POINT('Ctrl Pts',(-24.7141222949988,-7.41635971481243,
0.));
#233740=CARTESIAN_POINT('Ctrl Pts',(-24.7141222949988,-7.41635971481243,
12.));
#233741=CARTESIAN_POINT('Ctrl Pts',(-24.7415170994754,-7.41032159082173,
0.));
#233742=CARTESIAN_POINT('Ctrl Pts',(-24.7415170994754,-7.41032159082173,
12.));
#233743=CARTESIAN_POINT('Ctrl Pts',(-24.7689656669005,-7.40420718661754,
0.));
#233744=CARTESIAN_POINT('Ctrl Pts',(-24.7689656669005,-7.40420718661754,
12.));
#233745=CARTESIAN_POINT('Ctrl Pts',(-24.7964676646518,-7.39801641583612,
0.));
#233746=CARTESIAN_POINT('Ctrl Pts',(-24.7964676646518,-7.39801641583612,
12.));
#233747=CARTESIAN_POINT('Ctrl Pts',(-24.8240228521042,-7.39174922586841,
0.));
#233748=CARTESIAN_POINT('Ctrl Pts',(-24.8240228521042,-7.39174922586841,
12.));
#233749=CARTESIAN_POINT('Ctrl Pts',(-24.8516310625367,-7.38540558904945,
0.));
#233750=CARTESIAN_POINT('Ctrl Pts',(-24.8516310625367,-7.38540558904945,
12.));
#233751=CARTESIAN_POINT('Ctrl Pts',(-24.8792921911309,-7.3789854964161,
0.));
#233752=CARTESIAN_POINT('Ctrl Pts',(-24.8792921911309,-7.3789854964161,
12.));
#233753=CARTESIAN_POINT('Ctrl Pts',(-24.9014633826201,-7.37378825962717,
0.));
#233754=CARTESIAN_POINT('Ctrl Pts',(-24.9014633826201,-7.37378825962717,
12.));
#233755=CARTESIAN_POINT('Ctrl Pts',(-24.9181155530631,-7.36985593120696,
0.));
#233756=CARTESIAN_POINT('Ctrl Pts',(-24.9181155530631,-7.36985593120696,
12.));
#233757=CARTESIAN_POINT('Ctrl Pts',(-24.9292275670705,-7.36721909029059,
0.));
#233758=CARTESIAN_POINT('Ctrl Pts',(-24.9292275670705,-7.36721909029059,
12.));
#233759=CARTESIAN_POINT('Ctrl Pts',(-24.9347862158358,-7.36589684767343,
0.));
#233760=CARTESIAN_POINT('Ctrl Pts',(-24.9347862158358,-7.36589684767343,
12.));
#233761=CARTESIAN_POINT('',(-24.9347862158358,-7.36589684767343,0.));
#233762=CARTESIAN_POINT('Ctrl Pts',(-21.2610617890679,-7.52250298901264,
0.));
#233763=CARTESIAN_POINT('Ctrl Pts',(-21.2610673466886,-7.5225064970397,
0.));
#233764=CARTESIAN_POINT('Ctrl Pts',(-21.2611204474866,-7.52252744144903,
0.));
#233765=CARTESIAN_POINT('Ctrl Pts',(-21.261326054066,-7.5226006423166,0.));
#233766=CARTESIAN_POINT('Ctrl Pts',(-21.2618521283555,-7.52278182242669,
0.));
#233767=CARTESIAN_POINT('Ctrl Pts',(-21.262927782038,-7.52314642316199,
0.));
#233768=CARTESIAN_POINT('Ctrl Pts',(-21.2644161259962,-7.52364573027552,
0.));
#233769=CARTESIAN_POINT('Ctrl Pts',(-21.2663059157058,-7.52427261074297,
0.));
#233770=CARTESIAN_POINT('Ctrl Pts',(-21.2685823838671,-7.5250177033353,
0.));
#233771=CARTESIAN_POINT('Ctrl Pts',(-21.2712301573466,-7.52587126095529,
0.));
#233772=CARTESIAN_POINT('Ctrl Pts',(-21.2742366113579,-7.5268252691854,
0.));
#233773=CARTESIAN_POINT('Ctrl Pts',(-21.2775925269652,-7.52787386225332,
0.));
#233774=CARTESIAN_POINT('Ctrl Pts',(-21.2812902781143,-7.52901217930407,
0.));
#233775=CARTESIAN_POINT('Ctrl Pts',(-21.2853226580657,-7.53023562438229,
0.));
#233776=CARTESIAN_POINT('Ctrl Pts',(-21.2896816163842,-7.53153906987855,
0.));
#233777=CARTESIAN_POINT('Ctrl Pts',(-21.2943588989331,-7.53291726078526,
0.));
#233778=CARTESIAN_POINT('Ctrl Pts',(-21.2993464250717,-7.53436505309942,
0.));
#233779=CARTESIAN_POINT('Ctrl Pts',(-21.3046368712157,-7.53587778251735,
0.));
#233780=CARTESIAN_POINT('Ctrl Pts',(-21.310223716773,-7.53745129364616,
0.));
#233781=CARTESIAN_POINT('Ctrl Pts',(-21.3161009456256,-7.53908175169898,
0.));
#233782=CARTESIAN_POINT('Ctrl Pts',(-21.3222628524165,-7.54076552038278,
0.));
#233783=CARTESIAN_POINT('Ctrl Pts',(-21.328703791771,-7.5424990037703,0.));
#233784=CARTESIAN_POINT('Ctrl Pts',(-21.3354182340149,-7.54427868151267,
0.));
#233785=CARTESIAN_POINT('Ctrl Pts',(-21.3424008295038,-7.54610114948346,
0.));
#233786=CARTESIAN_POINT('Ctrl Pts',(-21.3496464761531,-7.5479631624633,
0.));
#233787=CARTESIAN_POINT('Ctrl Pts',(-21.3571503685855,-7.54986166521309,
0.));
#233788=CARTESIAN_POINT('Ctrl Pts',(-21.3649079431865,-7.55179375777443,
0.));
#233789=CARTESIAN_POINT('Ctrl Pts',(-21.3729148390243,-7.55375667080028,
0.));
#233790=CARTESIAN_POINT('Ctrl Pts',(-21.3811668478932,-7.55574773403502,
0.));
#233791=CARTESIAN_POINT('Ctrl Pts',(-21.3896598842117,-7.55776435731416,
0.));
#233792=CARTESIAN_POINT('Ctrl Pts',(-21.3983899952987,-7.5598040370061,
0.));
#233793=CARTESIAN_POINT('Ctrl Pts',(-21.4073533630365,-7.56186435703621,
0.));
#233794=CARTESIAN_POINT('Ctrl Pts',(-21.4165463106254,-7.56394299313684,
0.));
#233795=CARTESIAN_POINT('Ctrl Pts',(-21.4259653015736,-7.56603771218712,
0.));
#233796=CARTESIAN_POINT('Ctrl Pts',(-21.4356069261513,-7.56814636360847,
0.));
#233797=CARTESIAN_POINT('Ctrl Pts',(-21.4454678907509,-7.57026687261165,
0.));
#233798=CARTESIAN_POINT('Ctrl Pts',(-21.4555450053142,-7.57239723223505,
0.));
#233799=CARTESIAN_POINT('Ctrl Pts',(-21.4658351740128,-7.57453549743411,
0.));
#233800=CARTESIAN_POINT('Ctrl Pts',(-21.4763353936762,-7.57667978402987,
0.));
#233801=CARTESIAN_POINT('Ctrl Pts',(-21.4870427508194,-7.57882826679131,
0.));
#233802=CARTESIAN_POINT('Ctrl Pts',(-21.4979544192744,-7.58097917790744,
0.));
#233803=CARTESIAN_POINT('Ctrl Pts',(-21.5090676573873,-7.58313080519179,
0.));
#233804=CARTESIAN_POINT('Ctrl Pts',(-21.5203798035299,-7.58528148919129,
0.));
#233805=CARTESIAN_POINT('Ctrl Pts',(-21.5318882716736,-7.58742962034833,
0.));
#233806=CARTESIAN_POINT('Ctrl Pts',(-21.543590547011,-7.58957363620013,
0.));
#233807=CARTESIAN_POINT('Ctrl Pts',(-21.5554841813462,-7.59171201844776,
0.));
#233808=CARTESIAN_POINT('Ctrl Pts',(-21.5675667904726,-7.59384329124918,
0.));
#233809=CARTESIAN_POINT('Ctrl Pts',(-21.5798360518978,-7.59596601973583,
0.));
#233810=CARTESIAN_POINT('Ctrl Pts',(-21.5922897024466,-7.59807880846194,
0.));
#233811=CARTESIAN_POINT('Ctrl Pts',(-21.6049255358843,-7.6001802998824,
0.));
#233812=CARTESIAN_POINT('Ctrl Pts',(-21.617741400599,-7.60226917285428,
0.));
#233813=CARTESIAN_POINT('Ctrl Pts',(-21.6307351973822,-7.60434414118295,
0.));
#233814=CARTESIAN_POINT('Ctrl Pts',(-21.6439048771743,-7.60640395216356,
0.));
#233815=CARTESIAN_POINT('Ctrl Pts',(-21.6572484388081,-7.60844738512873,
0.));
#233816=CARTESIAN_POINT('Ctrl Pts',(-21.6707639267576,-7.61047325000955,
0.));
#233817=CARTESIAN_POINT('Ctrl Pts',(-21.6844494295815,-7.61248038630268,
0.));
#233818=CARTESIAN_POINT('Ctrl Pts',(-21.6983030783322,-7.61446766202786,
0.));
#233819=CARTESIAN_POINT('Ctrl Pts',(-21.7123230449834,-7.6164339727042,
0.));
#233820=CARTESIAN_POINT('Ctrl Pts',(-21.7265075407975,-7.61837824030537,
0.));
#233821=CARTESIAN_POINT('Ctrl Pts',(-21.7408548148656,-7.62029941230854,
0.));
#233822=CARTESIAN_POINT('Ctrl Pts',(-21.7553631528328,-7.62219646084228,
0.));
#233823=CARTESIAN_POINT('Ctrl Pts',(-21.7700308755584,-7.62406838181166,
0.));
#233824=CARTESIAN_POINT('Ctrl Pts',(-21.7848563378021,-7.62591419404512,
0.));
#233825=CARTESIAN_POINT('Ctrl Pts',(-21.799837926858,-7.62773293842389,
0.));
#233826=CARTESIAN_POINT('Ctrl Pts',(-21.814974061509,-7.62952367718126,
0.));
#233827=CARTESIAN_POINT('Ctrl Pts',(-21.8302631910195,-7.63128549323022,
0.));
#233828=CARTESIAN_POINT('Ctrl Pts',(-21.8457037941084,-7.63301748948935,
0.));
#233829=CARTESIAN_POINT('Ctrl Pts',(-21.8612943779089,-7.63471878821225,
0.));
#233830=CARTESIAN_POINT('Ctrl Pts',(-21.8770334769496,-7.63638853033399,
0.));
#233831=CARTESIAN_POINT('Ctrl Pts',(-21.8929196523514,-7.63802587492034,
0.));
#233832=CARTESIAN_POINT('Ctrl Pts',(-21.9089514909874,-7.63962999860927,
0.));
#233833=CARTESIAN_POINT('Ctrl Pts',(-21.9251276046546,-7.64120009506531,
0.));
#233834=CARTESIAN_POINT('Ctrl Pts',(-21.9414466292072,-7.64273537442682,
0.));
#233835=CARTESIAN_POINT('Ctrl Pts',(-21.9579072237651,-7.64423506279122,
0.));
#233836=CARTESIAN_POINT('Ctrl Pts',(-21.9745080700798,-7.64569840177335,
0.));
#233837=CARTESIAN_POINT('Ctrl Pts',(-21.9912478718542,-7.64712464805249,
0.));
#233838=CARTESIAN_POINT('Ctrl Pts',(-22.0081253540774,-7.64851307293351,
0.));
#233839=CARTESIAN_POINT('Ctrl Pts',(-22.0251392623209,-7.64986296190168,
0.));
#233840=CARTESIAN_POINT('Ctrl Pts',(-22.0422883621174,-7.65117361421358,
0.));
#233841=CARTESIAN_POINT('Ctrl Pts',(-22.0595714384431,-7.65244434253112,
0.));
#233842=CARTESIAN_POINT('Ctrl Pts',(-22.0769872951596,-7.65367447254949,
0.));
#233843=CARTESIAN_POINT('Ctrl Pts',(-22.094534754469,-7.65486334263643,
0.));
#233844=CARTESIAN_POINT('Ctrl Pts',(-22.1122126563329,-7.65601030346806,
0.));
#233845=CARTESIAN_POINT('Ctrl Pts',(-22.1300198579675,-7.65711471769396,
0.));
#233846=CARTESIAN_POINT('Ctrl Pts',(-22.1479552334211,-7.65817595963349,
0.));
#233847=CARTESIAN_POINT('Ctrl Pts',(-22.1660176731178,-7.6591934149693,
0.));
#233848=CARTESIAN_POINT('Ctrl Pts',(-22.1842060834091,-7.66016648045004,
0.));
#233849=CARTESIAN_POINT('Ctrl Pts',(-22.2025193860964,-7.6610945635927,
0.));
#233850=CARTESIAN_POINT('Ctrl Pts',(-22.2209565180085,-7.66197708240399,
0.));
#233851=CARTESIAN_POINT('Ctrl Pts',(-22.2395164306547,-7.66281346512508,
0.));
#233852=CARTESIAN_POINT('Ctrl Pts',(-22.258198089848,-7.6636031499764,0.));
#233853=CARTESIAN_POINT('Ctrl Pts',(-22.2770004753335,-7.66434558490978,
0.));
#233854=CARTESIAN_POINT('Ctrl Pts',(-22.2959225803937,-7.66504022736298,
0.));
#233855=CARTESIAN_POINT('Ctrl Pts',(-22.314963411484,-7.66568654402493,
0.));
#233856=CARTESIAN_POINT('Ctrl Pts',(-22.3341219879469,-7.66628401061952,
0.));
#233857=CARTESIAN_POINT('Ctrl Pts',(-22.3533973417021,-7.66683211169158,
0.));
#233858=CARTESIAN_POINT('Ctrl Pts',(-22.372788516936,-7.66733034039882,
0.));
#233859=CARTESIAN_POINT('Ctrl Pts',(-22.3922945697773,-7.66777819830789,
0.));
#233860=CARTESIAN_POINT('Ctrl Pts',(-22.4119145679758,-7.66817519519639,
0.));
#233861=CARTESIAN_POINT('Ctrl Pts',(-22.4316475906603,-7.66852084886704,
0.));
#233862=CARTESIAN_POINT('Ctrl Pts',(-22.4514927280855,-7.66881468496634,
0.));
#233863=CARTESIAN_POINT('Ctrl Pts',(-22.47144908137,-7.6690562368083,0.));
#233864=CARTESIAN_POINT('Ctrl Pts',(-22.4915157622312,-7.66924504520314,
0.));
#233865=CARTESIAN_POINT('Ctrl Pts',(-22.5116918927032,-7.66938065829107,
0.));
#233866=CARTESIAN_POINT('Ctrl Pts',(-22.53197660492,-7.66946263138143,0.));
#233867=CARTESIAN_POINT('Ctrl Pts',(-22.5523690409116,-7.66949052679692,
0.));
#233868=CARTESIAN_POINT('Ctrl Pts',(-22.5728683523831,-7.66946391372305,
0.));
#233869=CARTESIAN_POINT('Ctrl Pts',(-22.5934737004953,-7.66938236806232,
0.));
#233870=CARTESIAN_POINT('Ctrl Pts',(-22.6141842556243,-7.66924547229413,
0.));
#233871=CARTESIAN_POINT('Ctrl Pts',(-22.6349991971541,-7.66905281533714,
0.));
#233872=CARTESIAN_POINT('Ctrl Pts',(-22.6559177133127,-7.66880399241322,
0.));
#233873=CARTESIAN_POINT('Ctrl Pts',(-22.6769390009885,-7.66849860491742,
0.));
#233874=CARTESIAN_POINT('Ctrl Pts',(-22.6980622655446,-7.66813626029274,
0.));
#233875=CARTESIAN_POINT('Ctrl Pts',(-22.7192867206245,-7.66771657191027,
0.));
#233876=CARTESIAN_POINT('Ctrl Pts',(-22.7406115879513,-7.66723915895439,
0.));
#233877=CARTESIAN_POINT('Ctrl Pts',(-22.7620360971843,-7.66670364630298,
0.));
#233878=CARTESIAN_POINT('Ctrl Pts',(-22.7835594857699,-7.66610966441272,
0.));
#233879=CARTESIAN_POINT('Ctrl Pts',(-22.8051809987833,-7.66545684920987,
0.));
#233880=CARTESIAN_POINT('Ctrl Pts',(-22.8268998887678,-7.66474484198548,
0.));
#233881=CARTESIAN_POINT('Ctrl Pts',(-22.848715415557,-7.66397328929802,
0.));
#233882=CARTESIAN_POINT('Ctrl Pts',(-22.8706268461283,-7.66314184287336,
0.));
#233883=CARTESIAN_POINT('Ctrl Pts',(-22.8926334544883,-7.66225015950155,
0.));
#233884=CARTESIAN_POINT('Ctrl Pts',(-22.9147345215421,-7.66129790094107,
0.));
#233885=CARTESIAN_POINT('Ctrl Pts',(-22.9369293349593,-7.66028473382777,
0.));
#233886=CARTESIAN_POINT('Ctrl Pts',(-22.959217189033,-7.65921032958901,
0.));
#233887=CARTESIAN_POINT('Ctrl Pts',(-22.9815973845296,-7.65807436436431,
0.));
#233888=CARTESIAN_POINT('Ctrl Pts',(-23.0040692285814,-7.65687651891304,
0.));
#233889=CARTESIAN_POINT('Ctrl Pts',(-23.0266320345787,-7.65561647852533,
0.));
#233890=CARTESIAN_POINT('Ctrl Pts',(-23.0492851220528,-7.65429393293945,
0.));
#233891=CARTESIAN_POINT('Ctrl Pts',(-23.072027816555,-7.65290857626357,
0.));
#233892=CARTESIAN_POINT('Ctrl Pts',(-23.094859449525,-7.65146010690475,
0.));
#233893=CARTESIAN_POINT('Ctrl Pts',(-23.1177793581679,-7.64994822749859,
0.));
#233894=CARTESIAN_POINT('Ctrl Pts',(-23.1407868853819,-7.64837264482942,
0.));
#233895=CARTESIAN_POINT('Ctrl Pts',(-23.1638813796694,-7.64673306975804,
0.));
#233896=CARTESIAN_POINT('Ctrl Pts',(-23.1870621950452,-7.64502921715482,
0.));
#233897=CARTESIAN_POINT('Ctrl Pts',(-23.2103286909398,-7.64326080583679,
0.));
#233898=CARTESIAN_POINT('Ctrl Pts',(-23.2336802320912,-7.64142755851504,
0.));
#233899=CARTESIAN_POINT('Ctrl Pts',(-23.2571161884488,-7.63952920172835,
0.));
#233900=CARTESIAN_POINT('Ctrl Pts',(-23.2806359350855,-7.63756546576374,
0.));
#233901=CARTESIAN_POINT('Ctrl Pts',(-23.3042388521022,-7.63553608458782,
0.));
#233902=CARTESIAN_POINT('Ctrl Pts',(-23.3279243245241,-7.63344079578161,
0.));
#233903=CARTESIAN_POINT('Ctrl Pts',(-23.3516917421972,-7.63127934048136,
0.));
#233904=CARTESIAN_POINT('Ctrl Pts',(-23.3755404996636,-7.62905146332592,
0.));
#233905=CARTESIAN_POINT('Ctrl Pts',(-23.399469996112,-7.62675691240328,
0.));
#233906=CARTESIAN_POINT('Ctrl Pts',(-23.4234796353542,-7.62439543920049,
0.));
#233907=CARTESIAN_POINT('Ctrl Pts',(-23.4475688257854,-7.62196679855954,
0.));
#233908=CARTESIAN_POINT('Ctrl Pts',(-23.4717369803438,-7.61947074863976,
0.));
#233909=CARTESIAN_POINT('Ctrl Pts',(-23.4959835164609,-7.61690705088318,
0.));
#233910=CARTESIAN_POINT('Ctrl Pts',(-23.5203078560129,-7.61427546999297,
0.));
#233911=CARTESIAN_POINT('Ctrl Pts',(-23.544709425203,-7.61157577385371,
0.));
#233912=CARTESIAN_POINT('Ctrl Pts',(-23.5691876544244,-7.60880773344599,
0.));
#233913=CARTESIAN_POINT('Ctrl Pts',(-23.5937419781245,-7.60597112277093,
0.));
#233914=CARTESIAN_POINT('Ctrl Pts',(-23.6183718346576,-7.60306571877805,
0.));
#233915=CARTESIAN_POINT('Ctrl Pts',(-23.6430766661418,-7.60009130130125,
0.));
#233916=CARTESIAN_POINT('Ctrl Pts',(-23.6678559182875,-7.59704765299566,
0.));
#233917=CARTESIAN_POINT('Ctrl Pts',(-23.6927090405066,-7.59393455934034,
0.));
#233918=CARTESIAN_POINT('Ctrl Pts',(-23.7176354860457,-7.5907518086532,
0.));
#233919=CARTESIAN_POINT('Ctrl Pts',(-23.7426347121006,-7.58749919210825,
0.));
#233920=CARTESIAN_POINT('Ctrl Pts',(-23.7677061799376,-7.5841765037627,
0.));
#233921=CARTESIAN_POINT('Ctrl Pts',(-23.7928493549908,-7.58078354058212,
0.));
#233922=CARTESIAN_POINT('Ctrl Pts',(-23.8180637069976,-7.57732010249065,
0.));
#233923=CARTESIAN_POINT('Ctrl Pts',(-23.8433487096132,-7.57378599219814,
0.));
#233924=CARTESIAN_POINT('Ctrl Pts',(-23.8687038399595,-7.57018101500709,
0.));
#233925=CARTESIAN_POINT('Ctrl Pts',(-23.8941285782002,-7.5665049786379,
0.));
#233926=CARTESIAN_POINT('Ctrl Pts',(-23.9196224070759,-7.56275769304772,
0.));
#233927=CARTESIAN_POINT('Ctrl Pts',(-23.9451848115002,-7.55893897027679,
0.));
#233928=CARTESIAN_POINT('Ctrl Pts',(-23.9708152779886,-7.55504862424807,
0.));
#233929=CARTESIAN_POINT('Ctrl Pts',(-23.9965132953187,-7.55108647097431,
0.));
#233930=CARTESIAN_POINT('Ctrl Pts',(-24.0222783554531,-7.54705232885894,
0.));
#233931=CARTESIAN_POINT('Ctrl Pts',(-24.0481099543353,-7.54294601896127,
0.));
#233932=CARTESIAN_POINT('Ctrl Pts',(-24.0740075927984,-7.53876736531004,
0.));
#233933=CARTESIAN_POINT('Ctrl Pts',(-24.0999707772643,-7.53451619514658,
0.));
#233934=CARTESIAN_POINT('Ctrl Pts',(-24.1259990209211,-7.53019233935536,
0.));
#233935=CARTESIAN_POINT('Ctrl Pts',(-24.152091842537,-7.52579563201478,
0.));
#233936=CARTESIAN_POINT('Ctrl Pts',(-24.1782487641602,-7.52132590953862,
0.));
#233937=CARTESIAN_POINT('Ctrl Pts',(-24.2044693092356,-7.51678300997997,
0.));
#233938=CARTESIAN_POINT('Ctrl Pts',(-24.230753000389,-7.51216677222198,
0.));
#233939=CARTESIAN_POINT('Ctrl Pts',(-24.2570993577032,-7.50747703535114,
0.));
#233940=CARTESIAN_POINT('Ctrl Pts',(-24.2835078958966,-7.50271363765098,
0.));
#233941=CARTESIAN_POINT('Ctrl Pts',(-24.3099781253345,-7.49787641695358,
0.));
#233942=CARTESIAN_POINT('Ctrl Pts',(-24.3365095573673,-7.49296521252329,
0.));
#233943=CARTESIAN_POINT('Ctrl Pts',(-24.3631017084513,-7.48797986651827,
0.));
#233944=CARTESIAN_POINT('Ctrl Pts',(-24.3897541049248,-7.48292022569253,
0.));
#233945=CARTESIAN_POINT('Ctrl Pts',(-24.4164662871165,-7.47778614286573,
0.));
#233946=CARTESIAN_POINT('Ctrl Pts',(-24.4432378146501,-7.47257747883318,
0.));
#233947=CARTESIAN_POINT('Ctrl Pts',(-24.4700682684544,-7.46729410308922,
0.));
#233948=CARTESIAN_POINT('Ctrl Pts',(-24.4969572391509,-7.46193588961641,
0.));
#233949=CARTESIAN_POINT('Ctrl Pts',(-24.52390431731,-7.45650271336045,0.));
#233950=CARTESIAN_POINT('Ctrl Pts',(-24.5509090831579,-7.45099444651295,
0.));
#233951=CARTESIAN_POINT('Ctrl Pts',(-24.5779710960865,-7.44541095473162,
0.));
#233952=CARTESIAN_POINT('Ctrl Pts',(-24.6050898852349,-7.43975209375374,
0.));
#233953=CARTESIAN_POINT('Ctrl Pts',(-24.6322649369472,-7.4340177048922,
0.));
#233954=CARTESIAN_POINT('Ctrl Pts',(-24.659495712869,-7.4282076215868,0.));
#233955=CARTESIAN_POINT('Ctrl Pts',(-24.6867816727118,-7.42232167765762,
0.));
#233956=CARTESIAN_POINT('Ctrl Pts',(-24.7141222949988,-7.41635971481243,
0.));
#233957=CARTESIAN_POINT('Ctrl Pts',(-24.7415170994754,-7.41032159082173,
0.));
#233958=CARTESIAN_POINT('Ctrl Pts',(-24.7689656669005,-7.40420718661754,
0.));
#233959=CARTESIAN_POINT('Ctrl Pts',(-24.7964676646518,-7.39801641583612,
0.));
#233960=CARTESIAN_POINT('Ctrl Pts',(-24.8240228521042,-7.39174922586841,
0.));
#233961=CARTESIAN_POINT('Ctrl Pts',(-24.8516310625367,-7.38540558904945,
0.));
#233962=CARTESIAN_POINT('Ctrl Pts',(-24.8792921911309,-7.3789854964161,
0.));
#233963=CARTESIAN_POINT('Ctrl Pts',(-24.9014633826201,-7.37378825962717,
0.));
#233964=CARTESIAN_POINT('Ctrl Pts',(-24.9181155530631,-7.36985593120696,
0.));
#233965=CARTESIAN_POINT('Ctrl Pts',(-24.9292275670705,-7.36721909029059,
0.));
#233966=CARTESIAN_POINT('Ctrl Pts',(-24.9347862158358,-7.36589684767343,
0.));
#233967=CARTESIAN_POINT('',(-24.9347862158358,-7.36589684767343,12.));
#233968=CARTESIAN_POINT('Ctrl Pts',(-24.9347862158358,-7.36589684767343,
12.));
#233969=CARTESIAN_POINT('Ctrl Pts',(-24.9292275670705,-7.36721909029059,
12.));
#233970=CARTESIAN_POINT('Ctrl Pts',(-24.9181155530631,-7.36985593120696,
12.));
#233971=CARTESIAN_POINT('Ctrl Pts',(-24.9014633826201,-7.37378825962717,
12.));
#233972=CARTESIAN_POINT('Ctrl Pts',(-24.8792921911309,-7.3789854964161,
12.));
#233973=CARTESIAN_POINT('Ctrl Pts',(-24.8516310625367,-7.38540558904945,
12.));
#233974=CARTESIAN_POINT('Ctrl Pts',(-24.8240228521042,-7.39174922586841,
12.));
#233975=CARTESIAN_POINT('Ctrl Pts',(-24.7964676646518,-7.39801641583612,
12.));
#233976=CARTESIAN_POINT('Ctrl Pts',(-24.7689656669005,-7.40420718661754,
12.));
#233977=CARTESIAN_POINT('Ctrl Pts',(-24.7415170994754,-7.41032159082173,
12.));
#233978=CARTESIAN_POINT('Ctrl Pts',(-24.7141222949988,-7.41635971481243,
12.));
#233979=CARTESIAN_POINT('Ctrl Pts',(-24.6867816727118,-7.42232167765762,
12.));
#233980=CARTESIAN_POINT('Ctrl Pts',(-24.659495712869,-7.4282076215868,12.));
#233981=CARTESIAN_POINT('Ctrl Pts',(-24.6322649369472,-7.4340177048922,
12.));
#233982=CARTESIAN_POINT('Ctrl Pts',(-24.6050898852349,-7.43975209375374,
12.));
#233983=CARTESIAN_POINT('Ctrl Pts',(-24.5779710960865,-7.44541095473162,
12.));
#233984=CARTESIAN_POINT('Ctrl Pts',(-24.5509090831579,-7.45099444651295,
12.));
#233985=CARTESIAN_POINT('Ctrl Pts',(-24.52390431731,-7.45650271336045,12.));
#233986=CARTESIAN_POINT('Ctrl Pts',(-24.4969572391509,-7.46193588961641,
12.));
#233987=CARTESIAN_POINT('Ctrl Pts',(-24.4700682684544,-7.46729410308922,
12.));
#233988=CARTESIAN_POINT('Ctrl Pts',(-24.4432378146501,-7.47257747883318,
12.));
#233989=CARTESIAN_POINT('Ctrl Pts',(-24.4164662871165,-7.47778614286573,
12.));
#233990=CARTESIAN_POINT('Ctrl Pts',(-24.3897541049248,-7.48292022569253,
12.));
#233991=CARTESIAN_POINT('Ctrl Pts',(-24.3631017084513,-7.48797986651827,
12.));
#233992=CARTESIAN_POINT('Ctrl Pts',(-24.3365095573673,-7.49296521252329,
12.));
#233993=CARTESIAN_POINT('Ctrl Pts',(-24.3099781253345,-7.49787641695358,
12.));
#233994=CARTESIAN_POINT('Ctrl Pts',(-24.2835078958966,-7.50271363765098,
12.));
#233995=CARTESIAN_POINT('Ctrl Pts',(-24.2570993577032,-7.50747703535114,
12.));
#233996=CARTESIAN_POINT('Ctrl Pts',(-24.230753000389,-7.51216677222198,
12.));
#233997=CARTESIAN_POINT('Ctrl Pts',(-24.2044693092356,-7.51678300997997,
12.));
#233998=CARTESIAN_POINT('Ctrl Pts',(-24.1782487641602,-7.52132590953862,
12.));
#233999=CARTESIAN_POINT('Ctrl Pts',(-24.152091842537,-7.52579563201478,
12.));
#234000=CARTESIAN_POINT('Ctrl Pts',(-24.1259990209211,-7.53019233935536,
12.));
#234001=CARTESIAN_POINT('Ctrl Pts',(-24.0999707772643,-7.53451619514658,
12.));
#234002=CARTESIAN_POINT('Ctrl Pts',(-24.0740075927984,-7.53876736531004,
12.));
#234003=CARTESIAN_POINT('Ctrl Pts',(-24.0481099543353,-7.54294601896127,
12.));
#234004=CARTESIAN_POINT('Ctrl Pts',(-24.0222783554531,-7.54705232885894,
12.));
#234005=CARTESIAN_POINT('Ctrl Pts',(-23.9965132953187,-7.55108647097431,
12.));
#234006=CARTESIAN_POINT('Ctrl Pts',(-23.9708152779886,-7.55504862424807,
12.));
#234007=CARTESIAN_POINT('Ctrl Pts',(-23.9451848115002,-7.55893897027679,
12.));
#234008=CARTESIAN_POINT('Ctrl Pts',(-23.9196224070759,-7.56275769304772,
12.));
#234009=CARTESIAN_POINT('Ctrl Pts',(-23.8941285782002,-7.5665049786379,
12.));
#234010=CARTESIAN_POINT('Ctrl Pts',(-23.8687038399595,-7.57018101500709,
12.));
#234011=CARTESIAN_POINT('Ctrl Pts',(-23.8433487096132,-7.57378599219814,
12.));
#234012=CARTESIAN_POINT('Ctrl Pts',(-23.8180637069976,-7.57732010249065,
12.));
#234013=CARTESIAN_POINT('Ctrl Pts',(-23.7928493549908,-7.58078354058212,
12.));
#234014=CARTESIAN_POINT('Ctrl Pts',(-23.7677061799376,-7.5841765037627,
12.));
#234015=CARTESIAN_POINT('Ctrl Pts',(-23.7426347121006,-7.58749919210825,
12.));
#234016=CARTESIAN_POINT('Ctrl Pts',(-23.7176354860457,-7.5907518086532,
12.));
#234017=CARTESIAN_POINT('Ctrl Pts',(-23.6927090405066,-7.59393455934034,
12.));
#234018=CARTESIAN_POINT('Ctrl Pts',(-23.6678559182875,-7.59704765299566,
12.));
#234019=CARTESIAN_POINT('Ctrl Pts',(-23.6430766661418,-7.60009130130125,
12.));
#234020=CARTESIAN_POINT('Ctrl Pts',(-23.6183718346576,-7.60306571877805,
12.));
#234021=CARTESIAN_POINT('Ctrl Pts',(-23.5937419781245,-7.60597112277093,
12.));
#234022=CARTESIAN_POINT('Ctrl Pts',(-23.5691876544244,-7.60880773344599,
12.));
#234023=CARTESIAN_POINT('Ctrl Pts',(-23.544709425203,-7.61157577385371,
12.));
#234024=CARTESIAN_POINT('Ctrl Pts',(-23.5203078560129,-7.61427546999297,
12.));
#234025=CARTESIAN_POINT('Ctrl Pts',(-23.4959835164609,-7.61690705088318,
12.));
#234026=CARTESIAN_POINT('Ctrl Pts',(-23.4717369803438,-7.61947074863976,
12.));
#234027=CARTESIAN_POINT('Ctrl Pts',(-23.4475688257854,-7.62196679855954,
12.));
#234028=CARTESIAN_POINT('Ctrl Pts',(-23.4234796353542,-7.62439543920049,
12.));
#234029=CARTESIAN_POINT('Ctrl Pts',(-23.399469996112,-7.62675691240328,
12.));
#234030=CARTESIAN_POINT('Ctrl Pts',(-23.3755404996636,-7.62905146332592,
12.));
#234031=CARTESIAN_POINT('Ctrl Pts',(-23.3516917421972,-7.63127934048136,
12.));
#234032=CARTESIAN_POINT('Ctrl Pts',(-23.3279243245241,-7.63344079578161,
12.));
#234033=CARTESIAN_POINT('Ctrl Pts',(-23.3042388521022,-7.63553608458782,
12.));
#234034=CARTESIAN_POINT('Ctrl Pts',(-23.2806359350855,-7.63756546576374,
12.));
#234035=CARTESIAN_POINT('Ctrl Pts',(-23.2571161884488,-7.63952920172835,
12.));
#234036=CARTESIAN_POINT('Ctrl Pts',(-23.2336802320912,-7.64142755851504,
12.));
#234037=CARTESIAN_POINT('Ctrl Pts',(-23.2103286909398,-7.64326080583679,
12.));
#234038=CARTESIAN_POINT('Ctrl Pts',(-23.1870621950452,-7.64502921715482,
12.));
#234039=CARTESIAN_POINT('Ctrl Pts',(-23.1638813796694,-7.64673306975804,
12.));
#234040=CARTESIAN_POINT('Ctrl Pts',(-23.1407868853819,-7.64837264482942,
12.));
#234041=CARTESIAN_POINT('Ctrl Pts',(-23.1177793581679,-7.64994822749859,
12.));
#234042=CARTESIAN_POINT('Ctrl Pts',(-23.094859449525,-7.65146010690475,
12.));
#234043=CARTESIAN_POINT('Ctrl Pts',(-23.072027816555,-7.65290857626357,
12.));
#234044=CARTESIAN_POINT('Ctrl Pts',(-23.0492851220528,-7.65429393293945,
12.));
#234045=CARTESIAN_POINT('Ctrl Pts',(-23.0266320345787,-7.65561647852533,
12.));
#234046=CARTESIAN_POINT('Ctrl Pts',(-23.0040692285814,-7.65687651891304,
12.));
#234047=CARTESIAN_POINT('Ctrl Pts',(-22.9815973845296,-7.65807436436431,
12.));
#234048=CARTESIAN_POINT('Ctrl Pts',(-22.959217189033,-7.65921032958901,
12.));
#234049=CARTESIAN_POINT('Ctrl Pts',(-22.9369293349593,-7.66028473382777,
12.));
#234050=CARTESIAN_POINT('Ctrl Pts',(-22.9147345215421,-7.66129790094107,
12.));
#234051=CARTESIAN_POINT('Ctrl Pts',(-22.8926334544883,-7.66225015950155,
12.));
#234052=CARTESIAN_POINT('Ctrl Pts',(-22.8706268461283,-7.66314184287336,
12.));
#234053=CARTESIAN_POINT('Ctrl Pts',(-22.848715415557,-7.66397328929802,
12.));
#234054=CARTESIAN_POINT('Ctrl Pts',(-22.8268998887678,-7.66474484198548,
12.));
#234055=CARTESIAN_POINT('Ctrl Pts',(-22.8051809987833,-7.66545684920987,
12.));
#234056=CARTESIAN_POINT('Ctrl Pts',(-22.7835594857699,-7.66610966441272,
12.));
#234057=CARTESIAN_POINT('Ctrl Pts',(-22.7620360971843,-7.66670364630298,
12.));
#234058=CARTESIAN_POINT('Ctrl Pts',(-22.7406115879513,-7.66723915895439,
12.));
#234059=CARTESIAN_POINT('Ctrl Pts',(-22.7192867206245,-7.66771657191027,
12.));
#234060=CARTESIAN_POINT('Ctrl Pts',(-22.6980622655446,-7.66813626029274,
12.));
#234061=CARTESIAN_POINT('Ctrl Pts',(-22.6769390009885,-7.66849860491742,
12.));
#234062=CARTESIAN_POINT('Ctrl Pts',(-22.6559177133127,-7.66880399241322,
12.));
#234063=CARTESIAN_POINT('Ctrl Pts',(-22.6349991971541,-7.66905281533714,
12.));
#234064=CARTESIAN_POINT('Ctrl Pts',(-22.6141842556243,-7.66924547229413,
12.));
#234065=CARTESIAN_POINT('Ctrl Pts',(-22.5934737004953,-7.66938236806232,
12.));
#234066=CARTESIAN_POINT('Ctrl Pts',(-22.5728683523831,-7.66946391372305,
12.));
#234067=CARTESIAN_POINT('Ctrl Pts',(-22.5523690409116,-7.66949052679692,
12.));
#234068=CARTESIAN_POINT('Ctrl Pts',(-22.53197660492,-7.66946263138143,12.));
#234069=CARTESIAN_POINT('Ctrl Pts',(-22.5116918927032,-7.66938065829107,
12.));
#234070=CARTESIAN_POINT('Ctrl Pts',(-22.4915157622312,-7.66924504520314,
12.));
#234071=CARTESIAN_POINT('Ctrl Pts',(-22.47144908137,-7.6690562368083,12.));
#234072=CARTESIAN_POINT('Ctrl Pts',(-22.4514927280855,-7.66881468496634,
12.));
#234073=CARTESIAN_POINT('Ctrl Pts',(-22.4316475906603,-7.66852084886704,
12.));
#234074=CARTESIAN_POINT('Ctrl Pts',(-22.4119145679758,-7.66817519519639,
12.));
#234075=CARTESIAN_POINT('Ctrl Pts',(-22.3922945697773,-7.66777819830789,
12.));
#234076=CARTESIAN_POINT('Ctrl Pts',(-22.372788516936,-7.66733034039882,
12.));
#234077=CARTESIAN_POINT('Ctrl Pts',(-22.3533973417021,-7.66683211169158,
12.));
#234078=CARTESIAN_POINT('Ctrl Pts',(-22.3341219879469,-7.66628401061952,
12.));
#234079=CARTESIAN_POINT('Ctrl Pts',(-22.314963411484,-7.66568654402493,
12.));
#234080=CARTESIAN_POINT('Ctrl Pts',(-22.2959225803937,-7.66504022736298,
12.));
#234081=CARTESIAN_POINT('Ctrl Pts',(-22.2770004753335,-7.66434558490978,
12.));
#234082=CARTESIAN_POINT('Ctrl Pts',(-22.258198089848,-7.6636031499764,12.));
#234083=CARTESIAN_POINT('Ctrl Pts',(-22.2395164306547,-7.66281346512508,
12.));
#234084=CARTESIAN_POINT('Ctrl Pts',(-22.2209565180085,-7.66197708240399,
12.));
#234085=CARTESIAN_POINT('Ctrl Pts',(-22.2025193860964,-7.6610945635927,
12.));
#234086=CARTESIAN_POINT('Ctrl Pts',(-22.1842060834091,-7.66016648045004,
12.));
#234087=CARTESIAN_POINT('Ctrl Pts',(-22.1660176731178,-7.6591934149693,
12.));
#234088=CARTESIAN_POINT('Ctrl Pts',(-22.1479552334211,-7.65817595963349,
12.));
#234089=CARTESIAN_POINT('Ctrl Pts',(-22.1300198579675,-7.65711471769396,
12.));
#234090=CARTESIAN_POINT('Ctrl Pts',(-22.1122126563329,-7.65601030346806,
12.));
#234091=CARTESIAN_POINT('Ctrl Pts',(-22.094534754469,-7.65486334263643,
12.));
#234092=CARTESIAN_POINT('Ctrl Pts',(-22.0769872951596,-7.65367447254949,
12.));
#234093=CARTESIAN_POINT('Ctrl Pts',(-22.0595714384431,-7.65244434253112,
12.));
#234094=CARTESIAN_POINT('Ctrl Pts',(-22.0422883621174,-7.65117361421358,
12.));
#234095=CARTESIAN_POINT('Ctrl Pts',(-22.0251392623209,-7.64986296190168,
12.));
#234096=CARTESIAN_POINT('Ctrl Pts',(-22.0081253540774,-7.64851307293351,
12.));
#234097=CARTESIAN_POINT('Ctrl Pts',(-21.9912478718542,-7.64712464805249,
12.));
#234098=CARTESIAN_POINT('Ctrl Pts',(-21.9745080700798,-7.64569840177335,
12.));
#234099=CARTESIAN_POINT('Ctrl Pts',(-21.9579072237651,-7.64423506279122,
12.));
#234100=CARTESIAN_POINT('Ctrl Pts',(-21.9414466292072,-7.64273537442682,
12.));
#234101=CARTESIAN_POINT('Ctrl Pts',(-21.9251276046546,-7.64120009506531,
12.));
#234102=CARTESIAN_POINT('Ctrl Pts',(-21.9089514909874,-7.63962999860927,
12.));
#234103=CARTESIAN_POINT('Ctrl Pts',(-21.8929196523514,-7.63802587492034,
12.));
#234104=CARTESIAN_POINT('Ctrl Pts',(-21.8770334769496,-7.63638853033399,
12.));
#234105=CARTESIAN_POINT('Ctrl Pts',(-21.8612943779089,-7.63471878821225,
12.));
#234106=CARTESIAN_POINT('Ctrl Pts',(-21.8457037941084,-7.63301748948935,
12.));
#234107=CARTESIAN_POINT('Ctrl Pts',(-21.8302631910195,-7.63128549323022,
12.));
#234108=CARTESIAN_POINT('Ctrl Pts',(-21.814974061509,-7.62952367718126,
12.));
#234109=CARTESIAN_POINT('Ctrl Pts',(-21.799837926858,-7.62773293842389,
12.));
#234110=CARTESIAN_POINT('Ctrl Pts',(-21.7848563378021,-7.62591419404512,
12.));
#234111=CARTESIAN_POINT('Ctrl Pts',(-21.7700308755584,-7.62406838181166,
12.));
#234112=CARTESIAN_POINT('Ctrl Pts',(-21.7553631528328,-7.62219646084228,
12.));
#234113=CARTESIAN_POINT('Ctrl Pts',(-21.7408548148656,-7.62029941230854,
12.));
#234114=CARTESIAN_POINT('Ctrl Pts',(-21.7265075407975,-7.61837824030537,
12.));
#234115=CARTESIAN_POINT('Ctrl Pts',(-21.7123230449834,-7.6164339727042,
12.));
#234116=CARTESIAN_POINT('Ctrl Pts',(-21.6983030783322,-7.61446766202786,
12.));
#234117=CARTESIAN_POINT('Ctrl Pts',(-21.6844494295815,-7.61248038630268,
12.));
#234118=CARTESIAN_POINT('Ctrl Pts',(-21.6707639267576,-7.61047325000955,
12.));
#234119=CARTESIAN_POINT('Ctrl Pts',(-21.6572484388081,-7.60844738512873,
12.));
#234120=CARTESIAN_POINT('Ctrl Pts',(-21.6439048771743,-7.60640395216356,
12.));
#234121=CARTESIAN_POINT('Ctrl Pts',(-21.6307351973822,-7.60434414118295,
12.));
#234122=CARTESIAN_POINT('Ctrl Pts',(-21.617741400599,-7.60226917285428,
12.));
#234123=CARTESIAN_POINT('Ctrl Pts',(-21.6049255358843,-7.6001802998824,
12.));
#234124=CARTESIAN_POINT('Ctrl Pts',(-21.5922897024466,-7.59807880846194,
12.));
#234125=CARTESIAN_POINT('Ctrl Pts',(-21.5798360518978,-7.59596601973583,
12.));
#234126=CARTESIAN_POINT('Ctrl Pts',(-21.5675667904726,-7.59384329124918,
12.));
#234127=CARTESIAN_POINT('Ctrl Pts',(-21.5554841813462,-7.59171201844776,
12.));
#234128=CARTESIAN_POINT('Ctrl Pts',(-21.543590547011,-7.58957363620013,
12.));
#234129=CARTESIAN_POINT('Ctrl Pts',(-21.5318882716736,-7.58742962034833,
12.));
#234130=CARTESIAN_POINT('Ctrl Pts',(-21.5203798035299,-7.58528148919129,
12.));
#234131=CARTESIAN_POINT('Ctrl Pts',(-21.5090676573873,-7.58313080519179,
12.));
#234132=CARTESIAN_POINT('Ctrl Pts',(-21.4979544192744,-7.58097917790744,
12.));
#234133=CARTESIAN_POINT('Ctrl Pts',(-21.4870427508194,-7.57882826679131,
12.));
#234134=CARTESIAN_POINT('Ctrl Pts',(-21.4763353936762,-7.57667978402987,
12.));
#234135=CARTESIAN_POINT('Ctrl Pts',(-21.4658351740128,-7.57453549743411,
12.));
#234136=CARTESIAN_POINT('Ctrl Pts',(-21.4555450053142,-7.57239723223505,
12.));
#234137=CARTESIAN_POINT('Ctrl Pts',(-21.4454678907509,-7.57026687261165,
12.));
#234138=CARTESIAN_POINT('Ctrl Pts',(-21.4356069261513,-7.56814636360847,
12.));
#234139=CARTESIAN_POINT('Ctrl Pts',(-21.4259653015736,-7.56603771218712,
12.));
#234140=CARTESIAN_POINT('Ctrl Pts',(-21.4165463106254,-7.56394299313684,
12.));
#234141=CARTESIAN_POINT('Ctrl Pts',(-21.4073533630365,-7.56186435703621,
12.));
#234142=CARTESIAN_POINT('Ctrl Pts',(-21.3983899952987,-7.5598040370061,
12.));
#234143=CARTESIAN_POINT('Ctrl Pts',(-21.3896598842117,-7.55776435731416,
12.));
#234144=CARTESIAN_POINT('Ctrl Pts',(-21.3811668478932,-7.55574773403502,
12.));
#234145=CARTESIAN_POINT('Ctrl Pts',(-21.3729148390243,-7.55375667080028,
12.));
#234146=CARTESIAN_POINT('Ctrl Pts',(-21.3649079431865,-7.55179375777443,
12.));
#234147=CARTESIAN_POINT('Ctrl Pts',(-21.3571503685855,-7.54986166521309,
12.));
#234148=CARTESIAN_POINT('Ctrl Pts',(-21.3496464761531,-7.5479631624633,
12.));
#234149=CARTESIAN_POINT('Ctrl Pts',(-21.3424008295038,-7.54610114948346,
12.));
#234150=CARTESIAN_POINT('Ctrl Pts',(-21.3354182340149,-7.54427868151267,
12.));
#234151=CARTESIAN_POINT('Ctrl Pts',(-21.328703791771,-7.5424990037703,12.));
#234152=CARTESIAN_POINT('Ctrl Pts',(-21.3222628524165,-7.54076552038278,
12.));
#234153=CARTESIAN_POINT('Ctrl Pts',(-21.3161009456256,-7.53908175169898,
12.));
#234154=CARTESIAN_POINT('Ctrl Pts',(-21.310223716773,-7.53745129364616,
12.));
#234155=CARTESIAN_POINT('Ctrl Pts',(-21.3046368712157,-7.53587778251735,
12.));
#234156=CARTESIAN_POINT('Ctrl Pts',(-21.2993464250717,-7.53436505309942,
12.));
#234157=CARTESIAN_POINT('Ctrl Pts',(-21.2943588989331,-7.53291726078526,
12.));
#234158=CARTESIAN_POINT('Ctrl Pts',(-21.2896816163842,-7.53153906987855,
12.));
#234159=CARTESIAN_POINT('Ctrl Pts',(-21.2853226580657,-7.53023562438229,
12.));
#234160=CARTESIAN_POINT('Ctrl Pts',(-21.2812902781143,-7.52901217930407,
12.));
#234161=CARTESIAN_POINT('Ctrl Pts',(-21.2775925269652,-7.52787386225332,
12.));
#234162=CARTESIAN_POINT('Ctrl Pts',(-21.2742366113579,-7.5268252691854,
12.));
#234163=CARTESIAN_POINT('Ctrl Pts',(-21.2712301573466,-7.52587126095529,
12.));
#234164=CARTESIAN_POINT('Ctrl Pts',(-21.2685823838671,-7.5250177033353,
12.));
#234165=CARTESIAN_POINT('Ctrl Pts',(-21.2663059157058,-7.52427261074297,
12.));
#234166=CARTESIAN_POINT('Ctrl Pts',(-21.2644161259962,-7.52364573027552,
12.));
#234167=CARTESIAN_POINT('Ctrl Pts',(-21.262927782038,-7.52314642316199,
12.));
#234168=CARTESIAN_POINT('Ctrl Pts',(-21.2618521283555,-7.52278182242669,
12.));
#234169=CARTESIAN_POINT('Ctrl Pts',(-21.261326054066,-7.5226006423166,12.));
#234170=CARTESIAN_POINT('Ctrl Pts',(-21.2611204474866,-7.52252744144903,
12.));
#234171=CARTESIAN_POINT('Ctrl Pts',(-21.2610673466886,-7.5225064970397,
12.));
#234172=CARTESIAN_POINT('Ctrl Pts',(-21.2610617890679,-7.52250298901264,
12.));
#234173=CARTESIAN_POINT('',(-24.9347862158358,-7.36589684767343,0.));
#234174=CARTESIAN_POINT('Origin',(-21.4341755315424,-1.68110656504246,0.));
#234175=CARTESIAN_POINT('',(-22.4835757167854,-1.76341220531179,12.));
#234176=CARTESIAN_POINT('',(-10.7170877657712,-0.840553282521227,12.));
#234177=CARTESIAN_POINT('',(-22.4835757167854,-1.76341220531179,0.));
#234178=CARTESIAN_POINT('',(-22.4835757167854,-1.76341220531179,0.));
#234179=CARTESIAN_POINT('',(-10.7170877657712,-0.840553282521227,0.));
#234180=CARTESIAN_POINT('Ctrl Pts',(-25.2771067246846,-6.08833931617698,
0.));
#234181=CARTESIAN_POINT('Ctrl Pts',(-25.2771067246846,-6.08833931617698,
12.));
#234182=CARTESIAN_POINT('Ctrl Pts',(-25.2729539149479,-6.08441489609824,
0.));
#234183=CARTESIAN_POINT('Ctrl Pts',(-25.2729539149479,-6.08441489609824,
12.));
#234184=CARTESIAN_POINT('Ctrl Pts',(-25.2646490489816,-6.07657531787577,
0.));
#234185=CARTESIAN_POINT('Ctrl Pts',(-25.2646490489816,-6.07657531787577,
12.));
#234186=CARTESIAN_POINT('Ctrl Pts',(-25.2521940105523,-6.06484373634696,
0.));
#234187=CARTESIAN_POINT('Ctrl Pts',(-25.2521940105523,-6.06484373634696,
12.));
#234188=CARTESIAN_POINT('Ctrl Pts',(-25.2355918138798,-6.04925720151412,
0.));
#234189=CARTESIAN_POINT('Ctrl Pts',(-25.2355918138798,-6.04925720151412,
12.));
#234190=CARTESIAN_POINT('Ctrl Pts',(-25.2148466201368,-6.02986667390187,
0.));
#234191=CARTESIAN_POINT('Ctrl Pts',(-25.2148466201368,-6.02986667390187,
12.));
#234192=CARTESIAN_POINT('Ctrl Pts',(-25.1941090269638,-6.0105688180476,
0.));
#234193=CARTESIAN_POINT('Ctrl Pts',(-25.1941090269638,-6.0105688180476,
12.));
#234194=CARTESIAN_POINT('Ctrl Pts',(-25.1733791296154,-5.99136367859838,
0.));
#234195=CARTESIAN_POINT('Ctrl Pts',(-25.1733791296154,-5.99136367859838,
12.));
#234196=CARTESIAN_POINT('Ctrl Pts',(-25.1526570863065,-5.97225131495636,
0.));
#234197=CARTESIAN_POINT('Ctrl Pts',(-25.1526570863065,-5.97225131495636,
12.));
#234198=CARTESIAN_POINT('Ctrl Pts',(-25.1319431317273,-5.95323180187348,
0.));
#234199=CARTESIAN_POINT('Ctrl Pts',(-25.1319431317273,-5.95323180187348,
12.));
#234200=CARTESIAN_POINT('Ctrl Pts',(-25.1112375971182,-5.93430523086776,
0.));
#234201=CARTESIAN_POINT('Ctrl Pts',(-25.1112375971182,-5.93430523086776,
12.));
#234202=CARTESIAN_POINT('Ctrl Pts',(-25.0905409050863,-5.91547170844382,
0.));
#234203=CARTESIAN_POINT('Ctrl Pts',(-25.0905409050863,-5.91547170844382,
12.));
#234204=CARTESIAN_POINT('Ctrl Pts',(-25.0698535426593,-5.89673135155459,
0.));
#234205=CARTESIAN_POINT('Ctrl Pts',(-25.0698535426593,-5.89673135155459,
12.));
#234206=CARTESIAN_POINT('Ctrl Pts',(-25.0491760405965,-5.87808428385329,
0.));
#234207=CARTESIAN_POINT('Ctrl Pts',(-25.0491760405965,-5.87808428385329,
12.));
#234208=CARTESIAN_POINT('Ctrl Pts',(-25.0285089498922,-5.8595306315681,
0.));
#234209=CARTESIAN_POINT('Ctrl Pts',(-25.0285089498922,-5.8595306315681,
12.));
#234210=CARTESIAN_POINT('Ctrl Pts',(-25.0078528200558,-5.84107051963073,
0.));
#234211=CARTESIAN_POINT('Ctrl Pts',(-25.0078528200558,-5.84107051963073,
12.));
#234212=CARTESIAN_POINT('Ctrl Pts',(-24.9872081752709,-5.82270406744214,
0.));
#234213=CARTESIAN_POINT('Ctrl Pts',(-24.9872081752709,-5.82270406744214,
12.));
#234214=CARTESIAN_POINT('Ctrl Pts',(-24.9665754954462,-5.80443138549747,
0.));
#234215=CARTESIAN_POINT('Ctrl Pts',(-24.9665754954462,-5.80443138549747,
12.));
#234216=CARTESIAN_POINT('Ctrl Pts',(-24.9459552293308,-5.78625257775703,
0.));
#234217=CARTESIAN_POINT('Ctrl Pts',(-24.9459552293308,-5.78625257775703,
12.));
#234218=CARTESIAN_POINT('Ctrl Pts',(-24.9253478043632,-5.76816774342236,
0.));
#234219=CARTESIAN_POINT('Ctrl Pts',(-24.9253478043632,-5.76816774342236,
12.));
#234220=CARTESIAN_POINT('Ctrl Pts',(-24.9047536376467,-5.75017697890813,
0.));
#234221=CARTESIAN_POINT('Ctrl Pts',(-24.9047536376467,-5.75017697890813,
12.));
#234222=CARTESIAN_POINT('Ctrl Pts',(-24.8841731467219,-5.73228037976926,
0.));
#234223=CARTESIAN_POINT('Ctrl Pts',(-24.8841731467219,-5.73228037976926,
12.));
#234224=CARTESIAN_POINT('Ctrl Pts',(-24.8636067597677,-5.71447804252019,
0.));
#234225=CARTESIAN_POINT('Ctrl Pts',(-24.8636067597677,-5.71447804252019,
12.));
#234226=CARTESIAN_POINT('Ctrl Pts',(-24.8430549277634,-5.69677006679429,
0.));
#234227=CARTESIAN_POINT('Ctrl Pts',(-24.8430549277634,-5.69677006679429,
12.));
#234228=CARTESIAN_POINT('Ctrl Pts',(-24.822518122386,-5.67915655496524,
0.));
#234229=CARTESIAN_POINT('Ctrl Pts',(-24.822518122386,-5.67915655496524,
12.));
#234230=CARTESIAN_POINT('Ctrl Pts',(-24.8019968304618,-5.66163761114903,
0.));
#234231=CARTESIAN_POINT('Ctrl Pts',(-24.8019968304618,-5.66163761114903,
12.));
#234232=CARTESIAN_POINT('Ctrl Pts',(-24.7814915496728,-5.64421334042247,
0.));
#234233=CARTESIAN_POINT('Ctrl Pts',(-24.7814915496728,-5.64421334042247,
12.));
#234234=CARTESIAN_POINT('Ctrl Pts',(-24.76100278357,-5.62688384790919,0.));
#234235=CARTESIAN_POINT('Ctrl Pts',(-24.76100278357,-5.62688384790919,12.));
#234236=CARTESIAN_POINT('Ctrl Pts',(-24.7405310372736,-5.60964923798495,
0.));
#234237=CARTESIAN_POINT('Ctrl Pts',(-24.7405310372736,-5.60964923798495,
12.));
#234238=CARTESIAN_POINT('Ctrl Pts',(-24.7200768119079,-5.59250961323995,
0.));
#234239=CARTESIAN_POINT('Ctrl Pts',(-24.7200768119079,-5.59250961323995,
12.));
#234240=CARTESIAN_POINT('Ctrl Pts',(-24.6996406035507,-5.57546507427766,
0.));
#234241=CARTESIAN_POINT('Ctrl Pts',(-24.6996406035507,-5.57546507427766,
12.));
#234242=CARTESIAN_POINT('Ctrl Pts',(-24.6792229061785,-5.55851572025389,
0.));
#234243=CARTESIAN_POINT('Ctrl Pts',(-24.6792229061785,-5.55851572025389,
12.));
#234244=CARTESIAN_POINT('Ctrl Pts',(-24.6588242134733,-5.54166164919593,
0.));
#234245=CARTESIAN_POINT('Ctrl Pts',(-24.6588242134733,-5.54166164919593,
12.));
#234246=CARTESIAN_POINT('Ctrl Pts',(-24.6384450211466,-5.52490295840996,
0.));
#234247=CARTESIAN_POINT('Ctrl Pts',(-24.6384450211466,-5.52490295840996,
12.));
#234248=CARTESIAN_POINT('Ctrl Pts',(-24.618085828918,-5.50823974481959,
0.));
#234249=CARTESIAN_POINT('Ctrl Pts',(-24.618085828918,-5.50823974481959,
12.));
#234250=CARTESIAN_POINT('Ctrl Pts',(-24.5977471429365,-5.49167210537235,
0.));
#234251=CARTESIAN_POINT('Ctrl Pts',(-24.5977471429365,-5.49167210537235,
12.));
#234252=CARTESIAN_POINT('Ctrl Pts',(-24.5774294770329,-5.47520013724403,
0.));
#234253=CARTESIAN_POINT('Ctrl Pts',(-24.5774294770329,-5.47520013724403,
12.));
#234254=CARTESIAN_POINT('Ctrl Pts',(-24.5571333514841,-5.45882393762244,
0.));
#234255=CARTESIAN_POINT('Ctrl Pts',(-24.5571333514841,-5.45882393762244,
12.));
#234256=CARTESIAN_POINT('Ctrl Pts',(-24.5368592922861,-5.44254360356865,
0.));
#234257=CARTESIAN_POINT('Ctrl Pts',(-24.5368592922861,-5.44254360356865,
12.));
#234258=CARTESIAN_POINT('Ctrl Pts',(-24.5166078302107,-5.42635923183411,
0.));
#234259=CARTESIAN_POINT('Ctrl Pts',(-24.5166078302107,-5.42635923183411,
12.));
#234260=CARTESIAN_POINT('Ctrl Pts',(-24.4963794999831,-5.41027091869242,
0.));
#234261=CARTESIAN_POINT('Ctrl Pts',(-24.4963794999831,-5.41027091869242,
12.));
#234262=CARTESIAN_POINT('Ctrl Pts',(-24.4761748393322,-5.3942787597383,
0.));
#234263=CARTESIAN_POINT('Ctrl Pts',(-24.4761748393322,-5.3942787597383,
12.));
#234264=CARTESIAN_POINT('Ctrl Pts',(-24.4559943883159,-5.37838284973706,
0.));
#234265=CARTESIAN_POINT('Ctrl Pts',(-24.4559943883159,-5.37838284973706,
12.));
#234266=CARTESIAN_POINT('Ctrl Pts',(-24.4358386899152,-5.36258328273639,
0.));
#234267=CARTESIAN_POINT('Ctrl Pts',(-24.4358386899152,-5.36258328273639,
12.));
#234268=CARTESIAN_POINT('Ctrl Pts',(-24.4157082904615,-5.34688015213546,
0.));
#234269=CARTESIAN_POINT('Ctrl Pts',(-24.4157082904615,-5.34688015213546,
12.));
#234270=CARTESIAN_POINT('Ctrl Pts',(-24.3956037401293,-5.33127355076036,
0.));
#234271=CARTESIAN_POINT('Ctrl Pts',(-24.3956037401293,-5.33127355076036,
12.));
#234272=CARTESIAN_POINT('Ctrl Pts',(-24.3755255933917,-5.31576357092524,
0.));
#234273=CARTESIAN_POINT('Ctrl Pts',(-24.3755255933917,-5.31576357092524,
12.));
#234274=CARTESIAN_POINT('Ctrl Pts',(-24.3554744095075,-5.30035030449058,
0.));
#234275=CARTESIAN_POINT('Ctrl Pts',(-24.3554744095075,-5.30035030449058,
12.));
#234276=CARTESIAN_POINT('Ctrl Pts',(-24.3354507529415,-5.28503384290644,
0.));
#234277=CARTESIAN_POINT('Ctrl Pts',(-24.3354507529415,-5.28503384290644,
12.));
#234278=CARTESIAN_POINT('Ctrl Pts',(-24.3154551932222,-5.26981427718796,
0.));
#234279=CARTESIAN_POINT('Ctrl Pts',(-24.3154551932222,-5.26981427718796,
12.));
#234280=CARTESIAN_POINT('Ctrl Pts',(-24.2954883048448,-5.25469169788856,
0.));
#234281=CARTESIAN_POINT('Ctrl Pts',(-24.2954883048448,-5.25469169788856,
12.));
#234282=CARTESIAN_POINT('Ctrl Pts',(-24.2755506671526,-5.23966619506289,
0.));
#234283=CARTESIAN_POINT('Ctrl Pts',(-24.2755506671526,-5.23966619506289,
12.));
#234284=CARTESIAN_POINT('Ctrl Pts',(-24.2556428642294,-5.22473785822441,
0.));
#234285=CARTESIAN_POINT('Ctrl Pts',(-24.2556428642294,-5.22473785822441,
12.));
#234286=CARTESIAN_POINT('Ctrl Pts',(-24.2357654847765,-5.20990677629173,
0.));
#234287=CARTESIAN_POINT('Ctrl Pts',(-24.2357654847765,-5.20990677629173,
12.));
#234288=CARTESIAN_POINT('Ctrl Pts',(-24.215919122017,-5.19517303753643,
0.));
#234289=CARTESIAN_POINT('Ctrl Pts',(-24.215919122017,-5.19517303753643,
12.));
#234290=CARTESIAN_POINT('Ctrl Pts',(-24.1961043738754,-5.18053672961392,
0.));
#234291=CARTESIAN_POINT('Ctrl Pts',(-24.1961043738754,-5.18053672961392,
12.));
#234292=CARTESIAN_POINT('Ctrl Pts',(-24.1763218431343,-5.16599793957979,
0.));
#234293=CARTESIAN_POINT('Ctrl Pts',(-24.1763218431343,-5.16599793957979,
12.));
#234294=CARTESIAN_POINT('Ctrl Pts',(-24.156572137597,-5.15155675390075,
0.));
#234295=CARTESIAN_POINT('Ctrl Pts',(-24.156572137597,-5.15155675390075,
12.));
#234296=CARTESIAN_POINT('Ctrl Pts',(-24.1368558702443,-5.13721325845744,
0.));
#234297=CARTESIAN_POINT('Ctrl Pts',(-24.1368558702443,-5.13721325845744,
12.));
#234298=CARTESIAN_POINT('Ctrl Pts',(-24.117173659394,-5.12296753853859,
0.));
#234299=CARTESIAN_POINT('Ctrl Pts',(-24.117173659394,-5.12296753853859,
12.));
#234300=CARTESIAN_POINT('Ctrl Pts',(-24.0975261288446,-5.10881967883132,
0.));
#234301=CARTESIAN_POINT('Ctrl Pts',(-24.0975261288446,-5.10881967883132,
12.));
#234302=CARTESIAN_POINT('Ctrl Pts',(-24.0779139079266,-5.09476976342625,
0.));
#234303=CARTESIAN_POINT('Ctrl Pts',(-24.0779139079266,-5.09476976342625,
12.));
#234304=CARTESIAN_POINT('Ctrl Pts',(-24.0583376315638,-5.08081787581276,
0.));
#234305=CARTESIAN_POINT('Ctrl Pts',(-24.0583376315638,-5.08081787581276,
12.));
#234306=CARTESIAN_POINT('Ctrl Pts',(-24.0387979403268,-5.06696409886641,
0.));
#234307=CARTESIAN_POINT('Ctrl Pts',(-24.0387979403268,-5.06696409886641,
12.));
#234308=CARTESIAN_POINT('Ctrl Pts',(-24.0192954804896,-5.05320851483065,
0.));
#234309=CARTESIAN_POINT('Ctrl Pts',(-24.0192954804896,-5.05320851483065,
12.));
#234310=CARTESIAN_POINT('Ctrl Pts',(-23.9998309040746,-5.03955120528521,
0.));
#234311=CARTESIAN_POINT('Ctrl Pts',(-23.9998309040746,-5.03955120528521,
12.));
#234312=CARTESIAN_POINT('Ctrl Pts',(-23.9804048689227,-5.02599225112454,
0.));
#234313=CARTESIAN_POINT('Ctrl Pts',(-23.9804048689227,-5.02599225112454,
12.));
#234314=CARTESIAN_POINT('Ctrl Pts',(-23.9610180388271,-5.01253173257453,
0.));
#234315=CARTESIAN_POINT('Ctrl Pts',(-23.9610180388271,-5.01253173257453,
12.));
#234316=CARTESIAN_POINT('Ctrl Pts',(-23.9416710836529,-4.99916972919306,
0.));
#234317=CARTESIAN_POINT('Ctrl Pts',(-23.9416710836529,-4.99916972919306,
12.));
#234318=CARTESIAN_POINT('Ctrl Pts',(-23.9223646794592,-4.98590631986532,
0.));
#234319=CARTESIAN_POINT('Ctrl Pts',(-23.9223646794592,-4.98590631986532,
12.));
#234320=CARTESIAN_POINT('Ctrl Pts',(-23.9030995086163,-4.97274158279226,
0.));
#234321=CARTESIAN_POINT('Ctrl Pts',(-23.9030995086163,-4.97274158279226,
12.));
#234322=CARTESIAN_POINT('Ctrl Pts',(-23.8838762599218,-4.9596755954656,
0.));
#234323=CARTESIAN_POINT('Ctrl Pts',(-23.8838762599218,-4.9596755954656,
12.));
#234324=CARTESIAN_POINT('Ctrl Pts',(-23.8646956287168,-4.9467084346586,
0.));
#234325=CARTESIAN_POINT('Ctrl Pts',(-23.8646956287168,-4.9467084346586,
12.));
#234326=CARTESIAN_POINT('Ctrl Pts',(-23.8455583170057,-4.93384017643432,
0.));
#234327=CARTESIAN_POINT('Ctrl Pts',(-23.8455583170057,-4.93384017643432,
12.));
#234328=CARTESIAN_POINT('Ctrl Pts',(-23.8264650335717,-4.92107089613969,
0.));
#234329=CARTESIAN_POINT('Ctrl Pts',(-23.8264650335717,-4.92107089613969,
12.));
#234330=CARTESIAN_POINT('Ctrl Pts',(-23.8074164940896,-4.90840066839344,
0.));
#234331=CARTESIAN_POINT('Ctrl Pts',(-23.8074164940896,-4.90840066839344,
12.));
#234332=CARTESIAN_POINT('Ctrl Pts',(-23.7884134212384,-4.89582956706775,
0.));
#234333=CARTESIAN_POINT('Ctrl Pts',(-23.7884134212384,-4.89582956706775,
12.));
#234334=CARTESIAN_POINT('Ctrl Pts',(-23.7694565448049,-4.88335766525573,
0.));
#234335=CARTESIAN_POINT('Ctrl Pts',(-23.7694565448049,-4.88335766525573,
12.));
#234336=CARTESIAN_POINT('Ctrl Pts',(-23.7505466018245,-4.87098503527152,
0.));
#234337=CARTESIAN_POINT('Ctrl Pts',(-23.7505466018245,-4.87098503527152,
12.));
#234338=CARTESIAN_POINT('Ctrl Pts',(-23.7316843367313,-4.85871174865499,
0.));
#234339=CARTESIAN_POINT('Ctrl Pts',(-23.7316843367313,-4.85871174865499,
12.));
#234340=CARTESIAN_POINT('Ctrl Pts',(-23.7128705015017,-4.84653787616425,
0.));
#234341=CARTESIAN_POINT('Ctrl Pts',(-23.7128705015017,-4.84653787616425,
12.));
#234342=CARTESIAN_POINT('Ctrl Pts',(-23.6941058557971,-4.83446348776265,
0.));
#234343=CARTESIAN_POINT('Ctrl Pts',(-23.6941058557971,-4.83446348776265,
12.));
#234344=CARTESIAN_POINT('Ctrl Pts',(-23.675391167102,-4.82248865259562,
0.));
#234345=CARTESIAN_POINT('Ctrl Pts',(-23.675391167102,-4.82248865259562,
12.));
#234346=CARTESIAN_POINT('Ctrl Pts',(-23.6567272108628,-4.81061343896432,
0.));
#234347=CARTESIAN_POINT('Ctrl Pts',(-23.6567272108628,-4.81061343896432,
12.));
#234348=CARTESIAN_POINT('Ctrl Pts',(-23.6381147706579,-4.7988379143322,
0.));
#234349=CARTESIAN_POINT('Ctrl Pts',(-23.6381147706579,-4.7988379143322,
12.));
#234350=CARTESIAN_POINT('Ctrl Pts',(-23.6195546383624,-4.78716214532098,
0.));
#234351=CARTESIAN_POINT('Ctrl Pts',(-23.6195546383624,-4.78716214532098,
12.));
#234352=CARTESIAN_POINT('Ctrl Pts',(-23.6010476143099,-4.77558619769872,
0.));
#234353=CARTESIAN_POINT('Ctrl Pts',(-23.6010476143099,-4.77558619769872,
12.));
#234354=CARTESIAN_POINT('Ctrl Pts',(-23.5825945074535,-4.76411013636251,
0.));
#234355=CARTESIAN_POINT('Ctrl Pts',(-23.5825945074535,-4.76411013636251,
12.));
#234356=CARTESIAN_POINT('Ctrl Pts',(-23.5641961355168,-4.75273402530617,
0.));
#234357=CARTESIAN_POINT('Ctrl Pts',(-23.5641961355168,-4.75273402530617,
12.));
#234358=CARTESIAN_POINT('Ctrl Pts',(-23.545853325171,-4.74145792760698,
0.));
#234359=CARTESIAN_POINT('Ctrl Pts',(-23.545853325171,-4.74145792760698,
12.));
#234360=CARTESIAN_POINT('Ctrl Pts',(-23.5275669122372,-4.7302819054303,
0.));
#234361=CARTESIAN_POINT('Ctrl Pts',(-23.5275669122372,-4.7302819054303,
12.));
#234362=CARTESIAN_POINT('Ctrl Pts',(-23.509337741878,-4.71920602001901,
0.));
#234363=CARTESIAN_POINT('Ctrl Pts',(-23.509337741878,-4.71920602001901,
12.));
#234364=CARTESIAN_POINT('Ctrl Pts',(-23.491166668789,-4.70823033167818,
0.));
#234365=CARTESIAN_POINT('Ctrl Pts',(-23.491166668789,-4.70823033167818,
12.));
#234366=CARTESIAN_POINT('Ctrl Pts',(-23.4730545573853,-4.69735489975024,
0.));
#234367=CARTESIAN_POINT('Ctrl Pts',(-23.4730545573853,-4.69735489975024,
12.));
#234368=CARTESIAN_POINT('Ctrl Pts',(-23.455002281986,-4.68657978258303,
0.));
#234369=CARTESIAN_POINT('Ctrl Pts',(-23.455002281986,-4.68657978258303,
12.));
#234370=CARTESIAN_POINT('Ctrl Pts',(-23.4370107270451,-4.67590503753058,
0.));
#234371=CARTESIAN_POINT('Ctrl Pts',(-23.4370107270451,-4.67590503753058,
12.));
#234372=CARTESIAN_POINT('Ctrl Pts',(-23.4190807873803,-4.6653307209467,
0.));
#234373=CARTESIAN_POINT('Ctrl Pts',(-23.4190807873803,-4.6653307209467,
12.));
#234374=CARTESIAN_POINT('Ctrl Pts',(-23.4012133683959,-4.65485688816924,
0.));
#234375=CARTESIAN_POINT('Ctrl Pts',(-23.4012133683959,-4.65485688816924,
12.));
#234376=CARTESIAN_POINT('Ctrl Pts',(-23.3834093863068,-4.6444835934993,
0.));
#234377=CARTESIAN_POINT('Ctrl Pts',(-23.3834093863068,-4.6444835934993,
12.));
#234378=CARTESIAN_POINT('Ctrl Pts',(-23.3656697683489,-4.63421089016541,
0.));
#234379=CARTESIAN_POINT('Ctrl Pts',(-23.3656697683489,-4.63421089016541,
12.));
#234380=CARTESIAN_POINT('Ctrl Pts',(-23.3479954530272,-4.62403883030805,
0.));
#234381=CARTESIAN_POINT('Ctrl Pts',(-23.3479954530272,-4.62403883030805,
12.));
#234382=CARTESIAN_POINT('Ctrl Pts',(-23.3303873903938,-4.6139674649783,
0.));
#234383=CARTESIAN_POINT('Ctrl Pts',(-23.3303873903938,-4.6139674649783,
12.));
#234384=CARTESIAN_POINT('Ctrl Pts',(-23.3128465423115,-4.60399684412163,
0.));
#234385=CARTESIAN_POINT('Ctrl Pts',(-23.3128465423115,-4.60399684412163,
12.));
#234386=CARTESIAN_POINT('Ctrl Pts',(-23.2953738827191,-4.5941270165575,
0.));
#234387=CARTESIAN_POINT('Ctrl Pts',(-23.2953738827191,-4.5941270165575,
12.));
#234388=CARTESIAN_POINT('Ctrl Pts',(-23.2779703978876,-4.5843580299469,
0.));
#234389=CARTESIAN_POINT('Ctrl Pts',(-23.2779703978876,-4.5843580299469,
12.));
#234390=CARTESIAN_POINT('Ctrl Pts',(-23.2606370866866,-4.57468993076097,
0.));
#234391=CARTESIAN_POINT('Ctrl Pts',(-23.2606370866866,-4.57468993076097,
12.));
#234392=CARTESIAN_POINT('Ctrl Pts',(-23.2433749609131,-4.56512276427839,
0.));
#234393=CARTESIAN_POINT('Ctrl Pts',(-23.2433749609131,-4.56512276427839,
12.));
#234394=CARTESIAN_POINT('Ctrl Pts',(-23.2261850456064,-4.55565657456975,
0.));
#234395=CARTESIAN_POINT('Ctrl Pts',(-23.2261850456064,-4.55565657456975,
12.));
#234396=CARTESIAN_POINT('Ctrl Pts',(-23.2090683793629,-4.54629140447544,
0.));
#234397=CARTESIAN_POINT('Ctrl Pts',(-23.2090683793629,-4.54629140447544,
12.));
#234398=CARTESIAN_POINT('Ctrl Pts',(-23.1920260146465,-4.53702729557566,
0.));
#234399=CARTESIAN_POINT('Ctrl Pts',(-23.1920260146465,-4.53702729557566,
12.));
#234400=CARTESIAN_POINT('Ctrl Pts',(-23.1750590180908,-4.52786428815014,
0.));
#234401=CARTESIAN_POINT('Ctrl Pts',(-23.1750590180908,-4.52786428815014,
12.));
#234402=CARTESIAN_POINT('Ctrl Pts',(-23.1581684708761,-4.51880242116748,
0.));
#234403=CARTESIAN_POINT('Ctrl Pts',(-23.1581684708761,-4.51880242116748,
12.));
#234404=CARTESIAN_POINT('Ctrl Pts',(-23.1413554691123,-4.5098417322706,
0.));
#234405=CARTESIAN_POINT('Ctrl Pts',(-23.1413554691123,-4.5098417322706,
12.));
#234406=CARTESIAN_POINT('Ctrl Pts',(-23.1246211242115,-4.50098225775171,
0.));
#234407=CARTESIAN_POINT('Ctrl Pts',(-23.1246211242115,-4.50098225775171,
12.));
#234408=CARTESIAN_POINT('Ctrl Pts',(-23.1079665632636,-4.49222403252216,
0.));
#234409=CARTESIAN_POINT('Ctrl Pts',(-23.1079665632636,-4.49222403252216,
12.));
#234410=CARTESIAN_POINT('Ctrl Pts',(-23.0913929293922,-4.48356709006788,
0.));
#234411=CARTESIAN_POINT('Ctrl Pts',(-23.0913929293922,-4.48356709006788,
12.));
#234412=CARTESIAN_POINT('Ctrl Pts',(-23.0749013821881,-4.47501146242856,
0.));
#234413=CARTESIAN_POINT('Ctrl Pts',(-23.0749013821881,-4.47501146242856,
12.));
#234414=CARTESIAN_POINT('Ctrl Pts',(-23.0584930981732,-4.4665571801823,
0.));
#234415=CARTESIAN_POINT('Ctrl Pts',(-23.0584930981732,-4.4665571801823,
12.));
#234416=CARTESIAN_POINT('Ctrl Pts',(-23.0421692712467,-4.45820427241683,
0.));
#234417=CARTESIAN_POINT('Ctrl Pts',(-23.0421692712467,-4.45820427241683,
12.));
#234418=CARTESIAN_POINT('Ctrl Pts',(-23.0259311131392,-4.44995276669686,
0.));
#234419=CARTESIAN_POINT('Ctrl Pts',(-23.0259311131392,-4.44995276669686,
12.));
#234420=CARTESIAN_POINT('Ctrl Pts',(-23.0097798538395,-4.44180268901643,
0.));
#234421=CARTESIAN_POINT('Ctrl Pts',(-23.0097798538395,-4.44180268901643,
12.));
#234422=CARTESIAN_POINT('Ctrl Pts',(-22.9937167421006,-4.43375406376879,
0.));
#234423=CARTESIAN_POINT('Ctrl Pts',(-22.9937167421006,-4.43375406376879,
12.));
#234424=CARTESIAN_POINT('Ctrl Pts',(-22.977743046002,-4.42580691372751,
0.));
#234425=CARTESIAN_POINT('Ctrl Pts',(-22.977743046002,-4.42580691372751,
12.));
#234426=CARTESIAN_POINT('Ctrl Pts',(-22.9618600534866,-4.41796126001302,
0.));
#234427=CARTESIAN_POINT('Ctrl Pts',(-22.9618600534866,-4.41796126001302,
12.));
#234428=CARTESIAN_POINT('Ctrl Pts',(-22.9460690729093,-4.41021712205553,
0.));
#234429=CARTESIAN_POINT('Ctrl Pts',(-22.9460690729093,-4.41021712205553,
12.));
#234430=CARTESIAN_POINT('Ctrl Pts',(-22.930371433555,-4.40257451754323,
0.));
#234431=CARTESIAN_POINT('Ctrl Pts',(-22.930371433555,-4.40257451754323,
12.));
#234432=CARTESIAN_POINT('Ctrl Pts',(-22.9147684862426,-4.39503346238473,
0.));
#234433=CARTESIAN_POINT('Ctrl Pts',(-22.9147684862426,-4.39503346238473,
12.));
#234434=CARTESIAN_POINT('Ctrl Pts',(-22.8992616040108,-4.38759397068406,
0.));
#234435=CARTESIAN_POINT('Ctrl Pts',(-22.8992616040108,-4.38759397068406,
12.));
#234436=CARTESIAN_POINT('Ctrl Pts',(-22.8838521827701,-4.38025605470093,
0.));
#234437=CARTESIAN_POINT('Ctrl Pts',(-22.8838521827701,-4.38025605470093,
12.));
#234438=CARTESIAN_POINT('Ctrl Pts',(-22.8685416419725,-4.37301972480745,
0.));
#234439=CARTESIAN_POINT('Ctrl Pts',(-22.8685416419725,-4.37301972480745,
12.));
#234440=CARTESIAN_POINT('Ctrl Pts',(-22.8533314252422,-4.36588498942997,
0.));
#234441=CARTESIAN_POINT('Ctrl Pts',(-22.8533314252422,-4.36588498942997,
12.));
#234442=CARTESIAN_POINT('Ctrl Pts',(-22.8382230011184,-4.35885185500546,
0.));
#234443=CARTESIAN_POINT('Ctrl Pts',(-22.8382230011184,-4.35885185500546,
12.));
#234444=CARTESIAN_POINT('Ctrl Pts',(-22.8232178638876,-4.35192032594791,
0.));
#234445=CARTESIAN_POINT('Ctrl Pts',(-22.8232178638876,-4.35192032594791,
12.));
#234446=CARTESIAN_POINT('Ctrl Pts',(-22.8083175343791,-4.34509040460062,
0.));
#234447=CARTESIAN_POINT('Ctrl Pts',(-22.8083175343791,-4.34509040460062,
12.));
#234448=CARTESIAN_POINT('Ctrl Pts',(-22.7935235607806,-4.33836209118446,
0.));
#234449=CARTESIAN_POINT('Ctrl Pts',(-22.7935235607806,-4.33836209118446,
12.));
#234450=CARTESIAN_POINT('Ctrl Pts',(-22.7788375194076,-4.3317353837319,
0.));
#234451=CARTESIAN_POINT('Ctrl Pts',(-22.7788375194076,-4.3317353837319,
12.));
#234452=CARTESIAN_POINT('Ctrl Pts',(-22.7642610156475,-4.32521027803754,
0.));
#234453=CARTESIAN_POINT('Ctrl Pts',(-22.7642610156475,-4.32521027803754,
12.));
#234454=CARTESIAN_POINT('Ctrl Pts',(-22.7497956849848,-4.31878676761235,
0.));
#234455=CARTESIAN_POINT('Ctrl Pts',(-22.7497956849848,-4.31878676761235,
12.));
#234456=CARTESIAN_POINT('Ctrl Pts',(-22.7354431939926,-4.31246484362549,
0.));
#234457=CARTESIAN_POINT('Ctrl Pts',(-22.7354431939926,-4.31246484362549,
12.));
#234458=CARTESIAN_POINT('Ctrl Pts',(-22.7212052413386,-4.30624449484069,
0.));
#234459=CARTESIAN_POINT('Ctrl Pts',(-22.7212052413386,-4.30624449484069,
12.));
#234460=CARTESIAN_POINT('Ctrl Pts',(-22.7070835587564,-4.3001257075406,
0.));
#234461=CARTESIAN_POINT('Ctrl Pts',(-22.7070835587564,-4.3001257075406,
12.));
#234462=CARTESIAN_POINT('Ctrl Pts',(-22.6930799122548,-4.29410846547056,
0.));
#234463=CARTESIAN_POINT('Ctrl Pts',(-22.6930799122548,-4.29410846547056,
12.));
#234464=CARTESIAN_POINT('Ctrl Pts',(-22.6791961033538,-4.28819274977763,
0.));
#234465=CARTESIAN_POINT('Ctrl Pts',(-22.6791961033538,-4.28819274977763,
12.));
#234466=CARTESIAN_POINT('Ctrl Pts',(-22.6654339703109,-4.28237853894059,
0.));
#234467=CARTESIAN_POINT('Ctrl Pts',(-22.6654339703109,-4.28237853894059,
12.));
#234468=CARTESIAN_POINT('Ctrl Pts',(-22.6517953893303,-4.2766658086912,
0.));
#234469=CARTESIAN_POINT('Ctrl Pts',(-22.6517953893303,-4.2766658086912,
12.));
#234470=CARTESIAN_POINT('Ctrl Pts',(-22.6382822758172,-4.27105453193004,
0.));
#234471=CARTESIAN_POINT('Ctrl Pts',(-22.6382822758172,-4.27105453193004,
12.));
#234472=CARTESIAN_POINT('Ctrl Pts',(-22.6248965859977,-4.26554467865576,
0.));
#234473=CARTESIAN_POINT('Ctrl Pts',(-22.6248965859977,-4.26554467865576,
12.));
#234474=CARTESIAN_POINT('Ctrl Pts',(-22.6116403184821,-4.26013621588305,
0.));
#234475=CARTESIAN_POINT('Ctrl Pts',(-22.6116403184821,-4.26013621588305,
12.));
#234476=CARTESIAN_POINT('Ctrl Pts',(-22.5985155158636,-4.25482910755481,
0.));
#234477=CARTESIAN_POINT('Ctrl Pts',(-22.5985155158636,-4.25482910755481,
12.));
#234478=CARTESIAN_POINT('Ctrl Pts',(-22.5855242662477,-4.24962331444177,
0.));
#234479=CARTESIAN_POINT('Ctrl Pts',(-22.5855242662477,-4.24962331444177,
12.));
#234480=CARTESIAN_POINT('Ctrl Pts',(-22.572668704992,-4.24451879404851,
0.));
#234481=CARTESIAN_POINT('Ctrl Pts',(-22.572668704992,-4.24451879404851,
12.));
#234482=CARTESIAN_POINT('Ctrl Pts',(-22.5599510166429,-4.23951550052522,
0.));
#234483=CARTESIAN_POINT('Ctrl Pts',(-22.5599510166429,-4.23951550052522,
12.));
#234484=CARTESIAN_POINT('Ctrl Pts',(-22.5473734368086,-4.23461338456712,
0.));
#234485=CARTESIAN_POINT('Ctrl Pts',(-22.5473734368086,-4.23461338456712,
12.));
#234486=CARTESIAN_POINT('Ctrl Pts',(-22.5349382540588,-4.22981239330733,
0.));
#234487=CARTESIAN_POINT('Ctrl Pts',(-22.5349382540588,-4.22981239330733,
12.));
#234488=CARTESIAN_POINT('Ctrl Pts',(-22.5226478117886,-4.22511247020041,
0.));
#234489=CARTESIAN_POINT('Ctrl Pts',(-22.5226478117886,-4.22511247020041,
12.));
#234490=CARTESIAN_POINT('Ctrl Pts',(-22.5105045108881,-4.22051355490196,
0.));
#234491=CARTESIAN_POINT('Ctrl Pts',(-22.5105045108881,-4.22051355490196,
12.));
#234492=CARTESIAN_POINT('Ctrl Pts',(-22.4985108124228,-4.21601558313906,
0.));
#234493=CARTESIAN_POINT('Ctrl Pts',(-22.4985108124228,-4.21601558313906,
12.));
#234494=CARTESIAN_POINT('Ctrl Pts',(-22.4866692403147,-4.21161848657428,
0.));
#234495=CARTESIAN_POINT('Ctrl Pts',(-22.4866692403147,-4.21161848657428,
12.));
#234496=CARTESIAN_POINT('Ctrl Pts',(-22.4749823839917,-4.20732219265649,
0.));
#234497=CARTESIAN_POINT('Ctrl Pts',(-22.4749823839917,-4.20732219265649,
12.));
#234498=CARTESIAN_POINT('Ctrl Pts',(-22.4634529011437,-4.20312662448174,
0.));
#234499=CARTESIAN_POINT('Ctrl Pts',(-22.4634529011437,-4.20312662448174,
12.));
#234500=CARTESIAN_POINT('Ctrl Pts',(-22.4520835205422,-4.19903170066358,
0.));
#234501=CARTESIAN_POINT('Ctrl Pts',(-22.4520835205422,-4.19903170066358,
12.));
#234502=CARTESIAN_POINT('Ctrl Pts',(-22.4408770448917,-4.1950373351886,
0.));
#234503=CARTESIAN_POINT('Ctrl Pts',(-22.4408770448917,-4.1950373351886,
12.));
#234504=CARTESIAN_POINT('Ctrl Pts',(-22.4298363535416,-4.19114343726932,
0.));
#234505=CARTESIAN_POINT('Ctrl Pts',(-22.4298363535416,-4.19114343726932,
12.));
#234506=CARTESIAN_POINT('Ctrl Pts',(-22.4189644056109,-4.18734991117707,
0.));
#234507=CARTESIAN_POINT('Ctrl Pts',(-22.4189644056109,-4.18734991117707,
12.));
#234508=CARTESIAN_POINT('Ctrl Pts',(-22.4082642454448,-4.18365665600839,
0.));
#234509=CARTESIAN_POINT('Ctrl Pts',(-22.4082642454448,-4.18365665600839,
12.));
#234510=CARTESIAN_POINT('Ctrl Pts',(-22.3977390078074,-4.18006356544879,
0.));
#234511=CARTESIAN_POINT('Ctrl Pts',(-22.3977390078074,-4.18006356544879,
12.));
#234512=CARTESIAN_POINT('Ctrl Pts',(-22.3873919231339,-4.17657052752834,
0.));
#234513=CARTESIAN_POINT('Ctrl Pts',(-22.3873919231339,-4.17657052752834,
12.));
#234514=CARTESIAN_POINT('Ctrl Pts',(-22.3772263228624,-4.17317742436162,
0.));
#234515=CARTESIAN_POINT('Ctrl Pts',(-22.3772263228624,-4.17317742436162,
12.));
#234516=CARTESIAN_POINT('Ctrl Pts',(-22.3672456427605,-4.16988413199469,
0.));
#234517=CARTESIAN_POINT('Ctrl Pts',(-22.3672456427605,-4.16988413199469,
12.));
#234518=CARTESIAN_POINT('Ctrl Pts',(-22.3574534257397,-4.16669052026602,
0.));
#234519=CARTESIAN_POINT('Ctrl Pts',(-22.3574534257397,-4.16669052026602,
12.));
#234520=CARTESIAN_POINT('Ctrl Pts',(-22.3478533253886,-4.1635964526318,
0.));
#234521=CARTESIAN_POINT('Ctrl Pts',(-22.3478533253886,-4.1635964526318,
12.));
#234522=CARTESIAN_POINT('Ctrl Pts',(-22.3384491078599,-4.16060178604154,
0.));
#234523=CARTESIAN_POINT('Ctrl Pts',(-22.3384491078599,-4.16060178604154,
12.));
#234524=CARTESIAN_POINT('Ctrl Pts',(-22.3292446628957,-4.15770637047882,
0.));
#234525=CARTESIAN_POINT('Ctrl Pts',(-22.3292446628957,-4.15770637047882,
12.));
#234526=CARTESIAN_POINT('Ctrl Pts',(-22.3202440186979,-4.15491004835278,
0.));
#234527=CARTESIAN_POINT('Ctrl Pts',(-22.3202440186979,-4.15491004835278,
12.));
#234528=CARTESIAN_POINT('Ctrl Pts',(-22.3114513545186,-4.15221265396993,
0.));
#234529=CARTESIAN_POINT('Ctrl Pts',(-22.3114513545186,-4.15221265396993,
12.));
#234530=CARTESIAN_POINT('Ctrl Pts',(-22.3028710166935,-4.14961401285525,
0.));
#234531=CARTESIAN_POINT('Ctrl Pts',(-22.3028710166935,-4.14961401285525,
12.));
#234532=CARTESIAN_POINT('Ctrl Pts',(-22.2945075198468,-4.14711394168559,
0.));
#234533=CARTESIAN_POINT('Ctrl Pts',(-22.2945075198468,-4.14711394168559,
12.));
#234534=CARTESIAN_POINT('Ctrl Pts',(-22.2863655389167,-4.14471224859295,
0.));
#234535=CARTESIAN_POINT('Ctrl Pts',(-22.2863655389167,-4.14471224859295,
12.));
#234536=CARTESIAN_POINT('Ctrl Pts',(-22.2784499072026,-4.14240873321982,
0.));
#234537=CARTESIAN_POINT('Ctrl Pts',(-22.2784499072026,-4.14240873321982,
12.));
#234538=CARTESIAN_POINT('Ctrl Pts',(-22.2707656042456,-4.14020318715988,
0.));
#234539=CARTESIAN_POINT('Ctrl Pts',(-22.2707656042456,-4.14020318715988,
12.));
#234540=CARTESIAN_POINT('Ctrl Pts',(-22.263317791397,-4.13809539255418,
0.));
#234541=CARTESIAN_POINT('Ctrl Pts',(-22.263317791397,-4.13809539255418,
12.));
#234542=CARTESIAN_POINT('Ctrl Pts',(-22.2561118708422,-4.13608511977226,
0.));
#234543=CARTESIAN_POINT('Ctrl Pts',(-22.2561118708422,-4.13608511977226,
12.));
#234544=CARTESIAN_POINT('Ctrl Pts',(-22.2491535317789,-4.13417212558808,
0.));
#234545=CARTESIAN_POINT('Ctrl Pts',(-22.2491535317789,-4.13417212558808,
12.));
#234546=CARTESIAN_POINT('Ctrl Pts',(-22.2424488153523,-4.1323561506016,
0.));
#234547=CARTESIAN_POINT('Ctrl Pts',(-22.2424488153523,-4.1323561506016,
12.));
#234548=CARTESIAN_POINT('Ctrl Pts',(-22.2360040565534,-4.13063692157499,
0.));
#234549=CARTESIAN_POINT('Ctrl Pts',(-22.2360040565534,-4.13063692157499,
12.));
#234550=CARTESIAN_POINT('Ctrl Pts',(-22.2298258043947,-4.12901415463379,
0.));
#234551=CARTESIAN_POINT('Ctrl Pts',(-22.2298258043947,-4.12901415463379,
12.));
#234552=CARTESIAN_POINT('Ctrl Pts',(-22.2239207458781,-4.12748755830099,
0.));
#234553=CARTESIAN_POINT('Ctrl Pts',(-22.2239207458781,-4.12748755830099,
12.));
#234554=CARTESIAN_POINT('Ctrl Pts',(-22.2182956401341,-4.126056836133,0.));
#234555=CARTESIAN_POINT('Ctrl Pts',(-22.2182956401341,-4.126056836133,12.));
#234556=CARTESIAN_POINT('Ctrl Pts',(-22.2129576146671,-4.12472167516602,
0.));
#234557=CARTESIAN_POINT('Ctrl Pts',(-22.2129576146671,-4.12472167516602,
12.));
#234558=CARTESIAN_POINT('Ctrl Pts',(-22.2079143941719,-4.12348173702024,
0.));
#234559=CARTESIAN_POINT('Ctrl Pts',(-22.2079143941719,-4.12348173702024,
12.));
#234560=CARTESIAN_POINT('Ctrl Pts',(-22.2031746532106,-4.12233664408237,
0.));
#234561=CARTESIAN_POINT('Ctrl Pts',(-22.2031746532106,-4.12233664408237,
12.));
#234562=CARTESIAN_POINT('Ctrl Pts',(-22.1987479618246,-4.12128598183533,
0.));
#234563=CARTESIAN_POINT('Ctrl Pts',(-22.1987479618246,-4.12128598183533,
12.));
#234564=CARTESIAN_POINT('Ctrl Pts',(-22.1946440958098,-4.12032932637738,
0.));
#234565=CARTESIAN_POINT('Ctrl Pts',(-22.1946440958098,-4.12032932637738,
12.));
#234566=CARTESIAN_POINT('Ctrl Pts',(-22.1908725908525,-4.11946626228623,
0.));
#234567=CARTESIAN_POINT('Ctrl Pts',(-22.1908725908525,-4.11946626228623,
12.));
#234568=CARTESIAN_POINT('Ctrl Pts',(-22.1874419861496,-4.11869641271752,
0.));
#234569=CARTESIAN_POINT('Ctrl Pts',(-22.1874419861496,-4.11869641271752,
12.));
#234570=CARTESIAN_POINT('Ctrl Pts',(-22.1843613164855,-4.11801938107464,
0.));
#234571=CARTESIAN_POINT('Ctrl Pts',(-22.1843613164855,-4.11801938107464,
12.));
#234572=CARTESIAN_POINT('Ctrl Pts',(-22.1816414985788,-4.11743469691765,
0.));
#234573=CARTESIAN_POINT('Ctrl Pts',(-22.1816414985788,-4.11743469691765,
12.));
#234574=CARTESIAN_POINT('Ctrl Pts',(-22.179297473024,-4.11694173195041,
0.));
#234575=CARTESIAN_POINT('Ctrl Pts',(-22.179297473024,-4.11694173195041,
12.));
#234576=CARTESIAN_POINT('Ctrl Pts',(-22.177347426894,-4.11653973150558,
0.));
#234577=CARTESIAN_POINT('Ctrl Pts',(-22.177347426894,-4.11653973150558,
12.));
#234578=CARTESIAN_POINT('Ctrl Pts',(-22.1758088296598,-4.11622797217066,
0.));
#234579=CARTESIAN_POINT('Ctrl Pts',(-22.1758088296598,-4.11622797217066,
12.));
#234580=CARTESIAN_POINT('Ctrl Pts',(-22.1746949858773,-4.11600589882767,
0.));
#234581=CARTESIAN_POINT('Ctrl Pts',(-22.1746949858773,-4.11600589882767,
12.));
#234582=CARTESIAN_POINT('Ctrl Pts',(-22.174148802123,-4.11589976826061,
0.));
#234583=CARTESIAN_POINT('Ctrl Pts',(-22.174148802123,-4.11589976826061,
12.));
#234584=CARTESIAN_POINT('Ctrl Pts',(-22.1739341411684,-4.1158603587821,
0.));
#234585=CARTESIAN_POINT('Ctrl Pts',(-22.1739341411684,-4.1158603587821,
12.));
#234586=CARTESIAN_POINT('Ctrl Pts',(-22.1738776823239,-4.11585194677412,
0.));
#234587=CARTESIAN_POINT('Ctrl Pts',(-22.1738776823239,-4.11585194677412,
12.));
#234588=CARTESIAN_POINT('Ctrl Pts',(-22.1738711152697,-4.11585220600461,
0.));
#234589=CARTESIAN_POINT('Ctrl Pts',(-22.1738711152697,-4.11585220600461,
12.));
#234590=CARTESIAN_POINT('',(-25.2771067246846,-6.08833931617698,0.));
#234591=CARTESIAN_POINT('Ctrl Pts',(-25.2771067246846,-6.08833931617698,
0.));
#234592=CARTESIAN_POINT('Ctrl Pts',(-25.2729539149479,-6.08441489609824,
0.));
#234593=CARTESIAN_POINT('Ctrl Pts',(-25.2646490489816,-6.07657531787577,
0.));
#234594=CARTESIAN_POINT('Ctrl Pts',(-25.2521940105523,-6.06484373634696,
0.));
#234595=CARTESIAN_POINT('Ctrl Pts',(-25.2355918138798,-6.04925720151412,
0.));
#234596=CARTESIAN_POINT('Ctrl Pts',(-25.2148466201368,-6.02986667390187,
0.));
#234597=CARTESIAN_POINT('Ctrl Pts',(-25.1941090269638,-6.0105688180476,
0.));
#234598=CARTESIAN_POINT('Ctrl Pts',(-25.1733791296154,-5.99136367859838,
0.));
#234599=CARTESIAN_POINT('Ctrl Pts',(-25.1526570863065,-5.97225131495636,
0.));
#234600=CARTESIAN_POINT('Ctrl Pts',(-25.1319431317273,-5.95323180187348,
0.));
#234601=CARTESIAN_POINT('Ctrl Pts',(-25.1112375971182,-5.93430523086776,
0.));
#234602=CARTESIAN_POINT('Ctrl Pts',(-25.0905409050863,-5.91547170844382,
0.));
#234603=CARTESIAN_POINT('Ctrl Pts',(-25.0698535426593,-5.89673135155459,
0.));
#234604=CARTESIAN_POINT('Ctrl Pts',(-25.0491760405965,-5.87808428385329,
0.));
#234605=CARTESIAN_POINT('Ctrl Pts',(-25.0285089498922,-5.8595306315681,
0.));
#234606=CARTESIAN_POINT('Ctrl Pts',(-25.0078528200558,-5.84107051963073,
0.));
#234607=CARTESIAN_POINT('Ctrl Pts',(-24.9872081752709,-5.82270406744214,
0.));
#234608=CARTESIAN_POINT('Ctrl Pts',(-24.9665754954462,-5.80443138549747,
0.));
#234609=CARTESIAN_POINT('Ctrl Pts',(-24.9459552293308,-5.78625257775703,
0.));
#234610=CARTESIAN_POINT('Ctrl Pts',(-24.9253478043632,-5.76816774342236,
0.));
#234611=CARTESIAN_POINT('Ctrl Pts',(-24.9047536376467,-5.75017697890813,
0.));
#234612=CARTESIAN_POINT('Ctrl Pts',(-24.8841731467219,-5.73228037976926,
0.));
#234613=CARTESIAN_POINT('Ctrl Pts',(-24.8636067597677,-5.71447804252019,
0.));
#234614=CARTESIAN_POINT('Ctrl Pts',(-24.8430549277634,-5.69677006679429,
0.));
#234615=CARTESIAN_POINT('Ctrl Pts',(-24.822518122386,-5.67915655496524,
0.));
#234616=CARTESIAN_POINT('Ctrl Pts',(-24.8019968304618,-5.66163761114903,
0.));
#234617=CARTESIAN_POINT('Ctrl Pts',(-24.7814915496728,-5.64421334042247,
0.));
#234618=CARTESIAN_POINT('Ctrl Pts',(-24.76100278357,-5.62688384790919,0.));
#234619=CARTESIAN_POINT('Ctrl Pts',(-24.7405310372736,-5.60964923798495,
0.));
#234620=CARTESIAN_POINT('Ctrl Pts',(-24.7200768119079,-5.59250961323995,
0.));
#234621=CARTESIAN_POINT('Ctrl Pts',(-24.6996406035507,-5.57546507427766,
0.));
#234622=CARTESIAN_POINT('Ctrl Pts',(-24.6792229061785,-5.55851572025389,
0.));
#234623=CARTESIAN_POINT('Ctrl Pts',(-24.6588242134733,-5.54166164919593,
0.));
#234624=CARTESIAN_POINT('Ctrl Pts',(-24.6384450211466,-5.52490295840996,
0.));
#234625=CARTESIAN_POINT('Ctrl Pts',(-24.618085828918,-5.50823974481959,
0.));
#234626=CARTESIAN_POINT('Ctrl Pts',(-24.5977471429365,-5.49167210537235,
0.));
#234627=CARTESIAN_POINT('Ctrl Pts',(-24.5774294770329,-5.47520013724403,
0.));
#234628=CARTESIAN_POINT('Ctrl Pts',(-24.5571333514841,-5.45882393762244,
0.));
#234629=CARTESIAN_POINT('Ctrl Pts',(-24.5368592922861,-5.44254360356865,
0.));
#234630=CARTESIAN_POINT('Ctrl Pts',(-24.5166078302107,-5.42635923183411,
0.));
#234631=CARTESIAN_POINT('Ctrl Pts',(-24.4963794999831,-5.41027091869242,
0.));
#234632=CARTESIAN_POINT('Ctrl Pts',(-24.4761748393322,-5.3942787597383,
0.));
#234633=CARTESIAN_POINT('Ctrl Pts',(-24.4559943883159,-5.37838284973706,
0.));
#234634=CARTESIAN_POINT('Ctrl Pts',(-24.4358386899152,-5.36258328273639,
0.));
#234635=CARTESIAN_POINT('Ctrl Pts',(-24.4157082904615,-5.34688015213546,
0.));
#234636=CARTESIAN_POINT('Ctrl Pts',(-24.3956037401293,-5.33127355076036,
0.));
#234637=CARTESIAN_POINT('Ctrl Pts',(-24.3755255933917,-5.31576357092524,
0.));
#234638=CARTESIAN_POINT('Ctrl Pts',(-24.3554744095075,-5.30035030449058,
0.));
#234639=CARTESIAN_POINT('Ctrl Pts',(-24.3354507529415,-5.28503384290644,
0.));
#234640=CARTESIAN_POINT('Ctrl Pts',(-24.3154551932222,-5.26981427718796,
0.));
#234641=CARTESIAN_POINT('Ctrl Pts',(-24.2954883048448,-5.25469169788856,
0.));
#234642=CARTESIAN_POINT('Ctrl Pts',(-24.2755506671526,-5.23966619506289,
0.));
#234643=CARTESIAN_POINT('Ctrl Pts',(-24.2556428642294,-5.22473785822441,
0.));
#234644=CARTESIAN_POINT('Ctrl Pts',(-24.2357654847765,-5.20990677629173,
0.));
#234645=CARTESIAN_POINT('Ctrl Pts',(-24.215919122017,-5.19517303753643,
0.));
#234646=CARTESIAN_POINT('Ctrl Pts',(-24.1961043738754,-5.18053672961392,
0.));
#234647=CARTESIAN_POINT('Ctrl Pts',(-24.1763218431343,-5.16599793957979,
0.));
#234648=CARTESIAN_POINT('Ctrl Pts',(-24.156572137597,-5.15155675390075,
0.));
#234649=CARTESIAN_POINT('Ctrl Pts',(-24.1368558702443,-5.13721325845744,
0.));
#234650=CARTESIAN_POINT('Ctrl Pts',(-24.117173659394,-5.12296753853859,
0.));
#234651=CARTESIAN_POINT('Ctrl Pts',(-24.0975261288446,-5.10881967883132,
0.));
#234652=CARTESIAN_POINT('Ctrl Pts',(-24.0779139079266,-5.09476976342625,
0.));
#234653=CARTESIAN_POINT('Ctrl Pts',(-24.0583376315638,-5.08081787581276,
0.));
#234654=CARTESIAN_POINT('Ctrl Pts',(-24.0387979403268,-5.06696409886641,
0.));
#234655=CARTESIAN_POINT('Ctrl Pts',(-24.0192954804896,-5.05320851483065,
0.));
#234656=CARTESIAN_POINT('Ctrl Pts',(-23.9998309040746,-5.03955120528521,
0.));
#234657=CARTESIAN_POINT('Ctrl Pts',(-23.9804048689227,-5.02599225112454,
0.));
#234658=CARTESIAN_POINT('Ctrl Pts',(-23.9610180388271,-5.01253173257453,
0.));
#234659=CARTESIAN_POINT('Ctrl Pts',(-23.9416710836529,-4.99916972919306,
0.));
#234660=CARTESIAN_POINT('Ctrl Pts',(-23.9223646794592,-4.98590631986532,
0.));
#234661=CARTESIAN_POINT('Ctrl Pts',(-23.9030995086163,-4.97274158279226,
0.));
#234662=CARTESIAN_POINT('Ctrl Pts',(-23.8838762599218,-4.9596755954656,
0.));
#234663=CARTESIAN_POINT('Ctrl Pts',(-23.8646956287168,-4.9467084346586,
0.));
#234664=CARTESIAN_POINT('Ctrl Pts',(-23.8455583170057,-4.93384017643432,
0.));
#234665=CARTESIAN_POINT('Ctrl Pts',(-23.8264650335717,-4.92107089613969,
0.));
#234666=CARTESIAN_POINT('Ctrl Pts',(-23.8074164940896,-4.90840066839344,
0.));
#234667=CARTESIAN_POINT('Ctrl Pts',(-23.7884134212384,-4.89582956706775,
0.));
#234668=CARTESIAN_POINT('Ctrl Pts',(-23.7694565448049,-4.88335766525573,
0.));
#234669=CARTESIAN_POINT('Ctrl Pts',(-23.7505466018245,-4.87098503527152,
0.));
#234670=CARTESIAN_POINT('Ctrl Pts',(-23.7316843367313,-4.85871174865499,
0.));
#234671=CARTESIAN_POINT('Ctrl Pts',(-23.7128705015017,-4.84653787616425,
0.));
#234672=CARTESIAN_POINT('Ctrl Pts',(-23.6941058557971,-4.83446348776265,
0.));
#234673=CARTESIAN_POINT('Ctrl Pts',(-23.675391167102,-4.82248865259562,
0.));
#234674=CARTESIAN_POINT('Ctrl Pts',(-23.6567272108628,-4.81061343896432,
0.));
#234675=CARTESIAN_POINT('Ctrl Pts',(-23.6381147706579,-4.7988379143322,
0.));
#234676=CARTESIAN_POINT('Ctrl Pts',(-23.6195546383624,-4.78716214532098,
0.));
#234677=CARTESIAN_POINT('Ctrl Pts',(-23.6010476143099,-4.77558619769872,
0.));
#234678=CARTESIAN_POINT('Ctrl Pts',(-23.5825945074535,-4.76411013636251,
0.));
#234679=CARTESIAN_POINT('Ctrl Pts',(-23.5641961355168,-4.75273402530617,
0.));
#234680=CARTESIAN_POINT('Ctrl Pts',(-23.545853325171,-4.74145792760698,
0.));
#234681=CARTESIAN_POINT('Ctrl Pts',(-23.5275669122372,-4.7302819054303,
0.));
#234682=CARTESIAN_POINT('Ctrl Pts',(-23.509337741878,-4.71920602001901,
0.));
#234683=CARTESIAN_POINT('Ctrl Pts',(-23.491166668789,-4.70823033167818,
0.));
#234684=CARTESIAN_POINT('Ctrl Pts',(-23.4730545573853,-4.69735489975024,
0.));
#234685=CARTESIAN_POINT('Ctrl Pts',(-23.455002281986,-4.68657978258303,
0.));
#234686=CARTESIAN_POINT('Ctrl Pts',(-23.4370107270451,-4.67590503753058,
0.));
#234687=CARTESIAN_POINT('Ctrl Pts',(-23.4190807873803,-4.6653307209467,
0.));
#234688=CARTESIAN_POINT('Ctrl Pts',(-23.4012133683959,-4.65485688816924,
0.));
#234689=CARTESIAN_POINT('Ctrl Pts',(-23.3834093863068,-4.6444835934993,
0.));
#234690=CARTESIAN_POINT('Ctrl Pts',(-23.3656697683489,-4.63421089016541,
0.));
#234691=CARTESIAN_POINT('Ctrl Pts',(-23.3479954530272,-4.62403883030805,
0.));
#234692=CARTESIAN_POINT('Ctrl Pts',(-23.3303873903938,-4.6139674649783,
0.));
#234693=CARTESIAN_POINT('Ctrl Pts',(-23.3128465423115,-4.60399684412163,
0.));
#234694=CARTESIAN_POINT('Ctrl Pts',(-23.2953738827191,-4.5941270165575,
0.));
#234695=CARTESIAN_POINT('Ctrl Pts',(-23.2779703978876,-4.5843580299469,
0.));
#234696=CARTESIAN_POINT('Ctrl Pts',(-23.2606370866866,-4.57468993076097,
0.));
#234697=CARTESIAN_POINT('Ctrl Pts',(-23.2433749609131,-4.56512276427839,
0.));
#234698=CARTESIAN_POINT('Ctrl Pts',(-23.2261850456064,-4.55565657456975,
0.));
#234699=CARTESIAN_POINT('Ctrl Pts',(-23.2090683793629,-4.54629140447544,
0.));
#234700=CARTESIAN_POINT('Ctrl Pts',(-23.1920260146465,-4.53702729557566,
0.));
#234701=CARTESIAN_POINT('Ctrl Pts',(-23.1750590180908,-4.52786428815014,
0.));
#234702=CARTESIAN_POINT('Ctrl Pts',(-23.1581684708761,-4.51880242116748,
0.));
#234703=CARTESIAN_POINT('Ctrl Pts',(-23.1413554691123,-4.5098417322706,
0.));
#234704=CARTESIAN_POINT('Ctrl Pts',(-23.1246211242115,-4.50098225775171,
0.));
#234705=CARTESIAN_POINT('Ctrl Pts',(-23.1079665632636,-4.49222403252216,
0.));
#234706=CARTESIAN_POINT('Ctrl Pts',(-23.0913929293922,-4.48356709006788,
0.));
#234707=CARTESIAN_POINT('Ctrl Pts',(-23.0749013821881,-4.47501146242856,
0.));
#234708=CARTESIAN_POINT('Ctrl Pts',(-23.0584930981732,-4.4665571801823,
0.));
#234709=CARTESIAN_POINT('Ctrl Pts',(-23.0421692712467,-4.45820427241683,
0.));
#234710=CARTESIAN_POINT('Ctrl Pts',(-23.0259311131392,-4.44995276669686,
0.));
#234711=CARTESIAN_POINT('Ctrl Pts',(-23.0097798538395,-4.44180268901643,
0.));
#234712=CARTESIAN_POINT('Ctrl Pts',(-22.9937167421006,-4.43375406376879,
0.));
#234713=CARTESIAN_POINT('Ctrl Pts',(-22.977743046002,-4.42580691372751,
0.));
#234714=CARTESIAN_POINT('Ctrl Pts',(-22.9618600534866,-4.41796126001302,
0.));
#234715=CARTESIAN_POINT('Ctrl Pts',(-22.9460690729093,-4.41021712205553,
0.));
#234716=CARTESIAN_POINT('Ctrl Pts',(-22.930371433555,-4.40257451754323,
0.));
#234717=CARTESIAN_POINT('Ctrl Pts',(-22.9147684862426,-4.39503346238473,
0.));
#234718=CARTESIAN_POINT('Ctrl Pts',(-22.8992616040108,-4.38759397068406,
0.));
#234719=CARTESIAN_POINT('Ctrl Pts',(-22.8838521827701,-4.38025605470093,
0.));
#234720=CARTESIAN_POINT('Ctrl Pts',(-22.8685416419725,-4.37301972480745,
0.));
#234721=CARTESIAN_POINT('Ctrl Pts',(-22.8533314252422,-4.36588498942997,
0.));
#234722=CARTESIAN_POINT('Ctrl Pts',(-22.8382230011184,-4.35885185500546,
0.));
#234723=CARTESIAN_POINT('Ctrl Pts',(-22.8232178638876,-4.35192032594791,
0.));
#234724=CARTESIAN_POINT('Ctrl Pts',(-22.8083175343791,-4.34509040460062,
0.));
#234725=CARTESIAN_POINT('Ctrl Pts',(-22.7935235607806,-4.33836209118446,
0.));
#234726=CARTESIAN_POINT('Ctrl Pts',(-22.7788375194076,-4.3317353837319,
0.));
#234727=CARTESIAN_POINT('Ctrl Pts',(-22.7642610156475,-4.32521027803754,
0.));
#234728=CARTESIAN_POINT('Ctrl Pts',(-22.7497956849848,-4.31878676761235,
0.));
#234729=CARTESIAN_POINT('Ctrl Pts',(-22.7354431939926,-4.31246484362549,
0.));
#234730=CARTESIAN_POINT('Ctrl Pts',(-22.7212052413386,-4.30624449484069,
0.));
#234731=CARTESIAN_POINT('Ctrl Pts',(-22.7070835587564,-4.3001257075406,
0.));
#234732=CARTESIAN_POINT('Ctrl Pts',(-22.6930799122548,-4.29410846547056,
0.));
#234733=CARTESIAN_POINT('Ctrl Pts',(-22.6791961033538,-4.28819274977763,
0.));
#234734=CARTESIAN_POINT('Ctrl Pts',(-22.6654339703109,-4.28237853894059,
0.));
#234735=CARTESIAN_POINT('Ctrl Pts',(-22.6517953893303,-4.2766658086912,
0.));
#234736=CARTESIAN_POINT('Ctrl Pts',(-22.6382822758172,-4.27105453193004,
0.));
#234737=CARTESIAN_POINT('Ctrl Pts',(-22.6248965859977,-4.26554467865576,
0.));
#234738=CARTESIAN_POINT('Ctrl Pts',(-22.6116403184821,-4.26013621588305,
0.));
#234739=CARTESIAN_POINT('Ctrl Pts',(-22.5985155158636,-4.25482910755481,
0.));
#234740=CARTESIAN_POINT('Ctrl Pts',(-22.5855242662477,-4.24962331444177,
0.));
#234741=CARTESIAN_POINT('Ctrl Pts',(-22.572668704992,-4.24451879404851,
0.));
#234742=CARTESIAN_POINT('Ctrl Pts',(-22.5599510166429,-4.23951550052522,
0.));
#234743=CARTESIAN_POINT('Ctrl Pts',(-22.5473734368086,-4.23461338456712,
0.));
#234744=CARTESIAN_POINT('Ctrl Pts',(-22.5349382540588,-4.22981239330733,
0.));
#234745=CARTESIAN_POINT('Ctrl Pts',(-22.5226478117886,-4.22511247020041,
0.));
#234746=CARTESIAN_POINT('Ctrl Pts',(-22.5105045108881,-4.22051355490196,
0.));
#234747=CARTESIAN_POINT('Ctrl Pts',(-22.4985108124228,-4.21601558313906,
0.));
#234748=CARTESIAN_POINT('Ctrl Pts',(-22.4866692403147,-4.21161848657428,
0.));
#234749=CARTESIAN_POINT('Ctrl Pts',(-22.4749823839917,-4.20732219265649,
0.));
#234750=CARTESIAN_POINT('Ctrl Pts',(-22.4634529011437,-4.20312662448174,
0.));
#234751=CARTESIAN_POINT('Ctrl Pts',(-22.4520835205422,-4.19903170066358,
0.));
#234752=CARTESIAN_POINT('Ctrl Pts',(-22.4408770448917,-4.1950373351886,
0.));
#234753=CARTESIAN_POINT('Ctrl Pts',(-22.4298363535416,-4.19114343726932,
0.));
#234754=CARTESIAN_POINT('Ctrl Pts',(-22.4189644056109,-4.18734991117707,
0.));
#234755=CARTESIAN_POINT('Ctrl Pts',(-22.4082642454448,-4.18365665600839,
0.));
#234756=CARTESIAN_POINT('Ctrl Pts',(-22.3977390078074,-4.18006356544879,
0.));
#234757=CARTESIAN_POINT('Ctrl Pts',(-22.3873919231339,-4.17657052752834,
0.));
#234758=CARTESIAN_POINT('Ctrl Pts',(-22.3772263228624,-4.17317742436162,
0.));
#234759=CARTESIAN_POINT('Ctrl Pts',(-22.3672456427605,-4.16988413199469,
0.));
#234760=CARTESIAN_POINT('Ctrl Pts',(-22.3574534257397,-4.16669052026602,
0.));
#234761=CARTESIAN_POINT('Ctrl Pts',(-22.3478533253886,-4.1635964526318,
0.));
#234762=CARTESIAN_POINT('Ctrl Pts',(-22.3384491078599,-4.16060178604154,
0.));
#234763=CARTESIAN_POINT('Ctrl Pts',(-22.3292446628957,-4.15770637047882,
0.));
#234764=CARTESIAN_POINT('Ctrl Pts',(-22.3202440186979,-4.15491004835278,
0.));
#234765=CARTESIAN_POINT('Ctrl Pts',(-22.3114513545186,-4.15221265396993,
0.));
#234766=CARTESIAN_POINT('Ctrl Pts',(-22.3028710166935,-4.14961401285525,
0.));
#234767=CARTESIAN_POINT('Ctrl Pts',(-22.2945075198468,-4.14711394168559,
0.));
#234768=CARTESIAN_POINT('Ctrl Pts',(-22.2863655389167,-4.14471224859295,
0.));
#234769=CARTESIAN_POINT('Ctrl Pts',(-22.2784499072026,-4.14240873321982,
0.));
#234770=CARTESIAN_POINT('Ctrl Pts',(-22.2707656042456,-4.14020318715988,
0.));
#234771=CARTESIAN_POINT('Ctrl Pts',(-22.263317791397,-4.13809539255418,
0.));
#234772=CARTESIAN_POINT('Ctrl Pts',(-22.2561118708422,-4.13608511977226,
0.));
#234773=CARTESIAN_POINT('Ctrl Pts',(-22.2491535317789,-4.13417212558808,
0.));
#234774=CARTESIAN_POINT('Ctrl Pts',(-22.2424488153523,-4.1323561506016,
0.));
#234775=CARTESIAN_POINT('Ctrl Pts',(-22.2360040565534,-4.13063692157499,
0.));
#234776=CARTESIAN_POINT('Ctrl Pts',(-22.2298258043947,-4.12901415463379,
0.));
#234777=CARTESIAN_POINT('Ctrl Pts',(-22.2239207458781,-4.12748755830099,
0.));
#234778=CARTESIAN_POINT('Ctrl Pts',(-22.2182956401341,-4.126056836133,0.));
#234779=CARTESIAN_POINT('Ctrl Pts',(-22.2129576146671,-4.12472167516602,
0.));
#234780=CARTESIAN_POINT('Ctrl Pts',(-22.2079143941719,-4.12348173702024,
0.));
#234781=CARTESIAN_POINT('Ctrl Pts',(-22.2031746532106,-4.12233664408237,
0.));
#234782=CARTESIAN_POINT('Ctrl Pts',(-22.1987479618246,-4.12128598183533,
0.));
#234783=CARTESIAN_POINT('Ctrl Pts',(-22.1946440958098,-4.12032932637738,
0.));
#234784=CARTESIAN_POINT('Ctrl Pts',(-22.1908725908525,-4.11946626228623,
0.));
#234785=CARTESIAN_POINT('Ctrl Pts',(-22.1874419861496,-4.11869641271752,
0.));
#234786=CARTESIAN_POINT('Ctrl Pts',(-22.1843613164855,-4.11801938107464,
0.));
#234787=CARTESIAN_POINT('Ctrl Pts',(-22.1816414985788,-4.11743469691765,
0.));
#234788=CARTESIAN_POINT('Ctrl Pts',(-22.179297473024,-4.11694173195041,
0.));
#234789=CARTESIAN_POINT('Ctrl Pts',(-22.177347426894,-4.11653973150558,
0.));
#234790=CARTESIAN_POINT('Ctrl Pts',(-22.1758088296598,-4.11622797217066,
0.));
#234791=CARTESIAN_POINT('Ctrl Pts',(-22.1746949858773,-4.11600589882767,
0.));
#234792=CARTESIAN_POINT('Ctrl Pts',(-22.174148802123,-4.11589976826061,
0.));
#234793=CARTESIAN_POINT('Ctrl Pts',(-22.1739341411684,-4.1158603587821,
0.));
#234794=CARTESIAN_POINT('Ctrl Pts',(-22.1738776823239,-4.11585194677412,
0.));
#234795=CARTESIAN_POINT('Ctrl Pts',(-22.1738711152697,-4.11585220600461,
0.));
#234796=CARTESIAN_POINT('',(-25.2771067246846,-6.08833931617698,12.));
#234797=CARTESIAN_POINT('',(-25.2771067246846,-6.08833931617698,0.));
#234798=CARTESIAN_POINT('Ctrl Pts',(-22.1738711152697,-4.11585220600461,
12.));
#234799=CARTESIAN_POINT('Ctrl Pts',(-22.1738776823239,-4.11585194677412,
12.));
#234800=CARTESIAN_POINT('Ctrl Pts',(-22.1739341411684,-4.1158603587821,
12.));
#234801=CARTESIAN_POINT('Ctrl Pts',(-22.174148802123,-4.11589976826061,
12.));
#234802=CARTESIAN_POINT('Ctrl Pts',(-22.1746949858773,-4.11600589882767,
12.));
#234803=CARTESIAN_POINT('Ctrl Pts',(-22.1758088296598,-4.11622797217066,
12.));
#234804=CARTESIAN_POINT('Ctrl Pts',(-22.177347426894,-4.11653973150558,
12.));
#234805=CARTESIAN_POINT('Ctrl Pts',(-22.179297473024,-4.11694173195041,
12.));
#234806=CARTESIAN_POINT('Ctrl Pts',(-22.1816414985788,-4.11743469691765,
12.));
#234807=CARTESIAN_POINT('Ctrl Pts',(-22.1843613164855,-4.11801938107464,
12.));
#234808=CARTESIAN_POINT('Ctrl Pts',(-22.1874419861496,-4.11869641271752,
12.));
#234809=CARTESIAN_POINT('Ctrl Pts',(-22.1908725908525,-4.11946626228623,
12.));
#234810=CARTESIAN_POINT('Ctrl Pts',(-22.1946440958098,-4.12032932637738,
12.));
#234811=CARTESIAN_POINT('Ctrl Pts',(-22.1987479618246,-4.12128598183533,
12.));
#234812=CARTESIAN_POINT('Ctrl Pts',(-22.2031746532106,-4.12233664408237,
12.));
#234813=CARTESIAN_POINT('Ctrl Pts',(-22.2079143941719,-4.12348173702024,
12.));
#234814=CARTESIAN_POINT('Ctrl Pts',(-22.2129576146671,-4.12472167516602,
12.));
#234815=CARTESIAN_POINT('Ctrl Pts',(-22.2182956401341,-4.126056836133,12.));
#234816=CARTESIAN_POINT('Ctrl Pts',(-22.2239207458781,-4.12748755830099,
12.));
#234817=CARTESIAN_POINT('Ctrl Pts',(-22.2298258043947,-4.12901415463379,
12.));
#234818=CARTESIAN_POINT('Ctrl Pts',(-22.2360040565534,-4.13063692157499,
12.));
#234819=CARTESIAN_POINT('Ctrl Pts',(-22.2424488153523,-4.1323561506016,
12.));
#234820=CARTESIAN_POINT('Ctrl Pts',(-22.2491535317789,-4.13417212558808,
12.));
#234821=CARTESIAN_POINT('Ctrl Pts',(-22.2561118708422,-4.13608511977226,
12.));
#234822=CARTESIAN_POINT('Ctrl Pts',(-22.263317791397,-4.13809539255418,
12.));
#234823=CARTESIAN_POINT('Ctrl Pts',(-22.2707656042456,-4.14020318715988,
12.));
#234824=CARTESIAN_POINT('Ctrl Pts',(-22.2784499072026,-4.14240873321982,
12.));
#234825=CARTESIAN_POINT('Ctrl Pts',(-22.2863655389167,-4.14471224859295,
12.));
#234826=CARTESIAN_POINT('Ctrl Pts',(-22.2945075198468,-4.14711394168559,
12.));
#234827=CARTESIAN_POINT('Ctrl Pts',(-22.3028710166935,-4.14961401285525,
12.));
#234828=CARTESIAN_POINT('Ctrl Pts',(-22.3114513545186,-4.15221265396993,
12.));
#234829=CARTESIAN_POINT('Ctrl Pts',(-22.3202440186979,-4.15491004835278,
12.));
#234830=CARTESIAN_POINT('Ctrl Pts',(-22.3292446628957,-4.15770637047882,
12.));
#234831=CARTESIAN_POINT('Ctrl Pts',(-22.3384491078599,-4.16060178604154,
12.));
#234832=CARTESIAN_POINT('Ctrl Pts',(-22.3478533253886,-4.1635964526318,
12.));
#234833=CARTESIAN_POINT('Ctrl Pts',(-22.3574534257397,-4.16669052026602,
12.));
#234834=CARTESIAN_POINT('Ctrl Pts',(-22.3672456427605,-4.16988413199469,
12.));
#234835=CARTESIAN_POINT('Ctrl Pts',(-22.3772263228624,-4.17317742436162,
12.));
#234836=CARTESIAN_POINT('Ctrl Pts',(-22.3873919231339,-4.17657052752834,
12.));
#234837=CARTESIAN_POINT('Ctrl Pts',(-22.3977390078074,-4.18006356544879,
12.));
#234838=CARTESIAN_POINT('Ctrl Pts',(-22.4082642454448,-4.18365665600839,
12.));
#234839=CARTESIAN_POINT('Ctrl Pts',(-22.4189644056109,-4.18734991117707,
12.));
#234840=CARTESIAN_POINT('Ctrl Pts',(-22.4298363535416,-4.19114343726932,
12.));
#234841=CARTESIAN_POINT('Ctrl Pts',(-22.4408770448917,-4.1950373351886,
12.));
#234842=CARTESIAN_POINT('Ctrl Pts',(-22.4520835205422,-4.19903170066358,
12.));
#234843=CARTESIAN_POINT('Ctrl Pts',(-22.4634529011437,-4.20312662448174,
12.));
#234844=CARTESIAN_POINT('Ctrl Pts',(-22.4749823839917,-4.20732219265649,
12.));
#234845=CARTESIAN_POINT('Ctrl Pts',(-22.4866692403147,-4.21161848657428,
12.));
#234846=CARTESIAN_POINT('Ctrl Pts',(-22.4985108124228,-4.21601558313906,
12.));
#234847=CARTESIAN_POINT('Ctrl Pts',(-22.5105045108881,-4.22051355490196,
12.));
#234848=CARTESIAN_POINT('Ctrl Pts',(-22.5226478117886,-4.22511247020041,
12.));
#234849=CARTESIAN_POINT('Ctrl Pts',(-22.5349382540588,-4.22981239330733,
12.));
#234850=CARTESIAN_POINT('Ctrl Pts',(-22.5473734368086,-4.23461338456712,
12.));
#234851=CARTESIAN_POINT('Ctrl Pts',(-22.5599510166429,-4.23951550052522,
12.));
#234852=CARTESIAN_POINT('Ctrl Pts',(-22.572668704992,-4.24451879404851,
12.));
#234853=CARTESIAN_POINT('Ctrl Pts',(-22.5855242662477,-4.24962331444177,
12.));
#234854=CARTESIAN_POINT('Ctrl Pts',(-22.5985155158636,-4.25482910755481,
12.));
#234855=CARTESIAN_POINT('Ctrl Pts',(-22.6116403184821,-4.26013621588305,
12.));
#234856=CARTESIAN_POINT('Ctrl Pts',(-22.6248965859977,-4.26554467865576,
12.));
#234857=CARTESIAN_POINT('Ctrl Pts',(-22.6382822758172,-4.27105453193004,
12.));
#234858=CARTESIAN_POINT('Ctrl Pts',(-22.6517953893303,-4.2766658086912,
12.));
#234859=CARTESIAN_POINT('Ctrl Pts',(-22.6654339703109,-4.28237853894059,
12.));
#234860=CARTESIAN_POINT('Ctrl Pts',(-22.6791961033538,-4.28819274977763,
12.));
#234861=CARTESIAN_POINT('Ctrl Pts',(-22.6930799122548,-4.29410846547056,
12.));
#234862=CARTESIAN_POINT('Ctrl Pts',(-22.7070835587564,-4.3001257075406,
12.));
#234863=CARTESIAN_POINT('Ctrl Pts',(-22.7212052413386,-4.30624449484069,
12.));
#234864=CARTESIAN_POINT('Ctrl Pts',(-22.7354431939926,-4.31246484362549,
12.));
#234865=CARTESIAN_POINT('Ctrl Pts',(-22.7497956849848,-4.31878676761235,
12.));
#234866=CARTESIAN_POINT('Ctrl Pts',(-22.7642610156475,-4.32521027803754,
12.));
#234867=CARTESIAN_POINT('Ctrl Pts',(-22.7788375194076,-4.3317353837319,
12.));
#234868=CARTESIAN_POINT('Ctrl Pts',(-22.7935235607806,-4.33836209118446,
12.));
#234869=CARTESIAN_POINT('Ctrl Pts',(-22.8083175343791,-4.34509040460062,
12.));
#234870=CARTESIAN_POINT('Ctrl Pts',(-22.8232178638876,-4.35192032594791,
12.));
#234871=CARTESIAN_POINT('Ctrl Pts',(-22.8382230011184,-4.35885185500546,
12.));
#234872=CARTESIAN_POINT('Ctrl Pts',(-22.8533314252422,-4.36588498942997,
12.));
#234873=CARTESIAN_POINT('Ctrl Pts',(-22.8685416419725,-4.37301972480745,
12.));
#234874=CARTESIAN_POINT('Ctrl Pts',(-22.8838521827701,-4.38025605470093,
12.));
#234875=CARTESIAN_POINT('Ctrl Pts',(-22.8992616040108,-4.38759397068406,
12.));
#234876=CARTESIAN_POINT('Ctrl Pts',(-22.9147684862426,-4.39503346238473,
12.));
#234877=CARTESIAN_POINT('Ctrl Pts',(-22.930371433555,-4.40257451754323,
12.));
#234878=CARTESIAN_POINT('Ctrl Pts',(-22.9460690729093,-4.41021712205553,
12.));
#234879=CARTESIAN_POINT('Ctrl Pts',(-22.9618600534866,-4.41796126001302,
12.));
#234880=CARTESIAN_POINT('Ctrl Pts',(-22.977743046002,-4.42580691372751,
12.));
#234881=CARTESIAN_POINT('Ctrl Pts',(-22.9937167421006,-4.43375406376879,
12.));
#234882=CARTESIAN_POINT('Ctrl Pts',(-23.0097798538395,-4.44180268901643,
12.));
#234883=CARTESIAN_POINT('Ctrl Pts',(-23.0259311131392,-4.44995276669686,
12.));
#234884=CARTESIAN_POINT('Ctrl Pts',(-23.0421692712467,-4.45820427241683,
12.));
#234885=CARTESIAN_POINT('Ctrl Pts',(-23.0584930981732,-4.4665571801823,
12.));
#234886=CARTESIAN_POINT('Ctrl Pts',(-23.0749013821881,-4.47501146242856,
12.));
#234887=CARTESIAN_POINT('Ctrl Pts',(-23.0913929293922,-4.48356709006788,
12.));
#234888=CARTESIAN_POINT('Ctrl Pts',(-23.1079665632636,-4.49222403252216,
12.));
#234889=CARTESIAN_POINT('Ctrl Pts',(-23.1246211242115,-4.50098225775171,
12.));
#234890=CARTESIAN_POINT('Ctrl Pts',(-23.1413554691123,-4.5098417322706,
12.));
#234891=CARTESIAN_POINT('Ctrl Pts',(-23.1581684708761,-4.51880242116748,
12.));
#234892=CARTESIAN_POINT('Ctrl Pts',(-23.1750590180908,-4.52786428815014,
12.));
#234893=CARTESIAN_POINT('Ctrl Pts',(-23.1920260146465,-4.53702729557566,
12.));
#234894=CARTESIAN_POINT('Ctrl Pts',(-23.2090683793629,-4.54629140447544,
12.));
#234895=CARTESIAN_POINT('Ctrl Pts',(-23.2261850456064,-4.55565657456975,
12.));
#234896=CARTESIAN_POINT('Ctrl Pts',(-23.2433749609131,-4.56512276427839,
12.));
#234897=CARTESIAN_POINT('Ctrl Pts',(-23.2606370866866,-4.57468993076097,
12.));
#234898=CARTESIAN_POINT('Ctrl Pts',(-23.2779703978876,-4.5843580299469,
12.));
#234899=CARTESIAN_POINT('Ctrl Pts',(-23.2953738827191,-4.5941270165575,
12.));
#234900=CARTESIAN_POINT('Ctrl Pts',(-23.3128465423115,-4.60399684412163,
12.));
#234901=CARTESIAN_POINT('Ctrl Pts',(-23.3303873903938,-4.6139674649783,
12.));
#234902=CARTESIAN_POINT('Ctrl Pts',(-23.3479954530272,-4.62403883030805,
12.));
#234903=CARTESIAN_POINT('Ctrl Pts',(-23.3656697683489,-4.63421089016541,
12.));
#234904=CARTESIAN_POINT('Ctrl Pts',(-23.3834093863068,-4.6444835934993,
12.));
#234905=CARTESIAN_POINT('Ctrl Pts',(-23.4012133683959,-4.65485688816924,
12.));
#234906=CARTESIAN_POINT('Ctrl Pts',(-23.4190807873803,-4.6653307209467,
12.));
#234907=CARTESIAN_POINT('Ctrl Pts',(-23.4370107270451,-4.67590503753058,
12.));
#234908=CARTESIAN_POINT('Ctrl Pts',(-23.455002281986,-4.68657978258303,
12.));
#234909=CARTESIAN_POINT('Ctrl Pts',(-23.4730545573853,-4.69735489975024,
12.));
#234910=CARTESIAN_POINT('Ctrl Pts',(-23.491166668789,-4.70823033167818,
12.));
#234911=CARTESIAN_POINT('Ctrl Pts',(-23.509337741878,-4.71920602001901,
12.));
#234912=CARTESIAN_POINT('Ctrl Pts',(-23.5275669122372,-4.7302819054303,
12.));
#234913=CARTESIAN_POINT('Ctrl Pts',(-23.545853325171,-4.74145792760698,
12.));
#234914=CARTESIAN_POINT('Ctrl Pts',(-23.5641961355168,-4.75273402530617,
12.));
#234915=CARTESIAN_POINT('Ctrl Pts',(-23.5825945074535,-4.76411013636251,
12.));
#234916=CARTESIAN_POINT('Ctrl Pts',(-23.6010476143099,-4.77558619769872,
12.));
#234917=CARTESIAN_POINT('Ctrl Pts',(-23.6195546383624,-4.78716214532098,
12.));
#234918=CARTESIAN_POINT('Ctrl Pts',(-23.6381147706579,-4.7988379143322,
12.));
#234919=CARTESIAN_POINT('Ctrl Pts',(-23.6567272108628,-4.81061343896432,
12.));
#234920=CARTESIAN_POINT('Ctrl Pts',(-23.675391167102,-4.82248865259562,
12.));
#234921=CARTESIAN_POINT('Ctrl Pts',(-23.6941058557971,-4.83446348776265,
12.));
#234922=CARTESIAN_POINT('Ctrl Pts',(-23.7128705015017,-4.84653787616425,
12.));
#234923=CARTESIAN_POINT('Ctrl Pts',(-23.7316843367313,-4.85871174865499,
12.));
#234924=CARTESIAN_POINT('Ctrl Pts',(-23.7505466018245,-4.87098503527152,
12.));
#234925=CARTESIAN_POINT('Ctrl Pts',(-23.7694565448049,-4.88335766525573,
12.));
#234926=CARTESIAN_POINT('Ctrl Pts',(-23.7884134212384,-4.89582956706775,
12.));
#234927=CARTESIAN_POINT('Ctrl Pts',(-23.8074164940896,-4.90840066839344,
12.));
#234928=CARTESIAN_POINT('Ctrl Pts',(-23.8264650335717,-4.92107089613969,
12.));
#234929=CARTESIAN_POINT('Ctrl Pts',(-23.8455583170057,-4.93384017643432,
12.));
#234930=CARTESIAN_POINT('Ctrl Pts',(-23.8646956287168,-4.9467084346586,
12.));
#234931=CARTESIAN_POINT('Ctrl Pts',(-23.8838762599218,-4.9596755954656,
12.));
#234932=CARTESIAN_POINT('Ctrl Pts',(-23.9030995086163,-4.97274158279226,
12.));
#234933=CARTESIAN_POINT('Ctrl Pts',(-23.9223646794592,-4.98590631986532,
12.));
#234934=CARTESIAN_POINT('Ctrl Pts',(-23.9416710836529,-4.99916972919306,
12.));
#234935=CARTESIAN_POINT('Ctrl Pts',(-23.9610180388271,-5.01253173257453,
12.));
#234936=CARTESIAN_POINT('Ctrl Pts',(-23.9804048689227,-5.02599225112454,
12.));
#234937=CARTESIAN_POINT('Ctrl Pts',(-23.9998309040746,-5.03955120528521,
12.));
#234938=CARTESIAN_POINT('Ctrl Pts',(-24.0192954804896,-5.05320851483065,
12.));
#234939=CARTESIAN_POINT('Ctrl Pts',(-24.0387979403268,-5.06696409886641,
12.));
#234940=CARTESIAN_POINT('Ctrl Pts',(-24.0583376315638,-5.08081787581276,
12.));
#234941=CARTESIAN_POINT('Ctrl Pts',(-24.0779139079266,-5.09476976342625,
12.));
#234942=CARTESIAN_POINT('Ctrl Pts',(-24.0975261288446,-5.10881967883132,
12.));
#234943=CARTESIAN_POINT('Ctrl Pts',(-24.117173659394,-5.12296753853859,
12.));
#234944=CARTESIAN_POINT('Ctrl Pts',(-24.1368558702443,-5.13721325845744,
12.));
#234945=CARTESIAN_POINT('Ctrl Pts',(-24.156572137597,-5.15155675390075,
12.));
#234946=CARTESIAN_POINT('Ctrl Pts',(-24.1763218431343,-5.16599793957979,
12.));
#234947=CARTESIAN_POINT('Ctrl Pts',(-24.1961043738754,-5.18053672961392,
12.));
#234948=CARTESIAN_POINT('Ctrl Pts',(-24.215919122017,-5.19517303753643,
12.));
#234949=CARTESIAN_POINT('Ctrl Pts',(-24.2357654847765,-5.20990677629173,
12.));
#234950=CARTESIAN_POINT('Ctrl Pts',(-24.2556428642294,-5.22473785822441,
12.));
#234951=CARTESIAN_POINT('Ctrl Pts',(-24.2755506671526,-5.23966619506289,
12.));
#234952=CARTESIAN_POINT('Ctrl Pts',(-24.2954883048448,-5.25469169788856,
12.));
#234953=CARTESIAN_POINT('Ctrl Pts',(-24.3154551932222,-5.26981427718796,
12.));
#234954=CARTESIAN_POINT('Ctrl Pts',(-24.3354507529415,-5.28503384290644,
12.));
#234955=CARTESIAN_POINT('Ctrl Pts',(-24.3554744095075,-5.30035030449058,
12.));
#234956=CARTESIAN_POINT('Ctrl Pts',(-24.3755255933917,-5.31576357092524,
12.));
#234957=CARTESIAN_POINT('Ctrl Pts',(-24.3956037401293,-5.33127355076036,
12.));
#234958=CARTESIAN_POINT('Ctrl Pts',(-24.4157082904615,-5.34688015213546,
12.));
#234959=CARTESIAN_POINT('Ctrl Pts',(-24.4358386899152,-5.36258328273639,
12.));
#234960=CARTESIAN_POINT('Ctrl Pts',(-24.4559943883159,-5.37838284973706,
12.));
#234961=CARTESIAN_POINT('Ctrl Pts',(-24.4761748393322,-5.3942787597383,
12.));
#234962=CARTESIAN_POINT('Ctrl Pts',(-24.4963794999831,-5.41027091869242,
12.));
#234963=CARTESIAN_POINT('Ctrl Pts',(-24.5166078302107,-5.42635923183411,
12.));
#234964=CARTESIAN_POINT('Ctrl Pts',(-24.5368592922861,-5.44254360356865,
12.));
#234965=CARTESIAN_POINT('Ctrl Pts',(-24.5571333514841,-5.45882393762244,
12.));
#234966=CARTESIAN_POINT('Ctrl Pts',(-24.5774294770329,-5.47520013724403,
12.));
#234967=CARTESIAN_POINT('Ctrl Pts',(-24.5977471429365,-5.49167210537235,
12.));
#234968=CARTESIAN_POINT('Ctrl Pts',(-24.618085828918,-5.50823974481959,
12.));
#234969=CARTESIAN_POINT('Ctrl Pts',(-24.6384450211466,-5.52490295840996,
12.));
#234970=CARTESIAN_POINT('Ctrl Pts',(-24.6588242134733,-5.54166164919593,
12.));
#234971=CARTESIAN_POINT('Ctrl Pts',(-24.6792229061785,-5.55851572025389,
12.));
#234972=CARTESIAN_POINT('Ctrl Pts',(-24.6996406035507,-5.57546507427766,
12.));
#234973=CARTESIAN_POINT('Ctrl Pts',(-24.7200768119079,-5.59250961323995,
12.));
#234974=CARTESIAN_POINT('Ctrl Pts',(-24.7405310372736,-5.60964923798495,
12.));
#234975=CARTESIAN_POINT('Ctrl Pts',(-24.76100278357,-5.62688384790919,12.));
#234976=CARTESIAN_POINT('Ctrl Pts',(-24.7814915496728,-5.64421334042247,
12.));
#234977=CARTESIAN_POINT('Ctrl Pts',(-24.8019968304618,-5.66163761114903,
12.));
#234978=CARTESIAN_POINT('Ctrl Pts',(-24.822518122386,-5.67915655496524,
12.));
#234979=CARTESIAN_POINT('Ctrl Pts',(-24.8430549277634,-5.69677006679429,
12.));
#234980=CARTESIAN_POINT('Ctrl Pts',(-24.8636067597677,-5.71447804252019,
12.));
#234981=CARTESIAN_POINT('Ctrl Pts',(-24.8841731467219,-5.73228037976926,
12.));
#234982=CARTESIAN_POINT('Ctrl Pts',(-24.9047536376467,-5.75017697890813,
12.));
#234983=CARTESIAN_POINT('Ctrl Pts',(-24.9253478043632,-5.76816774342236,
12.));
#234984=CARTESIAN_POINT('Ctrl Pts',(-24.9459552293308,-5.78625257775703,
12.));
#234985=CARTESIAN_POINT('Ctrl Pts',(-24.9665754954462,-5.80443138549747,
12.));
#234986=CARTESIAN_POINT('Ctrl Pts',(-24.9872081752709,-5.82270406744214,
12.));
#234987=CARTESIAN_POINT('Ctrl Pts',(-25.0078528200558,-5.84107051963073,
12.));
#234988=CARTESIAN_POINT('Ctrl Pts',(-25.0285089498922,-5.8595306315681,
12.));
#234989=CARTESIAN_POINT('Ctrl Pts',(-25.0491760405965,-5.87808428385329,
12.));
#234990=CARTESIAN_POINT('Ctrl Pts',(-25.0698535426593,-5.89673135155459,
12.));
#234991=CARTESIAN_POINT('Ctrl Pts',(-25.0905409050863,-5.91547170844382,
12.));
#234992=CARTESIAN_POINT('Ctrl Pts',(-25.1112375971182,-5.93430523086776,
12.));
#234993=CARTESIAN_POINT('Ctrl Pts',(-25.1319431317273,-5.95323180187348,
12.));
#234994=CARTESIAN_POINT('Ctrl Pts',(-25.1526570863065,-5.97225131495636,
12.));
#234995=CARTESIAN_POINT('Ctrl Pts',(-25.1733791296154,-5.99136367859838,
12.));
#234996=CARTESIAN_POINT('Ctrl Pts',(-25.1941090269638,-6.0105688180476,
12.));
#234997=CARTESIAN_POINT('Ctrl Pts',(-25.2148466201368,-6.02986667390187,
12.));
#234998=CARTESIAN_POINT('Ctrl Pts',(-25.2355918138798,-6.04925720151412,
12.));
#234999=CARTESIAN_POINT('Ctrl Pts',(-25.2521940105523,-6.06484373634696,
12.));
#235000=CARTESIAN_POINT('Ctrl Pts',(-25.2646490489816,-6.07657531787577,
12.));
#235001=CARTESIAN_POINT('Ctrl Pts',(-25.2729539149479,-6.08441489609824,
12.));
#235002=CARTESIAN_POINT('Ctrl Pts',(-25.2771067246846,-6.08833931617698,
12.));
#235003=CARTESIAN_POINT('Ctrl Pts',(-22.4835757167854,-1.76341220531179,
0.));
#235004=CARTESIAN_POINT('Ctrl Pts',(-22.4835757167854,-1.76341220531179,
12.));
#235005=CARTESIAN_POINT('Ctrl Pts',(-22.483581992979,-1.76341415538764,
0.));
#235006=CARTESIAN_POINT('Ctrl Pts',(-22.483581992979,-1.76341415538764,
12.));
#235007=CARTESIAN_POINT('Ctrl Pts',(-22.4836387052232,-1.7634206426357,
0.));
#235008=CARTESIAN_POINT('Ctrl Pts',(-22.4836387052232,-1.7634206426357,
12.));
#235009=CARTESIAN_POINT('Ctrl Pts',(-22.483856251707,-1.76343813434565,
0.));
#235010=CARTESIAN_POINT('Ctrl Pts',(-22.483856251707,-1.76343813434565,
12.));
#235011=CARTESIAN_POINT('Ctrl Pts',(-22.4844112933129,-1.76347698284792,
0.));
#235012=CARTESIAN_POINT('Ctrl Pts',(-22.4844112933129,-1.76347698284792,
12.));
#235013=CARTESIAN_POINT('Ctrl Pts',(-22.4855446605991,-1.76355076045546,
0.));
#235014=CARTESIAN_POINT('Ctrl Pts',(-22.4855446605991,-1.76355076045546,
12.));
#235015=CARTESIAN_POINT('Ctrl Pts',(-22.4871115206571,-1.76364784232963,
0.));
#235016=CARTESIAN_POINT('Ctrl Pts',(-22.4871115206571,-1.76364784232963,
12.));
#235017=CARTESIAN_POINT('Ctrl Pts',(-22.4890991659478,-1.76376424879505,
0.));
#235018=CARTESIAN_POINT('Ctrl Pts',(-22.4890991659478,-1.76376424879505,
12.));
#235019=CARTESIAN_POINT('Ctrl Pts',(-22.4914909094908,-1.76389475965724,
0.));
#235020=CARTESIAN_POINT('Ctrl Pts',(-22.4914909094908,-1.76389475965724,
12.));
#235021=CARTESIAN_POINT('Ctrl Pts',(-22.4942693792449,-1.764033938803,0.));
#235022=CARTESIAN_POINT('Ctrl Pts',(-22.4942693792449,-1.764033938803,12.));
#235023=CARTESIAN_POINT('Ctrl Pts',(-22.4974203063191,-1.76417731243462,
0.));
#235024=CARTESIAN_POINT('Ctrl Pts',(-22.4974203063191,-1.76417731243462,
12.));
#235025=CARTESIAN_POINT('Ctrl Pts',(-22.5009332677316,-1.76432160068725,
0.));
#235026=CARTESIAN_POINT('Ctrl Pts',(-22.5009332677316,-1.76432160068725,
12.));
#235027=CARTESIAN_POINT('Ctrl Pts',(-22.5047996391978,-1.76446408210366,
0.));
#235028=CARTESIAN_POINT('Ctrl Pts',(-22.5047996391978,-1.76446408210366,
12.));
#235029=CARTESIAN_POINT('Ctrl Pts',(-22.5090112700212,-1.76460218257323,
0.));
#235030=CARTESIAN_POINT('Ctrl Pts',(-22.5090112700212,-1.76460218257323,
12.));
#235031=CARTESIAN_POINT('Ctrl Pts',(-22.5135590569554,-1.76473303281159,
0.));
#235032=CARTESIAN_POINT('Ctrl Pts',(-22.5135590569554,-1.76473303281159,
12.));
#235033=CARTESIAN_POINT('Ctrl Pts',(-22.5184336670207,-1.76485369319896,
0.));
#235034=CARTESIAN_POINT('Ctrl Pts',(-22.5184336670207,-1.76485369319896,
12.));
#235035=CARTESIAN_POINT('Ctrl Pts',(-22.5236259635515,-1.76496128643369,
0.));
#235036=CARTESIAN_POINT('Ctrl Pts',(-22.5236259635515,-1.76496128643369,
12.));
#235037=CARTESIAN_POINT('Ctrl Pts',(-22.529127665298,-1.76505320262751,
0.));
#235038=CARTESIAN_POINT('Ctrl Pts',(-22.529127665298,-1.76505320262751,
12.));
#235039=CARTESIAN_POINT('Ctrl Pts',(-22.5349313983571,-1.7651271156325,
0.));
#235040=CARTESIAN_POINT('Ctrl Pts',(-22.5349313983571,-1.7651271156325,
12.));
#235041=CARTESIAN_POINT('Ctrl Pts',(-22.5410303590891,-1.76518087841492,
0.));
#235042=CARTESIAN_POINT('Ctrl Pts',(-22.5410303590891,-1.76518087841492,
12.));
#235043=CARTESIAN_POINT('Ctrl Pts',(-22.5474180954006,-1.76521245524047,
0.));
#235044=CARTESIAN_POINT('Ctrl Pts',(-22.5474180954006,-1.76521245524047,
12.));
#235045=CARTESIAN_POINT('Ctrl Pts',(-22.5540882235837,-1.76521983384063,
0.));
#235046=CARTESIAN_POINT('Ctrl Pts',(-22.5540882235837,-1.76521983384063,
12.));
#235047=CARTESIAN_POINT('Ctrl Pts',(-22.5610344912501,-1.76520104500449,
0.));
#235048=CARTESIAN_POINT('Ctrl Pts',(-22.5610344912501,-1.76520104500449,
12.));
#235049=CARTESIAN_POINT('Ctrl Pts',(-22.5682508499873,-1.76515418518829,
0.));
#235050=CARTESIAN_POINT('Ctrl Pts',(-22.5682508499873,-1.76515418518829,
12.));
#235051=CARTESIAN_POINT('Ctrl Pts',(-22.5757315316355,-1.76507744026747,
0.));
#235052=CARTESIAN_POINT('Ctrl Pts',(-22.5757315316355,-1.76507744026747,
12.));
#235053=CARTESIAN_POINT('Ctrl Pts',(-22.5834711038024,-1.76496910283088,
0.));
#235054=CARTESIAN_POINT('Ctrl Pts',(-22.5834711038024,-1.76496910283088,
12.));
#235055=CARTESIAN_POINT('Ctrl Pts',(-22.5914644078106,-1.76482755288411,
0.));
#235056=CARTESIAN_POINT('Ctrl Pts',(-22.5914644078106,-1.76482755288411,
12.));
#235057=CARTESIAN_POINT('Ctrl Pts',(-22.5997065145638,-1.76465124413556,
0.));
#235058=CARTESIAN_POINT('Ctrl Pts',(-22.5997065145638,-1.76465124413556,
12.));
#235059=CARTESIAN_POINT('Ctrl Pts',(-22.6081926681342,-1.76443868648015,
0.));
#235060=CARTESIAN_POINT('Ctrl Pts',(-22.6081926681342,-1.76443868648015,
12.));
#235061=CARTESIAN_POINT('Ctrl Pts',(-22.6169182517693,-1.76418843543739,
0.));
#235062=CARTESIAN_POINT('Ctrl Pts',(-22.6169182517693,-1.76418843543739,
12.));
#235063=CARTESIAN_POINT('Ctrl Pts',(-22.6258787994847,-1.76389909571402,
0.));
#235064=CARTESIAN_POINT('Ctrl Pts',(-22.6258787994847,-1.76389909571402,
12.));
#235065=CARTESIAN_POINT('Ctrl Pts',(-22.635069997936,-1.76356932176272,
0.));
#235066=CARTESIAN_POINT('Ctrl Pts',(-22.635069997936,-1.76356932176272,
12.));
#235067=CARTESIAN_POINT('Ctrl Pts',(-22.6444876940425,-1.76319782013914,
0.));
#235068=CARTESIAN_POINT('Ctrl Pts',(-22.6444876940425,-1.76319782013914,
12.));
#235069=CARTESIAN_POINT('Ctrl Pts',(-22.6541278938413,-1.76278334912559,
0.));
#235070=CARTESIAN_POINT('Ctrl Pts',(-22.6541278938413,-1.76278334912559,
12.));
#235071=CARTESIAN_POINT('Ctrl Pts',(-22.6639867471756,-1.76232471392567,
0.));
#235072=CARTESIAN_POINT('Ctrl Pts',(-22.6639867471756,-1.76232471392567,
12.));
#235073=CARTESIAN_POINT('Ctrl Pts',(-22.6740605356699,-1.76182076289525,
0.));
#235074=CARTESIAN_POINT('Ctrl Pts',(-22.6740605356699,-1.76182076289525,
12.));
#235075=CARTESIAN_POINT('Ctrl Pts',(-22.6843456585245,-1.76127038310612,
0.));
#235076=CARTESIAN_POINT('Ctrl Pts',(-22.6843456585245,-1.76127038310612,
12.));
#235077=CARTESIAN_POINT('Ctrl Pts',(-22.6948386219843,-1.76067249704884,
0.));
#235078=CARTESIAN_POINT('Ctrl Pts',(-22.6948386219843,-1.76067249704884,
12.));
#235079=CARTESIAN_POINT('Ctrl Pts',(-22.7055360375481,-1.76002606202399,
0.));
#235080=CARTESIAN_POINT('Ctrl Pts',(-22.7055360375481,-1.76002606202399,
12.));
#235081=CARTESIAN_POINT('Ctrl Pts',(-22.7164346186007,-1.75933006905924,
0.));
#235082=CARTESIAN_POINT('Ctrl Pts',(-22.7164346186007,-1.75933006905924,
12.));
#235083=CARTESIAN_POINT('Ctrl Pts',(-22.7275311777305,-1.75858354204635,
0.));
#235084=CARTESIAN_POINT('Ctrl Pts',(-22.7275311777305,-1.75858354204635,
12.));
#235085=CARTESIAN_POINT('Ctrl Pts',(-22.7388226235565,-1.75778553673249,
0.));
#235086=CARTESIAN_POINT('Ctrl Pts',(-22.7388226235565,-1.75778553673249,
12.));
#235087=CARTESIAN_POINT('Ctrl Pts',(-22.7503059556455,-1.75693513908911,
0.));
#235088=CARTESIAN_POINT('Ctrl Pts',(-22.7503059556455,-1.75693513908911,
12.));
#235089=CARTESIAN_POINT('Ctrl Pts',(-22.7619782595013,-1.7560314637164,
0.));
#235090=CARTESIAN_POINT('Ctrl Pts',(-22.7619782595013,-1.7560314637164,
12.));
#235091=CARTESIAN_POINT('Ctrl Pts',(-22.7738367016115,-1.75507365227127,
0.));
#235092=CARTESIAN_POINT('Ctrl Pts',(-22.7738367016115,-1.75507365227127,
12.));
#235093=CARTESIAN_POINT('Ctrl Pts',(-22.7858785242358,-1.75406087182929,
0.));
#235094=CARTESIAN_POINT('Ctrl Pts',(-22.7858785242358,-1.75406087182929,
12.));
#235095=CARTESIAN_POINT('Ctrl Pts',(-22.7981010424312,-1.75299231391461,
0.));
#235096=CARTESIAN_POINT('Ctrl Pts',(-22.7981010424312,-1.75299231391461,
12.));
#235097=CARTESIAN_POINT('Ctrl Pts',(-22.8105016414712,-1.75186719365589,
0.));
#235098=CARTESIAN_POINT('Ctrl Pts',(-22.8105016414712,-1.75186719365589,
12.));
#235099=CARTESIAN_POINT('Ctrl Pts',(-22.8230777741285,-1.75068474890884,
0.));
#235100=CARTESIAN_POINT('Ctrl Pts',(-22.8230777741285,-1.75068474890884,
12.));
#235101=CARTESIAN_POINT('Ctrl Pts',(-22.8358269579854,-1.74944423940117,
0.));
#235102=CARTESIAN_POINT('Ctrl Pts',(-22.8358269579854,-1.74944423940117,
12.));
#235103=CARTESIAN_POINT('Ctrl Pts',(-22.8487467728075,-1.74814494588492,
0.));
#235104=CARTESIAN_POINT('Ctrl Pts',(-22.8487467728075,-1.74814494588492,
12.));
#235105=CARTESIAN_POINT('Ctrl Pts',(-22.8618348580234,-1.74678616930663,
0.));
#235106=CARTESIAN_POINT('Ctrl Pts',(-22.8618348580234,-1.74678616930663,
12.));
#235107=CARTESIAN_POINT('Ctrl Pts',(-22.8750889101696,-1.745367229982,0.));
#235108=CARTESIAN_POINT('Ctrl Pts',(-22.8750889101696,-1.745367229982,12.));
#235109=CARTESIAN_POINT('Ctrl Pts',(-22.8885066803351,-1.74388746677702,
0.));
#235110=CARTESIAN_POINT('Ctrl Pts',(-22.8885066803351,-1.74388746677702,
12.));
#235111=CARTESIAN_POINT('Ctrl Pts',(-22.9020859716144,-1.74234623630079,
0.));
#235112=CARTESIAN_POINT('Ctrl Pts',(-22.9020859716144,-1.74234623630079,
12.));
#235113=CARTESIAN_POINT('Ctrl Pts',(-22.9158246373365,-1.74074291231057,
0.));
#235114=CARTESIAN_POINT('Ctrl Pts',(-22.9158246373365,-1.74074291231057,
12.));
#235115=CARTESIAN_POINT('Ctrl Pts',(-22.9297205792587,-1.73907688511664,
0.));
#235116=CARTESIAN_POINT('Ctrl Pts',(-22.9297205792587,-1.73907688511664,
12.));
#235117=CARTESIAN_POINT('Ctrl Pts',(-22.9437717457825,-1.73734756100038,
0.));
#235118=CARTESIAN_POINT('Ctrl Pts',(-22.9437717457825,-1.73734756100038,
12.));
#235119=CARTESIAN_POINT('Ctrl Pts',(-22.9579761301062,-1.73555436162771,
0.));
#235120=CARTESIAN_POINT('Ctrl Pts',(-22.9579761301062,-1.73555436162771,
12.));
#235121=CARTESIAN_POINT('Ctrl Pts',(-22.9723317685688,-1.73369672350817,
0.));
#235122=CARTESIAN_POINT('Ctrl Pts',(-22.9723317685688,-1.73369672350817,
12.));
#235123=CARTESIAN_POINT('Ctrl Pts',(-22.9868367391978,-1.73177409750193,
0.));
#235124=CARTESIAN_POINT('Ctrl Pts',(-22.9868367391978,-1.73177409750193,
12.));
#235125=CARTESIAN_POINT('Ctrl Pts',(-23.0014891601891,-1.72978594832137,
0.));
#235126=CARTESIAN_POINT('Ctrl Pts',(-23.0014891601891,-1.72978594832137,
12.));
#235127=CARTESIAN_POINT('Ctrl Pts',(-23.0162871884167,-1.72773175404702,
0.));
#235128=CARTESIAN_POINT('Ctrl Pts',(-23.0162871884167,-1.72773175404702,
12.));
#235129=CARTESIAN_POINT('Ctrl Pts',(-23.031229017888,-1.72561100564033,
0.));
#235130=CARTESIAN_POINT('Ctrl Pts',(-23.031229017888,-1.72561100564033,
12.));
#235131=CARTESIAN_POINT('Ctrl Pts',(-23.0463128785528,-1.72342320653731,
0.));
#235132=CARTESIAN_POINT('Ctrl Pts',(-23.0463128785528,-1.72342320653731,
12.));
#235133=CARTESIAN_POINT('Ctrl Pts',(-23.061537035156,-1.7211678722598,0.));
#235134=CARTESIAN_POINT('Ctrl Pts',(-23.061537035156,-1.7211678722598,12.));
#235135=CARTESIAN_POINT('Ctrl Pts',(-23.0768997860709,-1.71884453003027,
0.));
#235136=CARTESIAN_POINT('Ctrl Pts',(-23.0768997860709,-1.71884453003027,
12.));
#235137=CARTESIAN_POINT('Ctrl Pts',(-23.0923994621216,-1.71645271839311,
0.));
#235138=CARTESIAN_POINT('Ctrl Pts',(-23.0923994621216,-1.71645271839311,
12.));
#235139=CARTESIAN_POINT('Ctrl Pts',(-23.1080344254291,-1.71399198684724,
0.));
#235140=CARTESIAN_POINT('Ctrl Pts',(-23.1080344254291,-1.71399198684724,
12.));
#235141=CARTESIAN_POINT('Ctrl Pts',(-23.1238030684929,-1.71146189552192,
0.));
#235142=CARTESIAN_POINT('Ctrl Pts',(-23.1238030684929,-1.71146189552192,
12.));
#235143=CARTESIAN_POINT('Ctrl Pts',(-23.1397038132358,-1.7088620148546,
0.));
#235144=CARTESIAN_POINT('Ctrl Pts',(-23.1397038132358,-1.7088620148546,
12.));
#235145=CARTESIAN_POINT('Ctrl Pts',(-23.1557351100613,-1.70619192527847,
0.));
#235146=CARTESIAN_POINT('Ctrl Pts',(-23.1557351100613,-1.70619192527847,
12.));
#235147=CARTESIAN_POINT('Ctrl Pts',(-23.1718954368749,-1.70345121691259,
0.));
#235148=CARTESIAN_POINT('Ctrl Pts',(-23.1718954368749,-1.70345121691259,
12.));
#235149=CARTESIAN_POINT('Ctrl Pts',(-23.1881832981848,-1.70063948926987,
0.));
#235150=CARTESIAN_POINT('Ctrl Pts',(-23.1881832981848,-1.70063948926987,
12.));
#235151=CARTESIAN_POINT('Ctrl Pts',(-23.2045972243765,-1.69775635099425,
0.));
#235152=CARTESIAN_POINT('Ctrl Pts',(-23.2045972243765,-1.69775635099425,
12.));
#235153=CARTESIAN_POINT('Ctrl Pts',(-23.2211357709374,-1.69480141959945,
0.));
#235154=CARTESIAN_POINT('Ctrl Pts',(-23.2211357709374,-1.69480141959945,
12.));
#235155=CARTESIAN_POINT('Ctrl Pts',(-23.2377975177014,-1.69177432121716,
0.));
#235156=CARTESIAN_POINT('Ctrl Pts',(-23.2377975177014,-1.69177432121716,
12.));
#235157=CARTESIAN_POINT('Ctrl Pts',(-23.2545810680536,-1.6886746903491,
0.));
#235158=CARTESIAN_POINT('Ctrl Pts',(-23.2545810680536,-1.6886746903491,
12.));
#235159=CARTESIAN_POINT('Ctrl Pts',(-23.2714850482245,-1.68550216963275,
0.));
#235160=CARTESIAN_POINT('Ctrl Pts',(-23.2714850482245,-1.68550216963275,
12.));
#235161=CARTESIAN_POINT('Ctrl Pts',(-23.2885081066949,-1.68225640962181,
0.));
#235162=CARTESIAN_POINT('Ctrl Pts',(-23.2885081066949,-1.68225640962181,
12.));
#235163=CARTESIAN_POINT('Ctrl Pts',(-23.3056489135611,-1.67893706857123,
0.));
#235164=CARTESIAN_POINT('Ctrl Pts',(-23.3056489135611,-1.67893706857123,
12.));
#235165=CARTESIAN_POINT('Ctrl Pts',(-23.3229061599145,-1.67554381222987,
0.));
#235166=CARTESIAN_POINT('Ctrl Pts',(-23.3229061599145,-1.67554381222987,
12.));
#235167=CARTESIAN_POINT('Ctrl Pts',(-23.3402785571866,-1.67207631363905,
0.));
#235168=CARTESIAN_POINT('Ctrl Pts',(-23.3402785571866,-1.67207631363905,
12.));
#235169=CARTESIAN_POINT('Ctrl Pts',(-23.3577648365747,-1.66853425293977,
0.));
#235170=CARTESIAN_POINT('Ctrl Pts',(-23.3577648365747,-1.66853425293977,
12.));
#235171=CARTESIAN_POINT('Ctrl Pts',(-23.375363748555,-1.66491731718864,
0.));
#235172=CARTESIAN_POINT('Ctrl Pts',(-23.375363748555,-1.66491731718864,
12.));
#235173=CARTESIAN_POINT('Ctrl Pts',(-23.3930740623622,-1.66122520018008,
0.));
#235174=CARTESIAN_POINT('Ctrl Pts',(-23.3930740623622,-1.66122520018008,
12.));
#235175=CARTESIAN_POINT('Ctrl Pts',(-23.4108945654803,-1.65745760227507,
0.));
#235176=CARTESIAN_POINT('Ctrl Pts',(-23.4108945654803,-1.65745760227507,
12.));
#235177=CARTESIAN_POINT('Ctrl Pts',(-23.4288240631034,-1.6536142302373,
0.));
#235178=CARTESIAN_POINT('Ctrl Pts',(-23.4288240631034,-1.6536142302373,
12.));
#235179=CARTESIAN_POINT('Ctrl Pts',(-23.446861377656,-1.64969479707339,
0.));
#235180=CARTESIAN_POINT('Ctrl Pts',(-23.446861377656,-1.64969479707339,
12.));
#235181=CARTESIAN_POINT('Ctrl Pts',(-23.4650053483919,-1.64569902187608,
0.));
#235182=CARTESIAN_POINT('Ctrl Pts',(-23.4650053483919,-1.64569902187608,
12.));
#235183=CARTESIAN_POINT('Ctrl Pts',(-23.4832548309638,-1.64162662967524,
0.));
#235184=CARTESIAN_POINT('Ctrl Pts',(-23.4832548309638,-1.64162662967524,
12.));
#235185=CARTESIAN_POINT('Ctrl Pts',(-23.5016086970006,-1.63747735129474,
0.));
#235186=CARTESIAN_POINT('Ctrl Pts',(-23.5016086970006,-1.63747735129474,
12.));
#235187=CARTESIAN_POINT('Ctrl Pts',(-23.5200658336624,-1.63325092321731,
0.));
#235188=CARTESIAN_POINT('Ctrl Pts',(-23.5200658336624,-1.63325092321731,
12.));
#235189=CARTESIAN_POINT('Ctrl Pts',(-23.5386251432278,-1.62894708745231,
0.));
#235190=CARTESIAN_POINT('Ctrl Pts',(-23.5386251432278,-1.62894708745231,
12.));
#235191=CARTESIAN_POINT('Ctrl Pts',(-23.5572855427617,-1.62456559140072,
0.));
#235192=CARTESIAN_POINT('Ctrl Pts',(-23.5572855427617,-1.62456559140072,
12.));
#235193=CARTESIAN_POINT('Ctrl Pts',(-23.5760459637608,-1.62010618772869,
0.));
#235194=CARTESIAN_POINT('Ctrl Pts',(-23.5760459637608,-1.62010618772869,
12.));
#235195=CARTESIAN_POINT('Ctrl Pts',(-23.5949053517996,-1.61556863424697,
0.));
#235196=CARTESIAN_POINT('Ctrl Pts',(-23.5949053517996,-1.61556863424697,
12.));
#235197=CARTESIAN_POINT('Ctrl Pts',(-23.6138626661644,-1.61095269379773,
0.));
#235198=CARTESIAN_POINT('Ctrl Pts',(-23.6138626661644,-1.61095269379773,
12.));
#235199=CARTESIAN_POINT('Ctrl Pts',(-23.6329168794916,-1.60625813414666,
0.));
#235200=CARTESIAN_POINT('Ctrl Pts',(-23.6329168794916,-1.60625813414666,
12.));
#235201=CARTESIAN_POINT('Ctrl Pts',(-23.6520669774863,-1.60148472786588,
0.));
#235202=CARTESIAN_POINT('Ctrl Pts',(-23.6520669774863,-1.60148472786588,
12.));
#235203=CARTESIAN_POINT('Ctrl Pts',(-23.6713119586302,-1.59663225222458,
0.));
#235204=CARTESIAN_POINT('Ctrl Pts',(-23.6713119586302,-1.59663225222458,
12.));
#235205=CARTESIAN_POINT('Ctrl Pts',(-23.6906508338833,-1.59170048908631,
0.));
#235206=CARTESIAN_POINT('Ctrl Pts',(-23.6906508338833,-1.59170048908631,
12.));
#235207=CARTESIAN_POINT('Ctrl Pts',(-23.7100826263835,-1.58668922481222,
0.));
#235208=CARTESIAN_POINT('Ctrl Pts',(-23.7100826263835,-1.58668922481222,
12.));
#235209=CARTESIAN_POINT('Ctrl Pts',(-23.7296063711308,-1.58159825017362,
0.));
#235210=CARTESIAN_POINT('Ctrl Pts',(-23.7296063711308,-1.58159825017362,
12.));
#235211=CARTESIAN_POINT('Ctrl Pts',(-23.7492211147369,-1.57642736025251,
0.));
#235212=CARTESIAN_POINT('Ctrl Pts',(-23.7492211147369,-1.57642736025251,
12.));
#235213=CARTESIAN_POINT('Ctrl Pts',(-23.7689259151869,-1.57117635434412,
0.));
#235214=CARTESIAN_POINT('Ctrl Pts',(-23.7689259151869,-1.57117635434412,
12.));
#235215=CARTESIAN_POINT('Ctrl Pts',(-23.788719841588,-1.56584503586844,
0.));
#235216=CARTESIAN_POINT('Ctrl Pts',(-23.788719841588,-1.56584503586844,
12.));
#235217=CARTESIAN_POINT('Ctrl Pts',(-23.8086019739192,-1.56043321228631,
0.));
#235218=CARTESIAN_POINT('Ctrl Pts',(-23.8086019739192,-1.56043321228631,
12.));
#235219=CARTESIAN_POINT('Ctrl Pts',(-23.8285714027631,-1.55494069502628,
0.));
#235220=CARTESIAN_POINT('Ctrl Pts',(-23.8285714027631,-1.55494069502628,
12.));
#235221=CARTESIAN_POINT('Ctrl Pts',(-23.8486272290698,-1.5493672994053,
0.));
#235222=CARTESIAN_POINT('Ctrl Pts',(-23.8486272290698,-1.5493672994053,
12.));
#235223=CARTESIAN_POINT('Ctrl Pts',(-23.8687685639635,-1.54371284453978,
0.));
#235224=CARTESIAN_POINT('Ctrl Pts',(-23.8687685639635,-1.54371284453978,
12.));
#235225=CARTESIAN_POINT('Ctrl Pts',(-23.8889945285313,-1.53797715326748,
0.));
#235226=CARTESIAN_POINT('Ctrl Pts',(-23.8889945285313,-1.53797715326748,
12.));
#235227=CARTESIAN_POINT('Ctrl Pts',(-23.9093042536119,-1.53216005207462,
0.));
#235228=CARTESIAN_POINT('Ctrl Pts',(-23.9093042536119,-1.53216005207462,
12.));
#235229=CARTESIAN_POINT('Ctrl Pts',(-23.9296968795761,-1.52626137103039,
0.));
#235230=CARTESIAN_POINT('Ctrl Pts',(-23.9296968795761,-1.52626137103039,
12.));
#235231=CARTESIAN_POINT('Ctrl Pts',(-23.9501715561038,-1.52028094372806,
0.));
#235232=CARTESIAN_POINT('Ctrl Pts',(-23.9501715561038,-1.52028094372806,
12.));
#235233=CARTESIAN_POINT('Ctrl Pts',(-23.9707274420145,-1.51421860720628,
0.));
#235234=CARTESIAN_POINT('Ctrl Pts',(-23.9707274420145,-1.51421860720628,
12.));
#235235=CARTESIAN_POINT('Ctrl Pts',(-23.991363705093,-1.50807420187702,
0.));
#235236=CARTESIAN_POINT('Ctrl Pts',(-23.991363705093,-1.50807420187702,
12.));
#235237=CARTESIAN_POINT('Ctrl Pts',(-24.0120795219086,-1.50184757146099,
0.));
#235238=CARTESIAN_POINT('Ctrl Pts',(-24.0120795219086,-1.50184757146099,
12.));
#235239=CARTESIAN_POINT('Ctrl Pts',(-24.0328740776331,-1.49553856292798,
0.));
#235240=CARTESIAN_POINT('Ctrl Pts',(-24.0328740776331,-1.49553856292798,
12.));
#235241=CARTESIAN_POINT('Ctrl Pts',(-24.053746565843,-1.48914702644883,
0.));
#235242=CARTESIAN_POINT('Ctrl Pts',(-24.053746565843,-1.48914702644883,
12.));
#235243=CARTESIAN_POINT('Ctrl Pts',(-24.074696188353,-1.4826728153368,0.));
#235244=CARTESIAN_POINT('Ctrl Pts',(-24.074696188353,-1.4826728153368,12.));
#235245=CARTESIAN_POINT('Ctrl Pts',(-24.0957221550782,-1.47611578597741,
0.));
#235246=CARTESIAN_POINT('Ctrl Pts',(-24.0957221550782,-1.47611578597741,
12.));
#235247=CARTESIAN_POINT('Ctrl Pts',(-24.1168236838827,-1.46947579776992,
0.));
#235248=CARTESIAN_POINT('Ctrl Pts',(-24.1168236838827,-1.46947579776992,
12.));
#235249=CARTESIAN_POINT('Ctrl Pts',(-24.1380000004272,-1.46275271307398,
0.));
#235250=CARTESIAN_POINT('Ctrl Pts',(-24.1380000004272,-1.46275271307398,
12.));
#235251=CARTESIAN_POINT('Ctrl Pts',(-24.1592503380105,-1.45594639716314,
0.));
#235252=CARTESIAN_POINT('Ctrl Pts',(-24.1592503380105,-1.45594639716314,
12.));
#235253=CARTESIAN_POINT('Ctrl Pts',(-24.1805739374033,-1.44905671818721,
0.));
#235254=CARTESIAN_POINT('Ctrl Pts',(-24.1805739374033,-1.44905671818721,
12.));
#235255=CARTESIAN_POINT('Ctrl Pts',(-24.2019700467214,-1.44208354711074,
0.));
#235256=CARTESIAN_POINT('Ctrl Pts',(-24.2019700467214,-1.44208354711074,
12.));
#235257=CARTESIAN_POINT('Ctrl Pts',(-24.2234379212978,-1.43502675765502,
0.));
#235258=CARTESIAN_POINT('Ctrl Pts',(-24.2234379212978,-1.43502675765502,
12.));
#235259=CARTESIAN_POINT('Ctrl Pts',(-24.2449768235485,-1.42788622624851,
0.));
#235260=CARTESIAN_POINT('Ctrl Pts',(-24.2449768235485,-1.42788622624851,
12.));
#235261=CARTESIAN_POINT('Ctrl Pts',(-24.2665860228357,-1.42066183198252,
0.));
#235262=CARTESIAN_POINT('Ctrl Pts',(-24.2665860228357,-1.42066183198252,
12.));
#235263=CARTESIAN_POINT('Ctrl Pts',(-24.2882647953214,-1.41335345657685,
0.));
#235264=CARTESIAN_POINT('Ctrl Pts',(-24.2882647953214,-1.41335345657685,
12.));
#235265=CARTESIAN_POINT('Ctrl Pts',(-24.3100124238316,-1.4059609843434,
0.));
#235266=CARTESIAN_POINT('Ctrl Pts',(-24.3100124238316,-1.4059609843434,
12.));
#235267=CARTESIAN_POINT('Ctrl Pts',(-24.3318281977647,-1.3984843021281,
0.));
#235268=CARTESIAN_POINT('Ctrl Pts',(-24.3318281977647,-1.3984843021281,
12.));
#235269=CARTESIAN_POINT('Ctrl Pts',(-24.3537114129877,-1.3909232992639,
0.));
#235270=CARTESIAN_POINT('Ctrl Pts',(-24.3537114129877,-1.3909232992639,
12.));
#235271=CARTESIAN_POINT('Ctrl Pts',(-24.37566137173,-1.38327786752998,0.));
#235272=CARTESIAN_POINT('Ctrl Pts',(-24.37566137173,-1.38327786752998,12.));
#235273=CARTESIAN_POINT('Ctrl Pts',(-24.3976773824731,-1.37554790111607,
0.));
#235274=CARTESIAN_POINT('Ctrl Pts',(-24.3976773824731,-1.37554790111607,
12.));
#235275=CARTESIAN_POINT('Ctrl Pts',(-24.4197587598337,-1.36773329659954,
0.));
#235276=CARTESIAN_POINT('Ctrl Pts',(-24.4197587598337,-1.36773329659954,
12.));
#235277=CARTESIAN_POINT('Ctrl Pts',(-24.4419048244524,-1.35983395290624,
0.));
#235278=CARTESIAN_POINT('Ctrl Pts',(-24.4419048244524,-1.35983395290624,
12.));
#235279=CARTESIAN_POINT('Ctrl Pts',(-24.4641149028894,-1.35184977125644,
0.));
#235280=CARTESIAN_POINT('Ctrl Pts',(-24.4641149028894,-1.35184977125644,
12.));
#235281=CARTESIAN_POINT('Ctrl Pts',(-24.4863883275135,-1.34378065512335,
0.));
#235282=CARTESIAN_POINT('Ctrl Pts',(-24.4863883275135,-1.34378065512335,
12.));
#235283=CARTESIAN_POINT('Ctrl Pts',(-24.5087244363856,-1.33562651019684,
0.));
#235284=CARTESIAN_POINT('Ctrl Pts',(-24.5087244363856,-1.33562651019684,
12.));
#235285=CARTESIAN_POINT('Ctrl Pts',(-24.5311225731434,-1.32738724435326,
0.));
#235286=CARTESIAN_POINT('Ctrl Pts',(-24.5311225731434,-1.32738724435326,
12.));
#235287=CARTESIAN_POINT('Ctrl Pts',(-24.5535820868671,-1.31906276763669,
0.));
#235288=CARTESIAN_POINT('Ctrl Pts',(-24.5535820868671,-1.31906276763669,
12.));
#235289=CARTESIAN_POINT('Ctrl Pts',(-24.576102332018,-1.31065299222023,
0.));
#235290=CARTESIAN_POINT('Ctrl Pts',(-24.576102332018,-1.31065299222023,
12.));
#235291=CARTESIAN_POINT('Ctrl Pts',(-24.5986826684025,-1.30215783236364,
0.));
#235292=CARTESIAN_POINT('Ctrl Pts',(-24.5986826684025,-1.30215783236364,
12.));
#235293=CARTESIAN_POINT('Ctrl Pts',(-24.6213224611228,-1.29357720438107,
0.));
#235294=CARTESIAN_POINT('Ctrl Pts',(-24.6213224611228,-1.29357720438107,
12.));
#235295=CARTESIAN_POINT('Ctrl Pts',(-24.6440210805278,-1.28491102661513,
0.));
#235296=CARTESIAN_POINT('Ctrl Pts',(-24.6440210805278,-1.28491102661513,
12.));
#235297=CARTESIAN_POINT('Ctrl Pts',(-24.666777902156,-1.2761592194164,0.));
#235298=CARTESIAN_POINT('Ctrl Pts',(-24.666777902156,-1.2761592194164,12.));
#235299=CARTESIAN_POINT('Ctrl Pts',(-24.6895923066837,-1.26732170513497,
0.));
#235300=CARTESIAN_POINT('Ctrl Pts',(-24.6895923066837,-1.26732170513497,
12.));
#235301=CARTESIAN_POINT('Ctrl Pts',(-24.7124636797895,-1.25839840807415,
0.));
#235302=CARTESIAN_POINT('Ctrl Pts',(-24.7124636797895,-1.25839840807415,
12.));
#235303=CARTESIAN_POINT('Ctrl Pts',(-24.7353914120012,-1.24938925444323,
0.));
#235304=CARTESIAN_POINT('Ctrl Pts',(-24.7353914120012,-1.24938925444323,
12.));
#235305=CARTESIAN_POINT('Ctrl Pts',(-24.7583748985439,-1.24029417231988,
0.));
#235306=CARTESIAN_POINT('Ctrl Pts',(-24.7583748985439,-1.24029417231988,
12.));
#235307=CARTESIAN_POINT('Ctrl Pts',(-24.78141353918,-1.23111309161843,0.));
#235308=CARTESIAN_POINT('Ctrl Pts',(-24.78141353918,-1.23111309161843,12.));
#235309=CARTESIAN_POINT('Ctrl Pts',(-24.8045067380536,-1.22184594406526,
0.));
#235310=CARTESIAN_POINT('Ctrl Pts',(-24.8045067380536,-1.22184594406526,
12.));
#235311=CARTESIAN_POINT('Ctrl Pts',(-24.8276539035092,-1.21249266318205,
0.));
#235312=CARTESIAN_POINT('Ctrl Pts',(-24.8276539035092,-1.21249266318205,
12.));
#235313=CARTESIAN_POINT('Ctrl Pts',(-24.8508544481973,-1.20305318426015,
0.));
#235314=CARTESIAN_POINT('Ctrl Pts',(-24.8508544481973,-1.20305318426015,
12.));
#235315=CARTESIAN_POINT('Ctrl Pts',(-24.8741077892074,-1.19352744434059,
0.));
#235316=CARTESIAN_POINT('Ctrl Pts',(-24.8741077892074,-1.19352744434059,
12.));
#235317=CARTESIAN_POINT('Ctrl Pts',(-24.8974133481829,-1.18391538220098,
0.));
#235318=CARTESIAN_POINT('Ctrl Pts',(-24.8974133481829,-1.18391538220098,
12.));
#235319=CARTESIAN_POINT('Ctrl Pts',(-24.9207705514449,-1.17421693835039,
0.));
#235320=CARTESIAN_POINT('Ctrl Pts',(-24.9207705514449,-1.17421693835039,
12.));
#235321=CARTESIAN_POINT('Ctrl Pts',(-24.9441788300932,-1.16443205502852,
0.));
#235322=CARTESIAN_POINT('Ctrl Pts',(-24.9441788300932,-1.16443205502852,
12.));
#235323=CARTESIAN_POINT('Ctrl Pts',(-24.9676376201501,-1.15456067621894,
0.));
#235324=CARTESIAN_POINT('Ctrl Pts',(-24.9676376201501,-1.15456067621894,
12.));
#235325=CARTESIAN_POINT('Ctrl Pts',(-24.9911463621431,-1.14460274758206,
0.));
#235326=CARTESIAN_POINT('Ctrl Pts',(-24.9911463621431,-1.14460274758206,
12.));
#235327=CARTESIAN_POINT('Ctrl Pts',(-25.0147045006193,-1.13455821638535,
0.));
#235328=CARTESIAN_POINT('Ctrl Pts',(-25.0147045006193,-1.13455821638535,
12.));
#235329=CARTESIAN_POINT('Ctrl Pts',(-25.0383114836898,-1.12442703144455,
0.));
#235330=CARTESIAN_POINT('Ctrl Pts',(-25.0383114836898,-1.12442703144455,
12.));
#235331=CARTESIAN_POINT('Ctrl Pts',(-25.0619667625336,-1.1142091430689,
0.));
#235332=CARTESIAN_POINT('Ctrl Pts',(-25.0619667625336,-1.1142091430689,
12.));
#235333=CARTESIAN_POINT('Ctrl Pts',(-25.085669790968,-1.1039045030174,0.));
#235334=CARTESIAN_POINT('Ctrl Pts',(-25.085669790968,-1.1039045030174,12.));
#235335=CARTESIAN_POINT('Ctrl Pts',(-25.1094200248448,-1.09351306445299,
0.));
#235336=CARTESIAN_POINT('Ctrl Pts',(-25.1094200248448,-1.09351306445299,
12.));
#235337=CARTESIAN_POINT('Ctrl Pts',(-25.1332169227415,-1.08303478197174,
0.));
#235338=CARTESIAN_POINT('Ctrl Pts',(-25.1332169227415,-1.08303478197174,
12.));
#235339=CARTESIAN_POINT('Ctrl Pts',(-25.1570599469311,-1.0724696116546,
0.));
#235340=CARTESIAN_POINT('Ctrl Pts',(-25.1570599469311,-1.0724696116546,
12.));
#235341=CARTESIAN_POINT('Ctrl Pts',(-25.1809485642191,-1.06181751111754,
0.));
#235342=CARTESIAN_POINT('Ctrl Pts',(-25.1809485642191,-1.06181751111754,
12.));
#235343=CARTESIAN_POINT('Ctrl Pts',(-25.2048822469027,-1.05107843957925,
0.));
#235344=CARTESIAN_POINT('Ctrl Pts',(-25.2048822469027,-1.05107843957925,
12.));
#235345=CARTESIAN_POINT('Ctrl Pts',(-25.2288604735087,-1.04025235791515,
0.));
#235346=CARTESIAN_POINT('Ctrl Pts',(-25.2288604735087,-1.04025235791515,
12.));
#235347=CARTESIAN_POINT('Ctrl Pts',(-25.2528827300427,-1.0293392287683,
0.));
#235348=CARTESIAN_POINT('Ctrl Pts',(-25.2528827300427,-1.0293392287683,
12.));
#235349=CARTESIAN_POINT('Ctrl Pts',(-25.2769485087268,-1.01833901642272,
0.));
#235350=CARTESIAN_POINT('Ctrl Pts',(-25.2769485087268,-1.01833901642272,
12.));
#235351=CARTESIAN_POINT('Ctrl Pts',(-25.3010573055557,-1.00725168656933,
0.));
#235352=CARTESIAN_POINT('Ctrl Pts',(-25.3010573055557,-1.00725168656933,
12.));
#235353=CARTESIAN_POINT('Ctrl Pts',(-25.3252086182976,-0.996077206120919,
0.));
#235354=CARTESIAN_POINT('Ctrl Pts',(-25.3252086182976,-0.996077206120919,
12.));
#235355=CARTESIAN_POINT('Ctrl Pts',(-25.3494019441444,-0.984815543004089,
0.));
#235356=CARTESIAN_POINT('Ctrl Pts',(-25.3494019441444,-0.984815543004089,
12.));
#235357=CARTESIAN_POINT('Ctrl Pts',(-25.3736367778842,-0.973466666000048,
0.));
#235358=CARTESIAN_POINT('Ctrl Pts',(-25.3736367778842,-0.973466666000048,
12.));
#235359=CARTESIAN_POINT('Ctrl Pts',(-25.3979126089155,-0.962030544502802,
0.));
#235360=CARTESIAN_POINT('Ctrl Pts',(-25.3979126089155,-0.962030544502802,
12.));
#235361=CARTESIAN_POINT('Ctrl Pts',(-25.4222289223155,-0.950507148596968,
0.));
#235362=CARTESIAN_POINT('Ctrl Pts',(-25.4222289223155,-0.950507148596968,
12.));
#235363=CARTESIAN_POINT('Ctrl Pts',(-25.4465852044835,-0.938896449495632,
0.));
#235364=CARTESIAN_POINT('Ctrl Pts',(-25.4465852044835,-0.938896449495632,
12.));
#235365=CARTESIAN_POINT('Ctrl Pts',(-25.4709809474996,-0.927198419885604,
0.));
#235366=CARTESIAN_POINT('Ctrl Pts',(-25.4709809474996,-0.927198419885604,
12.));
#235367=CARTESIAN_POINT('Ctrl Pts',(-25.4954156541787,-0.915413034335333,
0.));
#235368=CARTESIAN_POINT('Ctrl Pts',(-25.4954156541787,-0.915413034335333,
12.));
#235369=CARTESIAN_POINT('Ctrl Pts',(-25.5198888424195,-0.903540269651154,
0.));
#235370=CARTESIAN_POINT('Ctrl Pts',(-25.5198888424195,-0.903540269651154,
12.));
#235371=CARTESIAN_POINT('Ctrl Pts',(-25.5444000508223,-0.891580105349467,
0.));
#235372=CARTESIAN_POINT('Ctrl Pts',(-25.5444000508223,-0.891580105349467,
12.));
#235373=CARTESIAN_POINT('Ctrl Pts',(-25.568948840818,-0.87953252383509,
0.));
#235374=CARTESIAN_POINT('Ctrl Pts',(-25.568948840818,-0.87953252383509,
12.));
#235375=CARTESIAN_POINT('Ctrl Pts',(-25.5935347843616,-0.86739750933947,
0.));
#235376=CARTESIAN_POINT('Ctrl Pts',(-25.5935347843616,-0.86739750933947,
12.));
#235377=CARTESIAN_POINT('Ctrl Pts',(-25.618157453608,-0.855175047037614,
0.));
#235378=CARTESIAN_POINT('Ctrl Pts',(-25.618157453608,-0.855175047037614,
12.));
#235379=CARTESIAN_POINT('Ctrl Pts',(-25.6428164100078,-0.842865122121544,
0.));
#235380=CARTESIAN_POINT('Ctrl Pts',(-25.6428164100078,-0.842865122121544,
12.));
#235381=CARTESIAN_POINT('Ctrl Pts',(-25.6675111931957,-0.830467718864367,
0.));
#235382=CARTESIAN_POINT('Ctrl Pts',(-25.6675111931957,-0.830467718864367,
12.));
#235383=CARTESIAN_POINT('Ctrl Pts',(-25.6922413110172,-0.817982819786719,
0.));
#235384=CARTESIAN_POINT('Ctrl Pts',(-25.6922413110172,-0.817982819786719,
12.));
#235385=CARTESIAN_POINT('Ctrl Pts',(-25.7170062262474,-0.805410404552594,
0.));
#235386=CARTESIAN_POINT('Ctrl Pts',(-25.7170062262474,-0.805410404552594,
12.));
#235387=CARTESIAN_POINT('Ctrl Pts',(-25.7418053757671,-0.792750451613534,
0.));
#235388=CARTESIAN_POINT('Ctrl Pts',(-25.7418053757671,-0.792750451613534,
12.));
#235389=CARTESIAN_POINT('Ctrl Pts',(-25.7666381946871,-0.780002940289025,
0.));
#235390=CARTESIAN_POINT('Ctrl Pts',(-25.7666381946871,-0.780002940289025,
12.));
#235391=CARTESIAN_POINT('Ctrl Pts',(-25.7915041383304,-0.767167852648639,
0.));
#235392=CARTESIAN_POINT('Ctrl Pts',(-25.7915041383304,-0.767167852648639,
12.));
#235393=CARTESIAN_POINT('Ctrl Pts',(-25.816402705995,-0.754245175608288,
0.));
#235394=CARTESIAN_POINT('Ctrl Pts',(-25.816402705995,-0.754245175608288,
12.));
#235395=CARTESIAN_POINT('Ctrl Pts',(-25.841333461908,-0.741234902664697,
0.));
#235396=CARTESIAN_POINT('Ctrl Pts',(-25.841333461908,-0.741234902664697,
12.));
#235397=CARTESIAN_POINT('Ctrl Pts',(-25.8662960624285,-0.728137036485877,
0.));
#235398=CARTESIAN_POINT('Ctrl Pts',(-25.8662960624285,-0.728137036485877,
12.));
#235399=CARTESIAN_POINT('Ctrl Pts',(-25.8912902615141,-0.714951588533753,
0.));
#235400=CARTESIAN_POINT('Ctrl Pts',(-25.8912902615141,-0.714951588533753,
12.));
#235401=CARTESIAN_POINT('Ctrl Pts',(-25.9163158909645,-0.701678575236602,
0.));
#235402=CARTESIAN_POINT('Ctrl Pts',(-25.9163158909645,-0.701678575236602,
12.));
#235403=CARTESIAN_POINT('Ctrl Pts',(-25.941372847213,-0.688318015065678,
0.));
#235404=CARTESIAN_POINT('Ctrl Pts',(-25.941372847213,-0.688318015065678,
12.));
#235405=CARTESIAN_POINT('Ctrl Pts',(-25.9614434298092,-0.677559543215902,
0.));
#235406=CARTESIAN_POINT('Ctrl Pts',(-25.9614434298092,-0.677559543215902,
12.));
#235407=CARTESIAN_POINT('Ctrl Pts',(-25.9765104298171,-0.669451306784415,
0.));
#235408=CARTESIAN_POINT('Ctrl Pts',(-25.9765104298171,-0.669451306784415,
12.));
#235409=CARTESIAN_POINT('Ctrl Pts',(-25.9865613464809,-0.664028313188912,
0.));
#235410=CARTESIAN_POINT('Ctrl Pts',(-25.9865613464809,-0.664028313188912,
12.));
#235411=CARTESIAN_POINT('Ctrl Pts',(-25.991588367311,-0.661312440730891,
0.));
#235412=CARTESIAN_POINT('Ctrl Pts',(-25.991588367311,-0.661312440730891,
12.));
#235413=CARTESIAN_POINT('',(-25.991588367311,-0.661312440730891,0.));
#235414=CARTESIAN_POINT('Ctrl Pts',(-22.4835757167854,-1.76341220531179,
0.));
#235415=CARTESIAN_POINT('Ctrl Pts',(-22.483581992979,-1.76341415538764,
0.));
#235416=CARTESIAN_POINT('Ctrl Pts',(-22.4836387052232,-1.7634206426357,
0.));
#235417=CARTESIAN_POINT('Ctrl Pts',(-22.483856251707,-1.76343813434565,
0.));
#235418=CARTESIAN_POINT('Ctrl Pts',(-22.4844112933129,-1.76347698284792,
0.));
#235419=CARTESIAN_POINT('Ctrl Pts',(-22.4855446605991,-1.76355076045546,
0.));
#235420=CARTESIAN_POINT('Ctrl Pts',(-22.4871115206571,-1.76364784232963,
0.));
#235421=CARTESIAN_POINT('Ctrl Pts',(-22.4890991659478,-1.76376424879505,
0.));
#235422=CARTESIAN_POINT('Ctrl Pts',(-22.4914909094908,-1.76389475965724,
0.));
#235423=CARTESIAN_POINT('Ctrl Pts',(-22.4942693792449,-1.764033938803,0.));
#235424=CARTESIAN_POINT('Ctrl Pts',(-22.4974203063191,-1.76417731243462,
0.));
#235425=CARTESIAN_POINT('Ctrl Pts',(-22.5009332677316,-1.76432160068725,
0.));
#235426=CARTESIAN_POINT('Ctrl Pts',(-22.5047996391978,-1.76446408210366,
0.));
#235427=CARTESIAN_POINT('Ctrl Pts',(-22.5090112700212,-1.76460218257323,
0.));
#235428=CARTESIAN_POINT('Ctrl Pts',(-22.5135590569554,-1.76473303281159,
0.));
#235429=CARTESIAN_POINT('Ctrl Pts',(-22.5184336670207,-1.76485369319896,
0.));
#235430=CARTESIAN_POINT('Ctrl Pts',(-22.5236259635515,-1.76496128643369,
0.));
#235431=CARTESIAN_POINT('Ctrl Pts',(-22.529127665298,-1.76505320262751,
0.));
#235432=CARTESIAN_POINT('Ctrl Pts',(-22.5349313983571,-1.7651271156325,
0.));
#235433=CARTESIAN_POINT('Ctrl Pts',(-22.5410303590891,-1.76518087841492,
0.));
#235434=CARTESIAN_POINT('Ctrl Pts',(-22.5474180954006,-1.76521245524047,
0.));
#235435=CARTESIAN_POINT('Ctrl Pts',(-22.5540882235837,-1.76521983384063,
0.));
#235436=CARTESIAN_POINT('Ctrl Pts',(-22.5610344912501,-1.76520104500449,
0.));
#235437=CARTESIAN_POINT('Ctrl Pts',(-22.5682508499873,-1.76515418518829,
0.));
#235438=CARTESIAN_POINT('Ctrl Pts',(-22.5757315316355,-1.76507744026747,
0.));
#235439=CARTESIAN_POINT('Ctrl Pts',(-22.5834711038024,-1.76496910283088,
0.));
#235440=CARTESIAN_POINT('Ctrl Pts',(-22.5914644078106,-1.76482755288411,
0.));
#235441=CARTESIAN_POINT('Ctrl Pts',(-22.5997065145638,-1.76465124413556,
0.));
#235442=CARTESIAN_POINT('Ctrl Pts',(-22.6081926681342,-1.76443868648015,
0.));
#235443=CARTESIAN_POINT('Ctrl Pts',(-22.6169182517693,-1.76418843543739,
0.));
#235444=CARTESIAN_POINT('Ctrl Pts',(-22.6258787994847,-1.76389909571402,
0.));
#235445=CARTESIAN_POINT('Ctrl Pts',(-22.635069997936,-1.76356932176272,
0.));
#235446=CARTESIAN_POINT('Ctrl Pts',(-22.6444876940425,-1.76319782013914,
0.));
#235447=CARTESIAN_POINT('Ctrl Pts',(-22.6541278938413,-1.76278334912559,
0.));
#235448=CARTESIAN_POINT('Ctrl Pts',(-22.6639867471756,-1.76232471392567,
0.));
#235449=CARTESIAN_POINT('Ctrl Pts',(-22.6740605356699,-1.76182076289525,
0.));
#235450=CARTESIAN_POINT('Ctrl Pts',(-22.6843456585245,-1.76127038310612,
0.));
#235451=CARTESIAN_POINT('Ctrl Pts',(-22.6948386219843,-1.76067249704884,
0.));
#235452=CARTESIAN_POINT('Ctrl Pts',(-22.7055360375481,-1.76002606202399,
0.));
#235453=CARTESIAN_POINT('Ctrl Pts',(-22.7164346186007,-1.75933006905924,
0.));
#235454=CARTESIAN_POINT('Ctrl Pts',(-22.7275311777305,-1.75858354204635,
0.));
#235455=CARTESIAN_POINT('Ctrl Pts',(-22.7388226235565,-1.75778553673249,
0.));
#235456=CARTESIAN_POINT('Ctrl Pts',(-22.7503059556455,-1.75693513908911,
0.));
#235457=CARTESIAN_POINT('Ctrl Pts',(-22.7619782595013,-1.7560314637164,
0.));
#235458=CARTESIAN_POINT('Ctrl Pts',(-22.7738367016115,-1.75507365227127,
0.));
#235459=CARTESIAN_POINT('Ctrl Pts',(-22.7858785242358,-1.75406087182929,
0.));
#235460=CARTESIAN_POINT('Ctrl Pts',(-22.7981010424312,-1.75299231391461,
0.));
#235461=CARTESIAN_POINT('Ctrl Pts',(-22.8105016414712,-1.75186719365589,
0.));
#235462=CARTESIAN_POINT('Ctrl Pts',(-22.8230777741285,-1.75068474890884,
0.));
#235463=CARTESIAN_POINT('Ctrl Pts',(-22.8358269579854,-1.74944423940117,
0.));
#235464=CARTESIAN_POINT('Ctrl Pts',(-22.8487467728075,-1.74814494588492,
0.));
#235465=CARTESIAN_POINT('Ctrl Pts',(-22.8618348580234,-1.74678616930663,
0.));
#235466=CARTESIAN_POINT('Ctrl Pts',(-22.8750889101696,-1.745367229982,0.));
#235467=CARTESIAN_POINT('Ctrl Pts',(-22.8885066803351,-1.74388746677702,
0.));
#235468=CARTESIAN_POINT('Ctrl Pts',(-22.9020859716144,-1.74234623630079,
0.));
#235469=CARTESIAN_POINT('Ctrl Pts',(-22.9158246373365,-1.74074291231057,
0.));
#235470=CARTESIAN_POINT('Ctrl Pts',(-22.9297205792587,-1.73907688511664,
0.));
#235471=CARTESIAN_POINT('Ctrl Pts',(-22.9437717457825,-1.73734756100038,
0.));
#235472=CARTESIAN_POINT('Ctrl Pts',(-22.9579761301062,-1.73555436162771,
0.));
#235473=CARTESIAN_POINT('Ctrl Pts',(-22.9723317685688,-1.73369672350817,
0.));
#235474=CARTESIAN_POINT('Ctrl Pts',(-22.9868367391978,-1.73177409750193,
0.));
#235475=CARTESIAN_POINT('Ctrl Pts',(-23.0014891601891,-1.72978594832137,
0.));
#235476=CARTESIAN_POINT('Ctrl Pts',(-23.0162871884167,-1.72773175404702,
0.));
#235477=CARTESIAN_POINT('Ctrl Pts',(-23.031229017888,-1.72561100564033,
0.));
#235478=CARTESIAN_POINT('Ctrl Pts',(-23.0463128785528,-1.72342320653731,
0.));
#235479=CARTESIAN_POINT('Ctrl Pts',(-23.061537035156,-1.7211678722598,0.));
#235480=CARTESIAN_POINT('Ctrl Pts',(-23.0768997860709,-1.71884453003027,
0.));
#235481=CARTESIAN_POINT('Ctrl Pts',(-23.0923994621216,-1.71645271839311,
0.));
#235482=CARTESIAN_POINT('Ctrl Pts',(-23.1080344254291,-1.71399198684724,
0.));
#235483=CARTESIAN_POINT('Ctrl Pts',(-23.1238030684929,-1.71146189552192,
0.));
#235484=CARTESIAN_POINT('Ctrl Pts',(-23.1397038132358,-1.7088620148546,
0.));
#235485=CARTESIAN_POINT('Ctrl Pts',(-23.1557351100613,-1.70619192527847,
0.));
#235486=CARTESIAN_POINT('Ctrl Pts',(-23.1718954368749,-1.70345121691259,
0.));
#235487=CARTESIAN_POINT('Ctrl Pts',(-23.1881832981848,-1.70063948926987,
0.));
#235488=CARTESIAN_POINT('Ctrl Pts',(-23.2045972243765,-1.69775635099425,
0.));
#235489=CARTESIAN_POINT('Ctrl Pts',(-23.2211357709374,-1.69480141959945,
0.));
#235490=CARTESIAN_POINT('Ctrl Pts',(-23.2377975177014,-1.69177432121716,
0.));
#235491=CARTESIAN_POINT('Ctrl Pts',(-23.2545810680536,-1.6886746903491,
0.));
#235492=CARTESIAN_POINT('Ctrl Pts',(-23.2714850482245,-1.68550216963275,
0.));
#235493=CARTESIAN_POINT('Ctrl Pts',(-23.2885081066949,-1.68225640962181,
0.));
#235494=CARTESIAN_POINT('Ctrl Pts',(-23.3056489135611,-1.67893706857123,
0.));
#235495=CARTESIAN_POINT('Ctrl Pts',(-23.3229061599145,-1.67554381222987,
0.));
#235496=CARTESIAN_POINT('Ctrl Pts',(-23.3402785571866,-1.67207631363905,
0.));
#235497=CARTESIAN_POINT('Ctrl Pts',(-23.3577648365747,-1.66853425293977,
0.));
#235498=CARTESIAN_POINT('Ctrl Pts',(-23.375363748555,-1.66491731718864,
0.));
#235499=CARTESIAN_POINT('Ctrl Pts',(-23.3930740623622,-1.66122520018008,
0.));
#235500=CARTESIAN_POINT('Ctrl Pts',(-23.4108945654803,-1.65745760227507,
0.));
#235501=CARTESIAN_POINT('Ctrl Pts',(-23.4288240631034,-1.6536142302373,
0.));
#235502=CARTESIAN_POINT('Ctrl Pts',(-23.446861377656,-1.64969479707339,
0.));
#235503=CARTESIAN_POINT('Ctrl Pts',(-23.4650053483919,-1.64569902187608,
0.));
#235504=CARTESIAN_POINT('Ctrl Pts',(-23.4832548309638,-1.64162662967524,
0.));
#235505=CARTESIAN_POINT('Ctrl Pts',(-23.5016086970006,-1.63747735129474,
0.));
#235506=CARTESIAN_POINT('Ctrl Pts',(-23.5200658336624,-1.63325092321731,
0.));
#235507=CARTESIAN_POINT('Ctrl Pts',(-23.5386251432278,-1.62894708745231,
0.));
#235508=CARTESIAN_POINT('Ctrl Pts',(-23.5572855427617,-1.62456559140072,
0.));
#235509=CARTESIAN_POINT('Ctrl Pts',(-23.5760459637608,-1.62010618772869,
0.));
#235510=CARTESIAN_POINT('Ctrl Pts',(-23.5949053517996,-1.61556863424697,
0.));
#235511=CARTESIAN_POINT('Ctrl Pts',(-23.6138626661644,-1.61095269379773,
0.));
#235512=CARTESIAN_POINT('Ctrl Pts',(-23.6329168794916,-1.60625813414666,
0.));
#235513=CARTESIAN_POINT('Ctrl Pts',(-23.6520669774863,-1.60148472786588,
0.));
#235514=CARTESIAN_POINT('Ctrl Pts',(-23.6713119586302,-1.59663225222458,
0.));
#235515=CARTESIAN_POINT('Ctrl Pts',(-23.6906508338833,-1.59170048908631,
0.));
#235516=CARTESIAN_POINT('Ctrl Pts',(-23.7100826263835,-1.58668922481222,
0.));
#235517=CARTESIAN_POINT('Ctrl Pts',(-23.7296063711308,-1.58159825017362,
0.));
#235518=CARTESIAN_POINT('Ctrl Pts',(-23.7492211147369,-1.57642736025251,
0.));
#235519=CARTESIAN_POINT('Ctrl Pts',(-23.7689259151869,-1.57117635434412,
0.));
#235520=CARTESIAN_POINT('Ctrl Pts',(-23.788719841588,-1.56584503586844,
0.));
#235521=CARTESIAN_POINT('Ctrl Pts',(-23.8086019739192,-1.56043321228631,
0.));
#235522=CARTESIAN_POINT('Ctrl Pts',(-23.8285714027631,-1.55494069502628,
0.));
#235523=CARTESIAN_POINT('Ctrl Pts',(-23.8486272290698,-1.5493672994053,
0.));
#235524=CARTESIAN_POINT('Ctrl Pts',(-23.8687685639635,-1.54371284453978,
0.));
#235525=CARTESIAN_POINT('Ctrl Pts',(-23.8889945285313,-1.53797715326748,
0.));
#235526=CARTESIAN_POINT('Ctrl Pts',(-23.9093042536119,-1.53216005207462,
0.));
#235527=CARTESIAN_POINT('Ctrl Pts',(-23.9296968795761,-1.52626137103039,
0.));
#235528=CARTESIAN_POINT('Ctrl Pts',(-23.9501715561038,-1.52028094372806,
0.));
#235529=CARTESIAN_POINT('Ctrl Pts',(-23.9707274420145,-1.51421860720628,
0.));
#235530=CARTESIAN_POINT('Ctrl Pts',(-23.991363705093,-1.50807420187702,
0.));
#235531=CARTESIAN_POINT('Ctrl Pts',(-24.0120795219086,-1.50184757146099,
0.));
#235532=CARTESIAN_POINT('Ctrl Pts',(-24.0328740776331,-1.49553856292798,
0.));
#235533=CARTESIAN_POINT('Ctrl Pts',(-24.053746565843,-1.48914702644883,
0.));
#235534=CARTESIAN_POINT('Ctrl Pts',(-24.074696188353,-1.4826728153368,0.));
#235535=CARTESIAN_POINT('Ctrl Pts',(-24.0957221550782,-1.47611578597741,
0.));
#235536=CARTESIAN_POINT('Ctrl Pts',(-24.1168236838827,-1.46947579776992,
0.));
#235537=CARTESIAN_POINT('Ctrl Pts',(-24.1380000004272,-1.46275271307398,
0.));
#235538=CARTESIAN_POINT('Ctrl Pts',(-24.1592503380105,-1.45594639716314,
0.));
#235539=CARTESIAN_POINT('Ctrl Pts',(-24.1805739374033,-1.44905671818721,
0.));
#235540=CARTESIAN_POINT('Ctrl Pts',(-24.2019700467214,-1.44208354711074,
0.));
#235541=CARTESIAN_POINT('Ctrl Pts',(-24.2234379212978,-1.43502675765502,
0.));
#235542=CARTESIAN_POINT('Ctrl Pts',(-24.2449768235485,-1.42788622624851,
0.));
#235543=CARTESIAN_POINT('Ctrl Pts',(-24.2665860228357,-1.42066183198252,
0.));
#235544=CARTESIAN_POINT('Ctrl Pts',(-24.2882647953214,-1.41335345657685,
0.));
#235545=CARTESIAN_POINT('Ctrl Pts',(-24.3100124238316,-1.4059609843434,
0.));
#235546=CARTESIAN_POINT('Ctrl Pts',(-24.3318281977647,-1.3984843021281,
0.));
#235547=CARTESIAN_POINT('Ctrl Pts',(-24.3537114129877,-1.3909232992639,
0.));
#235548=CARTESIAN_POINT('Ctrl Pts',(-24.37566137173,-1.38327786752998,0.));
#235549=CARTESIAN_POINT('Ctrl Pts',(-24.3976773824731,-1.37554790111607,
0.));
#235550=CARTESIAN_POINT('Ctrl Pts',(-24.4197587598337,-1.36773329659954,
0.));
#235551=CARTESIAN_POINT('Ctrl Pts',(-24.4419048244524,-1.35983395290624,
0.));
#235552=CARTESIAN_POINT('Ctrl Pts',(-24.4641149028894,-1.35184977125644,
0.));
#235553=CARTESIAN_POINT('Ctrl Pts',(-24.4863883275135,-1.34378065512335,
0.));
#235554=CARTESIAN_POINT('Ctrl Pts',(-24.5087244363856,-1.33562651019684,
0.));
#235555=CARTESIAN_POINT('Ctrl Pts',(-24.5311225731434,-1.32738724435326,
0.));
#235556=CARTESIAN_POINT('Ctrl Pts',(-24.5535820868671,-1.31906276763669,
0.));
#235557=CARTESIAN_POINT('Ctrl Pts',(-24.576102332018,-1.31065299222023,
0.));
#235558=CARTESIAN_POINT('Ctrl Pts',(-24.5986826684025,-1.30215783236364,
0.));
#235559=CARTESIAN_POINT('Ctrl Pts',(-24.6213224611228,-1.29357720438107,
0.));
#235560=CARTESIAN_POINT('Ctrl Pts',(-24.6440210805278,-1.28491102661513,
0.));
#235561=CARTESIAN_POINT('Ctrl Pts',(-24.666777902156,-1.2761592194164,0.));
#235562=CARTESIAN_POINT('Ctrl Pts',(-24.6895923066837,-1.26732170513497,
0.));
#235563=CARTESIAN_POINT('Ctrl Pts',(-24.7124636797895,-1.25839840807415,
0.));
#235564=CARTESIAN_POINT('Ctrl Pts',(-24.7353914120012,-1.24938925444323,
0.));
#235565=CARTESIAN_POINT('Ctrl Pts',(-24.7583748985439,-1.24029417231988,
0.));
#235566=CARTESIAN_POINT('Ctrl Pts',(-24.78141353918,-1.23111309161843,0.));
#235567=CARTESIAN_POINT('Ctrl Pts',(-24.8045067380536,-1.22184594406526,
0.));
#235568=CARTESIAN_POINT('Ctrl Pts',(-24.8276539035092,-1.21249266318205,
0.));
#235569=CARTESIAN_POINT('Ctrl Pts',(-24.8508544481973,-1.20305318426015,
0.));
#235570=CARTESIAN_POINT('Ctrl Pts',(-24.8741077892074,-1.19352744434059,
0.));
#235571=CARTESIAN_POINT('Ctrl Pts',(-24.8974133481829,-1.18391538220098,
0.));
#235572=CARTESIAN_POINT('Ctrl Pts',(-24.9207705514449,-1.17421693835039,
0.));
#235573=CARTESIAN_POINT('Ctrl Pts',(-24.9441788300932,-1.16443205502852,
0.));
#235574=CARTESIAN_POINT('Ctrl Pts',(-24.9676376201501,-1.15456067621894,
0.));
#235575=CARTESIAN_POINT('Ctrl Pts',(-24.9911463621431,-1.14460274758206,
0.));
#235576=CARTESIAN_POINT('Ctrl Pts',(-25.0147045006193,-1.13455821638535,
0.));
#235577=CARTESIAN_POINT('Ctrl Pts',(-25.0383114836898,-1.12442703144455,
0.));
#235578=CARTESIAN_POINT('Ctrl Pts',(-25.0619667625336,-1.1142091430689,
0.));
#235579=CARTESIAN_POINT('Ctrl Pts',(-25.085669790968,-1.1039045030174,0.));
#235580=CARTESIAN_POINT('Ctrl Pts',(-25.1094200248448,-1.09351306445299,
0.));
#235581=CARTESIAN_POINT('Ctrl Pts',(-25.1332169227415,-1.08303478197174,
0.));
#235582=CARTESIAN_POINT('Ctrl Pts',(-25.1570599469311,-1.0724696116546,
0.));
#235583=CARTESIAN_POINT('Ctrl Pts',(-25.1809485642191,-1.06181751111754,
0.));
#235584=CARTESIAN_POINT('Ctrl Pts',(-25.2048822469027,-1.05107843957925,
0.));
#235585=CARTESIAN_POINT('Ctrl Pts',(-25.2288604735087,-1.04025235791515,
0.));
#235586=CARTESIAN_POINT('Ctrl Pts',(-25.2528827300427,-1.0293392287683,
0.));
#235587=CARTESIAN_POINT('Ctrl Pts',(-25.2769485087268,-1.01833901642272,
0.));
#235588=CARTESIAN_POINT('Ctrl Pts',(-25.3010573055557,-1.00725168656933,
0.));
#235589=CARTESIAN_POINT('Ctrl Pts',(-25.3252086182976,-0.996077206120919,
0.));
#235590=CARTESIAN_POINT('Ctrl Pts',(-25.3494019441444,-0.984815543004089,
0.));
#235591=CARTESIAN_POINT('Ctrl Pts',(-25.3736367778842,-0.973466666000048,
0.));
#235592=CARTESIAN_POINT('Ctrl Pts',(-25.3979126089155,-0.962030544502802,
0.));
#235593=CARTESIAN_POINT('Ctrl Pts',(-25.4222289223155,-0.950507148596968,
0.));
#235594=CARTESIAN_POINT('Ctrl Pts',(-25.4465852044835,-0.938896449495632,
0.));
#235595=CARTESIAN_POINT('Ctrl Pts',(-25.4709809474996,-0.927198419885604,
0.));
#235596=CARTESIAN_POINT('Ctrl Pts',(-25.4954156541787,-0.915413034335333,
0.));
#235597=CARTESIAN_POINT('Ctrl Pts',(-25.5198888424195,-0.903540269651154,
0.));
#235598=CARTESIAN_POINT('Ctrl Pts',(-25.5444000508223,-0.891580105349467,
0.));
#235599=CARTESIAN_POINT('Ctrl Pts',(-25.568948840818,-0.87953252383509,
0.));
#235600=CARTESIAN_POINT('Ctrl Pts',(-25.5935347843616,-0.86739750933947,
0.));
#235601=CARTESIAN_POINT('Ctrl Pts',(-25.618157453608,-0.855175047037614,
0.));
#235602=CARTESIAN_POINT('Ctrl Pts',(-25.6428164100078,-0.842865122121544,
0.));
#235603=CARTESIAN_POINT('Ctrl Pts',(-25.6675111931957,-0.830467718864367,
0.));
#235604=CARTESIAN_POINT('Ctrl Pts',(-25.6922413110172,-0.817982819786719,
0.));
#235605=CARTESIAN_POINT('Ctrl Pts',(-25.7170062262474,-0.805410404552594,
0.));
#235606=CARTESIAN_POINT('Ctrl Pts',(-25.7418053757671,-0.792750451613534,
0.));
#235607=CARTESIAN_POINT('Ctrl Pts',(-25.7666381946871,-0.780002940289025,
0.));
#235608=CARTESIAN_POINT('Ctrl Pts',(-25.7915041383304,-0.767167852648639,
0.));
#235609=CARTESIAN_POINT('Ctrl Pts',(-25.816402705995,-0.754245175608288,
0.));
#235610=CARTESIAN_POINT('Ctrl Pts',(-25.841333461908,-0.741234902664697,
0.));
#235611=CARTESIAN_POINT('Ctrl Pts',(-25.8662960624285,-0.728137036485877,
0.));
#235612=CARTESIAN_POINT('Ctrl Pts',(-25.8912902615141,-0.714951588533753,
0.));
#235613=CARTESIAN_POINT('Ctrl Pts',(-25.9163158909645,-0.701678575236602,
0.));
#235614=CARTESIAN_POINT('Ctrl Pts',(-25.941372847213,-0.688318015065678,
0.));
#235615=CARTESIAN_POINT('Ctrl Pts',(-25.9614434298092,-0.677559543215902,
0.));
#235616=CARTESIAN_POINT('Ctrl Pts',(-25.9765104298171,-0.669451306784415,
0.));
#235617=CARTESIAN_POINT('Ctrl Pts',(-25.9865613464809,-0.664028313188912,
0.));
#235618=CARTESIAN_POINT('Ctrl Pts',(-25.991588367311,-0.661312440730891,
0.));
#235619=CARTESIAN_POINT('',(-25.991588367311,-0.661312440730891,12.));
#235620=CARTESIAN_POINT('Ctrl Pts',(-25.991588367311,-0.661312440730891,
12.));
#235621=CARTESIAN_POINT('Ctrl Pts',(-25.9865613464809,-0.664028313188912,
12.));
#235622=CARTESIAN_POINT('Ctrl Pts',(-25.9765104298171,-0.669451306784415,
12.));
#235623=CARTESIAN_POINT('Ctrl Pts',(-25.9614434298092,-0.677559543215902,
12.));
#235624=CARTESIAN_POINT('Ctrl Pts',(-25.941372847213,-0.688318015065678,
12.));
#235625=CARTESIAN_POINT('Ctrl Pts',(-25.9163158909645,-0.701678575236602,
12.));
#235626=CARTESIAN_POINT('Ctrl Pts',(-25.8912902615141,-0.714951588533753,
12.));
#235627=CARTESIAN_POINT('Ctrl Pts',(-25.8662960624285,-0.728137036485877,
12.));
#235628=CARTESIAN_POINT('Ctrl Pts',(-25.841333461908,-0.741234902664697,
12.));
#235629=CARTESIAN_POINT('Ctrl Pts',(-25.816402705995,-0.754245175608288,
12.));
#235630=CARTESIAN_POINT('Ctrl Pts',(-25.7915041383304,-0.767167852648639,
12.));
#235631=CARTESIAN_POINT('Ctrl Pts',(-25.7666381946871,-0.780002940289025,
12.));
#235632=CARTESIAN_POINT('Ctrl Pts',(-25.7418053757671,-0.792750451613534,
12.));
#235633=CARTESIAN_POINT('Ctrl Pts',(-25.7170062262474,-0.805410404552594,
12.));
#235634=CARTESIAN_POINT('Ctrl Pts',(-25.6922413110172,-0.817982819786719,
12.));
#235635=CARTESIAN_POINT('Ctrl Pts',(-25.6675111931957,-0.830467718864367,
12.));
#235636=CARTESIAN_POINT('Ctrl Pts',(-25.6428164100078,-0.842865122121544,
12.));
#235637=CARTESIAN_POINT('Ctrl Pts',(-25.618157453608,-0.855175047037614,
12.));
#235638=CARTESIAN_POINT('Ctrl Pts',(-25.5935347843616,-0.86739750933947,
12.));
#235639=CARTESIAN_POINT('Ctrl Pts',(-25.568948840818,-0.87953252383509,
12.));
#235640=CARTESIAN_POINT('Ctrl Pts',(-25.5444000508223,-0.891580105349467,
12.));
#235641=CARTESIAN_POINT('Ctrl Pts',(-25.5198888424195,-0.903540269651154,
12.));
#235642=CARTESIAN_POINT('Ctrl Pts',(-25.4954156541787,-0.915413034335333,
12.));
#235643=CARTESIAN_POINT('Ctrl Pts',(-25.4709809474996,-0.927198419885604,
12.));
#235644=CARTESIAN_POINT('Ctrl Pts',(-25.4465852044835,-0.938896449495632,
12.));
#235645=CARTESIAN_POINT('Ctrl Pts',(-25.4222289223155,-0.950507148596968,
12.));
#235646=CARTESIAN_POINT('Ctrl Pts',(-25.3979126089155,-0.962030544502802,
12.));
#235647=CARTESIAN_POINT('Ctrl Pts',(-25.3736367778842,-0.973466666000048,
12.));
#235648=CARTESIAN_POINT('Ctrl Pts',(-25.3494019441444,-0.984815543004089,
12.));
#235649=CARTESIAN_POINT('Ctrl Pts',(-25.3252086182976,-0.996077206120919,
12.));
#235650=CARTESIAN_POINT('Ctrl Pts',(-25.3010573055557,-1.00725168656933,
12.));
#235651=CARTESIAN_POINT('Ctrl Pts',(-25.2769485087268,-1.01833901642272,
12.));
#235652=CARTESIAN_POINT('Ctrl Pts',(-25.2528827300427,-1.0293392287683,
12.));
#235653=CARTESIAN_POINT('Ctrl Pts',(-25.2288604735087,-1.04025235791515,
12.));
#235654=CARTESIAN_POINT('Ctrl Pts',(-25.2048822469027,-1.05107843957925,
12.));
#235655=CARTESIAN_POINT('Ctrl Pts',(-25.1809485642191,-1.06181751111754,
12.));
#235656=CARTESIAN_POINT('Ctrl Pts',(-25.1570599469311,-1.0724696116546,
12.));
#235657=CARTESIAN_POINT('Ctrl Pts',(-25.1332169227415,-1.08303478197174,
12.));
#235658=CARTESIAN_POINT('Ctrl Pts',(-25.1094200248448,-1.09351306445299,
12.));
#235659=CARTESIAN_POINT('Ctrl Pts',(-25.085669790968,-1.1039045030174,12.));
#235660=CARTESIAN_POINT('Ctrl Pts',(-25.0619667625336,-1.1142091430689,
12.));
#235661=CARTESIAN_POINT('Ctrl Pts',(-25.0383114836898,-1.12442703144455,
12.));
#235662=CARTESIAN_POINT('Ctrl Pts',(-25.0147045006193,-1.13455821638535,
12.));
#235663=CARTESIAN_POINT('Ctrl Pts',(-24.9911463621431,-1.14460274758206,
12.));
#235664=CARTESIAN_POINT('Ctrl Pts',(-24.9676376201501,-1.15456067621894,
12.));
#235665=CARTESIAN_POINT('Ctrl Pts',(-24.9441788300932,-1.16443205502852,
12.));
#235666=CARTESIAN_POINT('Ctrl Pts',(-24.9207705514449,-1.17421693835039,
12.));
#235667=CARTESIAN_POINT('Ctrl Pts',(-24.8974133481829,-1.18391538220098,
12.));
#235668=CARTESIAN_POINT('Ctrl Pts',(-24.8741077892074,-1.19352744434059,
12.));
#235669=CARTESIAN_POINT('Ctrl Pts',(-24.8508544481973,-1.20305318426015,
12.));
#235670=CARTESIAN_POINT('Ctrl Pts',(-24.8276539035092,-1.21249266318205,
12.));
#235671=CARTESIAN_POINT('Ctrl Pts',(-24.8045067380536,-1.22184594406526,
12.));
#235672=CARTESIAN_POINT('Ctrl Pts',(-24.78141353918,-1.23111309161843,12.));
#235673=CARTESIAN_POINT('Ctrl Pts',(-24.7583748985439,-1.24029417231988,
12.));
#235674=CARTESIAN_POINT('Ctrl Pts',(-24.7353914120012,-1.24938925444323,
12.));
#235675=CARTESIAN_POINT('Ctrl Pts',(-24.7124636797895,-1.25839840807415,
12.));
#235676=CARTESIAN_POINT('Ctrl Pts',(-24.6895923066837,-1.26732170513497,
12.));
#235677=CARTESIAN_POINT('Ctrl Pts',(-24.666777902156,-1.2761592194164,12.));
#235678=CARTESIAN_POINT('Ctrl Pts',(-24.6440210805278,-1.28491102661513,
12.));
#235679=CARTESIAN_POINT('Ctrl Pts',(-24.6213224611228,-1.29357720438107,
12.));
#235680=CARTESIAN_POINT('Ctrl Pts',(-24.5986826684025,-1.30215783236364,
12.));
#235681=CARTESIAN_POINT('Ctrl Pts',(-24.576102332018,-1.31065299222023,
12.));
#235682=CARTESIAN_POINT('Ctrl Pts',(-24.5535820868671,-1.31906276763669,
12.));
#235683=CARTESIAN_POINT('Ctrl Pts',(-24.5311225731434,-1.32738724435326,
12.));
#235684=CARTESIAN_POINT('Ctrl Pts',(-24.5087244363856,-1.33562651019684,
12.));
#235685=CARTESIAN_POINT('Ctrl Pts',(-24.4863883275135,-1.34378065512335,
12.));
#235686=CARTESIAN_POINT('Ctrl Pts',(-24.4641149028894,-1.35184977125644,
12.));
#235687=CARTESIAN_POINT('Ctrl Pts',(-24.4419048244524,-1.35983395290624,
12.));
#235688=CARTESIAN_POINT('Ctrl Pts',(-24.4197587598337,-1.36773329659954,
12.));
#235689=CARTESIAN_POINT('Ctrl Pts',(-24.3976773824731,-1.37554790111607,
12.));
#235690=CARTESIAN_POINT('Ctrl Pts',(-24.37566137173,-1.38327786752998,12.));
#235691=CARTESIAN_POINT('Ctrl Pts',(-24.3537114129877,-1.3909232992639,
12.));
#235692=CARTESIAN_POINT('Ctrl Pts',(-24.3318281977647,-1.3984843021281,
12.));
#235693=CARTESIAN_POINT('Ctrl Pts',(-24.3100124238316,-1.4059609843434,
12.));
#235694=CARTESIAN_POINT('Ctrl Pts',(-24.2882647953214,-1.41335345657685,
12.));
#235695=CARTESIAN_POINT('Ctrl Pts',(-24.2665860228357,-1.42066183198252,
12.));
#235696=CARTESIAN_POINT('Ctrl Pts',(-24.2449768235485,-1.42788622624851,
12.));
#235697=CARTESIAN_POINT('Ctrl Pts',(-24.2234379212978,-1.43502675765502,
12.));
#235698=CARTESIAN_POINT('Ctrl Pts',(-24.2019700467214,-1.44208354711074,
12.));
#235699=CARTESIAN_POINT('Ctrl Pts',(-24.1805739374033,-1.44905671818721,
12.));
#235700=CARTESIAN_POINT('Ctrl Pts',(-24.1592503380105,-1.45594639716314,
12.));
#235701=CARTESIAN_POINT('Ctrl Pts',(-24.1380000004272,-1.46275271307398,
12.));
#235702=CARTESIAN_POINT('Ctrl Pts',(-24.1168236838827,-1.46947579776992,
12.));
#235703=CARTESIAN_POINT('Ctrl Pts',(-24.0957221550782,-1.47611578597741,
12.));
#235704=CARTESIAN_POINT('Ctrl Pts',(-24.074696188353,-1.4826728153368,12.));
#235705=CARTESIAN_POINT('Ctrl Pts',(-24.053746565843,-1.48914702644883,
12.));
#235706=CARTESIAN_POINT('Ctrl Pts',(-24.0328740776331,-1.49553856292798,
12.));
#235707=CARTESIAN_POINT('Ctrl Pts',(-24.0120795219086,-1.50184757146099,
12.));
#235708=CARTESIAN_POINT('Ctrl Pts',(-23.991363705093,-1.50807420187702,
12.));
#235709=CARTESIAN_POINT('Ctrl Pts',(-23.9707274420145,-1.51421860720628,
12.));
#235710=CARTESIAN_POINT('Ctrl Pts',(-23.9501715561038,-1.52028094372806,
12.));
#235711=CARTESIAN_POINT('Ctrl Pts',(-23.9296968795761,-1.52626137103039,
12.));
#235712=CARTESIAN_POINT('Ctrl Pts',(-23.9093042536119,-1.53216005207462,
12.));
#235713=CARTESIAN_POINT('Ctrl Pts',(-23.8889945285313,-1.53797715326748,
12.));
#235714=CARTESIAN_POINT('Ctrl Pts',(-23.8687685639635,-1.54371284453978,
12.));
#235715=CARTESIAN_POINT('Ctrl Pts',(-23.8486272290698,-1.5493672994053,
12.));
#235716=CARTESIAN_POINT('Ctrl Pts',(-23.8285714027631,-1.55494069502628,
12.));
#235717=CARTESIAN_POINT('Ctrl Pts',(-23.8086019739192,-1.56043321228631,
12.));
#235718=CARTESIAN_POINT('Ctrl Pts',(-23.788719841588,-1.56584503586844,
12.));
#235719=CARTESIAN_POINT('Ctrl Pts',(-23.7689259151869,-1.57117635434412,
12.));
#235720=CARTESIAN_POINT('Ctrl Pts',(-23.7492211147369,-1.57642736025251,
12.));
#235721=CARTESIAN_POINT('Ctrl Pts',(-23.7296063711308,-1.58159825017362,
12.));
#235722=CARTESIAN_POINT('Ctrl Pts',(-23.7100826263835,-1.58668922481222,
12.));
#235723=CARTESIAN_POINT('Ctrl Pts',(-23.6906508338833,-1.59170048908631,
12.));
#235724=CARTESIAN_POINT('Ctrl Pts',(-23.6713119586302,-1.59663225222458,
12.));
#235725=CARTESIAN_POINT('Ctrl Pts',(-23.6520669774863,-1.60148472786588,
12.));
#235726=CARTESIAN_POINT('Ctrl Pts',(-23.6329168794916,-1.60625813414666,
12.));
#235727=CARTESIAN_POINT('Ctrl Pts',(-23.6138626661644,-1.61095269379773,
12.));
#235728=CARTESIAN_POINT('Ctrl Pts',(-23.5949053517996,-1.61556863424697,
12.));
#235729=CARTESIAN_POINT('Ctrl Pts',(-23.5760459637608,-1.62010618772869,
12.));
#235730=CARTESIAN_POINT('Ctrl Pts',(-23.5572855427617,-1.62456559140072,
12.));
#235731=CARTESIAN_POINT('Ctrl Pts',(-23.5386251432278,-1.62894708745231,
12.));
#235732=CARTESIAN_POINT('Ctrl Pts',(-23.5200658336624,-1.63325092321731,
12.));
#235733=CARTESIAN_POINT('Ctrl Pts',(-23.5016086970006,-1.63747735129474,
12.));
#235734=CARTESIAN_POINT('Ctrl Pts',(-23.4832548309638,-1.64162662967524,
12.));
#235735=CARTESIAN_POINT('Ctrl Pts',(-23.4650053483919,-1.64569902187608,
12.));
#235736=CARTESIAN_POINT('Ctrl Pts',(-23.446861377656,-1.64969479707339,
12.));
#235737=CARTESIAN_POINT('Ctrl Pts',(-23.4288240631034,-1.6536142302373,
12.));
#235738=CARTESIAN_POINT('Ctrl Pts',(-23.4108945654803,-1.65745760227507,
12.));
#235739=CARTESIAN_POINT('Ctrl Pts',(-23.3930740623622,-1.66122520018008,
12.));
#235740=CARTESIAN_POINT('Ctrl Pts',(-23.375363748555,-1.66491731718864,
12.));
#235741=CARTESIAN_POINT('Ctrl Pts',(-23.3577648365747,-1.66853425293977,
12.));
#235742=CARTESIAN_POINT('Ctrl Pts',(-23.3402785571866,-1.67207631363905,
12.));
#235743=CARTESIAN_POINT('Ctrl Pts',(-23.3229061599145,-1.67554381222987,
12.));
#235744=CARTESIAN_POINT('Ctrl Pts',(-23.3056489135611,-1.67893706857123,
12.));
#235745=CARTESIAN_POINT('Ctrl Pts',(-23.2885081066949,-1.68225640962181,
12.));
#235746=CARTESIAN_POINT('Ctrl Pts',(-23.2714850482245,-1.68550216963275,
12.));
#235747=CARTESIAN_POINT('Ctrl Pts',(-23.2545810680536,-1.6886746903491,
12.));
#235748=CARTESIAN_POINT('Ctrl Pts',(-23.2377975177014,-1.69177432121716,
12.));
#235749=CARTESIAN_POINT('Ctrl Pts',(-23.2211357709374,-1.69480141959945,
12.));
#235750=CARTESIAN_POINT('Ctrl Pts',(-23.2045972243765,-1.69775635099425,
12.));
#235751=CARTESIAN_POINT('Ctrl Pts',(-23.1881832981848,-1.70063948926987,
12.));
#235752=CARTESIAN_POINT('Ctrl Pts',(-23.1718954368749,-1.70345121691259,
12.));
#235753=CARTESIAN_POINT('Ctrl Pts',(-23.1557351100613,-1.70619192527847,
12.));
#235754=CARTESIAN_POINT('Ctrl Pts',(-23.1397038132358,-1.7088620148546,
12.));
#235755=CARTESIAN_POINT('Ctrl Pts',(-23.1238030684929,-1.71146189552192,
12.));
#235756=CARTESIAN_POINT('Ctrl Pts',(-23.1080344254291,-1.71399198684724,
12.));
#235757=CARTESIAN_POINT('Ctrl Pts',(-23.0923994621216,-1.71645271839311,
12.));
#235758=CARTESIAN_POINT('Ctrl Pts',(-23.0768997860709,-1.71884453003027,
12.));
#235759=CARTESIAN_POINT('Ctrl Pts',(-23.061537035156,-1.7211678722598,12.));
#235760=CARTESIAN_POINT('Ctrl Pts',(-23.0463128785528,-1.72342320653731,
12.));
#235761=CARTESIAN_POINT('Ctrl Pts',(-23.031229017888,-1.72561100564033,
12.));
#235762=CARTESIAN_POINT('Ctrl Pts',(-23.0162871884167,-1.72773175404702,
12.));
#235763=CARTESIAN_POINT('Ctrl Pts',(-23.0014891601891,-1.72978594832137,
12.));
#235764=CARTESIAN_POINT('Ctrl Pts',(-22.9868367391978,-1.73177409750193,
12.));
#235765=CARTESIAN_POINT('Ctrl Pts',(-22.9723317685688,-1.73369672350817,
12.));
#235766=CARTESIAN_POINT('Ctrl Pts',(-22.9579761301062,-1.73555436162771,
12.));
#235767=CARTESIAN_POINT('Ctrl Pts',(-22.9437717457825,-1.73734756100038,
12.));
#235768=CARTESIAN_POINT('Ctrl Pts',(-22.9297205792587,-1.73907688511664,
12.));
#235769=CARTESIAN_POINT('Ctrl Pts',(-22.9158246373365,-1.74074291231057,
12.));
#235770=CARTESIAN_POINT('Ctrl Pts',(-22.9020859716144,-1.74234623630079,
12.));
#235771=CARTESIAN_POINT('Ctrl Pts',(-22.8885066803351,-1.74388746677702,
12.));
#235772=CARTESIAN_POINT('Ctrl Pts',(-22.8750889101696,-1.745367229982,12.));
#235773=CARTESIAN_POINT('Ctrl Pts',(-22.8618348580234,-1.74678616930663,
12.));
#235774=CARTESIAN_POINT('Ctrl Pts',(-22.8487467728075,-1.74814494588492,
12.));
#235775=CARTESIAN_POINT('Ctrl Pts',(-22.8358269579854,-1.74944423940117,
12.));
#235776=CARTESIAN_POINT('Ctrl Pts',(-22.8230777741285,-1.75068474890884,
12.));
#235777=CARTESIAN_POINT('Ctrl Pts',(-22.8105016414712,-1.75186719365589,
12.));
#235778=CARTESIAN_POINT('Ctrl Pts',(-22.7981010424312,-1.75299231391461,
12.));
#235779=CARTESIAN_POINT('Ctrl Pts',(-22.7858785242358,-1.75406087182929,
12.));
#235780=CARTESIAN_POINT('Ctrl Pts',(-22.7738367016115,-1.75507365227127,
12.));
#235781=CARTESIAN_POINT('Ctrl Pts',(-22.7619782595013,-1.7560314637164,
12.));
#235782=CARTESIAN_POINT('Ctrl Pts',(-22.7503059556455,-1.75693513908911,
12.));
#235783=CARTESIAN_POINT('Ctrl Pts',(-22.7388226235565,-1.75778553673249,
12.));
#235784=CARTESIAN_POINT('Ctrl Pts',(-22.7275311777305,-1.75858354204635,
12.));
#235785=CARTESIAN_POINT('Ctrl Pts',(-22.7164346186007,-1.75933006905924,
12.));
#235786=CARTESIAN_POINT('Ctrl Pts',(-22.7055360375481,-1.76002606202399,
12.));
#235787=CARTESIAN_POINT('Ctrl Pts',(-22.6948386219843,-1.76067249704884,
12.));
#235788=CARTESIAN_POINT('Ctrl Pts',(-22.6843456585245,-1.76127038310612,
12.));
#235789=CARTESIAN_POINT('Ctrl Pts',(-22.6740605356699,-1.76182076289525,
12.));
#235790=CARTESIAN_POINT('Ctrl Pts',(-22.6639867471756,-1.76232471392567,
12.));
#235791=CARTESIAN_POINT('Ctrl Pts',(-22.6541278938413,-1.76278334912559,
12.));
#235792=CARTESIAN_POINT('Ctrl Pts',(-22.6444876940425,-1.76319782013914,
12.));
#235793=CARTESIAN_POINT('Ctrl Pts',(-22.635069997936,-1.76356932176272,
12.));
#235794=CARTESIAN_POINT('Ctrl Pts',(-22.6258787994847,-1.76389909571402,
12.));
#235795=CARTESIAN_POINT('Ctrl Pts',(-22.6169182517693,-1.76418843543739,
12.));
#235796=CARTESIAN_POINT('Ctrl Pts',(-22.6081926681342,-1.76443868648015,
12.));
#235797=CARTESIAN_POINT('Ctrl Pts',(-22.5997065145638,-1.76465124413556,
12.));
#235798=CARTESIAN_POINT('Ctrl Pts',(-22.5914644078106,-1.76482755288411,
12.));
#235799=CARTESIAN_POINT('Ctrl Pts',(-22.5834711038024,-1.76496910283088,
12.));
#235800=CARTESIAN_POINT('Ctrl Pts',(-22.5757315316355,-1.76507744026747,
12.));
#235801=CARTESIAN_POINT('Ctrl Pts',(-22.5682508499873,-1.76515418518829,
12.));
#235802=CARTESIAN_POINT('Ctrl Pts',(-22.5610344912501,-1.76520104500449,
12.));
#235803=CARTESIAN_POINT('Ctrl Pts',(-22.5540882235837,-1.76521983384063,
12.));
#235804=CARTESIAN_POINT('Ctrl Pts',(-22.5474180954006,-1.76521245524047,
12.));
#235805=CARTESIAN_POINT('Ctrl Pts',(-22.5410303590891,-1.76518087841492,
12.));
#235806=CARTESIAN_POINT('Ctrl Pts',(-22.5349313983571,-1.7651271156325,
12.));
#235807=CARTESIAN_POINT('Ctrl Pts',(-22.529127665298,-1.76505320262751,
12.));
#235808=CARTESIAN_POINT('Ctrl Pts',(-22.5236259635515,-1.76496128643369,
12.));
#235809=CARTESIAN_POINT('Ctrl Pts',(-22.5184336670207,-1.76485369319896,
12.));
#235810=CARTESIAN_POINT('Ctrl Pts',(-22.5135590569554,-1.76473303281159,
12.));
#235811=CARTESIAN_POINT('Ctrl Pts',(-22.5090112700212,-1.76460218257323,
12.));
#235812=CARTESIAN_POINT('Ctrl Pts',(-22.5047996391978,-1.76446408210366,
12.));
#235813=CARTESIAN_POINT('Ctrl Pts',(-22.5009332677316,-1.76432160068725,
12.));
#235814=CARTESIAN_POINT('Ctrl Pts',(-22.4974203063191,-1.76417731243462,
12.));
#235815=CARTESIAN_POINT('Ctrl Pts',(-22.4942693792449,-1.764033938803,12.));
#235816=CARTESIAN_POINT('Ctrl Pts',(-22.4914909094908,-1.76389475965724,
12.));
#235817=CARTESIAN_POINT('Ctrl Pts',(-22.4890991659478,-1.76376424879505,
12.));
#235818=CARTESIAN_POINT('Ctrl Pts',(-22.4871115206571,-1.76364784232963,
12.));
#235819=CARTESIAN_POINT('Ctrl Pts',(-22.4855446605991,-1.76355076045546,
12.));
#235820=CARTESIAN_POINT('Ctrl Pts',(-22.4844112933129,-1.76347698284792,
12.));
#235821=CARTESIAN_POINT('Ctrl Pts',(-22.483856251707,-1.76343813434565,
12.));
#235822=CARTESIAN_POINT('Ctrl Pts',(-22.4836387052232,-1.7634206426357,
12.));
#235823=CARTESIAN_POINT('Ctrl Pts',(-22.483581992979,-1.76341415538764,
12.));
#235824=CARTESIAN_POINT('Ctrl Pts',(-22.4835757167854,-1.76341220531179,
12.));
#235825=CARTESIAN_POINT('',(-25.991588367311,-0.661312440730891,0.));
#235826=CARTESIAN_POINT('Origin',(-21.1389261070099,3.92374859571501,0.));
#235827=CARTESIAN_POINT('',(-22.1738711152697,4.11585220600461,12.));
#235828=CARTESIAN_POINT('',(-10.5694630535049,1.96187429785751,12.));
#235829=CARTESIAN_POINT('',(-22.1738711152697,4.11585220600461,0.));
#235830=CARTESIAN_POINT('',(-22.1738711152697,4.11585220600461,0.));
#235831=CARTESIAN_POINT('',(-10.5694630535049,1.96187429785751,0.));
#235832=CARTESIAN_POINT('Ctrl Pts',(-25.991588367311,0.661312440730901,
0.));
#235833=CARTESIAN_POINT('Ctrl Pts',(-25.991588367311,0.661312440730901,
12.));
#235834=CARTESIAN_POINT('Ctrl Pts',(-25.9865613464773,0.664028313187627,
0.));
#235835=CARTESIAN_POINT('Ctrl Pts',(-25.9865613464773,0.664028313187627,
12.));
#235836=CARTESIAN_POINT('Ctrl Pts',(-25.9765104298071,0.669451306780825,
0.));
#235837=CARTESIAN_POINT('Ctrl Pts',(-25.9765104298071,0.669451306780825,
12.));
#235838=CARTESIAN_POINT('Ctrl Pts',(-25.9614434297919,0.677559543209725,
0.));
#235839=CARTESIAN_POINT('Ctrl Pts',(-25.9614434297919,0.677559543209725,
12.));
#235840=CARTESIAN_POINT('Ctrl Pts',(-25.9413728471909,0.688318015057729,
0.));
#235841=CARTESIAN_POINT('Ctrl Pts',(-25.9413728471909,0.688318015057729,
12.));
#235842=CARTESIAN_POINT('Ctrl Pts',(-25.9163158909426,0.701678575228756,
0.));
#235843=CARTESIAN_POINT('Ctrl Pts',(-25.9163158909426,0.701678575228756,
12.));
#235844=CARTESIAN_POINT('Ctrl Pts',(-25.891290261497,0.714951588527638,
0.));
#235845=CARTESIAN_POINT('Ctrl Pts',(-25.891290261497,0.714951588527638,
12.));
#235846=CARTESIAN_POINT('Ctrl Pts',(-25.8662960624185,0.728137036482335,
0.));
#235847=CARTESIAN_POINT('Ctrl Pts',(-25.8662960624185,0.728137036482335,
12.));
#235848=CARTESIAN_POINT('Ctrl Pts',(-25.8413334619055,0.741234902663807,
0.));
#235849=CARTESIAN_POINT('Ctrl Pts',(-25.8413334619055,0.741234902663807,
12.));
#235850=CARTESIAN_POINT('Ctrl Pts',(-25.8164027059984,0.754245175609524,
0.));
#235851=CARTESIAN_POINT('Ctrl Pts',(-25.8164027059984,0.754245175609524,
12.));
#235852=CARTESIAN_POINT('Ctrl Pts',(-25.7915041383376,0.767167852651168,
0.));
#235853=CARTESIAN_POINT('Ctrl Pts',(-25.7915041383376,0.767167852651168,
12.));
#235854=CARTESIAN_POINT('Ctrl Pts',(-25.7666381946955,0.780002940291965,
0.));
#235855=CARTESIAN_POINT('Ctrl Pts',(-25.7666381946955,0.780002940291965,
12.));
#235856=CARTESIAN_POINT('Ctrl Pts',(-25.7418053757746,0.792750451616127,
0.));
#235857=CARTESIAN_POINT('Ctrl Pts',(-25.7418053757746,0.792750451616127,
12.));
#235858=CARTESIAN_POINT('Ctrl Pts',(-25.7170062262525,0.805410404554352,
0.));
#235859=CARTESIAN_POINT('Ctrl Pts',(-25.7170062262525,0.805410404554352,
12.));
#235860=CARTESIAN_POINT('Ctrl Pts',(-25.6922413110194,0.817982819787464,
0.));
#235861=CARTESIAN_POINT('Ctrl Pts',(-25.6922413110194,0.817982819787464,
12.));
#235862=CARTESIAN_POINT('Ctrl Pts',(-25.6675111931952,0.830467718864205,
0.));
#235863=CARTESIAN_POINT('Ctrl Pts',(-25.6675111931952,0.830467718864205,
12.));
#235864=CARTESIAN_POINT('Ctrl Pts',(-25.6428164100055,0.842865122120758,
0.));
#235865=CARTESIAN_POINT('Ctrl Pts',(-25.6428164100055,0.842865122120758,
12.));
#235866=CARTESIAN_POINT('Ctrl Pts',(-25.6181574536049,0.855175047036549,
0.));
#235867=CARTESIAN_POINT('Ctrl Pts',(-25.6181574536049,0.855175047036549,
12.));
#235868=CARTESIAN_POINT('Ctrl Pts',(-25.5935347843585,0.867397509338431,
0.));
#235869=CARTESIAN_POINT('Ctrl Pts',(-25.5935347843585,0.867397509338431,
12.));
#235870=CARTESIAN_POINT('Ctrl Pts',(-25.5689488408156,0.879532523834294,
0.));
#235871=CARTESIAN_POINT('Ctrl Pts',(-25.5689488408156,0.879532523834294,
12.));
#235872=CARTESIAN_POINT('Ctrl Pts',(-25.5444000508211,0.89158010534904,
0.));
#235873=CARTESIAN_POINT('Ctrl Pts',(-25.5444000508211,0.89158010534904,
12.));
#235874=CARTESIAN_POINT('Ctrl Pts',(-25.5198888424194,0.903540269651106,
0.));
#235875=CARTESIAN_POINT('Ctrl Pts',(-25.5198888424194,0.903540269651106,
12.));
#235876=CARTESIAN_POINT('Ctrl Pts',(-25.4954156541795,0.915413034335613,
0.));
#235877=CARTESIAN_POINT('Ctrl Pts',(-25.4954156541795,0.915413034335613,
12.));
#235878=CARTESIAN_POINT('Ctrl Pts',(-25.4709809475009,0.927198419886094,
0.));
#235879=CARTESIAN_POINT('Ctrl Pts',(-25.4709809475009,0.927198419886094,
12.));
#235880=CARTESIAN_POINT('Ctrl Pts',(-25.4465852044849,0.938896449496192,
0.));
#235881=CARTESIAN_POINT('Ctrl Pts',(-25.4465852044849,0.938896449496192,
12.));
#235882=CARTESIAN_POINT('Ctrl Pts',(-25.4222289223167,0.950507148597468,
0.));
#235883=CARTESIAN_POINT('Ctrl Pts',(-25.4222289223167,0.950507148597468,
12.));
#235884=CARTESIAN_POINT('Ctrl Pts',(-25.3979126089163,0.962030544503142,
0.));
#235885=CARTESIAN_POINT('Ctrl Pts',(-25.3979126089163,0.962030544503142,
12.));
#235886=CARTESIAN_POINT('Ctrl Pts',(-25.3736367778845,0.973466666000163,
0.));
#235887=CARTESIAN_POINT('Ctrl Pts',(-25.3736367778845,0.973466666000163,
12.));
#235888=CARTESIAN_POINT('Ctrl Pts',(-25.3494019441441,0.984815543003973,
0.));
#235889=CARTESIAN_POINT('Ctrl Pts',(-25.3494019441441,0.984815543003973,
12.));
#235890=CARTESIAN_POINT('Ctrl Pts',(-25.3252086182968,0.996077206120624,
0.));
#235891=CARTESIAN_POINT('Ctrl Pts',(-25.3252086182968,0.996077206120624,
12.));
#235892=CARTESIAN_POINT('Ctrl Pts',(-25.3010573055547,1.00725168656896,
0.));
#235893=CARTESIAN_POINT('Ctrl Pts',(-25.3010573055547,1.00725168656896,
12.));
#235894=CARTESIAN_POINT('Ctrl Pts',(-25.276948508726,1.01833901642237,0.));
#235895=CARTESIAN_POINT('Ctrl Pts',(-25.276948508726,1.01833901642237,12.));
#235896=CARTESIAN_POINT('Ctrl Pts',(-25.2528827300422,1.02933922876806,
0.));
#235897=CARTESIAN_POINT('Ctrl Pts',(-25.2528827300422,1.02933922876806,
12.));
#235898=CARTESIAN_POINT('Ctrl Pts',(-25.2288604735086,1.04025235791507,
0.));
#235899=CARTESIAN_POINT('Ctrl Pts',(-25.2288604735086,1.04025235791507,
12.));
#235900=CARTESIAN_POINT('Ctrl Pts',(-25.2048822469028,1.05107843957931,
0.));
#235901=CARTESIAN_POINT('Ctrl Pts',(-25.2048822469028,1.05107843957931,
12.));
#235902=CARTESIAN_POINT('Ctrl Pts',(-25.1809485642192,1.06181751111768,
0.));
#235903=CARTESIAN_POINT('Ctrl Pts',(-25.1809485642192,1.06181751111768,
12.));
#235904=CARTESIAN_POINT('Ctrl Pts',(-25.157059946931,1.07246961165475,0.));
#235905=CARTESIAN_POINT('Ctrl Pts',(-25.157059946931,1.07246961165475,12.));
#235906=CARTESIAN_POINT('Ctrl Pts',(-25.1332169227413,1.08303478197187,
0.));
#235907=CARTESIAN_POINT('Ctrl Pts',(-25.1332169227413,1.08303478197187,
12.));
#235908=CARTESIAN_POINT('Ctrl Pts',(-25.1094200248446,1.09351306445308,
0.));
#235909=CARTESIAN_POINT('Ctrl Pts',(-25.1094200248446,1.09351306445308,
12.));
#235910=CARTESIAN_POINT('Ctrl Pts',(-25.0856697909679,1.10390450301745,
0.));
#235911=CARTESIAN_POINT('Ctrl Pts',(-25.0856697909679,1.10390450301745,
12.));
#235912=CARTESIAN_POINT('Ctrl Pts',(-25.0619667625336,1.11420914306889,
0.));
#235913=CARTESIAN_POINT('Ctrl Pts',(-25.0619667625336,1.11420914306889,
12.));
#235914=CARTESIAN_POINT('Ctrl Pts',(-25.0383114836899,1.12442703144451,
0.));
#235915=CARTESIAN_POINT('Ctrl Pts',(-25.0383114836899,1.12442703144451,
12.));
#235916=CARTESIAN_POINT('Ctrl Pts',(-25.0147045006196,1.1345582163853,0.));
#235917=CARTESIAN_POINT('Ctrl Pts',(-25.0147045006196,1.1345582163853,12.));
#235918=CARTESIAN_POINT('Ctrl Pts',(-24.9911463621433,1.144602747582,0.));
#235919=CARTESIAN_POINT('Ctrl Pts',(-24.9911463621433,1.144602747582,12.));
#235920=CARTESIAN_POINT('Ctrl Pts',(-24.9676376201502,1.15456067621889,
0.));
#235921=CARTESIAN_POINT('Ctrl Pts',(-24.9676376201502,1.15456067621889,
12.));
#235922=CARTESIAN_POINT('Ctrl Pts',(-24.9441788300932,1.16443205502849,
0.));
#235923=CARTESIAN_POINT('Ctrl Pts',(-24.9441788300932,1.16443205502849,
12.));
#235924=CARTESIAN_POINT('Ctrl Pts',(-24.9207705514449,1.17421693835041,
0.));
#235925=CARTESIAN_POINT('Ctrl Pts',(-24.9207705514449,1.17421693835041,
12.));
#235926=CARTESIAN_POINT('Ctrl Pts',(-24.8974133481829,1.18391538220103,
0.));
#235927=CARTESIAN_POINT('Ctrl Pts',(-24.8974133481829,1.18391538220103,
12.));
#235928=CARTESIAN_POINT('Ctrl Pts',(-24.8741077892075,1.19352744434064,
0.));
#235929=CARTESIAN_POINT('Ctrl Pts',(-24.8741077892075,1.19352744434064,
12.));
#235930=CARTESIAN_POINT('Ctrl Pts',(-24.8508544481974,1.2030531842602,0.));
#235931=CARTESIAN_POINT('Ctrl Pts',(-24.8508544481974,1.2030531842602,12.));
#235932=CARTESIAN_POINT('Ctrl Pts',(-24.8276539035092,1.21249266318208,
0.));
#235933=CARTESIAN_POINT('Ctrl Pts',(-24.8276539035092,1.21249266318208,
12.));
#235934=CARTESIAN_POINT('Ctrl Pts',(-24.8045067380536,1.22184594406528,
0.));
#235935=CARTESIAN_POINT('Ctrl Pts',(-24.8045067380536,1.22184594406528,
12.));
#235936=CARTESIAN_POINT('Ctrl Pts',(-24.7814135391799,1.23111309161843,
0.));
#235937=CARTESIAN_POINT('Ctrl Pts',(-24.7814135391799,1.23111309161843,
12.));
#235938=CARTESIAN_POINT('Ctrl Pts',(-24.7583748985438,1.24029417231989,
0.));
#235939=CARTESIAN_POINT('Ctrl Pts',(-24.7583748985438,1.24029417231989,
12.));
#235940=CARTESIAN_POINT('Ctrl Pts',(-24.7353914120011,1.24938925444325,
0.));
#235941=CARTESIAN_POINT('Ctrl Pts',(-24.7353914120011,1.24938925444325,
12.));
#235942=CARTESIAN_POINT('Ctrl Pts',(-24.7124636797894,1.25839840807418,
0.));
#235943=CARTESIAN_POINT('Ctrl Pts',(-24.7124636797894,1.25839840807418,
12.));
#235944=CARTESIAN_POINT('Ctrl Pts',(-24.6895923066836,1.267321705135,0.));
#235945=CARTESIAN_POINT('Ctrl Pts',(-24.6895923066836,1.267321705135,12.));
#235946=CARTESIAN_POINT('Ctrl Pts',(-24.666777902156,1.27615921941642,0.));
#235947=CARTESIAN_POINT('Ctrl Pts',(-24.666777902156,1.27615921941642,12.));
#235948=CARTESIAN_POINT('Ctrl Pts',(-24.6440210805278,1.28491102661514,
0.));
#235949=CARTESIAN_POINT('Ctrl Pts',(-24.6440210805278,1.28491102661514,
12.));
#235950=CARTESIAN_POINT('Ctrl Pts',(-24.6213224611229,1.29357720438107,
0.));
#235951=CARTESIAN_POINT('Ctrl Pts',(-24.6213224611229,1.29357720438107,
12.));
#235952=CARTESIAN_POINT('Ctrl Pts',(-24.5986826684027,1.30215783236362,
0.));
#235953=CARTESIAN_POINT('Ctrl Pts',(-24.5986826684027,1.30215783236362,
12.));
#235954=CARTESIAN_POINT('Ctrl Pts',(-24.5761023320183,1.31065299222021,
0.));
#235955=CARTESIAN_POINT('Ctrl Pts',(-24.5761023320183,1.31065299222021,
12.));
#235956=CARTESIAN_POINT('Ctrl Pts',(-24.5535820868674,1.31906276763668,
0.));
#235957=CARTESIAN_POINT('Ctrl Pts',(-24.5535820868674,1.31906276763668,
12.));
#235958=CARTESIAN_POINT('Ctrl Pts',(-24.5311225731435,1.32738724435326,
0.));
#235959=CARTESIAN_POINT('Ctrl Pts',(-24.5311225731435,1.32738724435326,
12.));
#235960=CARTESIAN_POINT('Ctrl Pts',(-24.5087244363856,1.33562651019686,
0.));
#235961=CARTESIAN_POINT('Ctrl Pts',(-24.5087244363856,1.33562651019686,
12.));
#235962=CARTESIAN_POINT('Ctrl Pts',(-24.4863883275134,1.34378065512337,
0.));
#235963=CARTESIAN_POINT('Ctrl Pts',(-24.4863883275134,1.34378065512337,
12.));
#235964=CARTESIAN_POINT('Ctrl Pts',(-24.4641149028892,1.35184977125648,
0.));
#235965=CARTESIAN_POINT('Ctrl Pts',(-24.4641149028892,1.35184977125648,
12.));
#235966=CARTESIAN_POINT('Ctrl Pts',(-24.4419048244523,1.35983395290627,
0.));
#235967=CARTESIAN_POINT('Ctrl Pts',(-24.4419048244523,1.35983395290627,
12.));
#235968=CARTESIAN_POINT('Ctrl Pts',(-24.4197587598337,1.36773329659956,
0.));
#235969=CARTESIAN_POINT('Ctrl Pts',(-24.4197587598337,1.36773329659956,
12.));
#235970=CARTESIAN_POINT('Ctrl Pts',(-24.3976773824732,1.37554790111609,
0.));
#235971=CARTESIAN_POINT('Ctrl Pts',(-24.3976773824732,1.37554790111609,
12.));
#235972=CARTESIAN_POINT('Ctrl Pts',(-24.3756613717299,1.38327786752998,
0.));
#235973=CARTESIAN_POINT('Ctrl Pts',(-24.3756613717299,1.38327786752998,
12.));
#235974=CARTESIAN_POINT('Ctrl Pts',(-24.3537114129875,1.39092329926388,
0.));
#235975=CARTESIAN_POINT('Ctrl Pts',(-24.3537114129875,1.39092329926388,
12.));
#235976=CARTESIAN_POINT('Ctrl Pts',(-24.3318281977643,1.39848430212807,
0.));
#235977=CARTESIAN_POINT('Ctrl Pts',(-24.3318281977643,1.39848430212807,
12.));
#235978=CARTESIAN_POINT('Ctrl Pts',(-24.3100124238311,1.40596098434337,
0.));
#235979=CARTESIAN_POINT('Ctrl Pts',(-24.3100124238311,1.40596098434337,
12.));
#235980=CARTESIAN_POINT('Ctrl Pts',(-24.288264795321,1.41335345657682,0.));
#235981=CARTESIAN_POINT('Ctrl Pts',(-24.288264795321,1.41335345657682,12.));
#235982=CARTESIAN_POINT('Ctrl Pts',(-24.2665860228356,1.42066183198252,
0.));
#235983=CARTESIAN_POINT('Ctrl Pts',(-24.2665860228356,1.42066183198252,
12.));
#235984=CARTESIAN_POINT('Ctrl Pts',(-24.2449768235488,1.42788622624854,
0.));
#235985=CARTESIAN_POINT('Ctrl Pts',(-24.2449768235488,1.42788622624854,
12.));
#235986=CARTESIAN_POINT('Ctrl Pts',(-24.2234379212984,1.43502675765508,
0.));
#235987=CARTESIAN_POINT('Ctrl Pts',(-24.2234379212984,1.43502675765508,
12.));
#235988=CARTESIAN_POINT('Ctrl Pts',(-24.201970046722,1.44208354711082,0.));
#235989=CARTESIAN_POINT('Ctrl Pts',(-24.201970046722,1.44208354711082,12.));
#235990=CARTESIAN_POINT('Ctrl Pts',(-24.1805739374038,1.44905671818727,
0.));
#235991=CARTESIAN_POINT('Ctrl Pts',(-24.1805739374038,1.44905671818727,
12.));
#235992=CARTESIAN_POINT('Ctrl Pts',(-24.1592503380107,1.45594639716317,
0.));
#235993=CARTESIAN_POINT('Ctrl Pts',(-24.1592503380107,1.45594639716317,
12.));
#235994=CARTESIAN_POINT('Ctrl Pts',(-24.1380000004272,1.46275271307397,
0.));
#235995=CARTESIAN_POINT('Ctrl Pts',(-24.1380000004272,1.46275271307397,
12.));
#235996=CARTESIAN_POINT('Ctrl Pts',(-24.1168236838824,1.46947579776991,
0.));
#235997=CARTESIAN_POINT('Ctrl Pts',(-24.1168236838824,1.46947579776991,
12.));
#235998=CARTESIAN_POINT('Ctrl Pts',(-24.0957221550778,1.47611578597742,
0.));
#235999=CARTESIAN_POINT('Ctrl Pts',(-24.0957221550778,1.47611578597742,
12.));
#236000=CARTESIAN_POINT('Ctrl Pts',(-24.0746961883528,1.48267281533683,
0.));
#236001=CARTESIAN_POINT('Ctrl Pts',(-24.0746961883528,1.48267281533683,
12.));
#236002=CARTESIAN_POINT('Ctrl Pts',(-24.0537465658429,1.48914702644887,
0.));
#236003=CARTESIAN_POINT('Ctrl Pts',(-24.0537465658429,1.48914702644887,
12.));
#236004=CARTESIAN_POINT('Ctrl Pts',(-24.0328740776331,1.49553856292801,
0.));
#236005=CARTESIAN_POINT('Ctrl Pts',(-24.0328740776331,1.49553856292801,
12.));
#236006=CARTESIAN_POINT('Ctrl Pts',(-24.0120795219086,1.50184757146098,
0.));
#236007=CARTESIAN_POINT('Ctrl Pts',(-24.0120795219086,1.50184757146098,
12.));
#236008=CARTESIAN_POINT('Ctrl Pts',(-23.9913637050927,1.50807420187694,
0.));
#236009=CARTESIAN_POINT('Ctrl Pts',(-23.9913637050927,1.50807420187694,
12.));
#236010=CARTESIAN_POINT('Ctrl Pts',(-23.970727442014,1.51421860720614,0.));
#236011=CARTESIAN_POINT('Ctrl Pts',(-23.970727442014,1.51421860720614,12.));
#236012=CARTESIAN_POINT('Ctrl Pts',(-23.9501715561033,1.52028094372792,
0.));
#236013=CARTESIAN_POINT('Ctrl Pts',(-23.9501715561033,1.52028094372792,
12.));
#236014=CARTESIAN_POINT('Ctrl Pts',(-23.9296968795757,1.52626137103032,
0.));
#236015=CARTESIAN_POINT('Ctrl Pts',(-23.9296968795757,1.52626137103032,
12.));
#236016=CARTESIAN_POINT('Ctrl Pts',(-23.9093042536119,1.53216005207463,
0.));
#236017=CARTESIAN_POINT('Ctrl Pts',(-23.9093042536119,1.53216005207463,
12.));
#236018=CARTESIAN_POINT('Ctrl Pts',(-23.8889945285318,1.53797715326758,
0.));
#236019=CARTESIAN_POINT('Ctrl Pts',(-23.8889945285318,1.53797715326758,
12.));
#236020=CARTESIAN_POINT('Ctrl Pts',(-23.8687685639642,1.5437128445399,0.));
#236021=CARTESIAN_POINT('Ctrl Pts',(-23.8687685639642,1.5437128445399,12.));
#236022=CARTESIAN_POINT('Ctrl Pts',(-23.8486272290705,1.54936729940541,
0.));
#236023=CARTESIAN_POINT('Ctrl Pts',(-23.8486272290705,1.54936729940541,
12.));
#236024=CARTESIAN_POINT('Ctrl Pts',(-23.8285714027636,1.55494069502635,
0.));
#236025=CARTESIAN_POINT('Ctrl Pts',(-23.8285714027636,1.55494069502635,
12.));
#236026=CARTESIAN_POINT('Ctrl Pts',(-23.8086019739194,1.56043321228633,
0.));
#236027=CARTESIAN_POINT('Ctrl Pts',(-23.8086019739194,1.56043321228633,
12.));
#236028=CARTESIAN_POINT('Ctrl Pts',(-23.7887198415878,1.56584503586843,
0.));
#236029=CARTESIAN_POINT('Ctrl Pts',(-23.7887198415878,1.56584503586843,
12.));
#236030=CARTESIAN_POINT('Ctrl Pts',(-23.7689259151862,1.57117635434408,
0.));
#236031=CARTESIAN_POINT('Ctrl Pts',(-23.7689259151862,1.57117635434408,
12.));
#236032=CARTESIAN_POINT('Ctrl Pts',(-23.749221114736,1.57642736025246,0.));
#236033=CARTESIAN_POINT('Ctrl Pts',(-23.749221114736,1.57642736025246,12.));
#236034=CARTESIAN_POINT('Ctrl Pts',(-23.72960637113,1.58159825017358,0.));
#236035=CARTESIAN_POINT('Ctrl Pts',(-23.72960637113,1.58159825017358,12.));
#236036=CARTESIAN_POINT('Ctrl Pts',(-23.710082626383,1.58668922481221,0.));
#236037=CARTESIAN_POINT('Ctrl Pts',(-23.710082626383,1.58668922481221,12.));
#236038=CARTESIAN_POINT('Ctrl Pts',(-23.6906508338833,1.59170048908633,
0.));
#236039=CARTESIAN_POINT('Ctrl Pts',(-23.6906508338833,1.59170048908633,
12.));
#236040=CARTESIAN_POINT('Ctrl Pts',(-23.671311958631,1.59663225222463,0.));
#236041=CARTESIAN_POINT('Ctrl Pts',(-23.671311958631,1.59663225222463,12.));
#236042=CARTESIAN_POINT('Ctrl Pts',(-23.6520669774876,1.60148472786595,
0.));
#236043=CARTESIAN_POINT('Ctrl Pts',(-23.6520669774876,1.60148472786595,
12.));
#236044=CARTESIAN_POINT('Ctrl Pts',(-23.6329168794929,1.60625813414672,
0.));
#236045=CARTESIAN_POINT('Ctrl Pts',(-23.6329168794929,1.60625813414672,
12.));
#236046=CARTESIAN_POINT('Ctrl Pts',(-23.6138626661653,1.61095269379778,
0.));
#236047=CARTESIAN_POINT('Ctrl Pts',(-23.6138626661653,1.61095269379778,
12.));
#236048=CARTESIAN_POINT('Ctrl Pts',(-23.5949053517997,1.61556863424698,
0.));
#236049=CARTESIAN_POINT('Ctrl Pts',(-23.5949053517997,1.61556863424698,
12.));
#236050=CARTESIAN_POINT('Ctrl Pts',(-23.57604596376,1.62010618772866,0.));
#236051=CARTESIAN_POINT('Ctrl Pts',(-23.57604596376,1.62010618772866,12.));
#236052=CARTESIAN_POINT('Ctrl Pts',(-23.5572855427601,1.62456559140064,
0.));
#236053=CARTESIAN_POINT('Ctrl Pts',(-23.5572855427601,1.62456559140064,
12.));
#236054=CARTESIAN_POINT('Ctrl Pts',(-23.538625143226,1.62894708745223,0.));
#236055=CARTESIAN_POINT('Ctrl Pts',(-23.538625143226,1.62894708745223,12.));
#236056=CARTESIAN_POINT('Ctrl Pts',(-23.5200658336612,1.63325092321725,
0.));
#236057=CARTESIAN_POINT('Ctrl Pts',(-23.5200658336612,1.63325092321725,
12.));
#236058=CARTESIAN_POINT('Ctrl Pts',(-23.5016086970003,1.63747735129474,
0.));
#236059=CARTESIAN_POINT('Ctrl Pts',(-23.5016086970003,1.63747735129474,
12.));
#236060=CARTESIAN_POINT('Ctrl Pts',(-23.4832548309645,1.64162662967528,
0.));
#236061=CARTESIAN_POINT('Ctrl Pts',(-23.4832548309645,1.64162662967528,
12.));
#236062=CARTESIAN_POINT('Ctrl Pts',(-23.4650053483932,1.64569902187611,
0.));
#236063=CARTESIAN_POINT('Ctrl Pts',(-23.4650053483932,1.64569902187611,
12.));
#236064=CARTESIAN_POINT('Ctrl Pts',(-23.4468613776574,1.6496947970734,0.));
#236065=CARTESIAN_POINT('Ctrl Pts',(-23.4468613776574,1.6496947970734,12.));
#236066=CARTESIAN_POINT('Ctrl Pts',(-23.4288240631043,1.65361423023728,
0.));
#236067=CARTESIAN_POINT('Ctrl Pts',(-23.4288240631043,1.65361423023728,
12.));
#236068=CARTESIAN_POINT('Ctrl Pts',(-23.4108945654805,1.65745760227505,
0.));
#236069=CARTESIAN_POINT('Ctrl Pts',(-23.4108945654805,1.65745760227505,
12.));
#236070=CARTESIAN_POINT('Ctrl Pts',(-23.3930740623619,1.66122520018011,
0.));
#236071=CARTESIAN_POINT('Ctrl Pts',(-23.3930740623619,1.66122520018011,
12.));
#236072=CARTESIAN_POINT('Ctrl Pts',(-23.3753637485545,1.66491731718876,
0.));
#236073=CARTESIAN_POINT('Ctrl Pts',(-23.3753637485545,1.66491731718876,
12.));
#236074=CARTESIAN_POINT('Ctrl Pts',(-23.3577648365744,1.66853425293995,
0.));
#236075=CARTESIAN_POINT('Ctrl Pts',(-23.3577648365744,1.66853425293995,
12.));
#236076=CARTESIAN_POINT('Ctrl Pts',(-23.3402785571865,1.67207631363921,
0.));
#236077=CARTESIAN_POINT('Ctrl Pts',(-23.3402785571865,1.67207631363921,
12.));
#236078=CARTESIAN_POINT('Ctrl Pts',(-23.3229061599145,1.67554381222994,
0.));
#236079=CARTESIAN_POINT('Ctrl Pts',(-23.3229061599145,1.67554381222994,
12.));
#236080=CARTESIAN_POINT('Ctrl Pts',(-23.3056489135611,1.67893706857117,
0.));
#236081=CARTESIAN_POINT('Ctrl Pts',(-23.3056489135611,1.67893706857117,
12.));
#236082=CARTESIAN_POINT('Ctrl Pts',(-23.2885081066951,1.68225640962168,
0.));
#236083=CARTESIAN_POINT('Ctrl Pts',(-23.2885081066951,1.68225640962168,
12.));
#236084=CARTESIAN_POINT('Ctrl Pts',(-23.2714850482246,1.68550216963258,
0.));
#236085=CARTESIAN_POINT('Ctrl Pts',(-23.2714850482246,1.68550216963258,
12.));
#236086=CARTESIAN_POINT('Ctrl Pts',(-23.2545810680537,1.68867469034896,
0.));
#236087=CARTESIAN_POINT('Ctrl Pts',(-23.2545810680537,1.68867469034896,
12.));
#236088=CARTESIAN_POINT('Ctrl Pts',(-23.2377975177013,1.69177432121711,
0.));
#236089=CARTESIAN_POINT('Ctrl Pts',(-23.2377975177013,1.69177432121711,
12.));
#236090=CARTESIAN_POINT('Ctrl Pts',(-23.2211357709374,1.69480141959953,
0.));
#236091=CARTESIAN_POINT('Ctrl Pts',(-23.2211357709374,1.69480141959953,
12.));
#236092=CARTESIAN_POINT('Ctrl Pts',(-23.2045972243767,1.69775635099443,
0.));
#236093=CARTESIAN_POINT('Ctrl Pts',(-23.2045972243767,1.69775635099443,
12.));
#236094=CARTESIAN_POINT('Ctrl Pts',(-23.1881832981851,1.7006394892701,0.));
#236095=CARTESIAN_POINT('Ctrl Pts',(-23.1881832981851,1.7006394892701,12.));
#236096=CARTESIAN_POINT('Ctrl Pts',(-23.1718954368751,1.70345121691276,
0.));
#236097=CARTESIAN_POINT('Ctrl Pts',(-23.1718954368751,1.70345121691276,
12.));
#236098=CARTESIAN_POINT('Ctrl Pts',(-23.1557351100614,1.70619192527852,
0.));
#236099=CARTESIAN_POINT('Ctrl Pts',(-23.1557351100614,1.70619192527852,
12.));
#236100=CARTESIAN_POINT('Ctrl Pts',(-23.1397038132356,1.70886201485452,
0.));
#236101=CARTESIAN_POINT('Ctrl Pts',(-23.1397038132356,1.70886201485452,
12.));
#236102=CARTESIAN_POINT('Ctrl Pts',(-23.1238030684925,1.71146189552174,
0.));
#236103=CARTESIAN_POINT('Ctrl Pts',(-23.1238030684925,1.71146189552174,
12.));
#236104=CARTESIAN_POINT('Ctrl Pts',(-23.1080344254286,1.71399198684704,
0.));
#236105=CARTESIAN_POINT('Ctrl Pts',(-23.1080344254286,1.71399198684704,
12.));
#236106=CARTESIAN_POINT('Ctrl Pts',(-23.0923994621213,1.71645271839296,
0.));
#236107=CARTESIAN_POINT('Ctrl Pts',(-23.0923994621213,1.71645271839296,
12.));
#236108=CARTESIAN_POINT('Ctrl Pts',(-23.0768997860709,1.71884453003027,
0.));
#236109=CARTESIAN_POINT('Ctrl Pts',(-23.0768997860709,1.71884453003027,
12.));
#236110=CARTESIAN_POINT('Ctrl Pts',(-23.0615370351562,1.72116787225991,
0.));
#236111=CARTESIAN_POINT('Ctrl Pts',(-23.0615370351562,1.72116787225991,
12.));
#236112=CARTESIAN_POINT('Ctrl Pts',(-23.0463128785531,1.72342320653746,
0.));
#236113=CARTESIAN_POINT('Ctrl Pts',(-23.0463128785531,1.72342320653746,
12.));
#236114=CARTESIAN_POINT('Ctrl Pts',(-23.0312290178883,1.72561100564045,
0.));
#236115=CARTESIAN_POINT('Ctrl Pts',(-23.0312290178883,1.72561100564045,
12.));
#236116=CARTESIAN_POINT('Ctrl Pts',(-23.0162871884168,1.72773175404708,
0.));
#236117=CARTESIAN_POINT('Ctrl Pts',(-23.0162871884168,1.72773175404708,
12.));
#236118=CARTESIAN_POINT('Ctrl Pts',(-23.001489160189,1.72978594832136,0.));
#236119=CARTESIAN_POINT('Ctrl Pts',(-23.001489160189,1.72978594832136,12.));
#236120=CARTESIAN_POINT('Ctrl Pts',(-22.9868367391978,1.7317740975019,0.));
#236121=CARTESIAN_POINT('Ctrl Pts',(-22.9868367391978,1.7317740975019,12.));
#236122=CARTESIAN_POINT('Ctrl Pts',(-22.9723317685688,1.73369672350814,
0.));
#236123=CARTESIAN_POINT('Ctrl Pts',(-22.9723317685688,1.73369672350814,
12.));
#236124=CARTESIAN_POINT('Ctrl Pts',(-22.9579761301063,1.73555436162769,
0.));
#236125=CARTESIAN_POINT('Ctrl Pts',(-22.9579761301063,1.73555436162769,
12.));
#236126=CARTESIAN_POINT('Ctrl Pts',(-22.9437717457826,1.73734756100039,
0.));
#236127=CARTESIAN_POINT('Ctrl Pts',(-22.9437717457826,1.73734756100039,
12.));
#236128=CARTESIAN_POINT('Ctrl Pts',(-22.9297205792586,1.73907688511666,
0.));
#236129=CARTESIAN_POINT('Ctrl Pts',(-22.9297205792586,1.73907688511666,
12.));
#236130=CARTESIAN_POINT('Ctrl Pts',(-22.9158246373363,1.74074291231058,
0.));
#236131=CARTESIAN_POINT('Ctrl Pts',(-22.9158246373363,1.74074291231058,
12.));
#236132=CARTESIAN_POINT('Ctrl Pts',(-22.9020859716141,1.7423462363008,0.));
#236133=CARTESIAN_POINT('Ctrl Pts',(-22.9020859716141,1.7423462363008,12.));
#236134=CARTESIAN_POINT('Ctrl Pts',(-22.888506680335,1.74388746677702,0.));
#236135=CARTESIAN_POINT('Ctrl Pts',(-22.888506680335,1.74388746677702,12.));
#236136=CARTESIAN_POINT('Ctrl Pts',(-22.8750889101696,1.74536722998201,
0.));
#236137=CARTESIAN_POINT('Ctrl Pts',(-22.8750889101696,1.74536722998201,
12.));
#236138=CARTESIAN_POINT('Ctrl Pts',(-22.8618348580235,1.74678616930664,
0.));
#236139=CARTESIAN_POINT('Ctrl Pts',(-22.8618348580235,1.74678616930664,
12.));
#236140=CARTESIAN_POINT('Ctrl Pts',(-22.8487467728076,1.74814494588492,
0.));
#236141=CARTESIAN_POINT('Ctrl Pts',(-22.8487467728076,1.74814494588492,
12.));
#236142=CARTESIAN_POINT('Ctrl Pts',(-22.8358269579853,1.74944423940115,
0.));
#236143=CARTESIAN_POINT('Ctrl Pts',(-22.8358269579853,1.74944423940115,
12.));
#236144=CARTESIAN_POINT('Ctrl Pts',(-22.8230777741284,1.75068474890883,
0.));
#236145=CARTESIAN_POINT('Ctrl Pts',(-22.8230777741284,1.75068474890883,
12.));
#236146=CARTESIAN_POINT('Ctrl Pts',(-22.8105016414713,1.75186719365592,
0.));
#236147=CARTESIAN_POINT('Ctrl Pts',(-22.8105016414713,1.75186719365592,
12.));
#236148=CARTESIAN_POINT('Ctrl Pts',(-22.7981010424314,1.75299231391466,
0.));
#236149=CARTESIAN_POINT('Ctrl Pts',(-22.7981010424314,1.75299231391466,
12.));
#236150=CARTESIAN_POINT('Ctrl Pts',(-22.7858785242361,1.75406087182936,
0.));
#236151=CARTESIAN_POINT('Ctrl Pts',(-22.7858785242361,1.75406087182936,
12.));
#236152=CARTESIAN_POINT('Ctrl Pts',(-22.7738367016118,1.75507365227131,
0.));
#236153=CARTESIAN_POINT('Ctrl Pts',(-22.7738367016118,1.75507365227131,
12.));
#236154=CARTESIAN_POINT('Ctrl Pts',(-22.7619782595013,1.75603146371641,
0.));
#236155=CARTESIAN_POINT('Ctrl Pts',(-22.7619782595013,1.75603146371641,
12.));
#236156=CARTESIAN_POINT('Ctrl Pts',(-22.750305955645,1.75693513908907,0.));
#236157=CARTESIAN_POINT('Ctrl Pts',(-22.750305955645,1.75693513908907,12.));
#236158=CARTESIAN_POINT('Ctrl Pts',(-22.7388226235559,1.75778553673244,
0.));
#236159=CARTESIAN_POINT('Ctrl Pts',(-22.7388226235559,1.75778553673244,
12.));
#236160=CARTESIAN_POINT('Ctrl Pts',(-22.72753117773,1.75858354204633,0.));
#236161=CARTESIAN_POINT('Ctrl Pts',(-22.72753117773,1.75858354204633,12.));
#236162=CARTESIAN_POINT('Ctrl Pts',(-22.7164346186006,1.75933006905925,
0.));
#236163=CARTESIAN_POINT('Ctrl Pts',(-22.7164346186006,1.75933006905925,
12.));
#236164=CARTESIAN_POINT('Ctrl Pts',(-22.7055360375485,1.76002606202401,
0.));
#236165=CARTESIAN_POINT('Ctrl Pts',(-22.7055360375485,1.76002606202401,
12.));
#236166=CARTESIAN_POINT('Ctrl Pts',(-22.6948386219851,1.76067249704886,
0.));
#236167=CARTESIAN_POINT('Ctrl Pts',(-22.6948386219851,1.76067249704886,
12.));
#236168=CARTESIAN_POINT('Ctrl Pts',(-22.684345658525,1.76127038310614,0.));
#236169=CARTESIAN_POINT('Ctrl Pts',(-22.684345658525,1.76127038310614,12.));
#236170=CARTESIAN_POINT('Ctrl Pts',(-22.67406053567,1.76182076289525,0.));
#236171=CARTESIAN_POINT('Ctrl Pts',(-22.67406053567,1.76182076289525,12.));
#236172=CARTESIAN_POINT('Ctrl Pts',(-22.6639867471753,1.76232471392568,
0.));
#236173=CARTESIAN_POINT('Ctrl Pts',(-22.6639867471753,1.76232471392568,
12.));
#236174=CARTESIAN_POINT('Ctrl Pts',(-22.6541278938409,1.76278334912561,
0.));
#236175=CARTESIAN_POINT('Ctrl Pts',(-22.6541278938409,1.76278334912561,
12.));
#236176=CARTESIAN_POINT('Ctrl Pts',(-22.6444876940423,1.76319782013916,
0.));
#236177=CARTESIAN_POINT('Ctrl Pts',(-22.6444876940423,1.76319782013916,
12.));
#236178=CARTESIAN_POINT('Ctrl Pts',(-22.6350699979359,1.76356932176273,
0.));
#236179=CARTESIAN_POINT('Ctrl Pts',(-22.6350699979359,1.76356932176273,
12.));
#236180=CARTESIAN_POINT('Ctrl Pts',(-22.6258787994848,1.76389909571403,
0.));
#236181=CARTESIAN_POINT('Ctrl Pts',(-22.6258787994848,1.76389909571403,
12.));
#236182=CARTESIAN_POINT('Ctrl Pts',(-22.6169182517694,1.76418843543739,
0.));
#236183=CARTESIAN_POINT('Ctrl Pts',(-22.6169182517694,1.76418843543739,
12.));
#236184=CARTESIAN_POINT('Ctrl Pts',(-22.6081926681343,1.76443868648015,
0.));
#236185=CARTESIAN_POINT('Ctrl Pts',(-22.6081926681343,1.76443868648015,
12.));
#236186=CARTESIAN_POINT('Ctrl Pts',(-22.5997065145638,1.76465124413557,
0.));
#236187=CARTESIAN_POINT('Ctrl Pts',(-22.5997065145638,1.76465124413557,
12.));
#236188=CARTESIAN_POINT('Ctrl Pts',(-22.5914644078106,1.76482755288411,
0.));
#236189=CARTESIAN_POINT('Ctrl Pts',(-22.5914644078106,1.76482755288411,
12.));
#236190=CARTESIAN_POINT('Ctrl Pts',(-22.5834711038022,1.76496910283088,
0.));
#236191=CARTESIAN_POINT('Ctrl Pts',(-22.5834711038022,1.76496910283088,
12.));
#236192=CARTESIAN_POINT('Ctrl Pts',(-22.5757315316353,1.76507744026746,
0.));
#236193=CARTESIAN_POINT('Ctrl Pts',(-22.5757315316353,1.76507744026746,
12.));
#236194=CARTESIAN_POINT('Ctrl Pts',(-22.5682508499873,1.76515418518831,
0.));
#236195=CARTESIAN_POINT('Ctrl Pts',(-22.5682508499873,1.76515418518831,
12.));
#236196=CARTESIAN_POINT('Ctrl Pts',(-22.5610344912501,1.7652010450045,0.));
#236197=CARTESIAN_POINT('Ctrl Pts',(-22.5610344912501,1.7652010450045,12.));
#236198=CARTESIAN_POINT('Ctrl Pts',(-22.5540882235837,1.76521983384062,
0.));
#236199=CARTESIAN_POINT('Ctrl Pts',(-22.5540882235837,1.76521983384062,
12.));
#236200=CARTESIAN_POINT('Ctrl Pts',(-22.5474180954006,1.76521245524047,
0.));
#236201=CARTESIAN_POINT('Ctrl Pts',(-22.5474180954006,1.76521245524047,
12.));
#236202=CARTESIAN_POINT('Ctrl Pts',(-22.5410303590892,1.76518087841493,
0.));
#236203=CARTESIAN_POINT('Ctrl Pts',(-22.5410303590892,1.76518087841493,
12.));
#236204=CARTESIAN_POINT('Ctrl Pts',(-22.5349313983571,1.76512711563254,
0.));
#236205=CARTESIAN_POINT('Ctrl Pts',(-22.5349313983571,1.76512711563254,
12.));
#236206=CARTESIAN_POINT('Ctrl Pts',(-22.529127665298,1.76505320262759,0.));
#236207=CARTESIAN_POINT('Ctrl Pts',(-22.529127665298,1.76505320262759,12.));
#236208=CARTESIAN_POINT('Ctrl Pts',(-22.5236259635515,1.76496128643375,
0.));
#236209=CARTESIAN_POINT('Ctrl Pts',(-22.5236259635515,1.76496128643375,
12.));
#236210=CARTESIAN_POINT('Ctrl Pts',(-22.5184336670207,1.76485369319895,
0.));
#236211=CARTESIAN_POINT('Ctrl Pts',(-22.5184336670207,1.76485369319895,
12.));
#236212=CARTESIAN_POINT('Ctrl Pts',(-22.5135590569554,1.76473303281149,
0.));
#236213=CARTESIAN_POINT('Ctrl Pts',(-22.5135590569554,1.76473303281149,
12.));
#236214=CARTESIAN_POINT('Ctrl Pts',(-22.5090112700212,1.76460218257313,
0.));
#236215=CARTESIAN_POINT('Ctrl Pts',(-22.5090112700212,1.76460218257313,
12.));
#236216=CARTESIAN_POINT('Ctrl Pts',(-22.5047996391978,1.76446408210364,
0.));
#236217=CARTESIAN_POINT('Ctrl Pts',(-22.5047996391978,1.76446408210364,
12.));
#236218=CARTESIAN_POINT('Ctrl Pts',(-22.5009332677316,1.76432160068737,
0.));
#236219=CARTESIAN_POINT('Ctrl Pts',(-22.5009332677316,1.76432160068737,
12.));
#236220=CARTESIAN_POINT('Ctrl Pts',(-22.4974203063191,1.76417731243483,
0.));
#236221=CARTESIAN_POINT('Ctrl Pts',(-22.4974203063191,1.76417731243483,
12.));
#236222=CARTESIAN_POINT('Ctrl Pts',(-22.4942693792449,1.76403393880316,
0.));
#236223=CARTESIAN_POINT('Ctrl Pts',(-22.4942693792449,1.76403393880316,
12.));
#236224=CARTESIAN_POINT('Ctrl Pts',(-22.4914909094908,1.76389475965714,
0.));
#236225=CARTESIAN_POINT('Ctrl Pts',(-22.4914909094908,1.76389475965714,
12.));
#236226=CARTESIAN_POINT('Ctrl Pts',(-22.4890991659479,1.76376424879468,
0.));
#236227=CARTESIAN_POINT('Ctrl Pts',(-22.4890991659479,1.76376424879468,
12.));
#236228=CARTESIAN_POINT('Ctrl Pts',(-22.4871115206572,1.76364784232925,
0.));
#236229=CARTESIAN_POINT('Ctrl Pts',(-22.4871115206572,1.76364784232925,
12.));
#236230=CARTESIAN_POINT('Ctrl Pts',(-22.4855446605991,1.76355076045549,
0.));
#236231=CARTESIAN_POINT('Ctrl Pts',(-22.4855446605991,1.76355076045549,
12.));
#236232=CARTESIAN_POINT('Ctrl Pts',(-22.4844112933125,1.76347698284861,
0.));
#236233=CARTESIAN_POINT('Ctrl Pts',(-22.4844112933125,1.76347698284861,
12.));
#236234=CARTESIAN_POINT('Ctrl Pts',(-22.4838562517064,1.76343813434659,
0.));
#236235=CARTESIAN_POINT('Ctrl Pts',(-22.4838562517064,1.76343813434659,
12.));
#236236=CARTESIAN_POINT('Ctrl Pts',(-22.4836387052228,1.76342064263637,
0.));
#236237=CARTESIAN_POINT('Ctrl Pts',(-22.4836387052228,1.76342064263637,
12.));
#236238=CARTESIAN_POINT('Ctrl Pts',(-22.4835819929788,1.7634141553879,0.));
#236239=CARTESIAN_POINT('Ctrl Pts',(-22.4835819929788,1.7634141553879,12.));
#236240=CARTESIAN_POINT('Ctrl Pts',(-22.4835757167854,1.7634122053118,0.));
#236241=CARTESIAN_POINT('Ctrl Pts',(-22.4835757167854,1.7634122053118,12.));
#236242=CARTESIAN_POINT('',(-25.991588367311,0.661312440730901,0.));
#236243=CARTESIAN_POINT('Ctrl Pts',(-25.991588367311,0.661312440730901,
0.));
#236244=CARTESIAN_POINT('Ctrl Pts',(-25.9865613464773,0.664028313187627,
0.));
#236245=CARTESIAN_POINT('Ctrl Pts',(-25.9765104298071,0.669451306780825,
0.));
#236246=CARTESIAN_POINT('Ctrl Pts',(-25.9614434297919,0.677559543209725,
0.));
#236247=CARTESIAN_POINT('Ctrl Pts',(-25.9413728471909,0.688318015057729,
0.));
#236248=CARTESIAN_POINT('Ctrl Pts',(-25.9163158909426,0.701678575228756,
0.));
#236249=CARTESIAN_POINT('Ctrl Pts',(-25.891290261497,0.714951588527638,
0.));
#236250=CARTESIAN_POINT('Ctrl Pts',(-25.8662960624185,0.728137036482335,
0.));
#236251=CARTESIAN_POINT('Ctrl Pts',(-25.8413334619055,0.741234902663807,
0.));
#236252=CARTESIAN_POINT('Ctrl Pts',(-25.8164027059984,0.754245175609524,
0.));
#236253=CARTESIAN_POINT('Ctrl Pts',(-25.7915041383376,0.767167852651168,
0.));
#236254=CARTESIAN_POINT('Ctrl Pts',(-25.7666381946955,0.780002940291965,
0.));
#236255=CARTESIAN_POINT('Ctrl Pts',(-25.7418053757746,0.792750451616127,
0.));
#236256=CARTESIAN_POINT('Ctrl Pts',(-25.7170062262525,0.805410404554352,
0.));
#236257=CARTESIAN_POINT('Ctrl Pts',(-25.6922413110194,0.817982819787464,
0.));
#236258=CARTESIAN_POINT('Ctrl Pts',(-25.6675111931952,0.830467718864205,
0.));
#236259=CARTESIAN_POINT('Ctrl Pts',(-25.6428164100055,0.842865122120758,
0.));
#236260=CARTESIAN_POINT('Ctrl Pts',(-25.6181574536049,0.855175047036549,
0.));
#236261=CARTESIAN_POINT('Ctrl Pts',(-25.5935347843585,0.867397509338431,
0.));
#236262=CARTESIAN_POINT('Ctrl Pts',(-25.5689488408156,0.879532523834294,
0.));
#236263=CARTESIAN_POINT('Ctrl Pts',(-25.5444000508211,0.89158010534904,
0.));
#236264=CARTESIAN_POINT('Ctrl Pts',(-25.5198888424194,0.903540269651106,
0.));
#236265=CARTESIAN_POINT('Ctrl Pts',(-25.4954156541795,0.915413034335613,
0.));
#236266=CARTESIAN_POINT('Ctrl Pts',(-25.4709809475009,0.927198419886094,
0.));
#236267=CARTESIAN_POINT('Ctrl Pts',(-25.4465852044849,0.938896449496192,
0.));
#236268=CARTESIAN_POINT('Ctrl Pts',(-25.4222289223167,0.950507148597468,
0.));
#236269=CARTESIAN_POINT('Ctrl Pts',(-25.3979126089163,0.962030544503142,
0.));
#236270=CARTESIAN_POINT('Ctrl Pts',(-25.3736367778845,0.973466666000163,
0.));
#236271=CARTESIAN_POINT('Ctrl Pts',(-25.3494019441441,0.984815543003973,
0.));
#236272=CARTESIAN_POINT('Ctrl Pts',(-25.3252086182968,0.996077206120624,
0.));
#236273=CARTESIAN_POINT('Ctrl Pts',(-25.3010573055547,1.00725168656896,
0.));
#236274=CARTESIAN_POINT('Ctrl Pts',(-25.276948508726,1.01833901642237,0.));
#236275=CARTESIAN_POINT('Ctrl Pts',(-25.2528827300422,1.02933922876806,
0.));
#236276=CARTESIAN_POINT('Ctrl Pts',(-25.2288604735086,1.04025235791507,
0.));
#236277=CARTESIAN_POINT('Ctrl Pts',(-25.2048822469028,1.05107843957931,
0.));
#236278=CARTESIAN_POINT('Ctrl Pts',(-25.1809485642192,1.06181751111768,
0.));
#236279=CARTESIAN_POINT('Ctrl Pts',(-25.157059946931,1.07246961165475,0.));
#236280=CARTESIAN_POINT('Ctrl Pts',(-25.1332169227413,1.08303478197187,
0.));
#236281=CARTESIAN_POINT('Ctrl Pts',(-25.1094200248446,1.09351306445308,
0.));
#236282=CARTESIAN_POINT('Ctrl Pts',(-25.0856697909679,1.10390450301745,
0.));
#236283=CARTESIAN_POINT('Ctrl Pts',(-25.0619667625336,1.11420914306889,
0.));
#236284=CARTESIAN_POINT('Ctrl Pts',(-25.0383114836899,1.12442703144451,
0.));
#236285=CARTESIAN_POINT('Ctrl Pts',(-25.0147045006196,1.1345582163853,0.));
#236286=CARTESIAN_POINT('Ctrl Pts',(-24.9911463621433,1.144602747582,0.));
#236287=CARTESIAN_POINT('Ctrl Pts',(-24.9676376201502,1.15456067621889,
0.));
#236288=CARTESIAN_POINT('Ctrl Pts',(-24.9441788300932,1.16443205502849,
0.));
#236289=CARTESIAN_POINT('Ctrl Pts',(-24.9207705514449,1.17421693835041,
0.));
#236290=CARTESIAN_POINT('Ctrl Pts',(-24.8974133481829,1.18391538220103,
0.));
#236291=CARTESIAN_POINT('Ctrl Pts',(-24.8741077892075,1.19352744434064,
0.));
#236292=CARTESIAN_POINT('Ctrl Pts',(-24.8508544481974,1.2030531842602,0.));
#236293=CARTESIAN_POINT('Ctrl Pts',(-24.8276539035092,1.21249266318208,
0.));
#236294=CARTESIAN_POINT('Ctrl Pts',(-24.8045067380536,1.22184594406528,
0.));
#236295=CARTESIAN_POINT('Ctrl Pts',(-24.7814135391799,1.23111309161843,
0.));
#236296=CARTESIAN_POINT('Ctrl Pts',(-24.7583748985438,1.24029417231989,
0.));
#236297=CARTESIAN_POINT('Ctrl Pts',(-24.7353914120011,1.24938925444325,
0.));
#236298=CARTESIAN_POINT('Ctrl Pts',(-24.7124636797894,1.25839840807418,
0.));
#236299=CARTESIAN_POINT('Ctrl Pts',(-24.6895923066836,1.267321705135,0.));
#236300=CARTESIAN_POINT('Ctrl Pts',(-24.666777902156,1.27615921941642,0.));
#236301=CARTESIAN_POINT('Ctrl Pts',(-24.6440210805278,1.28491102661514,
0.));
#236302=CARTESIAN_POINT('Ctrl Pts',(-24.6213224611229,1.29357720438107,
0.));
#236303=CARTESIAN_POINT('Ctrl Pts',(-24.5986826684027,1.30215783236362,
0.));
#236304=CARTESIAN_POINT('Ctrl Pts',(-24.5761023320183,1.31065299222021,
0.));
#236305=CARTESIAN_POINT('Ctrl Pts',(-24.5535820868674,1.31906276763668,
0.));
#236306=CARTESIAN_POINT('Ctrl Pts',(-24.5311225731435,1.32738724435326,
0.));
#236307=CARTESIAN_POINT('Ctrl Pts',(-24.5087244363856,1.33562651019686,
0.));
#236308=CARTESIAN_POINT('Ctrl Pts',(-24.4863883275134,1.34378065512337,
0.));
#236309=CARTESIAN_POINT('Ctrl Pts',(-24.4641149028892,1.35184977125648,
0.));
#236310=CARTESIAN_POINT('Ctrl Pts',(-24.4419048244523,1.35983395290627,
0.));
#236311=CARTESIAN_POINT('Ctrl Pts',(-24.4197587598337,1.36773329659956,
0.));
#236312=CARTESIAN_POINT('Ctrl Pts',(-24.3976773824732,1.37554790111609,
0.));
#236313=CARTESIAN_POINT('Ctrl Pts',(-24.3756613717299,1.38327786752998,
0.));
#236314=CARTESIAN_POINT('Ctrl Pts',(-24.3537114129875,1.39092329926388,
0.));
#236315=CARTESIAN_POINT('Ctrl Pts',(-24.3318281977643,1.39848430212807,
0.));
#236316=CARTESIAN_POINT('Ctrl Pts',(-24.3100124238311,1.40596098434337,
0.));
#236317=CARTESIAN_POINT('Ctrl Pts',(-24.288264795321,1.41335345657682,0.));
#236318=CARTESIAN_POINT('Ctrl Pts',(-24.2665860228356,1.42066183198252,
0.));
#236319=CARTESIAN_POINT('Ctrl Pts',(-24.2449768235488,1.42788622624854,
0.));
#236320=CARTESIAN_POINT('Ctrl Pts',(-24.2234379212984,1.43502675765508,
0.));
#236321=CARTESIAN_POINT('Ctrl Pts',(-24.201970046722,1.44208354711082,0.));
#236322=CARTESIAN_POINT('Ctrl Pts',(-24.1805739374038,1.44905671818727,
0.));
#236323=CARTESIAN_POINT('Ctrl Pts',(-24.1592503380107,1.45594639716317,
0.));
#236324=CARTESIAN_POINT('Ctrl Pts',(-24.1380000004272,1.46275271307397,
0.));
#236325=CARTESIAN_POINT('Ctrl Pts',(-24.1168236838824,1.46947579776991,
0.));
#236326=CARTESIAN_POINT('Ctrl Pts',(-24.0957221550778,1.47611578597742,
0.));
#236327=CARTESIAN_POINT('Ctrl Pts',(-24.0746961883528,1.48267281533683,
0.));
#236328=CARTESIAN_POINT('Ctrl Pts',(-24.0537465658429,1.48914702644887,
0.));
#236329=CARTESIAN_POINT('Ctrl Pts',(-24.0328740776331,1.49553856292801,
0.));
#236330=CARTESIAN_POINT('Ctrl Pts',(-24.0120795219086,1.50184757146098,
0.));
#236331=CARTESIAN_POINT('Ctrl Pts',(-23.9913637050927,1.50807420187694,
0.));
#236332=CARTESIAN_POINT('Ctrl Pts',(-23.970727442014,1.51421860720614,0.));
#236333=CARTESIAN_POINT('Ctrl Pts',(-23.9501715561033,1.52028094372792,
0.));
#236334=CARTESIAN_POINT('Ctrl Pts',(-23.9296968795757,1.52626137103032,
0.));
#236335=CARTESIAN_POINT('Ctrl Pts',(-23.9093042536119,1.53216005207463,
0.));
#236336=CARTESIAN_POINT('Ctrl Pts',(-23.8889945285318,1.53797715326758,
0.));
#236337=CARTESIAN_POINT('Ctrl Pts',(-23.8687685639642,1.5437128445399,0.));
#236338=CARTESIAN_POINT('Ctrl Pts',(-23.8486272290705,1.54936729940541,
0.));
#236339=CARTESIAN_POINT('Ctrl Pts',(-23.8285714027636,1.55494069502635,
0.));
#236340=CARTESIAN_POINT('Ctrl Pts',(-23.8086019739194,1.56043321228633,
0.));
#236341=CARTESIAN_POINT('Ctrl Pts',(-23.7887198415878,1.56584503586843,
0.));
#236342=CARTESIAN_POINT('Ctrl Pts',(-23.7689259151862,1.57117635434408,
0.));
#236343=CARTESIAN_POINT('Ctrl Pts',(-23.749221114736,1.57642736025246,0.));
#236344=CARTESIAN_POINT('Ctrl Pts',(-23.72960637113,1.58159825017358,0.));
#236345=CARTESIAN_POINT('Ctrl Pts',(-23.710082626383,1.58668922481221,0.));
#236346=CARTESIAN_POINT('Ctrl Pts',(-23.6906508338833,1.59170048908633,
0.));
#236347=CARTESIAN_POINT('Ctrl Pts',(-23.671311958631,1.59663225222463,0.));
#236348=CARTESIAN_POINT('Ctrl Pts',(-23.6520669774876,1.60148472786595,
0.));
#236349=CARTESIAN_POINT('Ctrl Pts',(-23.6329168794929,1.60625813414672,
0.));
#236350=CARTESIAN_POINT('Ctrl Pts',(-23.6138626661653,1.61095269379778,
0.));
#236351=CARTESIAN_POINT('Ctrl Pts',(-23.5949053517997,1.61556863424698,
0.));
#236352=CARTESIAN_POINT('Ctrl Pts',(-23.57604596376,1.62010618772866,0.));
#236353=CARTESIAN_POINT('Ctrl Pts',(-23.5572855427601,1.62456559140064,
0.));
#236354=CARTESIAN_POINT('Ctrl Pts',(-23.538625143226,1.62894708745223,0.));
#236355=CARTESIAN_POINT('Ctrl Pts',(-23.5200658336612,1.63325092321725,
0.));
#236356=CARTESIAN_POINT('Ctrl Pts',(-23.5016086970003,1.63747735129474,
0.));
#236357=CARTESIAN_POINT('Ctrl Pts',(-23.4832548309645,1.64162662967528,
0.));
#236358=CARTESIAN_POINT('Ctrl Pts',(-23.4650053483932,1.64569902187611,
0.));
#236359=CARTESIAN_POINT('Ctrl Pts',(-23.4468613776574,1.6496947970734,0.));
#236360=CARTESIAN_POINT('Ctrl Pts',(-23.4288240631043,1.65361423023728,
0.));
#236361=CARTESIAN_POINT('Ctrl Pts',(-23.4108945654805,1.65745760227505,
0.));
#236362=CARTESIAN_POINT('Ctrl Pts',(-23.3930740623619,1.66122520018011,
0.));
#236363=CARTESIAN_POINT('Ctrl Pts',(-23.3753637485545,1.66491731718876,
0.));
#236364=CARTESIAN_POINT('Ctrl Pts',(-23.3577648365744,1.66853425293995,
0.));
#236365=CARTESIAN_POINT('Ctrl Pts',(-23.3402785571865,1.67207631363921,
0.));
#236366=CARTESIAN_POINT('Ctrl Pts',(-23.3229061599145,1.67554381222994,
0.));
#236367=CARTESIAN_POINT('Ctrl Pts',(-23.3056489135611,1.67893706857117,
0.));
#236368=CARTESIAN_POINT('Ctrl Pts',(-23.2885081066951,1.68225640962168,
0.));
#236369=CARTESIAN_POINT('Ctrl Pts',(-23.2714850482246,1.68550216963258,
0.));
#236370=CARTESIAN_POINT('Ctrl Pts',(-23.2545810680537,1.68867469034896,
0.));
#236371=CARTESIAN_POINT('Ctrl Pts',(-23.2377975177013,1.69177432121711,
0.));
#236372=CARTESIAN_POINT('Ctrl Pts',(-23.2211357709374,1.69480141959953,
0.));
#236373=CARTESIAN_POINT('Ctrl Pts',(-23.2045972243767,1.69775635099443,
0.));
#236374=CARTESIAN_POINT('Ctrl Pts',(-23.1881832981851,1.7006394892701,0.));
#236375=CARTESIAN_POINT('Ctrl Pts',(-23.1718954368751,1.70345121691276,
0.));
#236376=CARTESIAN_POINT('Ctrl Pts',(-23.1557351100614,1.70619192527852,
0.));
#236377=CARTESIAN_POINT('Ctrl Pts',(-23.1397038132356,1.70886201485452,
0.));
#236378=CARTESIAN_POINT('Ctrl Pts',(-23.1238030684925,1.71146189552174,
0.));
#236379=CARTESIAN_POINT('Ctrl Pts',(-23.1080344254286,1.71399198684704,
0.));
#236380=CARTESIAN_POINT('Ctrl Pts',(-23.0923994621213,1.71645271839296,
0.));
#236381=CARTESIAN_POINT('Ctrl Pts',(-23.0768997860709,1.71884453003027,
0.));
#236382=CARTESIAN_POINT('Ctrl Pts',(-23.0615370351562,1.72116787225991,
0.));
#236383=CARTESIAN_POINT('Ctrl Pts',(-23.0463128785531,1.72342320653746,
0.));
#236384=CARTESIAN_POINT('Ctrl Pts',(-23.0312290178883,1.72561100564045,
0.));
#236385=CARTESIAN_POINT('Ctrl Pts',(-23.0162871884168,1.72773175404708,
0.));
#236386=CARTESIAN_POINT('Ctrl Pts',(-23.001489160189,1.72978594832136,0.));
#236387=CARTESIAN_POINT('Ctrl Pts',(-22.9868367391978,1.7317740975019,0.));
#236388=CARTESIAN_POINT('Ctrl Pts',(-22.9723317685688,1.73369672350814,
0.));
#236389=CARTESIAN_POINT('Ctrl Pts',(-22.9579761301063,1.73555436162769,
0.));
#236390=CARTESIAN_POINT('Ctrl Pts',(-22.9437717457826,1.73734756100039,
0.));
#236391=CARTESIAN_POINT('Ctrl Pts',(-22.9297205792586,1.73907688511666,
0.));
#236392=CARTESIAN_POINT('Ctrl Pts',(-22.9158246373363,1.74074291231058,
0.));
#236393=CARTESIAN_POINT('Ctrl Pts',(-22.9020859716141,1.7423462363008,0.));
#236394=CARTESIAN_POINT('Ctrl Pts',(-22.888506680335,1.74388746677702,0.));
#236395=CARTESIAN_POINT('Ctrl Pts',(-22.8750889101696,1.74536722998201,
0.));
#236396=CARTESIAN_POINT('Ctrl Pts',(-22.8618348580235,1.74678616930664,
0.));
#236397=CARTESIAN_POINT('Ctrl Pts',(-22.8487467728076,1.74814494588492,
0.));
#236398=CARTESIAN_POINT('Ctrl Pts',(-22.8358269579853,1.74944423940115,
0.));
#236399=CARTESIAN_POINT('Ctrl Pts',(-22.8230777741284,1.75068474890883,
0.));
#236400=CARTESIAN_POINT('Ctrl Pts',(-22.8105016414713,1.75186719365592,
0.));
#236401=CARTESIAN_POINT('Ctrl Pts',(-22.7981010424314,1.75299231391466,
0.));
#236402=CARTESIAN_POINT('Ctrl Pts',(-22.7858785242361,1.75406087182936,
0.));
#236403=CARTESIAN_POINT('Ctrl Pts',(-22.7738367016118,1.75507365227131,
0.));
#236404=CARTESIAN_POINT('Ctrl Pts',(-22.7619782595013,1.75603146371641,
0.));
#236405=CARTESIAN_POINT('Ctrl Pts',(-22.750305955645,1.75693513908907,0.));
#236406=CARTESIAN_POINT('Ctrl Pts',(-22.7388226235559,1.75778553673244,
0.));
#236407=CARTESIAN_POINT('Ctrl Pts',(-22.72753117773,1.75858354204633,0.));
#236408=CARTESIAN_POINT('Ctrl Pts',(-22.7164346186006,1.75933006905925,
0.));
#236409=CARTESIAN_POINT('Ctrl Pts',(-22.7055360375485,1.76002606202401,
0.));
#236410=CARTESIAN_POINT('Ctrl Pts',(-22.6948386219851,1.76067249704886,
0.));
#236411=CARTESIAN_POINT('Ctrl Pts',(-22.684345658525,1.76127038310614,0.));
#236412=CARTESIAN_POINT('Ctrl Pts',(-22.67406053567,1.76182076289525,0.));
#236413=CARTESIAN_POINT('Ctrl Pts',(-22.6639867471753,1.76232471392568,
0.));
#236414=CARTESIAN_POINT('Ctrl Pts',(-22.6541278938409,1.76278334912561,
0.));
#236415=CARTESIAN_POINT('Ctrl Pts',(-22.6444876940423,1.76319782013916,
0.));
#236416=CARTESIAN_POINT('Ctrl Pts',(-22.6350699979359,1.76356932176273,
0.));
#236417=CARTESIAN_POINT('Ctrl Pts',(-22.6258787994848,1.76389909571403,
0.));
#236418=CARTESIAN_POINT('Ctrl Pts',(-22.6169182517694,1.76418843543739,
0.));
#236419=CARTESIAN_POINT('Ctrl Pts',(-22.6081926681343,1.76443868648015,
0.));
#236420=CARTESIAN_POINT('Ctrl Pts',(-22.5997065145638,1.76465124413557,
0.));
#236421=CARTESIAN_POINT('Ctrl Pts',(-22.5914644078106,1.76482755288411,
0.));
#236422=CARTESIAN_POINT('Ctrl Pts',(-22.5834711038022,1.76496910283088,
0.));
#236423=CARTESIAN_POINT('Ctrl Pts',(-22.5757315316353,1.76507744026746,
0.));
#236424=CARTESIAN_POINT('Ctrl Pts',(-22.5682508499873,1.76515418518831,
0.));
#236425=CARTESIAN_POINT('Ctrl Pts',(-22.5610344912501,1.7652010450045,0.));
#236426=CARTESIAN_POINT('Ctrl Pts',(-22.5540882235837,1.76521983384062,
0.));
#236427=CARTESIAN_POINT('Ctrl Pts',(-22.5474180954006,1.76521245524047,
0.));
#236428=CARTESIAN_POINT('Ctrl Pts',(-22.5410303590892,1.76518087841493,
0.));
#236429=CARTESIAN_POINT('Ctrl Pts',(-22.5349313983571,1.76512711563254,
0.));
#236430=CARTESIAN_POINT('Ctrl Pts',(-22.529127665298,1.76505320262759,0.));
#236431=CARTESIAN_POINT('Ctrl Pts',(-22.5236259635515,1.76496128643375,
0.));
#236432=CARTESIAN_POINT('Ctrl Pts',(-22.5184336670207,1.76485369319895,
0.));
#236433=CARTESIAN_POINT('Ctrl Pts',(-22.5135590569554,1.76473303281149,
0.));
#236434=CARTESIAN_POINT('Ctrl Pts',(-22.5090112700212,1.76460218257313,
0.));
#236435=CARTESIAN_POINT('Ctrl Pts',(-22.5047996391978,1.76446408210364,
0.));
#236436=CARTESIAN_POINT('Ctrl Pts',(-22.5009332677316,1.76432160068737,
0.));
#236437=CARTESIAN_POINT('Ctrl Pts',(-22.4974203063191,1.76417731243483,
0.));
#236438=CARTESIAN_POINT('Ctrl Pts',(-22.4942693792449,1.76403393880316,
0.));
#236439=CARTESIAN_POINT('Ctrl Pts',(-22.4914909094908,1.76389475965714,
0.));
#236440=CARTESIAN_POINT('Ctrl Pts',(-22.4890991659479,1.76376424879468,
0.));
#236441=CARTESIAN_POINT('Ctrl Pts',(-22.4871115206572,1.76364784232925,
0.));
#236442=CARTESIAN_POINT('Ctrl Pts',(-22.4855446605991,1.76355076045549,
0.));
#236443=CARTESIAN_POINT('Ctrl Pts',(-22.4844112933125,1.76347698284861,
0.));
#236444=CARTESIAN_POINT('Ctrl Pts',(-22.4838562517064,1.76343813434659,
0.));
#236445=CARTESIAN_POINT('Ctrl Pts',(-22.4836387052228,1.76342064263637,
0.));
#236446=CARTESIAN_POINT('Ctrl Pts',(-22.4835819929788,1.7634141553879,0.));
#236447=CARTESIAN_POINT('Ctrl Pts',(-22.4835757167854,1.7634122053118,0.));
#236448=CARTESIAN_POINT('',(-25.991588367311,0.661312440730901,12.));
#236449=CARTESIAN_POINT('',(-25.991588367311,0.661312440730901,0.));
#236450=CARTESIAN_POINT('Ctrl Pts',(-22.4835757167854,1.7634122053118,12.));
#236451=CARTESIAN_POINT('Ctrl Pts',(-22.4835819929788,1.7634141553879,12.));
#236452=CARTESIAN_POINT('Ctrl Pts',(-22.4836387052228,1.76342064263637,
12.));
#236453=CARTESIAN_POINT('Ctrl Pts',(-22.4838562517064,1.76343813434659,
12.));
#236454=CARTESIAN_POINT('Ctrl Pts',(-22.4844112933125,1.76347698284861,
12.));
#236455=CARTESIAN_POINT('Ctrl Pts',(-22.4855446605991,1.76355076045549,
12.));
#236456=CARTESIAN_POINT('Ctrl Pts',(-22.4871115206572,1.76364784232925,
12.));
#236457=CARTESIAN_POINT('Ctrl Pts',(-22.4890991659479,1.76376424879468,
12.));
#236458=CARTESIAN_POINT('Ctrl Pts',(-22.4914909094908,1.76389475965714,
12.));
#236459=CARTESIAN_POINT('Ctrl Pts',(-22.4942693792449,1.76403393880316,
12.));
#236460=CARTESIAN_POINT('Ctrl Pts',(-22.4974203063191,1.76417731243483,
12.));
#236461=CARTESIAN_POINT('Ctrl Pts',(-22.5009332677316,1.76432160068737,
12.));
#236462=CARTESIAN_POINT('Ctrl Pts',(-22.5047996391978,1.76446408210364,
12.));
#236463=CARTESIAN_POINT('Ctrl Pts',(-22.5090112700212,1.76460218257313,
12.));
#236464=CARTESIAN_POINT('Ctrl Pts',(-22.5135590569554,1.76473303281149,
12.));
#236465=CARTESIAN_POINT('Ctrl Pts',(-22.5184336670207,1.76485369319895,
12.));
#236466=CARTESIAN_POINT('Ctrl Pts',(-22.5236259635515,1.76496128643375,
12.));
#236467=CARTESIAN_POINT('Ctrl Pts',(-22.529127665298,1.76505320262759,12.));
#236468=CARTESIAN_POINT('Ctrl Pts',(-22.5349313983571,1.76512711563254,
12.));
#236469=CARTESIAN_POINT('Ctrl Pts',(-22.5410303590892,1.76518087841493,
12.));
#236470=CARTESIAN_POINT('Ctrl Pts',(-22.5474180954006,1.76521245524047,
12.));
#236471=CARTESIAN_POINT('Ctrl Pts',(-22.5540882235837,1.76521983384062,
12.));
#236472=CARTESIAN_POINT('Ctrl Pts',(-22.5610344912501,1.7652010450045,12.));
#236473=CARTESIAN_POINT('Ctrl Pts',(-22.5682508499873,1.76515418518831,
12.));
#236474=CARTESIAN_POINT('Ctrl Pts',(-22.5757315316353,1.76507744026746,
12.));
#236475=CARTESIAN_POINT('Ctrl Pts',(-22.5834711038022,1.76496910283088,
12.));
#236476=CARTESIAN_POINT('Ctrl Pts',(-22.5914644078106,1.76482755288411,
12.));
#236477=CARTESIAN_POINT('Ctrl Pts',(-22.5997065145638,1.76465124413557,
12.));
#236478=CARTESIAN_POINT('Ctrl Pts',(-22.6081926681343,1.76443868648015,
12.));
#236479=CARTESIAN_POINT('Ctrl Pts',(-22.6169182517694,1.76418843543739,
12.));
#236480=CARTESIAN_POINT('Ctrl Pts',(-22.6258787994848,1.76389909571403,
12.));
#236481=CARTESIAN_POINT('Ctrl Pts',(-22.6350699979359,1.76356932176273,
12.));
#236482=CARTESIAN_POINT('Ctrl Pts',(-22.6444876940423,1.76319782013916,
12.));
#236483=CARTESIAN_POINT('Ctrl Pts',(-22.6541278938409,1.76278334912561,
12.));
#236484=CARTESIAN_POINT('Ctrl Pts',(-22.6639867471753,1.76232471392568,
12.));
#236485=CARTESIAN_POINT('Ctrl Pts',(-22.67406053567,1.76182076289525,12.));
#236486=CARTESIAN_POINT('Ctrl Pts',(-22.684345658525,1.76127038310614,12.));
#236487=CARTESIAN_POINT('Ctrl Pts',(-22.6948386219851,1.76067249704886,
12.));
#236488=CARTESIAN_POINT('Ctrl Pts',(-22.7055360375485,1.76002606202401,
12.));
#236489=CARTESIAN_POINT('Ctrl Pts',(-22.7164346186006,1.75933006905925,
12.));
#236490=CARTESIAN_POINT('Ctrl Pts',(-22.72753117773,1.75858354204633,12.));
#236491=CARTESIAN_POINT('Ctrl Pts',(-22.7388226235559,1.75778553673244,
12.));
#236492=CARTESIAN_POINT('Ctrl Pts',(-22.750305955645,1.75693513908907,12.));
#236493=CARTESIAN_POINT('Ctrl Pts',(-22.7619782595013,1.75603146371641,
12.));
#236494=CARTESIAN_POINT('Ctrl Pts',(-22.7738367016118,1.75507365227131,
12.));
#236495=CARTESIAN_POINT('Ctrl Pts',(-22.7858785242361,1.75406087182936,
12.));
#236496=CARTESIAN_POINT('Ctrl Pts',(-22.7981010424314,1.75299231391466,
12.));
#236497=CARTESIAN_POINT('Ctrl Pts',(-22.8105016414713,1.75186719365592,
12.));
#236498=CARTESIAN_POINT('Ctrl Pts',(-22.8230777741284,1.75068474890883,
12.));
#236499=CARTESIAN_POINT('Ctrl Pts',(-22.8358269579853,1.74944423940115,
12.));
#236500=CARTESIAN_POINT('Ctrl Pts',(-22.8487467728076,1.74814494588492,
12.));
#236501=CARTESIAN_POINT('Ctrl Pts',(-22.8618348580235,1.74678616930664,
12.));
#236502=CARTESIAN_POINT('Ctrl Pts',(-22.8750889101696,1.74536722998201,
12.));
#236503=CARTESIAN_POINT('Ctrl Pts',(-22.888506680335,1.74388746677702,12.));
#236504=CARTESIAN_POINT('Ctrl Pts',(-22.9020859716141,1.7423462363008,12.));
#236505=CARTESIAN_POINT('Ctrl Pts',(-22.9158246373363,1.74074291231058,
12.));
#236506=CARTESIAN_POINT('Ctrl Pts',(-22.9297205792586,1.73907688511666,
12.));
#236507=CARTESIAN_POINT('Ctrl Pts',(-22.9437717457826,1.73734756100039,
12.));
#236508=CARTESIAN_POINT('Ctrl Pts',(-22.9579761301063,1.73555436162769,
12.));
#236509=CARTESIAN_POINT('Ctrl Pts',(-22.9723317685688,1.73369672350814,
12.));
#236510=CARTESIAN_POINT('Ctrl Pts',(-22.9868367391978,1.7317740975019,12.));
#236511=CARTESIAN_POINT('Ctrl Pts',(-23.001489160189,1.72978594832136,12.));
#236512=CARTESIAN_POINT('Ctrl Pts',(-23.0162871884168,1.72773175404708,
12.));
#236513=CARTESIAN_POINT('Ctrl Pts',(-23.0312290178883,1.72561100564045,
12.));
#236514=CARTESIAN_POINT('Ctrl Pts',(-23.0463128785531,1.72342320653746,
12.));
#236515=CARTESIAN_POINT('Ctrl Pts',(-23.0615370351562,1.72116787225991,
12.));
#236516=CARTESIAN_POINT('Ctrl Pts',(-23.0768997860709,1.71884453003027,
12.));
#236517=CARTESIAN_POINT('Ctrl Pts',(-23.0923994621213,1.71645271839296,
12.));
#236518=CARTESIAN_POINT('Ctrl Pts',(-23.1080344254286,1.71399198684704,
12.));
#236519=CARTESIAN_POINT('Ctrl Pts',(-23.1238030684925,1.71146189552174,
12.));
#236520=CARTESIAN_POINT('Ctrl Pts',(-23.1397038132356,1.70886201485452,
12.));
#236521=CARTESIAN_POINT('Ctrl Pts',(-23.1557351100614,1.70619192527852,
12.));
#236522=CARTESIAN_POINT('Ctrl Pts',(-23.1718954368751,1.70345121691276,
12.));
#236523=CARTESIAN_POINT('Ctrl Pts',(-23.1881832981851,1.7006394892701,12.));
#236524=CARTESIAN_POINT('Ctrl Pts',(-23.2045972243767,1.69775635099443,
12.));
#236525=CARTESIAN_POINT('Ctrl Pts',(-23.2211357709374,1.69480141959953,
12.));
#236526=CARTESIAN_POINT('Ctrl Pts',(-23.2377975177013,1.69177432121711,
12.));
#236527=CARTESIAN_POINT('Ctrl Pts',(-23.2545810680537,1.68867469034896,
12.));
#236528=CARTESIAN_POINT('Ctrl Pts',(-23.2714850482246,1.68550216963258,
12.));
#236529=CARTESIAN_POINT('Ctrl Pts',(-23.2885081066951,1.68225640962168,
12.));
#236530=CARTESIAN_POINT('Ctrl Pts',(-23.3056489135611,1.67893706857117,
12.));
#236531=CARTESIAN_POINT('Ctrl Pts',(-23.3229061599145,1.67554381222994,
12.));
#236532=CARTESIAN_POINT('Ctrl Pts',(-23.3402785571865,1.67207631363921,
12.));
#236533=CARTESIAN_POINT('Ctrl Pts',(-23.3577648365744,1.66853425293995,
12.));
#236534=CARTESIAN_POINT('Ctrl Pts',(-23.3753637485545,1.66491731718876,
12.));
#236535=CARTESIAN_POINT('Ctrl Pts',(-23.3930740623619,1.66122520018011,
12.));
#236536=CARTESIAN_POINT('Ctrl Pts',(-23.4108945654805,1.65745760227505,
12.));
#236537=CARTESIAN_POINT('Ctrl Pts',(-23.4288240631043,1.65361423023728,
12.));
#236538=CARTESIAN_POINT('Ctrl Pts',(-23.4468613776574,1.6496947970734,12.));
#236539=CARTESIAN_POINT('Ctrl Pts',(-23.4650053483932,1.64569902187611,
12.));
#236540=CARTESIAN_POINT('Ctrl Pts',(-23.4832548309645,1.64162662967528,
12.));
#236541=CARTESIAN_POINT('Ctrl Pts',(-23.5016086970003,1.63747735129474,
12.));
#236542=CARTESIAN_POINT('Ctrl Pts',(-23.5200658336612,1.63325092321725,
12.));
#236543=CARTESIAN_POINT('Ctrl Pts',(-23.538625143226,1.62894708745223,12.));
#236544=CARTESIAN_POINT('Ctrl Pts',(-23.5572855427601,1.62456559140064,
12.));
#236545=CARTESIAN_POINT('Ctrl Pts',(-23.57604596376,1.62010618772866,12.));
#236546=CARTESIAN_POINT('Ctrl Pts',(-23.5949053517997,1.61556863424698,
12.));
#236547=CARTESIAN_POINT('Ctrl Pts',(-23.6138626661653,1.61095269379778,
12.));
#236548=CARTESIAN_POINT('Ctrl Pts',(-23.6329168794929,1.60625813414672,
12.));
#236549=CARTESIAN_POINT('Ctrl Pts',(-23.6520669774876,1.60148472786595,
12.));
#236550=CARTESIAN_POINT('Ctrl Pts',(-23.671311958631,1.59663225222463,12.));
#236551=CARTESIAN_POINT('Ctrl Pts',(-23.6906508338833,1.59170048908633,
12.));
#236552=CARTESIAN_POINT('Ctrl Pts',(-23.710082626383,1.58668922481221,12.));
#236553=CARTESIAN_POINT('Ctrl Pts',(-23.72960637113,1.58159825017358,12.));
#236554=CARTESIAN_POINT('Ctrl Pts',(-23.749221114736,1.57642736025246,12.));
#236555=CARTESIAN_POINT('Ctrl Pts',(-23.7689259151862,1.57117635434408,
12.));
#236556=CARTESIAN_POINT('Ctrl Pts',(-23.7887198415878,1.56584503586843,
12.));
#236557=CARTESIAN_POINT('Ctrl Pts',(-23.8086019739194,1.56043321228633,
12.));
#236558=CARTESIAN_POINT('Ctrl Pts',(-23.8285714027636,1.55494069502635,
12.));
#236559=CARTESIAN_POINT('Ctrl Pts',(-23.8486272290705,1.54936729940541,
12.));
#236560=CARTESIAN_POINT('Ctrl Pts',(-23.8687685639642,1.5437128445399,12.));
#236561=CARTESIAN_POINT('Ctrl Pts',(-23.8889945285318,1.53797715326758,
12.));
#236562=CARTESIAN_POINT('Ctrl Pts',(-23.9093042536119,1.53216005207463,
12.));
#236563=CARTESIAN_POINT('Ctrl Pts',(-23.9296968795757,1.52626137103032,
12.));
#236564=CARTESIAN_POINT('Ctrl Pts',(-23.9501715561033,1.52028094372792,
12.));
#236565=CARTESIAN_POINT('Ctrl Pts',(-23.970727442014,1.51421860720614,12.));
#236566=CARTESIAN_POINT('Ctrl Pts',(-23.9913637050927,1.50807420187694,
12.));
#236567=CARTESIAN_POINT('Ctrl Pts',(-24.0120795219086,1.50184757146098,
12.));
#236568=CARTESIAN_POINT('Ctrl Pts',(-24.0328740776331,1.49553856292801,
12.));
#236569=CARTESIAN_POINT('Ctrl Pts',(-24.0537465658429,1.48914702644887,
12.));
#236570=CARTESIAN_POINT('Ctrl Pts',(-24.0746961883528,1.48267281533683,
12.));
#236571=CARTESIAN_POINT('Ctrl Pts',(-24.0957221550778,1.47611578597742,
12.));
#236572=CARTESIAN_POINT('Ctrl Pts',(-24.1168236838824,1.46947579776991,
12.));
#236573=CARTESIAN_POINT('Ctrl Pts',(-24.1380000004272,1.46275271307397,
12.));
#236574=CARTESIAN_POINT('Ctrl Pts',(-24.1592503380107,1.45594639716317,
12.));
#236575=CARTESIAN_POINT('Ctrl Pts',(-24.1805739374038,1.44905671818727,
12.));
#236576=CARTESIAN_POINT('Ctrl Pts',(-24.201970046722,1.44208354711082,12.));
#236577=CARTESIAN_POINT('Ctrl Pts',(-24.2234379212984,1.43502675765508,
12.));
#236578=CARTESIAN_POINT('Ctrl Pts',(-24.2449768235488,1.42788622624854,
12.));
#236579=CARTESIAN_POINT('Ctrl Pts',(-24.2665860228356,1.42066183198252,
12.));
#236580=CARTESIAN_POINT('Ctrl Pts',(-24.288264795321,1.41335345657682,12.));
#236581=CARTESIAN_POINT('Ctrl Pts',(-24.3100124238311,1.40596098434337,
12.));
#236582=CARTESIAN_POINT('Ctrl Pts',(-24.3318281977643,1.39848430212807,
12.));
#236583=CARTESIAN_POINT('Ctrl Pts',(-24.3537114129875,1.39092329926388,
12.));
#236584=CARTESIAN_POINT('Ctrl Pts',(-24.3756613717299,1.38327786752998,
12.));
#236585=CARTESIAN_POINT('Ctrl Pts',(-24.3976773824732,1.37554790111609,
12.));
#236586=CARTESIAN_POINT('Ctrl Pts',(-24.4197587598337,1.36773329659956,
12.));
#236587=CARTESIAN_POINT('Ctrl Pts',(-24.4419048244523,1.35983395290627,
12.));
#236588=CARTESIAN_POINT('Ctrl Pts',(-24.4641149028892,1.35184977125648,
12.));
#236589=CARTESIAN_POINT('Ctrl Pts',(-24.4863883275134,1.34378065512337,
12.));
#236590=CARTESIAN_POINT('Ctrl Pts',(-24.5087244363856,1.33562651019686,
12.));
#236591=CARTESIAN_POINT('Ctrl Pts',(-24.5311225731435,1.32738724435326,
12.));
#236592=CARTESIAN_POINT('Ctrl Pts',(-24.5535820868674,1.31906276763668,
12.));
#236593=CARTESIAN_POINT('Ctrl Pts',(-24.5761023320183,1.31065299222021,
12.));
#236594=CARTESIAN_POINT('Ctrl Pts',(-24.5986826684027,1.30215783236362,
12.));
#236595=CARTESIAN_POINT('Ctrl Pts',(-24.6213224611229,1.29357720438107,
12.));
#236596=CARTESIAN_POINT('Ctrl Pts',(-24.6440210805278,1.28491102661514,
12.));
#236597=CARTESIAN_POINT('Ctrl Pts',(-24.666777902156,1.27615921941642,12.));
#236598=CARTESIAN_POINT('Ctrl Pts',(-24.6895923066836,1.267321705135,12.));
#236599=CARTESIAN_POINT('Ctrl Pts',(-24.7124636797894,1.25839840807418,
12.));
#236600=CARTESIAN_POINT('Ctrl Pts',(-24.7353914120011,1.24938925444325,
12.));
#236601=CARTESIAN_POINT('Ctrl Pts',(-24.7583748985438,1.24029417231989,
12.));
#236602=CARTESIAN_POINT('Ctrl Pts',(-24.7814135391799,1.23111309161843,
12.));
#236603=CARTESIAN_POINT('Ctrl Pts',(-24.8045067380536,1.22184594406528,
12.));
#236604=CARTESIAN_POINT('Ctrl Pts',(-24.8276539035092,1.21249266318208,
12.));
#236605=CARTESIAN_POINT('Ctrl Pts',(-24.8508544481974,1.2030531842602,12.));
#236606=CARTESIAN_POINT('Ctrl Pts',(-24.8741077892075,1.19352744434064,
12.));
#236607=CARTESIAN_POINT('Ctrl Pts',(-24.8974133481829,1.18391538220103,
12.));
#236608=CARTESIAN_POINT('Ctrl Pts',(-24.9207705514449,1.17421693835041,
12.));
#236609=CARTESIAN_POINT('Ctrl Pts',(-24.9441788300932,1.16443205502849,
12.));
#236610=CARTESIAN_POINT('Ctrl Pts',(-24.9676376201502,1.15456067621889,
12.));
#236611=CARTESIAN_POINT('Ctrl Pts',(-24.9911463621433,1.144602747582,12.));
#236612=CARTESIAN_POINT('Ctrl Pts',(-25.0147045006196,1.1345582163853,12.));
#236613=CARTESIAN_POINT('Ctrl Pts',(-25.0383114836899,1.12442703144451,
12.));
#236614=CARTESIAN_POINT('Ctrl Pts',(-25.0619667625336,1.11420914306889,
12.));
#236615=CARTESIAN_POINT('Ctrl Pts',(-25.0856697909679,1.10390450301745,
12.));
#236616=CARTESIAN_POINT('Ctrl Pts',(-25.1094200248446,1.09351306445308,
12.));
#236617=CARTESIAN_POINT('Ctrl Pts',(-25.1332169227413,1.08303478197187,
12.));
#236618=CARTESIAN_POINT('Ctrl Pts',(-25.157059946931,1.07246961165475,12.));
#236619=CARTESIAN_POINT('Ctrl Pts',(-25.1809485642192,1.06181751111768,
12.));
#236620=CARTESIAN_POINT('Ctrl Pts',(-25.2048822469028,1.05107843957931,
12.));
#236621=CARTESIAN_POINT('Ctrl Pts',(-25.2288604735086,1.04025235791507,
12.));
#236622=CARTESIAN_POINT('Ctrl Pts',(-25.2528827300422,1.02933922876806,
12.));
#236623=CARTESIAN_POINT('Ctrl Pts',(-25.276948508726,1.01833901642237,12.));
#236624=CARTESIAN_POINT('Ctrl Pts',(-25.3010573055547,1.00725168656896,
12.));
#236625=CARTESIAN_POINT('Ctrl Pts',(-25.3252086182968,0.996077206120624,
12.));
#236626=CARTESIAN_POINT('Ctrl Pts',(-25.3494019441441,0.984815543003973,
12.));
#236627=CARTESIAN_POINT('Ctrl Pts',(-25.3736367778845,0.973466666000163,
12.));
#236628=CARTESIAN_POINT('Ctrl Pts',(-25.3979126089163,0.962030544503142,
12.));
#236629=CARTESIAN_POINT('Ctrl Pts',(-25.4222289223167,0.950507148597468,
12.));
#236630=CARTESIAN_POINT('Ctrl Pts',(-25.4465852044849,0.938896449496192,
12.));
#236631=CARTESIAN_POINT('Ctrl Pts',(-25.4709809475009,0.927198419886094,
12.));
#236632=CARTESIAN_POINT('Ctrl Pts',(-25.4954156541795,0.915413034335613,
12.));
#236633=CARTESIAN_POINT('Ctrl Pts',(-25.5198888424194,0.903540269651106,
12.));
#236634=CARTESIAN_POINT('Ctrl Pts',(-25.5444000508211,0.89158010534904,
12.));
#236635=CARTESIAN_POINT('Ctrl Pts',(-25.5689488408156,0.879532523834294,
12.));
#236636=CARTESIAN_POINT('Ctrl Pts',(-25.5935347843585,0.867397509338431,
12.));
#236637=CARTESIAN_POINT('Ctrl Pts',(-25.6181574536049,0.855175047036549,
12.));
#236638=CARTESIAN_POINT('Ctrl Pts',(-25.6428164100055,0.842865122120758,
12.));
#236639=CARTESIAN_POINT('Ctrl Pts',(-25.6675111931952,0.830467718864205,
12.));
#236640=CARTESIAN_POINT('Ctrl Pts',(-25.6922413110194,0.817982819787464,
12.));
#236641=CARTESIAN_POINT('Ctrl Pts',(-25.7170062262525,0.805410404554352,
12.));
#236642=CARTESIAN_POINT('Ctrl Pts',(-25.7418053757746,0.792750451616127,
12.));
#236643=CARTESIAN_POINT('Ctrl Pts',(-25.7666381946955,0.780002940291965,
12.));
#236644=CARTESIAN_POINT('Ctrl Pts',(-25.7915041383376,0.767167852651168,
12.));
#236645=CARTESIAN_POINT('Ctrl Pts',(-25.8164027059984,0.754245175609524,
12.));
#236646=CARTESIAN_POINT('Ctrl Pts',(-25.8413334619055,0.741234902663807,
12.));
#236647=CARTESIAN_POINT('Ctrl Pts',(-25.8662960624185,0.728137036482335,
12.));
#236648=CARTESIAN_POINT('Ctrl Pts',(-25.891290261497,0.714951588527638,
12.));
#236649=CARTESIAN_POINT('Ctrl Pts',(-25.9163158909426,0.701678575228756,
12.));
#236650=CARTESIAN_POINT('Ctrl Pts',(-25.9413728471909,0.688318015057729,
12.));
#236651=CARTESIAN_POINT('Ctrl Pts',(-25.9614434297919,0.677559543209725,
12.));
#236652=CARTESIAN_POINT('Ctrl Pts',(-25.9765104298071,0.669451306780825,
12.));
#236653=CARTESIAN_POINT('Ctrl Pts',(-25.9865613464773,0.664028313187627,
12.));
#236654=CARTESIAN_POINT('Ctrl Pts',(-25.991588367311,0.661312440730901,
12.));
#236655=CARTESIAN_POINT('Ctrl Pts',(-22.1738711152697,4.11585220600461,
0.));
#236656=CARTESIAN_POINT('Ctrl Pts',(-22.1738711152697,4.11585220600461,
12.));
#236657=CARTESIAN_POINT('Ctrl Pts',(-22.173877682324,4.11585194677442,0.));
#236658=CARTESIAN_POINT('Ctrl Pts',(-22.173877682324,4.11585194677442,12.));
#236659=CARTESIAN_POINT('Ctrl Pts',(-22.1739341411687,4.11586035878287,
0.));
#236660=CARTESIAN_POINT('Ctrl Pts',(-22.1739341411687,4.11586035878287,
12.));
#236661=CARTESIAN_POINT('Ctrl Pts',(-22.1741488021234,4.11589976826166,
0.));
#236662=CARTESIAN_POINT('Ctrl Pts',(-22.1741488021234,4.11589976826166,
12.));
#236663=CARTESIAN_POINT('Ctrl Pts',(-22.1746949858775,4.11600589882845,
0.));
#236664=CARTESIAN_POINT('Ctrl Pts',(-22.1746949858775,4.11600589882845,
12.));
#236665=CARTESIAN_POINT('Ctrl Pts',(-22.1758088296598,4.11622797217068,
0.));
#236666=CARTESIAN_POINT('Ctrl Pts',(-22.1758088296598,4.11622797217068,
12.));
#236667=CARTESIAN_POINT('Ctrl Pts',(-22.177347426894,4.11653973150518,0.));
#236668=CARTESIAN_POINT('Ctrl Pts',(-22.177347426894,4.11653973150518,12.));
#236669=CARTESIAN_POINT('Ctrl Pts',(-22.179297473024,4.11694173195003,0.));
#236670=CARTESIAN_POINT('Ctrl Pts',(-22.179297473024,4.11694173195003,12.));
#236671=CARTESIAN_POINT('Ctrl Pts',(-22.1816414985788,4.11743469691756,
0.));
#236672=CARTESIAN_POINT('Ctrl Pts',(-22.1816414985788,4.11743469691756,
12.));
#236673=CARTESIAN_POINT('Ctrl Pts',(-22.1843613164855,4.11801938107479,
0.));
#236674=CARTESIAN_POINT('Ctrl Pts',(-22.1843613164855,4.11801938107479,
12.));
#236675=CARTESIAN_POINT('Ctrl Pts',(-22.1874419861496,4.11869641271773,
0.));
#236676=CARTESIAN_POINT('Ctrl Pts',(-22.1874419861496,4.11869641271773,
12.));
#236677=CARTESIAN_POINT('Ctrl Pts',(-22.1908725908525,4.11946626228636,
0.));
#236678=CARTESIAN_POINT('Ctrl Pts',(-22.1908725908525,4.11946626228636,
12.));
#236679=CARTESIAN_POINT('Ctrl Pts',(-22.1946440958098,4.12032932637736,
0.));
#236680=CARTESIAN_POINT('Ctrl Pts',(-22.1946440958098,4.12032932637736,
12.));
#236681=CARTESIAN_POINT('Ctrl Pts',(-22.1987479618246,4.12128598183522,
0.));
#236682=CARTESIAN_POINT('Ctrl Pts',(-22.1987479618246,4.12128598183522,
12.));
#236683=CARTESIAN_POINT('Ctrl Pts',(-22.2031746532106,4.12233664408227,
0.));
#236684=CARTESIAN_POINT('Ctrl Pts',(-22.2031746532106,4.12233664408227,
12.));
#236685=CARTESIAN_POINT('Ctrl Pts',(-22.2079143941719,4.12348173702023,
0.));
#236686=CARTESIAN_POINT('Ctrl Pts',(-22.2079143941719,4.12348173702023,
12.));
#236687=CARTESIAN_POINT('Ctrl Pts',(-22.2129576146671,4.12472167516607,
0.));
#236688=CARTESIAN_POINT('Ctrl Pts',(-22.2129576146671,4.12472167516607,
12.));
#236689=CARTESIAN_POINT('Ctrl Pts',(-22.2182956401341,4.12605683613307,
0.));
#236690=CARTESIAN_POINT('Ctrl Pts',(-22.2182956401341,4.12605683613307,
12.));
#236691=CARTESIAN_POINT('Ctrl Pts',(-22.2239207458781,4.12748755830104,
0.));
#236692=CARTESIAN_POINT('Ctrl Pts',(-22.2239207458781,4.12748755830104,
12.));
#236693=CARTESIAN_POINT('Ctrl Pts',(-22.2298258043947,4.12901415463379,
0.));
#236694=CARTESIAN_POINT('Ctrl Pts',(-22.2298258043947,4.12901415463379,
12.));
#236695=CARTESIAN_POINT('Ctrl Pts',(-22.2360040565533,4.13063692157498,
0.));
#236696=CARTESIAN_POINT('Ctrl Pts',(-22.2360040565533,4.13063692157498,
12.));
#236697=CARTESIAN_POINT('Ctrl Pts',(-22.2424488153523,4.1323561506016,0.));
#236698=CARTESIAN_POINT('Ctrl Pts',(-22.2424488153523,4.1323561506016,12.));
#236699=CARTESIAN_POINT('Ctrl Pts',(-22.249153531779,4.1341721255881,0.));
#236700=CARTESIAN_POINT('Ctrl Pts',(-22.249153531779,4.1341721255881,12.));
#236701=CARTESIAN_POINT('Ctrl Pts',(-22.2561118708421,4.13608511977225,
0.));
#236702=CARTESIAN_POINT('Ctrl Pts',(-22.2561118708421,4.13608511977225,
12.));
#236703=CARTESIAN_POINT('Ctrl Pts',(-22.2633177913972,4.13809539255421,
0.));
#236704=CARTESIAN_POINT('Ctrl Pts',(-22.2633177913972,4.13809539255421,
12.));
#236705=CARTESIAN_POINT('Ctrl Pts',(-22.2707656042457,4.14020318715991,
0.));
#236706=CARTESIAN_POINT('Ctrl Pts',(-22.2707656042457,4.14020318715991,
12.));
#236707=CARTESIAN_POINT('Ctrl Pts',(-22.2784499072027,4.14240873321984,
0.));
#236708=CARTESIAN_POINT('Ctrl Pts',(-22.2784499072027,4.14240873321984,
12.));
#236709=CARTESIAN_POINT('Ctrl Pts',(-22.2863655389166,4.14471224859295,
0.));
#236710=CARTESIAN_POINT('Ctrl Pts',(-22.2863655389166,4.14471224859295,
12.));
#236711=CARTESIAN_POINT('Ctrl Pts',(-22.2945075198467,4.14711394168556,
0.));
#236712=CARTESIAN_POINT('Ctrl Pts',(-22.2945075198467,4.14711394168556,
12.));
#236713=CARTESIAN_POINT('Ctrl Pts',(-22.3028710166933,4.14961401285522,
0.));
#236714=CARTESIAN_POINT('Ctrl Pts',(-22.3028710166933,4.14961401285522,
12.));
#236715=CARTESIAN_POINT('Ctrl Pts',(-22.3114513545185,4.1522126539699,0.));
#236716=CARTESIAN_POINT('Ctrl Pts',(-22.3114513545185,4.1522126539699,12.));
#236717=CARTESIAN_POINT('Ctrl Pts',(-22.3202440186979,4.15491004835281,
0.));
#236718=CARTESIAN_POINT('Ctrl Pts',(-22.3202440186979,4.15491004835281,
12.));
#236719=CARTESIAN_POINT('Ctrl Pts',(-22.3292446628959,4.15770637047889,
0.));
#236720=CARTESIAN_POINT('Ctrl Pts',(-22.3292446628959,4.15770637047889,
12.));
#236721=CARTESIAN_POINT('Ctrl Pts',(-22.3384491078602,4.16060178604164,
0.));
#236722=CARTESIAN_POINT('Ctrl Pts',(-22.3384491078602,4.16060178604164,
12.));
#236723=CARTESIAN_POINT('Ctrl Pts',(-22.3478533253889,4.16359645263187,
0.));
#236724=CARTESIAN_POINT('Ctrl Pts',(-22.3478533253889,4.16359645263187,
12.));
#236725=CARTESIAN_POINT('Ctrl Pts',(-22.3574534257396,4.166690520266,0.));
#236726=CARTESIAN_POINT('Ctrl Pts',(-22.3574534257396,4.166690520266,12.));
#236727=CARTESIAN_POINT('Ctrl Pts',(-22.36724564276,4.16988413199457,0.));
#236728=CARTESIAN_POINT('Ctrl Pts',(-22.36724564276,4.16988413199457,12.));
#236729=CARTESIAN_POINT('Ctrl Pts',(-22.3772263228617,4.17317742436145,
0.));
#236730=CARTESIAN_POINT('Ctrl Pts',(-22.3772263228617,4.17317742436145,
12.));
#236731=CARTESIAN_POINT('Ctrl Pts',(-22.3873919231334,4.17657052752825,
0.));
#236732=CARTESIAN_POINT('Ctrl Pts',(-22.3873919231334,4.17657052752825,
12.));
#236733=CARTESIAN_POINT('Ctrl Pts',(-22.3977390078075,4.18006356544882,
0.));
#236734=CARTESIAN_POINT('Ctrl Pts',(-22.3977390078075,4.18006356544882,
12.));
#236735=CARTESIAN_POINT('Ctrl Pts',(-22.4082642454453,4.1836566560085,0.));
#236736=CARTESIAN_POINT('Ctrl Pts',(-22.4082642454453,4.1836566560085,12.));
#236737=CARTESIAN_POINT('Ctrl Pts',(-22.4189644056115,4.1873499111772,0.));
#236738=CARTESIAN_POINT('Ctrl Pts',(-22.4189644056115,4.1873499111772,12.));
#236739=CARTESIAN_POINT('Ctrl Pts',(-22.4298363535421,4.19114343726941,
0.));
#236740=CARTESIAN_POINT('Ctrl Pts',(-22.4298363535421,4.19114343726941,
12.));
#236741=CARTESIAN_POINT('Ctrl Pts',(-22.4408770448917,4.1950373351886,0.));
#236742=CARTESIAN_POINT('Ctrl Pts',(-22.4408770448917,4.1950373351886,12.));
#236743=CARTESIAN_POINT('Ctrl Pts',(-22.4520835205419,4.19903170066354,
0.));
#236744=CARTESIAN_POINT('Ctrl Pts',(-22.4520835205419,4.19903170066354,
12.));
#236745=CARTESIAN_POINT('Ctrl Pts',(-22.4634529011433,4.2031266244817,0.));
#236746=CARTESIAN_POINT('Ctrl Pts',(-22.4634529011433,4.2031266244817,12.));
#236747=CARTESIAN_POINT('Ctrl Pts',(-22.4749823839915,4.20732219265648,
0.));
#236748=CARTESIAN_POINT('Ctrl Pts',(-22.4749823839915,4.20732219265648,
12.));
#236749=CARTESIAN_POINT('Ctrl Pts',(-22.4866692403147,4.21161848657428,
0.));
#236750=CARTESIAN_POINT('Ctrl Pts',(-22.4866692403147,4.21161848657428,
12.));
#236751=CARTESIAN_POINT('Ctrl Pts',(-22.4985108124229,4.21601558313908,
0.));
#236752=CARTESIAN_POINT('Ctrl Pts',(-22.4985108124229,4.21601558313908,
12.));
#236753=CARTESIAN_POINT('Ctrl Pts',(-22.5105045108882,4.22051355490196,
0.));
#236754=CARTESIAN_POINT('Ctrl Pts',(-22.5105045108882,4.22051355490196,
12.));
#236755=CARTESIAN_POINT('Ctrl Pts',(-22.5226478117885,4.2251124702004,0.));
#236756=CARTESIAN_POINT('Ctrl Pts',(-22.5226478117885,4.2251124702004,12.));
#236757=CARTESIAN_POINT('Ctrl Pts',(-22.5349382540587,4.22981239330731,
0.));
#236758=CARTESIAN_POINT('Ctrl Pts',(-22.5349382540587,4.22981239330731,
12.));
#236759=CARTESIAN_POINT('Ctrl Pts',(-22.5473734368086,4.23461338456713,
0.));
#236760=CARTESIAN_POINT('Ctrl Pts',(-22.5473734368086,4.23461338456713,
12.));
#236761=CARTESIAN_POINT('Ctrl Pts',(-22.559951016643,4.23951550052526,0.));
#236762=CARTESIAN_POINT('Ctrl Pts',(-22.559951016643,4.23951550052526,12.));
#236763=CARTESIAN_POINT('Ctrl Pts',(-22.5726687049922,4.24451879404858,
0.));
#236764=CARTESIAN_POINT('Ctrl Pts',(-22.5726687049922,4.24451879404858,
12.));
#236765=CARTESIAN_POINT('Ctrl Pts',(-22.5855242662479,4.24962331444184,
0.));
#236766=CARTESIAN_POINT('Ctrl Pts',(-22.5855242662479,4.24962331444184,
12.));
#236767=CARTESIAN_POINT('Ctrl Pts',(-22.5985155158637,4.25482910755485,
0.));
#236768=CARTESIAN_POINT('Ctrl Pts',(-22.5985155158637,4.25482910755485,
12.));
#236769=CARTESIAN_POINT('Ctrl Pts',(-22.611640318482,4.26013621588303,0.));
#236770=CARTESIAN_POINT('Ctrl Pts',(-22.611640318482,4.26013621588303,12.));
#236771=CARTESIAN_POINT('Ctrl Pts',(-22.6248965859975,4.26554467865571,
0.));
#236772=CARTESIAN_POINT('Ctrl Pts',(-22.6248965859975,4.26554467865571,
12.));
#236773=CARTESIAN_POINT('Ctrl Pts',(-22.6382822758171,4.27105453192999,
0.));
#236774=CARTESIAN_POINT('Ctrl Pts',(-22.6382822758171,4.27105453192999,
12.));
#236775=CARTESIAN_POINT('Ctrl Pts',(-22.6517953893303,4.27666580869117,
0.));
#236776=CARTESIAN_POINT('Ctrl Pts',(-22.6517953893303,4.27666580869117,
12.));
#236777=CARTESIAN_POINT('Ctrl Pts',(-22.665433970311,4.28237853894059,0.));
#236778=CARTESIAN_POINT('Ctrl Pts',(-22.665433970311,4.28237853894059,12.));
#236779=CARTESIAN_POINT('Ctrl Pts',(-22.6791961033537,4.28819274977766,
0.));
#236780=CARTESIAN_POINT('Ctrl Pts',(-22.6791961033537,4.28819274977766,
12.));
#236781=CARTESIAN_POINT('Ctrl Pts',(-22.6930799122545,4.29410846547061,
0.));
#236782=CARTESIAN_POINT('Ctrl Pts',(-22.6930799122545,4.29410846547061,
12.));
#236783=CARTESIAN_POINT('Ctrl Pts',(-22.707083558756,4.30012570754066,0.));
#236784=CARTESIAN_POINT('Ctrl Pts',(-22.707083558756,4.30012570754066,12.));
#236785=CARTESIAN_POINT('Ctrl Pts',(-22.7212052413384,4.30624449484074,
0.));
#236786=CARTESIAN_POINT('Ctrl Pts',(-22.7212052413384,4.30624449484074,
12.));
#236787=CARTESIAN_POINT('Ctrl Pts',(-22.7354431939927,4.3124648436255,0.));
#236788=CARTESIAN_POINT('Ctrl Pts',(-22.7354431939927,4.3124648436255,12.));
#236789=CARTESIAN_POINT('Ctrl Pts',(-22.7497956849852,4.3187867676123,0.));
#236790=CARTESIAN_POINT('Ctrl Pts',(-22.7497956849852,4.3187867676123,12.));
#236791=CARTESIAN_POINT('Ctrl Pts',(-22.764261015648,4.32521027803747,0.));
#236792=CARTESIAN_POINT('Ctrl Pts',(-22.764261015648,4.32521027803747,12.));
#236793=CARTESIAN_POINT('Ctrl Pts',(-22.7788375194081,4.33173538373182,
0.));
#236794=CARTESIAN_POINT('Ctrl Pts',(-22.7788375194081,4.33173538373182,
12.));
#236795=CARTESIAN_POINT('Ctrl Pts',(-22.7935235607807,4.33836209118442,
0.));
#236796=CARTESIAN_POINT('Ctrl Pts',(-22.7935235607807,4.33836209118442,
12.));
#236797=CARTESIAN_POINT('Ctrl Pts',(-22.808317534379,4.34509040460065,0.));
#236798=CARTESIAN_POINT('Ctrl Pts',(-22.808317534379,4.34509040460065,12.));
#236799=CARTESIAN_POINT('Ctrl Pts',(-22.8232178638873,4.35192032594801,
0.));
#236800=CARTESIAN_POINT('Ctrl Pts',(-22.8232178638873,4.35192032594801,
12.));
#236801=CARTESIAN_POINT('Ctrl Pts',(-22.838223001118,4.35885185500559,0.));
#236802=CARTESIAN_POINT('Ctrl Pts',(-22.838223001118,4.35885185500559,12.));
#236803=CARTESIAN_POINT('Ctrl Pts',(-22.8533314252419,4.36588498943009,
0.));
#236804=CARTESIAN_POINT('Ctrl Pts',(-22.8533314252419,4.36588498943009,
12.));
#236805=CARTESIAN_POINT('Ctrl Pts',(-22.8685416419725,4.37301972480752,
0.));
#236806=CARTESIAN_POINT('Ctrl Pts',(-22.8685416419725,4.37301972480752,
12.));
#236807=CARTESIAN_POINT('Ctrl Pts',(-22.8838521827702,4.38025605470089,
0.));
#236808=CARTESIAN_POINT('Ctrl Pts',(-22.8838521827702,4.38025605470089,
12.));
#236809=CARTESIAN_POINT('Ctrl Pts',(-22.8992616040108,4.38759397068391,
0.));
#236810=CARTESIAN_POINT('Ctrl Pts',(-22.8992616040108,4.38759397068391,
12.));
#236811=CARTESIAN_POINT('Ctrl Pts',(-22.9147684862425,4.39503346238454,
0.));
#236812=CARTESIAN_POINT('Ctrl Pts',(-22.9147684862425,4.39503346238454,
12.));
#236813=CARTESIAN_POINT('Ctrl Pts',(-22.9303714335549,4.40257451754307,
0.));
#236814=CARTESIAN_POINT('Ctrl Pts',(-22.9303714335549,4.40257451754307,
12.));
#236815=CARTESIAN_POINT('Ctrl Pts',(-22.9460690729093,4.41021712205547,
0.));
#236816=CARTESIAN_POINT('Ctrl Pts',(-22.9460690729093,4.41021712205547,
12.));
#236817=CARTESIAN_POINT('Ctrl Pts',(-22.9618600534866,4.41796126001309,
0.));
#236818=CARTESIAN_POINT('Ctrl Pts',(-22.9618600534866,4.41796126001309,
12.));
#236819=CARTESIAN_POINT('Ctrl Pts',(-22.9777430460021,4.42580691372771,
0.));
#236820=CARTESIAN_POINT('Ctrl Pts',(-22.9777430460021,4.42580691372771,
12.));
#236821=CARTESIAN_POINT('Ctrl Pts',(-22.9937167421009,4.43375406376904,
0.));
#236822=CARTESIAN_POINT('Ctrl Pts',(-22.9937167421009,4.43375406376904,
12.));
#236823=CARTESIAN_POINT('Ctrl Pts',(-23.0097798538399,4.44180268901666,
0.));
#236824=CARTESIAN_POINT('Ctrl Pts',(-23.0097798538399,4.44180268901666,
12.));
#236825=CARTESIAN_POINT('Ctrl Pts',(-23.0259311131395,4.44995276669698,
0.));
#236826=CARTESIAN_POINT('Ctrl Pts',(-23.0259311131395,4.44995276669698,
12.));
#236827=CARTESIAN_POINT('Ctrl Pts',(-23.0421692712466,4.45820427241676,
0.));
#236828=CARTESIAN_POINT('Ctrl Pts',(-23.0421692712466,4.45820427241676,
12.));
#236829=CARTESIAN_POINT('Ctrl Pts',(-23.0584930981723,4.46655718018205,
0.));
#236830=CARTESIAN_POINT('Ctrl Pts',(-23.0584930981723,4.46655718018205,
12.));
#236831=CARTESIAN_POINT('Ctrl Pts',(-23.0749013821868,4.47501146242821,
0.));
#236832=CARTESIAN_POINT('Ctrl Pts',(-23.0749013821868,4.47501146242821,
12.));
#236833=CARTESIAN_POINT('Ctrl Pts',(-23.0913929293909,4.48356709006756,
0.));
#236834=CARTESIAN_POINT('Ctrl Pts',(-23.0913929293909,4.48356709006756,
12.));
#236835=CARTESIAN_POINT('Ctrl Pts',(-23.1079665632629,4.49222403252201,
0.));
#236836=CARTESIAN_POINT('Ctrl Pts',(-23.1079665632629,4.49222403252201,
12.));
#236837=CARTESIAN_POINT('Ctrl Pts',(-23.1246211242117,4.50098225775178,
0.));
#236838=CARTESIAN_POINT('Ctrl Pts',(-23.1246211242117,4.50098225775178,
12.));
#236839=CARTESIAN_POINT('Ctrl Pts',(-23.1413554691136,4.50984173227087,
0.));
#236840=CARTESIAN_POINT('Ctrl Pts',(-23.1413554691136,4.50984173227087,
12.));
#236841=CARTESIAN_POINT('Ctrl Pts',(-23.1581684708778,4.51880242116785,
0.));
#236842=CARTESIAN_POINT('Ctrl Pts',(-23.1581684708778,4.51880242116785,
12.));
#236843=CARTESIAN_POINT('Ctrl Pts',(-23.1750590180923,4.52786428815047,
0.));
#236844=CARTESIAN_POINT('Ctrl Pts',(-23.1750590180923,4.52786428815047,
12.));
#236845=CARTESIAN_POINT('Ctrl Pts',(-23.1920260146474,4.53702729557585,
0.));
#236846=CARTESIAN_POINT('Ctrl Pts',(-23.1920260146474,4.53702729557585,
12.));
#236847=CARTESIAN_POINT('Ctrl Pts',(-23.2090683793627,4.54629140447542,
0.));
#236848=CARTESIAN_POINT('Ctrl Pts',(-23.2090683793627,4.54629140447542,
12.));
#236849=CARTESIAN_POINT('Ctrl Pts',(-23.2261850456055,4.55565657456956,
0.));
#236850=CARTESIAN_POINT('Ctrl Pts',(-23.2261850456055,4.55565657456956,
12.));
#236851=CARTESIAN_POINT('Ctrl Pts',(-23.2433749609117,4.5651227642781,0.));
#236852=CARTESIAN_POINT('Ctrl Pts',(-23.2433749609117,4.5651227642781,12.));
#236853=CARTESIAN_POINT('Ctrl Pts',(-23.2606370866853,4.5746899307607,0.));
#236854=CARTESIAN_POINT('Ctrl Pts',(-23.2606370866853,4.5746899307607,12.));
#236855=CARTESIAN_POINT('Ctrl Pts',(-23.2779703978868,4.58435802994674,
0.));
#236856=CARTESIAN_POINT('Ctrl Pts',(-23.2779703978868,4.58435802994674,
12.));
#236857=CARTESIAN_POINT('Ctrl Pts',(-23.295373882719,4.59412701655749,0.));
#236858=CARTESIAN_POINT('Ctrl Pts',(-23.295373882719,4.59412701655749,12.));
#236859=CARTESIAN_POINT('Ctrl Pts',(-23.3128465423119,4.60399684412174,
0.));
#236860=CARTESIAN_POINT('Ctrl Pts',(-23.3128465423119,4.60399684412174,
12.));
#236861=CARTESIAN_POINT('Ctrl Pts',(-23.3303873903947,4.61396746497848,
0.));
#236862=CARTESIAN_POINT('Ctrl Pts',(-23.3303873903947,4.61396746497848,
12.));
#236863=CARTESIAN_POINT('Ctrl Pts',(-23.3479954530281,4.62403883030823,
0.));
#236864=CARTESIAN_POINT('Ctrl Pts',(-23.3479954530281,4.62403883030823,
12.));
#236865=CARTESIAN_POINT('Ctrl Pts',(-23.3656697683496,4.63421089016554,
0.));
#236866=CARTESIAN_POINT('Ctrl Pts',(-23.3656697683496,4.63421089016554,
12.));
#236867=CARTESIAN_POINT('Ctrl Pts',(-23.383409386307,4.64448359349935,0.));
#236868=CARTESIAN_POINT('Ctrl Pts',(-23.383409386307,4.64448359349935,12.));
#236869=CARTESIAN_POINT('Ctrl Pts',(-23.4012133683957,4.65485688816921,
0.));
#236870=CARTESIAN_POINT('Ctrl Pts',(-23.4012133683957,4.65485688816921,
12.));
#236871=CARTESIAN_POINT('Ctrl Pts',(-23.4190807873798,4.66533072094663,
0.));
#236872=CARTESIAN_POINT('Ctrl Pts',(-23.4190807873798,4.66533072094663,
12.));
#236873=CARTESIAN_POINT('Ctrl Pts',(-23.4370107270444,4.6759050375305,0.));
#236874=CARTESIAN_POINT('Ctrl Pts',(-23.4370107270444,4.6759050375305,12.));
#236875=CARTESIAN_POINT('Ctrl Pts',(-23.4550022819853,4.68657978258297,
0.));
#236876=CARTESIAN_POINT('Ctrl Pts',(-23.4550022819853,4.68657978258297,
12.));
#236877=CARTESIAN_POINT('Ctrl Pts',(-23.4730545573849,4.69735489975023,
0.));
#236878=CARTESIAN_POINT('Ctrl Pts',(-23.4730545573849,4.69735489975023,
12.));
#236879=CARTESIAN_POINT('Ctrl Pts',(-23.491166668789,4.7082303316782,0.));
#236880=CARTESIAN_POINT('Ctrl Pts',(-23.491166668789,4.7082303316782,12.));
#236881=CARTESIAN_POINT('Ctrl Pts',(-23.5093377418784,4.71920602001904,
0.));
#236882=CARTESIAN_POINT('Ctrl Pts',(-23.5093377418784,4.71920602001904,
12.));
#236883=CARTESIAN_POINT('Ctrl Pts',(-23.5275669122378,4.73028190543031,
0.));
#236884=CARTESIAN_POINT('Ctrl Pts',(-23.5275669122378,4.73028190543031,
12.));
#236885=CARTESIAN_POINT('Ctrl Pts',(-23.5458533251715,4.74145792760698,
0.));
#236886=CARTESIAN_POINT('Ctrl Pts',(-23.5458533251715,4.74145792760698,
12.));
#236887=CARTESIAN_POINT('Ctrl Pts',(-23.564196135517,4.75273402530615,0.));
#236888=CARTESIAN_POINT('Ctrl Pts',(-23.564196135517,4.75273402530615,12.));
#236889=CARTESIAN_POINT('Ctrl Pts',(-23.5825945074535,4.7641101363625,0.));
#236890=CARTESIAN_POINT('Ctrl Pts',(-23.5825945074535,4.7641101363625,12.));
#236891=CARTESIAN_POINT('Ctrl Pts',(-23.6010476143099,4.77558619769875,
0.));
#236892=CARTESIAN_POINT('Ctrl Pts',(-23.6010476143099,4.77558619769875,
12.));
#236893=CARTESIAN_POINT('Ctrl Pts',(-23.6195546383625,4.78716214532104,
0.));
#236894=CARTESIAN_POINT('Ctrl Pts',(-23.6195546383625,4.78716214532104,
12.));
#236895=CARTESIAN_POINT('Ctrl Pts',(-23.6381147706581,4.79883791433229,
0.));
#236896=CARTESIAN_POINT('Ctrl Pts',(-23.6381147706581,4.79883791433229,
12.));
#236897=CARTESIAN_POINT('Ctrl Pts',(-23.6567272108631,4.81061343896442,
0.));
#236898=CARTESIAN_POINT('Ctrl Pts',(-23.6567272108631,4.81061343896442,
12.));
#236899=CARTESIAN_POINT('Ctrl Pts',(-23.6753911671023,4.82248865259569,
0.));
#236900=CARTESIAN_POINT('Ctrl Pts',(-23.6753911671023,4.82248865259569,
12.));
#236901=CARTESIAN_POINT('Ctrl Pts',(-23.6941058557971,4.83446348776267,
0.));
#236902=CARTESIAN_POINT('Ctrl Pts',(-23.6941058557971,4.83446348776267,
12.));
#236903=CARTESIAN_POINT('Ctrl Pts',(-23.7128705015014,4.84653787616422,
0.));
#236904=CARTESIAN_POINT('Ctrl Pts',(-23.7128705015014,4.84653787616422,
12.));
#236905=CARTESIAN_POINT('Ctrl Pts',(-23.7316843367308,4.85871174865491,
0.));
#236906=CARTESIAN_POINT('Ctrl Pts',(-23.7316843367308,4.85871174865491,
12.));
#236907=CARTESIAN_POINT('Ctrl Pts',(-23.7505466018239,4.87098503527142,
0.));
#236908=CARTESIAN_POINT('Ctrl Pts',(-23.7505466018239,4.87098503527142,
12.));
#236909=CARTESIAN_POINT('Ctrl Pts',(-23.7694565448044,4.88335766525565,
0.));
#236910=CARTESIAN_POINT('Ctrl Pts',(-23.7694565448044,4.88335766525565,
12.));
#236911=CARTESIAN_POINT('Ctrl Pts',(-23.7884134212381,4.89582956706771,
0.));
#236912=CARTESIAN_POINT('Ctrl Pts',(-23.7884134212381,4.89582956706771,
12.));
#236913=CARTESIAN_POINT('Ctrl Pts',(-23.8074164940897,4.90840066839346,
0.));
#236914=CARTESIAN_POINT('Ctrl Pts',(-23.8074164940897,4.90840066839346,
12.));
#236915=CARTESIAN_POINT('Ctrl Pts',(-23.8264650335721,4.92107089613976,
0.));
#236916=CARTESIAN_POINT('Ctrl Pts',(-23.8264650335721,4.92107089613976,
12.));
#236917=CARTESIAN_POINT('Ctrl Pts',(-23.8455583170062,4.93384017643441,
0.));
#236918=CARTESIAN_POINT('Ctrl Pts',(-23.8455583170062,4.93384017643441,
12.));
#236919=CARTESIAN_POINT('Ctrl Pts',(-23.8646956287172,4.94670843465868,
0.));
#236920=CARTESIAN_POINT('Ctrl Pts',(-23.8646956287172,4.94670843465868,
12.));
#236921=CARTESIAN_POINT('Ctrl Pts',(-23.883876259922,4.95967559546565,0.));
#236922=CARTESIAN_POINT('Ctrl Pts',(-23.883876259922,4.95967559546565,12.));
#236923=CARTESIAN_POINT('Ctrl Pts',(-23.9030995086164,4.97274158279228,
0.));
#236924=CARTESIAN_POINT('Ctrl Pts',(-23.9030995086164,4.97274158279228,
12.));
#236925=CARTESIAN_POINT('Ctrl Pts',(-23.9223646794591,4.98590631986532,
0.));
#236926=CARTESIAN_POINT('Ctrl Pts',(-23.9223646794591,4.98590631986532,
12.));
#236927=CARTESIAN_POINT('Ctrl Pts',(-23.9416710836529,4.99916972919309,
0.));
#236928=CARTESIAN_POINT('Ctrl Pts',(-23.9416710836529,4.99916972919309,
12.));
#236929=CARTESIAN_POINT('Ctrl Pts',(-23.9610180388271,5.01253173257458,
0.));
#236930=CARTESIAN_POINT('Ctrl Pts',(-23.9610180388271,5.01253173257458,
12.));
#236931=CARTESIAN_POINT('Ctrl Pts',(-23.9804048689228,5.02599225112461,
0.));
#236932=CARTESIAN_POINT('Ctrl Pts',(-23.9804048689228,5.02599225112461,
12.));
#236933=CARTESIAN_POINT('Ctrl Pts',(-23.9998309040747,5.03955120528527,
0.));
#236934=CARTESIAN_POINT('Ctrl Pts',(-23.9998309040747,5.03955120528527,
12.));
#236935=CARTESIAN_POINT('Ctrl Pts',(-24.0192954804896,5.05320851483068,
0.));
#236936=CARTESIAN_POINT('Ctrl Pts',(-24.0192954804896,5.05320851483068,
12.));
#236937=CARTESIAN_POINT('Ctrl Pts',(-24.0387979403268,5.06696409886639,
0.));
#236938=CARTESIAN_POINT('Ctrl Pts',(-24.0387979403268,5.06696409886639,
12.));
#236939=CARTESIAN_POINT('Ctrl Pts',(-24.0583376315636,5.0808178758127,0.));
#236940=CARTESIAN_POINT('Ctrl Pts',(-24.0583376315636,5.0808178758127,12.));
#236941=CARTESIAN_POINT('Ctrl Pts',(-24.0779139079264,5.09476976342616,
0.));
#236942=CARTESIAN_POINT('Ctrl Pts',(-24.0779139079264,5.09476976342616,
12.));
#236943=CARTESIAN_POINT('Ctrl Pts',(-24.0975261288444,5.10881967883124,
0.));
#236944=CARTESIAN_POINT('Ctrl Pts',(-24.0975261288444,5.10881967883124,
12.));
#236945=CARTESIAN_POINT('Ctrl Pts',(-24.117173659394,5.12296753853857,0.));
#236946=CARTESIAN_POINT('Ctrl Pts',(-24.117173659394,5.12296753853857,12.));
#236947=CARTESIAN_POINT('Ctrl Pts',(-24.1368558702443,5.13721325845745,
0.));
#236948=CARTESIAN_POINT('Ctrl Pts',(-24.1368558702443,5.13721325845745,
12.));
#236949=CARTESIAN_POINT('Ctrl Pts',(-24.1565721375971,5.15155675390079,
0.));
#236950=CARTESIAN_POINT('Ctrl Pts',(-24.1565721375971,5.15155675390079,
12.));
#236951=CARTESIAN_POINT('Ctrl Pts',(-24.1763218431344,5.16599793957985,
0.));
#236952=CARTESIAN_POINT('Ctrl Pts',(-24.1763218431344,5.16599793957985,
12.));
#236953=CARTESIAN_POINT('Ctrl Pts',(-24.1961043738756,5.18053672961398,
0.));
#236954=CARTESIAN_POINT('Ctrl Pts',(-24.1961043738756,5.18053672961398,
12.));
#236955=CARTESIAN_POINT('Ctrl Pts',(-24.2159191220171,5.19517303753647,
0.));
#236956=CARTESIAN_POINT('Ctrl Pts',(-24.2159191220171,5.19517303753647,
12.));
#236957=CARTESIAN_POINT('Ctrl Pts',(-24.2357654847766,5.20990677629176,
0.));
#236958=CARTESIAN_POINT('Ctrl Pts',(-24.2357654847766,5.20990677629176,
12.));
#236959=CARTESIAN_POINT('Ctrl Pts',(-24.2556428642294,5.22473785822442,
0.));
#236960=CARTESIAN_POINT('Ctrl Pts',(-24.2556428642294,5.22473785822442,
12.));
#236961=CARTESIAN_POINT('Ctrl Pts',(-24.2755506671525,5.23966619506289,
0.));
#236962=CARTESIAN_POINT('Ctrl Pts',(-24.2755506671525,5.23966619506289,
12.));
#236963=CARTESIAN_POINT('Ctrl Pts',(-24.2954883048447,5.25469169788856,
0.));
#236964=CARTESIAN_POINT('Ctrl Pts',(-24.2954883048447,5.25469169788856,
12.));
#236965=CARTESIAN_POINT('Ctrl Pts',(-24.3154551932221,5.26981427718798,
0.));
#236966=CARTESIAN_POINT('Ctrl Pts',(-24.3154551932221,5.26981427718798,
12.));
#236967=CARTESIAN_POINT('Ctrl Pts',(-24.3354507529414,5.28503384290648,
0.));
#236968=CARTESIAN_POINT('Ctrl Pts',(-24.3354507529414,5.28503384290648,
12.));
#236969=CARTESIAN_POINT('Ctrl Pts',(-24.3554744095075,5.30035030449063,
0.));
#236970=CARTESIAN_POINT('Ctrl Pts',(-24.3554744095075,5.30035030449063,
12.));
#236971=CARTESIAN_POINT('Ctrl Pts',(-24.3755255933917,5.31576357092526,
0.));
#236972=CARTESIAN_POINT('Ctrl Pts',(-24.3755255933917,5.31576357092526,
12.));
#236973=CARTESIAN_POINT('Ctrl Pts',(-24.3956037401293,5.33127355076033,
0.));
#236974=CARTESIAN_POINT('Ctrl Pts',(-24.3956037401293,5.33127355076033,
12.));
#236975=CARTESIAN_POINT('Ctrl Pts',(-24.4157082904614,5.34688015213537,
0.));
#236976=CARTESIAN_POINT('Ctrl Pts',(-24.4157082904614,5.34688015213537,
12.));
#236977=CARTESIAN_POINT('Ctrl Pts',(-24.435838689915,5.36258328273627,0.));
#236978=CARTESIAN_POINT('Ctrl Pts',(-24.435838689915,5.36258328273627,12.));
#236979=CARTESIAN_POINT('Ctrl Pts',(-24.4559943883157,5.37838284973695,
0.));
#236980=CARTESIAN_POINT('Ctrl Pts',(-24.4559943883157,5.37838284973695,
12.));
#236981=CARTESIAN_POINT('Ctrl Pts',(-24.4761748393321,5.39427875973824,
0.));
#236982=CARTESIAN_POINT('Ctrl Pts',(-24.4761748393321,5.39427875973824,
12.));
#236983=CARTESIAN_POINT('Ctrl Pts',(-24.4963794999831,5.41027091869241,
0.));
#236984=CARTESIAN_POINT('Ctrl Pts',(-24.4963794999831,5.41027091869241,
12.));
#236985=CARTESIAN_POINT('Ctrl Pts',(-24.5166078302108,5.42635923183419,
0.));
#236986=CARTESIAN_POINT('Ctrl Pts',(-24.5166078302108,5.42635923183419,
12.));
#236987=CARTESIAN_POINT('Ctrl Pts',(-24.5368592922863,5.4425436035688,0.));
#236988=CARTESIAN_POINT('Ctrl Pts',(-24.5368592922863,5.4425436035688,12.));
#236989=CARTESIAN_POINT('Ctrl Pts',(-24.5571333514842,5.45882393762261,
0.));
#236990=CARTESIAN_POINT('Ctrl Pts',(-24.5571333514842,5.45882393762261,
12.));
#236991=CARTESIAN_POINT('Ctrl Pts',(-24.5774294770329,5.47520013724419,
0.));
#236992=CARTESIAN_POINT('Ctrl Pts',(-24.5774294770329,5.47520013724419,
12.));
#236993=CARTESIAN_POINT('Ctrl Pts',(-24.5977471429364,5.49167210537246,
0.));
#236994=CARTESIAN_POINT('Ctrl Pts',(-24.5977471429364,5.49167210537246,
12.));
#236995=CARTESIAN_POINT('Ctrl Pts',(-24.6180858289179,5.50823974481962,
0.));
#236996=CARTESIAN_POINT('Ctrl Pts',(-24.6180858289179,5.50823974481962,
12.));
#236997=CARTESIAN_POINT('Ctrl Pts',(-24.6384450211467,5.52490295840991,
0.));
#236998=CARTESIAN_POINT('Ctrl Pts',(-24.6384450211467,5.52490295840991,
12.));
#236999=CARTESIAN_POINT('Ctrl Pts',(-24.6588242134738,5.54166164919583,
0.));
#237000=CARTESIAN_POINT('Ctrl Pts',(-24.6588242134738,5.54166164919583,
12.));
#237001=CARTESIAN_POINT('Ctrl Pts',(-24.6792229061794,5.55851572025376,
0.));
#237002=CARTESIAN_POINT('Ctrl Pts',(-24.6792229061794,5.55851572025376,
12.));
#237003=CARTESIAN_POINT('Ctrl Pts',(-24.6996406035517,5.57546507427754,
0.));
#237004=CARTESIAN_POINT('Ctrl Pts',(-24.6996406035517,5.57546507427754,
12.));
#237005=CARTESIAN_POINT('Ctrl Pts',(-24.7200768119088,5.59250961323987,
0.));
#237006=CARTESIAN_POINT('Ctrl Pts',(-24.7200768119088,5.59250961323987,
12.));
#237007=CARTESIAN_POINT('Ctrl Pts',(-24.7405310372739,5.60964923798491,
0.));
#237008=CARTESIAN_POINT('Ctrl Pts',(-24.7405310372739,5.60964923798491,
12.));
#237009=CARTESIAN_POINT('Ctrl Pts',(-24.7610027835697,5.62688384790923,
0.));
#237010=CARTESIAN_POINT('Ctrl Pts',(-24.7610027835697,5.62688384790923,
12.));
#237011=CARTESIAN_POINT('Ctrl Pts',(-24.781491549672,5.6442133404226,0.));
#237012=CARTESIAN_POINT('Ctrl Pts',(-24.781491549672,5.6442133404226,12.));
#237013=CARTESIAN_POINT('Ctrl Pts',(-24.8019968304605,5.66163761114921,
0.));
#237014=CARTESIAN_POINT('Ctrl Pts',(-24.8019968304605,5.66163761114921,
12.));
#237015=CARTESIAN_POINT('Ctrl Pts',(-24.8225181223845,5.67915655496542,
0.));
#237016=CARTESIAN_POINT('Ctrl Pts',(-24.8225181223845,5.67915655496542,
12.));
#237017=CARTESIAN_POINT('Ctrl Pts',(-24.8430549277621,5.69677006679444,
0.));
#237018=CARTESIAN_POINT('Ctrl Pts',(-24.8430549277621,5.69677006679444,
12.));
#237019=CARTESIAN_POINT('Ctrl Pts',(-24.8636067597669,5.71447804252027,
0.));
#237020=CARTESIAN_POINT('Ctrl Pts',(-24.8636067597669,5.71447804252027,
12.));
#237021=CARTESIAN_POINT('Ctrl Pts',(-24.884173146722,5.73228037976926,0.));
#237022=CARTESIAN_POINT('Ctrl Pts',(-24.884173146722,5.73228037976926,12.));
#237023=CARTESIAN_POINT('Ctrl Pts',(-24.904753637648,5.75017697890804,0.));
#237024=CARTESIAN_POINT('Ctrl Pts',(-24.904753637648,5.75017697890804,12.));
#237025=CARTESIAN_POINT('Ctrl Pts',(-24.9253478043656,5.76816774342219,
0.));
#237026=CARTESIAN_POINT('Ctrl Pts',(-24.9253478043656,5.76816774342219,
12.));
#237027=CARTESIAN_POINT('Ctrl Pts',(-24.945955229334,5.78625257775681,0.));
#237028=CARTESIAN_POINT('Ctrl Pts',(-24.945955229334,5.78625257775681,12.));
#237029=CARTESIAN_POINT('Ctrl Pts',(-24.9665754954496,5.80443138549726,
0.));
#237030=CARTESIAN_POINT('Ctrl Pts',(-24.9665754954496,5.80443138549726,
12.));
#237031=CARTESIAN_POINT('Ctrl Pts',(-24.9872081752734,5.82270406744198,
0.));
#237032=CARTESIAN_POINT('Ctrl Pts',(-24.9872081752734,5.82270406744198,
12.));
#237033=CARTESIAN_POINT('Ctrl Pts',(-25.0078528200564,5.84107051963071,
0.));
#237034=CARTESIAN_POINT('Ctrl Pts',(-25.0078528200564,5.84107051963071,
12.));
#237035=CARTESIAN_POINT('Ctrl Pts',(-25.0285089498899,5.85953063156826,
0.));
#237036=CARTESIAN_POINT('Ctrl Pts',(-25.0285089498899,5.85953063156826,
12.));
#237037=CARTESIAN_POINT('Ctrl Pts',(-25.0491760405911,5.87808428385365,
0.));
#237038=CARTESIAN_POINT('Ctrl Pts',(-25.0491760405911,5.87808428385365,
12.));
#237039=CARTESIAN_POINT('Ctrl Pts',(-25.0698535426514,5.89673135155514,
0.));
#237040=CARTESIAN_POINT('Ctrl Pts',(-25.0698535426514,5.89673135155514,
12.));
#237041=CARTESIAN_POINT('Ctrl Pts',(-25.0905409050773,5.91547170844447,
0.));
#237042=CARTESIAN_POINT('Ctrl Pts',(-25.0905409050773,5.91547170844447,
12.));
#237043=CARTESIAN_POINT('Ctrl Pts',(-25.1112375971106,5.93430523086834,
0.));
#237044=CARTESIAN_POINT('Ctrl Pts',(-25.1112375971106,5.93430523086834,
12.));
#237045=CARTESIAN_POINT('Ctrl Pts',(-25.1319431317237,5.95323180187378,
0.));
#237046=CARTESIAN_POINT('Ctrl Pts',(-25.1319431317237,5.95323180187378,
12.));
#237047=CARTESIAN_POINT('Ctrl Pts',(-25.1526570863092,5.97225131495616,
0.));
#237048=CARTESIAN_POINT('Ctrl Pts',(-25.1526570863092,5.97225131495616,
12.));
#237049=CARTESIAN_POINT('Ctrl Pts',(-25.1733791296259,5.99136367859754,
0.));
#237050=CARTESIAN_POINT('Ctrl Pts',(-25.1733791296259,5.99136367859754,
12.));
#237051=CARTESIAN_POINT('Ctrl Pts',(-25.1941090269819,6.01056881804612,
0.));
#237052=CARTESIAN_POINT('Ctrl Pts',(-25.1941090269819,6.01056881804612,
12.));
#237053=CARTESIAN_POINT('Ctrl Pts',(-25.21484662016,6.02986667389996,0.));
#237054=CARTESIAN_POINT('Ctrl Pts',(-25.21484662016,6.02986667389996,12.));
#237055=CARTESIAN_POINT('Ctrl Pts',(-25.2355918139032,6.04925720151218,
0.));
#237056=CARTESIAN_POINT('Ctrl Pts',(-25.2355918139032,6.04925720151218,
12.));
#237057=CARTESIAN_POINT('Ctrl Pts',(-25.2521940105705,6.06484373634546,
0.));
#237058=CARTESIAN_POINT('Ctrl Pts',(-25.2521940105705,6.06484373634546,
12.));
#237059=CARTESIAN_POINT('Ctrl Pts',(-25.2646490489923,6.0765753178749,0.));
#237060=CARTESIAN_POINT('Ctrl Pts',(-25.2646490489923,6.0765753178749,12.));
#237061=CARTESIAN_POINT('Ctrl Pts',(-25.2729539149517,6.08441489609793,
0.));
#237062=CARTESIAN_POINT('Ctrl Pts',(-25.2729539149517,6.08441489609793,
12.));
#237063=CARTESIAN_POINT('Ctrl Pts',(-25.2771067246846,6.08833931617699,
0.));
#237064=CARTESIAN_POINT('Ctrl Pts',(-25.2771067246846,6.08833931617699,
12.));
#237065=CARTESIAN_POINT('',(-25.2771067246846,6.08833931617699,0.));
#237066=CARTESIAN_POINT('Ctrl Pts',(-22.1738711152697,4.11585220600461,
0.));
#237067=CARTESIAN_POINT('Ctrl Pts',(-22.173877682324,4.11585194677442,0.));
#237068=CARTESIAN_POINT('Ctrl Pts',(-22.1739341411687,4.11586035878287,
0.));
#237069=CARTESIAN_POINT('Ctrl Pts',(-22.1741488021234,4.11589976826166,
0.));
#237070=CARTESIAN_POINT('Ctrl Pts',(-22.1746949858775,4.11600589882845,
0.));
#237071=CARTESIAN_POINT('Ctrl Pts',(-22.1758088296598,4.11622797217068,
0.));
#237072=CARTESIAN_POINT('Ctrl Pts',(-22.177347426894,4.11653973150518,0.));
#237073=CARTESIAN_POINT('Ctrl Pts',(-22.179297473024,4.11694173195003,0.));
#237074=CARTESIAN_POINT('Ctrl Pts',(-22.1816414985788,4.11743469691756,
0.));
#237075=CARTESIAN_POINT('Ctrl Pts',(-22.1843613164855,4.11801938107479,
0.));
#237076=CARTESIAN_POINT('Ctrl Pts',(-22.1874419861496,4.11869641271773,
0.));
#237077=CARTESIAN_POINT('Ctrl Pts',(-22.1908725908525,4.11946626228636,
0.));
#237078=CARTESIAN_POINT('Ctrl Pts',(-22.1946440958098,4.12032932637736,
0.));
#237079=CARTESIAN_POINT('Ctrl Pts',(-22.1987479618246,4.12128598183522,
0.));
#237080=CARTESIAN_POINT('Ctrl Pts',(-22.2031746532106,4.12233664408227,
0.));
#237081=CARTESIAN_POINT('Ctrl Pts',(-22.2079143941719,4.12348173702023,
0.));
#237082=CARTESIAN_POINT('Ctrl Pts',(-22.2129576146671,4.12472167516607,
0.));
#237083=CARTESIAN_POINT('Ctrl Pts',(-22.2182956401341,4.12605683613307,
0.));
#237084=CARTESIAN_POINT('Ctrl Pts',(-22.2239207458781,4.12748755830104,
0.));
#237085=CARTESIAN_POINT('Ctrl Pts',(-22.2298258043947,4.12901415463379,
0.));
#237086=CARTESIAN_POINT('Ctrl Pts',(-22.2360040565533,4.13063692157498,
0.));
#237087=CARTESIAN_POINT('Ctrl Pts',(-22.2424488153523,4.1323561506016,0.));
#237088=CARTESIAN_POINT('Ctrl Pts',(-22.249153531779,4.1341721255881,0.));
#237089=CARTESIAN_POINT('Ctrl Pts',(-22.2561118708421,4.13608511977225,
0.));
#237090=CARTESIAN_POINT('Ctrl Pts',(-22.2633177913972,4.13809539255421,
0.));
#237091=CARTESIAN_POINT('Ctrl Pts',(-22.2707656042457,4.14020318715991,
0.));
#237092=CARTESIAN_POINT('Ctrl Pts',(-22.2784499072027,4.14240873321984,
0.));
#237093=CARTESIAN_POINT('Ctrl Pts',(-22.2863655389166,4.14471224859295,
0.));
#237094=CARTESIAN_POINT('Ctrl Pts',(-22.2945075198467,4.14711394168556,
0.));
#237095=CARTESIAN_POINT('Ctrl Pts',(-22.3028710166933,4.14961401285522,
0.));
#237096=CARTESIAN_POINT('Ctrl Pts',(-22.3114513545185,4.1522126539699,0.));
#237097=CARTESIAN_POINT('Ctrl Pts',(-22.3202440186979,4.15491004835281,
0.));
#237098=CARTESIAN_POINT('Ctrl Pts',(-22.3292446628959,4.15770637047889,
0.));
#237099=CARTESIAN_POINT('Ctrl Pts',(-22.3384491078602,4.16060178604164,
0.));
#237100=CARTESIAN_POINT('Ctrl Pts',(-22.3478533253889,4.16359645263187,
0.));
#237101=CARTESIAN_POINT('Ctrl Pts',(-22.3574534257396,4.166690520266,0.));
#237102=CARTESIAN_POINT('Ctrl Pts',(-22.36724564276,4.16988413199457,0.));
#237103=CARTESIAN_POINT('Ctrl Pts',(-22.3772263228617,4.17317742436145,
0.));
#237104=CARTESIAN_POINT('Ctrl Pts',(-22.3873919231334,4.17657052752825,
0.));
#237105=CARTESIAN_POINT('Ctrl Pts',(-22.3977390078075,4.18006356544882,
0.));
#237106=CARTESIAN_POINT('Ctrl Pts',(-22.4082642454453,4.1836566560085,0.));
#237107=CARTESIAN_POINT('Ctrl Pts',(-22.4189644056115,4.1873499111772,0.));
#237108=CARTESIAN_POINT('Ctrl Pts',(-22.4298363535421,4.19114343726941,
0.));
#237109=CARTESIAN_POINT('Ctrl Pts',(-22.4408770448917,4.1950373351886,0.));
#237110=CARTESIAN_POINT('Ctrl Pts',(-22.4520835205419,4.19903170066354,
0.));
#237111=CARTESIAN_POINT('Ctrl Pts',(-22.4634529011433,4.2031266244817,0.));
#237112=CARTESIAN_POINT('Ctrl Pts',(-22.4749823839915,4.20732219265648,
0.));
#237113=CARTESIAN_POINT('Ctrl Pts',(-22.4866692403147,4.21161848657428,
0.));
#237114=CARTESIAN_POINT('Ctrl Pts',(-22.4985108124229,4.21601558313908,
0.));
#237115=CARTESIAN_POINT('Ctrl Pts',(-22.5105045108882,4.22051355490196,
0.));
#237116=CARTESIAN_POINT('Ctrl Pts',(-22.5226478117885,4.2251124702004,0.));
#237117=CARTESIAN_POINT('Ctrl Pts',(-22.5349382540587,4.22981239330731,
0.));
#237118=CARTESIAN_POINT('Ctrl Pts',(-22.5473734368086,4.23461338456713,
0.));
#237119=CARTESIAN_POINT('Ctrl Pts',(-22.559951016643,4.23951550052526,0.));
#237120=CARTESIAN_POINT('Ctrl Pts',(-22.5726687049922,4.24451879404858,
0.));
#237121=CARTESIAN_POINT('Ctrl Pts',(-22.5855242662479,4.24962331444184,
0.));
#237122=CARTESIAN_POINT('Ctrl Pts',(-22.5985155158637,4.25482910755485,
0.));
#237123=CARTESIAN_POINT('Ctrl Pts',(-22.611640318482,4.26013621588303,0.));
#237124=CARTESIAN_POINT('Ctrl Pts',(-22.6248965859975,4.26554467865571,
0.));
#237125=CARTESIAN_POINT('Ctrl Pts',(-22.6382822758171,4.27105453192999,
0.));
#237126=CARTESIAN_POINT('Ctrl Pts',(-22.6517953893303,4.27666580869117,
0.));
#237127=CARTESIAN_POINT('Ctrl Pts',(-22.665433970311,4.28237853894059,0.));
#237128=CARTESIAN_POINT('Ctrl Pts',(-22.6791961033537,4.28819274977766,
0.));
#237129=CARTESIAN_POINT('Ctrl Pts',(-22.6930799122545,4.29410846547061,
0.));
#237130=CARTESIAN_POINT('Ctrl Pts',(-22.707083558756,4.30012570754066,0.));
#237131=CARTESIAN_POINT('Ctrl Pts',(-22.7212052413384,4.30624449484074,
0.));
#237132=CARTESIAN_POINT('Ctrl Pts',(-22.7354431939927,4.3124648436255,0.));
#237133=CARTESIAN_POINT('Ctrl Pts',(-22.7497956849852,4.3187867676123,0.));
#237134=CARTESIAN_POINT('Ctrl Pts',(-22.764261015648,4.32521027803747,0.));
#237135=CARTESIAN_POINT('Ctrl Pts',(-22.7788375194081,4.33173538373182,
0.));
#237136=CARTESIAN_POINT('Ctrl Pts',(-22.7935235607807,4.33836209118442,
0.));
#237137=CARTESIAN_POINT('Ctrl Pts',(-22.808317534379,4.34509040460065,0.));
#237138=CARTESIAN_POINT('Ctrl Pts',(-22.8232178638873,4.35192032594801,
0.));
#237139=CARTESIAN_POINT('Ctrl Pts',(-22.838223001118,4.35885185500559,0.));
#237140=CARTESIAN_POINT('Ctrl Pts',(-22.8533314252419,4.36588498943009,
0.));
#237141=CARTESIAN_POINT('Ctrl Pts',(-22.8685416419725,4.37301972480752,
0.));
#237142=CARTESIAN_POINT('Ctrl Pts',(-22.8838521827702,4.38025605470089,
0.));
#237143=CARTESIAN_POINT('Ctrl Pts',(-22.8992616040108,4.38759397068391,
0.));
#237144=CARTESIAN_POINT('Ctrl Pts',(-22.9147684862425,4.39503346238454,
0.));
#237145=CARTESIAN_POINT('Ctrl Pts',(-22.9303714335549,4.40257451754307,
0.));
#237146=CARTESIAN_POINT('Ctrl Pts',(-22.9460690729093,4.41021712205547,
0.));
#237147=CARTESIAN_POINT('Ctrl Pts',(-22.9618600534866,4.41796126001309,
0.));
#237148=CARTESIAN_POINT('Ctrl Pts',(-22.9777430460021,4.42580691372771,
0.));
#237149=CARTESIAN_POINT('Ctrl Pts',(-22.9937167421009,4.43375406376904,
0.));
#237150=CARTESIAN_POINT('Ctrl Pts',(-23.0097798538399,4.44180268901666,
0.));
#237151=CARTESIAN_POINT('Ctrl Pts',(-23.0259311131395,4.44995276669698,
0.));
#237152=CARTESIAN_POINT('Ctrl Pts',(-23.0421692712466,4.45820427241676,
0.));
#237153=CARTESIAN_POINT('Ctrl Pts',(-23.0584930981723,4.46655718018205,
0.));
#237154=CARTESIAN_POINT('Ctrl Pts',(-23.0749013821868,4.47501146242821,
0.));
#237155=CARTESIAN_POINT('Ctrl Pts',(-23.0913929293909,4.48356709006756,
0.));
#237156=CARTESIAN_POINT('Ctrl Pts',(-23.1079665632629,4.49222403252201,
0.));
#237157=CARTESIAN_POINT('Ctrl Pts',(-23.1246211242117,4.50098225775178,
0.));
#237158=CARTESIAN_POINT('Ctrl Pts',(-23.1413554691136,4.50984173227087,
0.));
#237159=CARTESIAN_POINT('Ctrl Pts',(-23.1581684708778,4.51880242116785,
0.));
#237160=CARTESIAN_POINT('Ctrl Pts',(-23.1750590180923,4.52786428815047,
0.));
#237161=CARTESIAN_POINT('Ctrl Pts',(-23.1920260146474,4.53702729557585,
0.));
#237162=CARTESIAN_POINT('Ctrl Pts',(-23.2090683793627,4.54629140447542,
0.));
#237163=CARTESIAN_POINT('Ctrl Pts',(-23.2261850456055,4.55565657456956,
0.));
#237164=CARTESIAN_POINT('Ctrl Pts',(-23.2433749609117,4.5651227642781,0.));
#237165=CARTESIAN_POINT('Ctrl Pts',(-23.2606370866853,4.5746899307607,0.));
#237166=CARTESIAN_POINT('Ctrl Pts',(-23.2779703978868,4.58435802994674,
0.));
#237167=CARTESIAN_POINT('Ctrl Pts',(-23.295373882719,4.59412701655749,0.));
#237168=CARTESIAN_POINT('Ctrl Pts',(-23.3128465423119,4.60399684412174,
0.));
#237169=CARTESIAN_POINT('Ctrl Pts',(-23.3303873903947,4.61396746497848,
0.));
#237170=CARTESIAN_POINT('Ctrl Pts',(-23.3479954530281,4.62403883030823,
0.));
#237171=CARTESIAN_POINT('Ctrl Pts',(-23.3656697683496,4.63421089016554,
0.));
#237172=CARTESIAN_POINT('Ctrl Pts',(-23.383409386307,4.64448359349935,0.));
#237173=CARTESIAN_POINT('Ctrl Pts',(-23.4012133683957,4.65485688816921,
0.));
#237174=CARTESIAN_POINT('Ctrl Pts',(-23.4190807873798,4.66533072094663,
0.));
#237175=CARTESIAN_POINT('Ctrl Pts',(-23.4370107270444,4.6759050375305,0.));
#237176=CARTESIAN_POINT('Ctrl Pts',(-23.4550022819853,4.68657978258297,
0.));
#237177=CARTESIAN_POINT('Ctrl Pts',(-23.4730545573849,4.69735489975023,
0.));
#237178=CARTESIAN_POINT('Ctrl Pts',(-23.491166668789,4.7082303316782,0.));
#237179=CARTESIAN_POINT('Ctrl Pts',(-23.5093377418784,4.71920602001904,
0.));
#237180=CARTESIAN_POINT('Ctrl Pts',(-23.5275669122378,4.73028190543031,
0.));
#237181=CARTESIAN_POINT('Ctrl Pts',(-23.5458533251715,4.74145792760698,
0.));
#237182=CARTESIAN_POINT('Ctrl Pts',(-23.564196135517,4.75273402530615,0.));
#237183=CARTESIAN_POINT('Ctrl Pts',(-23.5825945074535,4.7641101363625,0.));
#237184=CARTESIAN_POINT('Ctrl Pts',(-23.6010476143099,4.77558619769875,
0.));
#237185=CARTESIAN_POINT('Ctrl Pts',(-23.6195546383625,4.78716214532104,
0.));
#237186=CARTESIAN_POINT('Ctrl Pts',(-23.6381147706581,4.79883791433229,
0.));
#237187=CARTESIAN_POINT('Ctrl Pts',(-23.6567272108631,4.81061343896442,
0.));
#237188=CARTESIAN_POINT('Ctrl Pts',(-23.6753911671023,4.82248865259569,
0.));
#237189=CARTESIAN_POINT('Ctrl Pts',(-23.6941058557971,4.83446348776267,
0.));
#237190=CARTESIAN_POINT('Ctrl Pts',(-23.7128705015014,4.84653787616422,
0.));
#237191=CARTESIAN_POINT('Ctrl Pts',(-23.7316843367308,4.85871174865491,
0.));
#237192=CARTESIAN_POINT('Ctrl Pts',(-23.7505466018239,4.87098503527142,
0.));
#237193=CARTESIAN_POINT('Ctrl Pts',(-23.7694565448044,4.88335766525565,
0.));
#237194=CARTESIAN_POINT('Ctrl Pts',(-23.7884134212381,4.89582956706771,
0.));
#237195=CARTESIAN_POINT('Ctrl Pts',(-23.8074164940897,4.90840066839346,
0.));
#237196=CARTESIAN_POINT('Ctrl Pts',(-23.8264650335721,4.92107089613976,
0.));
#237197=CARTESIAN_POINT('Ctrl Pts',(-23.8455583170062,4.93384017643441,
0.));
#237198=CARTESIAN_POINT('Ctrl Pts',(-23.8646956287172,4.94670843465868,
0.));
#237199=CARTESIAN_POINT('Ctrl Pts',(-23.883876259922,4.95967559546565,0.));
#237200=CARTESIAN_POINT('Ctrl Pts',(-23.9030995086164,4.97274158279228,
0.));
#237201=CARTESIAN_POINT('Ctrl Pts',(-23.9223646794591,4.98590631986532,
0.));
#237202=CARTESIAN_POINT('Ctrl Pts',(-23.9416710836529,4.99916972919309,
0.));
#237203=CARTESIAN_POINT('Ctrl Pts',(-23.9610180388271,5.01253173257458,
0.));
#237204=CARTESIAN_POINT('Ctrl Pts',(-23.9804048689228,5.02599225112461,
0.));
#237205=CARTESIAN_POINT('Ctrl Pts',(-23.9998309040747,5.03955120528527,
0.));
#237206=CARTESIAN_POINT('Ctrl Pts',(-24.0192954804896,5.05320851483068,
0.));
#237207=CARTESIAN_POINT('Ctrl Pts',(-24.0387979403268,5.06696409886639,
0.));
#237208=CARTESIAN_POINT('Ctrl Pts',(-24.0583376315636,5.0808178758127,0.));
#237209=CARTESIAN_POINT('Ctrl Pts',(-24.0779139079264,5.09476976342616,
0.));
#237210=CARTESIAN_POINT('Ctrl Pts',(-24.0975261288444,5.10881967883124,
0.));
#237211=CARTESIAN_POINT('Ctrl Pts',(-24.117173659394,5.12296753853857,0.));
#237212=CARTESIAN_POINT('Ctrl Pts',(-24.1368558702443,5.13721325845745,
0.));
#237213=CARTESIAN_POINT('Ctrl Pts',(-24.1565721375971,5.15155675390079,
0.));
#237214=CARTESIAN_POINT('Ctrl Pts',(-24.1763218431344,5.16599793957985,
0.));
#237215=CARTESIAN_POINT('Ctrl Pts',(-24.1961043738756,5.18053672961398,
0.));
#237216=CARTESIAN_POINT('Ctrl Pts',(-24.2159191220171,5.19517303753647,
0.));
#237217=CARTESIAN_POINT('Ctrl Pts',(-24.2357654847766,5.20990677629176,
0.));
#237218=CARTESIAN_POINT('Ctrl Pts',(-24.2556428642294,5.22473785822442,
0.));
#237219=CARTESIAN_POINT('Ctrl Pts',(-24.2755506671525,5.23966619506289,
0.));
#237220=CARTESIAN_POINT('Ctrl Pts',(-24.2954883048447,5.25469169788856,
0.));
#237221=CARTESIAN_POINT('Ctrl Pts',(-24.3154551932221,5.26981427718798,
0.));
#237222=CARTESIAN_POINT('Ctrl Pts',(-24.3354507529414,5.28503384290648,
0.));
#237223=CARTESIAN_POINT('Ctrl Pts',(-24.3554744095075,5.30035030449063,
0.));
#237224=CARTESIAN_POINT('Ctrl Pts',(-24.3755255933917,5.31576357092526,
0.));
#237225=CARTESIAN_POINT('Ctrl Pts',(-24.3956037401293,5.33127355076033,
0.));
#237226=CARTESIAN_POINT('Ctrl Pts',(-24.4157082904614,5.34688015213537,
0.));
#237227=CARTESIAN_POINT('Ctrl Pts',(-24.435838689915,5.36258328273627,0.));
#237228=CARTESIAN_POINT('Ctrl Pts',(-24.4559943883157,5.37838284973695,
0.));
#237229=CARTESIAN_POINT('Ctrl Pts',(-24.4761748393321,5.39427875973824,
0.));
#237230=CARTESIAN_POINT('Ctrl Pts',(-24.4963794999831,5.41027091869241,
0.));
#237231=CARTESIAN_POINT('Ctrl Pts',(-24.5166078302108,5.42635923183419,
0.));
#237232=CARTESIAN_POINT('Ctrl Pts',(-24.5368592922863,5.4425436035688,0.));
#237233=CARTESIAN_POINT('Ctrl Pts',(-24.5571333514842,5.45882393762261,
0.));
#237234=CARTESIAN_POINT('Ctrl Pts',(-24.5774294770329,5.47520013724419,
0.));
#237235=CARTESIAN_POINT('Ctrl Pts',(-24.5977471429364,5.49167210537246,
0.));
#237236=CARTESIAN_POINT('Ctrl Pts',(-24.6180858289179,5.50823974481962,
0.));
#237237=CARTESIAN_POINT('Ctrl Pts',(-24.6384450211467,5.52490295840991,
0.));
#237238=CARTESIAN_POINT('Ctrl Pts',(-24.6588242134738,5.54166164919583,
0.));
#237239=CARTESIAN_POINT('Ctrl Pts',(-24.6792229061794,5.55851572025376,
0.));
#237240=CARTESIAN_POINT('Ctrl Pts',(-24.6996406035517,5.57546507427754,
0.));
#237241=CARTESIAN_POINT('Ctrl Pts',(-24.7200768119088,5.59250961323987,
0.));
#237242=CARTESIAN_POINT('Ctrl Pts',(-24.7405310372739,5.60964923798491,
0.));
#237243=CARTESIAN_POINT('Ctrl Pts',(-24.7610027835697,5.62688384790923,
0.));
#237244=CARTESIAN_POINT('Ctrl Pts',(-24.781491549672,5.6442133404226,0.));
#237245=CARTESIAN_POINT('Ctrl Pts',(-24.8019968304605,5.66163761114921,
0.));
#237246=CARTESIAN_POINT('Ctrl Pts',(-24.8225181223845,5.67915655496542,
0.));
#237247=CARTESIAN_POINT('Ctrl Pts',(-24.8430549277621,5.69677006679444,
0.));
#237248=CARTESIAN_POINT('Ctrl Pts',(-24.8636067597669,5.71447804252027,
0.));
#237249=CARTESIAN_POINT('Ctrl Pts',(-24.884173146722,5.73228037976926,0.));
#237250=CARTESIAN_POINT('Ctrl Pts',(-24.904753637648,5.75017697890804,0.));
#237251=CARTESIAN_POINT('Ctrl Pts',(-24.9253478043656,5.76816774342219,
0.));
#237252=CARTESIAN_POINT('Ctrl Pts',(-24.945955229334,5.78625257775681,0.));
#237253=CARTESIAN_POINT('Ctrl Pts',(-24.9665754954496,5.80443138549726,
0.));
#237254=CARTESIAN_POINT('Ctrl Pts',(-24.9872081752734,5.82270406744198,
0.));
#237255=CARTESIAN_POINT('Ctrl Pts',(-25.0078528200564,5.84107051963071,
0.));
#237256=CARTESIAN_POINT('Ctrl Pts',(-25.0285089498899,5.85953063156826,
0.));
#237257=CARTESIAN_POINT('Ctrl Pts',(-25.0491760405911,5.87808428385365,
0.));
#237258=CARTESIAN_POINT('Ctrl Pts',(-25.0698535426514,5.89673135155514,
0.));
#237259=CARTESIAN_POINT('Ctrl Pts',(-25.0905409050773,5.91547170844447,
0.));
#237260=CARTESIAN_POINT('Ctrl Pts',(-25.1112375971106,5.93430523086834,
0.));
#237261=CARTESIAN_POINT('Ctrl Pts',(-25.1319431317237,5.95323180187378,
0.));
#237262=CARTESIAN_POINT('Ctrl Pts',(-25.1526570863092,5.97225131495616,
0.));
#237263=CARTESIAN_POINT('Ctrl Pts',(-25.1733791296259,5.99136367859754,
0.));
#237264=CARTESIAN_POINT('Ctrl Pts',(-25.1941090269819,6.01056881804612,
0.));
#237265=CARTESIAN_POINT('Ctrl Pts',(-25.21484662016,6.02986667389996,0.));
#237266=CARTESIAN_POINT('Ctrl Pts',(-25.2355918139032,6.04925720151218,
0.));
#237267=CARTESIAN_POINT('Ctrl Pts',(-25.2521940105705,6.06484373634546,
0.));
#237268=CARTESIAN_POINT('Ctrl Pts',(-25.2646490489923,6.0765753178749,0.));
#237269=CARTESIAN_POINT('Ctrl Pts',(-25.2729539149517,6.08441489609793,
0.));
#237270=CARTESIAN_POINT('Ctrl Pts',(-25.2771067246846,6.08833931617699,
0.));
#237271=CARTESIAN_POINT('',(-25.2771067246846,6.08833931617699,12.));
#237272=CARTESIAN_POINT('Ctrl Pts',(-25.2771067246846,6.08833931617699,
12.));
#237273=CARTESIAN_POINT('Ctrl Pts',(-25.2729539149517,6.08441489609793,
12.));
#237274=CARTESIAN_POINT('Ctrl Pts',(-25.2646490489923,6.0765753178749,12.));
#237275=CARTESIAN_POINT('Ctrl Pts',(-25.2521940105705,6.06484373634546,
12.));
#237276=CARTESIAN_POINT('Ctrl Pts',(-25.2355918139032,6.04925720151218,
12.));
#237277=CARTESIAN_POINT('Ctrl Pts',(-25.21484662016,6.02986667389996,12.));
#237278=CARTESIAN_POINT('Ctrl Pts',(-25.1941090269819,6.01056881804612,
12.));
#237279=CARTESIAN_POINT('Ctrl Pts',(-25.1733791296259,5.99136367859754,
12.));
#237280=CARTESIAN_POINT('Ctrl Pts',(-25.1526570863092,5.97225131495616,
12.));
#237281=CARTESIAN_POINT('Ctrl Pts',(-25.1319431317237,5.95323180187378,
12.));
#237282=CARTESIAN_POINT('Ctrl Pts',(-25.1112375971106,5.93430523086834,
12.));
#237283=CARTESIAN_POINT('Ctrl Pts',(-25.0905409050773,5.91547170844447,
12.));
#237284=CARTESIAN_POINT('Ctrl Pts',(-25.0698535426514,5.89673135155514,
12.));
#237285=CARTESIAN_POINT('Ctrl Pts',(-25.0491760405911,5.87808428385365,
12.));
#237286=CARTESIAN_POINT('Ctrl Pts',(-25.0285089498899,5.85953063156826,
12.));
#237287=CARTESIAN_POINT('Ctrl Pts',(-25.0078528200564,5.84107051963071,
12.));
#237288=CARTESIAN_POINT('Ctrl Pts',(-24.9872081752734,5.82270406744198,
12.));
#237289=CARTESIAN_POINT('Ctrl Pts',(-24.9665754954496,5.80443138549726,
12.));
#237290=CARTESIAN_POINT('Ctrl Pts',(-24.945955229334,5.78625257775681,12.));
#237291=CARTESIAN_POINT('Ctrl Pts',(-24.9253478043656,5.76816774342219,
12.));
#237292=CARTESIAN_POINT('Ctrl Pts',(-24.904753637648,5.75017697890804,12.));
#237293=CARTESIAN_POINT('Ctrl Pts',(-24.884173146722,5.73228037976926,12.));
#237294=CARTESIAN_POINT('Ctrl Pts',(-24.8636067597669,5.71447804252027,
12.));
#237295=CARTESIAN_POINT('Ctrl Pts',(-24.8430549277621,5.69677006679444,
12.));
#237296=CARTESIAN_POINT('Ctrl Pts',(-24.8225181223845,5.67915655496542,
12.));
#237297=CARTESIAN_POINT('Ctrl Pts',(-24.8019968304605,5.66163761114921,
12.));
#237298=CARTESIAN_POINT('Ctrl Pts',(-24.781491549672,5.6442133404226,12.));
#237299=CARTESIAN_POINT('Ctrl Pts',(-24.7610027835697,5.62688384790923,
12.));
#237300=CARTESIAN_POINT('Ctrl Pts',(-24.7405310372739,5.60964923798491,
12.));
#237301=CARTESIAN_POINT('Ctrl Pts',(-24.7200768119088,5.59250961323987,
12.));
#237302=CARTESIAN_POINT('Ctrl Pts',(-24.6996406035517,5.57546507427754,
12.));
#237303=CARTESIAN_POINT('Ctrl Pts',(-24.6792229061794,5.55851572025376,
12.));
#237304=CARTESIAN_POINT('Ctrl Pts',(-24.6588242134738,5.54166164919583,
12.));
#237305=CARTESIAN_POINT('Ctrl Pts',(-24.6384450211467,5.52490295840991,
12.));
#237306=CARTESIAN_POINT('Ctrl Pts',(-24.6180858289179,5.50823974481962,
12.));
#237307=CARTESIAN_POINT('Ctrl Pts',(-24.5977471429364,5.49167210537246,
12.));
#237308=CARTESIAN_POINT('Ctrl Pts',(-24.5774294770329,5.47520013724419,
12.));
#237309=CARTESIAN_POINT('Ctrl Pts',(-24.5571333514842,5.45882393762261,
12.));
#237310=CARTESIAN_POINT('Ctrl Pts',(-24.5368592922863,5.4425436035688,12.));
#237311=CARTESIAN_POINT('Ctrl Pts',(-24.5166078302108,5.42635923183419,
12.));
#237312=CARTESIAN_POINT('Ctrl Pts',(-24.4963794999831,5.41027091869241,
12.));
#237313=CARTESIAN_POINT('Ctrl Pts',(-24.4761748393321,5.39427875973824,
12.));
#237314=CARTESIAN_POINT('Ctrl Pts',(-24.4559943883157,5.37838284973695,
12.));
#237315=CARTESIAN_POINT('Ctrl Pts',(-24.435838689915,5.36258328273627,12.));
#237316=CARTESIAN_POINT('Ctrl Pts',(-24.4157082904614,5.34688015213537,
12.));
#237317=CARTESIAN_POINT('Ctrl Pts',(-24.3956037401293,5.33127355076033,
12.));
#237318=CARTESIAN_POINT('Ctrl Pts',(-24.3755255933917,5.31576357092526,
12.));
#237319=CARTESIAN_POINT('Ctrl Pts',(-24.3554744095075,5.30035030449063,
12.));
#237320=CARTESIAN_POINT('Ctrl Pts',(-24.3354507529414,5.28503384290648,
12.));
#237321=CARTESIAN_POINT('Ctrl Pts',(-24.3154551932221,5.26981427718798,
12.));
#237322=CARTESIAN_POINT('Ctrl Pts',(-24.2954883048447,5.25469169788856,
12.));
#237323=CARTESIAN_POINT('Ctrl Pts',(-24.2755506671525,5.23966619506289,
12.));
#237324=CARTESIAN_POINT('Ctrl Pts',(-24.2556428642294,5.22473785822442,
12.));
#237325=CARTESIAN_POINT('Ctrl Pts',(-24.2357654847766,5.20990677629176,
12.));
#237326=CARTESIAN_POINT('Ctrl Pts',(-24.2159191220171,5.19517303753647,
12.));
#237327=CARTESIAN_POINT('Ctrl Pts',(-24.1961043738756,5.18053672961398,
12.));
#237328=CARTESIAN_POINT('Ctrl Pts',(-24.1763218431344,5.16599793957985,
12.));
#237329=CARTESIAN_POINT('Ctrl Pts',(-24.1565721375971,5.15155675390079,
12.));
#237330=CARTESIAN_POINT('Ctrl Pts',(-24.1368558702443,5.13721325845745,
12.));
#237331=CARTESIAN_POINT('Ctrl Pts',(-24.117173659394,5.12296753853857,12.));
#237332=CARTESIAN_POINT('Ctrl Pts',(-24.0975261288444,5.10881967883124,
12.));
#237333=CARTESIAN_POINT('Ctrl Pts',(-24.0779139079264,5.09476976342616,
12.));
#237334=CARTESIAN_POINT('Ctrl Pts',(-24.0583376315636,5.0808178758127,12.));
#237335=CARTESIAN_POINT('Ctrl Pts',(-24.0387979403268,5.06696409886639,
12.));
#237336=CARTESIAN_POINT('Ctrl Pts',(-24.0192954804896,5.05320851483068,
12.));
#237337=CARTESIAN_POINT('Ctrl Pts',(-23.9998309040747,5.03955120528527,
12.));
#237338=CARTESIAN_POINT('Ctrl Pts',(-23.9804048689228,5.02599225112461,
12.));
#237339=CARTESIAN_POINT('Ctrl Pts',(-23.9610180388271,5.01253173257458,
12.));
#237340=CARTESIAN_POINT('Ctrl Pts',(-23.9416710836529,4.99916972919309,
12.));
#237341=CARTESIAN_POINT('Ctrl Pts',(-23.9223646794591,4.98590631986532,
12.));
#237342=CARTESIAN_POINT('Ctrl Pts',(-23.9030995086164,4.97274158279228,
12.));
#237343=CARTESIAN_POINT('Ctrl Pts',(-23.883876259922,4.95967559546565,12.));
#237344=CARTESIAN_POINT('Ctrl Pts',(-23.8646956287172,4.94670843465868,
12.));
#237345=CARTESIAN_POINT('Ctrl Pts',(-23.8455583170062,4.93384017643441,
12.));
#237346=CARTESIAN_POINT('Ctrl Pts',(-23.8264650335721,4.92107089613976,
12.));
#237347=CARTESIAN_POINT('Ctrl Pts',(-23.8074164940897,4.90840066839346,
12.));
#237348=CARTESIAN_POINT('Ctrl Pts',(-23.7884134212381,4.89582956706771,
12.));
#237349=CARTESIAN_POINT('Ctrl Pts',(-23.7694565448044,4.88335766525565,
12.));
#237350=CARTESIAN_POINT('Ctrl Pts',(-23.7505466018239,4.87098503527142,
12.));
#237351=CARTESIAN_POINT('Ctrl Pts',(-23.7316843367308,4.85871174865491,
12.));
#237352=CARTESIAN_POINT('Ctrl Pts',(-23.7128705015014,4.84653787616422,
12.));
#237353=CARTESIAN_POINT('Ctrl Pts',(-23.6941058557971,4.83446348776267,
12.));
#237354=CARTESIAN_POINT('Ctrl Pts',(-23.6753911671023,4.82248865259569,
12.));
#237355=CARTESIAN_POINT('Ctrl Pts',(-23.6567272108631,4.81061343896442,
12.));
#237356=CARTESIAN_POINT('Ctrl Pts',(-23.6381147706581,4.79883791433229,
12.));
#237357=CARTESIAN_POINT('Ctrl Pts',(-23.6195546383625,4.78716214532104,
12.));
#237358=CARTESIAN_POINT('Ctrl Pts',(-23.6010476143099,4.77558619769875,
12.));
#237359=CARTESIAN_POINT('Ctrl Pts',(-23.5825945074535,4.7641101363625,12.));
#237360=CARTESIAN_POINT('Ctrl Pts',(-23.564196135517,4.75273402530615,12.));
#237361=CARTESIAN_POINT('Ctrl Pts',(-23.5458533251715,4.74145792760698,
12.));
#237362=CARTESIAN_POINT('Ctrl Pts',(-23.5275669122378,4.73028190543031,
12.));
#237363=CARTESIAN_POINT('Ctrl Pts',(-23.5093377418784,4.71920602001904,
12.));
#237364=CARTESIAN_POINT('Ctrl Pts',(-23.491166668789,4.7082303316782,12.));
#237365=CARTESIAN_POINT('Ctrl Pts',(-23.4730545573849,4.69735489975023,
12.));
#237366=CARTESIAN_POINT('Ctrl Pts',(-23.4550022819853,4.68657978258297,
12.));
#237367=CARTESIAN_POINT('Ctrl Pts',(-23.4370107270444,4.6759050375305,12.));
#237368=CARTESIAN_POINT('Ctrl Pts',(-23.4190807873798,4.66533072094663,
12.));
#237369=CARTESIAN_POINT('Ctrl Pts',(-23.4012133683957,4.65485688816921,
12.));
#237370=CARTESIAN_POINT('Ctrl Pts',(-23.383409386307,4.64448359349935,12.));
#237371=CARTESIAN_POINT('Ctrl Pts',(-23.3656697683496,4.63421089016554,
12.));
#237372=CARTESIAN_POINT('Ctrl Pts',(-23.3479954530281,4.62403883030823,
12.));
#237373=CARTESIAN_POINT('Ctrl Pts',(-23.3303873903947,4.61396746497848,
12.));
#237374=CARTESIAN_POINT('Ctrl Pts',(-23.3128465423119,4.60399684412174,
12.));
#237375=CARTESIAN_POINT('Ctrl Pts',(-23.295373882719,4.59412701655749,12.));
#237376=CARTESIAN_POINT('Ctrl Pts',(-23.2779703978868,4.58435802994674,
12.));
#237377=CARTESIAN_POINT('Ctrl Pts',(-23.2606370866853,4.5746899307607,12.));
#237378=CARTESIAN_POINT('Ctrl Pts',(-23.2433749609117,4.5651227642781,12.));
#237379=CARTESIAN_POINT('Ctrl Pts',(-23.2261850456055,4.55565657456956,
12.));
#237380=CARTESIAN_POINT('Ctrl Pts',(-23.2090683793627,4.54629140447542,
12.));
#237381=CARTESIAN_POINT('Ctrl Pts',(-23.1920260146474,4.53702729557585,
12.));
#237382=CARTESIAN_POINT('Ctrl Pts',(-23.1750590180923,4.52786428815047,
12.));
#237383=CARTESIAN_POINT('Ctrl Pts',(-23.1581684708778,4.51880242116785,
12.));
#237384=CARTESIAN_POINT('Ctrl Pts',(-23.1413554691136,4.50984173227087,
12.));
#237385=CARTESIAN_POINT('Ctrl Pts',(-23.1246211242117,4.50098225775178,
12.));
#237386=CARTESIAN_POINT('Ctrl Pts',(-23.1079665632629,4.49222403252201,
12.));
#237387=CARTESIAN_POINT('Ctrl Pts',(-23.0913929293909,4.48356709006756,
12.));
#237388=CARTESIAN_POINT('Ctrl Pts',(-23.0749013821868,4.47501146242821,
12.));
#237389=CARTESIAN_POINT('Ctrl Pts',(-23.0584930981723,4.46655718018205,
12.));
#237390=CARTESIAN_POINT('Ctrl Pts',(-23.0421692712466,4.45820427241676,
12.));
#237391=CARTESIAN_POINT('Ctrl Pts',(-23.0259311131395,4.44995276669698,
12.));
#237392=CARTESIAN_POINT('Ctrl Pts',(-23.0097798538399,4.44180268901666,
12.));
#237393=CARTESIAN_POINT('Ctrl Pts',(-22.9937167421009,4.43375406376904,
12.));
#237394=CARTESIAN_POINT('Ctrl Pts',(-22.9777430460021,4.42580691372771,
12.));
#237395=CARTESIAN_POINT('Ctrl Pts',(-22.9618600534866,4.41796126001309,
12.));
#237396=CARTESIAN_POINT('Ctrl Pts',(-22.9460690729093,4.41021712205547,
12.));
#237397=CARTESIAN_POINT('Ctrl Pts',(-22.9303714335549,4.40257451754307,
12.));
#237398=CARTESIAN_POINT('Ctrl Pts',(-22.9147684862425,4.39503346238454,
12.));
#237399=CARTESIAN_POINT('Ctrl Pts',(-22.8992616040108,4.38759397068391,
12.));
#237400=CARTESIAN_POINT('Ctrl Pts',(-22.8838521827702,4.38025605470089,
12.));
#237401=CARTESIAN_POINT('Ctrl Pts',(-22.8685416419725,4.37301972480752,
12.));
#237402=CARTESIAN_POINT('Ctrl Pts',(-22.8533314252419,4.36588498943009,
12.));
#237403=CARTESIAN_POINT('Ctrl Pts',(-22.838223001118,4.35885185500559,12.));
#237404=CARTESIAN_POINT('Ctrl Pts',(-22.8232178638873,4.35192032594801,
12.));
#237405=CARTESIAN_POINT('Ctrl Pts',(-22.808317534379,4.34509040460065,12.));
#237406=CARTESIAN_POINT('Ctrl Pts',(-22.7935235607807,4.33836209118442,
12.));
#237407=CARTESIAN_POINT('Ctrl Pts',(-22.7788375194081,4.33173538373182,
12.));
#237408=CARTESIAN_POINT('Ctrl Pts',(-22.764261015648,4.32521027803747,12.));
#237409=CARTESIAN_POINT('Ctrl Pts',(-22.7497956849852,4.3187867676123,12.));
#237410=CARTESIAN_POINT('Ctrl Pts',(-22.7354431939927,4.3124648436255,12.));
#237411=CARTESIAN_POINT('Ctrl Pts',(-22.7212052413384,4.30624449484074,
12.));
#237412=CARTESIAN_POINT('Ctrl Pts',(-22.707083558756,4.30012570754066,12.));
#237413=CARTESIAN_POINT('Ctrl Pts',(-22.6930799122545,4.29410846547061,
12.));
#237414=CARTESIAN_POINT('Ctrl Pts',(-22.6791961033537,4.28819274977766,
12.));
#237415=CARTESIAN_POINT('Ctrl Pts',(-22.665433970311,4.28237853894059,12.));
#237416=CARTESIAN_POINT('Ctrl Pts',(-22.6517953893303,4.27666580869117,
12.));
#237417=CARTESIAN_POINT('Ctrl Pts',(-22.6382822758171,4.27105453192999,
12.));
#237418=CARTESIAN_POINT('Ctrl Pts',(-22.6248965859975,4.26554467865571,
12.));
#237419=CARTESIAN_POINT('Ctrl Pts',(-22.611640318482,4.26013621588303,12.));
#237420=CARTESIAN_POINT('Ctrl Pts',(-22.5985155158637,4.25482910755485,
12.));
#237421=CARTESIAN_POINT('Ctrl Pts',(-22.5855242662479,4.24962331444184,
12.));
#237422=CARTESIAN_POINT('Ctrl Pts',(-22.5726687049922,4.24451879404858,
12.));
#237423=CARTESIAN_POINT('Ctrl Pts',(-22.559951016643,4.23951550052526,12.));
#237424=CARTESIAN_POINT('Ctrl Pts',(-22.5473734368086,4.23461338456713,
12.));
#237425=CARTESIAN_POINT('Ctrl Pts',(-22.5349382540587,4.22981239330731,
12.));
#237426=CARTESIAN_POINT('Ctrl Pts',(-22.5226478117885,4.2251124702004,12.));
#237427=CARTESIAN_POINT('Ctrl Pts',(-22.5105045108882,4.22051355490196,
12.));
#237428=CARTESIAN_POINT('Ctrl Pts',(-22.4985108124229,4.21601558313908,
12.));
#237429=CARTESIAN_POINT('Ctrl Pts',(-22.4866692403147,4.21161848657428,
12.));
#237430=CARTESIAN_POINT('Ctrl Pts',(-22.4749823839915,4.20732219265648,
12.));
#237431=CARTESIAN_POINT('Ctrl Pts',(-22.4634529011433,4.2031266244817,12.));
#237432=CARTESIAN_POINT('Ctrl Pts',(-22.4520835205419,4.19903170066354,
12.));
#237433=CARTESIAN_POINT('Ctrl Pts',(-22.4408770448917,4.1950373351886,12.));
#237434=CARTESIAN_POINT('Ctrl Pts',(-22.4298363535421,4.19114343726941,
12.));
#237435=CARTESIAN_POINT('Ctrl Pts',(-22.4189644056115,4.1873499111772,12.));
#237436=CARTESIAN_POINT('Ctrl Pts',(-22.4082642454453,4.1836566560085,12.));
#237437=CARTESIAN_POINT('Ctrl Pts',(-22.3977390078075,4.18006356544882,
12.));
#237438=CARTESIAN_POINT('Ctrl Pts',(-22.3873919231334,4.17657052752825,
12.));
#237439=CARTESIAN_POINT('Ctrl Pts',(-22.3772263228617,4.17317742436145,
12.));
#237440=CARTESIAN_POINT('Ctrl Pts',(-22.36724564276,4.16988413199457,12.));
#237441=CARTESIAN_POINT('Ctrl Pts',(-22.3574534257396,4.166690520266,12.));
#237442=CARTESIAN_POINT('Ctrl Pts',(-22.3478533253889,4.16359645263187,
12.));
#237443=CARTESIAN_POINT('Ctrl Pts',(-22.3384491078602,4.16060178604164,
12.));
#237444=CARTESIAN_POINT('Ctrl Pts',(-22.3292446628959,4.15770637047889,
12.));
#237445=CARTESIAN_POINT('Ctrl Pts',(-22.3202440186979,4.15491004835281,
12.));
#237446=CARTESIAN_POINT('Ctrl Pts',(-22.3114513545185,4.1522126539699,12.));
#237447=CARTESIAN_POINT('Ctrl Pts',(-22.3028710166933,4.14961401285522,
12.));
#237448=CARTESIAN_POINT('Ctrl Pts',(-22.2945075198467,4.14711394168556,
12.));
#237449=CARTESIAN_POINT('Ctrl Pts',(-22.2863655389166,4.14471224859295,
12.));
#237450=CARTESIAN_POINT('Ctrl Pts',(-22.2784499072027,4.14240873321984,
12.));
#237451=CARTESIAN_POINT('Ctrl Pts',(-22.2707656042457,4.14020318715991,
12.));
#237452=CARTESIAN_POINT('Ctrl Pts',(-22.2633177913972,4.13809539255421,
12.));
#237453=CARTESIAN_POINT('Ctrl Pts',(-22.2561118708421,4.13608511977225,
12.));
#237454=CARTESIAN_POINT('Ctrl Pts',(-22.249153531779,4.1341721255881,12.));
#237455=CARTESIAN_POINT('Ctrl Pts',(-22.2424488153523,4.1323561506016,12.));
#237456=CARTESIAN_POINT('Ctrl Pts',(-22.2360040565533,4.13063692157498,
12.));
#237457=CARTESIAN_POINT('Ctrl Pts',(-22.2298258043947,4.12901415463379,
12.));
#237458=CARTESIAN_POINT('Ctrl Pts',(-22.2239207458781,4.12748755830104,
12.));
#237459=CARTESIAN_POINT('Ctrl Pts',(-22.2182956401341,4.12605683613307,
12.));
#237460=CARTESIAN_POINT('Ctrl Pts',(-22.2129576146671,4.12472167516607,
12.));
#237461=CARTESIAN_POINT('Ctrl Pts',(-22.2079143941719,4.12348173702023,
12.));
#237462=CARTESIAN_POINT('Ctrl Pts',(-22.2031746532106,4.12233664408227,
12.));
#237463=CARTESIAN_POINT('Ctrl Pts',(-22.1987479618246,4.12128598183522,
12.));
#237464=CARTESIAN_POINT('Ctrl Pts',(-22.1946440958098,4.12032932637736,
12.));
#237465=CARTESIAN_POINT('Ctrl Pts',(-22.1908725908525,4.11946626228636,
12.));
#237466=CARTESIAN_POINT('Ctrl Pts',(-22.1874419861496,4.11869641271773,
12.));
#237467=CARTESIAN_POINT('Ctrl Pts',(-22.1843613164855,4.11801938107479,
12.));
#237468=CARTESIAN_POINT('Ctrl Pts',(-22.1816414985788,4.11743469691756,
12.));
#237469=CARTESIAN_POINT('Ctrl Pts',(-22.179297473024,4.11694173195003,12.));
#237470=CARTESIAN_POINT('Ctrl Pts',(-22.177347426894,4.11653973150518,12.));
#237471=CARTESIAN_POINT('Ctrl Pts',(-22.1758088296598,4.11622797217068,
12.));
#237472=CARTESIAN_POINT('Ctrl Pts',(-22.1746949858775,4.11600589882845,
12.));
#237473=CARTESIAN_POINT('Ctrl Pts',(-22.1741488021234,4.11589976826166,
12.));
#237474=CARTESIAN_POINT('Ctrl Pts',(-22.1739341411687,4.11586035878287,
12.));
#237475=CARTESIAN_POINT('Ctrl Pts',(-22.173877682324,4.11585194677442,12.));
#237476=CARTESIAN_POINT('Ctrl Pts',(-22.1738711152697,4.11585220600461,
12.));
#237477=CARTESIAN_POINT('',(-25.2771067246846,6.08833931617699,0.));
#237478=CARTESIAN_POINT('Origin',(-19.4030938020118,9.26120677397565,0.));
#237479=CARTESIAN_POINT('',(-20.353053841303,9.71462809124917,12.));
#237480=CARTESIAN_POINT('',(-9.70154690100589,4.63060338698782,12.));
#237481=CARTESIAN_POINT('',(-20.353053841303,9.71462809124917,0.));
#237482=CARTESIAN_POINT('',(-20.353053841303,9.71462809124917,0.));
#237483=CARTESIAN_POINT('',(-9.70154690100589,4.63060338698782,0.));
#237484=CARTESIAN_POINT('Ctrl Pts',(-24.9347862158358,7.36589684767345,
0.));
#237485=CARTESIAN_POINT('Ctrl Pts',(-24.9347862158358,7.36589684767345,
12.));
#237486=CARTESIAN_POINT('Ctrl Pts',(-24.9292275670674,7.36721909028843,
0.));
#237487=CARTESIAN_POINT('Ctrl Pts',(-24.9292275670674,7.36721909028843,
12.));
#237488=CARTESIAN_POINT('Ctrl Pts',(-24.9181155530543,7.3698559312009,0.));
#237489=CARTESIAN_POINT('Ctrl Pts',(-24.9181155530543,7.3698559312009,12.));
#237490=CARTESIAN_POINT('Ctrl Pts',(-24.901463382605,7.37378825961676,0.));
#237491=CARTESIAN_POINT('Ctrl Pts',(-24.901463382605,7.37378825961676,12.));
#237492=CARTESIAN_POINT('Ctrl Pts',(-24.8792921911115,7.3789854964027,0.));
#237493=CARTESIAN_POINT('Ctrl Pts',(-24.8792921911115,7.3789854964027,12.));
#237494=CARTESIAN_POINT('Ctrl Pts',(-24.8516310625176,7.38540558903621,
0.));
#237495=CARTESIAN_POINT('Ctrl Pts',(-24.8516310625176,7.38540558903621,
12.));
#237496=CARTESIAN_POINT('Ctrl Pts',(-24.8240228520893,7.39174922585808,
0.));
#237497=CARTESIAN_POINT('Ctrl Pts',(-24.8240228520893,7.39174922585808,
12.));
#237498=CARTESIAN_POINT('Ctrl Pts',(-24.7964676646431,7.39801641583013,
0.));
#237499=CARTESIAN_POINT('Ctrl Pts',(-24.7964676646431,7.39801641583013,
12.));
#237500=CARTESIAN_POINT('Ctrl Pts',(-24.7689656668983,7.40420718661603,
0.));
#237501=CARTESIAN_POINT('Ctrl Pts',(-24.7689656668983,7.40420718661603,
12.));
#237502=CARTESIAN_POINT('Ctrl Pts',(-24.7415170994784,7.41032159082382,
0.));
#237503=CARTESIAN_POINT('Ctrl Pts',(-24.7415170994784,7.41032159082382,
12.));
#237504=CARTESIAN_POINT('Ctrl Pts',(-24.7141222950051,7.41635971481674,
0.));
#237505=CARTESIAN_POINT('Ctrl Pts',(-24.7141222950051,7.41635971481674,
12.));
#237506=CARTESIAN_POINT('Ctrl Pts',(-24.6867816727192,7.42232167766265,
0.));
#237507=CARTESIAN_POINT('Ctrl Pts',(-24.6867816727192,7.42232167766265,
12.));
#237508=CARTESIAN_POINT('Ctrl Pts',(-24.6594957128756,7.42820762159126,
0.));
#237509=CARTESIAN_POINT('Ctrl Pts',(-24.6594957128756,7.42820762159126,
12.));
#237510=CARTESIAN_POINT('Ctrl Pts',(-24.6322649369517,7.43401770489524,
0.));
#237511=CARTESIAN_POINT('Ctrl Pts',(-24.6322649369517,7.43401770489524,
12.));
#237512=CARTESIAN_POINT('Ctrl Pts',(-24.6050898852368,7.43975209375504,
0.));
#237513=CARTESIAN_POINT('Ctrl Pts',(-24.6050898852368,7.43975209375504,
12.));
#237514=CARTESIAN_POINT('Ctrl Pts',(-24.577971096086,7.44541095473134,0.));
#237515=CARTESIAN_POINT('Ctrl Pts',(-24.577971096086,7.44541095473134,12.));
#237516=CARTESIAN_POINT('Ctrl Pts',(-24.5509090831559,7.4509944465116,0.));
#237517=CARTESIAN_POINT('Ctrl Pts',(-24.5509090831559,7.4509944465116,12.));
#237518=CARTESIAN_POINT('Ctrl Pts',(-24.5239043173072,7.45650271335862,
0.));
#237519=CARTESIAN_POINT('Ctrl Pts',(-24.5239043173072,7.45650271335862,
12.));
#237520=CARTESIAN_POINT('Ctrl Pts',(-24.4969572391483,7.46193588961463,
0.));
#237521=CARTESIAN_POINT('Ctrl Pts',(-24.4969572391483,7.46193588961463,
12.));
#237522=CARTESIAN_POINT('Ctrl Pts',(-24.4700682684524,7.46729410308786,
0.));
#237523=CARTESIAN_POINT('Ctrl Pts',(-24.4700682684524,7.46729410308786,
12.));
#237524=CARTESIAN_POINT('Ctrl Pts',(-24.443237814649,7.47257747883246,0.));
#237525=CARTESIAN_POINT('Ctrl Pts',(-24.443237814649,7.47257747883246,12.));
#237526=CARTESIAN_POINT('Ctrl Pts',(-24.4164662871163,7.47778614286565,
0.));
#237527=CARTESIAN_POINT('Ctrl Pts',(-24.4164662871163,7.47778614286565,
12.));
#237528=CARTESIAN_POINT('Ctrl Pts',(-24.3897541049254,7.48292022569301,
0.));
#237529=CARTESIAN_POINT('Ctrl Pts',(-24.3897541049254,7.48292022569301,
12.));
#237530=CARTESIAN_POINT('Ctrl Pts',(-24.3631017084524,7.48797986651908,
0.));
#237531=CARTESIAN_POINT('Ctrl Pts',(-24.3631017084524,7.48797986651908,
12.));
#237532=CARTESIAN_POINT('Ctrl Pts',(-24.3365095573685,7.4929652125242,0.));
#237533=CARTESIAN_POINT('Ctrl Pts',(-24.3365095573685,7.4929652125242,12.));
#237534=CARTESIAN_POINT('Ctrl Pts',(-24.3099781253355,7.49787641695439,
0.));
#237535=CARTESIAN_POINT('Ctrl Pts',(-24.3099781253355,7.49787641695439,
12.));
#237536=CARTESIAN_POINT('Ctrl Pts',(-24.2835078958973,7.50271363765152,
0.));
#237537=CARTESIAN_POINT('Ctrl Pts',(-24.2835078958973,7.50271363765152,
12.));
#237538=CARTESIAN_POINT('Ctrl Pts',(-24.2570993577034,7.50747703535133,
0.));
#237539=CARTESIAN_POINT('Ctrl Pts',(-24.2570993577034,7.50747703535133,
12.));
#237540=CARTESIAN_POINT('Ctrl Pts',(-24.2307530003887,7.51216677222181,
0.));
#237541=CARTESIAN_POINT('Ctrl Pts',(-24.2307530003887,7.51216677222181,
12.));
#237542=CARTESIAN_POINT('Ctrl Pts',(-24.2044693092349,7.51678300997949,
0.));
#237543=CARTESIAN_POINT('Ctrl Pts',(-24.2044693092349,7.51678300997949,
12.));
#237544=CARTESIAN_POINT('Ctrl Pts',(-24.1782487641594,7.52132590953802,
0.));
#237545=CARTESIAN_POINT('Ctrl Pts',(-24.1782487641594,7.52132590953802,
12.));
#237546=CARTESIAN_POINT('Ctrl Pts',(-24.1520918425364,7.52579563201424,
0.));
#237547=CARTESIAN_POINT('Ctrl Pts',(-24.1520918425364,7.52579563201424,
12.));
#237548=CARTESIAN_POINT('Ctrl Pts',(-24.1259990209207,7.53019233935501,
0.));
#237549=CARTESIAN_POINT('Ctrl Pts',(-24.1259990209207,7.53019233935501,
12.));
#237550=CARTESIAN_POINT('Ctrl Pts',(-24.0999707772642,7.53451619514649,
0.));
#237551=CARTESIAN_POINT('Ctrl Pts',(-24.0999707772642,7.53451619514649,
12.));
#237552=CARTESIAN_POINT('Ctrl Pts',(-24.0740075927985,7.53876736531014,
0.));
#237553=CARTESIAN_POINT('Ctrl Pts',(-24.0740075927985,7.53876736531014,
12.));
#237554=CARTESIAN_POINT('Ctrl Pts',(-24.0481099543353,7.54294601896144,
0.));
#237555=CARTESIAN_POINT('Ctrl Pts',(-24.0481099543353,7.54294601896144,
12.));
#237556=CARTESIAN_POINT('Ctrl Pts',(-24.022278355453,7.5470523288591,0.));
#237557=CARTESIAN_POINT('Ctrl Pts',(-24.022278355453,7.5470523288591,12.));
#237558=CARTESIAN_POINT('Ctrl Pts',(-23.9965132953185,7.55108647097441,
0.));
#237559=CARTESIAN_POINT('Ctrl Pts',(-23.9965132953185,7.55108647097441,
12.));
#237560=CARTESIAN_POINT('Ctrl Pts',(-23.9708152779884,7.55504862424812,
0.));
#237561=CARTESIAN_POINT('Ctrl Pts',(-23.9708152779884,7.55504862424812,
12.));
#237562=CARTESIAN_POINT('Ctrl Pts',(-23.9451848115,7.55893897027682,0.));
#237563=CARTESIAN_POINT('Ctrl Pts',(-23.9451848115,7.55893897027682,12.));
#237564=CARTESIAN_POINT('Ctrl Pts',(-23.9196224070759,7.56275769304773,
0.));
#237565=CARTESIAN_POINT('Ctrl Pts',(-23.9196224070759,7.56275769304773,
12.));
#237566=CARTESIAN_POINT('Ctrl Pts',(-23.8941285782003,7.56650497863792,
0.));
#237567=CARTESIAN_POINT('Ctrl Pts',(-23.8941285782003,7.56650497863792,
12.));
#237568=CARTESIAN_POINT('Ctrl Pts',(-23.8687038399598,7.57018101500711,
0.));
#237569=CARTESIAN_POINT('Ctrl Pts',(-23.8687038399598,7.57018101500711,
12.));
#237570=CARTESIAN_POINT('Ctrl Pts',(-23.8433487096134,7.57378599219816,
0.));
#237571=CARTESIAN_POINT('Ctrl Pts',(-23.8433487096134,7.57378599219816,
12.));
#237572=CARTESIAN_POINT('Ctrl Pts',(-23.8180637069977,7.57732010249066,
0.));
#237573=CARTESIAN_POINT('Ctrl Pts',(-23.8180637069977,7.57732010249066,
12.));
#237574=CARTESIAN_POINT('Ctrl Pts',(-23.7928493549908,7.58078354058212,
0.));
#237575=CARTESIAN_POINT('Ctrl Pts',(-23.7928493549908,7.58078354058212,
12.));
#237576=CARTESIAN_POINT('Ctrl Pts',(-23.7677061799376,7.58417650376272,
0.));
#237577=CARTESIAN_POINT('Ctrl Pts',(-23.7677061799376,7.58417650376272,
12.));
#237578=CARTESIAN_POINT('Ctrl Pts',(-23.7426347121006,7.58749919210832,
0.));
#237579=CARTESIAN_POINT('Ctrl Pts',(-23.7426347121006,7.58749919210832,
12.));
#237580=CARTESIAN_POINT('Ctrl Pts',(-23.7176354860457,7.59075180865327,
0.));
#237581=CARTESIAN_POINT('Ctrl Pts',(-23.7176354860457,7.59075180865327,
12.));
#237582=CARTESIAN_POINT('Ctrl Pts',(-23.6927090405067,7.59393455934042,
0.));
#237583=CARTESIAN_POINT('Ctrl Pts',(-23.6927090405067,7.59393455934042,
12.));
#237584=CARTESIAN_POINT('Ctrl Pts',(-23.6678559182876,7.59704765299572,
0.));
#237585=CARTESIAN_POINT('Ctrl Pts',(-23.6678559182876,7.59704765299572,
12.));
#237586=CARTESIAN_POINT('Ctrl Pts',(-23.6430766661419,7.60009130130129,
0.));
#237587=CARTESIAN_POINT('Ctrl Pts',(-23.6430766661419,7.60009130130129,
12.));
#237588=CARTESIAN_POINT('Ctrl Pts',(-23.6183718346576,7.60306571877806,
0.));
#237589=CARTESIAN_POINT('Ctrl Pts',(-23.6183718346576,7.60306571877806,
12.));
#237590=CARTESIAN_POINT('Ctrl Pts',(-23.5937419781244,7.60597112277094,
0.));
#237591=CARTESIAN_POINT('Ctrl Pts',(-23.5937419781244,7.60597112277094,
12.));
#237592=CARTESIAN_POINT('Ctrl Pts',(-23.5691876544243,7.60880773344599,
0.));
#237593=CARTESIAN_POINT('Ctrl Pts',(-23.5691876544243,7.60880773344599,
12.));
#237594=CARTESIAN_POINT('Ctrl Pts',(-23.5447094252029,7.61157577385372,
0.));
#237595=CARTESIAN_POINT('Ctrl Pts',(-23.5447094252029,7.61157577385372,
12.));
#237596=CARTESIAN_POINT('Ctrl Pts',(-23.5203078560128,7.61427546999299,
0.));
#237597=CARTESIAN_POINT('Ctrl Pts',(-23.5203078560128,7.61427546999299,
12.));
#237598=CARTESIAN_POINT('Ctrl Pts',(-23.4959835164608,7.61690705088319,
0.));
#237599=CARTESIAN_POINT('Ctrl Pts',(-23.4959835164608,7.61690705088319,
12.));
#237600=CARTESIAN_POINT('Ctrl Pts',(-23.4717369803438,7.61947074863977,
0.));
#237601=CARTESIAN_POINT('Ctrl Pts',(-23.4717369803438,7.61947074863977,
12.));
#237602=CARTESIAN_POINT('Ctrl Pts',(-23.4475688257854,7.62196679855957,
0.));
#237603=CARTESIAN_POINT('Ctrl Pts',(-23.4475688257854,7.62196679855957,
12.));
#237604=CARTESIAN_POINT('Ctrl Pts',(-23.4234796353544,7.62439543920054,
0.));
#237605=CARTESIAN_POINT('Ctrl Pts',(-23.4234796353544,7.62439543920054,
12.));
#237606=CARTESIAN_POINT('Ctrl Pts',(-23.3994699961122,7.62675691240335,
0.));
#237607=CARTESIAN_POINT('Ctrl Pts',(-23.3994699961122,7.62675691240335,
12.));
#237608=CARTESIAN_POINT('Ctrl Pts',(-23.3755404996638,7.62905146332598,
0.));
#237609=CARTESIAN_POINT('Ctrl Pts',(-23.3755404996638,7.62905146332598,
12.));
#237610=CARTESIAN_POINT('Ctrl Pts',(-23.3516917421973,7.63127934048139,
0.));
#237611=CARTESIAN_POINT('Ctrl Pts',(-23.3516917421973,7.63127934048139,
12.));
#237612=CARTESIAN_POINT('Ctrl Pts',(-23.3279243245241,7.63344079578162,
0.));
#237613=CARTESIAN_POINT('Ctrl Pts',(-23.3279243245241,7.63344079578162,
12.));
#237614=CARTESIAN_POINT('Ctrl Pts',(-23.3042388521021,7.63553608458784,
0.));
#237615=CARTESIAN_POINT('Ctrl Pts',(-23.3042388521021,7.63553608458784,
12.));
#237616=CARTESIAN_POINT('Ctrl Pts',(-23.2806359350853,7.63756546576375,
0.));
#237617=CARTESIAN_POINT('Ctrl Pts',(-23.2806359350853,7.63756546576375,
12.));
#237618=CARTESIAN_POINT('Ctrl Pts',(-23.2571161884487,7.63952920172837,
0.));
#237619=CARTESIAN_POINT('Ctrl Pts',(-23.2571161884487,7.63952920172837,
12.));
#237620=CARTESIAN_POINT('Ctrl Pts',(-23.2336802320912,7.64142755851508,
0.));
#237621=CARTESIAN_POINT('Ctrl Pts',(-23.2336802320912,7.64142755851508,
12.));
#237622=CARTESIAN_POINT('Ctrl Pts',(-23.2103286909399,7.64326080583684,
0.));
#237623=CARTESIAN_POINT('Ctrl Pts',(-23.2103286909399,7.64326080583684,
12.));
#237624=CARTESIAN_POINT('Ctrl Pts',(-23.1870621950452,7.64502921715483,
0.));
#237625=CARTESIAN_POINT('Ctrl Pts',(-23.1870621950452,7.64502921715483,
12.));
#237626=CARTESIAN_POINT('Ctrl Pts',(-23.1638813796691,7.64673306975797,
0.));
#237627=CARTESIAN_POINT('Ctrl Pts',(-23.1638813796691,7.64673306975797,
12.));
#237628=CARTESIAN_POINT('Ctrl Pts',(-23.1407868853815,7.64837264482929,
0.));
#237629=CARTESIAN_POINT('Ctrl Pts',(-23.1407868853815,7.64837264482929,
12.));
#237630=CARTESIAN_POINT('Ctrl Pts',(-23.1177793581674,7.64994822749845,
0.));
#237631=CARTESIAN_POINT('Ctrl Pts',(-23.1177793581674,7.64994822749845,
12.));
#237632=CARTESIAN_POINT('Ctrl Pts',(-23.0948594495246,7.65146010690464,
0.));
#237633=CARTESIAN_POINT('Ctrl Pts',(-23.0948594495246,7.65146010690464,
12.));
#237634=CARTESIAN_POINT('Ctrl Pts',(-23.072027816555,7.65290857626356,0.));
#237635=CARTESIAN_POINT('Ctrl Pts',(-23.072027816555,7.65290857626356,12.));
#237636=CARTESIAN_POINT('Ctrl Pts',(-23.049285122053,7.65429393293955,0.));
#237637=CARTESIAN_POINT('Ctrl Pts',(-23.049285122053,7.65429393293955,12.));
#237638=CARTESIAN_POINT('Ctrl Pts',(-23.0266320345792,7.65561647852555,
0.));
#237639=CARTESIAN_POINT('Ctrl Pts',(-23.0266320345792,7.65561647852555,
12.));
#237640=CARTESIAN_POINT('Ctrl Pts',(-23.004069228582,7.6568765189133,0.));
#237641=CARTESIAN_POINT('Ctrl Pts',(-23.004069228582,7.6568765189133,12.));
#237642=CARTESIAN_POINT('Ctrl Pts',(-22.9815973845301,7.65807436436453,
0.));
#237643=CARTESIAN_POINT('Ctrl Pts',(-22.9815973845301,7.65807436436453,
12.));
#237644=CARTESIAN_POINT('Ctrl Pts',(-22.9592171890332,7.65921032958912,
0.));
#237645=CARTESIAN_POINT('Ctrl Pts',(-22.9592171890332,7.65921032958912,
12.));
#237646=CARTESIAN_POINT('Ctrl Pts',(-22.9369293349592,7.66028473382777,
0.));
#237647=CARTESIAN_POINT('Ctrl Pts',(-22.9369293349592,7.66028473382777,
12.));
#237648=CARTESIAN_POINT('Ctrl Pts',(-22.9147345215418,7.661297900941,0.));
#237649=CARTESIAN_POINT('Ctrl Pts',(-22.9147345215418,7.661297900941,12.));
#237650=CARTESIAN_POINT('Ctrl Pts',(-22.8926334544879,7.66225015950147,
0.));
#237651=CARTESIAN_POINT('Ctrl Pts',(-22.8926334544879,7.66225015950147,
12.));
#237652=CARTESIAN_POINT('Ctrl Pts',(-22.870626846128,7.66314184287334,0.));
#237653=CARTESIAN_POINT('Ctrl Pts',(-22.870626846128,7.66314184287334,12.));
#237654=CARTESIAN_POINT('Ctrl Pts',(-22.8487154155569,7.66397328929805,
0.));
#237655=CARTESIAN_POINT('Ctrl Pts',(-22.8487154155569,7.66397328929805,
12.));
#237656=CARTESIAN_POINT('Ctrl Pts',(-22.8268998887679,7.66474484198553,
0.));
#237657=CARTESIAN_POINT('Ctrl Pts',(-22.8268998887679,7.66474484198553,
12.));
#237658=CARTESIAN_POINT('Ctrl Pts',(-22.8051809987834,7.66545684920987,
0.));
#237659=CARTESIAN_POINT('Ctrl Pts',(-22.8051809987834,7.66545684920987,
12.));
#237660=CARTESIAN_POINT('Ctrl Pts',(-22.7835594857697,7.66610966441259,
0.));
#237661=CARTESIAN_POINT('Ctrl Pts',(-22.7835594857697,7.66610966441259,
12.));
#237662=CARTESIAN_POINT('Ctrl Pts',(-22.7620360971839,7.66670364630273,
0.));
#237663=CARTESIAN_POINT('Ctrl Pts',(-22.7620360971839,7.66670364630273,
12.));
#237664=CARTESIAN_POINT('Ctrl Pts',(-22.7406115879508,7.66723915895412,
0.));
#237665=CARTESIAN_POINT('Ctrl Pts',(-22.7406115879508,7.66723915895412,
12.));
#237666=CARTESIAN_POINT('Ctrl Pts',(-22.7192867206242,7.6677165719101,0.));
#237667=CARTESIAN_POINT('Ctrl Pts',(-22.7192867206242,7.6677165719101,12.));
#237668=CARTESIAN_POINT('Ctrl Pts',(-22.6980622655446,7.66813626029276,
0.));
#237669=CARTESIAN_POINT('Ctrl Pts',(-22.6980622655446,7.66813626029276,
12.));
#237670=CARTESIAN_POINT('Ctrl Pts',(-22.6769390009889,7.66849860491763,
0.));
#237671=CARTESIAN_POINT('Ctrl Pts',(-22.6769390009889,7.66849860491763,
12.));
#237672=CARTESIAN_POINT('Ctrl Pts',(-22.6559177133133,7.66880399241354,
0.));
#237673=CARTESIAN_POINT('Ctrl Pts',(-22.6559177133133,7.66880399241354,
12.));
#237674=CARTESIAN_POINT('Ctrl Pts',(-22.6349991971547,7.66905281533745,
0.));
#237675=CARTESIAN_POINT('Ctrl Pts',(-22.6349991971547,7.66905281533745,
12.));
#237676=CARTESIAN_POINT('Ctrl Pts',(-22.6141842556248,7.66924547229435,
0.));
#237677=CARTESIAN_POINT('Ctrl Pts',(-22.6141842556248,7.66924547229435,
12.));
#237678=CARTESIAN_POINT('Ctrl Pts',(-22.5934737004955,7.66938236806241,
0.));
#237679=CARTESIAN_POINT('Ctrl Pts',(-22.5934737004955,7.66938236806241,
12.));
#237680=CARTESIAN_POINT('Ctrl Pts',(-22.5728683523829,7.66946391372299,
0.));
#237681=CARTESIAN_POINT('Ctrl Pts',(-22.5728683523829,7.66946391372299,
12.));
#237682=CARTESIAN_POINT('Ctrl Pts',(-22.5523690409109,7.66949052679671,
0.));
#237683=CARTESIAN_POINT('Ctrl Pts',(-22.5523690409109,7.66949052679671,
12.));
#237684=CARTESIAN_POINT('Ctrl Pts',(-22.5319766049191,7.66946263138116,
0.));
#237685=CARTESIAN_POINT('Ctrl Pts',(-22.5319766049191,7.66946263138116,
12.));
#237686=CARTESIAN_POINT('Ctrl Pts',(-22.5116918927023,7.66938065829082,
0.));
#237687=CARTESIAN_POINT('Ctrl Pts',(-22.5116918927023,7.66938065829082,
12.));
#237688=CARTESIAN_POINT('Ctrl Pts',(-22.4915157622308,7.66924504520302,
0.));
#237689=CARTESIAN_POINT('Ctrl Pts',(-22.4915157622308,7.66924504520302,
12.));
#237690=CARTESIAN_POINT('Ctrl Pts',(-22.47144908137,7.66905623680835,0.));
#237691=CARTESIAN_POINT('Ctrl Pts',(-22.47144908137,7.66905623680835,12.));
#237692=CARTESIAN_POINT('Ctrl Pts',(-22.4514927280863,7.6688146849666,0.));
#237693=CARTESIAN_POINT('Ctrl Pts',(-22.4514927280863,7.6688146849666,12.));
#237694=CARTESIAN_POINT('Ctrl Pts',(-22.4316475906616,7.66852084886745,
0.));
#237695=CARTESIAN_POINT('Ctrl Pts',(-22.4316475906616,7.66852084886745,
12.));
#237696=CARTESIAN_POINT('Ctrl Pts',(-22.411914567977,7.66817519519682,0.));
#237697=CARTESIAN_POINT('Ctrl Pts',(-22.411914567977,7.66817519519682,12.));
#237698=CARTESIAN_POINT('Ctrl Pts',(-22.3922945697782,7.66777819830819,
0.));
#237699=CARTESIAN_POINT('Ctrl Pts',(-22.3922945697782,7.66777819830819,
12.));
#237700=CARTESIAN_POINT('Ctrl Pts',(-22.3727885169361,7.66733034039887,
0.));
#237701=CARTESIAN_POINT('Ctrl Pts',(-22.3727885169361,7.66733034039887,
12.));
#237702=CARTESIAN_POINT('Ctrl Pts',(-22.3533973417013,7.66683211169134,
0.));
#237703=CARTESIAN_POINT('Ctrl Pts',(-22.3533973417013,7.66683211169134,
12.));
#237704=CARTESIAN_POINT('Ctrl Pts',(-22.3341219879454,7.66628401061905,
0.));
#237705=CARTESIAN_POINT('Ctrl Pts',(-22.3341219879454,7.66628401061905,
12.));
#237706=CARTESIAN_POINT('Ctrl Pts',(-22.3149634114823,7.66568654402441,
0.));
#237707=CARTESIAN_POINT('Ctrl Pts',(-22.3149634114823,7.66568654402441,
12.));
#237708=CARTESIAN_POINT('Ctrl Pts',(-22.2959225803925,7.66504022736262,
0.));
#237709=CARTESIAN_POINT('Ctrl Pts',(-22.2959225803925,7.66504022736262,
12.));
#237710=CARTESIAN_POINT('Ctrl Pts',(-22.2770004753332,7.66434558490972,
0.));
#237711=CARTESIAN_POINT('Ctrl Pts',(-22.2770004753332,7.66434558490972,
12.));
#237712=CARTESIAN_POINT('Ctrl Pts',(-22.2581980898487,7.66360314997662,
0.));
#237713=CARTESIAN_POINT('Ctrl Pts',(-22.2581980898487,7.66360314997662,
12.));
#237714=CARTESIAN_POINT('Ctrl Pts',(-22.239516430656,7.66281346512545,0.));
#237715=CARTESIAN_POINT('Ctrl Pts',(-22.239516430656,7.66281346512545,12.));
#237716=CARTESIAN_POINT('Ctrl Pts',(-22.2209565180098,7.66197708240435,
0.));
#237717=CARTESIAN_POINT('Ctrl Pts',(-22.2209565180098,7.66197708240435,
12.));
#237718=CARTESIAN_POINT('Ctrl Pts',(-22.2025193860972,7.66109456359292,
0.));
#237719=CARTESIAN_POINT('Ctrl Pts',(-22.2025193860972,7.66109456359292,
12.));
#237720=CARTESIAN_POINT('Ctrl Pts',(-22.1842060834092,7.66016648045008,
0.));
#237721=CARTESIAN_POINT('Ctrl Pts',(-22.1842060834092,7.66016648045008,
12.));
#237722=CARTESIAN_POINT('Ctrl Pts',(-22.1660176731174,7.65919341496925,
0.));
#237723=CARTESIAN_POINT('Ctrl Pts',(-22.1660176731174,7.65919341496925,
12.));
#237724=CARTESIAN_POINT('Ctrl Pts',(-22.1479552334206,7.65817595963351,
0.));
#237725=CARTESIAN_POINT('Ctrl Pts',(-22.1479552334206,7.65817595963351,
12.));
#237726=CARTESIAN_POINT('Ctrl Pts',(-22.1300198579671,7.65711471769407,
0.));
#237727=CARTESIAN_POINT('Ctrl Pts',(-22.1300198579671,7.65711471769407,
12.));
#237728=CARTESIAN_POINT('Ctrl Pts',(-22.1122126563327,7.65601030346819,
0.));
#237729=CARTESIAN_POINT('Ctrl Pts',(-22.1122126563327,7.65601030346819,
12.));
#237730=CARTESIAN_POINT('Ctrl Pts',(-22.094534754469,7.6548633426365,0.));
#237731=CARTESIAN_POINT('Ctrl Pts',(-22.094534754469,7.6548633426365,12.));
#237732=CARTESIAN_POINT('Ctrl Pts',(-22.0769872951596,7.65367447254945,
0.));
#237733=CARTESIAN_POINT('Ctrl Pts',(-22.0769872951596,7.65367447254945,
12.));
#237734=CARTESIAN_POINT('Ctrl Pts',(-22.0595714384432,7.65244434253104,
0.));
#237735=CARTESIAN_POINT('Ctrl Pts',(-22.0595714384432,7.65244434253104,
12.));
#237736=CARTESIAN_POINT('Ctrl Pts',(-22.0422883621176,7.65117361421346,
0.));
#237737=CARTESIAN_POINT('Ctrl Pts',(-22.0422883621176,7.65117361421346,
12.));
#237738=CARTESIAN_POINT('Ctrl Pts',(-22.0251392623209,7.64986296190156,
0.));
#237739=CARTESIAN_POINT('Ctrl Pts',(-22.0251392623209,7.64986296190156,
12.));
#237740=CARTESIAN_POINT('Ctrl Pts',(-22.0081253540773,7.64851307293346,
0.));
#237741=CARTESIAN_POINT('Ctrl Pts',(-22.0081253540773,7.64851307293346,
12.));
#237742=CARTESIAN_POINT('Ctrl Pts',(-21.9912478718542,7.64712464805258,
0.));
#237743=CARTESIAN_POINT('Ctrl Pts',(-21.9912478718542,7.64712464805258,
12.));
#237744=CARTESIAN_POINT('Ctrl Pts',(-21.97450807008,7.64569840177359,0.));
#237745=CARTESIAN_POINT('Ctrl Pts',(-21.97450807008,7.64569840177359,12.));
#237746=CARTESIAN_POINT('Ctrl Pts',(-21.9579072237653,7.64423506279153,
0.));
#237747=CARTESIAN_POINT('Ctrl Pts',(-21.9579072237653,7.64423506279153,
12.));
#237748=CARTESIAN_POINT('Ctrl Pts',(-21.9414466292074,7.64273537442706,
0.));
#237749=CARTESIAN_POINT('Ctrl Pts',(-21.9414466292074,7.64273537442706,
12.));
#237750=CARTESIAN_POINT('Ctrl Pts',(-21.9251276046546,7.6412000950654,0.));
#237751=CARTESIAN_POINT('Ctrl Pts',(-21.9251276046546,7.6412000950654,12.));
#237752=CARTESIAN_POINT('Ctrl Pts',(-21.9089514909873,7.63962999860916,
0.));
#237753=CARTESIAN_POINT('Ctrl Pts',(-21.9089514909873,7.63962999860916,
12.));
#237754=CARTESIAN_POINT('Ctrl Pts',(-21.8929196523511,7.63802587492007,
0.));
#237755=CARTESIAN_POINT('Ctrl Pts',(-21.8929196523511,7.63802587492007,
12.));
#237756=CARTESIAN_POINT('Ctrl Pts',(-21.8770334769492,7.63638853033367,
0.));
#237757=CARTESIAN_POINT('Ctrl Pts',(-21.8770334769492,7.63638853033367,
12.));
#237758=CARTESIAN_POINT('Ctrl Pts',(-21.8612943779086,7.63471878821203,
0.));
#237759=CARTESIAN_POINT('Ctrl Pts',(-21.8612943779086,7.63471878821203,
12.));
#237760=CARTESIAN_POINT('Ctrl Pts',(-21.8457037941084,7.63301748948936,
0.));
#237761=CARTESIAN_POINT('Ctrl Pts',(-21.8457037941084,7.63301748948936,
12.));
#237762=CARTESIAN_POINT('Ctrl Pts',(-21.8302631910197,7.6312854932304,0.));
#237763=CARTESIAN_POINT('Ctrl Pts',(-21.8302631910197,7.6312854932304,12.));
#237764=CARTESIAN_POINT('Ctrl Pts',(-21.8149740615093,7.62952367718151,
0.));
#237765=CARTESIAN_POINT('Ctrl Pts',(-21.8149740615093,7.62952367718151,
12.));
#237766=CARTESIAN_POINT('Ctrl Pts',(-21.7998379268583,7.62773293842409,
0.));
#237767=CARTESIAN_POINT('Ctrl Pts',(-21.7998379268583,7.62773293842409,
12.));
#237768=CARTESIAN_POINT('Ctrl Pts',(-21.7848563378022,7.62591419404521,
0.));
#237769=CARTESIAN_POINT('Ctrl Pts',(-21.7848563378022,7.62591419404521,
12.));
#237770=CARTESIAN_POINT('Ctrl Pts',(-21.7700308755583,7.62406838181164,
0.));
#237771=CARTESIAN_POINT('Ctrl Pts',(-21.7700308755583,7.62406838181164,
12.));
#237772=CARTESIAN_POINT('Ctrl Pts',(-21.7553631528329,7.62219646084226,
0.));
#237773=CARTESIAN_POINT('Ctrl Pts',(-21.7553631528329,7.62219646084226,
12.));
#237774=CARTESIAN_POINT('Ctrl Pts',(-21.7408548148657,7.62029941230855,
0.));
#237775=CARTESIAN_POINT('Ctrl Pts',(-21.7408548148657,7.62029941230855,
12.));
#237776=CARTESIAN_POINT('Ctrl Pts',(-21.7265075407977,7.61837824030541,
0.));
#237777=CARTESIAN_POINT('Ctrl Pts',(-21.7265075407977,7.61837824030541,
12.));
#237778=CARTESIAN_POINT('Ctrl Pts',(-21.7123230449835,7.61643397270425,
0.));
#237779=CARTESIAN_POINT('Ctrl Pts',(-21.7123230449835,7.61643397270425,
12.));
#237780=CARTESIAN_POINT('Ctrl Pts',(-21.6983030783321,7.61446766202787,
0.));
#237781=CARTESIAN_POINT('Ctrl Pts',(-21.6983030783321,7.61446766202787,
12.));
#237782=CARTESIAN_POINT('Ctrl Pts',(-21.6844494295813,7.61248038630265,
0.));
#237783=CARTESIAN_POINT('Ctrl Pts',(-21.6844494295813,7.61248038630265,
12.));
#237784=CARTESIAN_POINT('Ctrl Pts',(-21.6707639267573,7.6104732500095,0.));
#237785=CARTESIAN_POINT('Ctrl Pts',(-21.6707639267573,7.6104732500095,12.));
#237786=CARTESIAN_POINT('Ctrl Pts',(-21.6572484388079,7.60844738512872,
0.));
#237787=CARTESIAN_POINT('Ctrl Pts',(-21.6572484388079,7.60844738512872,
12.));
#237788=CARTESIAN_POINT('Ctrl Pts',(-21.6439048771743,7.60640395216358,
0.));
#237789=CARTESIAN_POINT('Ctrl Pts',(-21.6439048771743,7.60640395216358,
12.));
#237790=CARTESIAN_POINT('Ctrl Pts',(-21.6307351973823,7.604344141183,0.));
#237791=CARTESIAN_POINT('Ctrl Pts',(-21.6307351973823,7.604344141183,12.));
#237792=CARTESIAN_POINT('Ctrl Pts',(-21.6177414005991,7.60226917285432,
0.));
#237793=CARTESIAN_POINT('Ctrl Pts',(-21.6177414005991,7.60226917285432,
12.));
#237794=CARTESIAN_POINT('Ctrl Pts',(-21.6049255358843,7.60018029988238,
0.));
#237795=CARTESIAN_POINT('Ctrl Pts',(-21.6049255358843,7.60018029988238,
12.));
#237796=CARTESIAN_POINT('Ctrl Pts',(-21.5922897024466,7.59807880846192,
0.));
#237797=CARTESIAN_POINT('Ctrl Pts',(-21.5922897024466,7.59807880846192,
12.));
#237798=CARTESIAN_POINT('Ctrl Pts',(-21.5798360518978,7.59596601973588,
0.));
#237799=CARTESIAN_POINT('Ctrl Pts',(-21.5798360518978,7.59596601973588,
12.));
#237800=CARTESIAN_POINT('Ctrl Pts',(-21.5675667904728,7.5938432912493,0.));
#237801=CARTESIAN_POINT('Ctrl Pts',(-21.5675667904728,7.5938432912493,12.));
#237802=CARTESIAN_POINT('Ctrl Pts',(-21.5554841813465,7.59171201844793,
0.));
#237803=CARTESIAN_POINT('Ctrl Pts',(-21.5554841813465,7.59171201844793,
12.));
#237804=CARTESIAN_POINT('Ctrl Pts',(-21.5435905470113,7.58957363620026,
0.));
#237805=CARTESIAN_POINT('Ctrl Pts',(-21.5435905470113,7.58957363620026,
12.));
#237806=CARTESIAN_POINT('Ctrl Pts',(-21.5318882716735,7.58742962034834,
0.));
#237807=CARTESIAN_POINT('Ctrl Pts',(-21.5318882716735,7.58742962034834,
12.));
#237808=CARTESIAN_POINT('Ctrl Pts',(-21.5203798035294,7.58528148919113,
0.));
#237809=CARTESIAN_POINT('Ctrl Pts',(-21.5203798035294,7.58528148919113,
12.));
#237810=CARTESIAN_POINT('Ctrl Pts',(-21.5090676573866,7.58313080519158,
0.));
#237811=CARTESIAN_POINT('Ctrl Pts',(-21.5090676573866,7.58313080519158,
12.));
#237812=CARTESIAN_POINT('Ctrl Pts',(-21.497954419274,7.5809791779073,0.));
#237813=CARTESIAN_POINT('Ctrl Pts',(-21.497954419274,7.5809791779073,12.));
#237814=CARTESIAN_POINT('Ctrl Pts',(-21.4870427508193,7.57882826679131,
0.));
#237815=CARTESIAN_POINT('Ctrl Pts',(-21.4870427508193,7.57882826679131,
12.));
#237816=CARTESIAN_POINT('Ctrl Pts',(-21.4763353936766,7.57667978403002,
0.));
#237817=CARTESIAN_POINT('Ctrl Pts',(-21.4763353936766,7.57667978403002,
12.));
#237818=CARTESIAN_POINT('Ctrl Pts',(-21.4658351740135,7.57453549743435,
0.));
#237819=CARTESIAN_POINT('Ctrl Pts',(-21.4658351740135,7.57453549743435,
12.));
#237820=CARTESIAN_POINT('Ctrl Pts',(-21.4555450053147,7.57239723223521,
0.));
#237821=CARTESIAN_POINT('Ctrl Pts',(-21.4555450053147,7.57239723223521,
12.));
#237822=CARTESIAN_POINT('Ctrl Pts',(-21.445467890751,7.57026687261169,0.));
#237823=CARTESIAN_POINT('Ctrl Pts',(-21.445467890751,7.57026687261169,12.));
#237824=CARTESIAN_POINT('Ctrl Pts',(-21.435606926151,7.56814636360842,0.));
#237825=CARTESIAN_POINT('Ctrl Pts',(-21.435606926151,7.56814636360842,12.));
#237826=CARTESIAN_POINT('Ctrl Pts',(-21.4259653015732,7.56603771218706,
0.));
#237827=CARTESIAN_POINT('Ctrl Pts',(-21.4259653015732,7.56603771218706,
12.));
#237828=CARTESIAN_POINT('Ctrl Pts',(-21.4165463106252,7.56394299313682,
0.));
#237829=CARTESIAN_POINT('Ctrl Pts',(-21.4165463106252,7.56394299313682,
12.));
#237830=CARTESIAN_POINT('Ctrl Pts',(-21.4073533630364,7.56186435703622,
0.));
#237831=CARTESIAN_POINT('Ctrl Pts',(-21.4073533630364,7.56186435703622,
12.));
#237832=CARTESIAN_POINT('Ctrl Pts',(-21.3983899952988,7.55980403700615,
0.));
#237833=CARTESIAN_POINT('Ctrl Pts',(-21.3983899952988,7.55980403700615,
12.));
#237834=CARTESIAN_POINT('Ctrl Pts',(-21.3896598842119,7.55776435731422,
0.));
#237835=CARTESIAN_POINT('Ctrl Pts',(-21.3896598842119,7.55776435731422,
12.));
#237836=CARTESIAN_POINT('Ctrl Pts',(-21.3811668478933,7.55574773403507,
0.));
#237837=CARTESIAN_POINT('Ctrl Pts',(-21.3811668478933,7.55574773403507,
12.));
#237838=CARTESIAN_POINT('Ctrl Pts',(-21.3729148390244,7.55375667080032,
0.));
#237839=CARTESIAN_POINT('Ctrl Pts',(-21.3729148390244,7.55375667080032,
12.));
#237840=CARTESIAN_POINT('Ctrl Pts',(-21.3649079431864,7.55179375777441,
0.));
#237841=CARTESIAN_POINT('Ctrl Pts',(-21.3649079431864,7.55179375777441,
12.));
#237842=CARTESIAN_POINT('Ctrl Pts',(-21.3571503685853,7.54986166521306,
0.));
#237843=CARTESIAN_POINT('Ctrl Pts',(-21.3571503685853,7.54986166521306,
12.));
#237844=CARTESIAN_POINT('Ctrl Pts',(-21.349646476153,7.54796316246327,0.));
#237845=CARTESIAN_POINT('Ctrl Pts',(-21.349646476153,7.54796316246327,12.));
#237846=CARTESIAN_POINT('Ctrl Pts',(-21.3424008295038,7.54610114948351,
0.));
#237847=CARTESIAN_POINT('Ctrl Pts',(-21.3424008295038,7.54610114948351,
12.));
#237848=CARTESIAN_POINT('Ctrl Pts',(-21.3354182340149,7.54427868151268,
0.));
#237849=CARTESIAN_POINT('Ctrl Pts',(-21.3354182340149,7.54427868151268,
12.));
#237850=CARTESIAN_POINT('Ctrl Pts',(-21.328703791771,7.54249900377031,0.));
#237851=CARTESIAN_POINT('Ctrl Pts',(-21.328703791771,7.54249900377031,12.));
#237852=CARTESIAN_POINT('Ctrl Pts',(-21.3222628524165,7.5407655203828,0.));
#237853=CARTESIAN_POINT('Ctrl Pts',(-21.3222628524165,7.5407655203828,12.));
#237854=CARTESIAN_POINT('Ctrl Pts',(-21.3161009456256,7.53908175169899,
0.));
#237855=CARTESIAN_POINT('Ctrl Pts',(-21.3161009456256,7.53908175169899,
12.));
#237856=CARTESIAN_POINT('Ctrl Pts',(-21.3102237167729,7.53745129364619,
0.));
#237857=CARTESIAN_POINT('Ctrl Pts',(-21.3102237167729,7.53745129364619,
12.));
#237858=CARTESIAN_POINT('Ctrl Pts',(-21.3046368712156,7.53587778251743,
0.));
#237859=CARTESIAN_POINT('Ctrl Pts',(-21.3046368712156,7.53587778251743,
12.));
#237860=CARTESIAN_POINT('Ctrl Pts',(-21.2993464250717,7.53436505309949,
0.));
#237861=CARTESIAN_POINT('Ctrl Pts',(-21.2993464250717,7.53436505309949,
12.));
#237862=CARTESIAN_POINT('Ctrl Pts',(-21.2943588989331,7.53291726078526,
0.));
#237863=CARTESIAN_POINT('Ctrl Pts',(-21.2943588989331,7.53291726078526,
12.));
#237864=CARTESIAN_POINT('Ctrl Pts',(-21.2896816163843,7.53153906987847,
0.));
#237865=CARTESIAN_POINT('Ctrl Pts',(-21.2896816163843,7.53153906987847,
12.));
#237866=CARTESIAN_POINT('Ctrl Pts',(-21.2853226580658,7.53023562438221,
0.));
#237867=CARTESIAN_POINT('Ctrl Pts',(-21.2853226580658,7.53023562438221,
12.));
#237868=CARTESIAN_POINT('Ctrl Pts',(-21.2812902781143,7.52901217930407,
0.));
#237869=CARTESIAN_POINT('Ctrl Pts',(-21.2812902781143,7.52901217930407,
12.));
#237870=CARTESIAN_POINT('Ctrl Pts',(-21.2775925269651,7.52787386225343,
0.));
#237871=CARTESIAN_POINT('Ctrl Pts',(-21.2775925269651,7.52787386225343,
12.));
#237872=CARTESIAN_POINT('Ctrl Pts',(-21.2742366113578,7.5268252691856,0.));
#237873=CARTESIAN_POINT('Ctrl Pts',(-21.2742366113578,7.5268252691856,12.));
#237874=CARTESIAN_POINT('Ctrl Pts',(-21.2712301573465,7.52587126095544,
0.));
#237875=CARTESIAN_POINT('Ctrl Pts',(-21.2712301573465,7.52587126095544,
12.));
#237876=CARTESIAN_POINT('Ctrl Pts',(-21.2685823838672,7.52501770333522,
0.));
#237877=CARTESIAN_POINT('Ctrl Pts',(-21.2685823838672,7.52501770333522,
12.));
#237878=CARTESIAN_POINT('Ctrl Pts',(-21.266305915706,7.52427261074264,0.));
#237879=CARTESIAN_POINT('Ctrl Pts',(-21.266305915706,7.52427261074264,12.));
#237880=CARTESIAN_POINT('Ctrl Pts',(-21.2644161259965,7.52364573027521,
0.));
#237881=CARTESIAN_POINT('Ctrl Pts',(-21.2644161259965,7.52364573027521,
12.));
#237882=CARTESIAN_POINT('Ctrl Pts',(-21.262927782038,7.52314642316202,0.));
#237883=CARTESIAN_POINT('Ctrl Pts',(-21.262927782038,7.52314642316202,12.));
#237884=CARTESIAN_POINT('Ctrl Pts',(-21.261852128355,7.52278182242727,0.));
#237885=CARTESIAN_POINT('Ctrl Pts',(-21.261852128355,7.52278182242727,12.));
#237886=CARTESIAN_POINT('Ctrl Pts',(-21.2613260540651,7.52260064231736,
0.));
#237887=CARTESIAN_POINT('Ctrl Pts',(-21.2613260540651,7.52260064231736,
12.));
#237888=CARTESIAN_POINT('Ctrl Pts',(-21.261120447486,7.52252744144958,0.));
#237889=CARTESIAN_POINT('Ctrl Pts',(-21.261120447486,7.52252744144958,12.));
#237890=CARTESIAN_POINT('Ctrl Pts',(-21.2610673466883,7.52250649703992,
0.));
#237891=CARTESIAN_POINT('Ctrl Pts',(-21.2610673466883,7.52250649703992,
12.));
#237892=CARTESIAN_POINT('Ctrl Pts',(-21.2610617890679,7.52250298901265,
0.));
#237893=CARTESIAN_POINT('Ctrl Pts',(-21.2610617890679,7.52250298901265,
12.));
#237894=CARTESIAN_POINT('',(-24.9347862158358,7.36589684767345,0.));
#237895=CARTESIAN_POINT('Ctrl Pts',(-24.9347862158358,7.36589684767345,
0.));
#237896=CARTESIAN_POINT('Ctrl Pts',(-24.9292275670674,7.36721909028843,
0.));
#237897=CARTESIAN_POINT('Ctrl Pts',(-24.9181155530543,7.3698559312009,0.));
#237898=CARTESIAN_POINT('Ctrl Pts',(-24.901463382605,7.37378825961676,0.));
#237899=CARTESIAN_POINT('Ctrl Pts',(-24.8792921911115,7.3789854964027,0.));
#237900=CARTESIAN_POINT('Ctrl Pts',(-24.8516310625176,7.38540558903621,
0.));
#237901=CARTESIAN_POINT('Ctrl Pts',(-24.8240228520893,7.39174922585808,
0.));
#237902=CARTESIAN_POINT('Ctrl Pts',(-24.7964676646431,7.39801641583013,
0.));
#237903=CARTESIAN_POINT('Ctrl Pts',(-24.7689656668983,7.40420718661603,
0.));
#237904=CARTESIAN_POINT('Ctrl Pts',(-24.7415170994784,7.41032159082382,
0.));
#237905=CARTESIAN_POINT('Ctrl Pts',(-24.7141222950051,7.41635971481674,
0.));
#237906=CARTESIAN_POINT('Ctrl Pts',(-24.6867816727192,7.42232167766265,
0.));
#237907=CARTESIAN_POINT('Ctrl Pts',(-24.6594957128756,7.42820762159126,
0.));
#237908=CARTESIAN_POINT('Ctrl Pts',(-24.6322649369517,7.43401770489524,
0.));
#237909=CARTESIAN_POINT('Ctrl Pts',(-24.6050898852368,7.43975209375504,
0.));
#237910=CARTESIAN_POINT('Ctrl Pts',(-24.577971096086,7.44541095473134,0.));
#237911=CARTESIAN_POINT('Ctrl Pts',(-24.5509090831559,7.4509944465116,0.));
#237912=CARTESIAN_POINT('Ctrl Pts',(-24.5239043173072,7.45650271335862,
0.));
#237913=CARTESIAN_POINT('Ctrl Pts',(-24.4969572391483,7.46193588961463,
0.));
#237914=CARTESIAN_POINT('Ctrl Pts',(-24.4700682684524,7.46729410308786,
0.));
#237915=CARTESIAN_POINT('Ctrl Pts',(-24.443237814649,7.47257747883246,0.));
#237916=CARTESIAN_POINT('Ctrl Pts',(-24.4164662871163,7.47778614286565,
0.));
#237917=CARTESIAN_POINT('Ctrl Pts',(-24.3897541049254,7.48292022569301,
0.));
#237918=CARTESIAN_POINT('Ctrl Pts',(-24.3631017084524,7.48797986651908,
0.));
#237919=CARTESIAN_POINT('Ctrl Pts',(-24.3365095573685,7.4929652125242,0.));
#237920=CARTESIAN_POINT('Ctrl Pts',(-24.3099781253355,7.49787641695439,
0.));
#237921=CARTESIAN_POINT('Ctrl Pts',(-24.2835078958973,7.50271363765152,
0.));
#237922=CARTESIAN_POINT('Ctrl Pts',(-24.2570993577034,7.50747703535133,
0.));
#237923=CARTESIAN_POINT('Ctrl Pts',(-24.2307530003887,7.51216677222181,
0.));
#237924=CARTESIAN_POINT('Ctrl Pts',(-24.2044693092349,7.51678300997949,
0.));
#237925=CARTESIAN_POINT('Ctrl Pts',(-24.1782487641594,7.52132590953802,
0.));
#237926=CARTESIAN_POINT('Ctrl Pts',(-24.1520918425364,7.52579563201424,
0.));
#237927=CARTESIAN_POINT('Ctrl Pts',(-24.1259990209207,7.53019233935501,
0.));
#237928=CARTESIAN_POINT('Ctrl Pts',(-24.0999707772642,7.53451619514649,
0.));
#237929=CARTESIAN_POINT('Ctrl Pts',(-24.0740075927985,7.53876736531014,
0.));
#237930=CARTESIAN_POINT('Ctrl Pts',(-24.0481099543353,7.54294601896144,
0.));
#237931=CARTESIAN_POINT('Ctrl Pts',(-24.022278355453,7.5470523288591,0.));
#237932=CARTESIAN_POINT('Ctrl Pts',(-23.9965132953185,7.55108647097441,
0.));
#237933=CARTESIAN_POINT('Ctrl Pts',(-23.9708152779884,7.55504862424812,
0.));
#237934=CARTESIAN_POINT('Ctrl Pts',(-23.9451848115,7.55893897027682,0.));
#237935=CARTESIAN_POINT('Ctrl Pts',(-23.9196224070759,7.56275769304773,
0.));
#237936=CARTESIAN_POINT('Ctrl Pts',(-23.8941285782003,7.56650497863792,
0.));
#237937=CARTESIAN_POINT('Ctrl Pts',(-23.8687038399598,7.57018101500711,
0.));
#237938=CARTESIAN_POINT('Ctrl Pts',(-23.8433487096134,7.57378599219816,
0.));
#237939=CARTESIAN_POINT('Ctrl Pts',(-23.8180637069977,7.57732010249066,
0.));
#237940=CARTESIAN_POINT('Ctrl Pts',(-23.7928493549908,7.58078354058212,
0.));
#237941=CARTESIAN_POINT('Ctrl Pts',(-23.7677061799376,7.58417650376272,
0.));
#237942=CARTESIAN_POINT('Ctrl Pts',(-23.7426347121006,7.58749919210832,
0.));
#237943=CARTESIAN_POINT('Ctrl Pts',(-23.7176354860457,7.59075180865327,
0.));
#237944=CARTESIAN_POINT('Ctrl Pts',(-23.6927090405067,7.59393455934042,
0.));
#237945=CARTESIAN_POINT('Ctrl Pts',(-23.6678559182876,7.59704765299572,
0.));
#237946=CARTESIAN_POINT('Ctrl Pts',(-23.6430766661419,7.60009130130129,
0.));
#237947=CARTESIAN_POINT('Ctrl Pts',(-23.6183718346576,7.60306571877806,
0.));
#237948=CARTESIAN_POINT('Ctrl Pts',(-23.5937419781244,7.60597112277094,
0.));
#237949=CARTESIAN_POINT('Ctrl Pts',(-23.5691876544243,7.60880773344599,
0.));
#237950=CARTESIAN_POINT('Ctrl Pts',(-23.5447094252029,7.61157577385372,
0.));
#237951=CARTESIAN_POINT('Ctrl Pts',(-23.5203078560128,7.61427546999299,
0.));
#237952=CARTESIAN_POINT('Ctrl Pts',(-23.4959835164608,7.61690705088319,
0.));
#237953=CARTESIAN_POINT('Ctrl Pts',(-23.4717369803438,7.61947074863977,
0.));
#237954=CARTESIAN_POINT('Ctrl Pts',(-23.4475688257854,7.62196679855957,
0.));
#237955=CARTESIAN_POINT('Ctrl Pts',(-23.4234796353544,7.62439543920054,
0.));
#237956=CARTESIAN_POINT('Ctrl Pts',(-23.3994699961122,7.62675691240335,
0.));
#237957=CARTESIAN_POINT('Ctrl Pts',(-23.3755404996638,7.62905146332598,
0.));
#237958=CARTESIAN_POINT('Ctrl Pts',(-23.3516917421973,7.63127934048139,
0.));
#237959=CARTESIAN_POINT('Ctrl Pts',(-23.3279243245241,7.63344079578162,
0.));
#237960=CARTESIAN_POINT('Ctrl Pts',(-23.3042388521021,7.63553608458784,
0.));
#237961=CARTESIAN_POINT('Ctrl Pts',(-23.2806359350853,7.63756546576375,
0.));
#237962=CARTESIAN_POINT('Ctrl Pts',(-23.2571161884487,7.63952920172837,
0.));
#237963=CARTESIAN_POINT('Ctrl Pts',(-23.2336802320912,7.64142755851508,
0.));
#237964=CARTESIAN_POINT('Ctrl Pts',(-23.2103286909399,7.64326080583684,
0.));
#237965=CARTESIAN_POINT('Ctrl Pts',(-23.1870621950452,7.64502921715483,
0.));
#237966=CARTESIAN_POINT('Ctrl Pts',(-23.1638813796691,7.64673306975797,
0.));
#237967=CARTESIAN_POINT('Ctrl Pts',(-23.1407868853815,7.64837264482929,
0.));
#237968=CARTESIAN_POINT('Ctrl Pts',(-23.1177793581674,7.64994822749845,
0.));
#237969=CARTESIAN_POINT('Ctrl Pts',(-23.0948594495246,7.65146010690464,
0.));
#237970=CARTESIAN_POINT('Ctrl Pts',(-23.072027816555,7.65290857626356,0.));
#237971=CARTESIAN_POINT('Ctrl Pts',(-23.049285122053,7.65429393293955,0.));
#237972=CARTESIAN_POINT('Ctrl Pts',(-23.0266320345792,7.65561647852555,
0.));
#237973=CARTESIAN_POINT('Ctrl Pts',(-23.004069228582,7.6568765189133,0.));
#237974=CARTESIAN_POINT('Ctrl Pts',(-22.9815973845301,7.65807436436453,
0.));
#237975=CARTESIAN_POINT('Ctrl Pts',(-22.9592171890332,7.65921032958912,
0.));
#237976=CARTESIAN_POINT('Ctrl Pts',(-22.9369293349592,7.66028473382777,
0.));
#237977=CARTESIAN_POINT('Ctrl Pts',(-22.9147345215418,7.661297900941,0.));
#237978=CARTESIAN_POINT('Ctrl Pts',(-22.8926334544879,7.66225015950147,
0.));
#237979=CARTESIAN_POINT('Ctrl Pts',(-22.870626846128,7.66314184287334,0.));
#237980=CARTESIAN_POINT('Ctrl Pts',(-22.8487154155569,7.66397328929805,
0.));
#237981=CARTESIAN_POINT('Ctrl Pts',(-22.8268998887679,7.66474484198553,
0.));
#237982=CARTESIAN_POINT('Ctrl Pts',(-22.8051809987834,7.66545684920987,
0.));
#237983=CARTESIAN_POINT('Ctrl Pts',(-22.7835594857697,7.66610966441259,
0.));
#237984=CARTESIAN_POINT('Ctrl Pts',(-22.7620360971839,7.66670364630273,
0.));
#237985=CARTESIAN_POINT('Ctrl Pts',(-22.7406115879508,7.66723915895412,
0.));
#237986=CARTESIAN_POINT('Ctrl Pts',(-22.7192867206242,7.6677165719101,0.));
#237987=CARTESIAN_POINT('Ctrl Pts',(-22.6980622655446,7.66813626029276,
0.));
#237988=CARTESIAN_POINT('Ctrl Pts',(-22.6769390009889,7.66849860491763,
0.));
#237989=CARTESIAN_POINT('Ctrl Pts',(-22.6559177133133,7.66880399241354,
0.));
#237990=CARTESIAN_POINT('Ctrl Pts',(-22.6349991971547,7.66905281533745,
0.));
#237991=CARTESIAN_POINT('Ctrl Pts',(-22.6141842556248,7.66924547229435,
0.));
#237992=CARTESIAN_POINT('Ctrl Pts',(-22.5934737004955,7.66938236806241,
0.));
#237993=CARTESIAN_POINT('Ctrl Pts',(-22.5728683523829,7.66946391372299,
0.));
#237994=CARTESIAN_POINT('Ctrl Pts',(-22.5523690409109,7.66949052679671,
0.));
#237995=CARTESIAN_POINT('Ctrl Pts',(-22.5319766049191,7.66946263138116,
0.));
#237996=CARTESIAN_POINT('Ctrl Pts',(-22.5116918927023,7.66938065829082,
0.));
#237997=CARTESIAN_POINT('Ctrl Pts',(-22.4915157622308,7.66924504520302,
0.));
#237998=CARTESIAN_POINT('Ctrl Pts',(-22.47144908137,7.66905623680835,0.));
#237999=CARTESIAN_POINT('Ctrl Pts',(-22.4514927280863,7.6688146849666,0.));
#238000=CARTESIAN_POINT('Ctrl Pts',(-22.4316475906616,7.66852084886745,
0.));
#238001=CARTESIAN_POINT('Ctrl Pts',(-22.411914567977,7.66817519519682,0.));
#238002=CARTESIAN_POINT('Ctrl Pts',(-22.3922945697782,7.66777819830819,
0.));
#238003=CARTESIAN_POINT('Ctrl Pts',(-22.3727885169361,7.66733034039887,
0.));
#238004=CARTESIAN_POINT('Ctrl Pts',(-22.3533973417013,7.66683211169134,
0.));
#238005=CARTESIAN_POINT('Ctrl Pts',(-22.3341219879454,7.66628401061905,
0.));
#238006=CARTESIAN_POINT('Ctrl Pts',(-22.3149634114823,7.66568654402441,
0.));
#238007=CARTESIAN_POINT('Ctrl Pts',(-22.2959225803925,7.66504022736262,
0.));
#238008=CARTESIAN_POINT('Ctrl Pts',(-22.2770004753332,7.66434558490972,
0.));
#238009=CARTESIAN_POINT('Ctrl Pts',(-22.2581980898487,7.66360314997662,
0.));
#238010=CARTESIAN_POINT('Ctrl Pts',(-22.239516430656,7.66281346512545,0.));
#238011=CARTESIAN_POINT('Ctrl Pts',(-22.2209565180098,7.66197708240435,
0.));
#238012=CARTESIAN_POINT('Ctrl Pts',(-22.2025193860972,7.66109456359292,
0.));
#238013=CARTESIAN_POINT('Ctrl Pts',(-22.1842060834092,7.66016648045008,
0.));
#238014=CARTESIAN_POINT('Ctrl Pts',(-22.1660176731174,7.65919341496925,
0.));
#238015=CARTESIAN_POINT('Ctrl Pts',(-22.1479552334206,7.65817595963351,
0.));
#238016=CARTESIAN_POINT('Ctrl Pts',(-22.1300198579671,7.65711471769407,
0.));
#238017=CARTESIAN_POINT('Ctrl Pts',(-22.1122126563327,7.65601030346819,
0.));
#238018=CARTESIAN_POINT('Ctrl Pts',(-22.094534754469,7.6548633426365,0.));
#238019=CARTESIAN_POINT('Ctrl Pts',(-22.0769872951596,7.65367447254945,
0.));
#238020=CARTESIAN_POINT('Ctrl Pts',(-22.0595714384432,7.65244434253104,
0.));
#238021=CARTESIAN_POINT('Ctrl Pts',(-22.0422883621176,7.65117361421346,
0.));
#238022=CARTESIAN_POINT('Ctrl Pts',(-22.0251392623209,7.64986296190156,
0.));
#238023=CARTESIAN_POINT('Ctrl Pts',(-22.0081253540773,7.64851307293346,
0.));
#238024=CARTESIAN_POINT('Ctrl Pts',(-21.9912478718542,7.64712464805258,
0.));
#238025=CARTESIAN_POINT('Ctrl Pts',(-21.97450807008,7.64569840177359,0.));
#238026=CARTESIAN_POINT('Ctrl Pts',(-21.9579072237653,7.64423506279153,
0.));
#238027=CARTESIAN_POINT('Ctrl Pts',(-21.9414466292074,7.64273537442706,
0.));
#238028=CARTESIAN_POINT('Ctrl Pts',(-21.9251276046546,7.6412000950654,0.));
#238029=CARTESIAN_POINT('Ctrl Pts',(-21.9089514909873,7.63962999860916,
0.));
#238030=CARTESIAN_POINT('Ctrl Pts',(-21.8929196523511,7.63802587492007,
0.));
#238031=CARTESIAN_POINT('Ctrl Pts',(-21.8770334769492,7.63638853033367,
0.));
#238032=CARTESIAN_POINT('Ctrl Pts',(-21.8612943779086,7.63471878821203,
0.));
#238033=CARTESIAN_POINT('Ctrl Pts',(-21.8457037941084,7.63301748948936,
0.));
#238034=CARTESIAN_POINT('Ctrl Pts',(-21.8302631910197,7.6312854932304,0.));
#238035=CARTESIAN_POINT('Ctrl Pts',(-21.8149740615093,7.62952367718151,
0.));
#238036=CARTESIAN_POINT('Ctrl Pts',(-21.7998379268583,7.62773293842409,
0.));
#238037=CARTESIAN_POINT('Ctrl Pts',(-21.7848563378022,7.62591419404521,
0.));
#238038=CARTESIAN_POINT('Ctrl Pts',(-21.7700308755583,7.62406838181164,
0.));
#238039=CARTESIAN_POINT('Ctrl Pts',(-21.7553631528329,7.62219646084226,
0.));
#238040=CARTESIAN_POINT('Ctrl Pts',(-21.7408548148657,7.62029941230855,
0.));
#238041=CARTESIAN_POINT('Ctrl Pts',(-21.7265075407977,7.61837824030541,
0.));
#238042=CARTESIAN_POINT('Ctrl Pts',(-21.7123230449835,7.61643397270425,
0.));
#238043=CARTESIAN_POINT('Ctrl Pts',(-21.6983030783321,7.61446766202787,
0.));
#238044=CARTESIAN_POINT('Ctrl Pts',(-21.6844494295813,7.61248038630265,
0.));
#238045=CARTESIAN_POINT('Ctrl Pts',(-21.6707639267573,7.6104732500095,0.));
#238046=CARTESIAN_POINT('Ctrl Pts',(-21.6572484388079,7.60844738512872,
0.));
#238047=CARTESIAN_POINT('Ctrl Pts',(-21.6439048771743,7.60640395216358,
0.));
#238048=CARTESIAN_POINT('Ctrl Pts',(-21.6307351973823,7.604344141183,0.));
#238049=CARTESIAN_POINT('Ctrl Pts',(-21.6177414005991,7.60226917285432,
0.));
#238050=CARTESIAN_POINT('Ctrl Pts',(-21.6049255358843,7.60018029988238,
0.));
#238051=CARTESIAN_POINT('Ctrl Pts',(-21.5922897024466,7.59807880846192,
0.));
#238052=CARTESIAN_POINT('Ctrl Pts',(-21.5798360518978,7.59596601973588,
0.));
#238053=CARTESIAN_POINT('Ctrl Pts',(-21.5675667904728,7.5938432912493,0.));
#238054=CARTESIAN_POINT('Ctrl Pts',(-21.5554841813465,7.59171201844793,
0.));
#238055=CARTESIAN_POINT('Ctrl Pts',(-21.5435905470113,7.58957363620026,
0.));
#238056=CARTESIAN_POINT('Ctrl Pts',(-21.5318882716735,7.58742962034834,
0.));
#238057=CARTESIAN_POINT('Ctrl Pts',(-21.5203798035294,7.58528148919113,
0.));
#238058=CARTESIAN_POINT('Ctrl Pts',(-21.5090676573866,7.58313080519158,
0.));
#238059=CARTESIAN_POINT('Ctrl Pts',(-21.497954419274,7.5809791779073,0.));
#238060=CARTESIAN_POINT('Ctrl Pts',(-21.4870427508193,7.57882826679131,
0.));
#238061=CARTESIAN_POINT('Ctrl Pts',(-21.4763353936766,7.57667978403002,
0.));
#238062=CARTESIAN_POINT('Ctrl Pts',(-21.4658351740135,7.57453549743435,
0.));
#238063=CARTESIAN_POINT('Ctrl Pts',(-21.4555450053147,7.57239723223521,
0.));
#238064=CARTESIAN_POINT('Ctrl Pts',(-21.445467890751,7.57026687261169,0.));
#238065=CARTESIAN_POINT('Ctrl Pts',(-21.435606926151,7.56814636360842,0.));
#238066=CARTESIAN_POINT('Ctrl Pts',(-21.4259653015732,7.56603771218706,
0.));
#238067=CARTESIAN_POINT('Ctrl Pts',(-21.4165463106252,7.56394299313682,
0.));
#238068=CARTESIAN_POINT('Ctrl Pts',(-21.4073533630364,7.56186435703622,
0.));
#238069=CARTESIAN_POINT('Ctrl Pts',(-21.3983899952988,7.55980403700615,
0.));
#238070=CARTESIAN_POINT('Ctrl Pts',(-21.3896598842119,7.55776435731422,
0.));
#238071=CARTESIAN_POINT('Ctrl Pts',(-21.3811668478933,7.55574773403507,
0.));
#238072=CARTESIAN_POINT('Ctrl Pts',(-21.3729148390244,7.55375667080032,
0.));
#238073=CARTESIAN_POINT('Ctrl Pts',(-21.3649079431864,7.55179375777441,
0.));
#238074=CARTESIAN_POINT('Ctrl Pts',(-21.3571503685853,7.54986166521306,
0.));
#238075=CARTESIAN_POINT('Ctrl Pts',(-21.349646476153,7.54796316246327,0.));
#238076=CARTESIAN_POINT('Ctrl Pts',(-21.3424008295038,7.54610114948351,
0.));
#238077=CARTESIAN_POINT('Ctrl Pts',(-21.3354182340149,7.54427868151268,
0.));
#238078=CARTESIAN_POINT('Ctrl Pts',(-21.328703791771,7.54249900377031,0.));
#238079=CARTESIAN_POINT('Ctrl Pts',(-21.3222628524165,7.5407655203828,0.));
#238080=CARTESIAN_POINT('Ctrl Pts',(-21.3161009456256,7.53908175169899,
0.));
#238081=CARTESIAN_POINT('Ctrl Pts',(-21.3102237167729,7.53745129364619,
0.));
#238082=CARTESIAN_POINT('Ctrl Pts',(-21.3046368712156,7.53587778251743,
0.));
#238083=CARTESIAN_POINT('Ctrl Pts',(-21.2993464250717,7.53436505309949,
0.));
#238084=CARTESIAN_POINT('Ctrl Pts',(-21.2943588989331,7.53291726078526,
0.));
#238085=CARTESIAN_POINT('Ctrl Pts',(-21.2896816163843,7.53153906987847,
0.));
#238086=CARTESIAN_POINT('Ctrl Pts',(-21.2853226580658,7.53023562438221,
0.));
#238087=CARTESIAN_POINT('Ctrl Pts',(-21.2812902781143,7.52901217930407,
0.));
#238088=CARTESIAN_POINT('Ctrl Pts',(-21.2775925269651,7.52787386225343,
0.));
#238089=CARTESIAN_POINT('Ctrl Pts',(-21.2742366113578,7.5268252691856,0.));
#238090=CARTESIAN_POINT('Ctrl Pts',(-21.2712301573465,7.52587126095544,
0.));
#238091=CARTESIAN_POINT('Ctrl Pts',(-21.2685823838672,7.52501770333522,
0.));
#238092=CARTESIAN_POINT('Ctrl Pts',(-21.266305915706,7.52427261074264,0.));
#238093=CARTESIAN_POINT('Ctrl Pts',(-21.2644161259965,7.52364573027521,
0.));
#238094=CARTESIAN_POINT('Ctrl Pts',(-21.262927782038,7.52314642316202,0.));
#238095=CARTESIAN_POINT('Ctrl Pts',(-21.261852128355,7.52278182242727,0.));
#238096=CARTESIAN_POINT('Ctrl Pts',(-21.2613260540651,7.52260064231736,
0.));
#238097=CARTESIAN_POINT('Ctrl Pts',(-21.261120447486,7.52252744144958,0.));
#238098=CARTESIAN_POINT('Ctrl Pts',(-21.2610673466883,7.52250649703992,
0.));
#238099=CARTESIAN_POINT('Ctrl Pts',(-21.2610617890679,7.52250298901265,
0.));
#238100=CARTESIAN_POINT('',(-24.9347862158358,7.36589684767345,12.));
#238101=CARTESIAN_POINT('',(-24.9347862158358,7.36589684767345,0.));
#238102=CARTESIAN_POINT('Ctrl Pts',(-21.2610617890679,7.52250298901265,
12.));
#238103=CARTESIAN_POINT('Ctrl Pts',(-21.2610673466883,7.52250649703992,
12.));
#238104=CARTESIAN_POINT('Ctrl Pts',(-21.261120447486,7.52252744144958,12.));
#238105=CARTESIAN_POINT('Ctrl Pts',(-21.2613260540651,7.52260064231736,
12.));
#238106=CARTESIAN_POINT('Ctrl Pts',(-21.261852128355,7.52278182242727,12.));
#238107=CARTESIAN_POINT('Ctrl Pts',(-21.262927782038,7.52314642316202,12.));
#238108=CARTESIAN_POINT('Ctrl Pts',(-21.2644161259965,7.52364573027521,
12.));
#238109=CARTESIAN_POINT('Ctrl Pts',(-21.266305915706,7.52427261074264,12.));
#238110=CARTESIAN_POINT('Ctrl Pts',(-21.2685823838672,7.52501770333522,
12.));
#238111=CARTESIAN_POINT('Ctrl Pts',(-21.2712301573465,7.52587126095544,
12.));
#238112=CARTESIAN_POINT('Ctrl Pts',(-21.2742366113578,7.5268252691856,12.));
#238113=CARTESIAN_POINT('Ctrl Pts',(-21.2775925269651,7.52787386225343,
12.));
#238114=CARTESIAN_POINT('Ctrl Pts',(-21.2812902781143,7.52901217930407,
12.));
#238115=CARTESIAN_POINT('Ctrl Pts',(-21.2853226580658,7.53023562438221,
12.));
#238116=CARTESIAN_POINT('Ctrl Pts',(-21.2896816163843,7.53153906987847,
12.));
#238117=CARTESIAN_POINT('Ctrl Pts',(-21.2943588989331,7.53291726078526,
12.));
#238118=CARTESIAN_POINT('Ctrl Pts',(-21.2993464250717,7.53436505309949,
12.));
#238119=CARTESIAN_POINT('Ctrl Pts',(-21.3046368712156,7.53587778251743,
12.));
#238120=CARTESIAN_POINT('Ctrl Pts',(-21.3102237167729,7.53745129364619,
12.));
#238121=CARTESIAN_POINT('Ctrl Pts',(-21.3161009456256,7.53908175169899,
12.));
#238122=CARTESIAN_POINT('Ctrl Pts',(-21.3222628524165,7.5407655203828,12.));
#238123=CARTESIAN_POINT('Ctrl Pts',(-21.328703791771,7.54249900377031,12.));
#238124=CARTESIAN_POINT('Ctrl Pts',(-21.3354182340149,7.54427868151268,
12.));
#238125=CARTESIAN_POINT('Ctrl Pts',(-21.3424008295038,7.54610114948351,
12.));
#238126=CARTESIAN_POINT('Ctrl Pts',(-21.349646476153,7.54796316246327,12.));
#238127=CARTESIAN_POINT('Ctrl Pts',(-21.3571503685853,7.54986166521306,
12.));
#238128=CARTESIAN_POINT('Ctrl Pts',(-21.3649079431864,7.55179375777441,
12.));
#238129=CARTESIAN_POINT('Ctrl Pts',(-21.3729148390244,7.55375667080032,
12.));
#238130=CARTESIAN_POINT('Ctrl Pts',(-21.3811668478933,7.55574773403507,
12.));
#238131=CARTESIAN_POINT('Ctrl Pts',(-21.3896598842119,7.55776435731422,
12.));
#238132=CARTESIAN_POINT('Ctrl Pts',(-21.3983899952988,7.55980403700615,
12.));
#238133=CARTESIAN_POINT('Ctrl Pts',(-21.4073533630364,7.56186435703622,
12.));
#238134=CARTESIAN_POINT('Ctrl Pts',(-21.4165463106252,7.56394299313682,
12.));
#238135=CARTESIAN_POINT('Ctrl Pts',(-21.4259653015732,7.56603771218706,
12.));
#238136=CARTESIAN_POINT('Ctrl Pts',(-21.435606926151,7.56814636360842,12.));
#238137=CARTESIAN_POINT('Ctrl Pts',(-21.445467890751,7.57026687261169,12.));
#238138=CARTESIAN_POINT('Ctrl Pts',(-21.4555450053147,7.57239723223521,
12.));
#238139=CARTESIAN_POINT('Ctrl Pts',(-21.4658351740135,7.57453549743435,
12.));
#238140=CARTESIAN_POINT('Ctrl Pts',(-21.4763353936766,7.57667978403002,
12.));
#238141=CARTESIAN_POINT('Ctrl Pts',(-21.4870427508193,7.57882826679131,
12.));
#238142=CARTESIAN_POINT('Ctrl Pts',(-21.497954419274,7.5809791779073,12.));
#238143=CARTESIAN_POINT('Ctrl Pts',(-21.5090676573866,7.58313080519158,
12.));
#238144=CARTESIAN_POINT('Ctrl Pts',(-21.5203798035294,7.58528148919113,
12.));
#238145=CARTESIAN_POINT('Ctrl Pts',(-21.5318882716735,7.58742962034834,
12.));
#238146=CARTESIAN_POINT('Ctrl Pts',(-21.5435905470113,7.58957363620026,
12.));
#238147=CARTESIAN_POINT('Ctrl Pts',(-21.5554841813465,7.59171201844793,
12.));
#238148=CARTESIAN_POINT('Ctrl Pts',(-21.5675667904728,7.5938432912493,12.));
#238149=CARTESIAN_POINT('Ctrl Pts',(-21.5798360518978,7.59596601973588,
12.));
#238150=CARTESIAN_POINT('Ctrl Pts',(-21.5922897024466,7.59807880846192,
12.));
#238151=CARTESIAN_POINT('Ctrl Pts',(-21.6049255358843,7.60018029988238,
12.));
#238152=CARTESIAN_POINT('Ctrl Pts',(-21.6177414005991,7.60226917285432,
12.));
#238153=CARTESIAN_POINT('Ctrl Pts',(-21.6307351973823,7.604344141183,12.));
#238154=CARTESIAN_POINT('Ctrl Pts',(-21.6439048771743,7.60640395216358,
12.));
#238155=CARTESIAN_POINT('Ctrl Pts',(-21.6572484388079,7.60844738512872,
12.));
#238156=CARTESIAN_POINT('Ctrl Pts',(-21.6707639267573,7.6104732500095,12.));
#238157=CARTESIAN_POINT('Ctrl Pts',(-21.6844494295813,7.61248038630265,
12.));
#238158=CARTESIAN_POINT('Ctrl Pts',(-21.6983030783321,7.61446766202787,
12.));
#238159=CARTESIAN_POINT('Ctrl Pts',(-21.7123230449835,7.61643397270425,
12.));
#238160=CARTESIAN_POINT('Ctrl Pts',(-21.7265075407977,7.61837824030541,
12.));
#238161=CARTESIAN_POINT('Ctrl Pts',(-21.7408548148657,7.62029941230855,
12.));
#238162=CARTESIAN_POINT('Ctrl Pts',(-21.7553631528329,7.62219646084226,
12.));
#238163=CARTESIAN_POINT('Ctrl Pts',(-21.7700308755583,7.62406838181164,
12.));
#238164=CARTESIAN_POINT('Ctrl Pts',(-21.7848563378022,7.62591419404521,
12.));
#238165=CARTESIAN_POINT('Ctrl Pts',(-21.7998379268583,7.62773293842409,
12.));
#238166=CARTESIAN_POINT('Ctrl Pts',(-21.8149740615093,7.62952367718151,
12.));
#238167=CARTESIAN_POINT('Ctrl Pts',(-21.8302631910197,7.6312854932304,12.));
#238168=CARTESIAN_POINT('Ctrl Pts',(-21.8457037941084,7.63301748948936,
12.));
#238169=CARTESIAN_POINT('Ctrl Pts',(-21.8612943779086,7.63471878821203,
12.));
#238170=CARTESIAN_POINT('Ctrl Pts',(-21.8770334769492,7.63638853033367,
12.));
#238171=CARTESIAN_POINT('Ctrl Pts',(-21.8929196523511,7.63802587492007,
12.));
#238172=CARTESIAN_POINT('Ctrl Pts',(-21.9089514909873,7.63962999860916,
12.));
#238173=CARTESIAN_POINT('Ctrl Pts',(-21.9251276046546,7.6412000950654,12.));
#238174=CARTESIAN_POINT('Ctrl Pts',(-21.9414466292074,7.64273537442706,
12.));
#238175=CARTESIAN_POINT('Ctrl Pts',(-21.9579072237653,7.64423506279153,
12.));
#238176=CARTESIAN_POINT('Ctrl Pts',(-21.97450807008,7.64569840177359,12.));
#238177=CARTESIAN_POINT('Ctrl Pts',(-21.9912478718542,7.64712464805258,
12.));
#238178=CARTESIAN_POINT('Ctrl Pts',(-22.0081253540773,7.64851307293346,
12.));
#238179=CARTESIAN_POINT('Ctrl Pts',(-22.0251392623209,7.64986296190156,
12.));
#238180=CARTESIAN_POINT('Ctrl Pts',(-22.0422883621176,7.65117361421346,
12.));
#238181=CARTESIAN_POINT('Ctrl Pts',(-22.0595714384432,7.65244434253104,
12.));
#238182=CARTESIAN_POINT('Ctrl Pts',(-22.0769872951596,7.65367447254945,
12.));
#238183=CARTESIAN_POINT('Ctrl Pts',(-22.094534754469,7.6548633426365,12.));
#238184=CARTESIAN_POINT('Ctrl Pts',(-22.1122126563327,7.65601030346819,
12.));
#238185=CARTESIAN_POINT('Ctrl Pts',(-22.1300198579671,7.65711471769407,
12.));
#238186=CARTESIAN_POINT('Ctrl Pts',(-22.1479552334206,7.65817595963351,
12.));
#238187=CARTESIAN_POINT('Ctrl Pts',(-22.1660176731174,7.65919341496925,
12.));
#238188=CARTESIAN_POINT('Ctrl Pts',(-22.1842060834092,7.66016648045008,
12.));
#238189=CARTESIAN_POINT('Ctrl Pts',(-22.2025193860972,7.66109456359292,
12.));
#238190=CARTESIAN_POINT('Ctrl Pts',(-22.2209565180098,7.66197708240435,
12.));
#238191=CARTESIAN_POINT('Ctrl Pts',(-22.239516430656,7.66281346512545,12.));
#238192=CARTESIAN_POINT('Ctrl Pts',(-22.2581980898487,7.66360314997662,
12.));
#238193=CARTESIAN_POINT('Ctrl Pts',(-22.2770004753332,7.66434558490972,
12.));
#238194=CARTESIAN_POINT('Ctrl Pts',(-22.2959225803925,7.66504022736262,
12.));
#238195=CARTESIAN_POINT('Ctrl Pts',(-22.3149634114823,7.66568654402441,
12.));
#238196=CARTESIAN_POINT('Ctrl Pts',(-22.3341219879454,7.66628401061905,
12.));
#238197=CARTESIAN_POINT('Ctrl Pts',(-22.3533973417013,7.66683211169134,
12.));
#238198=CARTESIAN_POINT('Ctrl Pts',(-22.3727885169361,7.66733034039887,
12.));
#238199=CARTESIAN_POINT('Ctrl Pts',(-22.3922945697782,7.66777819830819,
12.));
#238200=CARTESIAN_POINT('Ctrl Pts',(-22.411914567977,7.66817519519682,12.));
#238201=CARTESIAN_POINT('Ctrl Pts',(-22.4316475906616,7.66852084886745,
12.));
#238202=CARTESIAN_POINT('Ctrl Pts',(-22.4514927280863,7.6688146849666,12.));
#238203=CARTESIAN_POINT('Ctrl Pts',(-22.47144908137,7.66905623680835,12.));
#238204=CARTESIAN_POINT('Ctrl Pts',(-22.4915157622308,7.66924504520302,
12.));
#238205=CARTESIAN_POINT('Ctrl Pts',(-22.5116918927023,7.66938065829082,
12.));
#238206=CARTESIAN_POINT('Ctrl Pts',(-22.5319766049191,7.66946263138116,
12.));
#238207=CARTESIAN_POINT('Ctrl Pts',(-22.5523690409109,7.66949052679671,
12.));
#238208=CARTESIAN_POINT('Ctrl Pts',(-22.5728683523829,7.66946391372299,
12.));
#238209=CARTESIAN_POINT('Ctrl Pts',(-22.5934737004955,7.66938236806241,
12.));
#238210=CARTESIAN_POINT('Ctrl Pts',(-22.6141842556248,7.66924547229435,
12.));
#238211=CARTESIAN_POINT('Ctrl Pts',(-22.6349991971547,7.66905281533745,
12.));
#238212=CARTESIAN_POINT('Ctrl Pts',(-22.6559177133133,7.66880399241354,
12.));
#238213=CARTESIAN_POINT('Ctrl Pts',(-22.6769390009889,7.66849860491763,
12.));
#238214=CARTESIAN_POINT('Ctrl Pts',(-22.6980622655446,7.66813626029276,
12.));
#238215=CARTESIAN_POINT('Ctrl Pts',(-22.7192867206242,7.6677165719101,12.));
#238216=CARTESIAN_POINT('Ctrl Pts',(-22.7406115879508,7.66723915895412,
12.));
#238217=CARTESIAN_POINT('Ctrl Pts',(-22.7620360971839,7.66670364630273,
12.));
#238218=CARTESIAN_POINT('Ctrl Pts',(-22.7835594857697,7.66610966441259,
12.));
#238219=CARTESIAN_POINT('Ctrl Pts',(-22.8051809987834,7.66545684920987,
12.));
#238220=CARTESIAN_POINT('Ctrl Pts',(-22.8268998887679,7.66474484198553,
12.));
#238221=CARTESIAN_POINT('Ctrl Pts',(-22.8487154155569,7.66397328929805,
12.));
#238222=CARTESIAN_POINT('Ctrl Pts',(-22.870626846128,7.66314184287334,12.));
#238223=CARTESIAN_POINT('Ctrl Pts',(-22.8926334544879,7.66225015950147,
12.));
#238224=CARTESIAN_POINT('Ctrl Pts',(-22.9147345215418,7.661297900941,12.));
#238225=CARTESIAN_POINT('Ctrl Pts',(-22.9369293349592,7.66028473382777,
12.));
#238226=CARTESIAN_POINT('Ctrl Pts',(-22.9592171890332,7.65921032958912,
12.));
#238227=CARTESIAN_POINT('Ctrl Pts',(-22.9815973845301,7.65807436436453,
12.));
#238228=CARTESIAN_POINT('Ctrl Pts',(-23.004069228582,7.6568765189133,12.));
#238229=CARTESIAN_POINT('Ctrl Pts',(-23.0266320345792,7.65561647852555,
12.));
#238230=CARTESIAN_POINT('Ctrl Pts',(-23.049285122053,7.65429393293955,12.));
#238231=CARTESIAN_POINT('Ctrl Pts',(-23.072027816555,7.65290857626356,12.));
#238232=CARTESIAN_POINT('Ctrl Pts',(-23.0948594495246,7.65146010690464,
12.));
#238233=CARTESIAN_POINT('Ctrl Pts',(-23.1177793581674,7.64994822749845,
12.));
#238234=CARTESIAN_POINT('Ctrl Pts',(-23.1407868853815,7.64837264482929,
12.));
#238235=CARTESIAN_POINT('Ctrl Pts',(-23.1638813796691,7.64673306975797,
12.));
#238236=CARTESIAN_POINT('Ctrl Pts',(-23.1870621950452,7.64502921715483,
12.));
#238237=CARTESIAN_POINT('Ctrl Pts',(-23.2103286909399,7.64326080583684,
12.));
#238238=CARTESIAN_POINT('Ctrl Pts',(-23.2336802320912,7.64142755851508,
12.));
#238239=CARTESIAN_POINT('Ctrl Pts',(-23.2571161884487,7.63952920172837,
12.));
#238240=CARTESIAN_POINT('Ctrl Pts',(-23.2806359350853,7.63756546576375,
12.));
#238241=CARTESIAN_POINT('Ctrl Pts',(-23.3042388521021,7.63553608458784,
12.));
#238242=CARTESIAN_POINT('Ctrl Pts',(-23.3279243245241,7.63344079578162,
12.));
#238243=CARTESIAN_POINT('Ctrl Pts',(-23.3516917421973,7.63127934048139,
12.));
#238244=CARTESIAN_POINT('Ctrl Pts',(-23.3755404996638,7.62905146332598,
12.));
#238245=CARTESIAN_POINT('Ctrl Pts',(-23.3994699961122,7.62675691240335,
12.));
#238246=CARTESIAN_POINT('Ctrl Pts',(-23.4234796353544,7.62439543920054,
12.));
#238247=CARTESIAN_POINT('Ctrl Pts',(-23.4475688257854,7.62196679855957,
12.));
#238248=CARTESIAN_POINT('Ctrl Pts',(-23.4717369803438,7.61947074863977,
12.));
#238249=CARTESIAN_POINT('Ctrl Pts',(-23.4959835164608,7.61690705088319,
12.));
#238250=CARTESIAN_POINT('Ctrl Pts',(-23.5203078560128,7.61427546999299,
12.));
#238251=CARTESIAN_POINT('Ctrl Pts',(-23.5447094252029,7.61157577385372,
12.));
#238252=CARTESIAN_POINT('Ctrl Pts',(-23.5691876544243,7.60880773344599,
12.));
#238253=CARTESIAN_POINT('Ctrl Pts',(-23.5937419781244,7.60597112277094,
12.));
#238254=CARTESIAN_POINT('Ctrl Pts',(-23.6183718346576,7.60306571877806,
12.));
#238255=CARTESIAN_POINT('Ctrl Pts',(-23.6430766661419,7.60009130130129,
12.));
#238256=CARTESIAN_POINT('Ctrl Pts',(-23.6678559182876,7.59704765299572,
12.));
#238257=CARTESIAN_POINT('Ctrl Pts',(-23.6927090405067,7.59393455934042,
12.));
#238258=CARTESIAN_POINT('Ctrl Pts',(-23.7176354860457,7.59075180865327,
12.));
#238259=CARTESIAN_POINT('Ctrl Pts',(-23.7426347121006,7.58749919210832,
12.));
#238260=CARTESIAN_POINT('Ctrl Pts',(-23.7677061799376,7.58417650376272,
12.));
#238261=CARTESIAN_POINT('Ctrl Pts',(-23.7928493549908,7.58078354058212,
12.));
#238262=CARTESIAN_POINT('Ctrl Pts',(-23.8180637069977,7.57732010249066,
12.));
#238263=CARTESIAN_POINT('Ctrl Pts',(-23.8433487096134,7.57378599219816,
12.));
#238264=CARTESIAN_POINT('Ctrl Pts',(-23.8687038399598,7.57018101500711,
12.));
#238265=CARTESIAN_POINT('Ctrl Pts',(-23.8941285782003,7.56650497863792,
12.));
#238266=CARTESIAN_POINT('Ctrl Pts',(-23.9196224070759,7.56275769304773,
12.));
#238267=CARTESIAN_POINT('Ctrl Pts',(-23.9451848115,7.55893897027682,12.));
#238268=CARTESIAN_POINT('Ctrl Pts',(-23.9708152779884,7.55504862424812,
12.));
#238269=CARTESIAN_POINT('Ctrl Pts',(-23.9965132953185,7.55108647097441,
12.));
#238270=CARTESIAN_POINT('Ctrl Pts',(-24.022278355453,7.5470523288591,12.));
#238271=CARTESIAN_POINT('Ctrl Pts',(-24.0481099543353,7.54294601896144,
12.));
#238272=CARTESIAN_POINT('Ctrl Pts',(-24.0740075927985,7.53876736531014,
12.));
#238273=CARTESIAN_POINT('Ctrl Pts',(-24.0999707772642,7.53451619514649,
12.));
#238274=CARTESIAN_POINT('Ctrl Pts',(-24.1259990209207,7.53019233935501,
12.));
#238275=CARTESIAN_POINT('Ctrl Pts',(-24.1520918425364,7.52579563201424,
12.));
#238276=CARTESIAN_POINT('Ctrl Pts',(-24.1782487641594,7.52132590953802,
12.));
#238277=CARTESIAN_POINT('Ctrl Pts',(-24.2044693092349,7.51678300997949,
12.));
#238278=CARTESIAN_POINT('Ctrl Pts',(-24.2307530003887,7.51216677222181,
12.));
#238279=CARTESIAN_POINT('Ctrl Pts',(-24.2570993577034,7.50747703535133,
12.));
#238280=CARTESIAN_POINT('Ctrl Pts',(-24.2835078958973,7.50271363765152,
12.));
#238281=CARTESIAN_POINT('Ctrl Pts',(-24.3099781253355,7.49787641695439,
12.));
#238282=CARTESIAN_POINT('Ctrl Pts',(-24.3365095573685,7.4929652125242,12.));
#238283=CARTESIAN_POINT('Ctrl Pts',(-24.3631017084524,7.48797986651908,
12.));
#238284=CARTESIAN_POINT('Ctrl Pts',(-24.3897541049254,7.48292022569301,
12.));
#238285=CARTESIAN_POINT('Ctrl Pts',(-24.4164662871163,7.47778614286565,
12.));
#238286=CARTESIAN_POINT('Ctrl Pts',(-24.443237814649,7.47257747883246,12.));
#238287=CARTESIAN_POINT('Ctrl Pts',(-24.4700682684524,7.46729410308786,
12.));
#238288=CARTESIAN_POINT('Ctrl Pts',(-24.4969572391483,7.46193588961463,
12.));
#238289=CARTESIAN_POINT('Ctrl Pts',(-24.5239043173072,7.45650271335862,
12.));
#238290=CARTESIAN_POINT('Ctrl Pts',(-24.5509090831559,7.4509944465116,12.));
#238291=CARTESIAN_POINT('Ctrl Pts',(-24.577971096086,7.44541095473134,12.));
#238292=CARTESIAN_POINT('Ctrl Pts',(-24.6050898852368,7.43975209375504,
12.));
#238293=CARTESIAN_POINT('Ctrl Pts',(-24.6322649369517,7.43401770489524,
12.));
#238294=CARTESIAN_POINT('Ctrl Pts',(-24.6594957128756,7.42820762159126,
12.));
#238295=CARTESIAN_POINT('Ctrl Pts',(-24.6867816727192,7.42232167766265,
12.));
#238296=CARTESIAN_POINT('Ctrl Pts',(-24.7141222950051,7.41635971481674,
12.));
#238297=CARTESIAN_POINT('Ctrl Pts',(-24.7415170994784,7.41032159082382,
12.));
#238298=CARTESIAN_POINT('Ctrl Pts',(-24.7689656668983,7.40420718661603,
12.));
#238299=CARTESIAN_POINT('Ctrl Pts',(-24.7964676646431,7.39801641583013,
12.));
#238300=CARTESIAN_POINT('Ctrl Pts',(-24.8240228520893,7.39174922585808,
12.));
#238301=CARTESIAN_POINT('Ctrl Pts',(-24.8516310625176,7.38540558903621,
12.));
#238302=CARTESIAN_POINT('Ctrl Pts',(-24.8792921911115,7.3789854964027,12.));
#238303=CARTESIAN_POINT('Ctrl Pts',(-24.901463382605,7.37378825961676,12.));
#238304=CARTESIAN_POINT('Ctrl Pts',(-24.9181155530543,7.3698559312009,12.));
#238305=CARTESIAN_POINT('Ctrl Pts',(-24.9292275670674,7.36721909028843,
12.));
#238306=CARTESIAN_POINT('Ctrl Pts',(-24.9347862158358,7.36589684767345,
12.));
#238307=CARTESIAN_POINT('Ctrl Pts',(-20.353053841303,9.71462809124917,0.));
#238308=CARTESIAN_POINT('Ctrl Pts',(-20.353053841303,9.71462809124917,12.));
#238309=CARTESIAN_POINT('Ctrl Pts',(-20.353060251684,9.71462954053074,0.));
#238310=CARTESIAN_POINT('Ctrl Pts',(-20.353060251684,9.71462954053074,12.));
#238311=CARTESIAN_POINT('Ctrl Pts',(-20.3531126095522,9.71465227853122,
0.));
#238312=CARTESIAN_POINT('Ctrl Pts',(-20.3531126095522,9.71465227853122,
12.));
#238313=CARTESIAN_POINT('Ctrl Pts',(-20.3533097561886,9.71474590350791,
0.));
#238314=CARTESIAN_POINT('Ctrl Pts',(-20.3533097561886,9.71474590350791,
12.));
#238315=CARTESIAN_POINT('Ctrl Pts',(-20.3538098605706,9.71498978052101,
0.));
#238316=CARTESIAN_POINT('Ctrl Pts',(-20.3538098605706,9.71498978052101,
12.));
#238317=CARTESIAN_POINT('Ctrl Pts',(-20.3548282742361,9.71549257088175,
0.));
#238318=CARTESIAN_POINT('Ctrl Pts',(-20.3548282742361,9.71549257088175,
12.));
#238319=CARTESIAN_POINT('Ctrl Pts',(-20.3562337557875,9.71619192554147,
0.));
#238320=CARTESIAN_POINT('Ctrl Pts',(-20.3562337557875,9.71619192554147,
12.));
#238321=CARTESIAN_POINT('Ctrl Pts',(-20.3580133103357,9.71708493723061,
0.));
#238322=CARTESIAN_POINT('Ctrl Pts',(-20.3580133103357,9.71708493723061,
12.));
#238323=CARTESIAN_POINT('Ctrl Pts',(-20.3601498764344,9.71816778327999,
0.));
#238324=CARTESIAN_POINT('Ctrl Pts',(-20.3601498764344,9.71816778327999,
12.));
#238325=CARTESIAN_POINT('Ctrl Pts',(-20.362625691398,9.71943648548114,0.));
#238326=CARTESIAN_POINT('Ctrl Pts',(-20.362625691398,9.71943648548114,12.));
#238327=CARTESIAN_POINT('Ctrl Pts',(-20.3654261611055,9.72088778381102,
0.));
#238328=CARTESIAN_POINT('Ctrl Pts',(-20.3654261611055,9.72088778381102,
12.));
#238329=CARTESIAN_POINT('Ctrl Pts',(-20.3685406190576,9.72251930722504,
0.));
#238330=CARTESIAN_POINT('Ctrl Pts',(-20.3685406190576,9.72251930722504,
12.));
#238331=CARTESIAN_POINT('Ctrl Pts',(-20.371960235676,9.72432910043193,0.));
#238332=CARTESIAN_POINT('Ctrl Pts',(-20.371960235676,9.72432910043193,12.));
#238333=CARTESIAN_POINT('Ctrl Pts',(-20.3756766651952,9.72631531732871,
0.));
#238334=CARTESIAN_POINT('Ctrl Pts',(-20.3756766651952,9.72631531732871,
12.));
#238335=CARTESIAN_POINT('Ctrl Pts',(-20.3796805893304,9.72847589116533,
0.));
#238336=CARTESIAN_POINT('Ctrl Pts',(-20.3796805893304,9.72847589116533,
12.));
#238337=CARTESIAN_POINT('Ctrl Pts',(-20.3839624556742,9.73080870123726,
0.));
#238338=CARTESIAN_POINT('Ctrl Pts',(-20.3839624556742,9.73080870123726,
12.));
#238339=CARTESIAN_POINT('Ctrl Pts',(-20.3885129129912,9.73331167102812,
0.));
#238340=CARTESIAN_POINT('Ctrl Pts',(-20.3885129129912,9.73331167102812,
12.));
#238341=CARTESIAN_POINT('Ctrl Pts',(-20.3933234845646,9.7359829201425,0.));
#238342=CARTESIAN_POINT('Ctrl Pts',(-20.3933234845646,9.7359829201425,12.));
#238343=CARTESIAN_POINT('Ctrl Pts',(-20.3983866213331,9.73882077613206,
0.));
#238344=CARTESIAN_POINT('Ctrl Pts',(-20.3983866213331,9.73882077613206,
12.));
#238345=CARTESIAN_POINT('Ctrl Pts',(-20.4036953576549,9.74182369656272,
0.));
#238346=CARTESIAN_POINT('Ctrl Pts',(-20.4036953576549,9.74182369656272,
12.));
#238347=CARTESIAN_POINT('Ctrl Pts',(-20.4092430879861,9.74499021838536,
0.));
#238348=CARTESIAN_POINT('Ctrl Pts',(-20.4092430879861,9.74499021838536,
12.));
#238349=CARTESIAN_POINT('Ctrl Pts',(-20.4150232777393,9.74831889242175,
0.));
#238350=CARTESIAN_POINT('Ctrl Pts',(-20.4150232777393,9.74831889242175,
12.));
#238351=CARTESIAN_POINT('Ctrl Pts',(-20.4210295275818,9.75180829786433,
0.));
#238352=CARTESIAN_POINT('Ctrl Pts',(-20.4210295275818,9.75180829786433,
12.));
#238353=CARTESIAN_POINT('Ctrl Pts',(-20.4272556476629,9.75545705902416,
0.));
#238354=CARTESIAN_POINT('Ctrl Pts',(-20.4272556476629,9.75545705902416,
12.));
#238355=CARTESIAN_POINT('Ctrl Pts',(-20.4336957355474,9.7592638628993,0.));
#238356=CARTESIAN_POINT('Ctrl Pts',(-20.4336957355474,9.7592638628993,12.));
#238357=CARTESIAN_POINT('Ctrl Pts',(-20.4403442329401,9.76322747195502,
0.));
#238358=CARTESIAN_POINT('Ctrl Pts',(-20.4403442329401,9.76322747195502,
12.));
#238359=CARTESIAN_POINT('Ctrl Pts',(-20.447195862298,9.76734670980897,0.));
#238360=CARTESIAN_POINT('Ctrl Pts',(-20.447195862298,9.76734670980897,12.));
#238361=CARTESIAN_POINT('Ctrl Pts',(-20.4542455817527,9.7716204510407,0.));
#238362=CARTESIAN_POINT('Ctrl Pts',(-20.4542455817527,9.7716204510407,12.));
#238363=CARTESIAN_POINT('Ctrl Pts',(-20.4614885274973,9.77604760815523,
0.));
#238364=CARTESIAN_POINT('Ctrl Pts',(-20.4614885274973,9.77604760815523,
12.));
#238365=CARTESIAN_POINT('Ctrl Pts',(-20.4689199790668,9.78062712373313,
0.));
#238366=CARTESIAN_POINT('Ctrl Pts',(-20.4689199790668,9.78062712373313,
12.));
#238367=CARTESIAN_POINT('Ctrl Pts',(-20.4765353711585,9.78535797314162,
0.));
#238368=CARTESIAN_POINT('Ctrl Pts',(-20.4765353711585,9.78535797314162,
12.));
#238369=CARTESIAN_POINT('Ctrl Pts',(-20.4843302955329,9.7902391649866,0.));
#238370=CARTESIAN_POINT('Ctrl Pts',(-20.4843302955329,9.7902391649866,12.));
#238371=CARTESIAN_POINT('Ctrl Pts',(-20.4923005087945,9.79526974288344,
0.));
#238372=CARTESIAN_POINT('Ctrl Pts',(-20.4923005087945,9.79526974288344,
12.));
#238373=CARTESIAN_POINT('Ctrl Pts',(-20.500441931211,9.80044878520967,0.));
#238374=CARTESIAN_POINT('Ctrl Pts',(-20.500441931211,9.80044878520967,12.));
#238375=CARTESIAN_POINT('Ctrl Pts',(-20.5087506310507,9.80577540161103,
0.));
#238376=CARTESIAN_POINT('Ctrl Pts',(-20.5087506310507,9.80577540161103,
12.));
#238377=CARTESIAN_POINT('Ctrl Pts',(-20.5172228122839,9.81124873025278,
0.));
#238378=CARTESIAN_POINT('Ctrl Pts',(-20.5172228122839,9.81124873025278,
12.));
#238379=CARTESIAN_POINT('Ctrl Pts',(-20.5258548000625,9.81686793455918,
0.));
#238380=CARTESIAN_POINT('Ctrl Pts',(-20.5258548000625,9.81686793455918,
12.));
#238381=CARTESIAN_POINT('Ctrl Pts',(-20.534643029951,9.82263220080328,0.));
#238382=CARTESIAN_POINT('Ctrl Pts',(-20.534643029951,9.82263220080328,12.));
#238383=CARTESIAN_POINT('Ctrl Pts',(-20.5435840460717,9.82854073773857,
0.));
#238384=CARTESIAN_POINT('Ctrl Pts',(-20.5435840460717,9.82854073773857,
12.));
#238385=CARTESIAN_POINT('Ctrl Pts',(-20.5526744976461,9.83459277585321,
0.));
#238386=CARTESIAN_POINT('Ctrl Pts',(-20.5526744976461,9.83459277585321,
12.));
#238387=CARTESIAN_POINT('Ctrl Pts',(-20.5619111362406,9.84078756677589,
0.));
#238388=CARTESIAN_POINT('Ctrl Pts',(-20.5619111362406,9.84078756677589,
12.));
#238389=CARTESIAN_POINT('Ctrl Pts',(-20.5712908125145,9.84712438256308,
0.));
#238390=CARTESIAN_POINT('Ctrl Pts',(-20.5712908125145,9.84712438256308,
12.));
#238391=CARTESIAN_POINT('Ctrl Pts',(-20.580810471002,9.85360251457004,0.));
#238392=CARTESIAN_POINT('Ctrl Pts',(-20.580810471002,9.85360251457004,12.));
#238393=CARTESIAN_POINT('Ctrl Pts',(-20.5904671449754,9.86022127232749,
0.));
#238394=CARTESIAN_POINT('Ctrl Pts',(-20.5904671449754,9.86022127232749,
12.));
#238395=CARTESIAN_POINT('Ctrl Pts',(-20.6002579513696,9.86697998242612,
0.));
#238396=CARTESIAN_POINT('Ctrl Pts',(-20.6002579513696,9.86697998242612,
12.));
#238397=CARTESIAN_POINT('Ctrl Pts',(-20.6101800854491,9.87387798732944,
0.));
#238398=CARTESIAN_POINT('Ctrl Pts',(-20.6101800854491,9.87387798732944,
12.));
#238399=CARTESIAN_POINT('Ctrl Pts',(-20.6202308177472,9.88091464472669,
0.));
#238400=CARTESIAN_POINT('Ctrl Pts',(-20.6202308177472,9.88091464472669,
12.));
#238401=CARTESIAN_POINT('Ctrl Pts',(-20.6304074914086,9.88808932697305,
0.));
#238402=CARTESIAN_POINT('Ctrl Pts',(-20.6304074914086,9.88808932697305,
12.));
#238403=CARTESIAN_POINT('Ctrl Pts',(-20.6407075193977,9.89540142049124,
0.));
#238404=CARTESIAN_POINT('Ctrl Pts',(-20.6407075193977,9.89540142049124,
12.));
#238405=CARTESIAN_POINT('Ctrl Pts',(-20.6511283817415,9.90285032516696,
0.));
#238406=CARTESIAN_POINT('Ctrl Pts',(-20.6511283817415,9.90285032516696,
12.));
#238407=CARTESIAN_POINT('Ctrl Pts',(-20.6616676228315,9.91043545377004,
0.));
#238408=CARTESIAN_POINT('Ctrl Pts',(-20.6616676228315,9.91043545377004,
12.));
#238409=CARTESIAN_POINT('Ctrl Pts',(-20.6723228488262,9.91815623141284,
0.));
#238410=CARTESIAN_POINT('Ctrl Pts',(-20.6723228488262,9.91815623141284,
12.));
#238411=CARTESIAN_POINT('Ctrl Pts',(-20.6830917250255,9.9260120949875,0.));
#238412=CARTESIAN_POINT('Ctrl Pts',(-20.6830917250255,9.9260120949875,12.));
#238413=CARTESIAN_POINT('Ctrl Pts',(-20.6939719732485,9.93400249259736,
0.));
#238414=CARTESIAN_POINT('Ctrl Pts',(-20.6939719732485,9.93400249259736,
12.));
#238415=CARTESIAN_POINT('Ctrl Pts',(-20.7049613692237,9.94212688298251,
0.));
#238416=CARTESIAN_POINT('Ctrl Pts',(-20.7049613692237,9.94212688298251,
12.));
#238417=CARTESIAN_POINT('Ctrl Pts',(-20.716057740758,9.95038473514962,0.));
#238418=CARTESIAN_POINT('Ctrl Pts',(-20.716057740758,9.95038473514962,12.));
#238419=CARTESIAN_POINT('Ctrl Pts',(-20.7272589658752,9.95877552798403,
0.));
#238420=CARTESIAN_POINT('Ctrl Pts',(-20.7272589658752,9.95877552798403,
12.));
#238421=CARTESIAN_POINT('Ctrl Pts',(-20.7385629709795,9.96729874986198,
0.));
#238422=CARTESIAN_POINT('Ctrl Pts',(-20.7385629709795,9.96729874986198,
12.));
#238423=CARTESIAN_POINT('Ctrl Pts',(-20.7499677289625,9.97595389823461,
0.));
#238424=CARTESIAN_POINT('Ctrl Pts',(-20.7499677289625,9.97595389823461,
12.));
#238425=CARTESIAN_POINT('Ctrl Pts',(-20.7614712574989,9.98474047926846,
0.));
#238426=CARTESIAN_POINT('Ctrl Pts',(-20.7614712574989,9.98474047926846,
12.));
#238427=CARTESIAN_POINT('Ctrl Pts',(-20.7730716175417,9.99365800754638,
0.));
#238428=CARTESIAN_POINT('Ctrl Pts',(-20.7730716175417,9.99365800754638,
12.));
#238429=CARTESIAN_POINT('Ctrl Pts',(-20.7847669117568,10.0027060057389,
0.));
#238430=CARTESIAN_POINT('Ctrl Pts',(-20.7847669117568,10.0027060057389,
12.));
#238431=CARTESIAN_POINT('Ctrl Pts',(-20.7965552829907,10.0118840042786,
0.));
#238432=CARTESIAN_POINT('Ctrl Pts',(-20.7965552829907,10.0118840042786,
12.));
#238433=CARTESIAN_POINT('Ctrl Pts',(-20.8084349126885,10.0211915410095,
0.));
#238434=CARTESIAN_POINT('Ctrl Pts',(-20.8084349126885,10.0211915410095,
12.));
#238435=CARTESIAN_POINT('Ctrl Pts',(-20.8204040196599,10.0306281609435,
0.));
#238436=CARTESIAN_POINT('Ctrl Pts',(-20.8204040196599,10.0306281609435,
12.));
#238437=CARTESIAN_POINT('Ctrl Pts',(-20.8324608588906,10.0401934160234,
0.));
#238438=CARTESIAN_POINT('Ctrl Pts',(-20.8324608588906,10.0401934160234,
12.));
#238439=CARTESIAN_POINT('Ctrl Pts',(-20.8446037203402,10.0498868648733,
0.));
#238440=CARTESIAN_POINT('Ctrl Pts',(-20.8446037203402,10.0498868648733,
12.));
#238441=CARTESIAN_POINT('Ctrl Pts',(-20.856830927732,10.0597080725375,0.));
#238442=CARTESIAN_POINT('Ctrl Pts',(-20.856830927732,10.0597080725375,12.));
#238443=CARTESIAN_POINT('Ctrl Pts',(-20.8691408373705,10.0696566102219,
0.));
#238444=CARTESIAN_POINT('Ctrl Pts',(-20.8691408373705,10.0696566102219,
12.));
#238445=CARTESIAN_POINT('Ctrl Pts',(-20.8815318371844,10.0797320551154,
0.));
#238446=CARTESIAN_POINT('Ctrl Pts',(-20.8815318371844,10.0797320551154,
12.));
#238447=CARTESIAN_POINT('Ctrl Pts',(-20.8940023457371,10.0899339901916,
0.));
#238448=CARTESIAN_POINT('Ctrl Pts',(-20.8940023457371,10.0899339901916,
12.));
#238449=CARTESIAN_POINT('Ctrl Pts',(-20.9065508112556,10.1002620040076,
0.));
#238450=CARTESIAN_POINT('Ctrl Pts',(-20.9065508112556,10.1002620040076,
12.));
#238451=CARTESIAN_POINT('Ctrl Pts',(-20.9191757106266,10.1107156904836,
0.));
#238452=CARTESIAN_POINT('Ctrl Pts',(-20.9191757106266,10.1107156904836,
12.));
#238453=CARTESIAN_POINT('Ctrl Pts',(-20.931875548473,10.1212946487057,0.));
#238454=CARTESIAN_POINT('Ctrl Pts',(-20.931875548473,10.1212946487057,12.));
#238455=CARTESIAN_POINT('Ctrl Pts',(-20.944648856393,10.1319984827909,0.));
#238456=CARTESIAN_POINT('Ctrl Pts',(-20.944648856393,10.1319984827909,12.));
#238457=CARTESIAN_POINT('Ctrl Pts',(-20.9574941921591,10.1428268017257,
0.));
#238458=CARTESIAN_POINT('Ctrl Pts',(-20.9574941921591,10.1428268017257,
12.));
#238459=CARTESIAN_POINT('Ctrl Pts',(-20.970410138937,10.1537792192065,0.));
#238460=CARTESIAN_POINT('Ctrl Pts',(-20.970410138937,10.1537792192065,12.));
#238461=CARTESIAN_POINT('Ctrl Pts',(-20.9833953044737,10.1648553534567,
0.));
#238462=CARTESIAN_POINT('Ctrl Pts',(-20.9833953044737,10.1648553534567,
12.));
#238463=CARTESIAN_POINT('Ctrl Pts',(-20.9964483203685,10.1760548270765,
0.));
#238464=CARTESIAN_POINT('Ctrl Pts',(-20.9964483203685,10.1760548270765,
12.));
#238465=CARTESIAN_POINT('Ctrl Pts',(-21.0095678414486,10.1873772669358,
0.));
#238466=CARTESIAN_POINT('Ctrl Pts',(-21.0095678414486,10.1873772669358,
12.));
#238467=CARTESIAN_POINT('Ctrl Pts',(-21.0227525451107,10.1988223040425,
0.));
#238468=CARTESIAN_POINT('Ctrl Pts',(-21.0227525451107,10.1988223040425,
12.));
#238469=CARTESIAN_POINT('Ctrl Pts',(-21.0360011306814,10.2103895734123,
0.));
#238470=CARTESIAN_POINT('Ctrl Pts',(-21.0360011306814,10.2103895734123,
12.));
#238471=CARTESIAN_POINT('Ctrl Pts',(-21.0493123187483,10.2220787139157,
0.));
#238472=CARTESIAN_POINT('Ctrl Pts',(-21.0493123187483,10.2220787139157,
12.));
#238473=CARTESIAN_POINT('Ctrl Pts',(-21.0626848505665,10.233889368157,0.));
#238474=CARTESIAN_POINT('Ctrl Pts',(-21.0626848505665,10.233889368157,12.));
#238475=CARTESIAN_POINT('Ctrl Pts',(-21.0761174875448,10.2458211823915,
0.));
#238476=CARTESIAN_POINT('Ctrl Pts',(-21.0761174875448,10.2458211823915,
12.));
#238477=CARTESIAN_POINT('Ctrl Pts',(-21.0896090107066,10.2578738064183,
0.));
#238478=CARTESIAN_POINT('Ctrl Pts',(-21.0896090107066,10.2578738064183,
12.));
#238479=CARTESIAN_POINT('Ctrl Pts',(-21.1031582201625,10.2700468934743,
0.));
#238480=CARTESIAN_POINT('Ctrl Pts',(-21.1031582201625,10.2700468934743,
12.));
#238481=CARTESIAN_POINT('Ctrl Pts',(-21.1167639345623,10.2823401001067,
0.));
#238482=CARTESIAN_POINT('Ctrl Pts',(-21.1167639345623,10.2823401001067,
12.));
#238483=CARTESIAN_POINT('Ctrl Pts',(-21.130424990599,10.2947530860714,0.));
#238484=CARTESIAN_POINT('Ctrl Pts',(-21.130424990599,10.2947530860714,12.));
#238485=CARTESIAN_POINT('Ctrl Pts',(-21.1441402425831,10.307285514268,0.));
#238486=CARTESIAN_POINT('Ctrl Pts',(-21.1441402425831,10.307285514268,12.));
#238487=CARTESIAN_POINT('Ctrl Pts',(-21.1579085619959,10.3199370506541,
0.));
#238488=CARTESIAN_POINT('Ctrl Pts',(-21.1579085619959,10.3199370506541,
12.));
#238489=CARTESIAN_POINT('Ctrl Pts',(-21.1717288370512,10.3327073641574,
0.));
#238490=CARTESIAN_POINT('Ctrl Pts',(-21.1717288370512,10.3327073641574,
12.));
#238491=CARTESIAN_POINT('Ctrl Pts',(-21.1855999722427,10.3455961265706,
0.));
#238492=CARTESIAN_POINT('Ctrl Pts',(-21.1855999722427,10.3455961265706,
12.));
#238493=CARTESIAN_POINT('Ctrl Pts',(-21.1995208879205,10.3586030124595,
0.));
#238494=CARTESIAN_POINT('Ctrl Pts',(-21.1995208879205,10.3586030124595,
12.));
#238495=CARTESIAN_POINT('Ctrl Pts',(-21.2134905199359,10.3717276991137,
0.));
#238496=CARTESIAN_POINT('Ctrl Pts',(-21.2134905199359,10.3717276991137,
12.));
#238497=CARTESIAN_POINT('Ctrl Pts',(-21.2275078192708,10.384969866479,0.));
#238498=CARTESIAN_POINT('Ctrl Pts',(-21.2275078192708,10.384969866479,12.));
#238499=CARTESIAN_POINT('Ctrl Pts',(-21.2415717516713,10.3983291970846,
0.));
#238500=CARTESIAN_POINT('Ctrl Pts',(-21.2415717516713,10.3983291970846,
12.));
#238501=CARTESIAN_POINT('Ctrl Pts',(-21.2556812972741,10.4118053759584,
0.));
#238502=CARTESIAN_POINT('Ctrl Pts',(-21.2556812972741,10.4118053759584,
12.));
#238503=CARTESIAN_POINT('Ctrl Pts',(-21.2698354502391,10.4253980905394,
0.));
#238504=CARTESIAN_POINT('Ctrl Pts',(-21.2698354502391,10.4253980905394,
12.));
#238505=CARTESIAN_POINT('Ctrl Pts',(-21.2840332184471,10.4391070306385,
0.));
#238506=CARTESIAN_POINT('Ctrl Pts',(-21.2840332184471,10.4391070306385,
12.));
#238507=CARTESIAN_POINT('Ctrl Pts',(-21.2982736231924,10.452931888387,0.));
#238508=CARTESIAN_POINT('Ctrl Pts',(-21.2982736231924,10.452931888387,12.));
#238509=CARTESIAN_POINT('Ctrl Pts',(-21.312555698873,10.4668723581768,0.));
#238510=CARTESIAN_POINT('Ctrl Pts',(-21.312555698873,10.4668723581768,12.));
#238511=CARTESIAN_POINT('Ctrl Pts',(-21.3268784926823,10.4809281365933,
0.));
#238512=CARTESIAN_POINT('Ctrl Pts',(-21.3268784926823,10.4809281365933,
12.));
#238513=CARTESIAN_POINT('Ctrl Pts',(-21.3412410642912,10.4950989223341,
0.));
#238514=CARTESIAN_POINT('Ctrl Pts',(-21.3412410642912,10.4950989223341,
12.));
#238515=CARTESIAN_POINT('Ctrl Pts',(-21.3556424855822,10.5093844161689,
0.));
#238516=CARTESIAN_POINT('Ctrl Pts',(-21.3556424855822,10.5093844161689,
12.));
#238517=CARTESIAN_POINT('Ctrl Pts',(-21.3700818403942,10.523784320906,0.));
#238518=CARTESIAN_POINT('Ctrl Pts',(-21.3700818403942,10.523784320906,12.));
#238519=CARTESIAN_POINT('Ctrl Pts',(-21.3845582242604,10.5382983413422,
0.));
#238520=CARTESIAN_POINT('Ctrl Pts',(-21.3845582242604,10.5382983413422,
12.));
#238521=CARTESIAN_POINT('Ctrl Pts',(-21.3990707441495,10.5529261842107,
0.));
#238522=CARTESIAN_POINT('Ctrl Pts',(-21.3990707441495,10.5529261842107,
12.));
#238523=CARTESIAN_POINT('Ctrl Pts',(-21.4136185181974,10.5676675581106,
0.));
#238524=CARTESIAN_POINT('Ctrl Pts',(-21.4136185181974,10.5676675581106,
12.));
#238525=CARTESIAN_POINT('Ctrl Pts',(-21.4282006754624,10.582522173457,0.));
#238526=CARTESIAN_POINT('Ctrl Pts',(-21.4282006754624,10.582522173457,12.));
#238527=CARTESIAN_POINT('Ctrl Pts',(-21.4428163557137,10.597489742462,0.));
#238528=CARTESIAN_POINT('Ctrl Pts',(-21.4428163557137,10.597489742462,12.));
#238529=CARTESIAN_POINT('Ctrl Pts',(-21.4574647092093,10.612569979096,0.));
#238530=CARTESIAN_POINT('Ctrl Pts',(-21.4574647092093,10.612569979096,12.));
#238531=CARTESIAN_POINT('Ctrl Pts',(-21.4721448964766,10.6277625990457,
0.));
#238532=CARTESIAN_POINT('Ctrl Pts',(-21.4721448964766,10.6277625990457,
12.));
#238533=CARTESIAN_POINT('Ctrl Pts',(-21.4868560880893,10.6430673196609,
0.));
#238534=CARTESIAN_POINT('Ctrl Pts',(-21.4868560880893,10.6430673196609,
12.));
#238535=CARTESIAN_POINT('Ctrl Pts',(-21.5015974644454,10.658483859894,0.));
#238536=CARTESIAN_POINT('Ctrl Pts',(-21.5015974644454,10.658483859894,12.));
#238537=CARTESIAN_POINT('Ctrl Pts',(-21.5163682155805,10.6740119402835,
0.));
#238538=CARTESIAN_POINT('Ctrl Pts',(-21.5163682155805,10.6740119402835,
12.));
#238539=CARTESIAN_POINT('Ctrl Pts',(-21.531167540981,10.689651282929,0.));
#238540=CARTESIAN_POINT('Ctrl Pts',(-21.531167540981,10.689651282929,12.));
#238541=CARTESIAN_POINT('Ctrl Pts',(-21.5459946493955,10.7054016114571,
0.));
#238542=CARTESIAN_POINT('Ctrl Pts',(-21.5459946493955,10.7054016114571,
12.));
#238543=CARTESIAN_POINT('Ctrl Pts',(-21.5608487586467,10.7212626509816,
0.));
#238544=CARTESIAN_POINT('Ctrl Pts',(-21.5608487586467,10.7212626509816,
12.));
#238545=CARTESIAN_POINT('Ctrl Pts',(-21.5757290954372,10.7372341280468,
0.));
#238546=CARTESIAN_POINT('Ctrl Pts',(-21.5757290954372,10.7372341280468,
12.));
#238547=CARTESIAN_POINT('Ctrl Pts',(-21.5906348951745,10.7533157705943,
0.));
#238548=CARTESIAN_POINT('Ctrl Pts',(-21.5906348951745,10.7533157705943,
12.));
#238549=CARTESIAN_POINT('Ctrl Pts',(-21.6055654018179,10.7695073079554,
0.));
#238550=CARTESIAN_POINT('Ctrl Pts',(-21.6055654018179,10.7695073079554,
12.));
#238551=CARTESIAN_POINT('Ctrl Pts',(-21.6205198677176,10.7858084708262,
0.));
#238552=CARTESIAN_POINT('Ctrl Pts',(-21.6205198677176,10.7858084708262,
12.));
#238553=CARTESIAN_POINT('Ctrl Pts',(-21.6354975534557,10.8022189912369,
0.));
#238554=CARTESIAN_POINT('Ctrl Pts',(-21.6354975534557,10.8022189912369,
12.));
#238555=CARTESIAN_POINT('Ctrl Pts',(-21.6504977276864,10.8187386025135,
0.));
#238556=CARTESIAN_POINT('Ctrl Pts',(-21.6504977276864,10.8187386025135,
12.));
#238557=CARTESIAN_POINT('Ctrl Pts',(-21.6655196669727,10.835367039227,0.));
#238558=CARTESIAN_POINT('Ctrl Pts',(-21.6655196669727,10.835367039227,12.));
#238559=CARTESIAN_POINT('Ctrl Pts',(-21.6805626556461,10.8521040371832,
0.));
#238560=CARTESIAN_POINT('Ctrl Pts',(-21.6805626556461,10.8521040371832,
12.));
#238561=CARTESIAN_POINT('Ctrl Pts',(-21.6956259856667,10.8689493334093,
0.));
#238562=CARTESIAN_POINT('Ctrl Pts',(-21.6956259856667,10.8689493334093,
12.));
#238563=CARTESIAN_POINT('Ctrl Pts',(-21.7107089564822,10.8859026661292,
0.));
#238564=CARTESIAN_POINT('Ctrl Pts',(-21.7107089564822,10.8859026661292,
12.));
#238565=CARTESIAN_POINT('Ctrl Pts',(-21.7258108748874,10.9029637747341,
0.));
#238566=CARTESIAN_POINT('Ctrl Pts',(-21.7258108748874,10.9029637747341,
12.));
#238567=CARTESIAN_POINT('Ctrl Pts',(-21.74093105488,10.9201323997386,0.));
#238568=CARTESIAN_POINT('Ctrl Pts',(-21.74093105488,10.9201323997386,12.));
#238569=CARTESIAN_POINT('Ctrl Pts',(-21.7560688175252,10.9374082827446,
0.));
#238570=CARTESIAN_POINT('Ctrl Pts',(-21.7560688175252,10.9374082827446,
12.));
#238571=CARTESIAN_POINT('Ctrl Pts',(-21.7712234908468,10.9547911664457,
0.));
#238572=CARTESIAN_POINT('Ctrl Pts',(-21.7712234908468,10.9547911664457,
12.));
#238573=CARTESIAN_POINT('Ctrl Pts',(-21.7863944097143,10.9722807946157,
0.));
#238574=CARTESIAN_POINT('Ctrl Pts',(-21.7863944097143,10.9722807946157,
12.));
#238575=CARTESIAN_POINT('Ctrl Pts',(-21.8015809157302,10.9898769120913,
0.));
#238576=CARTESIAN_POINT('Ctrl Pts',(-21.8015809157302,10.9898769120913,
12.));
#238577=CARTESIAN_POINT('Ctrl Pts',(-21.8167823571168,11.0075792647477,
0.));
#238578=CARTESIAN_POINT('Ctrl Pts',(-21.8167823571168,11.0075792647477,
12.));
#238579=CARTESIAN_POINT('Ctrl Pts',(-21.8319980886033,11.0253875994598,
0.));
#238580=CARTESIAN_POINT('Ctrl Pts',(-21.8319980886033,11.0253875994598,
12.));
#238581=CARTESIAN_POINT('Ctrl Pts',(-21.8472274713103,11.0433016640808,
0.));
#238582=CARTESIAN_POINT('Ctrl Pts',(-21.8472274713103,11.0433016640808,
12.));
#238583=CARTESIAN_POINT('Ctrl Pts',(-21.8624698726319,11.0613212074364,
0.));
#238584=CARTESIAN_POINT('Ctrl Pts',(-21.8624698726319,11.0613212074364,
12.));
#238585=CARTESIAN_POINT('Ctrl Pts',(-21.8777246661191,11.0794459793058,
0.));
#238586=CARTESIAN_POINT('Ctrl Pts',(-21.8777246661191,11.0794459793058,
12.));
#238587=CARTESIAN_POINT('Ctrl Pts',(-21.8929912313608,11.0976757303944,
0.));
#238588=CARTESIAN_POINT('Ctrl Pts',(-21.8929912313608,11.0976757303944,
12.));
#238589=CARTESIAN_POINT('Ctrl Pts',(-21.9082689538687,11.1160102123024,
0.));
#238590=CARTESIAN_POINT('Ctrl Pts',(-21.9082689538687,11.1160102123024,
12.));
#238591=CARTESIAN_POINT('Ctrl Pts',(-21.9235572249518,11.134449177474,0.));
#238592=CARTESIAN_POINT('Ctrl Pts',(-21.9235572249518,11.134449177474,12.));
#238593=CARTESIAN_POINT('Ctrl Pts',(-21.9388554416437,11.1529923792002,
0.));
#238594=CARTESIAN_POINT('Ctrl Pts',(-21.9388554416437,11.1529923792002,
12.));
#238595=CARTESIAN_POINT('Ctrl Pts',(-21.9541630066504,11.1716395716375,
0.));
#238596=CARTESIAN_POINT('Ctrl Pts',(-21.9541630066504,11.1716395716375,
12.));
#238597=CARTESIAN_POINT('Ctrl Pts',(-21.9694793282913,11.1903905098109,
0.));
#238598=CARTESIAN_POINT('Ctrl Pts',(-21.9694793282913,11.1903905098109,
12.));
#238599=CARTESIAN_POINT('Ctrl Pts',(-21.9848038204439,11.2092449496125,
0.));
#238600=CARTESIAN_POINT('Ctrl Pts',(-21.9848038204439,11.2092449496125,
12.));
#238601=CARTESIAN_POINT('Ctrl Pts',(-22.0001359024839,11.2282026477897,
0.));
#238602=CARTESIAN_POINT('Ctrl Pts',(-22.0001359024839,11.2282026477897,
12.));
#238603=CARTESIAN_POINT('Ctrl Pts',(-22.0154749992364,11.2472633619276,
0.));
#238604=CARTESIAN_POINT('Ctrl Pts',(-22.0154749992364,11.2472633619276,
12.));
#238605=CARTESIAN_POINT('Ctrl Pts',(-22.0308205408351,11.2664268504207,
0.));
#238606=CARTESIAN_POINT('Ctrl Pts',(-22.0308205408351,11.2664268504207,
12.));
#238607=CARTESIAN_POINT('Ctrl Pts',(-22.046171962566,11.2856928724374,0.));
#238608=CARTESIAN_POINT('Ctrl Pts',(-22.046171962566,11.2856928724374,12.));
#238609=CARTESIAN_POINT('Ctrl Pts',(-22.0615287047179,11.3050611878771,
0.));
#238610=CARTESIAN_POINT('Ctrl Pts',(-22.0615287047179,11.3050611878771,
12.));
#238611=CARTESIAN_POINT('Ctrl Pts',(-22.0768902124267,11.3245315573168,
0.));
#238612=CARTESIAN_POINT('Ctrl Pts',(-22.0768902124267,11.3245315573168,
12.));
#238613=CARTESIAN_POINT('Ctrl Pts',(-22.0922559355293,11.3441037419553,
0.));
#238614=CARTESIAN_POINT('Ctrl Pts',(-22.0922559355293,11.3441037419553,
12.));
#238615=CARTESIAN_POINT('Ctrl Pts',(-22.1076253283978,11.3637775035367,
0.));
#238616=CARTESIAN_POINT('Ctrl Pts',(-22.1076253283978,11.3637775035367,
12.));
#238617=CARTESIAN_POINT('Ctrl Pts',(-22.1229978500185,11.3835526044256,
0.));
#238618=CARTESIAN_POINT('Ctrl Pts',(-22.1229978500185,11.3835526044256,
12.));
#238619=CARTESIAN_POINT('Ctrl Pts',(-22.1383729640963,11.4034288076908,
0.));
#238620=CARTESIAN_POINT('Ctrl Pts',(-22.1383729640963,11.4034288076908,
12.));
#238621=CARTESIAN_POINT('Ctrl Pts',(-22.1537501391486,11.4234058771742,
0.));
#238622=CARTESIAN_POINT('Ctrl Pts',(-22.1537501391486,11.4234058771742,
12.));
#238623=CARTESIAN_POINT('Ctrl Pts',(-22.1691288486096,11.443483577557,0.));
#238624=CARTESIAN_POINT('Ctrl Pts',(-22.1691288486096,11.443483577557,12.));
#238625=CARTESIAN_POINT('Ctrl Pts',(-22.184508570917,11.463661674411,0.));
#238626=CARTESIAN_POINT('Ctrl Pts',(-22.184508570917,11.463661674411,12.));
#238627=CARTESIAN_POINT('Ctrl Pts',(-22.1998887896435,11.4839399342589,
0.));
#238628=CARTESIAN_POINT('Ctrl Pts',(-22.1998887896435,11.4839399342589,
12.));
#238629=CARTESIAN_POINT('Ctrl Pts',(-22.215268993102,11.504318124424,0.));
#238630=CARTESIAN_POINT('Ctrl Pts',(-22.215268993102,11.504318124424,12.));
#238631=CARTESIAN_POINT('Ctrl Pts',(-22.2306486738899,11.5247960128476,
0.));
#238632=CARTESIAN_POINT('Ctrl Pts',(-22.2306486738899,11.5247960128476,
12.));
#238633=CARTESIAN_POINT('Ctrl Pts',(-22.2460273284653,11.545373367912,0.));
#238634=CARTESIAN_POINT('Ctrl Pts',(-22.2460273284653,11.545373367912,12.));
#238635=CARTESIAN_POINT('Ctrl Pts',(-22.2614044566898,11.5660499582403,
0.));
#238636=CARTESIAN_POINT('Ctrl Pts',(-22.2614044566898,11.5660499582403,
12.));
#238637=CARTESIAN_POINT('Ctrl Pts',(-22.2767795614349,11.5868255525189,
0.));
#238638=CARTESIAN_POINT('Ctrl Pts',(-22.2767795614349,11.5868255525189,
12.));
#238639=CARTESIAN_POINT('Ctrl Pts',(-22.2921521480358,11.6076999192359,
0.));
#238640=CARTESIAN_POINT('Ctrl Pts',(-22.2921521480358,11.6076999192359,
12.));
#238641=CARTESIAN_POINT('Ctrl Pts',(-22.3075217249049,11.6286728270011,
0.));
#238642=CARTESIAN_POINT('Ctrl Pts',(-22.3075217249049,11.6286728270011,
12.));
#238643=CARTESIAN_POINT('Ctrl Pts',(-22.3228878043976,11.6497440449858,
0.));
#238644=CARTESIAN_POINT('Ctrl Pts',(-22.3228878043976,11.6497440449858,
12.));
#238645=CARTESIAN_POINT('Ctrl Pts',(-22.3382499035618,11.6709133432986,
0.));
#238646=CARTESIAN_POINT('Ctrl Pts',(-22.3382499035618,11.6709133432986,
12.));
#238647=CARTESIAN_POINT('Ctrl Pts',(-22.3536075450028,11.6921804934056,
0.));
#238648=CARTESIAN_POINT('Ctrl Pts',(-22.3536075450028,11.6921804934056,
12.));
#238649=CARTESIAN_POINT('Ctrl Pts',(-22.3689602575492,11.7135452684532,
0.));
#238650=CARTESIAN_POINT('Ctrl Pts',(-22.3689602575492,11.7135452684532,
12.));
#238651=CARTESIAN_POINT('Ctrl Pts',(-22.3843075773905,11.7350074437961,
0.));
#238652=CARTESIAN_POINT('Ctrl Pts',(-22.3843075773905,11.7350074437961,
12.));
#238653=CARTESIAN_POINT('Ctrl Pts',(-22.39964904692,11.7565667964765,0.));
#238654=CARTESIAN_POINT('Ctrl Pts',(-22.39964904692,11.7565667964765,12.));
#238655=CARTESIAN_POINT('Ctrl Pts',(-22.4149842125018,11.7782231042041,
0.));
#238656=CARTESIAN_POINT('Ctrl Pts',(-22.4149842125018,11.7782231042041,
12.));
#238657=CARTESIAN_POINT('Ctrl Pts',(-22.4303126226468,11.7999761445175,
0.));
#238658=CARTESIAN_POINT('Ctrl Pts',(-22.4303126226468,11.7999761445175,
12.));
#238659=CARTESIAN_POINT('Ctrl Pts',(-22.4456338258738,11.8218256937889,
0.));
#238660=CARTESIAN_POINT('Ctrl Pts',(-22.4456338258738,11.8218256937889,
12.));
#238661=CARTESIAN_POINT('Ctrl Pts',(-22.4609473690469,11.8437715264487,
0.));
#238662=CARTESIAN_POINT('Ctrl Pts',(-22.4609473690469,11.8437715264487,
12.));
#238663=CARTESIAN_POINT('Ctrl Pts',(-22.4762527946694,11.8658134137018,
0.));
#238664=CARTESIAN_POINT('Ctrl Pts',(-22.4762527946694,11.8658134137018,
12.));
#238665=CARTESIAN_POINT('Ctrl Pts',(-22.4915496418472,11.8879511239941,
0.));
#238666=CARTESIAN_POINT('Ctrl Pts',(-22.4915496418472,11.8879511239941,
12.));
#238667=CARTESIAN_POINT('Ctrl Pts',(-22.5068374513958,11.9101844254555,
0.));
#238668=CARTESIAN_POINT('Ctrl Pts',(-22.5068374513958,11.9101844254555,
12.));
#238669=CARTESIAN_POINT('Ctrl Pts',(-22.5221157697869,11.9325130877801,
0.));
#238670=CARTESIAN_POINT('Ctrl Pts',(-22.5221157697869,11.9325130877801,
12.));
#238671=CARTESIAN_POINT('Ctrl Pts',(-22.5373841537299,11.9549368843996,
0.));
#238672=CARTESIAN_POINT('Ctrl Pts',(-22.5373841537299,11.9549368843996,
12.));
#238673=CARTESIAN_POINT('Ctrl Pts',(-22.5526421741159,11.9774555943496,
0.));
#238674=CARTESIAN_POINT('Ctrl Pts',(-22.5526421741159,11.9774555943496,
12.));
#238675=CARTESIAN_POINT('Ctrl Pts',(-22.5678894211194,12.0000690046697,
0.));
#238676=CARTESIAN_POINT('Ctrl Pts',(-22.5678894211194,12.0000690046697,
12.));
#238677=CARTESIAN_POINT('Ctrl Pts',(-22.5831255061306,12.0227769113132,
0.));
#238678=CARTESIAN_POINT('Ctrl Pts',(-22.5831255061306,12.0227769113132,
12.));
#238679=CARTESIAN_POINT('Ctrl Pts',(-22.5983500505675,12.0455791139135,
0.));
#238680=CARTESIAN_POINT('Ctrl Pts',(-22.5983500505675,12.0455791139135,
12.));
#238681=CARTESIAN_POINT('Ctrl Pts',(-22.613562676493,12.0684754113869,0.));
#238682=CARTESIAN_POINT('Ctrl Pts',(-22.613562676493,12.0684754113869,12.));
#238683=CARTESIAN_POINT('Ctrl Pts',(-22.628762996708,12.0914655972828,0.));
#238684=CARTESIAN_POINT('Ctrl Pts',(-22.628762996708,12.0914655972828,12.));
#238685=CARTESIAN_POINT('Ctrl Pts',(-22.6439506046611,12.1145494550384,
0.));
#238686=CARTESIAN_POINT('Ctrl Pts',(-22.6439506046611,12.1145494550384,
12.));
#238687=CARTESIAN_POINT('Ctrl Pts',(-22.6591250653942,12.1377267537141,
0.));
#238688=CARTESIAN_POINT('Ctrl Pts',(-22.6591250653942,12.1377267537141,
12.));
#238689=CARTESIAN_POINT('Ctrl Pts',(-22.6742859034891,12.1609972423088,
0.));
#238690=CARTESIAN_POINT('Ctrl Pts',(-22.6742859034891,12.1609972423088,
12.));
#238691=CARTESIAN_POINT('Ctrl Pts',(-22.6894326204959,12.1843606579246,
0.));
#238692=CARTESIAN_POINT('Ctrl Pts',(-22.6894326204959,12.1843606579246,
12.));
#238693=CARTESIAN_POINT('Ctrl Pts',(-22.7045647168659,12.2078167360267,
0.));
#238694=CARTESIAN_POINT('Ctrl Pts',(-22.7045647168659,12.2078167360267,
12.));
#238695=CARTESIAN_POINT('Ctrl Pts',(-22.7196817119299,12.2313652198047,
0.));
#238696=CARTESIAN_POINT('Ctrl Pts',(-22.7196817119299,12.2313652198047,
12.));
#238697=CARTESIAN_POINT('Ctrl Pts',(-22.7347831655251,12.2550058702389,
0.));
#238698=CARTESIAN_POINT('Ctrl Pts',(-22.7347831655251,12.2550058702389,
12.));
#238699=CARTESIAN_POINT('Ctrl Pts',(-22.7498686970096,12.2787384750747,
0.));
#238700=CARTESIAN_POINT('Ctrl Pts',(-22.7498686970096,12.2787384750747,
12.));
#238701=CARTESIAN_POINT('Ctrl Pts',(-22.7649380101154,12.3025628601812,
0.));
#238702=CARTESIAN_POINT('Ctrl Pts',(-22.7649380101154,12.3025628601812,
12.));
#238703=CARTESIAN_POINT('Ctrl Pts',(-22.7799908974947,12.3264788926108,
0.));
#238704=CARTESIAN_POINT('Ctrl Pts',(-22.7799908974947,12.3264788926108,
12.));
#238705=CARTESIAN_POINT('Ctrl Pts',(-22.7950272216959,12.3504864740361,
0.));
#238706=CARTESIAN_POINT('Ctrl Pts',(-22.7950272216959,12.3504864740361,
12.));
#238707=CARTESIAN_POINT('Ctrl Pts',(-22.8100469022632,12.3745855366772,
0.));
#238708=CARTESIAN_POINT('Ctrl Pts',(-22.8100469022632,12.3745855366772,
12.));
#238709=CARTESIAN_POINT('Ctrl Pts',(-22.8220493007353,12.393937937903,0.));
#238710=CARTESIAN_POINT('Ctrl Pts',(-22.8220493007353,12.393937937903,12.));
#238711=CARTESIAN_POINT('Ctrl Pts',(-22.8310435872852,12.4084933766366,
0.));
#238712=CARTESIAN_POINT('Ctrl Pts',(-22.8310435872852,12.4084933766366,
12.));
#238713=CARTESIAN_POINT('Ctrl Pts',(-22.8370364396497,12.4182152851867,
0.));
#238714=CARTESIAN_POINT('Ctrl Pts',(-22.8370364396497,12.4182152851867,
12.));
#238715=CARTESIAN_POINT('Ctrl Pts',(-22.8400320311648,12.4230808101438,
0.));
#238716=CARTESIAN_POINT('Ctrl Pts',(-22.8400320311648,12.4230808101438,
12.));
#238717=CARTESIAN_POINT('',(-22.8400320311648,12.4230808101438,0.));
#238718=CARTESIAN_POINT('Ctrl Pts',(-20.353053841303,9.71462809124917,0.));
#238719=CARTESIAN_POINT('Ctrl Pts',(-20.353060251684,9.71462954053074,0.));
#238720=CARTESIAN_POINT('Ctrl Pts',(-20.3531126095522,9.71465227853122,
0.));
#238721=CARTESIAN_POINT('Ctrl Pts',(-20.3533097561886,9.71474590350791,
0.));
#238722=CARTESIAN_POINT('Ctrl Pts',(-20.3538098605706,9.71498978052101,
0.));
#238723=CARTESIAN_POINT('Ctrl Pts',(-20.3548282742361,9.71549257088175,
0.));
#238724=CARTESIAN_POINT('Ctrl Pts',(-20.3562337557875,9.71619192554147,
0.));
#238725=CARTESIAN_POINT('Ctrl Pts',(-20.3580133103357,9.71708493723061,
0.));
#238726=CARTESIAN_POINT('Ctrl Pts',(-20.3601498764344,9.71816778327999,
0.));
#238727=CARTESIAN_POINT('Ctrl Pts',(-20.362625691398,9.71943648548114,0.));
#238728=CARTESIAN_POINT('Ctrl Pts',(-20.3654261611055,9.72088778381102,
0.));
#238729=CARTESIAN_POINT('Ctrl Pts',(-20.3685406190576,9.72251930722504,
0.));
#238730=CARTESIAN_POINT('Ctrl Pts',(-20.371960235676,9.72432910043193,0.));
#238731=CARTESIAN_POINT('Ctrl Pts',(-20.3756766651952,9.72631531732871,
0.));
#238732=CARTESIAN_POINT('Ctrl Pts',(-20.3796805893304,9.72847589116533,
0.));
#238733=CARTESIAN_POINT('Ctrl Pts',(-20.3839624556742,9.73080870123726,
0.));
#238734=CARTESIAN_POINT('Ctrl Pts',(-20.3885129129912,9.73331167102812,
0.));
#238735=CARTESIAN_POINT('Ctrl Pts',(-20.3933234845646,9.7359829201425,0.));
#238736=CARTESIAN_POINT('Ctrl Pts',(-20.3983866213331,9.73882077613206,
0.));
#238737=CARTESIAN_POINT('Ctrl Pts',(-20.4036953576549,9.74182369656272,
0.));
#238738=CARTESIAN_POINT('Ctrl Pts',(-20.4092430879861,9.74499021838536,
0.));
#238739=CARTESIAN_POINT('Ctrl Pts',(-20.4150232777393,9.74831889242175,
0.));
#238740=CARTESIAN_POINT('Ctrl Pts',(-20.4210295275818,9.75180829786433,
0.));
#238741=CARTESIAN_POINT('Ctrl Pts',(-20.4272556476629,9.75545705902416,
0.));
#238742=CARTESIAN_POINT('Ctrl Pts',(-20.4336957355474,9.7592638628993,0.));
#238743=CARTESIAN_POINT('Ctrl Pts',(-20.4403442329401,9.76322747195502,
0.));
#238744=CARTESIAN_POINT('Ctrl Pts',(-20.447195862298,9.76734670980897,0.));
#238745=CARTESIAN_POINT('Ctrl Pts',(-20.4542455817527,9.7716204510407,0.));
#238746=CARTESIAN_POINT('Ctrl Pts',(-20.4614885274973,9.77604760815523,
0.));
#238747=CARTESIAN_POINT('Ctrl Pts',(-20.4689199790668,9.78062712373313,
0.));
#238748=CARTESIAN_POINT('Ctrl Pts',(-20.4765353711585,9.78535797314162,
0.));
#238749=CARTESIAN_POINT('Ctrl Pts',(-20.4843302955329,9.7902391649866,0.));
#238750=CARTESIAN_POINT('Ctrl Pts',(-20.4923005087945,9.79526974288344,
0.));
#238751=CARTESIAN_POINT('Ctrl Pts',(-20.500441931211,9.80044878520967,0.));
#238752=CARTESIAN_POINT('Ctrl Pts',(-20.5087506310507,9.80577540161103,
0.));
#238753=CARTESIAN_POINT('Ctrl Pts',(-20.5172228122839,9.81124873025278,
0.));
#238754=CARTESIAN_POINT('Ctrl Pts',(-20.5258548000625,9.81686793455918,
0.));
#238755=CARTESIAN_POINT('Ctrl Pts',(-20.534643029951,9.82263220080328,0.));
#238756=CARTESIAN_POINT('Ctrl Pts',(-20.5435840460717,9.82854073773857,
0.));
#238757=CARTESIAN_POINT('Ctrl Pts',(-20.5526744976461,9.83459277585321,
0.));
#238758=CARTESIAN_POINT('Ctrl Pts',(-20.5619111362406,9.84078756677589,
0.));
#238759=CARTESIAN_POINT('Ctrl Pts',(-20.5712908125145,9.84712438256308,
0.));
#238760=CARTESIAN_POINT('Ctrl Pts',(-20.580810471002,9.85360251457004,0.));
#238761=CARTESIAN_POINT('Ctrl Pts',(-20.5904671449754,9.86022127232749,
0.));
#238762=CARTESIAN_POINT('Ctrl Pts',(-20.6002579513696,9.86697998242612,
0.));
#238763=CARTESIAN_POINT('Ctrl Pts',(-20.6101800854491,9.87387798732944,
0.));
#238764=CARTESIAN_POINT('Ctrl Pts',(-20.6202308177472,9.88091464472669,
0.));
#238765=CARTESIAN_POINT('Ctrl Pts',(-20.6304074914086,9.88808932697305,
0.));
#238766=CARTESIAN_POINT('Ctrl Pts',(-20.6407075193977,9.89540142049124,
0.));
#238767=CARTESIAN_POINT('Ctrl Pts',(-20.6511283817415,9.90285032516696,
0.));
#238768=CARTESIAN_POINT('Ctrl Pts',(-20.6616676228315,9.91043545377004,
0.));
#238769=CARTESIAN_POINT('Ctrl Pts',(-20.6723228488262,9.91815623141284,
0.));
#238770=CARTESIAN_POINT('Ctrl Pts',(-20.6830917250255,9.9260120949875,0.));
#238771=CARTESIAN_POINT('Ctrl Pts',(-20.6939719732485,9.93400249259736,
0.));
#238772=CARTESIAN_POINT('Ctrl Pts',(-20.7049613692237,9.94212688298251,
0.));
#238773=CARTESIAN_POINT('Ctrl Pts',(-20.716057740758,9.95038473514962,0.));
#238774=CARTESIAN_POINT('Ctrl Pts',(-20.7272589658752,9.95877552798403,
0.));
#238775=CARTESIAN_POINT('Ctrl Pts',(-20.7385629709795,9.96729874986198,
0.));
#238776=CARTESIAN_POINT('Ctrl Pts',(-20.7499677289625,9.97595389823461,
0.));
#238777=CARTESIAN_POINT('Ctrl Pts',(-20.7614712574989,9.98474047926846,
0.));
#238778=CARTESIAN_POINT('Ctrl Pts',(-20.7730716175417,9.99365800754638,
0.));
#238779=CARTESIAN_POINT('Ctrl Pts',(-20.7847669117568,10.0027060057389,
0.));
#238780=CARTESIAN_POINT('Ctrl Pts',(-20.7965552829907,10.0118840042786,
0.));
#238781=CARTESIAN_POINT('Ctrl Pts',(-20.8084349126885,10.0211915410095,
0.));
#238782=CARTESIAN_POINT('Ctrl Pts',(-20.8204040196599,10.0306281609435,
0.));
#238783=CARTESIAN_POINT('Ctrl Pts',(-20.8324608588906,10.0401934160234,
0.));
#238784=CARTESIAN_POINT('Ctrl Pts',(-20.8446037203402,10.0498868648733,
0.));
#238785=CARTESIAN_POINT('Ctrl Pts',(-20.856830927732,10.0597080725375,0.));
#238786=CARTESIAN_POINT('Ctrl Pts',(-20.8691408373705,10.0696566102219,
0.));
#238787=CARTESIAN_POINT('Ctrl Pts',(-20.8815318371844,10.0797320551154,
0.));
#238788=CARTESIAN_POINT('Ctrl Pts',(-20.8940023457371,10.0899339901916,
0.));
#238789=CARTESIAN_POINT('Ctrl Pts',(-20.9065508112556,10.1002620040076,
0.));
#238790=CARTESIAN_POINT('Ctrl Pts',(-20.9191757106266,10.1107156904836,
0.));
#238791=CARTESIAN_POINT('Ctrl Pts',(-20.931875548473,10.1212946487057,0.));
#238792=CARTESIAN_POINT('Ctrl Pts',(-20.944648856393,10.1319984827909,0.));
#238793=CARTESIAN_POINT('Ctrl Pts',(-20.9574941921591,10.1428268017257,
0.));
#238794=CARTESIAN_POINT('Ctrl Pts',(-20.970410138937,10.1537792192065,0.));
#238795=CARTESIAN_POINT('Ctrl Pts',(-20.9833953044737,10.1648553534567,
0.));
#238796=CARTESIAN_POINT('Ctrl Pts',(-20.9964483203685,10.1760548270765,
0.));
#238797=CARTESIAN_POINT('Ctrl Pts',(-21.0095678414486,10.1873772669358,
0.));
#238798=CARTESIAN_POINT('Ctrl Pts',(-21.0227525451107,10.1988223040425,
0.));
#238799=CARTESIAN_POINT('Ctrl Pts',(-21.0360011306814,10.2103895734123,
0.));
#238800=CARTESIAN_POINT('Ctrl Pts',(-21.0493123187483,10.2220787139157,
0.));
#238801=CARTESIAN_POINT('Ctrl Pts',(-21.0626848505665,10.233889368157,0.));
#238802=CARTESIAN_POINT('Ctrl Pts',(-21.0761174875448,10.2458211823915,
0.));
#238803=CARTESIAN_POINT('Ctrl Pts',(-21.0896090107066,10.2578738064183,
0.));
#238804=CARTESIAN_POINT('Ctrl Pts',(-21.1031582201625,10.2700468934743,
0.));
#238805=CARTESIAN_POINT('Ctrl Pts',(-21.1167639345623,10.2823401001067,
0.));
#238806=CARTESIAN_POINT('Ctrl Pts',(-21.130424990599,10.2947530860714,0.));
#238807=CARTESIAN_POINT('Ctrl Pts',(-21.1441402425831,10.307285514268,0.));
#238808=CARTESIAN_POINT('Ctrl Pts',(-21.1579085619959,10.3199370506541,
0.));
#238809=CARTESIAN_POINT('Ctrl Pts',(-21.1717288370512,10.3327073641574,
0.));
#238810=CARTESIAN_POINT('Ctrl Pts',(-21.1855999722427,10.3455961265706,
0.));
#238811=CARTESIAN_POINT('Ctrl Pts',(-21.1995208879205,10.3586030124595,
0.));
#238812=CARTESIAN_POINT('Ctrl Pts',(-21.2134905199359,10.3717276991137,
0.));
#238813=CARTESIAN_POINT('Ctrl Pts',(-21.2275078192708,10.384969866479,0.));
#238814=CARTESIAN_POINT('Ctrl Pts',(-21.2415717516713,10.3983291970846,
0.));
#238815=CARTESIAN_POINT('Ctrl Pts',(-21.2556812972741,10.4118053759584,
0.));
#238816=CARTESIAN_POINT('Ctrl Pts',(-21.2698354502391,10.4253980905394,
0.));
#238817=CARTESIAN_POINT('Ctrl Pts',(-21.2840332184471,10.4391070306385,
0.));
#238818=CARTESIAN_POINT('Ctrl Pts',(-21.2982736231924,10.452931888387,0.));
#238819=CARTESIAN_POINT('Ctrl Pts',(-21.312555698873,10.4668723581768,0.));
#238820=CARTESIAN_POINT('Ctrl Pts',(-21.3268784926823,10.4809281365933,
0.));
#238821=CARTESIAN_POINT('Ctrl Pts',(-21.3412410642912,10.4950989223341,
0.));
#238822=CARTESIAN_POINT('Ctrl Pts',(-21.3556424855822,10.5093844161689,
0.));
#238823=CARTESIAN_POINT('Ctrl Pts',(-21.3700818403942,10.523784320906,0.));
#238824=CARTESIAN_POINT('Ctrl Pts',(-21.3845582242604,10.5382983413422,
0.));
#238825=CARTESIAN_POINT('Ctrl Pts',(-21.3990707441495,10.5529261842107,
0.));
#238826=CARTESIAN_POINT('Ctrl Pts',(-21.4136185181974,10.5676675581106,
0.));
#238827=CARTESIAN_POINT('Ctrl Pts',(-21.4282006754624,10.582522173457,0.));
#238828=CARTESIAN_POINT('Ctrl Pts',(-21.4428163557137,10.597489742462,0.));
#238829=CARTESIAN_POINT('Ctrl Pts',(-21.4574647092093,10.612569979096,0.));
#238830=CARTESIAN_POINT('Ctrl Pts',(-21.4721448964766,10.6277625990457,
0.));
#238831=CARTESIAN_POINT('Ctrl Pts',(-21.4868560880893,10.6430673196609,
0.));
#238832=CARTESIAN_POINT('Ctrl Pts',(-21.5015974644454,10.658483859894,0.));
#238833=CARTESIAN_POINT('Ctrl Pts',(-21.5163682155805,10.6740119402835,
0.));
#238834=CARTESIAN_POINT('Ctrl Pts',(-21.531167540981,10.689651282929,0.));
#238835=CARTESIAN_POINT('Ctrl Pts',(-21.5459946493955,10.7054016114571,
0.));
#238836=CARTESIAN_POINT('Ctrl Pts',(-21.5608487586467,10.7212626509816,
0.));
#238837=CARTESIAN_POINT('Ctrl Pts',(-21.5757290954372,10.7372341280468,
0.));
#238838=CARTESIAN_POINT('Ctrl Pts',(-21.5906348951745,10.7533157705943,
0.));
#238839=CARTESIAN_POINT('Ctrl Pts',(-21.6055654018179,10.7695073079554,
0.));
#238840=CARTESIAN_POINT('Ctrl Pts',(-21.6205198677176,10.7858084708262,
0.));
#238841=CARTESIAN_POINT('Ctrl Pts',(-21.6354975534557,10.8022189912369,
0.));
#238842=CARTESIAN_POINT('Ctrl Pts',(-21.6504977276864,10.8187386025135,
0.));
#238843=CARTESIAN_POINT('Ctrl Pts',(-21.6655196669727,10.835367039227,0.));
#238844=CARTESIAN_POINT('Ctrl Pts',(-21.6805626556461,10.8521040371832,
0.));
#238845=CARTESIAN_POINT('Ctrl Pts',(-21.6956259856667,10.8689493334093,
0.));
#238846=CARTESIAN_POINT('Ctrl Pts',(-21.7107089564822,10.8859026661292,
0.));
#238847=CARTESIAN_POINT('Ctrl Pts',(-21.7258108748874,10.9029637747341,
0.));
#238848=CARTESIAN_POINT('Ctrl Pts',(-21.74093105488,10.9201323997386,0.));
#238849=CARTESIAN_POINT('Ctrl Pts',(-21.7560688175252,10.9374082827446,
0.));
#238850=CARTESIAN_POINT('Ctrl Pts',(-21.7712234908468,10.9547911664457,
0.));
#238851=CARTESIAN_POINT('Ctrl Pts',(-21.7863944097143,10.9722807946157,
0.));
#238852=CARTESIAN_POINT('Ctrl Pts',(-21.8015809157302,10.9898769120913,
0.));
#238853=CARTESIAN_POINT('Ctrl Pts',(-21.8167823571168,11.0075792647477,
0.));
#238854=CARTESIAN_POINT('Ctrl Pts',(-21.8319980886033,11.0253875994598,
0.));
#238855=CARTESIAN_POINT('Ctrl Pts',(-21.8472274713103,11.0433016640808,
0.));
#238856=CARTESIAN_POINT('Ctrl Pts',(-21.8624698726319,11.0613212074364,
0.));
#238857=CARTESIAN_POINT('Ctrl Pts',(-21.8777246661191,11.0794459793058,
0.));
#238858=CARTESIAN_POINT('Ctrl Pts',(-21.8929912313608,11.0976757303944,
0.));
#238859=CARTESIAN_POINT('Ctrl Pts',(-21.9082689538687,11.1160102123024,
0.));
#238860=CARTESIAN_POINT('Ctrl Pts',(-21.9235572249518,11.134449177474,0.));
#238861=CARTESIAN_POINT('Ctrl Pts',(-21.9388554416437,11.1529923792002,
0.));
#238862=CARTESIAN_POINT('Ctrl Pts',(-21.9541630066504,11.1716395716375,
0.));
#238863=CARTESIAN_POINT('Ctrl Pts',(-21.9694793282913,11.1903905098109,
0.));
#238864=CARTESIAN_POINT('Ctrl Pts',(-21.9848038204439,11.2092449496125,
0.));
#238865=CARTESIAN_POINT('Ctrl Pts',(-22.0001359024839,11.2282026477897,
0.));
#238866=CARTESIAN_POINT('Ctrl Pts',(-22.0154749992364,11.2472633619276,
0.));
#238867=CARTESIAN_POINT('Ctrl Pts',(-22.0308205408351,11.2664268504207,
0.));
#238868=CARTESIAN_POINT('Ctrl Pts',(-22.046171962566,11.2856928724374,0.));
#238869=CARTESIAN_POINT('Ctrl Pts',(-22.0615287047179,11.3050611878771,
0.));
#238870=CARTESIAN_POINT('Ctrl Pts',(-22.0768902124267,11.3245315573168,
0.));
#238871=CARTESIAN_POINT('Ctrl Pts',(-22.0922559355293,11.3441037419553,
0.));
#238872=CARTESIAN_POINT('Ctrl Pts',(-22.1076253283978,11.3637775035367,
0.));
#238873=CARTESIAN_POINT('Ctrl Pts',(-22.1229978500185,11.3835526044256,
0.));
#238874=CARTESIAN_POINT('Ctrl Pts',(-22.1383729640963,11.4034288076908,
0.));
#238875=CARTESIAN_POINT('Ctrl Pts',(-22.1537501391486,11.4234058771742,
0.));
#238876=CARTESIAN_POINT('Ctrl Pts',(-22.1691288486096,11.443483577557,0.));
#238877=CARTESIAN_POINT('Ctrl Pts',(-22.184508570917,11.463661674411,0.));
#238878=CARTESIAN_POINT('Ctrl Pts',(-22.1998887896435,11.4839399342589,
0.));
#238879=CARTESIAN_POINT('Ctrl Pts',(-22.215268993102,11.504318124424,0.));
#238880=CARTESIAN_POINT('Ctrl Pts',(-22.2306486738899,11.5247960128476,
0.));
#238881=CARTESIAN_POINT('Ctrl Pts',(-22.2460273284653,11.545373367912,0.));
#238882=CARTESIAN_POINT('Ctrl Pts',(-22.2614044566898,11.5660499582403,
0.));
#238883=CARTESIAN_POINT('Ctrl Pts',(-22.2767795614349,11.5868255525189,
0.));
#238884=CARTESIAN_POINT('Ctrl Pts',(-22.2921521480358,11.6076999192359,
0.));
#238885=CARTESIAN_POINT('Ctrl Pts',(-22.3075217249049,11.6286728270011,
0.));
#238886=CARTESIAN_POINT('Ctrl Pts',(-22.3228878043976,11.6497440449858,
0.));
#238887=CARTESIAN_POINT('Ctrl Pts',(-22.3382499035618,11.6709133432986,
0.));
#238888=CARTESIAN_POINT('Ctrl Pts',(-22.3536075450028,11.6921804934056,
0.));
#238889=CARTESIAN_POINT('Ctrl Pts',(-22.3689602575492,11.7135452684532,
0.));
#238890=CARTESIAN_POINT('Ctrl Pts',(-22.3843075773905,11.7350074437961,
0.));
#238891=CARTESIAN_POINT('Ctrl Pts',(-22.39964904692,11.7565667964765,0.));
#238892=CARTESIAN_POINT('Ctrl Pts',(-22.4149842125018,11.7782231042041,
0.));
#238893=CARTESIAN_POINT('Ctrl Pts',(-22.4303126226468,11.7999761445175,
0.));
#238894=CARTESIAN_POINT('Ctrl Pts',(-22.4456338258738,11.8218256937889,
0.));
#238895=CARTESIAN_POINT('Ctrl Pts',(-22.4609473690469,11.8437715264487,
0.));
#238896=CARTESIAN_POINT('Ctrl Pts',(-22.4762527946694,11.8658134137018,
0.));
#238897=CARTESIAN_POINT('Ctrl Pts',(-22.4915496418472,11.8879511239941,
0.));
#238898=CARTESIAN_POINT('Ctrl Pts',(-22.5068374513958,11.9101844254555,
0.));
#238899=CARTESIAN_POINT('Ctrl Pts',(-22.5221157697869,11.9325130877801,
0.));
#238900=CARTESIAN_POINT('Ctrl Pts',(-22.5373841537299,11.9549368843996,
0.));
#238901=CARTESIAN_POINT('Ctrl Pts',(-22.5526421741159,11.9774555943496,
0.));
#238902=CARTESIAN_POINT('Ctrl Pts',(-22.5678894211194,12.0000690046697,
0.));
#238903=CARTESIAN_POINT('Ctrl Pts',(-22.5831255061306,12.0227769113132,
0.));
#238904=CARTESIAN_POINT('Ctrl Pts',(-22.5983500505675,12.0455791139135,
0.));
#238905=CARTESIAN_POINT('Ctrl Pts',(-22.613562676493,12.0684754113869,0.));
#238906=CARTESIAN_POINT('Ctrl Pts',(-22.628762996708,12.0914655972828,0.));
#238907=CARTESIAN_POINT('Ctrl Pts',(-22.6439506046611,12.1145494550384,
0.));
#238908=CARTESIAN_POINT('Ctrl Pts',(-22.6591250653942,12.1377267537141,
0.));
#238909=CARTESIAN_POINT('Ctrl Pts',(-22.6742859034891,12.1609972423088,
0.));
#238910=CARTESIAN_POINT('Ctrl Pts',(-22.6894326204959,12.1843606579246,
0.));
#238911=CARTESIAN_POINT('Ctrl Pts',(-22.7045647168659,12.2078167360267,
0.));
#238912=CARTESIAN_POINT('Ctrl Pts',(-22.7196817119299,12.2313652198047,
0.));
#238913=CARTESIAN_POINT('Ctrl Pts',(-22.7347831655251,12.2550058702389,
0.));
#238914=CARTESIAN_POINT('Ctrl Pts',(-22.7498686970096,12.2787384750747,
0.));
#238915=CARTESIAN_POINT('Ctrl Pts',(-22.7649380101154,12.3025628601812,
0.));
#238916=CARTESIAN_POINT('Ctrl Pts',(-22.7799908974947,12.3264788926108,
0.));
#238917=CARTESIAN_POINT('Ctrl Pts',(-22.7950272216959,12.3504864740361,
0.));
#238918=CARTESIAN_POINT('Ctrl Pts',(-22.8100469022632,12.3745855366772,
0.));
#238919=CARTESIAN_POINT('Ctrl Pts',(-22.8220493007353,12.393937937903,0.));
#238920=CARTESIAN_POINT('Ctrl Pts',(-22.8310435872852,12.4084933766366,
0.));
#238921=CARTESIAN_POINT('Ctrl Pts',(-22.8370364396497,12.4182152851867,
0.));
#238922=CARTESIAN_POINT('Ctrl Pts',(-22.8400320311648,12.4230808101438,
0.));
#238923=CARTESIAN_POINT('',(-22.8400320311648,12.4230808101438,12.));
#238924=CARTESIAN_POINT('Ctrl Pts',(-22.8400320311648,12.4230808101438,
12.));
#238925=CARTESIAN_POINT('Ctrl Pts',(-22.8370364396497,12.4182152851867,
12.));
#238926=CARTESIAN_POINT('Ctrl Pts',(-22.8310435872852,12.4084933766366,
12.));
#238927=CARTESIAN_POINT('Ctrl Pts',(-22.8220493007353,12.393937937903,12.));
#238928=CARTESIAN_POINT('Ctrl Pts',(-22.8100469022632,12.3745855366772,
12.));
#238929=CARTESIAN_POINT('Ctrl Pts',(-22.7950272216959,12.3504864740361,
12.));
#238930=CARTESIAN_POINT('Ctrl Pts',(-22.7799908974947,12.3264788926108,
12.));
#238931=CARTESIAN_POINT('Ctrl Pts',(-22.7649380101154,12.3025628601812,
12.));
#238932=CARTESIAN_POINT('Ctrl Pts',(-22.7498686970096,12.2787384750747,
12.));
#238933=CARTESIAN_POINT('Ctrl Pts',(-22.7347831655251,12.2550058702389,
12.));
#238934=CARTESIAN_POINT('Ctrl Pts',(-22.7196817119299,12.2313652198047,
12.));
#238935=CARTESIAN_POINT('Ctrl Pts',(-22.7045647168659,12.2078167360267,
12.));
#238936=CARTESIAN_POINT('Ctrl Pts',(-22.6894326204959,12.1843606579246,
12.));
#238937=CARTESIAN_POINT('Ctrl Pts',(-22.6742859034891,12.1609972423088,
12.));
#238938=CARTESIAN_POINT('Ctrl Pts',(-22.6591250653942,12.1377267537141,
12.));
#238939=CARTESIAN_POINT('Ctrl Pts',(-22.6439506046611,12.1145494550384,
12.));
#238940=CARTESIAN_POINT('Ctrl Pts',(-22.628762996708,12.0914655972828,12.));
#238941=CARTESIAN_POINT('Ctrl Pts',(-22.613562676493,12.0684754113869,12.));
#238942=CARTESIAN_POINT('Ctrl Pts',(-22.5983500505675,12.0455791139135,
12.));
#238943=CARTESIAN_POINT('Ctrl Pts',(-22.5831255061306,12.0227769113132,
12.));
#238944=CARTESIAN_POINT('Ctrl Pts',(-22.5678894211194,12.0000690046697,
12.));
#238945=CARTESIAN_POINT('Ctrl Pts',(-22.5526421741159,11.9774555943496,
12.));
#238946=CARTESIAN_POINT('Ctrl Pts',(-22.5373841537299,11.9549368843996,
12.));
#238947=CARTESIAN_POINT('Ctrl Pts',(-22.5221157697869,11.9325130877801,
12.));
#238948=CARTESIAN_POINT('Ctrl Pts',(-22.5068374513958,11.9101844254555,
12.));
#238949=CARTESIAN_POINT('Ctrl Pts',(-22.4915496418472,11.8879511239941,
12.));
#238950=CARTESIAN_POINT('Ctrl Pts',(-22.4762527946694,11.8658134137018,
12.));
#238951=CARTESIAN_POINT('Ctrl Pts',(-22.4609473690469,11.8437715264487,
12.));
#238952=CARTESIAN_POINT('Ctrl Pts',(-22.4456338258738,11.8218256937889,
12.));
#238953=CARTESIAN_POINT('Ctrl Pts',(-22.4303126226468,11.7999761445175,
12.));
#238954=CARTESIAN_POINT('Ctrl Pts',(-22.4149842125018,11.7782231042041,
12.));
#238955=CARTESIAN_POINT('Ctrl Pts',(-22.39964904692,11.7565667964765,12.));
#238956=CARTESIAN_POINT('Ctrl Pts',(-22.3843075773905,11.7350074437961,
12.));
#238957=CARTESIAN_POINT('Ctrl Pts',(-22.3689602575492,11.7135452684532,
12.));
#238958=CARTESIAN_POINT('Ctrl Pts',(-22.3536075450028,11.6921804934056,
12.));
#238959=CARTESIAN_POINT('Ctrl Pts',(-22.3382499035618,11.6709133432986,
12.));
#238960=CARTESIAN_POINT('Ctrl Pts',(-22.3228878043976,11.6497440449858,
12.));
#238961=CARTESIAN_POINT('Ctrl Pts',(-22.3075217249049,11.6286728270011,
12.));
#238962=CARTESIAN_POINT('Ctrl Pts',(-22.2921521480358,11.6076999192359,
12.));
#238963=CARTESIAN_POINT('Ctrl Pts',(-22.2767795614349,11.5868255525189,
12.));
#238964=CARTESIAN_POINT('Ctrl Pts',(-22.2614044566898,11.5660499582403,
12.));
#238965=CARTESIAN_POINT('Ctrl Pts',(-22.2460273284653,11.545373367912,12.));
#238966=CARTESIAN_POINT('Ctrl Pts',(-22.2306486738899,11.5247960128476,
12.));
#238967=CARTESIAN_POINT('Ctrl Pts',(-22.215268993102,11.504318124424,12.));
#238968=CARTESIAN_POINT('Ctrl Pts',(-22.1998887896435,11.4839399342589,
12.));
#238969=CARTESIAN_POINT('Ctrl Pts',(-22.184508570917,11.463661674411,12.));
#238970=CARTESIAN_POINT('Ctrl Pts',(-22.1691288486096,11.443483577557,12.));
#238971=CARTESIAN_POINT('Ctrl Pts',(-22.1537501391486,11.4234058771742,
12.));
#238972=CARTESIAN_POINT('Ctrl Pts',(-22.1383729640963,11.4034288076908,
12.));
#238973=CARTESIAN_POINT('Ctrl Pts',(-22.1229978500185,11.3835526044256,
12.));
#238974=CARTESIAN_POINT('Ctrl Pts',(-22.1076253283978,11.3637775035367,
12.));
#238975=CARTESIAN_POINT('Ctrl Pts',(-22.0922559355293,11.3441037419553,
12.));
#238976=CARTESIAN_POINT('Ctrl Pts',(-22.0768902124267,11.3245315573168,
12.));
#238977=CARTESIAN_POINT('Ctrl Pts',(-22.0615287047179,11.3050611878771,
12.));
#238978=CARTESIAN_POINT('Ctrl Pts',(-22.046171962566,11.2856928724374,12.));
#238979=CARTESIAN_POINT('Ctrl Pts',(-22.0308205408351,11.2664268504207,
12.));
#238980=CARTESIAN_POINT('Ctrl Pts',(-22.0154749992364,11.2472633619276,
12.));
#238981=CARTESIAN_POINT('Ctrl Pts',(-22.0001359024839,11.2282026477897,
12.));
#238982=CARTESIAN_POINT('Ctrl Pts',(-21.9848038204439,11.2092449496125,
12.));
#238983=CARTESIAN_POINT('Ctrl Pts',(-21.9694793282913,11.1903905098109,
12.));
#238984=CARTESIAN_POINT('Ctrl Pts',(-21.9541630066504,11.1716395716375,
12.));
#238985=CARTESIAN_POINT('Ctrl Pts',(-21.9388554416437,11.1529923792002,
12.));
#238986=CARTESIAN_POINT('Ctrl Pts',(-21.9235572249518,11.134449177474,12.));
#238987=CARTESIAN_POINT('Ctrl Pts',(-21.9082689538687,11.1160102123024,
12.));
#238988=CARTESIAN_POINT('Ctrl Pts',(-21.8929912313608,11.0976757303944,
12.));
#238989=CARTESIAN_POINT('Ctrl Pts',(-21.8777246661191,11.0794459793058,
12.));
#238990=CARTESIAN_POINT('Ctrl Pts',(-21.8624698726319,11.0613212074364,
12.));
#238991=CARTESIAN_POINT('Ctrl Pts',(-21.8472274713103,11.0433016640808,
12.));
#238992=CARTESIAN_POINT('Ctrl Pts',(-21.8319980886033,11.0253875994598,
12.));
#238993=CARTESIAN_POINT('Ctrl Pts',(-21.8167823571168,11.0075792647477,
12.));
#238994=CARTESIAN_POINT('Ctrl Pts',(-21.8015809157302,10.9898769120913,
12.));
#238995=CARTESIAN_POINT('Ctrl Pts',(-21.7863944097143,10.9722807946157,
12.));
#238996=CARTESIAN_POINT('Ctrl Pts',(-21.7712234908468,10.9547911664457,
12.));
#238997=CARTESIAN_POINT('Ctrl Pts',(-21.7560688175252,10.9374082827446,
12.));
#238998=CARTESIAN_POINT('Ctrl Pts',(-21.74093105488,10.9201323997386,12.));
#238999=CARTESIAN_POINT('Ctrl Pts',(-21.7258108748874,10.9029637747341,
12.));
#239000=CARTESIAN_POINT('Ctrl Pts',(-21.7107089564822,10.8859026661292,
12.));
#239001=CARTESIAN_POINT('Ctrl Pts',(-21.6956259856667,10.8689493334093,
12.));
#239002=CARTESIAN_POINT('Ctrl Pts',(-21.6805626556461,10.8521040371832,
12.));
#239003=CARTESIAN_POINT('Ctrl Pts',(-21.6655196669727,10.835367039227,12.));
#239004=CARTESIAN_POINT('Ctrl Pts',(-21.6504977276864,10.8187386025135,
12.));
#239005=CARTESIAN_POINT('Ctrl Pts',(-21.6354975534557,10.8022189912369,
12.));
#239006=CARTESIAN_POINT('Ctrl Pts',(-21.6205198677176,10.7858084708262,
12.));
#239007=CARTESIAN_POINT('Ctrl Pts',(-21.6055654018179,10.7695073079554,
12.));
#239008=CARTESIAN_POINT('Ctrl Pts',(-21.5906348951745,10.7533157705943,
12.));
#239009=CARTESIAN_POINT('Ctrl Pts',(-21.5757290954372,10.7372341280468,
12.));
#239010=CARTESIAN_POINT('Ctrl Pts',(-21.5608487586467,10.7212626509816,
12.));
#239011=CARTESIAN_POINT('Ctrl Pts',(-21.5459946493955,10.7054016114571,
12.));
#239012=CARTESIAN_POINT('Ctrl Pts',(-21.531167540981,10.689651282929,12.));
#239013=CARTESIAN_POINT('Ctrl Pts',(-21.5163682155805,10.6740119402835,
12.));
#239014=CARTESIAN_POINT('Ctrl Pts',(-21.5015974644454,10.658483859894,12.));
#239015=CARTESIAN_POINT('Ctrl Pts',(-21.4868560880893,10.6430673196609,
12.));
#239016=CARTESIAN_POINT('Ctrl Pts',(-21.4721448964766,10.6277625990457,
12.));
#239017=CARTESIAN_POINT('Ctrl Pts',(-21.4574647092093,10.612569979096,12.));
#239018=CARTESIAN_POINT('Ctrl Pts',(-21.4428163557137,10.597489742462,12.));
#239019=CARTESIAN_POINT('Ctrl Pts',(-21.4282006754624,10.582522173457,12.));
#239020=CARTESIAN_POINT('Ctrl Pts',(-21.4136185181974,10.5676675581106,
12.));
#239021=CARTESIAN_POINT('Ctrl Pts',(-21.3990707441495,10.5529261842107,
12.));
#239022=CARTESIAN_POINT('Ctrl Pts',(-21.3845582242604,10.5382983413422,
12.));
#239023=CARTESIAN_POINT('Ctrl Pts',(-21.3700818403942,10.523784320906,12.));
#239024=CARTESIAN_POINT('Ctrl Pts',(-21.3556424855822,10.5093844161689,
12.));
#239025=CARTESIAN_POINT('Ctrl Pts',(-21.3412410642912,10.4950989223341,
12.));
#239026=CARTESIAN_POINT('Ctrl Pts',(-21.3268784926823,10.4809281365933,
12.));
#239027=CARTESIAN_POINT('Ctrl Pts',(-21.312555698873,10.4668723581768,12.));
#239028=CARTESIAN_POINT('Ctrl Pts',(-21.2982736231924,10.452931888387,12.));
#239029=CARTESIAN_POINT('Ctrl Pts',(-21.2840332184471,10.4391070306385,
12.));
#239030=CARTESIAN_POINT('Ctrl Pts',(-21.2698354502391,10.4253980905394,
12.));
#239031=CARTESIAN_POINT('Ctrl Pts',(-21.2556812972741,10.4118053759584,
12.));
#239032=CARTESIAN_POINT('Ctrl Pts',(-21.2415717516713,10.3983291970846,
12.));
#239033=CARTESIAN_POINT('Ctrl Pts',(-21.2275078192708,10.384969866479,12.));
#239034=CARTESIAN_POINT('Ctrl Pts',(-21.2134905199359,10.3717276991137,
12.));
#239035=CARTESIAN_POINT('Ctrl Pts',(-21.1995208879205,10.3586030124595,
12.));
#239036=CARTESIAN_POINT('Ctrl Pts',(-21.1855999722427,10.3455961265706,
12.));
#239037=CARTESIAN_POINT('Ctrl Pts',(-21.1717288370512,10.3327073641574,
12.));
#239038=CARTESIAN_POINT('Ctrl Pts',(-21.1579085619959,10.3199370506541,
12.));
#239039=CARTESIAN_POINT('Ctrl Pts',(-21.1441402425831,10.307285514268,12.));
#239040=CARTESIAN_POINT('Ctrl Pts',(-21.130424990599,10.2947530860714,12.));
#239041=CARTESIAN_POINT('Ctrl Pts',(-21.1167639345623,10.2823401001067,
12.));
#239042=CARTESIAN_POINT('Ctrl Pts',(-21.1031582201625,10.2700468934743,
12.));
#239043=CARTESIAN_POINT('Ctrl Pts',(-21.0896090107066,10.2578738064183,
12.));
#239044=CARTESIAN_POINT('Ctrl Pts',(-21.0761174875448,10.2458211823915,
12.));
#239045=CARTESIAN_POINT('Ctrl Pts',(-21.0626848505665,10.233889368157,12.));
#239046=CARTESIAN_POINT('Ctrl Pts',(-21.0493123187483,10.2220787139157,
12.));
#239047=CARTESIAN_POINT('Ctrl Pts',(-21.0360011306814,10.2103895734123,
12.));
#239048=CARTESIAN_POINT('Ctrl Pts',(-21.0227525451107,10.1988223040425,
12.));
#239049=CARTESIAN_POINT('Ctrl Pts',(-21.0095678414486,10.1873772669358,
12.));
#239050=CARTESIAN_POINT('Ctrl Pts',(-20.9964483203685,10.1760548270765,
12.));
#239051=CARTESIAN_POINT('Ctrl Pts',(-20.9833953044737,10.1648553534567,
12.));
#239052=CARTESIAN_POINT('Ctrl Pts',(-20.970410138937,10.1537792192065,12.));
#239053=CARTESIAN_POINT('Ctrl Pts',(-20.9574941921591,10.1428268017257,
12.));
#239054=CARTESIAN_POINT('Ctrl Pts',(-20.944648856393,10.1319984827909,12.));
#239055=CARTESIAN_POINT('Ctrl Pts',(-20.931875548473,10.1212946487057,12.));
#239056=CARTESIAN_POINT('Ctrl Pts',(-20.9191757106266,10.1107156904836,
12.));
#239057=CARTESIAN_POINT('Ctrl Pts',(-20.9065508112556,10.1002620040076,
12.));
#239058=CARTESIAN_POINT('Ctrl Pts',(-20.8940023457371,10.0899339901916,
12.));
#239059=CARTESIAN_POINT('Ctrl Pts',(-20.8815318371844,10.0797320551154,
12.));
#239060=CARTESIAN_POINT('Ctrl Pts',(-20.8691408373705,10.0696566102219,
12.));
#239061=CARTESIAN_POINT('Ctrl Pts',(-20.856830927732,10.0597080725375,12.));
#239062=CARTESIAN_POINT('Ctrl Pts',(-20.8446037203402,10.0498868648733,
12.));
#239063=CARTESIAN_POINT('Ctrl Pts',(-20.8324608588906,10.0401934160234,
12.));
#239064=CARTESIAN_POINT('Ctrl Pts',(-20.8204040196599,10.0306281609435,
12.));
#239065=CARTESIAN_POINT('Ctrl Pts',(-20.8084349126885,10.0211915410095,
12.));
#239066=CARTESIAN_POINT('Ctrl Pts',(-20.7965552829907,10.0118840042786,
12.));
#239067=CARTESIAN_POINT('Ctrl Pts',(-20.7847669117568,10.0027060057389,
12.));
#239068=CARTESIAN_POINT('Ctrl Pts',(-20.7730716175417,9.99365800754638,
12.));
#239069=CARTESIAN_POINT('Ctrl Pts',(-20.7614712574989,9.98474047926846,
12.));
#239070=CARTESIAN_POINT('Ctrl Pts',(-20.7499677289625,9.97595389823461,
12.));
#239071=CARTESIAN_POINT('Ctrl Pts',(-20.7385629709795,9.96729874986198,
12.));
#239072=CARTESIAN_POINT('Ctrl Pts',(-20.7272589658752,9.95877552798403,
12.));
#239073=CARTESIAN_POINT('Ctrl Pts',(-20.716057740758,9.95038473514962,12.));
#239074=CARTESIAN_POINT('Ctrl Pts',(-20.7049613692237,9.94212688298251,
12.));
#239075=CARTESIAN_POINT('Ctrl Pts',(-20.6939719732485,9.93400249259736,
12.));
#239076=CARTESIAN_POINT('Ctrl Pts',(-20.6830917250255,9.9260120949875,12.));
#239077=CARTESIAN_POINT('Ctrl Pts',(-20.6723228488262,9.91815623141284,
12.));
#239078=CARTESIAN_POINT('Ctrl Pts',(-20.6616676228315,9.91043545377004,
12.));
#239079=CARTESIAN_POINT('Ctrl Pts',(-20.6511283817415,9.90285032516696,
12.));
#239080=CARTESIAN_POINT('Ctrl Pts',(-20.6407075193977,9.89540142049124,
12.));
#239081=CARTESIAN_POINT('Ctrl Pts',(-20.6304074914086,9.88808932697305,
12.));
#239082=CARTESIAN_POINT('Ctrl Pts',(-20.6202308177472,9.88091464472669,
12.));
#239083=CARTESIAN_POINT('Ctrl Pts',(-20.6101800854491,9.87387798732944,
12.));
#239084=CARTESIAN_POINT('Ctrl Pts',(-20.6002579513696,9.86697998242612,
12.));
#239085=CARTESIAN_POINT('Ctrl Pts',(-20.5904671449754,9.86022127232749,
12.));
#239086=CARTESIAN_POINT('Ctrl Pts',(-20.580810471002,9.85360251457004,12.));
#239087=CARTESIAN_POINT('Ctrl Pts',(-20.5712908125145,9.84712438256308,
12.));
#239088=CARTESIAN_POINT('Ctrl Pts',(-20.5619111362406,9.84078756677589,
12.));
#239089=CARTESIAN_POINT('Ctrl Pts',(-20.5526744976461,9.83459277585321,
12.));
#239090=CARTESIAN_POINT('Ctrl Pts',(-20.5435840460717,9.82854073773857,
12.));
#239091=CARTESIAN_POINT('Ctrl Pts',(-20.534643029951,9.82263220080328,12.));
#239092=CARTESIAN_POINT('Ctrl Pts',(-20.5258548000625,9.81686793455918,
12.));
#239093=CARTESIAN_POINT('Ctrl Pts',(-20.5172228122839,9.81124873025278,
12.));
#239094=CARTESIAN_POINT('Ctrl Pts',(-20.5087506310507,9.80577540161103,
12.));
#239095=CARTESIAN_POINT('Ctrl Pts',(-20.500441931211,9.80044878520967,12.));
#239096=CARTESIAN_POINT('Ctrl Pts',(-20.4923005087945,9.79526974288344,
12.));
#239097=CARTESIAN_POINT('Ctrl Pts',(-20.4843302955329,9.7902391649866,12.));
#239098=CARTESIAN_POINT('Ctrl Pts',(-20.4765353711585,9.78535797314162,
12.));
#239099=CARTESIAN_POINT('Ctrl Pts',(-20.4689199790668,9.78062712373313,
12.));
#239100=CARTESIAN_POINT('Ctrl Pts',(-20.4614885274973,9.77604760815523,
12.));
#239101=CARTESIAN_POINT('Ctrl Pts',(-20.4542455817527,9.7716204510407,12.));
#239102=CARTESIAN_POINT('Ctrl Pts',(-20.447195862298,9.76734670980897,12.));
#239103=CARTESIAN_POINT('Ctrl Pts',(-20.4403442329401,9.76322747195502,
12.));
#239104=CARTESIAN_POINT('Ctrl Pts',(-20.4336957355474,9.7592638628993,12.));
#239105=CARTESIAN_POINT('Ctrl Pts',(-20.4272556476629,9.75545705902416,
12.));
#239106=CARTESIAN_POINT('Ctrl Pts',(-20.4210295275818,9.75180829786433,
12.));
#239107=CARTESIAN_POINT('Ctrl Pts',(-20.4150232777393,9.74831889242175,
12.));
#239108=CARTESIAN_POINT('Ctrl Pts',(-20.4092430879861,9.74499021838536,
12.));
#239109=CARTESIAN_POINT('Ctrl Pts',(-20.4036953576549,9.74182369656272,
12.));
#239110=CARTESIAN_POINT('Ctrl Pts',(-20.3983866213331,9.73882077613206,
12.));
#239111=CARTESIAN_POINT('Ctrl Pts',(-20.3933234845646,9.7359829201425,12.));
#239112=CARTESIAN_POINT('Ctrl Pts',(-20.3885129129912,9.73331167102812,
12.));
#239113=CARTESIAN_POINT('Ctrl Pts',(-20.3839624556742,9.73080870123726,
12.));
#239114=CARTESIAN_POINT('Ctrl Pts',(-20.3796805893304,9.72847589116533,
12.));
#239115=CARTESIAN_POINT('Ctrl Pts',(-20.3756766651952,9.72631531732871,
12.));
#239116=CARTESIAN_POINT('Ctrl Pts',(-20.371960235676,9.72432910043193,12.));
#239117=CARTESIAN_POINT('Ctrl Pts',(-20.3685406190576,9.72251930722504,
12.));
#239118=CARTESIAN_POINT('Ctrl Pts',(-20.3654261611055,9.72088778381102,
12.));
#239119=CARTESIAN_POINT('Ctrl Pts',(-20.362625691398,9.71943648548114,12.));
#239120=CARTESIAN_POINT('Ctrl Pts',(-20.3601498764344,9.71816778327999,
12.));
#239121=CARTESIAN_POINT('Ctrl Pts',(-20.3580133103357,9.71708493723061,
12.));
#239122=CARTESIAN_POINT('Ctrl Pts',(-20.3562337557875,9.71619192554147,
12.));
#239123=CARTESIAN_POINT('Ctrl Pts',(-20.3548282742361,9.71549257088175,
12.));
#239124=CARTESIAN_POINT('Ctrl Pts',(-20.3538098605706,9.71498978052101,
12.));
#239125=CARTESIAN_POINT('Ctrl Pts',(-20.3533097561886,9.71474590350791,
12.));
#239126=CARTESIAN_POINT('Ctrl Pts',(-20.3531126095522,9.71465227853122,
12.));
#239127=CARTESIAN_POINT('Ctrl Pts',(-20.353060251684,9.71462954053074,12.));
#239128=CARTESIAN_POINT('Ctrl Pts',(-20.353053841303,9.71462809124917,12.));
#239129=CARTESIAN_POINT('',(-22.8400320311648,12.4230808101438,0.));
#239130=CARTESIAN_POINT('Origin',(-16.3449727195352,13.9675290154577,0.));
#239131=CARTESIAN_POINT('',(-17.1452095830633,14.6513681262571,12.));
#239132=CARTESIAN_POINT('',(-8.17248635976757,6.98376450772883,12.));
#239133=CARTESIAN_POINT('',(-17.1452095830633,14.6513681262571,0.));
#239134=CARTESIAN_POINT('',(-17.1452095830633,14.6513681262571,0.));
#239135=CARTESIAN_POINT('',(-8.17248635976757,6.98376450772883,0.));
#239136=CARTESIAN_POINT('Ctrl Pts',(-22.1787195904339,13.5685075571671,
0.));
#239137=CARTESIAN_POINT('Ctrl Pts',(-22.1787195904339,13.5685075571671,
12.));
#239138=CARTESIAN_POINT('Ctrl Pts',(-22.1730081264583,13.5683460612913,
0.));
#239139=CARTESIAN_POINT('Ctrl Pts',(-22.1730081264583,13.5683460612913,
12.));
#239140=CARTESIAN_POINT('Ctrl Pts',(-22.1615922804939,13.5680170531724,
0.));
#239141=CARTESIAN_POINT('Ctrl Pts',(-22.1615922804939,13.5680170531724,
12.));
#239142=CARTESIAN_POINT('Ctrl Pts',(-22.1444897575076,13.5675054918922,
0.));
#239143=CARTESIAN_POINT('Ctrl Pts',(-22.1444897575076,13.5675054918922,
12.));
#239144=CARTESIAN_POINT('Ctrl Pts',(-22.1217288871823,13.5667873105179,
0.));
#239145=CARTESIAN_POINT('Ctrl Pts',(-22.1217288871823,13.5667873105179,
12.));
#239146=CARTESIAN_POINT('Ctrl Pts',(-22.0933486464442,13.5658294169106,
0.));
#239147=CARTESIAN_POINT('Ctrl Pts',(-22.0933486464442,13.5658294169106,
12.));
#239148=CARTESIAN_POINT('Ctrl Pts',(-22.0650393089492,13.5648113688894,
0.));
#239149=CARTESIAN_POINT('Ctrl Pts',(-22.0650393089492,13.5648113688894,
12.));
#239150=CARTESIAN_POINT('Ctrl Pts',(-22.0368009736227,13.5637332022393,
0.));
#239151=CARTESIAN_POINT('Ctrl Pts',(-22.0368009736227,13.5637332022393,
12.));
#239152=CARTESIAN_POINT('Ctrl Pts',(-22.0086337943431,13.5625949868313,
0.));
#239153=CARTESIAN_POINT('Ctrl Pts',(-22.0086337943431,13.5625949868313,
12.));
#239154=CARTESIAN_POINT('Ctrl Pts',(-21.9805379899192,13.5613968357589,
0.));
#239155=CARTESIAN_POINT('Ctrl Pts',(-21.9805379899192,13.5613968357589,
12.));
#239156=CARTESIAN_POINT('Ctrl Pts',(-21.9525138592862,13.5601389185315,
0.));
#239157=CARTESIAN_POINT('Ctrl Pts',(-21.9525138592862,13.5601389185315,
12.));
#239158=CARTESIAN_POINT('Ctrl Pts',(-21.9245617765827,13.5588214586672,
0.));
#239159=CARTESIAN_POINT('Ctrl Pts',(-21.9245617765827,13.5588214586672,
12.));
#239160=CARTESIAN_POINT('Ctrl Pts',(-21.8966821688876,13.5574447178484,
0.));
#239161=CARTESIAN_POINT('Ctrl Pts',(-21.8966821688876,13.5574447178484,
12.));
#239162=CARTESIAN_POINT('Ctrl Pts',(-21.8688754989401,13.5560089839426,
0.));
#239163=CARTESIAN_POINT('Ctrl Pts',(-21.8688754989401,13.5560089839426,
12.));
#239164=CARTESIAN_POINT('Ctrl Pts',(-21.841142245609,13.5545145573048,0.));
#239165=CARTESIAN_POINT('Ctrl Pts',(-21.841142245609,13.5545145573048,12.));
#239166=CARTESIAN_POINT('Ctrl Pts',(-21.8134828857963,13.5529617381569,
0.));
#239167=CARTESIAN_POINT('Ctrl Pts',(-21.8134828857963,13.5529617381569,
12.));
#239168=CARTESIAN_POINT('Ctrl Pts',(-21.7858978745848,13.5513508127232,
0.));
#239169=CARTESIAN_POINT('Ctrl Pts',(-21.7858978745848,13.5513508127232,
12.));
#239170=CARTESIAN_POINT('Ctrl Pts',(-21.7583876294532,13.5496820422186,
0.));
#239171=CARTESIAN_POINT('Ctrl Pts',(-21.7583876294532,13.5496820422186,
12.));
#239172=CARTESIAN_POINT('Ctrl Pts',(-21.730952541226,13.5479556704457,0.));
#239173=CARTESIAN_POINT('Ctrl Pts',(-21.730952541226,13.5479556704457,12.));
#239174=CARTESIAN_POINT('Ctrl Pts',(-21.7035929822939,13.546171929503,0.));
#239175=CARTESIAN_POINT('Ctrl Pts',(-21.7035929822939,13.546171929503,12.));
#239176=CARTESIAN_POINT('Ctrl Pts',(-21.676309315769,13.5443310461516,0.));
#239177=CARTESIAN_POINT('Ctrl Pts',(-21.676309315769,13.5443310461516,12.));
#239178=CARTESIAN_POINT('Ctrl Pts',(-21.6491019044647,13.5424332480698,
0.));
#239179=CARTESIAN_POINT('Ctrl Pts',(-21.6491019044647,13.5424332480698,
12.));
#239180=CARTESIAN_POINT('Ctrl Pts',(-21.6219711193951,13.5404787697798,
0.));
#239181=CARTESIAN_POINT('Ctrl Pts',(-21.6219711193951,13.5404787697798,
12.));
#239182=CARTESIAN_POINT('Ctrl Pts',(-21.5949173499022,13.5384678597206,
0.));
#239183=CARTESIAN_POINT('Ctrl Pts',(-21.5949173499022,13.5384678597206,
12.));
#239184=CARTESIAN_POINT('Ctrl Pts',(-21.5679410019011,13.5364007790292,
0.));
#239185=CARTESIAN_POINT('Ctrl Pts',(-21.5679410019011,13.5364007790292,
12.));
#239186=CARTESIAN_POINT('Ctrl Pts',(-21.5410424932511,13.5342777983225,
0.));
#239187=CARTESIAN_POINT('Ctrl Pts',(-21.5410424932511,13.5342777983225,
12.));
#239188=CARTESIAN_POINT('Ctrl Pts',(-21.5142222501671,13.5320991952145,
0.));
#239189=CARTESIAN_POINT('Ctrl Pts',(-21.5142222501671,13.5320991952145,
12.));
#239190=CARTESIAN_POINT('Ctrl Pts',(-21.487480703047,13.5298652514357,0.));
#239191=CARTESIAN_POINT('Ctrl Pts',(-21.487480703047,13.5298652514357,12.));
#239192=CARTESIAN_POINT('Ctrl Pts',(-21.4608182828695,13.5275762503553,
0.));
#239193=CARTESIAN_POINT('Ctrl Pts',(-21.4608182828695,13.5275762503553,
12.));
#239194=CARTESIAN_POINT('Ctrl Pts',(-21.4342354165254,13.5252324737795,
0.));
#239195=CARTESIAN_POINT('Ctrl Pts',(-21.4342354165254,13.5252324737795,
12.));
#239196=CARTESIAN_POINT('Ctrl Pts',(-21.4077325259318,13.5228342013508,
0.));
#239197=CARTESIAN_POINT('Ctrl Pts',(-21.4077325259318,13.5228342013508,
12.));
#239198=CARTESIAN_POINT('Ctrl Pts',(-21.3813100304967,13.5203817122496,
0.));
#239199=CARTESIAN_POINT('Ctrl Pts',(-21.3813100304967,13.5203817122496,
12.));
#239200=CARTESIAN_POINT('Ctrl Pts',(-21.3549683486219,13.5178752862461,
0.));
#239201=CARTESIAN_POINT('Ctrl Pts',(-21.3549683486219,13.5178752862461,
12.));
#239202=CARTESIAN_POINT('Ctrl Pts',(-21.328707899634,13.5153152050554,0.));
#239203=CARTESIAN_POINT('Ctrl Pts',(-21.328707899634,13.5153152050554,12.));
#239204=CARTESIAN_POINT('Ctrl Pts',(-21.3025291054236,13.5127017534972,
0.));
#239205=CARTESIAN_POINT('Ctrl Pts',(-21.3025291054236,13.5127017534972,
12.));
#239206=CARTESIAN_POINT('Ctrl Pts',(-21.2764323924442,13.5100352209207,
0.));
#239207=CARTESIAN_POINT('Ctrl Pts',(-21.2764323924442,13.5100352209207,
12.));
#239208=CARTESIAN_POINT('Ctrl Pts',(-21.2504181927429,13.5073159019454,
0.));
#239209=CARTESIAN_POINT('Ctrl Pts',(-21.2504181927429,13.5073159019454,
12.));
#239210=CARTESIAN_POINT('Ctrl Pts',(-21.224486942933,13.5045440957404,0.));
#239211=CARTESIAN_POINT('Ctrl Pts',(-21.224486942933,13.5045440957404,12.));
#239212=CARTESIAN_POINT('Ctrl Pts',(-21.1986390835825,13.5017201056088,
0.));
#239213=CARTESIAN_POINT('Ctrl Pts',(-21.1986390835825,13.5017201056088,
12.));
#239214=CARTESIAN_POINT('Ctrl Pts',(-21.1728750584173,13.4988442384491,
0.));
#239215=CARTESIAN_POINT('Ctrl Pts',(-21.1728750584173,13.4988442384491,
12.));
#239216=CARTESIAN_POINT('Ctrl Pts',(-21.1471953136209,13.4959168042934,
0.));
#239217=CARTESIAN_POINT('Ctrl Pts',(-21.1471953136209,13.4959168042934,
12.));
#239218=CARTESIAN_POINT('Ctrl Pts',(-21.1216002970209,13.4929381157778,
0.));
#239219=CARTESIAN_POINT('Ctrl Pts',(-21.1216002970209,13.4929381157778,
12.));
#239220=CARTESIAN_POINT('Ctrl Pts',(-21.0960904575048,13.4899084877718,
0.));
#239221=CARTESIAN_POINT('Ctrl Pts',(-21.0960904575048,13.4899084877718,
12.));
#239222=CARTESIAN_POINT('Ctrl Pts',(-21.0706662455202,13.4868282377191,
0.));
#239223=CARTESIAN_POINT('Ctrl Pts',(-21.0706662455202,13.4868282377191,
12.));
#239224=CARTESIAN_POINT('Ctrl Pts',(-21.0453281134247,13.4836976858912,
0.));
#239225=CARTESIAN_POINT('Ctrl Pts',(-21.0453281134247,13.4836976858912,
12.));
#239226=CARTESIAN_POINT('Ctrl Pts',(-21.0200765158885,13.4805171556822,
0.));
#239227=CARTESIAN_POINT('Ctrl Pts',(-21.0200765158885,13.4805171556822,
12.));
#239228=CARTESIAN_POINT('Ctrl Pts',(-20.9949119102592,13.4772869738879,
0.));
#239229=CARTESIAN_POINT('Ctrl Pts',(-20.9949119102592,13.4772869738879,
12.));
#239230=CARTESIAN_POINT('Ctrl Pts',(-20.9698347569476,13.4740074710087,
0.));
#239231=CARTESIAN_POINT('Ctrl Pts',(-20.9698347569476,13.4740074710087,
12.));
#239232=CARTESIAN_POINT('Ctrl Pts',(-20.9448455197557,13.4706789815166,
0.));
#239233=CARTESIAN_POINT('Ctrl Pts',(-20.9448455197557,13.4706789815166,
12.));
#239234=CARTESIAN_POINT('Ctrl Pts',(-20.9199446657584,13.4673018437718,
0.));
#239235=CARTESIAN_POINT('Ctrl Pts',(-20.9199446657584,13.4673018437718,
12.));
#239236=CARTESIAN_POINT('Ctrl Pts',(-20.8951326652158,13.4638763999725,
0.));
#239237=CARTESIAN_POINT('Ctrl Pts',(-20.8951326652158,13.4638763999725,
12.));
#239238=CARTESIAN_POINT('Ctrl Pts',(-20.8704099914641,13.4604029960983,
0.));
#239239=CARTESIAN_POINT('Ctrl Pts',(-20.8704099914641,13.4604029960983,
12.));
#239240=CARTESIAN_POINT('Ctrl Pts',(-20.8457771208082,13.4568819818631,
0.));
#239241=CARTESIAN_POINT('Ctrl Pts',(-20.8457771208082,13.4568819818631,
12.));
#239242=CARTESIAN_POINT('Ctrl Pts',(-20.821234532398,13.4533137106667,0.));
#239243=CARTESIAN_POINT('Ctrl Pts',(-20.821234532398,13.4533137106667,12.));
#239244=CARTESIAN_POINT('Ctrl Pts',(-20.7967827081227,13.4496985395637,
0.));
#239245=CARTESIAN_POINT('Ctrl Pts',(-20.7967827081227,13.4496985395637,
12.));
#239246=CARTESIAN_POINT('Ctrl Pts',(-20.7724221327608,13.4460368293688,
0.));
#239247=CARTESIAN_POINT('Ctrl Pts',(-20.7724221327608,13.4460368293688,
12.));
#239248=CARTESIAN_POINT('Ctrl Pts',(-20.7481532941013,13.4423289447561,
0.));
#239249=CARTESIAN_POINT('Ctrl Pts',(-20.7481532941013,13.4423289447561,
12.));
#239250=CARTESIAN_POINT('Ctrl Pts',(-20.7239766830675,13.4385752543663,
0.));
#239251=CARTESIAN_POINT('Ctrl Pts',(-20.7239766830675,13.4385752543663,
12.));
#239252=CARTESIAN_POINT('Ctrl Pts',(-20.6998927938288,13.4347761309154,
0.));
#239253=CARTESIAN_POINT('Ctrl Pts',(-20.6998927938288,13.4347761309154,
12.));
#239254=CARTESIAN_POINT('Ctrl Pts',(-20.6759021239103,13.4309319513119,
0.));
#239255=CARTESIAN_POINT('Ctrl Pts',(-20.6759021239103,13.4309319513119,
12.));
#239256=CARTESIAN_POINT('Ctrl Pts',(-20.6520051742869,13.4270430967651,
0.));
#239257=CARTESIAN_POINT('Ctrl Pts',(-20.6520051742869,13.4270430967651,
12.));
#239258=CARTESIAN_POINT('Ctrl Pts',(-20.6282024494237,13.4231099528179,
0.));
#239259=CARTESIAN_POINT('Ctrl Pts',(-20.6282024494237,13.4231099528179,
12.));
#239260=CARTESIAN_POINT('Ctrl Pts',(-20.6044944573153,13.4191329093932,
0.));
#239261=CARTESIAN_POINT('Ctrl Pts',(-20.6044944573153,13.4191329093932,
12.));
#239262=CARTESIAN_POINT('Ctrl Pts',(-20.5808817095155,13.4151123608411,
0.));
#239263=CARTESIAN_POINT('Ctrl Pts',(-20.5808817095155,13.4151123608411,
12.));
#239264=CARTESIAN_POINT('Ctrl Pts',(-20.5573647211639,13.4110487059912,
0.));
#239265=CARTESIAN_POINT('Ctrl Pts',(-20.5573647211639,13.4110487059912,
12.));
#239266=CARTESIAN_POINT('Ctrl Pts',(-20.5339440109956,13.4069423482076,
0.));
#239267=CARTESIAN_POINT('Ctrl Pts',(-20.5339440109956,13.4069423482076,
12.));
#239268=CARTESIAN_POINT('Ctrl Pts',(-20.5106201013753,13.4027936954529,
0.));
#239269=CARTESIAN_POINT('Ctrl Pts',(-20.5106201013753,13.4027936954529,
12.));
#239270=CARTESIAN_POINT('Ctrl Pts',(-20.487393518404,13.3986031603716,0.));
#239271=CARTESIAN_POINT('Ctrl Pts',(-20.487393518404,13.3986031603716,12.));
#239272=CARTESIAN_POINT('Ctrl Pts',(-20.4642647920038,13.3943711603739,
0.));
#239273=CARTESIAN_POINT('Ctrl Pts',(-20.4642647920038,13.3943711603739,
12.));
#239274=CARTESIAN_POINT('Ctrl Pts',(-20.4412344560008,13.3900981177255,
0.));
#239275=CARTESIAN_POINT('Ctrl Pts',(-20.4412344560008,13.3900981177255,
12.));
#239276=CARTESIAN_POINT('Ctrl Pts',(-20.4183030482002,13.3857844596387,
0.));
#239277=CARTESIAN_POINT('Ctrl Pts',(-20.4183030482002,13.3857844596387,
12.));
#239278=CARTESIAN_POINT('Ctrl Pts',(-20.3954711104502,13.3814306183719,
0.));
#239279=CARTESIAN_POINT('Ctrl Pts',(-20.3954711104502,13.3814306183719,
12.));
#239280=CARTESIAN_POINT('Ctrl Pts',(-20.3727391887184,13.3770370313188,
0.));
#239281=CARTESIAN_POINT('Ctrl Pts',(-20.3727391887184,13.3770370313188,
12.));
#239282=CARTESIAN_POINT('Ctrl Pts',(-20.3501078331814,13.3726041410867,
0.));
#239283=CARTESIAN_POINT('Ctrl Pts',(-20.3501078331814,13.3726041410867,
12.));
#239284=CARTESIAN_POINT('Ctrl Pts',(-20.3275775983029,13.3681323955826,
0.));
#239285=CARTESIAN_POINT('Ctrl Pts',(-20.3275775983029,13.3681323955826,
12.));
#239286=CARTESIAN_POINT('Ctrl Pts',(-20.3051490429048,13.3636222481016,
0.));
#239287=CARTESIAN_POINT('Ctrl Pts',(-20.3051490429048,13.3636222481016,
12.));
#239288=CARTESIAN_POINT('Ctrl Pts',(-20.2828227302339,13.3590741574195,
0.));
#239289=CARTESIAN_POINT('Ctrl Pts',(-20.2828227302339,13.3590741574195,
12.));
#239290=CARTESIAN_POINT('Ctrl Pts',(-20.2605992280122,13.3544885878889,
0.));
#239291=CARTESIAN_POINT('Ctrl Pts',(-20.2605992280122,13.3544885878889,
12.));
#239292=CARTESIAN_POINT('Ctrl Pts',(-20.2384791085359,13.3498660095386,
0.));
#239293=CARTESIAN_POINT('Ctrl Pts',(-20.2384791085359,13.3498660095386,
12.));
#239294=CARTESIAN_POINT('Ctrl Pts',(-20.216462948786,13.3452068981766,0.));
#239295=CARTESIAN_POINT('Ctrl Pts',(-20.216462948786,13.3452068981766,12.));
#239296=CARTESIAN_POINT('Ctrl Pts',(-20.1945513305235,13.3405117354971,
0.));
#239297=CARTESIAN_POINT('Ctrl Pts',(-20.1945513305235,13.3405117354971,
12.));
#239298=CARTESIAN_POINT('Ctrl Pts',(-20.1727448403817,13.3357810091903,
0.));
#239299=CARTESIAN_POINT('Ctrl Pts',(-20.1727448403817,13.3357810091903,
12.));
#239300=CARTESIAN_POINT('Ctrl Pts',(-20.1510440699474,13.3310152130564,
0.));
#239301=CARTESIAN_POINT('Ctrl Pts',(-20.1510440699474,13.3310152130564,
12.));
#239302=CARTESIAN_POINT('Ctrl Pts',(-20.1294496158402,13.3262148471226,
0.));
#239303=CARTESIAN_POINT('Ctrl Pts',(-20.1294496158402,13.3262148471226,
12.));
#239304=CARTESIAN_POINT('Ctrl Pts',(-20.1079620798375,13.3213804177587,
0.));
#239305=CARTESIAN_POINT('Ctrl Pts',(-20.1079620798375,13.3213804177587,
12.));
#239306=CARTESIAN_POINT('Ctrl Pts',(-20.0865820689883,13.3165124377962,
0.));
#239307=CARTESIAN_POINT('Ctrl Pts',(-20.0865820689883,13.3165124377962,
12.));
#239308=CARTESIAN_POINT('Ctrl Pts',(-20.0653101957188,13.3116114266515,
0.));
#239309=CARTESIAN_POINT('Ctrl Pts',(-20.0653101957188,13.3116114266515,
12.));
#239310=CARTESIAN_POINT('Ctrl Pts',(-20.0441470779345,13.3066779104515,
0.));
#239311=CARTESIAN_POINT('Ctrl Pts',(-20.0441470779345,13.3066779104515,
12.));
#239312=CARTESIAN_POINT('Ctrl Pts',(-20.0230933391038,13.3017124221637,
0.));
#239313=CARTESIAN_POINT('Ctrl Pts',(-20.0230933391038,13.3017124221637,
12.));
#239314=CARTESIAN_POINT('Ctrl Pts',(-20.0021496083738,13.2967155017306,
0.));
#239315=CARTESIAN_POINT('Ctrl Pts',(-20.0021496083738,13.2967155017306,
12.));
#239316=CARTESIAN_POINT('Ctrl Pts',(-19.981316520717,13.2916876962094,0.));
#239317=CARTESIAN_POINT('Ctrl Pts',(-19.981316520717,13.2916876962094,12.));
#239318=CARTESIAN_POINT('Ctrl Pts',(-19.9605947170586,13.286629559915,0.));
#239319=CARTESIAN_POINT('Ctrl Pts',(-19.9605947170586,13.286629559915,12.));
#239320=CARTESIAN_POINT('Ctrl Pts',(-19.9399848444019,13.2815416545663,
0.));
#239321=CARTESIAN_POINT('Ctrl Pts',(-19.9399848444019,13.2815416545663,
12.));
#239322=CARTESIAN_POINT('Ctrl Pts',(-19.9194875559422,13.2764245494357,
0.));
#239323=CARTESIAN_POINT('Ctrl Pts',(-19.9194875559422,13.2764245494357,
12.));
#239324=CARTESIAN_POINT('Ctrl Pts',(-19.8991035111745,13.271278821502,0.));
#239325=CARTESIAN_POINT('Ctrl Pts',(-19.8991035111745,13.271278821502,12.));
#239326=CARTESIAN_POINT('Ctrl Pts',(-19.8788333760577,13.2661050556132,
0.));
#239327=CARTESIAN_POINT('Ctrl Pts',(-19.8788333760577,13.2661050556132,
12.));
#239328=CARTESIAN_POINT('Ctrl Pts',(-19.8586778231715,13.2609038446529,
0.));
#239329=CARTESIAN_POINT('Ctrl Pts',(-19.8586778231715,13.2609038446529,
12.));
#239330=CARTESIAN_POINT('Ctrl Pts',(-19.8386375318634,13.2556757897086,
0.));
#239331=CARTESIAN_POINT('Ctrl Pts',(-19.8386375318634,13.2556757897086,
12.));
#239332=CARTESIAN_POINT('Ctrl Pts',(-19.8187131883917,13.2504215002457,
0.));
#239333=CARTESIAN_POINT('Ctrl Pts',(-19.8187131883917,13.2504215002457,
12.));
#239334=CARTESIAN_POINT('Ctrl Pts',(-19.7989054860495,13.2451415942805,
0.));
#239335=CARTESIAN_POINT('Ctrl Pts',(-19.7989054860495,13.2451415942805,
12.));
#239336=CARTESIAN_POINT('Ctrl Pts',(-19.7792151253289,13.2398366985675,
0.));
#239337=CARTESIAN_POINT('Ctrl Pts',(-19.7792151253289,13.2398366985675,
12.));
#239338=CARTESIAN_POINT('Ctrl Pts',(-19.7596428141168,13.2345074487963,
0.));
#239339=CARTESIAN_POINT('Ctrl Pts',(-19.7596428141168,13.2345074487963,
12.));
#239340=CARTESIAN_POINT('Ctrl Pts',(-19.7401892678697,13.2291544897899,
0.));
#239341=CARTESIAN_POINT('Ctrl Pts',(-19.7401892678697,13.2291544897899,
12.));
#239342=CARTESIAN_POINT('Ctrl Pts',(-19.7208552097868,13.2237784757065,
0.));
#239343=CARTESIAN_POINT('Ctrl Pts',(-19.7208552097868,13.2237784757065,
12.));
#239344=CARTESIAN_POINT('Ctrl Pts',(-19.7016413709685,13.2183800702436,
0.));
#239345=CARTESIAN_POINT('Ctrl Pts',(-19.7016413709685,13.2183800702436,
12.));
#239346=CARTESIAN_POINT('Ctrl Pts',(-19.6825484905823,13.2129599468485,
0.));
#239347=CARTESIAN_POINT('Ctrl Pts',(-19.6825484905823,13.2129599468485,
12.));
#239348=CARTESIAN_POINT('Ctrl Pts',(-19.6635773160936,13.2075187889529,
0.));
#239349=CARTESIAN_POINT('Ctrl Pts',(-19.6635773160936,13.2075187889529,
12.));
#239350=CARTESIAN_POINT('Ctrl Pts',(-19.6447286034772,13.2020572902065,
0.));
#239351=CARTESIAN_POINT('Ctrl Pts',(-19.6447286034772,13.2020572902065,
12.));
#239352=CARTESIAN_POINT('Ctrl Pts',(-19.6260031174244,13.1965761547151,
0.));
#239353=CARTESIAN_POINT('Ctrl Pts',(-19.6260031174244,13.1965761547151,
12.));
#239354=CARTESIAN_POINT('Ctrl Pts',(-19.6074016315414,13.1910760972814,
0.));
#239355=CARTESIAN_POINT('Ctrl Pts',(-19.6074016315414,13.1910760972814,
12.));
#239356=CARTESIAN_POINT('Ctrl Pts',(-19.5889249285338,13.1855578436471,
0.));
#239357=CARTESIAN_POINT('Ctrl Pts',(-19.5889249285338,13.1855578436471,
12.));
#239358=CARTESIAN_POINT('Ctrl Pts',(-19.5705738004667,13.1800221307673,
0.));
#239359=CARTESIAN_POINT('Ctrl Pts',(-19.5705738004667,13.1800221307673,
12.));
#239360=CARTESIAN_POINT('Ctrl Pts',(-19.5523490490244,13.1744697070911,
0.));
#239361=CARTESIAN_POINT('Ctrl Pts',(-19.5523490490244,13.1744697070911,
12.));
#239362=CARTESIAN_POINT('Ctrl Pts',(-19.5342514857562,13.168901332843,0.));
#239363=CARTESIAN_POINT('Ctrl Pts',(-19.5342514857562,13.168901332843,12.));
#239364=CARTESIAN_POINT('Ctrl Pts',(-19.5162819323213,13.1633177803101,
0.));
#239365=CARTESIAN_POINT('Ctrl Pts',(-19.5162819323213,13.1633177803101,
12.));
#239366=CARTESIAN_POINT('Ctrl Pts',(-19.4984412207082,13.1577198341245,
0.));
#239367=CARTESIAN_POINT('Ctrl Pts',(-19.4984412207082,13.1577198341245,
12.));
#239368=CARTESIAN_POINT('Ctrl Pts',(-19.4807301935268,13.1521082915853,
0.));
#239369=CARTESIAN_POINT('Ctrl Pts',(-19.4807301935268,13.1521082915853,
12.));
#239370=CARTESIAN_POINT('Ctrl Pts',(-19.4631497043258,13.1464839629971,
0.));
#239371=CARTESIAN_POINT('Ctrl Pts',(-19.4631497043258,13.1464839629971,
12.));
#239372=CARTESIAN_POINT('Ctrl Pts',(-19.4457006178876,13.1408476720061,
0.));
#239373=CARTESIAN_POINT('Ctrl Pts',(-19.4457006178876,13.1408476720061,
12.));
#239374=CARTESIAN_POINT('Ctrl Pts',(-19.4283838105262,13.1352002559438,
0.));
#239375=CARTESIAN_POINT('Ctrl Pts',(-19.4283838105262,13.1352002559438,
12.));
#239376=CARTESIAN_POINT('Ctrl Pts',(-19.4112001703557,13.1295425661634,
0.));
#239377=CARTESIAN_POINT('Ctrl Pts',(-19.4112001703557,13.1295425661634,
12.));
#239378=CARTESIAN_POINT('Ctrl Pts',(-19.3941505976263,13.1238754684177,
0.));
#239379=CARTESIAN_POINT('Ctrl Pts',(-19.3941505976263,13.1238754684177,
12.));
#239380=CARTESIAN_POINT('Ctrl Pts',(-19.3772360051091,13.118199843271,0.));
#239381=CARTESIAN_POINT('Ctrl Pts',(-19.3772360051091,13.118199843271,12.));
#239382=CARTESIAN_POINT('Ctrl Pts',(-19.3604573184515,13.1125165865022,
0.));
#239383=CARTESIAN_POINT('Ctrl Pts',(-19.3604573184515,13.1125165865022,
12.));
#239384=CARTESIAN_POINT('Ctrl Pts',(-19.3438154765395,13.1068266095186,
0.));
#239385=CARTESIAN_POINT('Ctrl Pts',(-19.3438154765395,13.1068266095186,
12.));
#239386=CARTESIAN_POINT('Ctrl Pts',(-19.3273114318269,13.1011308397591,
0.));
#239387=CARTESIAN_POINT('Ctrl Pts',(-19.3273114318269,13.1011308397591,
12.));
#239388=CARTESIAN_POINT('Ctrl Pts',(-19.310946150736,13.0954302211479,0.));
#239389=CARTESIAN_POINT('Ctrl Pts',(-19.310946150736,13.0954302211479,12.));
#239390=CARTESIAN_POINT('Ctrl Pts',(-19.2947206141247,13.0897257145968,
0.));
#239391=CARTESIAN_POINT('Ctrl Pts',(-19.2947206141247,13.0897257145968,
12.));
#239392=CARTESIAN_POINT('Ctrl Pts',(-19.2786358177198,13.0840182984949,
0.));
#239393=CARTESIAN_POINT('Ctrl Pts',(-19.2786358177198,13.0840182984949,
12.));
#239394=CARTESIAN_POINT('Ctrl Pts',(-19.2626927725596,13.0783089692118,
0.));
#239395=CARTESIAN_POINT('Ctrl Pts',(-19.2626927725596,13.0783089692118,
12.));
#239396=CARTESIAN_POINT('Ctrl Pts',(-19.2468925053989,13.0725987415859,
0.));
#239397=CARTESIAN_POINT('Ctrl Pts',(-19.2468925053989,13.0725987415859,
12.));
#239398=CARTESIAN_POINT('Ctrl Pts',(-19.2312360592033,13.0668886494795,
0.));
#239399=CARTESIAN_POINT('Ctrl Pts',(-19.2312360592033,13.0668886494795,
12.));
#239400=CARTESIAN_POINT('Ctrl Pts',(-19.2157244937142,13.0611797463915,
0.));
#239401=CARTESIAN_POINT('Ctrl Pts',(-19.2157244937142,13.0611797463915,
12.));
#239402=CARTESIAN_POINT('Ctrl Pts',(-19.2003588859772,13.0554731060538,
0.));
#239403=CARTESIAN_POINT('Ctrl Pts',(-19.2003588859772,13.0554731060538,
12.));
#239404=CARTESIAN_POINT('Ctrl Pts',(-19.1851403308825,13.0497698230441,
0.));
#239405=CARTESIAN_POINT('Ctrl Pts',(-19.1851403308825,13.0497698230441,
12.));
#239406=CARTESIAN_POINT('Ctrl Pts',(-19.1700699416622,13.0440710133772,
0.));
#239407=CARTESIAN_POINT('Ctrl Pts',(-19.1700699416622,13.0440710133772,
12.));
#239408=CARTESIAN_POINT('Ctrl Pts',(-19.155148850523,13.0383778152068,0.));
#239409=CARTESIAN_POINT('Ctrl Pts',(-19.155148850523,13.0383778152068,12.));
#239410=CARTESIAN_POINT('Ctrl Pts',(-19.1403782093386,13.0326913895838,
0.));
#239411=CARTESIAN_POINT('Ctrl Pts',(-19.1403782093386,13.0326913895838,
12.));
#239412=CARTESIAN_POINT('Ctrl Pts',(-19.1257591903099,13.0270129211976,
0.));
#239413=CARTESIAN_POINT('Ctrl Pts',(-19.1257591903099,13.0270129211976,
12.));
#239414=CARTESIAN_POINT('Ctrl Pts',(-19.111292986631,13.0213436191328,0.));
#239415=CARTESIAN_POINT('Ctrl Pts',(-19.111292986631,13.0213436191328,12.));
#239416=CARTESIAN_POINT('Ctrl Pts',(-19.0969808131228,13.0156847176096,
0.));
#239417=CARTESIAN_POINT('Ctrl Pts',(-19.0969808131228,13.0156847176096,
12.));
#239418=CARTESIAN_POINT('Ctrl Pts',(-19.0828239070484,13.0100374768788,
0.));
#239419=CARTESIAN_POINT('Ctrl Pts',(-19.0828239070484,13.0100374768788,
12.));
#239420=CARTESIAN_POINT('Ctrl Pts',(-19.0688235289437,13.0044031841382,
0.));
#239421=CARTESIAN_POINT('Ctrl Pts',(-19.0688235289437,13.0044031841382,
12.));
#239422=CARTESIAN_POINT('Ctrl Pts',(-19.0549809634354,12.9987831544502,
0.));
#239423=CARTESIAN_POINT('Ctrl Pts',(-19.0549809634354,12.9987831544502,
12.));
#239424=CARTESIAN_POINT('Ctrl Pts',(-19.0412975200398,12.9931787316514,
0.));
#239425=CARTESIAN_POINT('Ctrl Pts',(-19.0412975200398,12.9931787316514,
12.));
#239426=CARTESIAN_POINT('Ctrl Pts',(-19.0277745339909,12.9875912893003,
0.));
#239427=CARTESIAN_POINT('Ctrl Pts',(-19.0277745339909,12.9875912893003,
12.));
#239428=CARTESIAN_POINT('Ctrl Pts',(-19.014413367335,12.9820222318716,0.));
#239429=CARTESIAN_POINT('Ctrl Pts',(-19.014413367335,12.9820222318716,12.));
#239430=CARTESIAN_POINT('Ctrl Pts',(-19.0012154099792,12.9764729959206,
0.));
#239431=CARTESIAN_POINT('Ctrl Pts',(-19.0012154099792,12.9764729959206,
12.));
#239432=CARTESIAN_POINT('Ctrl Pts',(-18.9881820807585,12.9709450512747,
0.));
#239433=CARTESIAN_POINT('Ctrl Pts',(-18.9881820807585,12.9709450512747,
12.));
#239434=CARTESIAN_POINT('Ctrl Pts',(-18.9753148284473,12.9654399021868,
0.));
#239435=CARTESIAN_POINT('Ctrl Pts',(-18.9753148284473,12.9654399021868,
12.));
#239436=CARTESIAN_POINT('Ctrl Pts',(-18.9626151329226,12.9599590886317,
0.));
#239437=CARTESIAN_POINT('Ctrl Pts',(-18.9626151329226,12.9599590886317,
12.));
#239438=CARTESIAN_POINT('Ctrl Pts',(-18.9500845064714,12.9545041877377,
0.));
#239439=CARTESIAN_POINT('Ctrl Pts',(-18.9500845064714,12.9545041877377,
12.));
#239440=CARTESIAN_POINT('Ctrl Pts',(-18.9377244950435,12.9490768151821,
0.));
#239441=CARTESIAN_POINT('Ctrl Pts',(-18.9377244950435,12.9490768151821,
12.));
#239442=CARTESIAN_POINT('Ctrl Pts',(-18.9255366795196,12.9436786266106,
0.));
#239443=CARTESIAN_POINT('Ctrl Pts',(-18.9255366795196,12.9436786266106,
12.));
#239444=CARTESIAN_POINT('Ctrl Pts',(-18.9135226769466,12.9383113190375,
0.));
#239445=CARTESIAN_POINT('Ctrl Pts',(-18.9135226769466,12.9383113190375,
12.));
#239446=CARTESIAN_POINT('Ctrl Pts',(-18.9016841423402,12.9329766328184,
0.));
#239447=CARTESIAN_POINT('Ctrl Pts',(-18.9016841423402,12.9329766328184,
12.));
#239448=CARTESIAN_POINT('Ctrl Pts',(-18.8900227704888,12.9276763536372,
0.));
#239449=CARTESIAN_POINT('Ctrl Pts',(-18.8900227704888,12.9276763536372,
12.));
#239450=CARTESIAN_POINT('Ctrl Pts',(-18.8785402977528,12.9224123144982,
0.));
#239451=CARTESIAN_POINT('Ctrl Pts',(-18.8785402977528,12.9224123144982,
12.));
#239452=CARTESIAN_POINT('Ctrl Pts',(-18.8672385038328,12.9171863977047,
0.));
#239453=CARTESIAN_POINT('Ctrl Pts',(-18.8672385038328,12.9171863977047,
12.));
#239454=CARTESIAN_POINT('Ctrl Pts',(-18.8561192136201,12.9120005369066,
0.));
#239455=CARTESIAN_POINT('Ctrl Pts',(-18.8561192136201,12.9120005369066,
12.));
#239456=CARTESIAN_POINT('Ctrl Pts',(-18.8451842990986,12.9068567191856,
0.));
#239457=CARTESIAN_POINT('Ctrl Pts',(-18.8451842990986,12.9068567191856,
12.));
#239458=CARTESIAN_POINT('Ctrl Pts',(-18.834435681259,12.9017569871738,0.));
#239459=CARTESIAN_POINT('Ctrl Pts',(-18.834435681259,12.9017569871738,12.));
#239460=CARTESIAN_POINT('Ctrl Pts',(-18.8238753319124,12.8967034410752,
0.));
#239461=CARTESIAN_POINT('Ctrl Pts',(-18.8238753319124,12.8967034410752,
12.));
#239462=CARTESIAN_POINT('Ctrl Pts',(-18.8135052757815,12.8916982409931,
0.));
#239463=CARTESIAN_POINT('Ctrl Pts',(-18.8135052757815,12.8916982409931,
12.));
#239464=CARTESIAN_POINT('Ctrl Pts',(-18.8033275941939,12.8867436109543,
0.));
#239465=CARTESIAN_POINT('Ctrl Pts',(-18.8033275941939,12.8867436109543,
12.));
#239466=CARTESIAN_POINT('Ctrl Pts',(-18.7933444285867,12.8818418427474,
0.));
#239467=CARTESIAN_POINT('Ctrl Pts',(-18.7933444285867,12.8818418427474,
12.));
#239468=CARTESIAN_POINT('Ctrl Pts',(-18.7835579840481,12.8769952998097,
0.));
#239469=CARTESIAN_POINT('Ctrl Pts',(-18.7835579840481,12.8769952998097,
12.));
#239470=CARTESIAN_POINT('Ctrl Pts',(-18.7739705329029,12.8722064211814,
0.));
#239471=CARTESIAN_POINT('Ctrl Pts',(-18.7739705329029,12.8722064211814,
12.));
#239472=CARTESIAN_POINT('Ctrl Pts',(-18.7645844169568,12.8674777239656,
0.));
#239473=CARTESIAN_POINT('Ctrl Pts',(-18.7645844169568,12.8674777239656,
12.));
#239474=CARTESIAN_POINT('Ctrl Pts',(-18.7554020493888,12.8628118054172,
0.));
#239475=CARTESIAN_POINT('Ctrl Pts',(-18.7554020493888,12.8628118054172,
12.));
#239476=CARTESIAN_POINT('Ctrl Pts',(-18.7464259171248,12.8582113455644,
0.));
#239477=CARTESIAN_POINT('Ctrl Pts',(-18.7464259171248,12.8582113455644,
12.));
#239478=CARTESIAN_POINT('Ctrl Pts',(-18.7376585820851,12.8536791086315,
0.));
#239479=CARTESIAN_POINT('Ctrl Pts',(-18.7376585820851,12.8536791086315,
12.));
#239480=CARTESIAN_POINT('Ctrl Pts',(-18.7291026886552,12.849217951159,0.));
#239481=CARTESIAN_POINT('Ctrl Pts',(-18.7291026886552,12.849217951159,12.));
#239482=CARTESIAN_POINT('Ctrl Pts',(-18.7207609737701,12.8448308329494,
0.));
#239483=CARTESIAN_POINT('Ctrl Pts',(-18.7207609737701,12.8448308329494,
12.));
#239484=CARTESIAN_POINT('Ctrl Pts',(-18.7126362754446,12.8405208263432,
0.));
#239485=CARTESIAN_POINT('Ctrl Pts',(-18.7126362754446,12.8405208263432,
12.));
#239486=CARTESIAN_POINT('Ctrl Pts',(-18.7047315436296,12.8362911280362,
0.));
#239487=CARTESIAN_POINT('Ctrl Pts',(-18.7047315436296,12.8362911280362,
12.));
#239488=CARTESIAN_POINT('Ctrl Pts',(-18.6970498410173,12.832145059979,0.));
#239489=CARTESIAN_POINT('Ctrl Pts',(-18.6970498410173,12.832145059979,12.));
#239490=CARTESIAN_POINT('Ctrl Pts',(-18.6895943376172,12.8280860635231,
0.));
#239491=CARTESIAN_POINT('Ctrl Pts',(-18.6895943376172,12.8280860635231,
12.));
#239492=CARTESIAN_POINT('Ctrl Pts',(-18.6823683094139,12.8241176980016,
0.));
#239493=CARTESIAN_POINT('Ctrl Pts',(-18.6823683094139,12.8241176980016,
12.));
#239494=CARTESIAN_POINT('Ctrl Pts',(-18.6753751301091,12.8202436318473,
0.));
#239495=CARTESIAN_POINT('Ctrl Pts',(-18.6753751301091,12.8202436318473,
12.));
#239496=CARTESIAN_POINT('Ctrl Pts',(-18.6686182952798,12.8164676687361,
0.));
#239497=CARTESIAN_POINT('Ctrl Pts',(-18.6686182952798,12.8164676687361,
12.));
#239498=CARTESIAN_POINT('Ctrl Pts',(-18.6621014624746,12.8127937909632,
0.));
#239499=CARTESIAN_POINT('Ctrl Pts',(-18.6621014624746,12.8127937909632,
12.));
#239500=CARTESIAN_POINT('Ctrl Pts',(-18.6558284825772,12.8092261933858,
0.));
#239501=CARTESIAN_POINT('Ctrl Pts',(-18.6558284825772,12.8092261933858,
12.));
#239502=CARTESIAN_POINT('Ctrl Pts',(-18.6498034438986,12.805769331162,0.));
#239503=CARTESIAN_POINT('Ctrl Pts',(-18.6498034438986,12.805769331162,12.));
#239504=CARTESIAN_POINT('Ctrl Pts',(-18.6440306327457,12.8024278770153,
0.));
#239505=CARTESIAN_POINT('Ctrl Pts',(-18.6440306327457,12.8024278770153,
12.));
#239506=CARTESIAN_POINT('Ctrl Pts',(-18.63851447924,12.7992066625264,0.));
#239507=CARTESIAN_POINT('Ctrl Pts',(-18.63851447924,12.7992066625264,12.));
#239508=CARTESIAN_POINT('Ctrl Pts',(-18.6332595057005,12.7961106222251,
0.));
#239509=CARTESIAN_POINT('Ctrl Pts',(-18.6332595057005,12.7961106222251,
12.));
#239510=CARTESIAN_POINT('Ctrl Pts',(-18.6282702819371,12.7931447451556,
0.));
#239511=CARTESIAN_POINT('Ctrl Pts',(-18.6282702819371,12.7931447451556,
12.));
#239512=CARTESIAN_POINT('Ctrl Pts',(-18.6235516265575,12.7903142925234,
0.));
#239513=CARTESIAN_POINT('Ctrl Pts',(-18.6235516265575,12.7903142925234,
12.));
#239514=CARTESIAN_POINT('Ctrl Pts',(-18.6191087624752,12.7876249657834,
0.));
#239515=CARTESIAN_POINT('Ctrl Pts',(-18.6191087624752,12.7876249657834,
12.));
#239516=CARTESIAN_POINT('Ctrl Pts',(-18.6149475565189,12.78508316579,0.));
#239517=CARTESIAN_POINT('Ctrl Pts',(-18.6149475565189,12.78508316579,12.));
#239518=CARTESIAN_POINT('Ctrl Pts',(-18.611074482622,12.7826959526924,0.));
#239519=CARTESIAN_POINT('Ctrl Pts',(-18.611074482622,12.7826959526924,12.));
#239520=CARTESIAN_POINT('Ctrl Pts',(-18.6074961535723,12.7804705387658,
0.));
#239521=CARTESIAN_POINT('Ctrl Pts',(-18.6074961535723,12.7804705387658,
12.));
#239522=CARTESIAN_POINT('Ctrl Pts',(-18.6042190183703,12.7784139605067,
0.));
#239523=CARTESIAN_POINT('Ctrl Pts',(-18.6042190183703,12.7784139605067,
12.));
#239524=CARTESIAN_POINT('Ctrl Pts',(-18.6012488486708,12.7765325225082,
0.));
#239525=CARTESIAN_POINT('Ctrl Pts',(-18.6012488486708,12.7765325225082,
12.));
#239526=CARTESIAN_POINT('Ctrl Pts',(-18.5985917525949,12.7748328937639,
0.));
#239527=CARTESIAN_POINT('Ctrl Pts',(-18.5985917525949,12.7748328937639,
12.));
#239528=CARTESIAN_POINT('Ctrl Pts',(-18.5962551167772,12.7733231262107,
0.));
#239529=CARTESIAN_POINT('Ctrl Pts',(-18.5962551167772,12.7733231262107,
12.));
#239530=CARTESIAN_POINT('Ctrl Pts',(-18.5942490615409,12.7720142287169,
0.));
#239531=CARTESIAN_POINT('Ctrl Pts',(-18.5942490615409,12.7720142287169,
12.));
#239532=CARTESIAN_POINT('Ctrl Pts',(-18.5925859134582,12.7709195951153,
0.));
#239533=CARTESIAN_POINT('Ctrl Pts',(-18.5925859134582,12.7709195951153,
12.));
#239534=CARTESIAN_POINT('Ctrl Pts',(-18.5912775137806,12.7700520897174,
0.));
#239535=CARTESIAN_POINT('Ctrl Pts',(-18.5912775137806,12.7700520897174,
12.));
#239536=CARTESIAN_POINT('Ctrl Pts',(-18.590332877722,12.7694215127923,0.));
#239537=CARTESIAN_POINT('Ctrl Pts',(-18.590332877722,12.7694215127923,12.));
#239538=CARTESIAN_POINT('Ctrl Pts',(-18.589871621842,12.7691103481996,0.));
#239539=CARTESIAN_POINT('Ctrl Pts',(-18.589871621842,12.7691103481996,12.));
#239540=CARTESIAN_POINT('Ctrl Pts',(-18.5896919669158,12.7689864266924,
0.));
#239541=CARTESIAN_POINT('Ctrl Pts',(-18.5896919669158,12.7689864266924,
12.));
#239542=CARTESIAN_POINT('Ctrl Pts',(-18.5896460962961,12.7689524524484,
0.));
#239543=CARTESIAN_POINT('Ctrl Pts',(-18.5896460962961,12.7689524524484,
12.));
#239544=CARTESIAN_POINT('Ctrl Pts',(-18.5896416359912,12.7689476255363,
0.));
#239545=CARTESIAN_POINT('Ctrl Pts',(-18.5896416359912,12.7689476255363,
12.));
#239546=CARTESIAN_POINT('',(-22.1787195904339,13.5685075571671,0.));
#239547=CARTESIAN_POINT('Ctrl Pts',(-22.1787195904339,13.5685075571671,
0.));
#239548=CARTESIAN_POINT('Ctrl Pts',(-22.1730081264583,13.5683460612913,
0.));
#239549=CARTESIAN_POINT('Ctrl Pts',(-22.1615922804939,13.5680170531724,
0.));
#239550=CARTESIAN_POINT('Ctrl Pts',(-22.1444897575076,13.5675054918922,
0.));
#239551=CARTESIAN_POINT('Ctrl Pts',(-22.1217288871823,13.5667873105179,
0.));
#239552=CARTESIAN_POINT('Ctrl Pts',(-22.0933486464442,13.5658294169106,
0.));
#239553=CARTESIAN_POINT('Ctrl Pts',(-22.0650393089492,13.5648113688894,
0.));
#239554=CARTESIAN_POINT('Ctrl Pts',(-22.0368009736227,13.5637332022393,
0.));
#239555=CARTESIAN_POINT('Ctrl Pts',(-22.0086337943431,13.5625949868313,
0.));
#239556=CARTESIAN_POINT('Ctrl Pts',(-21.9805379899192,13.5613968357589,
0.));
#239557=CARTESIAN_POINT('Ctrl Pts',(-21.9525138592862,13.5601389185315,
0.));
#239558=CARTESIAN_POINT('Ctrl Pts',(-21.9245617765827,13.5588214586672,
0.));
#239559=CARTESIAN_POINT('Ctrl Pts',(-21.8966821688876,13.5574447178484,
0.));
#239560=CARTESIAN_POINT('Ctrl Pts',(-21.8688754989401,13.5560089839426,
0.));
#239561=CARTESIAN_POINT('Ctrl Pts',(-21.841142245609,13.5545145573048,0.));
#239562=CARTESIAN_POINT('Ctrl Pts',(-21.8134828857963,13.5529617381569,
0.));
#239563=CARTESIAN_POINT('Ctrl Pts',(-21.7858978745848,13.5513508127232,
0.));
#239564=CARTESIAN_POINT('Ctrl Pts',(-21.7583876294532,13.5496820422186,
0.));
#239565=CARTESIAN_POINT('Ctrl Pts',(-21.730952541226,13.5479556704457,0.));
#239566=CARTESIAN_POINT('Ctrl Pts',(-21.7035929822939,13.546171929503,0.));
#239567=CARTESIAN_POINT('Ctrl Pts',(-21.676309315769,13.5443310461516,0.));
#239568=CARTESIAN_POINT('Ctrl Pts',(-21.6491019044647,13.5424332480698,
0.));
#239569=CARTESIAN_POINT('Ctrl Pts',(-21.6219711193951,13.5404787697798,
0.));
#239570=CARTESIAN_POINT('Ctrl Pts',(-21.5949173499022,13.5384678597206,
0.));
#239571=CARTESIAN_POINT('Ctrl Pts',(-21.5679410019011,13.5364007790292,
0.));
#239572=CARTESIAN_POINT('Ctrl Pts',(-21.5410424932511,13.5342777983225,
0.));
#239573=CARTESIAN_POINT('Ctrl Pts',(-21.5142222501671,13.5320991952145,
0.));
#239574=CARTESIAN_POINT('Ctrl Pts',(-21.487480703047,13.5298652514357,0.));
#239575=CARTESIAN_POINT('Ctrl Pts',(-21.4608182828695,13.5275762503553,
0.));
#239576=CARTESIAN_POINT('Ctrl Pts',(-21.4342354165254,13.5252324737795,
0.));
#239577=CARTESIAN_POINT('Ctrl Pts',(-21.4077325259318,13.5228342013508,
0.));
#239578=CARTESIAN_POINT('Ctrl Pts',(-21.3813100304967,13.5203817122496,
0.));
#239579=CARTESIAN_POINT('Ctrl Pts',(-21.3549683486219,13.5178752862461,
0.));
#239580=CARTESIAN_POINT('Ctrl Pts',(-21.328707899634,13.5153152050554,0.));
#239581=CARTESIAN_POINT('Ctrl Pts',(-21.3025291054236,13.5127017534972,
0.));
#239582=CARTESIAN_POINT('Ctrl Pts',(-21.2764323924442,13.5100352209207,
0.));
#239583=CARTESIAN_POINT('Ctrl Pts',(-21.2504181927429,13.5073159019454,
0.));
#239584=CARTESIAN_POINT('Ctrl Pts',(-21.224486942933,13.5045440957404,0.));
#239585=CARTESIAN_POINT('Ctrl Pts',(-21.1986390835825,13.5017201056088,
0.));
#239586=CARTESIAN_POINT('Ctrl Pts',(-21.1728750584173,13.4988442384491,
0.));
#239587=CARTESIAN_POINT('Ctrl Pts',(-21.1471953136209,13.4959168042934,
0.));
#239588=CARTESIAN_POINT('Ctrl Pts',(-21.1216002970209,13.4929381157778,
0.));
#239589=CARTESIAN_POINT('Ctrl Pts',(-21.0960904575048,13.4899084877718,
0.));
#239590=CARTESIAN_POINT('Ctrl Pts',(-21.0706662455202,13.4868282377191,
0.));
#239591=CARTESIAN_POINT('Ctrl Pts',(-21.0453281134247,13.4836976858912,
0.));
#239592=CARTESIAN_POINT('Ctrl Pts',(-21.0200765158885,13.4805171556822,
0.));
#239593=CARTESIAN_POINT('Ctrl Pts',(-20.9949119102592,13.4772869738879,
0.));
#239594=CARTESIAN_POINT('Ctrl Pts',(-20.9698347569476,13.4740074710087,
0.));
#239595=CARTESIAN_POINT('Ctrl Pts',(-20.9448455197557,13.4706789815166,
0.));
#239596=CARTESIAN_POINT('Ctrl Pts',(-20.9199446657584,13.4673018437718,
0.));
#239597=CARTESIAN_POINT('Ctrl Pts',(-20.8951326652158,13.4638763999725,
0.));
#239598=CARTESIAN_POINT('Ctrl Pts',(-20.8704099914641,13.4604029960983,
0.));
#239599=CARTESIAN_POINT('Ctrl Pts',(-20.8457771208082,13.4568819818631,
0.));
#239600=CARTESIAN_POINT('Ctrl Pts',(-20.821234532398,13.4533137106667,0.));
#239601=CARTESIAN_POINT('Ctrl Pts',(-20.7967827081227,13.4496985395637,
0.));
#239602=CARTESIAN_POINT('Ctrl Pts',(-20.7724221327608,13.4460368293688,
0.));
#239603=CARTESIAN_POINT('Ctrl Pts',(-20.7481532941013,13.4423289447561,
0.));
#239604=CARTESIAN_POINT('Ctrl Pts',(-20.7239766830675,13.4385752543663,
0.));
#239605=CARTESIAN_POINT('Ctrl Pts',(-20.6998927938288,13.4347761309154,
0.));
#239606=CARTESIAN_POINT('Ctrl Pts',(-20.6759021239103,13.4309319513119,
0.));
#239607=CARTESIAN_POINT('Ctrl Pts',(-20.6520051742869,13.4270430967651,
0.));
#239608=CARTESIAN_POINT('Ctrl Pts',(-20.6282024494237,13.4231099528179,
0.));
#239609=CARTESIAN_POINT('Ctrl Pts',(-20.6044944573153,13.4191329093932,
0.));
#239610=CARTESIAN_POINT('Ctrl Pts',(-20.5808817095155,13.4151123608411,
0.));
#239611=CARTESIAN_POINT('Ctrl Pts',(-20.5573647211639,13.4110487059912,
0.));
#239612=CARTESIAN_POINT('Ctrl Pts',(-20.5339440109956,13.4069423482076,
0.));
#239613=CARTESIAN_POINT('Ctrl Pts',(-20.5106201013753,13.4027936954529,
0.));
#239614=CARTESIAN_POINT('Ctrl Pts',(-20.487393518404,13.3986031603716,0.));
#239615=CARTESIAN_POINT('Ctrl Pts',(-20.4642647920038,13.3943711603739,
0.));
#239616=CARTESIAN_POINT('Ctrl Pts',(-20.4412344560008,13.3900981177255,
0.));
#239617=CARTESIAN_POINT('Ctrl Pts',(-20.4183030482002,13.3857844596387,
0.));
#239618=CARTESIAN_POINT('Ctrl Pts',(-20.3954711104502,13.3814306183719,
0.));
#239619=CARTESIAN_POINT('Ctrl Pts',(-20.3727391887184,13.3770370313188,
0.));
#239620=CARTESIAN_POINT('Ctrl Pts',(-20.3501078331814,13.3726041410867,
0.));
#239621=CARTESIAN_POINT('Ctrl Pts',(-20.3275775983029,13.3681323955826,
0.));
#239622=CARTESIAN_POINT('Ctrl Pts',(-20.3051490429048,13.3636222481016,
0.));
#239623=CARTESIAN_POINT('Ctrl Pts',(-20.2828227302339,13.3590741574195,
0.));
#239624=CARTESIAN_POINT('Ctrl Pts',(-20.2605992280122,13.3544885878889,
0.));
#239625=CARTESIAN_POINT('Ctrl Pts',(-20.2384791085359,13.3498660095386,
0.));
#239626=CARTESIAN_POINT('Ctrl Pts',(-20.216462948786,13.3452068981766,0.));
#239627=CARTESIAN_POINT('Ctrl Pts',(-20.1945513305235,13.3405117354971,
0.));
#239628=CARTESIAN_POINT('Ctrl Pts',(-20.1727448403817,13.3357810091903,
0.));
#239629=CARTESIAN_POINT('Ctrl Pts',(-20.1510440699474,13.3310152130564,
0.));
#239630=CARTESIAN_POINT('Ctrl Pts',(-20.1294496158402,13.3262148471226,
0.));
#239631=CARTESIAN_POINT('Ctrl Pts',(-20.1079620798375,13.3213804177587,
0.));
#239632=CARTESIAN_POINT('Ctrl Pts',(-20.0865820689883,13.3165124377962,
0.));
#239633=CARTESIAN_POINT('Ctrl Pts',(-20.0653101957188,13.3116114266515,
0.));
#239634=CARTESIAN_POINT('Ctrl Pts',(-20.0441470779345,13.3066779104515,
0.));
#239635=CARTESIAN_POINT('Ctrl Pts',(-20.0230933391038,13.3017124221637,
0.));
#239636=CARTESIAN_POINT('Ctrl Pts',(-20.0021496083738,13.2967155017306,
0.));
#239637=CARTESIAN_POINT('Ctrl Pts',(-19.981316520717,13.2916876962094,0.));
#239638=CARTESIAN_POINT('Ctrl Pts',(-19.9605947170586,13.286629559915,0.));
#239639=CARTESIAN_POINT('Ctrl Pts',(-19.9399848444019,13.2815416545663,
0.));
#239640=CARTESIAN_POINT('Ctrl Pts',(-19.9194875559422,13.2764245494357,
0.));
#239641=CARTESIAN_POINT('Ctrl Pts',(-19.8991035111745,13.271278821502,0.));
#239642=CARTESIAN_POINT('Ctrl Pts',(-19.8788333760577,13.2661050556132,
0.));
#239643=CARTESIAN_POINT('Ctrl Pts',(-19.8586778231715,13.2609038446529,
0.));
#239644=CARTESIAN_POINT('Ctrl Pts',(-19.8386375318634,13.2556757897086,
0.));
#239645=CARTESIAN_POINT('Ctrl Pts',(-19.8187131883917,13.2504215002457,
0.));
#239646=CARTESIAN_POINT('Ctrl Pts',(-19.7989054860495,13.2451415942805,
0.));
#239647=CARTESIAN_POINT('Ctrl Pts',(-19.7792151253289,13.2398366985675,
0.));
#239648=CARTESIAN_POINT('Ctrl Pts',(-19.7596428141168,13.2345074487963,
0.));
#239649=CARTESIAN_POINT('Ctrl Pts',(-19.7401892678697,13.2291544897899,
0.));
#239650=CARTESIAN_POINT('Ctrl Pts',(-19.7208552097868,13.2237784757065,
0.));
#239651=CARTESIAN_POINT('Ctrl Pts',(-19.7016413709685,13.2183800702436,
0.));
#239652=CARTESIAN_POINT('Ctrl Pts',(-19.6825484905823,13.2129599468485,
0.));
#239653=CARTESIAN_POINT('Ctrl Pts',(-19.6635773160936,13.2075187889529,
0.));
#239654=CARTESIAN_POINT('Ctrl Pts',(-19.6447286034772,13.2020572902065,
0.));
#239655=CARTESIAN_POINT('Ctrl Pts',(-19.6260031174244,13.1965761547151,
0.));
#239656=CARTESIAN_POINT('Ctrl Pts',(-19.6074016315414,13.1910760972814,
0.));
#239657=CARTESIAN_POINT('Ctrl Pts',(-19.5889249285338,13.1855578436471,
0.));
#239658=CARTESIAN_POINT('Ctrl Pts',(-19.5705738004667,13.1800221307673,
0.));
#239659=CARTESIAN_POINT('Ctrl Pts',(-19.5523490490244,13.1744697070911,
0.));
#239660=CARTESIAN_POINT('Ctrl Pts',(-19.5342514857562,13.168901332843,0.));
#239661=CARTESIAN_POINT('Ctrl Pts',(-19.5162819323213,13.1633177803101,
0.));
#239662=CARTESIAN_POINT('Ctrl Pts',(-19.4984412207082,13.1577198341245,
0.));
#239663=CARTESIAN_POINT('Ctrl Pts',(-19.4807301935268,13.1521082915853,
0.));
#239664=CARTESIAN_POINT('Ctrl Pts',(-19.4631497043258,13.1464839629971,
0.));
#239665=CARTESIAN_POINT('Ctrl Pts',(-19.4457006178876,13.1408476720061,
0.));
#239666=CARTESIAN_POINT('Ctrl Pts',(-19.4283838105262,13.1352002559438,
0.));
#239667=CARTESIAN_POINT('Ctrl Pts',(-19.4112001703557,13.1295425661634,
0.));
#239668=CARTESIAN_POINT('Ctrl Pts',(-19.3941505976263,13.1238754684177,
0.));
#239669=CARTESIAN_POINT('Ctrl Pts',(-19.3772360051091,13.118199843271,0.));
#239670=CARTESIAN_POINT('Ctrl Pts',(-19.3604573184515,13.1125165865022,
0.));
#239671=CARTESIAN_POINT('Ctrl Pts',(-19.3438154765395,13.1068266095186,
0.));
#239672=CARTESIAN_POINT('Ctrl Pts',(-19.3273114318269,13.1011308397591,
0.));
#239673=CARTESIAN_POINT('Ctrl Pts',(-19.310946150736,13.0954302211479,0.));
#239674=CARTESIAN_POINT('Ctrl Pts',(-19.2947206141247,13.0897257145968,
0.));
#239675=CARTESIAN_POINT('Ctrl Pts',(-19.2786358177198,13.0840182984949,
0.));
#239676=CARTESIAN_POINT('Ctrl Pts',(-19.2626927725596,13.0783089692118,
0.));
#239677=CARTESIAN_POINT('Ctrl Pts',(-19.2468925053989,13.0725987415859,
0.));
#239678=CARTESIAN_POINT('Ctrl Pts',(-19.2312360592033,13.0668886494795,
0.));
#239679=CARTESIAN_POINT('Ctrl Pts',(-19.2157244937142,13.0611797463915,
0.));
#239680=CARTESIAN_POINT('Ctrl Pts',(-19.2003588859772,13.0554731060538,
0.));
#239681=CARTESIAN_POINT('Ctrl Pts',(-19.1851403308825,13.0497698230441,
0.));
#239682=CARTESIAN_POINT('Ctrl Pts',(-19.1700699416622,13.0440710133772,
0.));
#239683=CARTESIAN_POINT('Ctrl Pts',(-19.155148850523,13.0383778152068,0.));
#239684=CARTESIAN_POINT('Ctrl Pts',(-19.1403782093386,13.0326913895838,
0.));
#239685=CARTESIAN_POINT('Ctrl Pts',(-19.1257591903099,13.0270129211976,
0.));
#239686=CARTESIAN_POINT('Ctrl Pts',(-19.111292986631,13.0213436191328,0.));
#239687=CARTESIAN_POINT('Ctrl Pts',(-19.0969808131228,13.0156847176096,
0.));
#239688=CARTESIAN_POINT('Ctrl Pts',(-19.0828239070484,13.0100374768788,
0.));
#239689=CARTESIAN_POINT('Ctrl Pts',(-19.0688235289437,13.0044031841382,
0.));
#239690=CARTESIAN_POINT('Ctrl Pts',(-19.0549809634354,12.9987831544502,
0.));
#239691=CARTESIAN_POINT('Ctrl Pts',(-19.0412975200398,12.9931787316514,
0.));
#239692=CARTESIAN_POINT('Ctrl Pts',(-19.0277745339909,12.9875912893003,
0.));
#239693=CARTESIAN_POINT('Ctrl Pts',(-19.014413367335,12.9820222318716,0.));
#239694=CARTESIAN_POINT('Ctrl Pts',(-19.0012154099792,12.9764729959206,
0.));
#239695=CARTESIAN_POINT('Ctrl Pts',(-18.9881820807585,12.9709450512747,
0.));
#239696=CARTESIAN_POINT('Ctrl Pts',(-18.9753148284473,12.9654399021868,
0.));
#239697=CARTESIAN_POINT('Ctrl Pts',(-18.9626151329226,12.9599590886317,
0.));
#239698=CARTESIAN_POINT('Ctrl Pts',(-18.9500845064714,12.9545041877377,
0.));
#239699=CARTESIAN_POINT('Ctrl Pts',(-18.9377244950435,12.9490768151821,
0.));
#239700=CARTESIAN_POINT('Ctrl Pts',(-18.9255366795196,12.9436786266106,
0.));
#239701=CARTESIAN_POINT('Ctrl Pts',(-18.9135226769466,12.9383113190375,
0.));
#239702=CARTESIAN_POINT('Ctrl Pts',(-18.9016841423402,12.9329766328184,
0.));
#239703=CARTESIAN_POINT('Ctrl Pts',(-18.8900227704888,12.9276763536372,
0.));
#239704=CARTESIAN_POINT('Ctrl Pts',(-18.8785402977528,12.9224123144982,
0.));
#239705=CARTESIAN_POINT('Ctrl Pts',(-18.8672385038328,12.9171863977047,
0.));
#239706=CARTESIAN_POINT('Ctrl Pts',(-18.8561192136201,12.9120005369066,
0.));
#239707=CARTESIAN_POINT('Ctrl Pts',(-18.8451842990986,12.9068567191856,
0.));
#239708=CARTESIAN_POINT('Ctrl Pts',(-18.834435681259,12.9017569871738,0.));
#239709=CARTESIAN_POINT('Ctrl Pts',(-18.8238753319124,12.8967034410752,
0.));
#239710=CARTESIAN_POINT('Ctrl Pts',(-18.8135052757815,12.8916982409931,
0.));
#239711=CARTESIAN_POINT('Ctrl Pts',(-18.8033275941939,12.8867436109543,
0.));
#239712=CARTESIAN_POINT('Ctrl Pts',(-18.7933444285867,12.8818418427474,
0.));
#239713=CARTESIAN_POINT('Ctrl Pts',(-18.7835579840481,12.8769952998097,
0.));
#239714=CARTESIAN_POINT('Ctrl Pts',(-18.7739705329029,12.8722064211814,
0.));
#239715=CARTESIAN_POINT('Ctrl Pts',(-18.7645844169568,12.8674777239656,
0.));
#239716=CARTESIAN_POINT('Ctrl Pts',(-18.7554020493888,12.8628118054172,
0.));
#239717=CARTESIAN_POINT('Ctrl Pts',(-18.7464259171248,12.8582113455644,
0.));
#239718=CARTESIAN_POINT('Ctrl Pts',(-18.7376585820851,12.8536791086315,
0.));
#239719=CARTESIAN_POINT('Ctrl Pts',(-18.7291026886552,12.849217951159,0.));
#239720=CARTESIAN_POINT('Ctrl Pts',(-18.7207609737701,12.8448308329494,
0.));
#239721=CARTESIAN_POINT('Ctrl Pts',(-18.7126362754446,12.8405208263432,
0.));
#239722=CARTESIAN_POINT('Ctrl Pts',(-18.7047315436296,12.8362911280362,
0.));
#239723=CARTESIAN_POINT('Ctrl Pts',(-18.6970498410173,12.832145059979,0.));
#239724=CARTESIAN_POINT('Ctrl Pts',(-18.6895943376172,12.8280860635231,
0.));
#239725=CARTESIAN_POINT('Ctrl Pts',(-18.6823683094139,12.8241176980016,
0.));
#239726=CARTESIAN_POINT('Ctrl Pts',(-18.6753751301091,12.8202436318473,
0.));
#239727=CARTESIAN_POINT('Ctrl Pts',(-18.6686182952798,12.8164676687361,
0.));
#239728=CARTESIAN_POINT('Ctrl Pts',(-18.6621014624746,12.8127937909632,
0.));
#239729=CARTESIAN_POINT('Ctrl Pts',(-18.6558284825772,12.8092261933858,
0.));
#239730=CARTESIAN_POINT('Ctrl Pts',(-18.6498034438986,12.805769331162,0.));
#239731=CARTESIAN_POINT('Ctrl Pts',(-18.6440306327457,12.8024278770153,
0.));
#239732=CARTESIAN_POINT('Ctrl Pts',(-18.63851447924,12.7992066625264,0.));
#239733=CARTESIAN_POINT('Ctrl Pts',(-18.6332595057005,12.7961106222251,
0.));
#239734=CARTESIAN_POINT('Ctrl Pts',(-18.6282702819371,12.7931447451556,
0.));
#239735=CARTESIAN_POINT('Ctrl Pts',(-18.6235516265575,12.7903142925234,
0.));
#239736=CARTESIAN_POINT('Ctrl Pts',(-18.6191087624752,12.7876249657834,
0.));
#239737=CARTESIAN_POINT('Ctrl Pts',(-18.6149475565189,12.78508316579,0.));
#239738=CARTESIAN_POINT('Ctrl Pts',(-18.611074482622,12.7826959526924,0.));
#239739=CARTESIAN_POINT('Ctrl Pts',(-18.6074961535723,12.7804705387658,
0.));
#239740=CARTESIAN_POINT('Ctrl Pts',(-18.6042190183703,12.7784139605067,
0.));
#239741=CARTESIAN_POINT('Ctrl Pts',(-18.6012488486708,12.7765325225082,
0.));
#239742=CARTESIAN_POINT('Ctrl Pts',(-18.5985917525949,12.7748328937639,
0.));
#239743=CARTESIAN_POINT('Ctrl Pts',(-18.5962551167772,12.7733231262107,
0.));
#239744=CARTESIAN_POINT('Ctrl Pts',(-18.5942490615409,12.7720142287169,
0.));
#239745=CARTESIAN_POINT('Ctrl Pts',(-18.5925859134582,12.7709195951153,
0.));
#239746=CARTESIAN_POINT('Ctrl Pts',(-18.5912775137806,12.7700520897174,
0.));
#239747=CARTESIAN_POINT('Ctrl Pts',(-18.590332877722,12.7694215127923,0.));
#239748=CARTESIAN_POINT('Ctrl Pts',(-18.589871621842,12.7691103481996,0.));
#239749=CARTESIAN_POINT('Ctrl Pts',(-18.5896919669158,12.7689864266924,
0.));
#239750=CARTESIAN_POINT('Ctrl Pts',(-18.5896460962961,12.7689524524484,
0.));
#239751=CARTESIAN_POINT('Ctrl Pts',(-18.5896416359912,12.7689476255363,
0.));
#239752=CARTESIAN_POINT('',(-22.1787195904339,13.5685075571671,12.));
#239753=CARTESIAN_POINT('',(-22.1787195904339,13.5685075571671,0.));
#239754=CARTESIAN_POINT('Ctrl Pts',(-18.5896416359912,12.7689476255363,
12.));
#239755=CARTESIAN_POINT('Ctrl Pts',(-18.5896460962961,12.7689524524484,
12.));
#239756=CARTESIAN_POINT('Ctrl Pts',(-18.5896919669158,12.7689864266924,
12.));
#239757=CARTESIAN_POINT('Ctrl Pts',(-18.589871621842,12.7691103481996,12.));
#239758=CARTESIAN_POINT('Ctrl Pts',(-18.590332877722,12.7694215127923,12.));
#239759=CARTESIAN_POINT('Ctrl Pts',(-18.5912775137806,12.7700520897174,
12.));
#239760=CARTESIAN_POINT('Ctrl Pts',(-18.5925859134582,12.7709195951153,
12.));
#239761=CARTESIAN_POINT('Ctrl Pts',(-18.5942490615409,12.7720142287169,
12.));
#239762=CARTESIAN_POINT('Ctrl Pts',(-18.5962551167772,12.7733231262107,
12.));
#239763=CARTESIAN_POINT('Ctrl Pts',(-18.5985917525949,12.7748328937639,
12.));
#239764=CARTESIAN_POINT('Ctrl Pts',(-18.6012488486708,12.7765325225082,
12.));
#239765=CARTESIAN_POINT('Ctrl Pts',(-18.6042190183703,12.7784139605067,
12.));
#239766=CARTESIAN_POINT('Ctrl Pts',(-18.6074961535723,12.7804705387658,
12.));
#239767=CARTESIAN_POINT('Ctrl Pts',(-18.611074482622,12.7826959526924,12.));
#239768=CARTESIAN_POINT('Ctrl Pts',(-18.6149475565189,12.78508316579,12.));
#239769=CARTESIAN_POINT('Ctrl Pts',(-18.6191087624752,12.7876249657834,
12.));
#239770=CARTESIAN_POINT('Ctrl Pts',(-18.6235516265575,12.7903142925234,
12.));
#239771=CARTESIAN_POINT('Ctrl Pts',(-18.6282702819371,12.7931447451556,
12.));
#239772=CARTESIAN_POINT('Ctrl Pts',(-18.6332595057005,12.7961106222251,
12.));
#239773=CARTESIAN_POINT('Ctrl Pts',(-18.63851447924,12.7992066625264,12.));
#239774=CARTESIAN_POINT('Ctrl Pts',(-18.6440306327457,12.8024278770153,
12.));
#239775=CARTESIAN_POINT('Ctrl Pts',(-18.6498034438986,12.805769331162,12.));
#239776=CARTESIAN_POINT('Ctrl Pts',(-18.6558284825772,12.8092261933858,
12.));
#239777=CARTESIAN_POINT('Ctrl Pts',(-18.6621014624746,12.8127937909632,
12.));
#239778=CARTESIAN_POINT('Ctrl Pts',(-18.6686182952798,12.8164676687361,
12.));
#239779=CARTESIAN_POINT('Ctrl Pts',(-18.6753751301091,12.8202436318473,
12.));
#239780=CARTESIAN_POINT('Ctrl Pts',(-18.6823683094139,12.8241176980016,
12.));
#239781=CARTESIAN_POINT('Ctrl Pts',(-18.6895943376172,12.8280860635231,
12.));
#239782=CARTESIAN_POINT('Ctrl Pts',(-18.6970498410173,12.832145059979,12.));
#239783=CARTESIAN_POINT('Ctrl Pts',(-18.7047315436296,12.8362911280362,
12.));
#239784=CARTESIAN_POINT('Ctrl Pts',(-18.7126362754446,12.8405208263432,
12.));
#239785=CARTESIAN_POINT('Ctrl Pts',(-18.7207609737701,12.8448308329494,
12.));
#239786=CARTESIAN_POINT('Ctrl Pts',(-18.7291026886552,12.849217951159,12.));
#239787=CARTESIAN_POINT('Ctrl Pts',(-18.7376585820851,12.8536791086315,
12.));
#239788=CARTESIAN_POINT('Ctrl Pts',(-18.7464259171248,12.8582113455644,
12.));
#239789=CARTESIAN_POINT('Ctrl Pts',(-18.7554020493888,12.8628118054172,
12.));
#239790=CARTESIAN_POINT('Ctrl Pts',(-18.7645844169568,12.8674777239656,
12.));
#239791=CARTESIAN_POINT('Ctrl Pts',(-18.7739705329029,12.8722064211814,
12.));
#239792=CARTESIAN_POINT('Ctrl Pts',(-18.7835579840481,12.8769952998097,
12.));
#239793=CARTESIAN_POINT('Ctrl Pts',(-18.7933444285867,12.8818418427474,
12.));
#239794=CARTESIAN_POINT('Ctrl Pts',(-18.8033275941939,12.8867436109543,
12.));
#239795=CARTESIAN_POINT('Ctrl Pts',(-18.8135052757815,12.8916982409931,
12.));
#239796=CARTESIAN_POINT('Ctrl Pts',(-18.8238753319124,12.8967034410752,
12.));
#239797=CARTESIAN_POINT('Ctrl Pts',(-18.834435681259,12.9017569871738,12.));
#239798=CARTESIAN_POINT('Ctrl Pts',(-18.8451842990986,12.9068567191856,
12.));
#239799=CARTESIAN_POINT('Ctrl Pts',(-18.8561192136201,12.9120005369066,
12.));
#239800=CARTESIAN_POINT('Ctrl Pts',(-18.8672385038328,12.9171863977047,
12.));
#239801=CARTESIAN_POINT('Ctrl Pts',(-18.8785402977528,12.9224123144982,
12.));
#239802=CARTESIAN_POINT('Ctrl Pts',(-18.8900227704888,12.9276763536372,
12.));
#239803=CARTESIAN_POINT('Ctrl Pts',(-18.9016841423402,12.9329766328184,
12.));
#239804=CARTESIAN_POINT('Ctrl Pts',(-18.9135226769466,12.9383113190375,
12.));
#239805=CARTESIAN_POINT('Ctrl Pts',(-18.9255366795196,12.9436786266106,
12.));
#239806=CARTESIAN_POINT('Ctrl Pts',(-18.9377244950435,12.9490768151821,
12.));
#239807=CARTESIAN_POINT('Ctrl Pts',(-18.9500845064714,12.9545041877377,
12.));
#239808=CARTESIAN_POINT('Ctrl Pts',(-18.9626151329226,12.9599590886317,
12.));
#239809=CARTESIAN_POINT('Ctrl Pts',(-18.9753148284473,12.9654399021868,
12.));
#239810=CARTESIAN_POINT('Ctrl Pts',(-18.9881820807585,12.9709450512747,
12.));
#239811=CARTESIAN_POINT('Ctrl Pts',(-19.0012154099792,12.9764729959206,
12.));
#239812=CARTESIAN_POINT('Ctrl Pts',(-19.014413367335,12.9820222318716,12.));
#239813=CARTESIAN_POINT('Ctrl Pts',(-19.0277745339909,12.9875912893003,
12.));
#239814=CARTESIAN_POINT('Ctrl Pts',(-19.0412975200398,12.9931787316514,
12.));
#239815=CARTESIAN_POINT('Ctrl Pts',(-19.0549809634354,12.9987831544502,
12.));
#239816=CARTESIAN_POINT('Ctrl Pts',(-19.0688235289437,13.0044031841382,
12.));
#239817=CARTESIAN_POINT('Ctrl Pts',(-19.0828239070484,13.0100374768788,
12.));
#239818=CARTESIAN_POINT('Ctrl Pts',(-19.0969808131228,13.0156847176096,
12.));
#239819=CARTESIAN_POINT('Ctrl Pts',(-19.111292986631,13.0213436191328,12.));
#239820=CARTESIAN_POINT('Ctrl Pts',(-19.1257591903099,13.0270129211976,
12.));
#239821=CARTESIAN_POINT('Ctrl Pts',(-19.1403782093386,13.0326913895838,
12.));
#239822=CARTESIAN_POINT('Ctrl Pts',(-19.155148850523,13.0383778152068,12.));
#239823=CARTESIAN_POINT('Ctrl Pts',(-19.1700699416622,13.0440710133772,
12.));
#239824=CARTESIAN_POINT('Ctrl Pts',(-19.1851403308825,13.0497698230441,
12.));
#239825=CARTESIAN_POINT('Ctrl Pts',(-19.2003588859772,13.0554731060538,
12.));
#239826=CARTESIAN_POINT('Ctrl Pts',(-19.2157244937142,13.0611797463915,
12.));
#239827=CARTESIAN_POINT('Ctrl Pts',(-19.2312360592033,13.0668886494795,
12.));
#239828=CARTESIAN_POINT('Ctrl Pts',(-19.2468925053989,13.0725987415859,
12.));
#239829=CARTESIAN_POINT('Ctrl Pts',(-19.2626927725596,13.0783089692118,
12.));
#239830=CARTESIAN_POINT('Ctrl Pts',(-19.2786358177198,13.0840182984949,
12.));
#239831=CARTESIAN_POINT('Ctrl Pts',(-19.2947206141247,13.0897257145968,
12.));
#239832=CARTESIAN_POINT('Ctrl Pts',(-19.310946150736,13.0954302211479,12.));
#239833=CARTESIAN_POINT('Ctrl Pts',(-19.3273114318269,13.1011308397591,
12.));
#239834=CARTESIAN_POINT('Ctrl Pts',(-19.3438154765395,13.1068266095186,
12.));
#239835=CARTESIAN_POINT('Ctrl Pts',(-19.3604573184515,13.1125165865022,
12.));
#239836=CARTESIAN_POINT('Ctrl Pts',(-19.3772360051091,13.118199843271,12.));
#239837=CARTESIAN_POINT('Ctrl Pts',(-19.3941505976263,13.1238754684177,
12.));
#239838=CARTESIAN_POINT('Ctrl Pts',(-19.4112001703557,13.1295425661634,
12.));
#239839=CARTESIAN_POINT('Ctrl Pts',(-19.4283838105262,13.1352002559438,
12.));
#239840=CARTESIAN_POINT('Ctrl Pts',(-19.4457006178876,13.1408476720061,
12.));
#239841=CARTESIAN_POINT('Ctrl Pts',(-19.4631497043258,13.1464839629971,
12.));
#239842=CARTESIAN_POINT('Ctrl Pts',(-19.4807301935268,13.1521082915853,
12.));
#239843=CARTESIAN_POINT('Ctrl Pts',(-19.4984412207082,13.1577198341245,
12.));
#239844=CARTESIAN_POINT('Ctrl Pts',(-19.5162819323213,13.1633177803101,
12.));
#239845=CARTESIAN_POINT('Ctrl Pts',(-19.5342514857562,13.168901332843,12.));
#239846=CARTESIAN_POINT('Ctrl Pts',(-19.5523490490244,13.1744697070911,
12.));
#239847=CARTESIAN_POINT('Ctrl Pts',(-19.5705738004667,13.1800221307673,
12.));
#239848=CARTESIAN_POINT('Ctrl Pts',(-19.5889249285338,13.1855578436471,
12.));
#239849=CARTESIAN_POINT('Ctrl Pts',(-19.6074016315414,13.1910760972814,
12.));
#239850=CARTESIAN_POINT('Ctrl Pts',(-19.6260031174244,13.1965761547151,
12.));
#239851=CARTESIAN_POINT('Ctrl Pts',(-19.6447286034772,13.2020572902065,
12.));
#239852=CARTESIAN_POINT('Ctrl Pts',(-19.6635773160936,13.2075187889529,
12.));
#239853=CARTESIAN_POINT('Ctrl Pts',(-19.6825484905823,13.2129599468485,
12.));
#239854=CARTESIAN_POINT('Ctrl Pts',(-19.7016413709685,13.2183800702436,
12.));
#239855=CARTESIAN_POINT('Ctrl Pts',(-19.7208552097868,13.2237784757065,
12.));
#239856=CARTESIAN_POINT('Ctrl Pts',(-19.7401892678697,13.2291544897899,
12.));
#239857=CARTESIAN_POINT('Ctrl Pts',(-19.7596428141168,13.2345074487963,
12.));
#239858=CARTESIAN_POINT('Ctrl Pts',(-19.7792151253289,13.2398366985675,
12.));
#239859=CARTESIAN_POINT('Ctrl Pts',(-19.7989054860495,13.2451415942805,
12.));
#239860=CARTESIAN_POINT('Ctrl Pts',(-19.8187131883917,13.2504215002457,
12.));
#239861=CARTESIAN_POINT('Ctrl Pts',(-19.8386375318634,13.2556757897086,
12.));
#239862=CARTESIAN_POINT('Ctrl Pts',(-19.8586778231715,13.2609038446529,
12.));
#239863=CARTESIAN_POINT('Ctrl Pts',(-19.8788333760577,13.2661050556132,
12.));
#239864=CARTESIAN_POINT('Ctrl Pts',(-19.8991035111745,13.271278821502,12.));
#239865=CARTESIAN_POINT('Ctrl Pts',(-19.9194875559422,13.2764245494357,
12.));
#239866=CARTESIAN_POINT('Ctrl Pts',(-19.9399848444019,13.2815416545663,
12.));
#239867=CARTESIAN_POINT('Ctrl Pts',(-19.9605947170586,13.286629559915,12.));
#239868=CARTESIAN_POINT('Ctrl Pts',(-19.981316520717,13.2916876962094,12.));
#239869=CARTESIAN_POINT('Ctrl Pts',(-20.0021496083738,13.2967155017306,
12.));
#239870=CARTESIAN_POINT('Ctrl Pts',(-20.0230933391038,13.3017124221637,
12.));
#239871=CARTESIAN_POINT('Ctrl Pts',(-20.0441470779345,13.3066779104515,
12.));
#239872=CARTESIAN_POINT('Ctrl Pts',(-20.0653101957188,13.3116114266515,
12.));
#239873=CARTESIAN_POINT('Ctrl Pts',(-20.0865820689883,13.3165124377962,
12.));
#239874=CARTESIAN_POINT('Ctrl Pts',(-20.1079620798375,13.3213804177587,
12.));
#239875=CARTESIAN_POINT('Ctrl Pts',(-20.1294496158402,13.3262148471226,
12.));
#239876=CARTESIAN_POINT('Ctrl Pts',(-20.1510440699474,13.3310152130564,
12.));
#239877=CARTESIAN_POINT('Ctrl Pts',(-20.1727448403817,13.3357810091903,
12.));
#239878=CARTESIAN_POINT('Ctrl Pts',(-20.1945513305235,13.3405117354971,
12.));
#239879=CARTESIAN_POINT('Ctrl Pts',(-20.216462948786,13.3452068981766,12.));
#239880=CARTESIAN_POINT('Ctrl Pts',(-20.2384791085359,13.3498660095386,
12.));
#239881=CARTESIAN_POINT('Ctrl Pts',(-20.2605992280122,13.3544885878889,
12.));
#239882=CARTESIAN_POINT('Ctrl Pts',(-20.2828227302339,13.3590741574195,
12.));
#239883=CARTESIAN_POINT('Ctrl Pts',(-20.3051490429048,13.3636222481016,
12.));
#239884=CARTESIAN_POINT('Ctrl Pts',(-20.3275775983029,13.3681323955826,
12.));
#239885=CARTESIAN_POINT('Ctrl Pts',(-20.3501078331814,13.3726041410867,
12.));
#239886=CARTESIAN_POINT('Ctrl Pts',(-20.3727391887184,13.3770370313188,
12.));
#239887=CARTESIAN_POINT('Ctrl Pts',(-20.3954711104502,13.3814306183719,
12.));
#239888=CARTESIAN_POINT('Ctrl Pts',(-20.4183030482002,13.3857844596387,
12.));
#239889=CARTESIAN_POINT('Ctrl Pts',(-20.4412344560008,13.3900981177255,
12.));
#239890=CARTESIAN_POINT('Ctrl Pts',(-20.4642647920038,13.3943711603739,
12.));
#239891=CARTESIAN_POINT('Ctrl Pts',(-20.487393518404,13.3986031603716,12.));
#239892=CARTESIAN_POINT('Ctrl Pts',(-20.5106201013753,13.4027936954529,
12.));
#239893=CARTESIAN_POINT('Ctrl Pts',(-20.5339440109956,13.4069423482076,
12.));
#239894=CARTESIAN_POINT('Ctrl Pts',(-20.5573647211639,13.4110487059912,
12.));
#239895=CARTESIAN_POINT('Ctrl Pts',(-20.5808817095155,13.4151123608411,
12.));
#239896=CARTESIAN_POINT('Ctrl Pts',(-20.6044944573153,13.4191329093932,
12.));
#239897=CARTESIAN_POINT('Ctrl Pts',(-20.6282024494237,13.4231099528179,
12.));
#239898=CARTESIAN_POINT('Ctrl Pts',(-20.6520051742869,13.4270430967651,
12.));
#239899=CARTESIAN_POINT('Ctrl Pts',(-20.6759021239103,13.4309319513119,
12.));
#239900=CARTESIAN_POINT('Ctrl Pts',(-20.6998927938288,13.4347761309154,
12.));
#239901=CARTESIAN_POINT('Ctrl Pts',(-20.7239766830675,13.4385752543663,
12.));
#239902=CARTESIAN_POINT('Ctrl Pts',(-20.7481532941013,13.4423289447561,
12.));
#239903=CARTESIAN_POINT('Ctrl Pts',(-20.7724221327608,13.4460368293688,
12.));
#239904=CARTESIAN_POINT('Ctrl Pts',(-20.7967827081227,13.4496985395637,
12.));
#239905=CARTESIAN_POINT('Ctrl Pts',(-20.821234532398,13.4533137106667,12.));
#239906=CARTESIAN_POINT('Ctrl Pts',(-20.8457771208082,13.4568819818631,
12.));
#239907=CARTESIAN_POINT('Ctrl Pts',(-20.8704099914641,13.4604029960983,
12.));
#239908=CARTESIAN_POINT('Ctrl Pts',(-20.8951326652158,13.4638763999725,
12.));
#239909=CARTESIAN_POINT('Ctrl Pts',(-20.9199446657584,13.4673018437718,
12.));
#239910=CARTESIAN_POINT('Ctrl Pts',(-20.9448455197557,13.4706789815166,
12.));
#239911=CARTESIAN_POINT('Ctrl Pts',(-20.9698347569476,13.4740074710087,
12.));
#239912=CARTESIAN_POINT('Ctrl Pts',(-20.9949119102592,13.4772869738879,
12.));
#239913=CARTESIAN_POINT('Ctrl Pts',(-21.0200765158885,13.4805171556822,
12.));
#239914=CARTESIAN_POINT('Ctrl Pts',(-21.0453281134247,13.4836976858912,
12.));
#239915=CARTESIAN_POINT('Ctrl Pts',(-21.0706662455202,13.4868282377191,
12.));
#239916=CARTESIAN_POINT('Ctrl Pts',(-21.0960904575048,13.4899084877718,
12.));
#239917=CARTESIAN_POINT('Ctrl Pts',(-21.1216002970209,13.4929381157778,
12.));
#239918=CARTESIAN_POINT('Ctrl Pts',(-21.1471953136209,13.4959168042934,
12.));
#239919=CARTESIAN_POINT('Ctrl Pts',(-21.1728750584173,13.4988442384491,
12.));
#239920=CARTESIAN_POINT('Ctrl Pts',(-21.1986390835825,13.5017201056088,
12.));
#239921=CARTESIAN_POINT('Ctrl Pts',(-21.224486942933,13.5045440957404,12.));
#239922=CARTESIAN_POINT('Ctrl Pts',(-21.2504181927429,13.5073159019454,
12.));
#239923=CARTESIAN_POINT('Ctrl Pts',(-21.2764323924442,13.5100352209207,
12.));
#239924=CARTESIAN_POINT('Ctrl Pts',(-21.3025291054236,13.5127017534972,
12.));
#239925=CARTESIAN_POINT('Ctrl Pts',(-21.328707899634,13.5153152050554,12.));
#239926=CARTESIAN_POINT('Ctrl Pts',(-21.3549683486219,13.5178752862461,
12.));
#239927=CARTESIAN_POINT('Ctrl Pts',(-21.3813100304967,13.5203817122496,
12.));
#239928=CARTESIAN_POINT('Ctrl Pts',(-21.4077325259318,13.5228342013508,
12.));
#239929=CARTESIAN_POINT('Ctrl Pts',(-21.4342354165254,13.5252324737795,
12.));
#239930=CARTESIAN_POINT('Ctrl Pts',(-21.4608182828695,13.5275762503553,
12.));
#239931=CARTESIAN_POINT('Ctrl Pts',(-21.487480703047,13.5298652514357,12.));
#239932=CARTESIAN_POINT('Ctrl Pts',(-21.5142222501671,13.5320991952145,
12.));
#239933=CARTESIAN_POINT('Ctrl Pts',(-21.5410424932511,13.5342777983225,
12.));
#239934=CARTESIAN_POINT('Ctrl Pts',(-21.5679410019011,13.5364007790292,
12.));
#239935=CARTESIAN_POINT('Ctrl Pts',(-21.5949173499022,13.5384678597206,
12.));
#239936=CARTESIAN_POINT('Ctrl Pts',(-21.6219711193951,13.5404787697798,
12.));
#239937=CARTESIAN_POINT('Ctrl Pts',(-21.6491019044647,13.5424332480698,
12.));
#239938=CARTESIAN_POINT('Ctrl Pts',(-21.676309315769,13.5443310461516,12.));
#239939=CARTESIAN_POINT('Ctrl Pts',(-21.7035929822939,13.546171929503,12.));
#239940=CARTESIAN_POINT('Ctrl Pts',(-21.730952541226,13.5479556704457,12.));
#239941=CARTESIAN_POINT('Ctrl Pts',(-21.7583876294532,13.5496820422186,
12.));
#239942=CARTESIAN_POINT('Ctrl Pts',(-21.7858978745848,13.5513508127232,
12.));
#239943=CARTESIAN_POINT('Ctrl Pts',(-21.8134828857963,13.5529617381569,
12.));
#239944=CARTESIAN_POINT('Ctrl Pts',(-21.841142245609,13.5545145573048,12.));
#239945=CARTESIAN_POINT('Ctrl Pts',(-21.8688754989401,13.5560089839426,
12.));
#239946=CARTESIAN_POINT('Ctrl Pts',(-21.8966821688876,13.5574447178484,
12.));
#239947=CARTESIAN_POINT('Ctrl Pts',(-21.9245617765827,13.5588214586672,
12.));
#239948=CARTESIAN_POINT('Ctrl Pts',(-21.9525138592862,13.5601389185315,
12.));
#239949=CARTESIAN_POINT('Ctrl Pts',(-21.9805379899192,13.5613968357589,
12.));
#239950=CARTESIAN_POINT('Ctrl Pts',(-22.0086337943431,13.5625949868313,
12.));
#239951=CARTESIAN_POINT('Ctrl Pts',(-22.0368009736227,13.5637332022393,
12.));
#239952=CARTESIAN_POINT('Ctrl Pts',(-22.0650393089492,13.5648113688894,
12.));
#239953=CARTESIAN_POINT('Ctrl Pts',(-22.0933486464442,13.5658294169106,
12.));
#239954=CARTESIAN_POINT('Ctrl Pts',(-22.1217288871823,13.5667873105179,
12.));
#239955=CARTESIAN_POINT('Ctrl Pts',(-22.1444897575076,13.5675054918922,
12.));
#239956=CARTESIAN_POINT('Ctrl Pts',(-22.1615922804939,13.5680170531724,
12.));
#239957=CARTESIAN_POINT('Ctrl Pts',(-22.1730081264583,13.5683460612913,
12.));
#239958=CARTESIAN_POINT('Ctrl Pts',(-22.1787195904339,13.5685075571671,
12.));
#239959=CARTESIAN_POINT('Ctrl Pts',(-17.1452095830633,14.6513681262571,
0.));
#239960=CARTESIAN_POINT('Ctrl Pts',(-17.1452095830633,14.6513681262571,
12.));
#239961=CARTESIAN_POINT('Ctrl Pts',(-17.1452153999142,14.6513711852843,
0.));
#239962=CARTESIAN_POINT('Ctrl Pts',(-17.1452153999142,14.6513711852843,
12.));
#239963=CARTESIAN_POINT('Ctrl Pts',(-17.1452600887037,14.6514066997196,
0.));
#239964=CARTESIAN_POINT('Ctrl Pts',(-17.1452600887037,14.6514066997196,
12.));
#239965=CARTESIAN_POINT('Ctrl Pts',(-17.1454262858043,14.6515481598068,
0.));
#239966=CARTESIAN_POINT('Ctrl Pts',(-17.1454262858043,14.6515481598068,
12.));
#239967=CARTESIAN_POINT('Ctrl Pts',(-17.1458462295271,14.6519131634508,
0.));
#239968=CARTESIAN_POINT('Ctrl Pts',(-17.1458462295271,14.6519131634508,
12.));
#239969=CARTESIAN_POINT('Ctrl Pts',(-17.1466998098673,14.6526624064978,
0.));
#239970=CARTESIAN_POINT('Ctrl Pts',(-17.1466998098673,14.6526624064978,
12.));
#239971=CARTESIAN_POINT('Ctrl Pts',(-17.147876394491,14.6537016966184,0.));
#239972=CARTESIAN_POINT('Ctrl Pts',(-17.147876394491,14.6537016966184,12.));
#239973=CARTESIAN_POINT('Ctrl Pts',(-17.1493641837558,14.655024862281,0.));
#239974=CARTESIAN_POINT('Ctrl Pts',(-17.1493641837558,14.655024862281,12.));
#239975=CARTESIAN_POINT('Ctrl Pts',(-17.1511476869496,14.6566237952435,
0.));
#239976=CARTESIAN_POINT('Ctrl Pts',(-17.1511476869496,14.6566237952435,
12.));
#239977=CARTESIAN_POINT('Ctrl Pts',(-17.1532107762718,14.6584900555302,
0.));
#239978=CARTESIAN_POINT('Ctrl Pts',(-17.1532107762718,14.6584900555302,
12.));
#239979=CARTESIAN_POINT('Ctrl Pts',(-17.1555401986401,14.6606167169642,
0.));
#239980=CARTESIAN_POINT('Ctrl Pts',(-17.1555401986401,14.6606167169642,
12.));
#239981=CARTESIAN_POINT('Ctrl Pts',(-17.1581262646789,14.6629987285992,
0.));
#239982=CARTESIAN_POINT('Ctrl Pts',(-17.1581262646789,14.6629987285992,
12.));
#239983=CARTESIAN_POINT('Ctrl Pts',(-17.1609609517369,14.6656319165057,
0.));
#239984=CARTESIAN_POINT('Ctrl Pts',(-17.1609609517369,14.6656319165057,
12.));
#239985=CARTESIAN_POINT('Ctrl Pts',(-17.1640366762305,14.6685123374423,
0.));
#239986=CARTESIAN_POINT('Ctrl Pts',(-17.1640366762305,14.6685123374423,
12.));
#239987=CARTESIAN_POINT('Ctrl Pts',(-17.167344972302,14.671635583332,0.));
#239988=CARTESIAN_POINT('Ctrl Pts',(-17.167344972302,14.671635583332,12.));
#239989=CARTESIAN_POINT('Ctrl Pts',(-17.1708771619129,14.6749971333867,
0.));
#239990=CARTESIAN_POINT('Ctrl Pts',(-17.1708771619129,14.6749971333867,
12.));
#239991=CARTESIAN_POINT('Ctrl Pts',(-17.1746247499057,14.6785925615677,
0.));
#239992=CARTESIAN_POINT('Ctrl Pts',(-17.1746247499057,14.6785925615677,
12.));
#239993=CARTESIAN_POINT('Ctrl Pts',(-17.1785800350826,14.6824178576167,
0.));
#239994=CARTESIAN_POINT('Ctrl Pts',(-17.1785800350826,14.6824178576167,
12.));
#239995=CARTESIAN_POINT('Ctrl Pts',(-17.182736158472,14.686469452232,0.));
#239996=CARTESIAN_POINT('Ctrl Pts',(-17.182736158472,14.686469452232,12.));
#239997=CARTESIAN_POINT('Ctrl Pts',(-17.1870867909918,14.6907440526958,
0.));
#239998=CARTESIAN_POINT('Ctrl Pts',(-17.1870867909918,14.6907440526958,
12.));
#239999=CARTESIAN_POINT('Ctrl Pts',(-17.1916259308415,14.6952385361705,
0.));
#240000=CARTESIAN_POINT('Ctrl Pts',(-17.1916259308415,14.6952385361705,
12.));
#240001=CARTESIAN_POINT('Ctrl Pts',(-17.1963476411694,14.699949811582,0.));
#240002=CARTESIAN_POINT('Ctrl Pts',(-17.1963476411694,14.699949811582,12.));
#240003=CARTESIAN_POINT('Ctrl Pts',(-17.2012461084268,14.7048748502663,
0.));
#240004=CARTESIAN_POINT('Ctrl Pts',(-17.2012461084268,14.7048748502663,
12.));
#240005=CARTESIAN_POINT('Ctrl Pts',(-17.2063157097315,14.7100107213586,
0.));
#240006=CARTESIAN_POINT('Ctrl Pts',(-17.2063157097315,14.7100107213586,
12.));
#240007=CARTESIAN_POINT('Ctrl Pts',(-17.2115510835989,14.7153546289339,
0.));
#240008=CARTESIAN_POINT('Ctrl Pts',(-17.2115510835989,14.7153546289339,
12.));
#240009=CARTESIAN_POINT('Ctrl Pts',(-17.2169471814256,14.7209039390327,
0.));
#240010=CARTESIAN_POINT('Ctrl Pts',(-17.2169471814256,14.7209039390327,
12.));
#240011=CARTESIAN_POINT('Ctrl Pts',(-17.2224992099667,14.7266561494282,
0.));
#240012=CARTESIAN_POINT('Ctrl Pts',(-17.2224992099667,14.7266561494282,
12.));
#240013=CARTESIAN_POINT('Ctrl Pts',(-17.2282025904314,14.7326088681163,
0.));
#240014=CARTESIAN_POINT('Ctrl Pts',(-17.2282025904314,14.7326088681163,
12.));
#240015=CARTESIAN_POINT('Ctrl Pts',(-17.2340529062076,14.7387597858116,
0.));
#240016=CARTESIAN_POINT('Ctrl Pts',(-17.2340529062076,14.7387597858116,
12.));
#240017=CARTESIAN_POINT('Ctrl Pts',(-17.2400458713565,14.7451066593792,
0.));
#240018=CARTESIAN_POINT('Ctrl Pts',(-17.2400458713565,14.7451066593792,
12.));
#240019=CARTESIAN_POINT('Ctrl Pts',(-17.2461773413288,14.7516473175124,
0.));
#240020=CARTESIAN_POINT('Ctrl Pts',(-17.2461773413288,14.7516473175124,
12.));
#240021=CARTESIAN_POINT('Ctrl Pts',(-17.2524433146837,14.7583796616617,
0.));
#240022=CARTESIAN_POINT('Ctrl Pts',(-17.2524433146837,14.7583796616617,
12.));
#240023=CARTESIAN_POINT('Ctrl Pts',(-17.2588399401465,14.7653016697591,
0.));
#240024=CARTESIAN_POINT('Ctrl Pts',(-17.2588399401465,14.7653016697591,
12.));
#240025=CARTESIAN_POINT('Ctrl Pts',(-17.2653635155319,14.7724113956731,
0.));
#240026=CARTESIAN_POINT('Ctrl Pts',(-17.2653635155319,14.7724113956731,
12.));
#240027=CARTESIAN_POINT('Ctrl Pts',(-17.2720104735194,14.7797069617804,
0.));
#240028=CARTESIAN_POINT('Ctrl Pts',(-17.2720104735194,14.7797069617804,
12.));
#240029=CARTESIAN_POINT('Ctrl Pts',(-17.2787773704849,14.787186553128,0.));
#240030=CARTESIAN_POINT('Ctrl Pts',(-17.2787773704849,14.787186553128,12.));
#240031=CARTESIAN_POINT('Ctrl Pts',(-17.2856608733196,14.7948484105249,
0.));
#240032=CARTESIAN_POINT('Ctrl Pts',(-17.2856608733196,14.7948484105249,
12.));
#240033=CARTESIAN_POINT('Ctrl Pts',(-17.2926577496513,14.8026908254276,
0.));
#240034=CARTESIAN_POINT('Ctrl Pts',(-17.2926577496513,14.8026908254276,
12.));
#240035=CARTESIAN_POINT('Ctrl Pts',(-17.299764866148,14.8107121391035,0.));
#240036=CARTESIAN_POINT('Ctrl Pts',(-17.299764866148,14.8107121391035,12.));
#240037=CARTESIAN_POINT('Ctrl Pts',(-17.3069791853706,14.8189107410162,
0.));
#240038=CARTESIAN_POINT('Ctrl Pts',(-17.3069791853706,14.8189107410162,
12.));
#240039=CARTESIAN_POINT('Ctrl Pts',(-17.3142977632659,14.8272850675379,
0.));
#240040=CARTESIAN_POINT('Ctrl Pts',(-17.3142977632659,14.8272850675379,
12.));
#240041=CARTESIAN_POINT('Ctrl Pts',(-17.3217177462101,14.8358336004197,
0.));
#240042=CARTESIAN_POINT('Ctrl Pts',(-17.3217177462101,14.8358336004197,
12.));
#240043=CARTESIAN_POINT('Ctrl Pts',(-17.3292363662605,14.8445548643508,
0.));
#240044=CARTESIAN_POINT('Ctrl Pts',(-17.3292363662605,14.8445548643508,
12.));
#240045=CARTESIAN_POINT('Ctrl Pts',(-17.336850936485,14.8534474245433,0.));
#240046=CARTESIAN_POINT('Ctrl Pts',(-17.336850936485,14.8534474245433,12.));
#240047=CARTESIAN_POINT('Ctrl Pts',(-17.3445588463475,14.8625098843417,
0.));
#240048=CARTESIAN_POINT('Ctrl Pts',(-17.3445588463475,14.8625098843417,
12.));
#240049=CARTESIAN_POINT('Ctrl Pts',(-17.3523575568645,14.8717408826955,
0.));
#240050=CARTESIAN_POINT('Ctrl Pts',(-17.3523575568645,14.8717408826955,
12.));
#240051=CARTESIAN_POINT('Ctrl Pts',(-17.3602445978161,14.8811390927423,
0.));
#240052=CARTESIAN_POINT('Ctrl Pts',(-17.3602445978161,14.8811390927423,
12.));
#240053=CARTESIAN_POINT('Ctrl Pts',(-17.3682175653235,14.8907032205788,
0.));
#240054=CARTESIAN_POINT('Ctrl Pts',(-17.3682175653235,14.8907032205788,
12.));
#240055=CARTESIAN_POINT('Ctrl Pts',(-17.3762741193076,14.900432003961,0.));
#240056=CARTESIAN_POINT('Ctrl Pts',(-17.3762741193076,14.900432003961,12.));
#240057=CARTESIAN_POINT('Ctrl Pts',(-17.3844119809824,14.9103242110057,
0.));
#240058=CARTESIAN_POINT('Ctrl Pts',(-17.3844119809824,14.9103242110057,
12.));
#240059=CARTESIAN_POINT('Ctrl Pts',(-17.3926289303986,14.9203786389342,
0.));
#240060=CARTESIAN_POINT('Ctrl Pts',(-17.3926289303986,14.9203786389342,
12.));
#240061=CARTESIAN_POINT('Ctrl Pts',(-17.4009228040749,14.9305941128757,
0.));
#240062=CARTESIAN_POINT('Ctrl Pts',(-17.4009228040749,14.9305941128757,
12.));
#240063=CARTESIAN_POINT('Ctrl Pts',(-17.4092914926071,14.940969484645,0.));
#240064=CARTESIAN_POINT('Ctrl Pts',(-17.4092914926071,14.940969484645,12.));
#240065=CARTESIAN_POINT('Ctrl Pts',(-17.4177329382828,14.9515036315143,
0.));
#240066=CARTESIAN_POINT('Ctrl Pts',(-17.4177329382828,14.9515036315143,
12.));
#240067=CARTESIAN_POINT('Ctrl Pts',(-17.426245132709,14.9621954549827,0.));
#240068=CARTESIAN_POINT('Ctrl Pts',(-17.426245132709,14.9621954549827,12.));
#240069=CARTESIAN_POINT('Ctrl Pts',(-17.4348261151396,14.9730438799452,
0.));
#240070=CARTESIAN_POINT('Ctrl Pts',(-17.4348261151396,14.9730438799452,
12.));
#240071=CARTESIAN_POINT('Ctrl Pts',(-17.4434739707773,14.9840478538358,
0.));
#240072=CARTESIAN_POINT('Ctrl Pts',(-17.4434739707773,14.9840478538358,
12.));
#240073=CARTESIAN_POINT('Ctrl Pts',(-17.4521868291004,14.9952063457778,
0.));
#240074=CARTESIAN_POINT('Ctrl Pts',(-17.4521868291004,14.9952063457778,
12.));
#240075=CARTESIAN_POINT('Ctrl Pts',(-17.4609628621418,15.0065183456921,
0.));
#240076=CARTESIAN_POINT('Ctrl Pts',(-17.4609628621418,15.0065183456921,
12.));
#240077=CARTESIAN_POINT('Ctrl Pts',(-17.4698002829357,15.0179828635086,
0.));
#240078=CARTESIAN_POINT('Ctrl Pts',(-17.4698002829357,15.0179828635086,
12.));
#240079=CARTESIAN_POINT('Ctrl Pts',(-17.4786973441417,15.029598928488,0.));
#240080=CARTESIAN_POINT('Ctrl Pts',(-17.4786973441417,15.029598928488,12.));
#240081=CARTESIAN_POINT('Ctrl Pts',(-17.4876523366178,15.0413655884993,
0.));
#240082=CARTESIAN_POINT('Ctrl Pts',(-17.4876523366178,15.0413655884993,
12.));
#240083=CARTESIAN_POINT('Ctrl Pts',(-17.4966635880245,15.0532819093085,
0.));
#240084=CARTESIAN_POINT('Ctrl Pts',(-17.4966635880245,15.0532819093085,
12.));
#240085=CARTESIAN_POINT('Ctrl Pts',(-17.5057294613874,15.0653469738306,
0.));
#240086=CARTESIAN_POINT('Ctrl Pts',(-17.5057294613874,15.0653469738306,
12.));
#240087=CARTESIAN_POINT('Ctrl Pts',(-17.5148483539684,15.0775598815748,
0.));
#240088=CARTESIAN_POINT('Ctrl Pts',(-17.5148483539684,15.0775598815748,
12.));
#240089=CARTESIAN_POINT('Ctrl Pts',(-17.5240186961788,15.0899197481082,
0.));
#240090=CARTESIAN_POINT('Ctrl Pts',(-17.5240186961788,15.0899197481082,
12.));
#240091=CARTESIAN_POINT('Ctrl Pts',(-17.5332389504829,15.1024257045033,
0.));
#240092=CARTESIAN_POINT('Ctrl Pts',(-17.5332389504829,15.1024257045033,
12.));
#240093=CARTESIAN_POINT('Ctrl Pts',(-17.5425076102966,15.1150768967729,
0.));
#240094=CARTESIAN_POINT('Ctrl Pts',(-17.5425076102966,15.1150768967729,
12.));
#240095=CARTESIAN_POINT('Ctrl Pts',(-17.5518231989122,15.127872485314,0.));
#240096=CARTESIAN_POINT('Ctrl Pts',(-17.5518231989122,15.127872485314,12.));
#240097=CARTESIAN_POINT('Ctrl Pts',(-17.5611842686196,15.1408116444877,
0.));
#240098=CARTESIAN_POINT('Ctrl Pts',(-17.5611842686196,15.1408116444877,
12.));
#240099=CARTESIAN_POINT('Ctrl Pts',(-17.570589399803,15.1538935621714,0.));
#240100=CARTESIAN_POINT('Ctrl Pts',(-17.570589399803,15.1538935621714,12.));
#240101=CARTESIAN_POINT('Ctrl Pts',(-17.5800372000539,15.1671174393136,
0.));
#240102=CARTESIAN_POINT('Ctrl Pts',(-17.5800372000539,15.1671174393136,
12.));
#240103=CARTESIAN_POINT('Ctrl Pts',(-17.5895263032592,15.1804824894605,
0.));
#240104=CARTESIAN_POINT('Ctrl Pts',(-17.5895263032592,15.1804824894605,
12.));
#240105=CARTESIAN_POINT('Ctrl Pts',(-17.5990553687595,15.1939879383268,
0.));
#240106=CARTESIAN_POINT('Ctrl Pts',(-17.5990553687595,15.1939879383268,
12.));
#240107=CARTESIAN_POINT('Ctrl Pts',(-17.6086230806497,15.2076330234686,
0.));
#240108=CARTESIAN_POINT('Ctrl Pts',(-17.6086230806497,15.2076330234686,
12.));
#240109=CARTESIAN_POINT('Ctrl Pts',(-17.6182281470467,15.22141699392,0.));
#240110=CARTESIAN_POINT('Ctrl Pts',(-17.6182281470467,15.22141699392,12.));
#240111=CARTESIAN_POINT('Ctrl Pts',(-17.6278692993765,15.2353391098367,
0.));
#240112=CARTESIAN_POINT('Ctrl Pts',(-17.6278692993765,15.2353391098367,
12.));
#240113=CARTESIAN_POINT('Ctrl Pts',(-17.637545291637,15.2493986421091,0.));
#240114=CARTESIAN_POINT('Ctrl Pts',(-17.637545291637,15.2493986421091,12.));
#240115=CARTESIAN_POINT('Ctrl Pts',(-17.6472548997329,15.263594872029,0.));
#240116=CARTESIAN_POINT('Ctrl Pts',(-17.6472548997329,15.263594872029,12.));
#240117=CARTESIAN_POINT('Ctrl Pts',(-17.6569969209,15.2779270910238,0.));
#240118=CARTESIAN_POINT('Ctrl Pts',(-17.6569969209,15.2779270910238,12.));
#240119=CARTESIAN_POINT('Ctrl Pts',(-17.6667701731041,15.2923946003598,
0.));
#240120=CARTESIAN_POINT('Ctrl Pts',(-17.6667701731041,15.2923946003598,
12.));
#240121=CARTESIAN_POINT('Ctrl Pts',(-17.6765734944559,15.3069967108501,
0.));
#240122=CARTESIAN_POINT('Ctrl Pts',(-17.6765734944559,15.3069967108501,
12.));
#240123=CARTESIAN_POINT('Ctrl Pts',(-17.6864057426052,15.3217327425341,
0.));
#240124=CARTESIAN_POINT('Ctrl Pts',(-17.6864057426052,15.3217327425341,
12.));
#240125=CARTESIAN_POINT('Ctrl Pts',(-17.6962657941984,15.3366020244069,
0.));
#240126=CARTESIAN_POINT('Ctrl Pts',(-17.6962657941984,15.3366020244069,
12.));
#240127=CARTESIAN_POINT('Ctrl Pts',(-17.7061525444044,15.3516038942064,
0.));
#240128=CARTESIAN_POINT('Ctrl Pts',(-17.7061525444044,15.3516038942064,
12.));
#240129=CARTESIAN_POINT('Ctrl Pts',(-17.7160649064208,15.3667376981702,
0.));
#240130=CARTESIAN_POINT('Ctrl Pts',(-17.7160649064208,15.3667376981702,
12.));
#240131=CARTESIAN_POINT('Ctrl Pts',(-17.7260018109923,15.3820027907965,
0.));
#240132=CARTESIAN_POINT('Ctrl Pts',(-17.7260018109923,15.3820027907965,
12.));
#240133=CARTESIAN_POINT('Ctrl Pts',(-17.7359622059143,15.3973985345796,
0.));
#240134=CARTESIAN_POINT('Ctrl Pts',(-17.7359622059143,15.3973985345796,
12.));
#240135=CARTESIAN_POINT('Ctrl Pts',(-17.7459450555803,15.4129242997828,
0.));
#240136=CARTESIAN_POINT('Ctrl Pts',(-17.7459450555803,15.4129242997828,
12.));
#240137=CARTESIAN_POINT('Ctrl Pts',(-17.7559493405871,15.4285794642658,
0.));
#240138=CARTESIAN_POINT('Ctrl Pts',(-17.7559493405871,15.4285794642658,
12.));
#240139=CARTESIAN_POINT('Ctrl Pts',(-17.765974057326,15.4443634132865,0.));
#240140=CARTESIAN_POINT('Ctrl Pts',(-17.765974057326,15.4443634132865,12.));
#240141=CARTESIAN_POINT('Ctrl Pts',(-17.7760182175817,15.4602755393019,
0.));
#240142=CARTESIAN_POINT('Ctrl Pts',(-17.7760182175817,15.4602755393019,
12.));
#240143=CARTESIAN_POINT('Ctrl Pts',(-17.7860808481229,15.4763152417506,
0.));
#240144=CARTESIAN_POINT('Ctrl Pts',(-17.7860808481229,15.4763152417506,
12.));
#240145=CARTESIAN_POINT('Ctrl Pts',(-17.7961609903161,15.4924819268529,
0.));
#240146=CARTESIAN_POINT('Ctrl Pts',(-17.7961609903161,15.4924819268529,
12.));
#240147=CARTESIAN_POINT('Ctrl Pts',(-17.8062576997964,15.5087750074728,
0.));
#240148=CARTESIAN_POINT('Ctrl Pts',(-17.8062576997964,15.5087750074728,
12.));
#240149=CARTESIAN_POINT('Ctrl Pts',(-17.8163700461263,15.5251939029558,
0.));
#240150=CARTESIAN_POINT('Ctrl Pts',(-17.8163700461263,15.5251939029558,
12.));
#240151=CARTESIAN_POINT('Ctrl Pts',(-17.8264971124606,15.5417380389639,
0.));
#240152=CARTESIAN_POINT('Ctrl Pts',(-17.8264971124606,15.5417380389639,
12.));
#240153=CARTESIAN_POINT('Ctrl Pts',(-17.8366379952078,15.5584068472976,
0.));
#240154=CARTESIAN_POINT('Ctrl Pts',(-17.8366379952078,15.5584068472976,
12.));
#240155=CARTESIAN_POINT('Ctrl Pts',(-17.8467918036977,15.5751997657153,
0.));
#240156=CARTESIAN_POINT('Ctrl Pts',(-17.8467918036977,15.5751997657153,
12.));
#240157=CARTESIAN_POINT('Ctrl Pts',(-17.8569576598996,15.5921162378183,
0.));
#240158=CARTESIAN_POINT('Ctrl Pts',(-17.8569576598996,15.5921162378183,
12.));
#240159=CARTESIAN_POINT('Ctrl Pts',(-17.8671346981388,15.6091557129205,
0.));
#240160=CARTESIAN_POINT('Ctrl Pts',(-17.8671346981388,15.6091557129205,
12.));
#240161=CARTESIAN_POINT('Ctrl Pts',(-17.8773220648125,15.6263176459107,
0.));
#240162=CARTESIAN_POINT('Ctrl Pts',(-17.8773220648125,15.6263176459107,
12.));
#240163=CARTESIAN_POINT('Ctrl Pts',(-17.8875189181095,15.6436014971088,
0.));
#240164=CARTESIAN_POINT('Ctrl Pts',(-17.8875189181095,15.6436014971088,
12.));
#240165=CARTESIAN_POINT('Ctrl Pts',(-17.8977244277247,15.6610067321036,
0.));
#240166=CARTESIAN_POINT('Ctrl Pts',(-17.8977244277247,15.6610067321036,
12.));
#240167=CARTESIAN_POINT('Ctrl Pts',(-17.9079377746118,15.6785328216467,
0.));
#240168=CARTESIAN_POINT('Ctrl Pts',(-17.9079377746118,15.6785328216467,
12.));
#240169=CARTESIAN_POINT('Ctrl Pts',(-17.918158150746,15.6961792415526,0.));
#240170=CARTESIAN_POINT('Ctrl Pts',(-17.918158150746,15.6961792415526,12.));
#240171=CARTESIAN_POINT('Ctrl Pts',(-17.9283847588837,15.713945472584,0.));
#240172=CARTESIAN_POINT('Ctrl Pts',(-17.9283847588837,15.713945472584,12.));
#240173=CARTESIAN_POINT('Ctrl Pts',(-17.9386168123261,15.7318310003334,
0.));
#240174=CARTESIAN_POINT('Ctrl Pts',(-17.9386168123261,15.7318310003334,
12.));
#240175=CARTESIAN_POINT('Ctrl Pts',(-17.9488535346776,15.7498353150856,
0.));
#240176=CARTESIAN_POINT('Ctrl Pts',(-17.9488535346776,15.7498353150856,
12.));
#240177=CARTESIAN_POINT('Ctrl Pts',(-17.9590941596236,15.7679579117072,
0.));
#240178=CARTESIAN_POINT('Ctrl Pts',(-17.9590941596236,15.7679579117072,
12.));
#240179=CARTESIAN_POINT('Ctrl Pts',(-17.9693379307297,15.786198289572,0.));
#240180=CARTESIAN_POINT('Ctrl Pts',(-17.9693379307297,15.786198289572,12.));
#240181=CARTESIAN_POINT('Ctrl Pts',(-17.9795841012383,15.8045559524674,
0.));
#240182=CARTESIAN_POINT('Ctrl Pts',(-17.9795841012383,15.8045559524674,
12.));
#240183=CARTESIAN_POINT('Ctrl Pts',(-17.9898319338664,15.8230304084963,
0.));
#240184=CARTESIAN_POINT('Ctrl Pts',(-17.9898319338664,15.8230304084963,
12.));
#240185=CARTESIAN_POINT('Ctrl Pts',(-18.0000807006055,15.8416211699681,
0.));
#240186=CARTESIAN_POINT('Ctrl Pts',(-18.0000807006055,15.8416211699681,
12.));
#240187=CARTESIAN_POINT('Ctrl Pts',(-18.010329682521,15.8603277532834,0.));
#240188=CARTESIAN_POINT('Ctrl Pts',(-18.010329682521,15.8603277532834,12.));
#240189=CARTESIAN_POINT('Ctrl Pts',(-18.0205781695773,15.8791496788685,
0.));
#240190=CARTESIAN_POINT('Ctrl Pts',(-18.0205781695773,15.8791496788685,
12.));
#240191=CARTESIAN_POINT('Ctrl Pts',(-18.0308254604638,15.8980864711043,
0.));
#240192=CARTESIAN_POINT('Ctrl Pts',(-18.0308254604638,15.8980864711043,
12.));
#240193=CARTESIAN_POINT('Ctrl Pts',(-18.0410708624208,15.9171376582436,
0.));
#240194=CARTESIAN_POINT('Ctrl Pts',(-18.0410708624208,15.9171376582436,
12.));
#240195=CARTESIAN_POINT('Ctrl Pts',(-18.0513136910691,15.9363027723244,
0.));
#240196=CARTESIAN_POINT('Ctrl Pts',(-18.0513136910691,15.9363027723244,
12.));
#240197=CARTESIAN_POINT('Ctrl Pts',(-18.061553270236,15.9555813490645,0.));
#240198=CARTESIAN_POINT('Ctrl Pts',(-18.061553270236,15.9555813490645,12.));
#240199=CARTESIAN_POINT('Ctrl Pts',(-18.071788931796,15.9749729277848,0.));
#240200=CARTESIAN_POINT('Ctrl Pts',(-18.071788931796,15.9749729277848,12.));
#240201=CARTESIAN_POINT('Ctrl Pts',(-18.0820200155239,15.9944770513616,
0.));
#240202=CARTESIAN_POINT('Ctrl Pts',(-18.0820200155239,15.9944770513616,
12.));
#240203=CARTESIAN_POINT('Ctrl Pts',(-18.0922458689464,16.0140932661612,
0.));
#240204=CARTESIAN_POINT('Ctrl Pts',(-18.0922458689464,16.0140932661612,
12.));
#240205=CARTESIAN_POINT('Ctrl Pts',(-18.1024658471966,16.0338211219693,
0.));
#240206=CARTESIAN_POINT('Ctrl Pts',(-18.1024658471966,16.0338211219693,
12.));
#240207=CARTESIAN_POINT('Ctrl Pts',(-18.1126793128688,16.0536601719124,
0.));
#240208=CARTESIAN_POINT('Ctrl Pts',(-18.1126793128688,16.0536601719124,
12.));
#240209=CARTESIAN_POINT('Ctrl Pts',(-18.1228856358746,16.0736099723664,
0.));
#240210=CARTESIAN_POINT('Ctrl Pts',(-18.1228856358746,16.0736099723664,
12.));
#240211=CARTESIAN_POINT('Ctrl Pts',(-18.1330841933099,16.0936700829108,
0.));
#240212=CARTESIAN_POINT('Ctrl Pts',(-18.1330841933099,16.0936700829108,
12.));
#240213=CARTESIAN_POINT('Ctrl Pts',(-18.1432743693231,16.113840066279,0.));
#240214=CARTESIAN_POINT('Ctrl Pts',(-18.1432743693231,16.113840066279,12.));
#240215=CARTESIAN_POINT('Ctrl Pts',(-18.1534555549851,16.1341194882987,
0.));
#240216=CARTESIAN_POINT('Ctrl Pts',(-18.1534555549851,16.1341194882987,
12.));
#240217=CARTESIAN_POINT('Ctrl Pts',(-18.1636271481616,16.1545079178261,
0.));
#240218=CARTESIAN_POINT('Ctrl Pts',(-18.1636271481616,16.1545079178261,
12.));
#240219=CARTESIAN_POINT('Ctrl Pts',(-18.1737885533852,16.1750049266673,
0.));
#240220=CARTESIAN_POINT('Ctrl Pts',(-18.1737885533852,16.1750049266673,
12.));
#240221=CARTESIAN_POINT('Ctrl Pts',(-18.1839391817335,16.1956100895076,
0.));
#240222=CARTESIAN_POINT('Ctrl Pts',(-18.1839391817335,16.1956100895076,
12.));
#240223=CARTESIAN_POINT('Ctrl Pts',(-18.1940784507232,16.2163229838878,
0.));
#240224=CARTESIAN_POINT('Ctrl Pts',(-18.1940784507232,16.2163229838878,
12.));
#240225=CARTESIAN_POINT('Ctrl Pts',(-18.2042057842037,16.237143190164,0.));
#240226=CARTESIAN_POINT('Ctrl Pts',(-18.2042057842037,16.237143190164,12.));
#240227=CARTESIAN_POINT('Ctrl Pts',(-18.214320612253,16.2580702914615,0.));
#240228=CARTESIAN_POINT('Ctrl Pts',(-18.214320612253,16.2580702914615,12.));
#240229=CARTESIAN_POINT('Ctrl Pts',(-18.2244223710745,16.2791038736223,
0.));
#240230=CARTESIAN_POINT('Ctrl Pts',(-18.2244223710745,16.2791038736223,
12.));
#240231=CARTESIAN_POINT('Ctrl Pts',(-18.2345105028981,16.3002435251378,
0.));
#240232=CARTESIAN_POINT('Ctrl Pts',(-18.2345105028981,16.3002435251378,
12.));
#240233=CARTESIAN_POINT('Ctrl Pts',(-18.2445844558742,16.3214888370988,
0.));
#240234=CARTESIAN_POINT('Ctrl Pts',(-18.2445844558742,16.3214888370988,
12.));
#240235=CARTESIAN_POINT('Ctrl Pts',(-18.2546436839609,16.342839403159,0.));
#240236=CARTESIAN_POINT('Ctrl Pts',(-18.2546436839609,16.342839403159,12.));
#240237=CARTESIAN_POINT('Ctrl Pts',(-18.2646876468169,16.3642948194869,
0.));
#240238=CARTESIAN_POINT('Ctrl Pts',(-18.2646876468169,16.3642948194869,
12.));
#240239=CARTESIAN_POINT('Ctrl Pts',(-18.2747158096934,16.385854684708,0.));
#240240=CARTESIAN_POINT('Ctrl Pts',(-18.2747158096934,16.385854684708,12.));
#240241=CARTESIAN_POINT('Ctrl Pts',(-18.2847276433308,16.4075185998454,
0.));
#240242=CARTESIAN_POINT('Ctrl Pts',(-18.2847276433308,16.4075185998454,
12.));
#240243=CARTESIAN_POINT('Ctrl Pts',(-18.2947226238509,16.4292861682377,
0.));
#240244=CARTESIAN_POINT('Ctrl Pts',(-18.2947226238509,16.4292861682377,
12.));
#240245=CARTESIAN_POINT('Ctrl Pts',(-18.3047002326858,16.4511569955231,
0.));
#240246=CARTESIAN_POINT('Ctrl Pts',(-18.3047002326858,16.4511569955231,
12.));
#240247=CARTESIAN_POINT('Ctrl Pts',(-18.3146599565229,16.4731306896439,
0.));
#240248=CARTESIAN_POINT('Ctrl Pts',(-18.3146599565229,16.4731306896439,
12.));
#240249=CARTESIAN_POINT('Ctrl Pts',(-18.3246012872468,16.4952068608344,
0.));
#240250=CARTESIAN_POINT('Ctrl Pts',(-18.3246012872468,16.4952068608344,
12.));
#240251=CARTESIAN_POINT('Ctrl Pts',(-18.3345237218864,16.5173851216045,
0.));
#240252=CARTESIAN_POINT('Ctrl Pts',(-18.3345237218864,16.5173851216045,
12.));
#240253=CARTESIAN_POINT('Ctrl Pts',(-18.3444267625601,16.5396650867139,
0.));
#240254=CARTESIAN_POINT('Ctrl Pts',(-18.3444267625601,16.5396650867139,
12.));
#240255=CARTESIAN_POINT('Ctrl Pts',(-18.3543099164331,16.5620463731414,
0.));
#240256=CARTESIAN_POINT('Ctrl Pts',(-18.3543099164331,16.5620463731414,
12.));
#240257=CARTESIAN_POINT('Ctrl Pts',(-18.364172695589,16.5845286000218,0.));
#240258=CARTESIAN_POINT('Ctrl Pts',(-18.364172695589,16.5845286000218,12.));
#240259=CARTESIAN_POINT('Ctrl Pts',(-18.3740146168879,16.6071113885711,
0.));
#240260=CARTESIAN_POINT('Ctrl Pts',(-18.3740146168879,16.6071113885711,
12.));
#240261=CARTESIAN_POINT('Ctrl Pts',(-18.3838352018327,16.6297943620056,
0.));
#240262=CARTESIAN_POINT('Ctrl Pts',(-18.3838352018327,16.6297943620056,
12.));
#240263=CARTESIAN_POINT('Ctrl Pts',(-18.3936339764332,16.6525771454513,
0.));
#240264=CARTESIAN_POINT('Ctrl Pts',(-18.3936339764332,16.6525771454513,
12.));
#240265=CARTESIAN_POINT('Ctrl Pts',(-18.4034104710789,16.6754593658513,
0.));
#240266=CARTESIAN_POINT('Ctrl Pts',(-18.4034104710789,16.6754593658513,
12.));
#240267=CARTESIAN_POINT('Ctrl Pts',(-18.413164220399,16.698440651849,0.));
#240268=CARTESIAN_POINT('Ctrl Pts',(-18.413164220399,16.698440651849,12.));
#240269=CARTESIAN_POINT('Ctrl Pts',(-18.4228947633186,16.7215206338818,
0.));
#240270=CARTESIAN_POINT('Ctrl Pts',(-18.4228947633186,16.7215206338818,
12.));
#240271=CARTESIAN_POINT('Ctrl Pts',(-18.4326016431392,16.7446989442882,
0.));
#240272=CARTESIAN_POINT('Ctrl Pts',(-18.4326016431392,16.7446989442882,
12.));
#240273=CARTESIAN_POINT('Ctrl Pts',(-18.4422844076099,16.7679752173992,
0.));
#240274=CARTESIAN_POINT('Ctrl Pts',(-18.4422844076099,16.7679752173992,
12.));
#240275=CARTESIAN_POINT('Ctrl Pts',(-18.4519426090124,16.791349089629,0.));
#240276=CARTESIAN_POINT('Ctrl Pts',(-18.4519426090124,16.791349089629,12.));
#240277=CARTESIAN_POINT('Ctrl Pts',(-18.4615758042305,16.8148201995472,
0.));
#240278=CARTESIAN_POINT('Ctrl Pts',(-18.4615758042305,16.8148201995472,
12.));
#240279=CARTESIAN_POINT('Ctrl Pts',(-18.4711835548622,16.8383881879707,
0.));
#240280=CARTESIAN_POINT('Ctrl Pts',(-18.4711835548622,16.8383881879707,
12.));
#240281=CARTESIAN_POINT('Ctrl Pts',(-18.4807654268769,16.8620526977169,
0.));
#240282=CARTESIAN_POINT('Ctrl Pts',(-18.4807654268769,16.8620526977169,
12.));
#240283=CARTESIAN_POINT('Ctrl Pts',(-18.4903209902226,16.8858133733086,
0.));
#240284=CARTESIAN_POINT('Ctrl Pts',(-18.4903209902226,16.8858133733086,
12.));
#240285=CARTESIAN_POINT('Ctrl Pts',(-18.4998498184619,16.9096698606942,
0.));
#240286=CARTESIAN_POINT('Ctrl Pts',(-18.4998498184619,16.9096698606942,
12.));
#240287=CARTESIAN_POINT('Ctrl Pts',(-18.5093514883835,16.9336218069353,
0.));
#240288=CARTESIAN_POINT('Ctrl Pts',(-18.5093514883835,16.9336218069353,
12.));
#240289=CARTESIAN_POINT('Ctrl Pts',(-18.518825579666,16.957668859934,0.));
#240290=CARTESIAN_POINT('Ctrl Pts',(-18.518825579666,16.957668859934,12.));
#240291=CARTESIAN_POINT('Ctrl Pts',(-18.5282716744198,16.9818106680382,
0.));
#240292=CARTESIAN_POINT('Ctrl Pts',(-18.5282716744198,16.9818106680382,
12.));
#240293=CARTESIAN_POINT('Ctrl Pts',(-18.5376893576961,17.0060468805099,
0.));
#240294=CARTESIAN_POINT('Ctrl Pts',(-18.5376893576961,17.0060468805099,
12.));
#240295=CARTESIAN_POINT('Ctrl Pts',(-18.5470782182089,17.030377148174,0.));
#240296=CARTESIAN_POINT('Ctrl Pts',(-18.5470782182089,17.030377148174,12.));
#240297=CARTESIAN_POINT('Ctrl Pts',(-18.5564378489628,17.0548011239751,
0.));
#240298=CARTESIAN_POINT('Ctrl Pts',(-18.5564378489628,17.0548011239751,
12.));
#240299=CARTESIAN_POINT('Ctrl Pts',(-18.5657678479788,17.0793184636079,
0.));
#240300=CARTESIAN_POINT('Ctrl Pts',(-18.5657678479788,17.0793184636079,
12.));
#240301=CARTESIAN_POINT('Ctrl Pts',(-18.5750678188543,17.1039288260001,
0.));
#240302=CARTESIAN_POINT('Ctrl Pts',(-18.5750678188543,17.1039288260001,
12.));
#240303=CARTESIAN_POINT('Ctrl Pts',(-18.5843373717253,17.1286318741185,
0.));
#240304=CARTESIAN_POINT('Ctrl Pts',(-18.5843373717253,17.1286318741185,
12.));
#240305=CARTESIAN_POINT('Ctrl Pts',(-18.5935761222833,17.1534272741646,
0.));
#240306=CARTESIAN_POINT('Ctrl Pts',(-18.5935761222833,17.1534272741646,
12.));
#240307=CARTESIAN_POINT('Ctrl Pts',(-18.6027836898826,17.1783146940131,
0.));
#240308=CARTESIAN_POINT('Ctrl Pts',(-18.6027836898826,17.1783146940131,
12.));
#240309=CARTESIAN_POINT('Ctrl Pts',(-18.6119596959957,17.2032938019288,
0.));
#240310=CARTESIAN_POINT('Ctrl Pts',(-18.6119596959957,17.2032938019288,
12.));
#240311=CARTESIAN_POINT('Ctrl Pts',(-18.6211037624041,17.2283642650519,
0.));
#240312=CARTESIAN_POINT('Ctrl Pts',(-18.6211037624041,17.2283642650519,
12.));
#240313=CARTESIAN_POINT('Ctrl Pts',(-18.630215509794,17.2535257482186,0.));
#240314=CARTESIAN_POINT('Ctrl Pts',(-18.630215509794,17.2535257482186,12.));
#240315=CARTESIAN_POINT('Ctrl Pts',(-18.639294555474,17.278777912021,0.));
#240316=CARTESIAN_POINT('Ctrl Pts',(-18.639294555474,17.278777912021,12.));
#240317=CARTESIAN_POINT('Ctrl Pts',(-18.6483405141853,17.3041204135069,
0.));
#240318=CARTESIAN_POINT('Ctrl Pts',(-18.6483405141853,17.3041204135069,
12.));
#240319=CARTESIAN_POINT('Ctrl Pts',(-18.6573530024019,17.3295529098612,
0.));
#240320=CARTESIAN_POINT('Ctrl Pts',(-18.6573530024019,17.3295529098612,
12.));
#240321=CARTESIAN_POINT('Ctrl Pts',(-18.6663316416569,17.3550750612438,
0.));
#240322=CARTESIAN_POINT('Ctrl Pts',(-18.6663316416569,17.3550750612438,
12.));
#240323=CARTESIAN_POINT('Ctrl Pts',(-18.6752760624045,17.3806865340744,
0.));
#240324=CARTESIAN_POINT('Ctrl Pts',(-18.6752760624045,17.3806865340744,
12.));
#240325=CARTESIAN_POINT('Ctrl Pts',(-18.6841859073472,17.4063870038563,
0.));
#240326=CARTESIAN_POINT('Ctrl Pts',(-18.6841859073472,17.4063870038563,
12.));
#240327=CARTESIAN_POINT('Ctrl Pts',(-18.6930608357421,17.4321761588148,
0.));
#240328=CARTESIAN_POINT('Ctrl Pts',(-18.6930608357421,17.4321761588148,
12.));
#240329=CARTESIAN_POINT('Ctrl Pts',(-18.7019005250322,17.4580537012764,
0.));
#240330=CARTESIAN_POINT('Ctrl Pts',(-18.7019005250322,17.4580537012764,
12.));
#240331=CARTESIAN_POINT('Ctrl Pts',(-18.7107046613941,17.4840193397176,
0.));
#240332=CARTESIAN_POINT('Ctrl Pts',(-18.7107046613941,17.4840193397176,
12.));
#240333=CARTESIAN_POINT('Ctrl Pts',(-18.7194729318128,17.5100727820891,
0.));
#240334=CARTESIAN_POINT('Ctrl Pts',(-18.7194729318128,17.5100727820891,
12.));
#240335=CARTESIAN_POINT('Ctrl Pts',(-18.728205015716,17.5362137287604,0.));
#240336=CARTESIAN_POINT('Ctrl Pts',(-18.728205015716,17.5362137287604,12.));
#240337=CARTESIAN_POINT('Ctrl Pts',(-18.7369005764558,17.5624418653248,
0.));
#240338=CARTESIAN_POINT('Ctrl Pts',(-18.7369005764558,17.5624418653248,
12.));
#240339=CARTESIAN_POINT('Ctrl Pts',(-18.7455592536667,17.5887568561361,
0.));
#240340=CARTESIAN_POINT('Ctrl Pts',(-18.7455592536667,17.5887568561361,
12.));
#240341=CARTESIAN_POINT('Ctrl Pts',(-18.7541806530935,17.6151583356988,
0.));
#240342=CARTESIAN_POINT('Ctrl Pts',(-18.7541806530935,17.6151583356988,
12.));
#240343=CARTESIAN_POINT('Ctrl Pts',(-18.7627643613139,17.6416459210646,
0.));
#240344=CARTESIAN_POINT('Ctrl Pts',(-18.7627643613139,17.6416459210646,
12.));
#240345=CARTESIAN_POINT('Ctrl Pts',(-18.7713099642673,17.6682192274197,
0.));
#240346=CARTESIAN_POINT('Ctrl Pts',(-18.7713099642673,17.6682192274197,
12.));
#240347=CARTESIAN_POINT('Ctrl Pts',(-18.7798170641305,17.6948778822981,
0.));
#240348=CARTESIAN_POINT('Ctrl Pts',(-18.7798170641305,17.6948778822981,
12.));
#240349=CARTESIAN_POINT('Ctrl Pts',(-18.7882852976016,17.7216215409019,
0.));
#240350=CARTESIAN_POINT('Ctrl Pts',(-18.7882852976016,17.7216215409019,
12.));
#240351=CARTESIAN_POINT('Ctrl Pts',(-18.7967143519444,17.7484498996916,
0.));
#240352=CARTESIAN_POINT('Ctrl Pts',(-18.7967143519444,17.7484498996916,
12.));
#240353=CARTESIAN_POINT('Ctrl Pts',(-18.8051039860543,17.7753627137898,
0.));
#240354=CARTESIAN_POINT('Ctrl Pts',(-18.8051039860543,17.7753627137898,
12.));
#240355=CARTESIAN_POINT('Ctrl Pts',(-18.8134540340581,17.8023598011135,
0.));
#240356=CARTESIAN_POINT('Ctrl Pts',(-18.8134540340581,17.8023598011135,
12.));
#240357=CARTESIAN_POINT('Ctrl Pts',(-18.8217643886368,17.8294410311105,
0.));
#240358=CARTESIAN_POINT('Ctrl Pts',(-18.8217643886368,17.8294410311105,
12.));
#240359=CARTESIAN_POINT('Ctrl Pts',(-18.8300349896187,17.8566063174871,
0.));
#240360=CARTESIAN_POINT('Ctrl Pts',(-18.8300349896187,17.8566063174871,
12.));
#240361=CARTESIAN_POINT('Ctrl Pts',(-18.8366196462746,17.8784057509434,
0.));
#240362=CARTESIAN_POINT('Ctrl Pts',(-18.8366196462746,17.8784057509434,
12.));
#240363=CARTESIAN_POINT('Ctrl Pts',(-18.8415402351882,17.8947931177853,
0.));
#240364=CARTESIAN_POINT('Ctrl Pts',(-18.8415402351882,17.8947931177853,
12.));
#240365=CARTESIAN_POINT('Ctrl Pts',(-18.8448126709726,17.9057348246611,
0.));
#240366=CARTESIAN_POINT('Ctrl Pts',(-18.8448126709726,17.9057348246611,
12.));
#240367=CARTESIAN_POINT('Ctrl Pts',(-18.8464468996588,17.9112098770111,
0.));
#240368=CARTESIAN_POINT('Ctrl Pts',(-18.8464468996588,17.9112098770111,
12.));
#240369=CARTESIAN_POINT('',(-18.8464468996588,17.9112098770111,0.));
#240370=CARTESIAN_POINT('Ctrl Pts',(-17.1452095830633,14.6513681262571,
0.));
#240371=CARTESIAN_POINT('Ctrl Pts',(-17.1452153999142,14.6513711852843,
0.));
#240372=CARTESIAN_POINT('Ctrl Pts',(-17.1452600887037,14.6514066997196,
0.));
#240373=CARTESIAN_POINT('Ctrl Pts',(-17.1454262858043,14.6515481598068,
0.));
#240374=CARTESIAN_POINT('Ctrl Pts',(-17.1458462295271,14.6519131634508,
0.));
#240375=CARTESIAN_POINT('Ctrl Pts',(-17.1466998098673,14.6526624064978,
0.));
#240376=CARTESIAN_POINT('Ctrl Pts',(-17.147876394491,14.6537016966184,0.));
#240377=CARTESIAN_POINT('Ctrl Pts',(-17.1493641837558,14.655024862281,0.));
#240378=CARTESIAN_POINT('Ctrl Pts',(-17.1511476869496,14.6566237952435,
0.));
#240379=CARTESIAN_POINT('Ctrl Pts',(-17.1532107762718,14.6584900555302,
0.));
#240380=CARTESIAN_POINT('Ctrl Pts',(-17.1555401986401,14.6606167169642,
0.));
#240381=CARTESIAN_POINT('Ctrl Pts',(-17.1581262646789,14.6629987285992,
0.));
#240382=CARTESIAN_POINT('Ctrl Pts',(-17.1609609517369,14.6656319165057,
0.));
#240383=CARTESIAN_POINT('Ctrl Pts',(-17.1640366762305,14.6685123374423,
0.));
#240384=CARTESIAN_POINT('Ctrl Pts',(-17.167344972302,14.671635583332,0.));
#240385=CARTESIAN_POINT('Ctrl Pts',(-17.1708771619129,14.6749971333867,
0.));
#240386=CARTESIAN_POINT('Ctrl Pts',(-17.1746247499057,14.6785925615677,
0.));
#240387=CARTESIAN_POINT('Ctrl Pts',(-17.1785800350826,14.6824178576167,
0.));
#240388=CARTESIAN_POINT('Ctrl Pts',(-17.182736158472,14.686469452232,0.));
#240389=CARTESIAN_POINT('Ctrl Pts',(-17.1870867909918,14.6907440526958,
0.));
#240390=CARTESIAN_POINT('Ctrl Pts',(-17.1916259308415,14.6952385361705,
0.));
#240391=CARTESIAN_POINT('Ctrl Pts',(-17.1963476411694,14.699949811582,0.));
#240392=CARTESIAN_POINT('Ctrl Pts',(-17.2012461084268,14.7048748502663,
0.));
#240393=CARTESIAN_POINT('Ctrl Pts',(-17.2063157097315,14.7100107213586,
0.));
#240394=CARTESIAN_POINT('Ctrl Pts',(-17.2115510835989,14.7153546289339,
0.));
#240395=CARTESIAN_POINT('Ctrl Pts',(-17.2169471814256,14.7209039390327,
0.));
#240396=CARTESIAN_POINT('Ctrl Pts',(-17.2224992099667,14.7266561494282,
0.));
#240397=CARTESIAN_POINT('Ctrl Pts',(-17.2282025904314,14.7326088681163,
0.));
#240398=CARTESIAN_POINT('Ctrl Pts',(-17.2340529062076,14.7387597858116,
0.));
#240399=CARTESIAN_POINT('Ctrl Pts',(-17.2400458713565,14.7451066593792,
0.));
#240400=CARTESIAN_POINT('Ctrl Pts',(-17.2461773413288,14.7516473175124,
0.));
#240401=CARTESIAN_POINT('Ctrl Pts',(-17.2524433146837,14.7583796616617,
0.));
#240402=CARTESIAN_POINT('Ctrl Pts',(-17.2588399401465,14.7653016697591,
0.));
#240403=CARTESIAN_POINT('Ctrl Pts',(-17.2653635155319,14.7724113956731,
0.));
#240404=CARTESIAN_POINT('Ctrl Pts',(-17.2720104735194,14.7797069617804,
0.));
#240405=CARTESIAN_POINT('Ctrl Pts',(-17.2787773704849,14.787186553128,0.));
#240406=CARTESIAN_POINT('Ctrl Pts',(-17.2856608733196,14.7948484105249,
0.));
#240407=CARTESIAN_POINT('Ctrl Pts',(-17.2926577496513,14.8026908254276,
0.));
#240408=CARTESIAN_POINT('Ctrl Pts',(-17.299764866148,14.8107121391035,0.));
#240409=CARTESIAN_POINT('Ctrl Pts',(-17.3069791853706,14.8189107410162,
0.));
#240410=CARTESIAN_POINT('Ctrl Pts',(-17.3142977632659,14.8272850675379,
0.));
#240411=CARTESIAN_POINT('Ctrl Pts',(-17.3217177462101,14.8358336004197,
0.));
#240412=CARTESIAN_POINT('Ctrl Pts',(-17.3292363662605,14.8445548643508,
0.));
#240413=CARTESIAN_POINT('Ctrl Pts',(-17.336850936485,14.8534474245433,0.));
#240414=CARTESIAN_POINT('Ctrl Pts',(-17.3445588463475,14.8625098843417,
0.));
#240415=CARTESIAN_POINT('Ctrl Pts',(-17.3523575568645,14.8717408826955,
0.));
#240416=CARTESIAN_POINT('Ctrl Pts',(-17.3602445978161,14.8811390927423,
0.));
#240417=CARTESIAN_POINT('Ctrl Pts',(-17.3682175653235,14.8907032205788,
0.));
#240418=CARTESIAN_POINT('Ctrl Pts',(-17.3762741193076,14.900432003961,0.));
#240419=CARTESIAN_POINT('Ctrl Pts',(-17.3844119809824,14.9103242110057,
0.));
#240420=CARTESIAN_POINT('Ctrl Pts',(-17.3926289303986,14.9203786389342,
0.));
#240421=CARTESIAN_POINT('Ctrl Pts',(-17.4009228040749,14.9305941128757,
0.));
#240422=CARTESIAN_POINT('Ctrl Pts',(-17.4092914926071,14.940969484645,0.));
#240423=CARTESIAN_POINT('Ctrl Pts',(-17.4177329382828,14.9515036315143,
0.));
#240424=CARTESIAN_POINT('Ctrl Pts',(-17.426245132709,14.9621954549827,0.));
#240425=CARTESIAN_POINT('Ctrl Pts',(-17.4348261151396,14.9730438799452,
0.));
#240426=CARTESIAN_POINT('Ctrl Pts',(-17.4434739707773,14.9840478538358,
0.));
#240427=CARTESIAN_POINT('Ctrl Pts',(-17.4521868291004,14.9952063457778,
0.));
#240428=CARTESIAN_POINT('Ctrl Pts',(-17.4609628621418,15.0065183456921,
0.));
#240429=CARTESIAN_POINT('Ctrl Pts',(-17.4698002829357,15.0179828635086,
0.));
#240430=CARTESIAN_POINT('Ctrl Pts',(-17.4786973441417,15.029598928488,0.));
#240431=CARTESIAN_POINT('Ctrl Pts',(-17.4876523366178,15.0413655884993,
0.));
#240432=CARTESIAN_POINT('Ctrl Pts',(-17.4966635880245,15.0532819093085,
0.));
#240433=CARTESIAN_POINT('Ctrl Pts',(-17.5057294613874,15.0653469738306,
0.));
#240434=CARTESIAN_POINT('Ctrl Pts',(-17.5148483539684,15.0775598815748,
0.));
#240435=CARTESIAN_POINT('Ctrl Pts',(-17.5240186961788,15.0899197481082,
0.));
#240436=CARTESIAN_POINT('Ctrl Pts',(-17.5332389504829,15.1024257045033,
0.));
#240437=CARTESIAN_POINT('Ctrl Pts',(-17.5425076102966,15.1150768967729,
0.));
#240438=CARTESIAN_POINT('Ctrl Pts',(-17.5518231989122,15.127872485314,0.));
#240439=CARTESIAN_POINT('Ctrl Pts',(-17.5611842686196,15.1408116444877,
0.));
#240440=CARTESIAN_POINT('Ctrl Pts',(-17.570589399803,15.1538935621714,0.));
#240441=CARTESIAN_POINT('Ctrl Pts',(-17.5800372000539,15.1671174393136,
0.));
#240442=CARTESIAN_POINT('Ctrl Pts',(-17.5895263032592,15.1804824894605,
0.));
#240443=CARTESIAN_POINT('Ctrl Pts',(-17.5990553687595,15.1939879383268,
0.));
#240444=CARTESIAN_POINT('Ctrl Pts',(-17.6086230806497,15.2076330234686,
0.));
#240445=CARTESIAN_POINT('Ctrl Pts',(-17.6182281470467,15.22141699392,0.));
#240446=CARTESIAN_POINT('Ctrl Pts',(-17.6278692993765,15.2353391098367,
0.));
#240447=CARTESIAN_POINT('Ctrl Pts',(-17.637545291637,15.2493986421091,0.));
#240448=CARTESIAN_POINT('Ctrl Pts',(-17.6472548997329,15.263594872029,0.));
#240449=CARTESIAN_POINT('Ctrl Pts',(-17.6569969209,15.2779270910238,0.));
#240450=CARTESIAN_POINT('Ctrl Pts',(-17.6667701731041,15.2923946003598,
0.));
#240451=CARTESIAN_POINT('Ctrl Pts',(-17.6765734944559,15.3069967108501,
0.));
#240452=CARTESIAN_POINT('Ctrl Pts',(-17.6864057426052,15.3217327425341,
0.));
#240453=CARTESIAN_POINT('Ctrl Pts',(-17.6962657941984,15.3366020244069,
0.));
#240454=CARTESIAN_POINT('Ctrl Pts',(-17.7061525444044,15.3516038942064,
0.));
#240455=CARTESIAN_POINT('Ctrl Pts',(-17.7160649064208,15.3667376981702,
0.));
#240456=CARTESIAN_POINT('Ctrl Pts',(-17.7260018109923,15.3820027907965,
0.));
#240457=CARTESIAN_POINT('Ctrl Pts',(-17.7359622059143,15.3973985345796,
0.));
#240458=CARTESIAN_POINT('Ctrl Pts',(-17.7459450555803,15.4129242997828,
0.));
#240459=CARTESIAN_POINT('Ctrl Pts',(-17.7559493405871,15.4285794642658,
0.));
#240460=CARTESIAN_POINT('Ctrl Pts',(-17.765974057326,15.4443634132865,0.));
#240461=CARTESIAN_POINT('Ctrl Pts',(-17.7760182175817,15.4602755393019,
0.));
#240462=CARTESIAN_POINT('Ctrl Pts',(-17.7860808481229,15.4763152417506,
0.));
#240463=CARTESIAN_POINT('Ctrl Pts',(-17.7961609903161,15.4924819268529,
0.));
#240464=CARTESIAN_POINT('Ctrl Pts',(-17.8062576997964,15.5087750074728,
0.));
#240465=CARTESIAN_POINT('Ctrl Pts',(-17.8163700461263,15.5251939029558,
0.));
#240466=CARTESIAN_POINT('Ctrl Pts',(-17.8264971124606,15.5417380389639,
0.));
#240467=CARTESIAN_POINT('Ctrl Pts',(-17.8366379952078,15.5584068472976,
0.));
#240468=CARTESIAN_POINT('Ctrl Pts',(-17.8467918036977,15.5751997657153,
0.));
#240469=CARTESIAN_POINT('Ctrl Pts',(-17.8569576598996,15.5921162378183,
0.));
#240470=CARTESIAN_POINT('Ctrl Pts',(-17.8671346981388,15.6091557129205,
0.));
#240471=CARTESIAN_POINT('Ctrl Pts',(-17.8773220648125,15.6263176459107,
0.));
#240472=CARTESIAN_POINT('Ctrl Pts',(-17.8875189181095,15.6436014971088,
0.));
#240473=CARTESIAN_POINT('Ctrl Pts',(-17.8977244277247,15.6610067321036,
0.));
#240474=CARTESIAN_POINT('Ctrl Pts',(-17.9079377746118,15.6785328216467,
0.));
#240475=CARTESIAN_POINT('Ctrl Pts',(-17.918158150746,15.6961792415526,0.));
#240476=CARTESIAN_POINT('Ctrl Pts',(-17.9283847588837,15.713945472584,0.));
#240477=CARTESIAN_POINT('Ctrl Pts',(-17.9386168123261,15.7318310003334,
0.));
#240478=CARTESIAN_POINT('Ctrl Pts',(-17.9488535346776,15.7498353150856,
0.));
#240479=CARTESIAN_POINT('Ctrl Pts',(-17.9590941596236,15.7679579117072,
0.));
#240480=CARTESIAN_POINT('Ctrl Pts',(-17.9693379307297,15.786198289572,0.));
#240481=CARTESIAN_POINT('Ctrl Pts',(-17.9795841012383,15.8045559524674,
0.));
#240482=CARTESIAN_POINT('Ctrl Pts',(-17.9898319338664,15.8230304084963,
0.));
#240483=CARTESIAN_POINT('Ctrl Pts',(-18.0000807006055,15.8416211699681,
0.));
#240484=CARTESIAN_POINT('Ctrl Pts',(-18.010329682521,15.8603277532834,0.));
#240485=CARTESIAN_POINT('Ctrl Pts',(-18.0205781695773,15.8791496788685,
0.));
#240486=CARTESIAN_POINT('Ctrl Pts',(-18.0308254604638,15.8980864711043,
0.));
#240487=CARTESIAN_POINT('Ctrl Pts',(-18.0410708624208,15.9171376582436,
0.));
#240488=CARTESIAN_POINT('Ctrl Pts',(-18.0513136910691,15.9363027723244,
0.));
#240489=CARTESIAN_POINT('Ctrl Pts',(-18.061553270236,15.9555813490645,0.));
#240490=CARTESIAN_POINT('Ctrl Pts',(-18.071788931796,15.9749729277848,0.));
#240491=CARTESIAN_POINT('Ctrl Pts',(-18.0820200155239,15.9944770513616,
0.));
#240492=CARTESIAN_POINT('Ctrl Pts',(-18.0922458689464,16.0140932661612,
0.));
#240493=CARTESIAN_POINT('Ctrl Pts',(-18.1024658471966,16.0338211219693,
0.));
#240494=CARTESIAN_POINT('Ctrl Pts',(-18.1126793128688,16.0536601719124,
0.));
#240495=CARTESIAN_POINT('Ctrl Pts',(-18.1228856358746,16.0736099723664,
0.));
#240496=CARTESIAN_POINT('Ctrl Pts',(-18.1330841933099,16.0936700829108,
0.));
#240497=CARTESIAN_POINT('Ctrl Pts',(-18.1432743693231,16.113840066279,0.));
#240498=CARTESIAN_POINT('Ctrl Pts',(-18.1534555549851,16.1341194882987,
0.));
#240499=CARTESIAN_POINT('Ctrl Pts',(-18.1636271481616,16.1545079178261,
0.));
#240500=CARTESIAN_POINT('Ctrl Pts',(-18.1737885533852,16.1750049266673,
0.));
#240501=CARTESIAN_POINT('Ctrl Pts',(-18.1839391817335,16.1956100895076,
0.));
#240502=CARTESIAN_POINT('Ctrl Pts',(-18.1940784507232,16.2163229838878,
0.));
#240503=CARTESIAN_POINT('Ctrl Pts',(-18.2042057842037,16.237143190164,0.));
#240504=CARTESIAN_POINT('Ctrl Pts',(-18.214320612253,16.2580702914615,0.));
#240505=CARTESIAN_POINT('Ctrl Pts',(-18.2244223710745,16.2791038736223,
0.));
#240506=CARTESIAN_POINT('Ctrl Pts',(-18.2345105028981,16.3002435251378,
0.));
#240507=CARTESIAN_POINT('Ctrl Pts',(-18.2445844558742,16.3214888370988,
0.));
#240508=CARTESIAN_POINT('Ctrl Pts',(-18.2546436839609,16.342839403159,0.));
#240509=CARTESIAN_POINT('Ctrl Pts',(-18.2646876468169,16.3642948194869,
0.));
#240510=CARTESIAN_POINT('Ctrl Pts',(-18.2747158096934,16.385854684708,0.));
#240511=CARTESIAN_POINT('Ctrl Pts',(-18.2847276433308,16.4075185998454,
0.));
#240512=CARTESIAN_POINT('Ctrl Pts',(-18.2947226238509,16.4292861682377,
0.));
#240513=CARTESIAN_POINT('Ctrl Pts',(-18.3047002326858,16.4511569955231,
0.));
#240514=CARTESIAN_POINT('Ctrl Pts',(-18.3146599565229,16.4731306896439,
0.));
#240515=CARTESIAN_POINT('Ctrl Pts',(-18.3246012872468,16.4952068608344,
0.));
#240516=CARTESIAN_POINT('Ctrl Pts',(-18.3345237218864,16.5173851216045,
0.));
#240517=CARTESIAN_POINT('Ctrl Pts',(-18.3444267625601,16.5396650867139,
0.));
#240518=CARTESIAN_POINT('Ctrl Pts',(-18.3543099164331,16.5620463731414,
0.));
#240519=CARTESIAN_POINT('Ctrl Pts',(-18.364172695589,16.5845286000218,0.));
#240520=CARTESIAN_POINT('Ctrl Pts',(-18.3740146168879,16.6071113885711,
0.));
#240521=CARTESIAN_POINT('Ctrl Pts',(-18.3838352018327,16.6297943620056,
0.));
#240522=CARTESIAN_POINT('Ctrl Pts',(-18.3936339764332,16.6525771454513,
0.));
#240523=CARTESIAN_POINT('Ctrl Pts',(-18.4034104710789,16.6754593658513,
0.));
#240524=CARTESIAN_POINT('Ctrl Pts',(-18.413164220399,16.698440651849,0.));
#240525=CARTESIAN_POINT('Ctrl Pts',(-18.4228947633186,16.7215206338818,
0.));
#240526=CARTESIAN_POINT('Ctrl Pts',(-18.4326016431392,16.7446989442882,
0.));
#240527=CARTESIAN_POINT('Ctrl Pts',(-18.4422844076099,16.7679752173992,
0.));
#240528=CARTESIAN_POINT('Ctrl Pts',(-18.4519426090124,16.791349089629,0.));
#240529=CARTESIAN_POINT('Ctrl Pts',(-18.4615758042305,16.8148201995472,
0.));
#240530=CARTESIAN_POINT('Ctrl Pts',(-18.4711835548622,16.8383881879707,
0.));
#240531=CARTESIAN_POINT('Ctrl Pts',(-18.4807654268769,16.8620526977169,
0.));
#240532=CARTESIAN_POINT('Ctrl Pts',(-18.4903209902226,16.8858133733086,
0.));
#240533=CARTESIAN_POINT('Ctrl Pts',(-18.4998498184619,16.9096698606942,
0.));
#240534=CARTESIAN_POINT('Ctrl Pts',(-18.5093514883835,16.9336218069353,
0.));
#240535=CARTESIAN_POINT('Ctrl Pts',(-18.518825579666,16.957668859934,0.));
#240536=CARTESIAN_POINT('Ctrl Pts',(-18.5282716744198,16.9818106680382,
0.));
#240537=CARTESIAN_POINT('Ctrl Pts',(-18.5376893576961,17.0060468805099,
0.));
#240538=CARTESIAN_POINT('Ctrl Pts',(-18.5470782182089,17.030377148174,0.));
#240539=CARTESIAN_POINT('Ctrl Pts',(-18.5564378489628,17.0548011239751,
0.));
#240540=CARTESIAN_POINT('Ctrl Pts',(-18.5657678479788,17.0793184636079,
0.));
#240541=CARTESIAN_POINT('Ctrl Pts',(-18.5750678188543,17.1039288260001,
0.));
#240542=CARTESIAN_POINT('Ctrl Pts',(-18.5843373717253,17.1286318741185,
0.));
#240543=CARTESIAN_POINT('Ctrl Pts',(-18.5935761222833,17.1534272741646,
0.));
#240544=CARTESIAN_POINT('Ctrl Pts',(-18.6027836898826,17.1783146940131,
0.));
#240545=CARTESIAN_POINT('Ctrl Pts',(-18.6119596959957,17.2032938019288,
0.));
#240546=CARTESIAN_POINT('Ctrl Pts',(-18.6211037624041,17.2283642650519,
0.));
#240547=CARTESIAN_POINT('Ctrl Pts',(-18.630215509794,17.2535257482186,0.));
#240548=CARTESIAN_POINT('Ctrl Pts',(-18.639294555474,17.278777912021,0.));
#240549=CARTESIAN_POINT('Ctrl Pts',(-18.6483405141853,17.3041204135069,
0.));
#240550=CARTESIAN_POINT('Ctrl Pts',(-18.6573530024019,17.3295529098612,
0.));
#240551=CARTESIAN_POINT('Ctrl Pts',(-18.6663316416569,17.3550750612438,
0.));
#240552=CARTESIAN_POINT('Ctrl Pts',(-18.6752760624045,17.3806865340744,
0.));
#240553=CARTESIAN_POINT('Ctrl Pts',(-18.6841859073472,17.4063870038563,
0.));
#240554=CARTESIAN_POINT('Ctrl Pts',(-18.6930608357421,17.4321761588148,
0.));
#240555=CARTESIAN_POINT('Ctrl Pts',(-18.7019005250322,17.4580537012764,
0.));
#240556=CARTESIAN_POINT('Ctrl Pts',(-18.7107046613941,17.4840193397176,
0.));
#240557=CARTESIAN_POINT('Ctrl Pts',(-18.7194729318128,17.5100727820891,
0.));
#240558=CARTESIAN_POINT('Ctrl Pts',(-18.728205015716,17.5362137287604,0.));
#240559=CARTESIAN_POINT('Ctrl Pts',(-18.7369005764558,17.5624418653248,
0.));
#240560=CARTESIAN_POINT('Ctrl Pts',(-18.7455592536667,17.5887568561361,
0.));
#240561=CARTESIAN_POINT('Ctrl Pts',(-18.7541806530935,17.6151583356988,
0.));
#240562=CARTESIAN_POINT('Ctrl Pts',(-18.7627643613139,17.6416459210646,
0.));
#240563=CARTESIAN_POINT('Ctrl Pts',(-18.7713099642673,17.6682192274197,
0.));
#240564=CARTESIAN_POINT('Ctrl Pts',(-18.7798170641305,17.6948778822981,
0.));
#240565=CARTESIAN_POINT('Ctrl Pts',(-18.7882852976016,17.7216215409019,
0.));
#240566=CARTESIAN_POINT('Ctrl Pts',(-18.7967143519444,17.7484498996916,
0.));
#240567=CARTESIAN_POINT('Ctrl Pts',(-18.8051039860543,17.7753627137898,
0.));
#240568=CARTESIAN_POINT('Ctrl Pts',(-18.8134540340581,17.8023598011135,
0.));
#240569=CARTESIAN_POINT('Ctrl Pts',(-18.8217643886368,17.8294410311105,
0.));
#240570=CARTESIAN_POINT('Ctrl Pts',(-18.8300349896187,17.8566063174871,
0.));
#240571=CARTESIAN_POINT('Ctrl Pts',(-18.8366196462746,17.8784057509434,
0.));
#240572=CARTESIAN_POINT('Ctrl Pts',(-18.8415402351882,17.8947931177853,
0.));
#240573=CARTESIAN_POINT('Ctrl Pts',(-18.8448126709726,17.9057348246611,
0.));
#240574=CARTESIAN_POINT('Ctrl Pts',(-18.8464468996588,17.9112098770111,
0.));
#240575=CARTESIAN_POINT('',(-18.8464468996588,17.9112098770111,12.));
#240576=CARTESIAN_POINT('Ctrl Pts',(-18.8464468996588,17.9112098770111,
12.));
#240577=CARTESIAN_POINT('Ctrl Pts',(-18.8448126709726,17.9057348246611,
12.));
#240578=CARTESIAN_POINT('Ctrl Pts',(-18.8415402351882,17.8947931177853,
12.));
#240579=CARTESIAN_POINT('Ctrl Pts',(-18.8366196462746,17.8784057509434,
12.));
#240580=CARTESIAN_POINT('Ctrl Pts',(-18.8300349896187,17.8566063174871,
12.));
#240581=CARTESIAN_POINT('Ctrl Pts',(-18.8217643886368,17.8294410311105,
12.));
#240582=CARTESIAN_POINT('Ctrl Pts',(-18.8134540340581,17.8023598011135,
12.));
#240583=CARTESIAN_POINT('Ctrl Pts',(-18.8051039860543,17.7753627137898,
12.));
#240584=CARTESIAN_POINT('Ctrl Pts',(-18.7967143519444,17.7484498996916,
12.));
#240585=CARTESIAN_POINT('Ctrl Pts',(-18.7882852976016,17.7216215409019,
12.));
#240586=CARTESIAN_POINT('Ctrl Pts',(-18.7798170641305,17.6948778822981,
12.));
#240587=CARTESIAN_POINT('Ctrl Pts',(-18.7713099642673,17.6682192274197,
12.));
#240588=CARTESIAN_POINT('Ctrl Pts',(-18.7627643613139,17.6416459210646,
12.));
#240589=CARTESIAN_POINT('Ctrl Pts',(-18.7541806530935,17.6151583356988,
12.));
#240590=CARTESIAN_POINT('Ctrl Pts',(-18.7455592536667,17.5887568561361,
12.));
#240591=CARTESIAN_POINT('Ctrl Pts',(-18.7369005764558,17.5624418653248,
12.));
#240592=CARTESIAN_POINT('Ctrl Pts',(-18.728205015716,17.5362137287604,12.));
#240593=CARTESIAN_POINT('Ctrl Pts',(-18.7194729318128,17.5100727820891,
12.));
#240594=CARTESIAN_POINT('Ctrl Pts',(-18.7107046613941,17.4840193397176,
12.));
#240595=CARTESIAN_POINT('Ctrl Pts',(-18.7019005250322,17.4580537012764,
12.));
#240596=CARTESIAN_POINT('Ctrl Pts',(-18.6930608357421,17.4321761588148,
12.));
#240597=CARTESIAN_POINT('Ctrl Pts',(-18.6841859073472,17.4063870038563,
12.));
#240598=CARTESIAN_POINT('Ctrl Pts',(-18.6752760624045,17.3806865340744,
12.));
#240599=CARTESIAN_POINT('Ctrl Pts',(-18.6663316416569,17.3550750612438,
12.));
#240600=CARTESIAN_POINT('Ctrl Pts',(-18.6573530024019,17.3295529098612,
12.));
#240601=CARTESIAN_POINT('Ctrl Pts',(-18.6483405141853,17.3041204135069,
12.));
#240602=CARTESIAN_POINT('Ctrl Pts',(-18.639294555474,17.278777912021,12.));
#240603=CARTESIAN_POINT('Ctrl Pts',(-18.630215509794,17.2535257482186,12.));
#240604=CARTESIAN_POINT('Ctrl Pts',(-18.6211037624041,17.2283642650519,
12.));
#240605=CARTESIAN_POINT('Ctrl Pts',(-18.6119596959957,17.2032938019288,
12.));
#240606=CARTESIAN_POINT('Ctrl Pts',(-18.6027836898826,17.1783146940131,
12.));
#240607=CARTESIAN_POINT('Ctrl Pts',(-18.5935761222833,17.1534272741646,
12.));
#240608=CARTESIAN_POINT('Ctrl Pts',(-18.5843373717253,17.1286318741185,
12.));
#240609=CARTESIAN_POINT('Ctrl Pts',(-18.5750678188543,17.1039288260001,
12.));
#240610=CARTESIAN_POINT('Ctrl Pts',(-18.5657678479788,17.0793184636079,
12.));
#240611=CARTESIAN_POINT('Ctrl Pts',(-18.5564378489628,17.0548011239751,
12.));
#240612=CARTESIAN_POINT('Ctrl Pts',(-18.5470782182089,17.030377148174,12.));
#240613=CARTESIAN_POINT('Ctrl Pts',(-18.5376893576961,17.0060468805099,
12.));
#240614=CARTESIAN_POINT('Ctrl Pts',(-18.5282716744198,16.9818106680382,
12.));
#240615=CARTESIAN_POINT('Ctrl Pts',(-18.518825579666,16.957668859934,12.));
#240616=CARTESIAN_POINT('Ctrl Pts',(-18.5093514883835,16.9336218069353,
12.));
#240617=CARTESIAN_POINT('Ctrl Pts',(-18.4998498184619,16.9096698606942,
12.));
#240618=CARTESIAN_POINT('Ctrl Pts',(-18.4903209902226,16.8858133733086,
12.));
#240619=CARTESIAN_POINT('Ctrl Pts',(-18.4807654268769,16.8620526977169,
12.));
#240620=CARTESIAN_POINT('Ctrl Pts',(-18.4711835548622,16.8383881879707,
12.));
#240621=CARTESIAN_POINT('Ctrl Pts',(-18.4615758042305,16.8148201995472,
12.));
#240622=CARTESIAN_POINT('Ctrl Pts',(-18.4519426090124,16.791349089629,12.));
#240623=CARTESIAN_POINT('Ctrl Pts',(-18.4422844076099,16.7679752173992,
12.));
#240624=CARTESIAN_POINT('Ctrl Pts',(-18.4326016431392,16.7446989442882,
12.));
#240625=CARTESIAN_POINT('Ctrl Pts',(-18.4228947633186,16.7215206338818,
12.));
#240626=CARTESIAN_POINT('Ctrl Pts',(-18.413164220399,16.698440651849,12.));
#240627=CARTESIAN_POINT('Ctrl Pts',(-18.4034104710789,16.6754593658513,
12.));
#240628=CARTESIAN_POINT('Ctrl Pts',(-18.3936339764332,16.6525771454513,
12.));
#240629=CARTESIAN_POINT('Ctrl Pts',(-18.3838352018327,16.6297943620056,
12.));
#240630=CARTESIAN_POINT('Ctrl Pts',(-18.3740146168879,16.6071113885711,
12.));
#240631=CARTESIAN_POINT('Ctrl Pts',(-18.364172695589,16.5845286000218,12.));
#240632=CARTESIAN_POINT('Ctrl Pts',(-18.3543099164331,16.5620463731414,
12.));
#240633=CARTESIAN_POINT('Ctrl Pts',(-18.3444267625601,16.5396650867139,
12.));
#240634=CARTESIAN_POINT('Ctrl Pts',(-18.3345237218864,16.5173851216045,
12.));
#240635=CARTESIAN_POINT('Ctrl Pts',(-18.3246012872468,16.4952068608344,
12.));
#240636=CARTESIAN_POINT('Ctrl Pts',(-18.3146599565229,16.4731306896439,
12.));
#240637=CARTESIAN_POINT('Ctrl Pts',(-18.3047002326858,16.4511569955231,
12.));
#240638=CARTESIAN_POINT('Ctrl Pts',(-18.2947226238509,16.4292861682377,
12.));
#240639=CARTESIAN_POINT('Ctrl Pts',(-18.2847276433308,16.4075185998454,
12.));
#240640=CARTESIAN_POINT('Ctrl Pts',(-18.2747158096934,16.385854684708,12.));
#240641=CARTESIAN_POINT('Ctrl Pts',(-18.2646876468169,16.3642948194869,
12.));
#240642=CARTESIAN_POINT('Ctrl Pts',(-18.2546436839609,16.342839403159,12.));
#240643=CARTESIAN_POINT('Ctrl Pts',(-18.2445844558742,16.3214888370988,
12.));
#240644=CARTESIAN_POINT('Ctrl Pts',(-18.2345105028981,16.3002435251378,
12.));
#240645=CARTESIAN_POINT('Ctrl Pts',(-18.2244223710745,16.2791038736223,
12.));
#240646=CARTESIAN_POINT('Ctrl Pts',(-18.214320612253,16.2580702914615,12.));
#240647=CARTESIAN_POINT('Ctrl Pts',(-18.2042057842037,16.237143190164,12.));
#240648=CARTESIAN_POINT('Ctrl Pts',(-18.1940784507232,16.2163229838878,
12.));
#240649=CARTESIAN_POINT('Ctrl Pts',(-18.1839391817335,16.1956100895076,
12.));
#240650=CARTESIAN_POINT('Ctrl Pts',(-18.1737885533852,16.1750049266673,
12.));
#240651=CARTESIAN_POINT('Ctrl Pts',(-18.1636271481616,16.1545079178261,
12.));
#240652=CARTESIAN_POINT('Ctrl Pts',(-18.1534555549851,16.1341194882987,
12.));
#240653=CARTESIAN_POINT('Ctrl Pts',(-18.1432743693231,16.113840066279,12.));
#240654=CARTESIAN_POINT('Ctrl Pts',(-18.1330841933099,16.0936700829108,
12.));
#240655=CARTESIAN_POINT('Ctrl Pts',(-18.1228856358746,16.0736099723664,
12.));
#240656=CARTESIAN_POINT('Ctrl Pts',(-18.1126793128688,16.0536601719124,
12.));
#240657=CARTESIAN_POINT('Ctrl Pts',(-18.1024658471966,16.0338211219693,
12.));
#240658=CARTESIAN_POINT('Ctrl Pts',(-18.0922458689464,16.0140932661612,
12.));
#240659=CARTESIAN_POINT('Ctrl Pts',(-18.0820200155239,15.9944770513616,
12.));
#240660=CARTESIAN_POINT('Ctrl Pts',(-18.071788931796,15.9749729277848,12.));
#240661=CARTESIAN_POINT('Ctrl Pts',(-18.061553270236,15.9555813490645,12.));
#240662=CARTESIAN_POINT('Ctrl Pts',(-18.0513136910691,15.9363027723244,
12.));
#240663=CARTESIAN_POINT('Ctrl Pts',(-18.0410708624208,15.9171376582436,
12.));
#240664=CARTESIAN_POINT('Ctrl Pts',(-18.0308254604638,15.8980864711043,
12.));
#240665=CARTESIAN_POINT('Ctrl Pts',(-18.0205781695773,15.8791496788685,
12.));
#240666=CARTESIAN_POINT('Ctrl Pts',(-18.010329682521,15.8603277532834,12.));
#240667=CARTESIAN_POINT('Ctrl Pts',(-18.0000807006055,15.8416211699681,
12.));
#240668=CARTESIAN_POINT('Ctrl Pts',(-17.9898319338664,15.8230304084963,
12.));
#240669=CARTESIAN_POINT('Ctrl Pts',(-17.9795841012383,15.8045559524674,
12.));
#240670=CARTESIAN_POINT('Ctrl Pts',(-17.9693379307297,15.786198289572,12.));
#240671=CARTESIAN_POINT('Ctrl Pts',(-17.9590941596236,15.7679579117072,
12.));
#240672=CARTESIAN_POINT('Ctrl Pts',(-17.9488535346776,15.7498353150856,
12.));
#240673=CARTESIAN_POINT('Ctrl Pts',(-17.9386168123261,15.7318310003334,
12.));
#240674=CARTESIAN_POINT('Ctrl Pts',(-17.9283847588837,15.713945472584,12.));
#240675=CARTESIAN_POINT('Ctrl Pts',(-17.918158150746,15.6961792415526,12.));
#240676=CARTESIAN_POINT('Ctrl Pts',(-17.9079377746118,15.6785328216467,
12.));
#240677=CARTESIAN_POINT('Ctrl Pts',(-17.8977244277247,15.6610067321036,
12.));
#240678=CARTESIAN_POINT('Ctrl Pts',(-17.8875189181095,15.6436014971088,
12.));
#240679=CARTESIAN_POINT('Ctrl Pts',(-17.8773220648125,15.6263176459107,
12.));
#240680=CARTESIAN_POINT('Ctrl Pts',(-17.8671346981388,15.6091557129205,
12.));
#240681=CARTESIAN_POINT('Ctrl Pts',(-17.8569576598996,15.5921162378183,
12.));
#240682=CARTESIAN_POINT('Ctrl Pts',(-17.8467918036977,15.5751997657153,
12.));
#240683=CARTESIAN_POINT('Ctrl Pts',(-17.8366379952078,15.5584068472976,
12.));
#240684=CARTESIAN_POINT('Ctrl Pts',(-17.8264971124606,15.5417380389639,
12.));
#240685=CARTESIAN_POINT('Ctrl Pts',(-17.8163700461263,15.5251939029558,
12.));
#240686=CARTESIAN_POINT('Ctrl Pts',(-17.8062576997964,15.5087750074728,
12.));
#240687=CARTESIAN_POINT('Ctrl Pts',(-17.7961609903161,15.4924819268529,
12.));
#240688=CARTESIAN_POINT('Ctrl Pts',(-17.7860808481229,15.4763152417506,
12.));
#240689=CARTESIAN_POINT('Ctrl Pts',(-17.7760182175817,15.4602755393019,
12.));
#240690=CARTESIAN_POINT('Ctrl Pts',(-17.765974057326,15.4443634132865,12.));
#240691=CARTESIAN_POINT('Ctrl Pts',(-17.7559493405871,15.4285794642658,
12.));
#240692=CARTESIAN_POINT('Ctrl Pts',(-17.7459450555803,15.4129242997828,
12.));
#240693=CARTESIAN_POINT('Ctrl Pts',(-17.7359622059143,15.3973985345796,
12.));
#240694=CARTESIAN_POINT('Ctrl Pts',(-17.7260018109923,15.3820027907965,
12.));
#240695=CARTESIAN_POINT('Ctrl Pts',(-17.7160649064208,15.3667376981702,
12.));
#240696=CARTESIAN_POINT('Ctrl Pts',(-17.7061525444044,15.3516038942064,
12.));
#240697=CARTESIAN_POINT('Ctrl Pts',(-17.6962657941984,15.3366020244069,
12.));
#240698=CARTESIAN_POINT('Ctrl Pts',(-17.6864057426052,15.3217327425341,
12.));
#240699=CARTESIAN_POINT('Ctrl Pts',(-17.6765734944559,15.3069967108501,
12.));
#240700=CARTESIAN_POINT('Ctrl Pts',(-17.6667701731041,15.2923946003598,
12.));
#240701=CARTESIAN_POINT('Ctrl Pts',(-17.6569969209,15.2779270910238,12.));
#240702=CARTESIAN_POINT('Ctrl Pts',(-17.6472548997329,15.263594872029,12.));
#240703=CARTESIAN_POINT('Ctrl Pts',(-17.637545291637,15.2493986421091,12.));
#240704=CARTESIAN_POINT('Ctrl Pts',(-17.6278692993765,15.2353391098367,
12.));
#240705=CARTESIAN_POINT('Ctrl Pts',(-17.6182281470467,15.22141699392,12.));
#240706=CARTESIAN_POINT('Ctrl Pts',(-17.6086230806497,15.2076330234686,
12.));
#240707=CARTESIAN_POINT('Ctrl Pts',(-17.5990553687595,15.1939879383268,
12.));
#240708=CARTESIAN_POINT('Ctrl Pts',(-17.5895263032592,15.1804824894605,
12.));
#240709=CARTESIAN_POINT('Ctrl Pts',(-17.5800372000539,15.1671174393136,
12.));
#240710=CARTESIAN_POINT('Ctrl Pts',(-17.570589399803,15.1538935621714,12.));
#240711=CARTESIAN_POINT('Ctrl Pts',(-17.5611842686196,15.1408116444877,
12.));
#240712=CARTESIAN_POINT('Ctrl Pts',(-17.5518231989122,15.127872485314,12.));
#240713=CARTESIAN_POINT('Ctrl Pts',(-17.5425076102966,15.1150768967729,
12.));
#240714=CARTESIAN_POINT('Ctrl Pts',(-17.5332389504829,15.1024257045033,
12.));
#240715=CARTESIAN_POINT('Ctrl Pts',(-17.5240186961788,15.0899197481082,
12.));
#240716=CARTESIAN_POINT('Ctrl Pts',(-17.5148483539684,15.0775598815748,
12.));
#240717=CARTESIAN_POINT('Ctrl Pts',(-17.5057294613874,15.0653469738306,
12.));
#240718=CARTESIAN_POINT('Ctrl Pts',(-17.4966635880245,15.0532819093085,
12.));
#240719=CARTESIAN_POINT('Ctrl Pts',(-17.4876523366178,15.0413655884993,
12.));
#240720=CARTESIAN_POINT('Ctrl Pts',(-17.4786973441417,15.029598928488,12.));
#240721=CARTESIAN_POINT('Ctrl Pts',(-17.4698002829357,15.0179828635086,
12.));
#240722=CARTESIAN_POINT('Ctrl Pts',(-17.4609628621418,15.0065183456921,
12.));
#240723=CARTESIAN_POINT('Ctrl Pts',(-17.4521868291004,14.9952063457778,
12.));
#240724=CARTESIAN_POINT('Ctrl Pts',(-17.4434739707773,14.9840478538358,
12.));
#240725=CARTESIAN_POINT('Ctrl Pts',(-17.4348261151396,14.9730438799452,
12.));
#240726=CARTESIAN_POINT('Ctrl Pts',(-17.426245132709,14.9621954549827,12.));
#240727=CARTESIAN_POINT('Ctrl Pts',(-17.4177329382828,14.9515036315143,
12.));
#240728=CARTESIAN_POINT('Ctrl Pts',(-17.4092914926071,14.940969484645,12.));
#240729=CARTESIAN_POINT('Ctrl Pts',(-17.4009228040749,14.9305941128757,
12.));
#240730=CARTESIAN_POINT('Ctrl Pts',(-17.3926289303986,14.9203786389342,
12.));
#240731=CARTESIAN_POINT('Ctrl Pts',(-17.3844119809824,14.9103242110057,
12.));
#240732=CARTESIAN_POINT('Ctrl Pts',(-17.3762741193076,14.900432003961,12.));
#240733=CARTESIAN_POINT('Ctrl Pts',(-17.3682175653235,14.8907032205788,
12.));
#240734=CARTESIAN_POINT('Ctrl Pts',(-17.3602445978161,14.8811390927423,
12.));
#240735=CARTESIAN_POINT('Ctrl Pts',(-17.3523575568645,14.8717408826955,
12.));
#240736=CARTESIAN_POINT('Ctrl Pts',(-17.3445588463475,14.8625098843417,
12.));
#240737=CARTESIAN_POINT('Ctrl Pts',(-17.336850936485,14.8534474245433,12.));
#240738=CARTESIAN_POINT('Ctrl Pts',(-17.3292363662605,14.8445548643508,
12.));
#240739=CARTESIAN_POINT('Ctrl Pts',(-17.3217177462101,14.8358336004197,
12.));
#240740=CARTESIAN_POINT('Ctrl Pts',(-17.3142977632659,14.8272850675379,
12.));
#240741=CARTESIAN_POINT('Ctrl Pts',(-17.3069791853706,14.8189107410162,
12.));
#240742=CARTESIAN_POINT('Ctrl Pts',(-17.299764866148,14.8107121391035,12.));
#240743=CARTESIAN_POINT('Ctrl Pts',(-17.2926577496513,14.8026908254276,
12.));
#240744=CARTESIAN_POINT('Ctrl Pts',(-17.2856608733196,14.7948484105249,
12.));
#240745=CARTESIAN_POINT('Ctrl Pts',(-17.2787773704849,14.787186553128,12.));
#240746=CARTESIAN_POINT('Ctrl Pts',(-17.2720104735194,14.7797069617804,
12.));
#240747=CARTESIAN_POINT('Ctrl Pts',(-17.2653635155319,14.7724113956731,
12.));
#240748=CARTESIAN_POINT('Ctrl Pts',(-17.2588399401465,14.7653016697591,
12.));
#240749=CARTESIAN_POINT('Ctrl Pts',(-17.2524433146837,14.7583796616617,
12.));
#240750=CARTESIAN_POINT('Ctrl Pts',(-17.2461773413288,14.7516473175124,
12.));
#240751=CARTESIAN_POINT('Ctrl Pts',(-17.2400458713565,14.7451066593792,
12.));
#240752=CARTESIAN_POINT('Ctrl Pts',(-17.2340529062076,14.7387597858116,
12.));
#240753=CARTESIAN_POINT('Ctrl Pts',(-17.2282025904314,14.7326088681163,
12.));
#240754=CARTESIAN_POINT('Ctrl Pts',(-17.2224992099667,14.7266561494282,
12.));
#240755=CARTESIAN_POINT('Ctrl Pts',(-17.2169471814256,14.7209039390327,
12.));
#240756=CARTESIAN_POINT('Ctrl Pts',(-17.2115510835989,14.7153546289339,
12.));
#240757=CARTESIAN_POINT('Ctrl Pts',(-17.2063157097315,14.7100107213586,
12.));
#240758=CARTESIAN_POINT('Ctrl Pts',(-17.2012461084268,14.7048748502663,
12.));
#240759=CARTESIAN_POINT('Ctrl Pts',(-17.1963476411694,14.699949811582,12.));
#240760=CARTESIAN_POINT('Ctrl Pts',(-17.1916259308415,14.6952385361705,
12.));
#240761=CARTESIAN_POINT('Ctrl Pts',(-17.1870867909918,14.6907440526958,
12.));
#240762=CARTESIAN_POINT('Ctrl Pts',(-17.182736158472,14.686469452232,12.));
#240763=CARTESIAN_POINT('Ctrl Pts',(-17.1785800350826,14.6824178576167,
12.));
#240764=CARTESIAN_POINT('Ctrl Pts',(-17.1746247499057,14.6785925615677,
12.));
#240765=CARTESIAN_POINT('Ctrl Pts',(-17.1708771619129,14.6749971333867,
12.));
#240766=CARTESIAN_POINT('Ctrl Pts',(-17.167344972302,14.671635583332,12.));
#240767=CARTESIAN_POINT('Ctrl Pts',(-17.1640366762305,14.6685123374423,
12.));
#240768=CARTESIAN_POINT('Ctrl Pts',(-17.1609609517369,14.6656319165057,
12.));
#240769=CARTESIAN_POINT('Ctrl Pts',(-17.1581262646789,14.6629987285992,
12.));
#240770=CARTESIAN_POINT('Ctrl Pts',(-17.1555401986401,14.6606167169642,
12.));
#240771=CARTESIAN_POINT('Ctrl Pts',(-17.1532107762718,14.6584900555302,
12.));
#240772=CARTESIAN_POINT('Ctrl Pts',(-17.1511476869496,14.6566237952435,
12.));
#240773=CARTESIAN_POINT('Ctrl Pts',(-17.1493641837558,14.655024862281,12.));
#240774=CARTESIAN_POINT('Ctrl Pts',(-17.147876394491,14.6537016966184,12.));
#240775=CARTESIAN_POINT('Ctrl Pts',(-17.1466998098673,14.6526624064978,
12.));
#240776=CARTESIAN_POINT('Ctrl Pts',(-17.1458462295271,14.6519131634508,
12.));
#240777=CARTESIAN_POINT('Ctrl Pts',(-17.1454262858043,14.6515481598068,
12.));
#240778=CARTESIAN_POINT('Ctrl Pts',(-17.1452600887037,14.6514066997196,
12.));
#240779=CARTESIAN_POINT('Ctrl Pts',(-17.1452153999142,14.6513711852843,
12.));
#240780=CARTESIAN_POINT('Ctrl Pts',(-17.1452095830633,14.6513681262571,
12.));
#240781=CARTESIAN_POINT('',(-18.8464468996588,17.9112098770111,0.));
#240782=CARTESIAN_POINT('Origin',(-12.1729687575668,17.7219872369693,0.));
#240783=CARTESIAN_POINT('',(-12.7689476255363,18.5896416359912,12.));
#240784=CARTESIAN_POINT('',(-6.08648437878338,8.86099361848466,12.));
#240785=CARTESIAN_POINT('',(-12.7689476255363,18.5896416359912,0.));
#240786=CARTESIAN_POINT('',(-12.7689476255363,18.5896416359912,0.));
#240787=CARTESIAN_POINT('',(-6.08648437878338,8.86099361848466,0.));
#240788=CARTESIAN_POINT('Ctrl Pts',(-17.9112098770111,18.8464468996588,
0.));
#240789=CARTESIAN_POINT('Ctrl Pts',(-17.9112098770111,18.8464468996588,
12.));
#240790=CARTESIAN_POINT('Ctrl Pts',(-17.9057348246595,18.8448126709691,
0.));
#240791=CARTESIAN_POINT('Ctrl Pts',(-17.9057348246595,18.8448126709691,
12.));
#240792=CARTESIAN_POINT('Ctrl Pts',(-17.8947931177807,18.8415402351786,
0.));
#240793=CARTESIAN_POINT('Ctrl Pts',(-17.8947931177807,18.8415402351786,
12.));
#240794=CARTESIAN_POINT('Ctrl Pts',(-17.8784057509356,18.8366196462581,
0.));
#240795=CARTESIAN_POINT('Ctrl Pts',(-17.8784057509356,18.8366196462581,
12.));
#240796=CARTESIAN_POINT('Ctrl Pts',(-17.8566063174771,18.8300349895974,
0.));
#240797=CARTESIAN_POINT('Ctrl Pts',(-17.8566063174771,18.8300349895974,
12.));
#240798=CARTESIAN_POINT('Ctrl Pts',(-17.8294410311006,18.8217643886157,
0.));
#240799=CARTESIAN_POINT('Ctrl Pts',(-17.8294410311006,18.8217643886157,
12.));
#240800=CARTESIAN_POINT('Ctrl Pts',(-17.8023598011057,18.8134540340417,
0.));
#240801=CARTESIAN_POINT('Ctrl Pts',(-17.8023598011057,18.8134540340417,
12.));
#240802=CARTESIAN_POINT('Ctrl Pts',(-17.7753627137853,18.8051039860448,
0.));
#240803=CARTESIAN_POINT('Ctrl Pts',(-17.7753627137853,18.8051039860448,
12.));
#240804=CARTESIAN_POINT('Ctrl Pts',(-17.7484498996905,18.7967143519419,
0.));
#240805=CARTESIAN_POINT('Ctrl Pts',(-17.7484498996905,18.7967143519419,
12.));
#240806=CARTESIAN_POINT('Ctrl Pts',(-17.7216215409035,18.7882852976049,
0.));
#240807=CARTESIAN_POINT('Ctrl Pts',(-17.7216215409035,18.7882852976049,
12.));
#240808=CARTESIAN_POINT('Ctrl Pts',(-17.6948778823014,18.7798170641374,
0.));
#240809=CARTESIAN_POINT('Ctrl Pts',(-17.6948778823014,18.7798170641374,
12.));
#240810=CARTESIAN_POINT('Ctrl Pts',(-17.6682192274236,18.7713099642754,
0.));
#240811=CARTESIAN_POINT('Ctrl Pts',(-17.6682192274236,18.7713099642754,
12.));
#240812=CARTESIAN_POINT('Ctrl Pts',(-17.6416459210681,18.762764361321,0.));
#240813=CARTESIAN_POINT('Ctrl Pts',(-17.6416459210681,18.762764361321,12.));
#240814=CARTESIAN_POINT('Ctrl Pts',(-17.6151583357012,18.7541806530984,
0.));
#240815=CARTESIAN_POINT('Ctrl Pts',(-17.6151583357012,18.7541806530984,
12.));
#240816=CARTESIAN_POINT('Ctrl Pts',(-17.5887568561371,18.7455592536687,
0.));
#240817=CARTESIAN_POINT('Ctrl Pts',(-17.5887568561371,18.7455592536687,
12.));
#240818=CARTESIAN_POINT('Ctrl Pts',(-17.5624418653245,18.7369005764553,
0.));
#240819=CARTESIAN_POINT('Ctrl Pts',(-17.5624418653245,18.7369005764553,
12.));
#240820=CARTESIAN_POINT('Ctrl Pts',(-17.5362137287593,18.7282050157138,
0.));
#240821=CARTESIAN_POINT('Ctrl Pts',(-17.5362137287593,18.7282050157138,
12.));
#240822=CARTESIAN_POINT('Ctrl Pts',(-17.5100727820876,18.7194729318098,
0.));
#240823=CARTESIAN_POINT('Ctrl Pts',(-17.5100727820876,18.7194729318098,
12.));
#240824=CARTESIAN_POINT('Ctrl Pts',(-17.4840193397162,18.7107046613912,
0.));
#240825=CARTESIAN_POINT('Ctrl Pts',(-17.4840193397162,18.7107046613912,
12.));
#240826=CARTESIAN_POINT('Ctrl Pts',(-17.4580537012753,18.70190052503,0.));
#240827=CARTESIAN_POINT('Ctrl Pts',(-17.4580537012753,18.70190052503,12.));
#240828=CARTESIAN_POINT('Ctrl Pts',(-17.4321761588142,18.6930608357409,
0.));
#240829=CARTESIAN_POINT('Ctrl Pts',(-17.4321761588142,18.6930608357409,
12.));
#240830=CARTESIAN_POINT('Ctrl Pts',(-17.4063870038562,18.6841859073471,
0.));
#240831=CARTESIAN_POINT('Ctrl Pts',(-17.4063870038562,18.6841859073471,
12.));
#240832=CARTESIAN_POINT('Ctrl Pts',(-17.3806865340747,18.6752760624052,
0.));
#240833=CARTESIAN_POINT('Ctrl Pts',(-17.3806865340747,18.6752760624052,
12.));
#240834=CARTESIAN_POINT('Ctrl Pts',(-17.3550750612443,18.6663316416582,
0.));
#240835=CARTESIAN_POINT('Ctrl Pts',(-17.3550750612443,18.6663316416582,
12.));
#240836=CARTESIAN_POINT('Ctrl Pts',(-17.3295529098618,18.6573530024033,
0.));
#240837=CARTESIAN_POINT('Ctrl Pts',(-17.3295529098618,18.6573530024033,
12.));
#240838=CARTESIAN_POINT('Ctrl Pts',(-17.3041204135074,18.6483405141865,
0.));
#240839=CARTESIAN_POINT('Ctrl Pts',(-17.3041204135074,18.6483405141865,
12.));
#240840=CARTESIAN_POINT('Ctrl Pts',(-17.2787779120213,18.6392945554748,
0.));
#240841=CARTESIAN_POINT('Ctrl Pts',(-17.2787779120213,18.6392945554748,
12.));
#240842=CARTESIAN_POINT('Ctrl Pts',(-17.2535257482187,18.6302155097943,
0.));
#240843=CARTESIAN_POINT('Ctrl Pts',(-17.2535257482187,18.6302155097943,
12.));
#240844=CARTESIAN_POINT('Ctrl Pts',(-17.2283642650518,18.6211037624038,
0.));
#240845=CARTESIAN_POINT('Ctrl Pts',(-17.2283642650518,18.6211037624038,
12.));
#240846=CARTESIAN_POINT('Ctrl Pts',(-17.2032938019284,18.6119596959949,
0.));
#240847=CARTESIAN_POINT('Ctrl Pts',(-17.2032938019284,18.6119596959949,
12.));
#240848=CARTESIAN_POINT('Ctrl Pts',(-17.1783146940127,18.6027836898817,
0.));
#240849=CARTESIAN_POINT('Ctrl Pts',(-17.1783146940127,18.6027836898817,
12.));
#240850=CARTESIAN_POINT('Ctrl Pts',(-17.1534272741643,18.5935761222825,
0.));
#240851=CARTESIAN_POINT('Ctrl Pts',(-17.1534272741643,18.5935761222825,
12.));
#240852=CARTESIAN_POINT('Ctrl Pts',(-17.1286318741183,18.5843373717247,
0.));
#240853=CARTESIAN_POINT('Ctrl Pts',(-17.1286318741183,18.5843373717247,
12.));
#240854=CARTESIAN_POINT('Ctrl Pts',(-17.1039288260001,18.5750678188542,
0.));
#240855=CARTESIAN_POINT('Ctrl Pts',(-17.1039288260001,18.5750678188542,
12.));
#240856=CARTESIAN_POINT('Ctrl Pts',(-17.0793184636079,18.5657678479789,
0.));
#240857=CARTESIAN_POINT('Ctrl Pts',(-17.0793184636079,18.5657678479789,
12.));
#240858=CARTESIAN_POINT('Ctrl Pts',(-17.0548011239751,18.556437848963,0.));
#240859=CARTESIAN_POINT('Ctrl Pts',(-17.0548011239751,18.556437848963,12.));
#240860=CARTESIAN_POINT('Ctrl Pts',(-17.0303771481738,18.547078218209,0.));
#240861=CARTESIAN_POINT('Ctrl Pts',(-17.0303771481738,18.547078218209,12.));
#240862=CARTESIAN_POINT('Ctrl Pts',(-17.0060468805097,18.5376893576961,
0.));
#240863=CARTESIAN_POINT('Ctrl Pts',(-17.0060468805097,18.5376893576961,
12.));
#240864=CARTESIAN_POINT('Ctrl Pts',(-16.981810668038,18.5282716744197,0.));
#240865=CARTESIAN_POINT('Ctrl Pts',(-16.981810668038,18.5282716744197,12.));
#240866=CARTESIAN_POINT('Ctrl Pts',(-16.9576688599339,18.5188255796659,
0.));
#240867=CARTESIAN_POINT('Ctrl Pts',(-16.9576688599339,18.5188255796659,
12.));
#240868=CARTESIAN_POINT('Ctrl Pts',(-16.9336218069353,18.5093514883835,
0.));
#240869=CARTESIAN_POINT('Ctrl Pts',(-16.9336218069353,18.5093514883835,
12.));
#240870=CARTESIAN_POINT('Ctrl Pts',(-16.9096698606943,18.499849818462,0.));
#240871=CARTESIAN_POINT('Ctrl Pts',(-16.9096698606943,18.499849818462,12.));
#240872=CARTESIAN_POINT('Ctrl Pts',(-16.8858133733088,18.4903209902227,
0.));
#240873=CARTESIAN_POINT('Ctrl Pts',(-16.8858133733088,18.4903209902227,
12.));
#240874=CARTESIAN_POINT('Ctrl Pts',(-16.8620526977171,18.480765426877,0.));
#240875=CARTESIAN_POINT('Ctrl Pts',(-16.8620526977171,18.480765426877,12.));
#240876=CARTESIAN_POINT('Ctrl Pts',(-16.8383881879709,18.4711835548623,
0.));
#240877=CARTESIAN_POINT('Ctrl Pts',(-16.8383881879709,18.4711835548623,
12.));
#240878=CARTESIAN_POINT('Ctrl Pts',(-16.8148201995472,18.4615758042305,
0.));
#240879=CARTESIAN_POINT('Ctrl Pts',(-16.8148201995472,18.4615758042305,
12.));
#240880=CARTESIAN_POINT('Ctrl Pts',(-16.791349089629,18.4519426090123,0.));
#240881=CARTESIAN_POINT('Ctrl Pts',(-16.791349089629,18.4519426090123,12.));
#240882=CARTESIAN_POINT('Ctrl Pts',(-16.7679752173992,18.44228440761,0.));
#240883=CARTESIAN_POINT('Ctrl Pts',(-16.7679752173992,18.44228440761,12.));
#240884=CARTESIAN_POINT('Ctrl Pts',(-16.7446989442882,18.4326016431392,
0.));
#240885=CARTESIAN_POINT('Ctrl Pts',(-16.7446989442882,18.4326016431392,
12.));
#240886=CARTESIAN_POINT('Ctrl Pts',(-16.7215206338818,18.4228947633187,
0.));
#240887=CARTESIAN_POINT('Ctrl Pts',(-16.7215206338818,18.4228947633187,
12.));
#240888=CARTESIAN_POINT('Ctrl Pts',(-16.6984406518491,18.413164220399,0.));
#240889=CARTESIAN_POINT('Ctrl Pts',(-16.6984406518491,18.413164220399,12.));
#240890=CARTESIAN_POINT('Ctrl Pts',(-16.6754593658513,18.403410471079,0.));
#240891=CARTESIAN_POINT('Ctrl Pts',(-16.6754593658513,18.403410471079,12.));
#240892=CARTESIAN_POINT('Ctrl Pts',(-16.6525771454513,18.3936339764332,
0.));
#240893=CARTESIAN_POINT('Ctrl Pts',(-16.6525771454513,18.3936339764332,
12.));
#240894=CARTESIAN_POINT('Ctrl Pts',(-16.6297943620056,18.3838352018327,
0.));
#240895=CARTESIAN_POINT('Ctrl Pts',(-16.6297943620056,18.3838352018327,
12.));
#240896=CARTESIAN_POINT('Ctrl Pts',(-16.607111388571,18.3740146168879,0.));
#240897=CARTESIAN_POINT('Ctrl Pts',(-16.607111388571,18.3740146168879,12.));
#240898=CARTESIAN_POINT('Ctrl Pts',(-16.5845286000217,18.3641726955889,
0.));
#240899=CARTESIAN_POINT('Ctrl Pts',(-16.5845286000217,18.3641726955889,
12.));
#240900=CARTESIAN_POINT('Ctrl Pts',(-16.5620463731413,18.354309916433,0.));
#240901=CARTESIAN_POINT('Ctrl Pts',(-16.5620463731413,18.354309916433,12.));
#240902=CARTESIAN_POINT('Ctrl Pts',(-16.5396650867139,18.34442676256,0.));
#240903=CARTESIAN_POINT('Ctrl Pts',(-16.5396650867139,18.34442676256,12.));
#240904=CARTESIAN_POINT('Ctrl Pts',(-16.5173851216045,18.3345237218864,
0.));
#240905=CARTESIAN_POINT('Ctrl Pts',(-16.5173851216045,18.3345237218864,
12.));
#240906=CARTESIAN_POINT('Ctrl Pts',(-16.4952068608345,18.3246012872469,
0.));
#240907=CARTESIAN_POINT('Ctrl Pts',(-16.4952068608345,18.3246012872469,
12.));
#240908=CARTESIAN_POINT('Ctrl Pts',(-16.4731306896441,18.3146599565231,
0.));
#240909=CARTESIAN_POINT('Ctrl Pts',(-16.4731306896441,18.3146599565231,
12.));
#240910=CARTESIAN_POINT('Ctrl Pts',(-16.4511569955233,18.304700232686,0.));
#240911=CARTESIAN_POINT('Ctrl Pts',(-16.4511569955233,18.304700232686,12.));
#240912=CARTESIAN_POINT('Ctrl Pts',(-16.4292861682379,18.294722623851,0.));
#240913=CARTESIAN_POINT('Ctrl Pts',(-16.4292861682379,18.294722623851,12.));
#240914=CARTESIAN_POINT('Ctrl Pts',(-16.4075185998455,18.2847276433309,
0.));
#240915=CARTESIAN_POINT('Ctrl Pts',(-16.4075185998455,18.2847276433309,
12.));
#240916=CARTESIAN_POINT('Ctrl Pts',(-16.385854684708,18.2747158096934,0.));
#240917=CARTESIAN_POINT('Ctrl Pts',(-16.385854684708,18.2747158096934,12.));
#240918=CARTESIAN_POINT('Ctrl Pts',(-16.3642948194868,18.2646876468169,
0.));
#240919=CARTESIAN_POINT('Ctrl Pts',(-16.3642948194868,18.2646876468169,
12.));
#240920=CARTESIAN_POINT('Ctrl Pts',(-16.3428394031589,18.2546436839608,
0.));
#240921=CARTESIAN_POINT('Ctrl Pts',(-16.3428394031589,18.2546436839608,
12.));
#240922=CARTESIAN_POINT('Ctrl Pts',(-16.3214888370987,18.2445844558741,
0.));
#240923=CARTESIAN_POINT('Ctrl Pts',(-16.3214888370987,18.2445844558741,
12.));
#240924=CARTESIAN_POINT('Ctrl Pts',(-16.3002435251378,18.2345105028982,
0.));
#240925=CARTESIAN_POINT('Ctrl Pts',(-16.3002435251378,18.2345105028982,
12.));
#240926=CARTESIAN_POINT('Ctrl Pts',(-16.2791038736223,18.2244223710745,
0.));
#240927=CARTESIAN_POINT('Ctrl Pts',(-16.2791038736223,18.2244223710745,
12.));
#240928=CARTESIAN_POINT('Ctrl Pts',(-16.2580702914615,18.2143206122529,
0.));
#240929=CARTESIAN_POINT('Ctrl Pts',(-16.2580702914615,18.2143206122529,
12.));
#240930=CARTESIAN_POINT('Ctrl Pts',(-16.2371431901638,18.2042057842035,
0.));
#240931=CARTESIAN_POINT('Ctrl Pts',(-16.2371431901638,18.2042057842035,
12.));
#240932=CARTESIAN_POINT('Ctrl Pts',(-16.2163229838875,18.1940784507229,
0.));
#240933=CARTESIAN_POINT('Ctrl Pts',(-16.2163229838875,18.1940784507229,
12.));
#240934=CARTESIAN_POINT('Ctrl Pts',(-16.1956100895073,18.1839391817331,
0.));
#240935=CARTESIAN_POINT('Ctrl Pts',(-16.1956100895073,18.1839391817331,
12.));
#240936=CARTESIAN_POINT('Ctrl Pts',(-16.1750049266671,18.1737885533849,
0.));
#240937=CARTESIAN_POINT('Ctrl Pts',(-16.1750049266671,18.1737885533849,
12.));
#240938=CARTESIAN_POINT('Ctrl Pts',(-16.154507917826,18.1636271481615,0.));
#240939=CARTESIAN_POINT('Ctrl Pts',(-16.154507917826,18.1636271481615,12.));
#240940=CARTESIAN_POINT('Ctrl Pts',(-16.1341194882988,18.1534555549852,
0.));
#240941=CARTESIAN_POINT('Ctrl Pts',(-16.1341194882988,18.1534555549852,
12.));
#240942=CARTESIAN_POINT('Ctrl Pts',(-16.1138400662794,18.1432743693235,
0.));
#240943=CARTESIAN_POINT('Ctrl Pts',(-16.1138400662794,18.1432743693235,
12.));
#240944=CARTESIAN_POINT('Ctrl Pts',(-16.0936700829112,18.1330841933105,
0.));
#240945=CARTESIAN_POINT('Ctrl Pts',(-16.0936700829112,18.1330841933105,
12.));
#240946=CARTESIAN_POINT('Ctrl Pts',(-16.0736099723668,18.1228856358751,
0.));
#240947=CARTESIAN_POINT('Ctrl Pts',(-16.0736099723668,18.1228856358751,
12.));
#240948=CARTESIAN_POINT('Ctrl Pts',(-16.0536601719126,18.112679312869,0.));
#240949=CARTESIAN_POINT('Ctrl Pts',(-16.0536601719126,18.112679312869,12.));
#240950=CARTESIAN_POINT('Ctrl Pts',(-16.0338211219693,18.1024658471966,
0.));
#240951=CARTESIAN_POINT('Ctrl Pts',(-16.0338211219693,18.1024658471966,
12.));
#240952=CARTESIAN_POINT('Ctrl Pts',(-16.014093266161,18.0922458689462,0.));
#240953=CARTESIAN_POINT('Ctrl Pts',(-16.014093266161,18.0922458689462,12.));
#240954=CARTESIAN_POINT('Ctrl Pts',(-15.9944770513613,18.0820200155236,
0.));
#240955=CARTESIAN_POINT('Ctrl Pts',(-15.9944770513613,18.0820200155236,
12.));
#240956=CARTESIAN_POINT('Ctrl Pts',(-15.9749729277846,18.0717889317958,
0.));
#240957=CARTESIAN_POINT('Ctrl Pts',(-15.9749729277846,18.0717889317958,
12.));
#240958=CARTESIAN_POINT('Ctrl Pts',(-15.9555813490644,18.0615532702359,
0.));
#240959=CARTESIAN_POINT('Ctrl Pts',(-15.9555813490644,18.0615532702359,
12.));
#240960=CARTESIAN_POINT('Ctrl Pts',(-15.9363027723244,18.0513136910691,
0.));
#240961=CARTESIAN_POINT('Ctrl Pts',(-15.9363027723244,18.0513136910691,
12.));
#240962=CARTESIAN_POINT('Ctrl Pts',(-15.9171376582436,18.0410708624208,
0.));
#240963=CARTESIAN_POINT('Ctrl Pts',(-15.9171376582436,18.0410708624208,
12.));
#240964=CARTESIAN_POINT('Ctrl Pts',(-15.8980864711042,18.0308254604636,
0.));
#240965=CARTESIAN_POINT('Ctrl Pts',(-15.8980864711042,18.0308254604636,
12.));
#240966=CARTESIAN_POINT('Ctrl Pts',(-15.8791496788683,18.0205781695769,
0.));
#240967=CARTESIAN_POINT('Ctrl Pts',(-15.8791496788683,18.0205781695769,
12.));
#240968=CARTESIAN_POINT('Ctrl Pts',(-15.8603277532831,18.0103296825205,
0.));
#240969=CARTESIAN_POINT('Ctrl Pts',(-15.8603277532831,18.0103296825205,
12.));
#240970=CARTESIAN_POINT('Ctrl Pts',(-15.8416211699679,18.0000807006052,
0.));
#240971=CARTESIAN_POINT('Ctrl Pts',(-15.8416211699679,18.0000807006052,
12.));
#240972=CARTESIAN_POINT('Ctrl Pts',(-15.8230304084962,17.9898319338664,
0.));
#240973=CARTESIAN_POINT('Ctrl Pts',(-15.8230304084962,17.9898319338664,
12.));
#240974=CARTESIAN_POINT('Ctrl Pts',(-15.8045559524676,17.9795841012386,
0.));
#240975=CARTESIAN_POINT('Ctrl Pts',(-15.8045559524676,17.9795841012386,
12.));
#240976=CARTESIAN_POINT('Ctrl Pts',(-15.7861982895724,17.9693379307303,
0.));
#240977=CARTESIAN_POINT('Ctrl Pts',(-15.7861982895724,17.9693379307303,
12.));
#240978=CARTESIAN_POINT('Ctrl Pts',(-15.7679579117077,17.9590941596242,
0.));
#240979=CARTESIAN_POINT('Ctrl Pts',(-15.7679579117077,17.9590941596242,
12.));
#240980=CARTESIAN_POINT('Ctrl Pts',(-15.749835315086,17.9488535346781,0.));
#240981=CARTESIAN_POINT('Ctrl Pts',(-15.749835315086,17.9488535346781,12.));
#240982=CARTESIAN_POINT('Ctrl Pts',(-15.7318310003335,17.9386168123262,
0.));
#240983=CARTESIAN_POINT('Ctrl Pts',(-15.7318310003335,17.9386168123262,
12.));
#240984=CARTESIAN_POINT('Ctrl Pts',(-15.7139454725838,17.9283847588835,
0.));
#240985=CARTESIAN_POINT('Ctrl Pts',(-15.7139454725838,17.9283847588835,
12.));
#240986=CARTESIAN_POINT('Ctrl Pts',(-15.6961792415522,17.9181581507455,
0.));
#240987=CARTESIAN_POINT('Ctrl Pts',(-15.6961792415522,17.9181581507455,
12.));
#240988=CARTESIAN_POINT('Ctrl Pts',(-15.678532821646,17.9079377746111,0.));
#240989=CARTESIAN_POINT('Ctrl Pts',(-15.678532821646,17.9079377746111,12.));
#240990=CARTESIAN_POINT('Ctrl Pts',(-15.661006732103,17.897724427724,0.));
#240991=CARTESIAN_POINT('Ctrl Pts',(-15.661006732103,17.897724427724,12.));
#240992=CARTESIAN_POINT('Ctrl Pts',(-15.6436014971084,17.8875189181091,
0.));
#240993=CARTESIAN_POINT('Ctrl Pts',(-15.6436014971084,17.8875189181091,
12.));
#240994=CARTESIAN_POINT('Ctrl Pts',(-15.6263176459108,17.8773220648125,
0.));
#240995=CARTESIAN_POINT('Ctrl Pts',(-15.6263176459108,17.8773220648125,
12.));
#240996=CARTESIAN_POINT('Ctrl Pts',(-15.609155712921,17.8671346981394,0.));
#240997=CARTESIAN_POINT('Ctrl Pts',(-15.609155712921,17.8671346981394,12.));
#240998=CARTESIAN_POINT('Ctrl Pts',(-15.5921162378192,17.8569576599006,
0.));
#240999=CARTESIAN_POINT('Ctrl Pts',(-15.5921162378192,17.8569576599006,
12.));
#241000=CARTESIAN_POINT('Ctrl Pts',(-15.5751997657163,17.8467918036987,
0.));
#241001=CARTESIAN_POINT('Ctrl Pts',(-15.5751997657163,17.8467918036987,
12.));
#241002=CARTESIAN_POINT('Ctrl Pts',(-15.5584068472982,17.8366379952085,
0.));
#241003=CARTESIAN_POINT('Ctrl Pts',(-15.5584068472982,17.8366379952085,
12.));
#241004=CARTESIAN_POINT('Ctrl Pts',(-15.541738038964,17.8264971124606,0.));
#241005=CARTESIAN_POINT('Ctrl Pts',(-15.541738038964,17.8264971124606,12.));
#241006=CARTESIAN_POINT('Ctrl Pts',(-15.5251939029552,17.8163700461256,
0.));
#241007=CARTESIAN_POINT('Ctrl Pts',(-15.5251939029552,17.8163700461256,
12.));
#241008=CARTESIAN_POINT('Ctrl Pts',(-15.5087750074718,17.8062576997952,
0.));
#241009=CARTESIAN_POINT('Ctrl Pts',(-15.5087750074718,17.8062576997952,
12.));
#241010=CARTESIAN_POINT('Ctrl Pts',(-15.4924819268517,17.7961609903148,
0.));
#241011=CARTESIAN_POINT('Ctrl Pts',(-15.4924819268517,17.7961609903148,
12.));
#241012=CARTESIAN_POINT('Ctrl Pts',(-15.4763152417497,17.7860808481219,
0.));
#241013=CARTESIAN_POINT('Ctrl Pts',(-15.4763152417497,17.7860808481219,
12.));
#241014=CARTESIAN_POINT('Ctrl Pts',(-15.4602755393017,17.7760182175815,
0.));
#241015=CARTESIAN_POINT('Ctrl Pts',(-15.4602755393017,17.7760182175815,
12.));
#241016=CARTESIAN_POINT('Ctrl Pts',(-15.4443634132869,17.7659740573265,
0.));
#241017=CARTESIAN_POINT('Ctrl Pts',(-15.4443634132869,17.7659740573265,
12.));
#241018=CARTESIAN_POINT('Ctrl Pts',(-15.4285794642668,17.7559493405881,
0.));
#241019=CARTESIAN_POINT('Ctrl Pts',(-15.4285794642668,17.7559493405881,
12.));
#241020=CARTESIAN_POINT('Ctrl Pts',(-15.4129242997837,17.7459450555812,
0.));
#241021=CARTESIAN_POINT('Ctrl Pts',(-15.4129242997837,17.7459450555812,
12.));
#241022=CARTESIAN_POINT('Ctrl Pts',(-15.3973985345802,17.7359622059149,
0.));
#241023=CARTESIAN_POINT('Ctrl Pts',(-15.3973985345802,17.7359622059149,
12.));
#241024=CARTESIAN_POINT('Ctrl Pts',(-15.3820027907967,17.7260018109924,
0.));
#241025=CARTESIAN_POINT('Ctrl Pts',(-15.3820027907967,17.7260018109924,
12.));
#241026=CARTESIAN_POINT('Ctrl Pts',(-15.3667376981699,17.7160649064206,
0.));
#241027=CARTESIAN_POINT('Ctrl Pts',(-15.3667376981699,17.7160649064206,
12.));
#241028=CARTESIAN_POINT('Ctrl Pts',(-15.351603894206,17.7061525444042,0.));
#241029=CARTESIAN_POINT('Ctrl Pts',(-15.351603894206,17.7061525444042,12.));
#241030=CARTESIAN_POINT('Ctrl Pts',(-15.3366020244066,17.6962657941983,
0.));
#241031=CARTESIAN_POINT('Ctrl Pts',(-15.3366020244066,17.6962657941983,
12.));
#241032=CARTESIAN_POINT('Ctrl Pts',(-15.3217327425338,17.6864057426052,
0.));
#241033=CARTESIAN_POINT('Ctrl Pts',(-15.3217327425338,17.6864057426052,
12.));
#241034=CARTESIAN_POINT('Ctrl Pts',(-15.3069967108501,17.676573494456,0.));
#241035=CARTESIAN_POINT('Ctrl Pts',(-15.3069967108501,17.676573494456,12.));
#241036=CARTESIAN_POINT('Ctrl Pts',(-15.2923946003598,17.6667701731041,
0.));
#241037=CARTESIAN_POINT('Ctrl Pts',(-15.2923946003598,17.6667701731041,
12.));
#241038=CARTESIAN_POINT('Ctrl Pts',(-15.2779270910239,17.6569969209,0.));
#241039=CARTESIAN_POINT('Ctrl Pts',(-15.2779270910239,17.6569969209,12.));
#241040=CARTESIAN_POINT('Ctrl Pts',(-15.2635948720292,17.6472548997328,
0.));
#241041=CARTESIAN_POINT('Ctrl Pts',(-15.2635948720292,17.6472548997328,
12.));
#241042=CARTESIAN_POINT('Ctrl Pts',(-15.2493986421092,17.6375452916369,
0.));
#241043=CARTESIAN_POINT('Ctrl Pts',(-15.2493986421092,17.6375452916369,
12.));
#241044=CARTESIAN_POINT('Ctrl Pts',(-15.2353391098366,17.6278692993764,
0.));
#241045=CARTESIAN_POINT('Ctrl Pts',(-15.2353391098366,17.6278692993764,
12.));
#241046=CARTESIAN_POINT('Ctrl Pts',(-15.2214169939199,17.6182281470468,
0.));
#241047=CARTESIAN_POINT('Ctrl Pts',(-15.2214169939199,17.6182281470468,
12.));
#241048=CARTESIAN_POINT('Ctrl Pts',(-15.2076330234686,17.60862308065,0.));
#241049=CARTESIAN_POINT('Ctrl Pts',(-15.2076330234686,17.60862308065,12.));
#241050=CARTESIAN_POINT('Ctrl Pts',(-15.1939879383268,17.5990553687599,
0.));
#241051=CARTESIAN_POINT('Ctrl Pts',(-15.1939879383268,17.5990553687599,
12.));
#241052=CARTESIAN_POINT('Ctrl Pts',(-15.1804824894605,17.5895263032595,
0.));
#241053=CARTESIAN_POINT('Ctrl Pts',(-15.1804824894605,17.5895263032595,
12.));
#241054=CARTESIAN_POINT('Ctrl Pts',(-15.1671174393137,17.580037200054,0.));
#241055=CARTESIAN_POINT('Ctrl Pts',(-15.1671174393137,17.580037200054,12.));
#241056=CARTESIAN_POINT('Ctrl Pts',(-15.1538935621714,17.5705893998029,
0.));
#241057=CARTESIAN_POINT('Ctrl Pts',(-15.1538935621714,17.5705893998029,
12.));
#241058=CARTESIAN_POINT('Ctrl Pts',(-15.1408116444876,17.5611842686192,
0.));
#241059=CARTESIAN_POINT('Ctrl Pts',(-15.1408116444876,17.5611842686192,
12.));
#241060=CARTESIAN_POINT('Ctrl Pts',(-15.1278724853138,17.5518231989117,
0.));
#241061=CARTESIAN_POINT('Ctrl Pts',(-15.1278724853138,17.5518231989117,
12.));
#241062=CARTESIAN_POINT('Ctrl Pts',(-15.1150768967728,17.5425076102963,
0.));
#241063=CARTESIAN_POINT('Ctrl Pts',(-15.1150768967728,17.5425076102963,
12.));
#241064=CARTESIAN_POINT('Ctrl Pts',(-15.1024257045033,17.5332389504829,
0.));
#241065=CARTESIAN_POINT('Ctrl Pts',(-15.1024257045033,17.5332389504829,
12.));
#241066=CARTESIAN_POINT('Ctrl Pts',(-15.0899197481082,17.524018696179,0.));
#241067=CARTESIAN_POINT('Ctrl Pts',(-15.0899197481082,17.524018696179,12.));
#241068=CARTESIAN_POINT('Ctrl Pts',(-15.0775598815749,17.5148483539687,
0.));
#241069=CARTESIAN_POINT('Ctrl Pts',(-15.0775598815749,17.5148483539687,
12.));
#241070=CARTESIAN_POINT('Ctrl Pts',(-15.0653469738307,17.5057294613877,
0.));
#241071=CARTESIAN_POINT('Ctrl Pts',(-15.0653469738307,17.5057294613877,
12.));
#241072=CARTESIAN_POINT('Ctrl Pts',(-15.0532819093085,17.4966635880246,
0.));
#241073=CARTESIAN_POINT('Ctrl Pts',(-15.0532819093085,17.4966635880246,
12.));
#241074=CARTESIAN_POINT('Ctrl Pts',(-15.0413655884993,17.4876523366178,
0.));
#241075=CARTESIAN_POINT('Ctrl Pts',(-15.0413655884993,17.4876523366178,
12.));
#241076=CARTESIAN_POINT('Ctrl Pts',(-15.029598928488,17.4786973441417,0.));
#241077=CARTESIAN_POINT('Ctrl Pts',(-15.029598928488,17.4786973441417,12.));
#241078=CARTESIAN_POINT('Ctrl Pts',(-15.0179828635087,17.4698002829357,
0.));
#241079=CARTESIAN_POINT('Ctrl Pts',(-15.0179828635087,17.4698002829357,
12.));
#241080=CARTESIAN_POINT('Ctrl Pts',(-15.0065183456922,17.4609628621419,
0.));
#241081=CARTESIAN_POINT('Ctrl Pts',(-15.0065183456922,17.4609628621419,
12.));
#241082=CARTESIAN_POINT('Ctrl Pts',(-14.9952063457779,17.4521868291005,
0.));
#241083=CARTESIAN_POINT('Ctrl Pts',(-14.9952063457779,17.4521868291005,
12.));
#241084=CARTESIAN_POINT('Ctrl Pts',(-14.9840478538357,17.4434739707773,
0.));
#241085=CARTESIAN_POINT('Ctrl Pts',(-14.9840478538357,17.4434739707773,
12.));
#241086=CARTESIAN_POINT('Ctrl Pts',(-14.973043879945,17.4348261151395,0.));
#241087=CARTESIAN_POINT('Ctrl Pts',(-14.973043879945,17.4348261151395,12.));
#241088=CARTESIAN_POINT('Ctrl Pts',(-14.9621954549825,17.4262451327088,
0.));
#241089=CARTESIAN_POINT('Ctrl Pts',(-14.9621954549825,17.4262451327088,
12.));
#241090=CARTESIAN_POINT('Ctrl Pts',(-14.9515036315142,17.4177329382827,
0.));
#241091=CARTESIAN_POINT('Ctrl Pts',(-14.9515036315142,17.4177329382827,
12.));
#241092=CARTESIAN_POINT('Ctrl Pts',(-14.940969484645,17.4092914926071,0.));
#241093=CARTESIAN_POINT('Ctrl Pts',(-14.940969484645,17.4092914926071,12.));
#241094=CARTESIAN_POINT('Ctrl Pts',(-14.9305941128758,17.400922804075,0.));
#241095=CARTESIAN_POINT('Ctrl Pts',(-14.9305941128758,17.400922804075,12.));
#241096=CARTESIAN_POINT('Ctrl Pts',(-14.9203786389343,17.3926289303987,
0.));
#241097=CARTESIAN_POINT('Ctrl Pts',(-14.9203786389343,17.3926289303987,
12.));
#241098=CARTESIAN_POINT('Ctrl Pts',(-14.9103242110057,17.3844119809823,
0.));
#241099=CARTESIAN_POINT('Ctrl Pts',(-14.9103242110057,17.3844119809823,
12.));
#241100=CARTESIAN_POINT('Ctrl Pts',(-14.9004320039609,17.3762741193075,
0.));
#241101=CARTESIAN_POINT('Ctrl Pts',(-14.9004320039609,17.3762741193075,
12.));
#241102=CARTESIAN_POINT('Ctrl Pts',(-14.8907032205789,17.3682175653236,
0.));
#241103=CARTESIAN_POINT('Ctrl Pts',(-14.8907032205789,17.3682175653236,
12.));
#241104=CARTESIAN_POINT('Ctrl Pts',(-14.8811390927424,17.3602445978163,
0.));
#241105=CARTESIAN_POINT('Ctrl Pts',(-14.8811390927424,17.3602445978163,
12.));
#241106=CARTESIAN_POINT('Ctrl Pts',(-14.8717408826958,17.3523575568648,
0.));
#241107=CARTESIAN_POINT('Ctrl Pts',(-14.8717408826958,17.3523575568648,
12.));
#241108=CARTESIAN_POINT('Ctrl Pts',(-14.8625098843419,17.3445588463477,
0.));
#241109=CARTESIAN_POINT('Ctrl Pts',(-14.8625098843419,17.3445588463477,
12.));
#241110=CARTESIAN_POINT('Ctrl Pts',(-14.8534474245433,17.336850936485,0.));
#241111=CARTESIAN_POINT('Ctrl Pts',(-14.8534474245433,17.336850936485,12.));
#241112=CARTESIAN_POINT('Ctrl Pts',(-14.8445548643504,17.3292363662601,
0.));
#241113=CARTESIAN_POINT('Ctrl Pts',(-14.8445548643504,17.3292363662601,
12.));
#241114=CARTESIAN_POINT('Ctrl Pts',(-14.8358336004193,17.3217177462096,
0.));
#241115=CARTESIAN_POINT('Ctrl Pts',(-14.8358336004193,17.3217177462096,
12.));
#241116=CARTESIAN_POINT('Ctrl Pts',(-14.8272850675375,17.3142977632656,
0.));
#241117=CARTESIAN_POINT('Ctrl Pts',(-14.8272850675375,17.3142977632656,
12.));
#241118=CARTESIAN_POINT('Ctrl Pts',(-14.8189107410161,17.3069791853705,
0.));
#241119=CARTESIAN_POINT('Ctrl Pts',(-14.8189107410161,17.3069791853705,
12.));
#241120=CARTESIAN_POINT('Ctrl Pts',(-14.8107121391038,17.2997648661483,
0.));
#241121=CARTESIAN_POINT('Ctrl Pts',(-14.8107121391038,17.2997648661483,
12.));
#241122=CARTESIAN_POINT('Ctrl Pts',(-14.8026908254281,17.2926577496519,
0.));
#241123=CARTESIAN_POINT('Ctrl Pts',(-14.8026908254281,17.2926577496519,
12.));
#241124=CARTESIAN_POINT('Ctrl Pts',(-14.7948484105253,17.28566087332,0.));
#241125=CARTESIAN_POINT('Ctrl Pts',(-14.7948484105253,17.28566087332,12.));
#241126=CARTESIAN_POINT('Ctrl Pts',(-14.787186553128,17.278777370485,0.));
#241127=CARTESIAN_POINT('Ctrl Pts',(-14.787186553128,17.278777370485,12.));
#241128=CARTESIAN_POINT('Ctrl Pts',(-14.7797069617802,17.2720104735192,
0.));
#241129=CARTESIAN_POINT('Ctrl Pts',(-14.7797069617802,17.2720104735192,
12.));
#241130=CARTESIAN_POINT('Ctrl Pts',(-14.7724113956728,17.2653635155317,
0.));
#241131=CARTESIAN_POINT('Ctrl Pts',(-14.7724113956728,17.2653635155317,
12.));
#241132=CARTESIAN_POINT('Ctrl Pts',(-14.7653016697589,17.2588399401464,
0.));
#241133=CARTESIAN_POINT('Ctrl Pts',(-14.7653016697589,17.2588399401464,
12.));
#241134=CARTESIAN_POINT('Ctrl Pts',(-14.7583796616617,17.2524433146837,
0.));
#241135=CARTESIAN_POINT('Ctrl Pts',(-14.7583796616617,17.2524433146837,
12.));
#241136=CARTESIAN_POINT('Ctrl Pts',(-14.7516473175125,17.2461773413289,
0.));
#241137=CARTESIAN_POINT('Ctrl Pts',(-14.7516473175125,17.2461773413289,
12.));
#241138=CARTESIAN_POINT('Ctrl Pts',(-14.7451066593793,17.2400458713566,
0.));
#241139=CARTESIAN_POINT('Ctrl Pts',(-14.7451066593793,17.2400458713566,
12.));
#241140=CARTESIAN_POINT('Ctrl Pts',(-14.7387597858117,17.2340529062077,
0.));
#241141=CARTESIAN_POINT('Ctrl Pts',(-14.7387597858117,17.2340529062077,
12.));
#241142=CARTESIAN_POINT('Ctrl Pts',(-14.7326088681163,17.2282025904314,
0.));
#241143=CARTESIAN_POINT('Ctrl Pts',(-14.7326088681163,17.2282025904314,
12.));
#241144=CARTESIAN_POINT('Ctrl Pts',(-14.7266561494282,17.2224992099666,
0.));
#241145=CARTESIAN_POINT('Ctrl Pts',(-14.7266561494282,17.2224992099666,
12.));
#241146=CARTESIAN_POINT('Ctrl Pts',(-14.7209039390326,17.2169471814255,
0.));
#241147=CARTESIAN_POINT('Ctrl Pts',(-14.7209039390326,17.2169471814255,
12.));
#241148=CARTESIAN_POINT('Ctrl Pts',(-14.7153546289338,17.2115510835988,
0.));
#241149=CARTESIAN_POINT('Ctrl Pts',(-14.7153546289338,17.2115510835988,
12.));
#241150=CARTESIAN_POINT('Ctrl Pts',(-14.7100107213586,17.2063157097316,
0.));
#241151=CARTESIAN_POINT('Ctrl Pts',(-14.7100107213586,17.2063157097316,
12.));
#241152=CARTESIAN_POINT('Ctrl Pts',(-14.7048748502663,17.2012461084268,
0.));
#241153=CARTESIAN_POINT('Ctrl Pts',(-14.7048748502663,17.2012461084268,
12.));
#241154=CARTESIAN_POINT('Ctrl Pts',(-14.699949811582,17.1963476411694,0.));
#241155=CARTESIAN_POINT('Ctrl Pts',(-14.699949811582,17.1963476411694,12.));
#241156=CARTESIAN_POINT('Ctrl Pts',(-14.6952385361706,17.1916259308415,
0.));
#241157=CARTESIAN_POINT('Ctrl Pts',(-14.6952385361706,17.1916259308415,
12.));
#241158=CARTESIAN_POINT('Ctrl Pts',(-14.6907440526958,17.1870867909918,
0.));
#241159=CARTESIAN_POINT('Ctrl Pts',(-14.6907440526958,17.1870867909918,
12.));
#241160=CARTESIAN_POINT('Ctrl Pts',(-14.6864694522319,17.182736158472,0.));
#241161=CARTESIAN_POINT('Ctrl Pts',(-14.6864694522319,17.182736158472,12.));
#241162=CARTESIAN_POINT('Ctrl Pts',(-14.6824178576167,17.1785800350827,
0.));
#241163=CARTESIAN_POINT('Ctrl Pts',(-14.6824178576167,17.1785800350827,
12.));
#241164=CARTESIAN_POINT('Ctrl Pts',(-14.6785925615676,17.1746247499057,
0.));
#241165=CARTESIAN_POINT('Ctrl Pts',(-14.6785925615676,17.1746247499057,
12.));
#241166=CARTESIAN_POINT('Ctrl Pts',(-14.6749971333867,17.1708771619129,
0.));
#241167=CARTESIAN_POINT('Ctrl Pts',(-14.6749971333867,17.1708771619129,
12.));
#241168=CARTESIAN_POINT('Ctrl Pts',(-14.6716355833321,17.1673449723019,
0.));
#241169=CARTESIAN_POINT('Ctrl Pts',(-14.6716355833321,17.1673449723019,
12.));
#241170=CARTESIAN_POINT('Ctrl Pts',(-14.6685123374424,17.1640366762304,
0.));
#241171=CARTESIAN_POINT('Ctrl Pts',(-14.6685123374424,17.1640366762304,
12.));
#241172=CARTESIAN_POINT('Ctrl Pts',(-14.6656319165057,17.1609609517369,
0.));
#241173=CARTESIAN_POINT('Ctrl Pts',(-14.6656319165057,17.1609609517369,
12.));
#241174=CARTESIAN_POINT('Ctrl Pts',(-14.662998728599,17.1581262646789,0.));
#241175=CARTESIAN_POINT('Ctrl Pts',(-14.662998728599,17.1581262646789,12.));
#241176=CARTESIAN_POINT('Ctrl Pts',(-14.660616716964,17.1555401986403,0.));
#241177=CARTESIAN_POINT('Ctrl Pts',(-14.660616716964,17.1555401986403,12.));
#241178=CARTESIAN_POINT('Ctrl Pts',(-14.6584900555301,17.1532107762719,
0.));
#241179=CARTESIAN_POINT('Ctrl Pts',(-14.6584900555301,17.1532107762719,
12.));
#241180=CARTESIAN_POINT('Ctrl Pts',(-14.6566237952435,17.1511476869495,
0.));
#241181=CARTESIAN_POINT('Ctrl Pts',(-14.6566237952435,17.1511476869495,
12.));
#241182=CARTESIAN_POINT('Ctrl Pts',(-14.6550248622813,17.1493641837556,
0.));
#241183=CARTESIAN_POINT('Ctrl Pts',(-14.6550248622813,17.1493641837556,
12.));
#241184=CARTESIAN_POINT('Ctrl Pts',(-14.6537016966188,17.1478763944909,
0.));
#241185=CARTESIAN_POINT('Ctrl Pts',(-14.6537016966188,17.1478763944909,
12.));
#241186=CARTESIAN_POINT('Ctrl Pts',(-14.6526624064978,17.1466998098673,
0.));
#241187=CARTESIAN_POINT('Ctrl Pts',(-14.6526624064978,17.1466998098673,
12.));
#241188=CARTESIAN_POINT('Ctrl Pts',(-14.65191316345,17.1458462295273,0.));
#241189=CARTESIAN_POINT('Ctrl Pts',(-14.65191316345,17.1458462295273,12.));
#241190=CARTESIAN_POINT('Ctrl Pts',(-14.6515481598057,17.1454262858045,
0.));
#241191=CARTESIAN_POINT('Ctrl Pts',(-14.6515481598057,17.1454262858045,
12.));
#241192=CARTESIAN_POINT('Ctrl Pts',(-14.6514066997188,17.1452600887039,
0.));
#241193=CARTESIAN_POINT('Ctrl Pts',(-14.6514066997188,17.1452600887039,
12.));
#241194=CARTESIAN_POINT('Ctrl Pts',(-14.651371185284,17.1452153999142,0.));
#241195=CARTESIAN_POINT('Ctrl Pts',(-14.651371185284,17.1452153999142,12.));
#241196=CARTESIAN_POINT('Ctrl Pts',(-14.6513681262571,17.1452095830633,
0.));
#241197=CARTESIAN_POINT('Ctrl Pts',(-14.6513681262571,17.1452095830633,
12.));
#241198=CARTESIAN_POINT('',(-17.9112098770111,18.8464468996588,0.));
#241199=CARTESIAN_POINT('Ctrl Pts',(-17.9112098770111,18.8464468996588,
0.));
#241200=CARTESIAN_POINT('Ctrl Pts',(-17.9057348246595,18.8448126709691,
0.));
#241201=CARTESIAN_POINT('Ctrl Pts',(-17.8947931177807,18.8415402351786,
0.));
#241202=CARTESIAN_POINT('Ctrl Pts',(-17.8784057509356,18.8366196462581,
0.));
#241203=CARTESIAN_POINT('Ctrl Pts',(-17.8566063174771,18.8300349895974,
0.));
#241204=CARTESIAN_POINT('Ctrl Pts',(-17.8294410311006,18.8217643886157,
0.));
#241205=CARTESIAN_POINT('Ctrl Pts',(-17.8023598011057,18.8134540340417,
0.));
#241206=CARTESIAN_POINT('Ctrl Pts',(-17.7753627137853,18.8051039860448,
0.));
#241207=CARTESIAN_POINT('Ctrl Pts',(-17.7484498996905,18.7967143519419,
0.));
#241208=CARTESIAN_POINT('Ctrl Pts',(-17.7216215409035,18.7882852976049,
0.));
#241209=CARTESIAN_POINT('Ctrl Pts',(-17.6948778823014,18.7798170641374,
0.));
#241210=CARTESIAN_POINT('Ctrl Pts',(-17.6682192274236,18.7713099642754,
0.));
#241211=CARTESIAN_POINT('Ctrl Pts',(-17.6416459210681,18.762764361321,0.));
#241212=CARTESIAN_POINT('Ctrl Pts',(-17.6151583357012,18.7541806530984,
0.));
#241213=CARTESIAN_POINT('Ctrl Pts',(-17.5887568561371,18.7455592536687,
0.));
#241214=CARTESIAN_POINT('Ctrl Pts',(-17.5624418653245,18.7369005764553,
0.));
#241215=CARTESIAN_POINT('Ctrl Pts',(-17.5362137287593,18.7282050157138,
0.));
#241216=CARTESIAN_POINT('Ctrl Pts',(-17.5100727820876,18.7194729318098,
0.));
#241217=CARTESIAN_POINT('Ctrl Pts',(-17.4840193397162,18.7107046613912,
0.));
#241218=CARTESIAN_POINT('Ctrl Pts',(-17.4580537012753,18.70190052503,0.));
#241219=CARTESIAN_POINT('Ctrl Pts',(-17.4321761588142,18.6930608357409,
0.));
#241220=CARTESIAN_POINT('Ctrl Pts',(-17.4063870038562,18.6841859073471,
0.));
#241221=CARTESIAN_POINT('Ctrl Pts',(-17.3806865340747,18.6752760624052,
0.));
#241222=CARTESIAN_POINT('Ctrl Pts',(-17.3550750612443,18.6663316416582,
0.));
#241223=CARTESIAN_POINT('Ctrl Pts',(-17.3295529098618,18.6573530024033,
0.));
#241224=CARTESIAN_POINT('Ctrl Pts',(-17.3041204135074,18.6483405141865,
0.));
#241225=CARTESIAN_POINT('Ctrl Pts',(-17.2787779120213,18.6392945554748,
0.));
#241226=CARTESIAN_POINT('Ctrl Pts',(-17.2535257482187,18.6302155097943,
0.));
#241227=CARTESIAN_POINT('Ctrl Pts',(-17.2283642650518,18.6211037624038,
0.));
#241228=CARTESIAN_POINT('Ctrl Pts',(-17.2032938019284,18.6119596959949,
0.));
#241229=CARTESIAN_POINT('Ctrl Pts',(-17.1783146940127,18.6027836898817,
0.));
#241230=CARTESIAN_POINT('Ctrl Pts',(-17.1534272741643,18.5935761222825,
0.));
#241231=CARTESIAN_POINT('Ctrl Pts',(-17.1286318741183,18.5843373717247,
0.));
#241232=CARTESIAN_POINT('Ctrl Pts',(-17.1039288260001,18.5750678188542,
0.));
#241233=CARTESIAN_POINT('Ctrl Pts',(-17.0793184636079,18.5657678479789,
0.));
#241234=CARTESIAN_POINT('Ctrl Pts',(-17.0548011239751,18.556437848963,0.));
#241235=CARTESIAN_POINT('Ctrl Pts',(-17.0303771481738,18.547078218209,0.));
#241236=CARTESIAN_POINT('Ctrl Pts',(-17.0060468805097,18.5376893576961,
0.));
#241237=CARTESIAN_POINT('Ctrl Pts',(-16.981810668038,18.5282716744197,0.));
#241238=CARTESIAN_POINT('Ctrl Pts',(-16.9576688599339,18.5188255796659,
0.));
#241239=CARTESIAN_POINT('Ctrl Pts',(-16.9336218069353,18.5093514883835,
0.));
#241240=CARTESIAN_POINT('Ctrl Pts',(-16.9096698606943,18.499849818462,0.));
#241241=CARTESIAN_POINT('Ctrl Pts',(-16.8858133733088,18.4903209902227,
0.));
#241242=CARTESIAN_POINT('Ctrl Pts',(-16.8620526977171,18.480765426877,0.));
#241243=CARTESIAN_POINT('Ctrl Pts',(-16.8383881879709,18.4711835548623,
0.));
#241244=CARTESIAN_POINT('Ctrl Pts',(-16.8148201995472,18.4615758042305,
0.));
#241245=CARTESIAN_POINT('Ctrl Pts',(-16.791349089629,18.4519426090123,0.));
#241246=CARTESIAN_POINT('Ctrl Pts',(-16.7679752173992,18.44228440761,0.));
#241247=CARTESIAN_POINT('Ctrl Pts',(-16.7446989442882,18.4326016431392,
0.));
#241248=CARTESIAN_POINT('Ctrl Pts',(-16.7215206338818,18.4228947633187,
0.));
#241249=CARTESIAN_POINT('Ctrl Pts',(-16.6984406518491,18.413164220399,0.));
#241250=CARTESIAN_POINT('Ctrl Pts',(-16.6754593658513,18.403410471079,0.));
#241251=CARTESIAN_POINT('Ctrl Pts',(-16.6525771454513,18.3936339764332,
0.));
#241252=CARTESIAN_POINT('Ctrl Pts',(-16.6297943620056,18.3838352018327,
0.));
#241253=CARTESIAN_POINT('Ctrl Pts',(-16.607111388571,18.3740146168879,0.));
#241254=CARTESIAN_POINT('Ctrl Pts',(-16.5845286000217,18.3641726955889,
0.));
#241255=CARTESIAN_POINT('Ctrl Pts',(-16.5620463731413,18.354309916433,0.));
#241256=CARTESIAN_POINT('Ctrl Pts',(-16.5396650867139,18.34442676256,0.));
#241257=CARTESIAN_POINT('Ctrl Pts',(-16.5173851216045,18.3345237218864,
0.));
#241258=CARTESIAN_POINT('Ctrl Pts',(-16.4952068608345,18.3246012872469,
0.));
#241259=CARTESIAN_POINT('Ctrl Pts',(-16.4731306896441,18.3146599565231,
0.));
#241260=CARTESIAN_POINT('Ctrl Pts',(-16.4511569955233,18.304700232686,0.));
#241261=CARTESIAN_POINT('Ctrl Pts',(-16.4292861682379,18.294722623851,0.));
#241262=CARTESIAN_POINT('Ctrl Pts',(-16.4075185998455,18.2847276433309,
0.));
#241263=CARTESIAN_POINT('Ctrl Pts',(-16.385854684708,18.2747158096934,0.));
#241264=CARTESIAN_POINT('Ctrl Pts',(-16.3642948194868,18.2646876468169,
0.));
#241265=CARTESIAN_POINT('Ctrl Pts',(-16.3428394031589,18.2546436839608,
0.));
#241266=CARTESIAN_POINT('Ctrl Pts',(-16.3214888370987,18.2445844558741,
0.));
#241267=CARTESIAN_POINT('Ctrl Pts',(-16.3002435251378,18.2345105028982,
0.));
#241268=CARTESIAN_POINT('Ctrl Pts',(-16.2791038736223,18.2244223710745,
0.));
#241269=CARTESIAN_POINT('Ctrl Pts',(-16.2580702914615,18.2143206122529,
0.));
#241270=CARTESIAN_POINT('Ctrl Pts',(-16.2371431901638,18.2042057842035,
0.));
#241271=CARTESIAN_POINT('Ctrl Pts',(-16.2163229838875,18.1940784507229,
0.));
#241272=CARTESIAN_POINT('Ctrl Pts',(-16.1956100895073,18.1839391817331,
0.));
#241273=CARTESIAN_POINT('Ctrl Pts',(-16.1750049266671,18.1737885533849,
0.));
#241274=CARTESIAN_POINT('Ctrl Pts',(-16.154507917826,18.1636271481615,0.));
#241275=CARTESIAN_POINT('Ctrl Pts',(-16.1341194882988,18.1534555549852,
0.));
#241276=CARTESIAN_POINT('Ctrl Pts',(-16.1138400662794,18.1432743693235,
0.));
#241277=CARTESIAN_POINT('Ctrl Pts',(-16.0936700829112,18.1330841933105,
0.));
#241278=CARTESIAN_POINT('Ctrl Pts',(-16.0736099723668,18.1228856358751,
0.));
#241279=CARTESIAN_POINT('Ctrl Pts',(-16.0536601719126,18.112679312869,0.));
#241280=CARTESIAN_POINT('Ctrl Pts',(-16.0338211219693,18.1024658471966,
0.));
#241281=CARTESIAN_POINT('Ctrl Pts',(-16.014093266161,18.0922458689462,0.));
#241282=CARTESIAN_POINT('Ctrl Pts',(-15.9944770513613,18.0820200155236,
0.));
#241283=CARTESIAN_POINT('Ctrl Pts',(-15.9749729277846,18.0717889317958,
0.));
#241284=CARTESIAN_POINT('Ctrl Pts',(-15.9555813490644,18.0615532702359,
0.));
#241285=CARTESIAN_POINT('Ctrl Pts',(-15.9363027723244,18.0513136910691,
0.));
#241286=CARTESIAN_POINT('Ctrl Pts',(-15.9171376582436,18.0410708624208,
0.));
#241287=CARTESIAN_POINT('Ctrl Pts',(-15.8980864711042,18.0308254604636,
0.));
#241288=CARTESIAN_POINT('Ctrl Pts',(-15.8791496788683,18.0205781695769,
0.));
#241289=CARTESIAN_POINT('Ctrl Pts',(-15.8603277532831,18.0103296825205,
0.));
#241290=CARTESIAN_POINT('Ctrl Pts',(-15.8416211699679,18.0000807006052,
0.));
#241291=CARTESIAN_POINT('Ctrl Pts',(-15.8230304084962,17.9898319338664,
0.));
#241292=CARTESIAN_POINT('Ctrl Pts',(-15.8045559524676,17.9795841012386,
0.));
#241293=CARTESIAN_POINT('Ctrl Pts',(-15.7861982895724,17.9693379307303,
0.));
#241294=CARTESIAN_POINT('Ctrl Pts',(-15.7679579117077,17.9590941596242,
0.));
#241295=CARTESIAN_POINT('Ctrl Pts',(-15.749835315086,17.9488535346781,0.));
#241296=CARTESIAN_POINT('Ctrl Pts',(-15.7318310003335,17.9386168123262,
0.));
#241297=CARTESIAN_POINT('Ctrl Pts',(-15.7139454725838,17.9283847588835,
0.));
#241298=CARTESIAN_POINT('Ctrl Pts',(-15.6961792415522,17.9181581507455,
0.));
#241299=CARTESIAN_POINT('Ctrl Pts',(-15.678532821646,17.9079377746111,0.));
#241300=CARTESIAN_POINT('Ctrl Pts',(-15.661006732103,17.897724427724,0.));
#241301=CARTESIAN_POINT('Ctrl Pts',(-15.6436014971084,17.8875189181091,
0.));
#241302=CARTESIAN_POINT('Ctrl Pts',(-15.6263176459108,17.8773220648125,
0.));
#241303=CARTESIAN_POINT('Ctrl Pts',(-15.609155712921,17.8671346981394,0.));
#241304=CARTESIAN_POINT('Ctrl Pts',(-15.5921162378192,17.8569576599006,
0.));
#241305=CARTESIAN_POINT('Ctrl Pts',(-15.5751997657163,17.8467918036987,
0.));
#241306=CARTESIAN_POINT('Ctrl Pts',(-15.5584068472982,17.8366379952085,
0.));
#241307=CARTESIAN_POINT('Ctrl Pts',(-15.541738038964,17.8264971124606,0.));
#241308=CARTESIAN_POINT('Ctrl Pts',(-15.5251939029552,17.8163700461256,
0.));
#241309=CARTESIAN_POINT('Ctrl Pts',(-15.5087750074718,17.8062576997952,
0.));
#241310=CARTESIAN_POINT('Ctrl Pts',(-15.4924819268517,17.7961609903148,
0.));
#241311=CARTESIAN_POINT('Ctrl Pts',(-15.4763152417497,17.7860808481219,
0.));
#241312=CARTESIAN_POINT('Ctrl Pts',(-15.4602755393017,17.7760182175815,
0.));
#241313=CARTESIAN_POINT('Ctrl Pts',(-15.4443634132869,17.7659740573265,
0.));
#241314=CARTESIAN_POINT('Ctrl Pts',(-15.4285794642668,17.7559493405881,
0.));
#241315=CARTESIAN_POINT('Ctrl Pts',(-15.4129242997837,17.7459450555812,
0.));
#241316=CARTESIAN_POINT('Ctrl Pts',(-15.3973985345802,17.7359622059149,
0.));
#241317=CARTESIAN_POINT('Ctrl Pts',(-15.3820027907967,17.7260018109924,
0.));
#241318=CARTESIAN_POINT('Ctrl Pts',(-15.3667376981699,17.7160649064206,
0.));
#241319=CARTESIAN_POINT('Ctrl Pts',(-15.351603894206,17.7061525444042,0.));
#241320=CARTESIAN_POINT('Ctrl Pts',(-15.3366020244066,17.6962657941983,
0.));
#241321=CARTESIAN_POINT('Ctrl Pts',(-15.3217327425338,17.6864057426052,
0.));
#241322=CARTESIAN_POINT('Ctrl Pts',(-15.3069967108501,17.676573494456,0.));
#241323=CARTESIAN_POINT('Ctrl Pts',(-15.2923946003598,17.6667701731041,
0.));
#241324=CARTESIAN_POINT('Ctrl Pts',(-15.2779270910239,17.6569969209,0.));
#241325=CARTESIAN_POINT('Ctrl Pts',(-15.2635948720292,17.6472548997328,
0.));
#241326=CARTESIAN_POINT('Ctrl Pts',(-15.2493986421092,17.6375452916369,
0.));
#241327=CARTESIAN_POINT('Ctrl Pts',(-15.2353391098366,17.6278692993764,
0.));
#241328=CARTESIAN_POINT('Ctrl Pts',(-15.2214169939199,17.6182281470468,
0.));
#241329=CARTESIAN_POINT('Ctrl Pts',(-15.2076330234686,17.60862308065,0.));
#241330=CARTESIAN_POINT('Ctrl Pts',(-15.1939879383268,17.5990553687599,
0.));
#241331=CARTESIAN_POINT('Ctrl Pts',(-15.1804824894605,17.5895263032595,
0.));
#241332=CARTESIAN_POINT('Ctrl Pts',(-15.1671174393137,17.580037200054,0.));
#241333=CARTESIAN_POINT('Ctrl Pts',(-15.1538935621714,17.5705893998029,
0.));
#241334=CARTESIAN_POINT('Ctrl Pts',(-15.1408116444876,17.5611842686192,
0.));
#241335=CARTESIAN_POINT('Ctrl Pts',(-15.1278724853138,17.5518231989117,
0.));
#241336=CARTESIAN_POINT('Ctrl Pts',(-15.1150768967728,17.5425076102963,
0.));
#241337=CARTESIAN_POINT('Ctrl Pts',(-15.1024257045033,17.5332389504829,
0.));
#241338=CARTESIAN_POINT('Ctrl Pts',(-15.0899197481082,17.524018696179,0.));
#241339=CARTESIAN_POINT('Ctrl Pts',(-15.0775598815749,17.5148483539687,
0.));
#241340=CARTESIAN_POINT('Ctrl Pts',(-15.0653469738307,17.5057294613877,
0.));
#241341=CARTESIAN_POINT('Ctrl Pts',(-15.0532819093085,17.4966635880246,
0.));
#241342=CARTESIAN_POINT('Ctrl Pts',(-15.0413655884993,17.4876523366178,
0.));
#241343=CARTESIAN_POINT('Ctrl Pts',(-15.029598928488,17.4786973441417,0.));
#241344=CARTESIAN_POINT('Ctrl Pts',(-15.0179828635087,17.4698002829357,
0.));
#241345=CARTESIAN_POINT('Ctrl Pts',(-15.0065183456922,17.4609628621419,
0.));
#241346=CARTESIAN_POINT('Ctrl Pts',(-14.9952063457779,17.4521868291005,
0.));
#241347=CARTESIAN_POINT('Ctrl Pts',(-14.9840478538357,17.4434739707773,
0.));
#241348=CARTESIAN_POINT('Ctrl Pts',(-14.973043879945,17.4348261151395,0.));
#241349=CARTESIAN_POINT('Ctrl Pts',(-14.9621954549825,17.4262451327088,
0.));
#241350=CARTESIAN_POINT('Ctrl Pts',(-14.9515036315142,17.4177329382827,
0.));
#241351=CARTESIAN_POINT('Ctrl Pts',(-14.940969484645,17.4092914926071,0.));
#241352=CARTESIAN_POINT('Ctrl Pts',(-14.9305941128758,17.400922804075,0.));
#241353=CARTESIAN_POINT('Ctrl Pts',(-14.9203786389343,17.3926289303987,
0.));
#241354=CARTESIAN_POINT('Ctrl Pts',(-14.9103242110057,17.3844119809823,
0.));
#241355=CARTESIAN_POINT('Ctrl Pts',(-14.9004320039609,17.3762741193075,
0.));
#241356=CARTESIAN_POINT('Ctrl Pts',(-14.8907032205789,17.3682175653236,
0.));
#241357=CARTESIAN_POINT('Ctrl Pts',(-14.8811390927424,17.3602445978163,
0.));
#241358=CARTESIAN_POINT('Ctrl Pts',(-14.8717408826958,17.3523575568648,
0.));
#241359=CARTESIAN_POINT('Ctrl Pts',(-14.8625098843419,17.3445588463477,
0.));
#241360=CARTESIAN_POINT('Ctrl Pts',(-14.8534474245433,17.336850936485,0.));
#241361=CARTESIAN_POINT('Ctrl Pts',(-14.8445548643504,17.3292363662601,
0.));
#241362=CARTESIAN_POINT('Ctrl Pts',(-14.8358336004193,17.3217177462096,
0.));
#241363=CARTESIAN_POINT('Ctrl Pts',(-14.8272850675375,17.3142977632656,
0.));
#241364=CARTESIAN_POINT('Ctrl Pts',(-14.8189107410161,17.3069791853705,
0.));
#241365=CARTESIAN_POINT('Ctrl Pts',(-14.8107121391038,17.2997648661483,
0.));
#241366=CARTESIAN_POINT('Ctrl Pts',(-14.8026908254281,17.2926577496519,
0.));
#241367=CARTESIAN_POINT('Ctrl Pts',(-14.7948484105253,17.28566087332,0.));
#241368=CARTESIAN_POINT('Ctrl Pts',(-14.787186553128,17.278777370485,0.));
#241369=CARTESIAN_POINT('Ctrl Pts',(-14.7797069617802,17.2720104735192,
0.));
#241370=CARTESIAN_POINT('Ctrl Pts',(-14.7724113956728,17.2653635155317,
0.));
#241371=CARTESIAN_POINT('Ctrl Pts',(-14.7653016697589,17.2588399401464,
0.));
#241372=CARTESIAN_POINT('Ctrl Pts',(-14.7583796616617,17.2524433146837,
0.));
#241373=CARTESIAN_POINT('Ctrl Pts',(-14.7516473175125,17.2461773413289,
0.));
#241374=CARTESIAN_POINT('Ctrl Pts',(-14.7451066593793,17.2400458713566,
0.));
#241375=CARTESIAN_POINT('Ctrl Pts',(-14.7387597858117,17.2340529062077,
0.));
#241376=CARTESIAN_POINT('Ctrl Pts',(-14.7326088681163,17.2282025904314,
0.));
#241377=CARTESIAN_POINT('Ctrl Pts',(-14.7266561494282,17.2224992099666,
0.));
#241378=CARTESIAN_POINT('Ctrl Pts',(-14.7209039390326,17.2169471814255,
0.));
#241379=CARTESIAN_POINT('Ctrl Pts',(-14.7153546289338,17.2115510835988,
0.));
#241380=CARTESIAN_POINT('Ctrl Pts',(-14.7100107213586,17.2063157097316,
0.));
#241381=CARTESIAN_POINT('Ctrl Pts',(-14.7048748502663,17.2012461084268,
0.));
#241382=CARTESIAN_POINT('Ctrl Pts',(-14.699949811582,17.1963476411694,0.));
#241383=CARTESIAN_POINT('Ctrl Pts',(-14.6952385361706,17.1916259308415,
0.));
#241384=CARTESIAN_POINT('Ctrl Pts',(-14.6907440526958,17.1870867909918,
0.));
#241385=CARTESIAN_POINT('Ctrl Pts',(-14.6864694522319,17.182736158472,0.));
#241386=CARTESIAN_POINT('Ctrl Pts',(-14.6824178576167,17.1785800350827,
0.));
#241387=CARTESIAN_POINT('Ctrl Pts',(-14.6785925615676,17.1746247499057,
0.));
#241388=CARTESIAN_POINT('Ctrl Pts',(-14.6749971333867,17.1708771619129,
0.));
#241389=CARTESIAN_POINT('Ctrl Pts',(-14.6716355833321,17.1673449723019,
0.));
#241390=CARTESIAN_POINT('Ctrl Pts',(-14.6685123374424,17.1640366762304,
0.));
#241391=CARTESIAN_POINT('Ctrl Pts',(-14.6656319165057,17.1609609517369,
0.));
#241392=CARTESIAN_POINT('Ctrl Pts',(-14.662998728599,17.1581262646789,0.));
#241393=CARTESIAN_POINT('Ctrl Pts',(-14.660616716964,17.1555401986403,0.));
#241394=CARTESIAN_POINT('Ctrl Pts',(-14.6584900555301,17.1532107762719,
0.));
#241395=CARTESIAN_POINT('Ctrl Pts',(-14.6566237952435,17.1511476869495,
0.));
#241396=CARTESIAN_POINT('Ctrl Pts',(-14.6550248622813,17.1493641837556,
0.));
#241397=CARTESIAN_POINT('Ctrl Pts',(-14.6537016966188,17.1478763944909,
0.));
#241398=CARTESIAN_POINT('Ctrl Pts',(-14.6526624064978,17.1466998098673,
0.));
#241399=CARTESIAN_POINT('Ctrl Pts',(-14.65191316345,17.1458462295273,0.));
#241400=CARTESIAN_POINT('Ctrl Pts',(-14.6515481598057,17.1454262858045,
0.));
#241401=CARTESIAN_POINT('Ctrl Pts',(-14.6514066997188,17.1452600887039,
0.));
#241402=CARTESIAN_POINT('Ctrl Pts',(-14.651371185284,17.1452153999142,0.));
#241403=CARTESIAN_POINT('Ctrl Pts',(-14.6513681262571,17.1452095830633,
0.));
#241404=CARTESIAN_POINT('',(-17.9112098770111,18.8464468996588,12.));
#241405=CARTESIAN_POINT('',(-17.9112098770111,18.8464468996588,0.));
#241406=CARTESIAN_POINT('Ctrl Pts',(-14.6513681262571,17.1452095830633,
12.));
#241407=CARTESIAN_POINT('Ctrl Pts',(-14.651371185284,17.1452153999142,12.));
#241408=CARTESIAN_POINT('Ctrl Pts',(-14.6514066997188,17.1452600887039,
12.));
#241409=CARTESIAN_POINT('Ctrl Pts',(-14.6515481598057,17.1454262858045,
12.));
#241410=CARTESIAN_POINT('Ctrl Pts',(-14.65191316345,17.1458462295273,12.));
#241411=CARTESIAN_POINT('Ctrl Pts',(-14.6526624064978,17.1466998098673,
12.));
#241412=CARTESIAN_POINT('Ctrl Pts',(-14.6537016966188,17.1478763944909,
12.));
#241413=CARTESIAN_POINT('Ctrl Pts',(-14.6550248622813,17.1493641837556,
12.));
#241414=CARTESIAN_POINT('Ctrl Pts',(-14.6566237952435,17.1511476869495,
12.));
#241415=CARTESIAN_POINT('Ctrl Pts',(-14.6584900555301,17.1532107762719,
12.));
#241416=CARTESIAN_POINT('Ctrl Pts',(-14.660616716964,17.1555401986403,12.));
#241417=CARTESIAN_POINT('Ctrl Pts',(-14.662998728599,17.1581262646789,12.));
#241418=CARTESIAN_POINT('Ctrl Pts',(-14.6656319165057,17.1609609517369,
12.));
#241419=CARTESIAN_POINT('Ctrl Pts',(-14.6685123374424,17.1640366762304,
12.));
#241420=CARTESIAN_POINT('Ctrl Pts',(-14.6716355833321,17.1673449723019,
12.));
#241421=CARTESIAN_POINT('Ctrl Pts',(-14.6749971333867,17.1708771619129,
12.));
#241422=CARTESIAN_POINT('Ctrl Pts',(-14.6785925615676,17.1746247499057,
12.));
#241423=CARTESIAN_POINT('Ctrl Pts',(-14.6824178576167,17.1785800350827,
12.));
#241424=CARTESIAN_POINT('Ctrl Pts',(-14.6864694522319,17.182736158472,12.));
#241425=CARTESIAN_POINT('Ctrl Pts',(-14.6907440526958,17.1870867909918,
12.));
#241426=CARTESIAN_POINT('Ctrl Pts',(-14.6952385361706,17.1916259308415,
12.));
#241427=CARTESIAN_POINT('Ctrl Pts',(-14.699949811582,17.1963476411694,12.));
#241428=CARTESIAN_POINT('Ctrl Pts',(-14.7048748502663,17.2012461084268,
12.));
#241429=CARTESIAN_POINT('Ctrl Pts',(-14.7100107213586,17.2063157097316,
12.));
#241430=CARTESIAN_POINT('Ctrl Pts',(-14.7153546289338,17.2115510835988,
12.));
#241431=CARTESIAN_POINT('Ctrl Pts',(-14.7209039390326,17.2169471814255,
12.));
#241432=CARTESIAN_POINT('Ctrl Pts',(-14.7266561494282,17.2224992099666,
12.));
#241433=CARTESIAN_POINT('Ctrl Pts',(-14.7326088681163,17.2282025904314,
12.));
#241434=CARTESIAN_POINT('Ctrl Pts',(-14.7387597858117,17.2340529062077,
12.));
#241435=CARTESIAN_POINT('Ctrl Pts',(-14.7451066593793,17.2400458713566,
12.));
#241436=CARTESIAN_POINT('Ctrl Pts',(-14.7516473175125,17.2461773413289,
12.));
#241437=CARTESIAN_POINT('Ctrl Pts',(-14.7583796616617,17.2524433146837,
12.));
#241438=CARTESIAN_POINT('Ctrl Pts',(-14.7653016697589,17.2588399401464,
12.));
#241439=CARTESIAN_POINT('Ctrl Pts',(-14.7724113956728,17.2653635155317,
12.));
#241440=CARTESIAN_POINT('Ctrl Pts',(-14.7797069617802,17.2720104735192,
12.));
#241441=CARTESIAN_POINT('Ctrl Pts',(-14.787186553128,17.278777370485,12.));
#241442=CARTESIAN_POINT('Ctrl Pts',(-14.7948484105253,17.28566087332,12.));
#241443=CARTESIAN_POINT('Ctrl Pts',(-14.8026908254281,17.2926577496519,
12.));
#241444=CARTESIAN_POINT('Ctrl Pts',(-14.8107121391038,17.2997648661483,
12.));
#241445=CARTESIAN_POINT('Ctrl Pts',(-14.8189107410161,17.3069791853705,
12.));
#241446=CARTESIAN_POINT('Ctrl Pts',(-14.8272850675375,17.3142977632656,
12.));
#241447=CARTESIAN_POINT('Ctrl Pts',(-14.8358336004193,17.3217177462096,
12.));
#241448=CARTESIAN_POINT('Ctrl Pts',(-14.8445548643504,17.3292363662601,
12.));
#241449=CARTESIAN_POINT('Ctrl Pts',(-14.8534474245433,17.336850936485,12.));
#241450=CARTESIAN_POINT('Ctrl Pts',(-14.8625098843419,17.3445588463477,
12.));
#241451=CARTESIAN_POINT('Ctrl Pts',(-14.8717408826958,17.3523575568648,
12.));
#241452=CARTESIAN_POINT('Ctrl Pts',(-14.8811390927424,17.3602445978163,
12.));
#241453=CARTESIAN_POINT('Ctrl Pts',(-14.8907032205789,17.3682175653236,
12.));
#241454=CARTESIAN_POINT('Ctrl Pts',(-14.9004320039609,17.3762741193075,
12.));
#241455=CARTESIAN_POINT('Ctrl Pts',(-14.9103242110057,17.3844119809823,
12.));
#241456=CARTESIAN_POINT('Ctrl Pts',(-14.9203786389343,17.3926289303987,
12.));
#241457=CARTESIAN_POINT('Ctrl Pts',(-14.9305941128758,17.400922804075,12.));
#241458=CARTESIAN_POINT('Ctrl Pts',(-14.940969484645,17.4092914926071,12.));
#241459=CARTESIAN_POINT('Ctrl Pts',(-14.9515036315142,17.4177329382827,
12.));
#241460=CARTESIAN_POINT('Ctrl Pts',(-14.9621954549825,17.4262451327088,
12.));
#241461=CARTESIAN_POINT('Ctrl Pts',(-14.973043879945,17.4348261151395,12.));
#241462=CARTESIAN_POINT('Ctrl Pts',(-14.9840478538357,17.4434739707773,
12.));
#241463=CARTESIAN_POINT('Ctrl Pts',(-14.9952063457779,17.4521868291005,
12.));
#241464=CARTESIAN_POINT('Ctrl Pts',(-15.0065183456922,17.4609628621419,
12.));
#241465=CARTESIAN_POINT('Ctrl Pts',(-15.0179828635087,17.4698002829357,
12.));
#241466=CARTESIAN_POINT('Ctrl Pts',(-15.029598928488,17.4786973441417,12.));
#241467=CARTESIAN_POINT('Ctrl Pts',(-15.0413655884993,17.4876523366178,
12.));
#241468=CARTESIAN_POINT('Ctrl Pts',(-15.0532819093085,17.4966635880246,
12.));
#241469=CARTESIAN_POINT('Ctrl Pts',(-15.0653469738307,17.5057294613877,
12.));
#241470=CARTESIAN_POINT('Ctrl Pts',(-15.0775598815749,17.5148483539687,
12.));
#241471=CARTESIAN_POINT('Ctrl Pts',(-15.0899197481082,17.524018696179,12.));
#241472=CARTESIAN_POINT('Ctrl Pts',(-15.1024257045033,17.5332389504829,
12.));
#241473=CARTESIAN_POINT('Ctrl Pts',(-15.1150768967728,17.5425076102963,
12.));
#241474=CARTESIAN_POINT('Ctrl Pts',(-15.1278724853138,17.5518231989117,
12.));
#241475=CARTESIAN_POINT('Ctrl Pts',(-15.1408116444876,17.5611842686192,
12.));
#241476=CARTESIAN_POINT('Ctrl Pts',(-15.1538935621714,17.5705893998029,
12.));
#241477=CARTESIAN_POINT('Ctrl Pts',(-15.1671174393137,17.580037200054,12.));
#241478=CARTESIAN_POINT('Ctrl Pts',(-15.1804824894605,17.5895263032595,
12.));
#241479=CARTESIAN_POINT('Ctrl Pts',(-15.1939879383268,17.5990553687599,
12.));
#241480=CARTESIAN_POINT('Ctrl Pts',(-15.2076330234686,17.60862308065,12.));
#241481=CARTESIAN_POINT('Ctrl Pts',(-15.2214169939199,17.6182281470468,
12.));
#241482=CARTESIAN_POINT('Ctrl Pts',(-15.2353391098366,17.6278692993764,
12.));
#241483=CARTESIAN_POINT('Ctrl Pts',(-15.2493986421092,17.6375452916369,
12.));
#241484=CARTESIAN_POINT('Ctrl Pts',(-15.2635948720292,17.6472548997328,
12.));
#241485=CARTESIAN_POINT('Ctrl Pts',(-15.2779270910239,17.6569969209,12.));
#241486=CARTESIAN_POINT('Ctrl Pts',(-15.2923946003598,17.6667701731041,
12.));
#241487=CARTESIAN_POINT('Ctrl Pts',(-15.3069967108501,17.676573494456,12.));
#241488=CARTESIAN_POINT('Ctrl Pts',(-15.3217327425338,17.6864057426052,
12.));
#241489=CARTESIAN_POINT('Ctrl Pts',(-15.3366020244066,17.6962657941983,
12.));
#241490=CARTESIAN_POINT('Ctrl Pts',(-15.351603894206,17.7061525444042,12.));
#241491=CARTESIAN_POINT('Ctrl Pts',(-15.3667376981699,17.7160649064206,
12.));
#241492=CARTESIAN_POINT('Ctrl Pts',(-15.3820027907967,17.7260018109924,
12.));
#241493=CARTESIAN_POINT('Ctrl Pts',(-15.3973985345802,17.7359622059149,
12.));
#241494=CARTESIAN_POINT('Ctrl Pts',(-15.4129242997837,17.7459450555812,
12.));
#241495=CARTESIAN_POINT('Ctrl Pts',(-15.4285794642668,17.7559493405881,
12.));
#241496=CARTESIAN_POINT('Ctrl Pts',(-15.4443634132869,17.7659740573265,
12.));
#241497=CARTESIAN_POINT('Ctrl Pts',(-15.4602755393017,17.7760182175815,
12.));
#241498=CARTESIAN_POINT('Ctrl Pts',(-15.4763152417497,17.7860808481219,
12.));
#241499=CARTESIAN_POINT('Ctrl Pts',(-15.4924819268517,17.7961609903148,
12.));
#241500=CARTESIAN_POINT('Ctrl Pts',(-15.5087750074718,17.8062576997952,
12.));
#241501=CARTESIAN_POINT('Ctrl Pts',(-15.5251939029552,17.8163700461256,
12.));
#241502=CARTESIAN_POINT('Ctrl Pts',(-15.541738038964,17.8264971124606,12.));
#241503=CARTESIAN_POINT('Ctrl Pts',(-15.5584068472982,17.8366379952085,
12.));
#241504=CARTESIAN_POINT('Ctrl Pts',(-15.5751997657163,17.8467918036987,
12.));
#241505=CARTESIAN_POINT('Ctrl Pts',(-15.5921162378192,17.8569576599006,
12.));
#241506=CARTESIAN_POINT('Ctrl Pts',(-15.609155712921,17.8671346981394,12.));
#241507=CARTESIAN_POINT('Ctrl Pts',(-15.6263176459108,17.8773220648125,
12.));
#241508=CARTESIAN_POINT('Ctrl Pts',(-15.6436014971084,17.8875189181091,
12.));
#241509=CARTESIAN_POINT('Ctrl Pts',(-15.661006732103,17.897724427724,12.));
#241510=CARTESIAN_POINT('Ctrl Pts',(-15.678532821646,17.9079377746111,12.));
#241511=CARTESIAN_POINT('Ctrl Pts',(-15.6961792415522,17.9181581507455,
12.));
#241512=CARTESIAN_POINT('Ctrl Pts',(-15.7139454725838,17.9283847588835,
12.));
#241513=CARTESIAN_POINT('Ctrl Pts',(-15.7318310003335,17.9386168123262,
12.));
#241514=CARTESIAN_POINT('Ctrl Pts',(-15.749835315086,17.9488535346781,12.));
#241515=CARTESIAN_POINT('Ctrl Pts',(-15.7679579117077,17.9590941596242,
12.));
#241516=CARTESIAN_POINT('Ctrl Pts',(-15.7861982895724,17.9693379307303,
12.));
#241517=CARTESIAN_POINT('Ctrl Pts',(-15.8045559524676,17.9795841012386,
12.));
#241518=CARTESIAN_POINT('Ctrl Pts',(-15.8230304084962,17.9898319338664,
12.));
#241519=CARTESIAN_POINT('Ctrl Pts',(-15.8416211699679,18.0000807006052,
12.));
#241520=CARTESIAN_POINT('Ctrl Pts',(-15.8603277532831,18.0103296825205,
12.));
#241521=CARTESIAN_POINT('Ctrl Pts',(-15.8791496788683,18.0205781695769,
12.));
#241522=CARTESIAN_POINT('Ctrl Pts',(-15.8980864711042,18.0308254604636,
12.));
#241523=CARTESIAN_POINT('Ctrl Pts',(-15.9171376582436,18.0410708624208,
12.));
#241524=CARTESIAN_POINT('Ctrl Pts',(-15.9363027723244,18.0513136910691,
12.));
#241525=CARTESIAN_POINT('Ctrl Pts',(-15.9555813490644,18.0615532702359,
12.));
#241526=CARTESIAN_POINT('Ctrl Pts',(-15.9749729277846,18.0717889317958,
12.));
#241527=CARTESIAN_POINT('Ctrl Pts',(-15.9944770513613,18.0820200155236,
12.));
#241528=CARTESIAN_POINT('Ctrl Pts',(-16.014093266161,18.0922458689462,12.));
#241529=CARTESIAN_POINT('Ctrl Pts',(-16.0338211219693,18.1024658471966,
12.));
#241530=CARTESIAN_POINT('Ctrl Pts',(-16.0536601719126,18.112679312869,12.));
#241531=CARTESIAN_POINT('Ctrl Pts',(-16.0736099723668,18.1228856358751,
12.));
#241532=CARTESIAN_POINT('Ctrl Pts',(-16.0936700829112,18.1330841933105,
12.));
#241533=CARTESIAN_POINT('Ctrl Pts',(-16.1138400662794,18.1432743693235,
12.));
#241534=CARTESIAN_POINT('Ctrl Pts',(-16.1341194882988,18.1534555549852,
12.));
#241535=CARTESIAN_POINT('Ctrl Pts',(-16.154507917826,18.1636271481615,12.));
#241536=CARTESIAN_POINT('Ctrl Pts',(-16.1750049266671,18.1737885533849,
12.));
#241537=CARTESIAN_POINT('Ctrl Pts',(-16.1956100895073,18.1839391817331,
12.));
#241538=CARTESIAN_POINT('Ctrl Pts',(-16.2163229838875,18.1940784507229,
12.));
#241539=CARTESIAN_POINT('Ctrl Pts',(-16.2371431901638,18.2042057842035,
12.));
#241540=CARTESIAN_POINT('Ctrl Pts',(-16.2580702914615,18.2143206122529,
12.));
#241541=CARTESIAN_POINT('Ctrl Pts',(-16.2791038736223,18.2244223710745,
12.));
#241542=CARTESIAN_POINT('Ctrl Pts',(-16.3002435251378,18.2345105028982,
12.));
#241543=CARTESIAN_POINT('Ctrl Pts',(-16.3214888370987,18.2445844558741,
12.));
#241544=CARTESIAN_POINT('Ctrl Pts',(-16.3428394031589,18.2546436839608,
12.));
#241545=CARTESIAN_POINT('Ctrl Pts',(-16.3642948194868,18.2646876468169,
12.));
#241546=CARTESIAN_POINT('Ctrl Pts',(-16.385854684708,18.2747158096934,12.));
#241547=CARTESIAN_POINT('Ctrl Pts',(-16.4075185998455,18.2847276433309,
12.));
#241548=CARTESIAN_POINT('Ctrl Pts',(-16.4292861682379,18.294722623851,12.));
#241549=CARTESIAN_POINT('Ctrl Pts',(-16.4511569955233,18.304700232686,12.));
#241550=CARTESIAN_POINT('Ctrl Pts',(-16.4731306896441,18.3146599565231,
12.));
#241551=CARTESIAN_POINT('Ctrl Pts',(-16.4952068608345,18.3246012872469,
12.));
#241552=CARTESIAN_POINT('Ctrl Pts',(-16.5173851216045,18.3345237218864,
12.));
#241553=CARTESIAN_POINT('Ctrl Pts',(-16.5396650867139,18.34442676256,12.));
#241554=CARTESIAN_POINT('Ctrl Pts',(-16.5620463731413,18.354309916433,12.));
#241555=CARTESIAN_POINT('Ctrl Pts',(-16.5845286000217,18.3641726955889,
12.));
#241556=CARTESIAN_POINT('Ctrl Pts',(-16.607111388571,18.3740146168879,12.));
#241557=CARTESIAN_POINT('Ctrl Pts',(-16.6297943620056,18.3838352018327,
12.));
#241558=CARTESIAN_POINT('Ctrl Pts',(-16.6525771454513,18.3936339764332,
12.));
#241559=CARTESIAN_POINT('Ctrl Pts',(-16.6754593658513,18.403410471079,12.));
#241560=CARTESIAN_POINT('Ctrl Pts',(-16.6984406518491,18.413164220399,12.));
#241561=CARTESIAN_POINT('Ctrl Pts',(-16.7215206338818,18.4228947633187,
12.));
#241562=CARTESIAN_POINT('Ctrl Pts',(-16.7446989442882,18.4326016431392,
12.));
#241563=CARTESIAN_POINT('Ctrl Pts',(-16.7679752173992,18.44228440761,12.));
#241564=CARTESIAN_POINT('Ctrl Pts',(-16.791349089629,18.4519426090123,12.));
#241565=CARTESIAN_POINT('Ctrl Pts',(-16.8148201995472,18.4615758042305,
12.));
#241566=CARTESIAN_POINT('Ctrl Pts',(-16.8383881879709,18.4711835548623,
12.));
#241567=CARTESIAN_POINT('Ctrl Pts',(-16.8620526977171,18.480765426877,12.));
#241568=CARTESIAN_POINT('Ctrl Pts',(-16.8858133733088,18.4903209902227,
12.));
#241569=CARTESIAN_POINT('Ctrl Pts',(-16.9096698606943,18.499849818462,12.));
#241570=CARTESIAN_POINT('Ctrl Pts',(-16.9336218069353,18.5093514883835,
12.));
#241571=CARTESIAN_POINT('Ctrl Pts',(-16.9576688599339,18.5188255796659,
12.));
#241572=CARTESIAN_POINT('Ctrl Pts',(-16.981810668038,18.5282716744197,12.));
#241573=CARTESIAN_POINT('Ctrl Pts',(-17.0060468805097,18.5376893576961,
12.));
#241574=CARTESIAN_POINT('Ctrl Pts',(-17.0303771481738,18.547078218209,12.));
#241575=CARTESIAN_POINT('Ctrl Pts',(-17.0548011239751,18.556437848963,12.));
#241576=CARTESIAN_POINT('Ctrl Pts',(-17.0793184636079,18.5657678479789,
12.));
#241577=CARTESIAN_POINT('Ctrl Pts',(-17.1039288260001,18.5750678188542,
12.));
#241578=CARTESIAN_POINT('Ctrl Pts',(-17.1286318741183,18.5843373717247,
12.));
#241579=CARTESIAN_POINT('Ctrl Pts',(-17.1534272741643,18.5935761222825,
12.));
#241580=CARTESIAN_POINT('Ctrl Pts',(-17.1783146940127,18.6027836898817,
12.));
#241581=CARTESIAN_POINT('Ctrl Pts',(-17.2032938019284,18.6119596959949,
12.));
#241582=CARTESIAN_POINT('Ctrl Pts',(-17.2283642650518,18.6211037624038,
12.));
#241583=CARTESIAN_POINT('Ctrl Pts',(-17.2535257482187,18.6302155097943,
12.));
#241584=CARTESIAN_POINT('Ctrl Pts',(-17.2787779120213,18.6392945554748,
12.));
#241585=CARTESIAN_POINT('Ctrl Pts',(-17.3041204135074,18.6483405141865,
12.));
#241586=CARTESIAN_POINT('Ctrl Pts',(-17.3295529098618,18.6573530024033,
12.));
#241587=CARTESIAN_POINT('Ctrl Pts',(-17.3550750612443,18.6663316416582,
12.));
#241588=CARTESIAN_POINT('Ctrl Pts',(-17.3806865340747,18.6752760624052,
12.));
#241589=CARTESIAN_POINT('Ctrl Pts',(-17.4063870038562,18.6841859073471,
12.));
#241590=CARTESIAN_POINT('Ctrl Pts',(-17.4321761588142,18.6930608357409,
12.));
#241591=CARTESIAN_POINT('Ctrl Pts',(-17.4580537012753,18.70190052503,12.));
#241592=CARTESIAN_POINT('Ctrl Pts',(-17.4840193397162,18.7107046613912,
12.));
#241593=CARTESIAN_POINT('Ctrl Pts',(-17.5100727820876,18.7194729318098,
12.));
#241594=CARTESIAN_POINT('Ctrl Pts',(-17.5362137287593,18.7282050157138,
12.));
#241595=CARTESIAN_POINT('Ctrl Pts',(-17.5624418653245,18.7369005764553,
12.));
#241596=CARTESIAN_POINT('Ctrl Pts',(-17.5887568561371,18.7455592536687,
12.));
#241597=CARTESIAN_POINT('Ctrl Pts',(-17.6151583357012,18.7541806530984,
12.));
#241598=CARTESIAN_POINT('Ctrl Pts',(-17.6416459210681,18.762764361321,12.));
#241599=CARTESIAN_POINT('Ctrl Pts',(-17.6682192274236,18.7713099642754,
12.));
#241600=CARTESIAN_POINT('Ctrl Pts',(-17.6948778823014,18.7798170641374,
12.));
#241601=CARTESIAN_POINT('Ctrl Pts',(-17.7216215409035,18.7882852976049,
12.));
#241602=CARTESIAN_POINT('Ctrl Pts',(-17.7484498996905,18.7967143519419,
12.));
#241603=CARTESIAN_POINT('Ctrl Pts',(-17.7753627137853,18.8051039860448,
12.));
#241604=CARTESIAN_POINT('Ctrl Pts',(-17.8023598011057,18.8134540340417,
12.));
#241605=CARTESIAN_POINT('Ctrl Pts',(-17.8294410311006,18.8217643886157,
12.));
#241606=CARTESIAN_POINT('Ctrl Pts',(-17.8566063174771,18.8300349895974,
12.));
#241607=CARTESIAN_POINT('Ctrl Pts',(-17.8784057509356,18.8366196462581,
12.));
#241608=CARTESIAN_POINT('Ctrl Pts',(-17.8947931177807,18.8415402351786,
12.));
#241609=CARTESIAN_POINT('Ctrl Pts',(-17.9057348246595,18.8448126709691,
12.));
#241610=CARTESIAN_POINT('Ctrl Pts',(-17.9112098770111,18.8464468996588,
12.));
#241611=CARTESIAN_POINT('Ctrl Pts',(-12.7689476255363,18.5896416359912,
0.));
#241612=CARTESIAN_POINT('Ctrl Pts',(-12.7689476255363,18.5896416359912,
12.));
#241613=CARTESIAN_POINT('Ctrl Pts',(-12.7689524524483,18.5896460962964,
0.));
#241614=CARTESIAN_POINT('Ctrl Pts',(-12.7689524524483,18.5896460962964,
12.));
#241615=CARTESIAN_POINT('Ctrl Pts',(-12.768986426692,18.5896919669165,0.));
#241616=CARTESIAN_POINT('Ctrl Pts',(-12.768986426692,18.5896919669165,12.));
#241617=CARTESIAN_POINT('Ctrl Pts',(-12.769110348199,18.589871621843,0.));
#241618=CARTESIAN_POINT('Ctrl Pts',(-12.769110348199,18.589871621843,12.));
#241619=CARTESIAN_POINT('Ctrl Pts',(-12.7694215127919,18.5903328777227,
0.));
#241620=CARTESIAN_POINT('Ctrl Pts',(-12.7694215127919,18.5903328777227,
12.));
#241621=CARTESIAN_POINT('Ctrl Pts',(-12.7700520897173,18.5912775137806,
0.));
#241622=CARTESIAN_POINT('Ctrl Pts',(-12.7700520897173,18.5912775137806,
12.));
#241623=CARTESIAN_POINT('Ctrl Pts',(-12.7709195951156,18.5925859134579,
0.));
#241624=CARTESIAN_POINT('Ctrl Pts',(-12.7709195951156,18.5925859134579,
12.));
#241625=CARTESIAN_POINT('Ctrl Pts',(-12.7720142287172,18.5942490615407,
0.));
#241626=CARTESIAN_POINT('Ctrl Pts',(-12.7720142287172,18.5942490615407,
12.));
#241627=CARTESIAN_POINT('Ctrl Pts',(-12.7733231262108,18.5962551167772,
0.));
#241628=CARTESIAN_POINT('Ctrl Pts',(-12.7733231262108,18.5962551167772,
12.));
#241629=CARTESIAN_POINT('Ctrl Pts',(-12.7748328937638,18.598591752595,0.));
#241630=CARTESIAN_POINT('Ctrl Pts',(-12.7748328937638,18.598591752595,12.));
#241631=CARTESIAN_POINT('Ctrl Pts',(-12.7765325225081,18.6012488486709,
0.));
#241632=CARTESIAN_POINT('Ctrl Pts',(-12.7765325225081,18.6012488486709,
12.));
#241633=CARTESIAN_POINT('Ctrl Pts',(-12.7784139605066,18.6042190183704,
0.));
#241634=CARTESIAN_POINT('Ctrl Pts',(-12.7784139605066,18.6042190183704,
12.));
#241635=CARTESIAN_POINT('Ctrl Pts',(-12.7804705387658,18.6074961535723,
0.));
#241636=CARTESIAN_POINT('Ctrl Pts',(-12.7804705387658,18.6074961535723,
12.));
#241637=CARTESIAN_POINT('Ctrl Pts',(-12.7826959526925,18.6110744826219,
0.));
#241638=CARTESIAN_POINT('Ctrl Pts',(-12.7826959526925,18.6110744826219,
12.));
#241639=CARTESIAN_POINT('Ctrl Pts',(-12.7850831657901,18.6149475565188,
0.));
#241640=CARTESIAN_POINT('Ctrl Pts',(-12.7850831657901,18.6149475565188,
12.));
#241641=CARTESIAN_POINT('Ctrl Pts',(-12.7876249657834,18.6191087624752,
0.));
#241642=CARTESIAN_POINT('Ctrl Pts',(-12.7876249657834,18.6191087624752,
12.));
#241643=CARTESIAN_POINT('Ctrl Pts',(-12.7903142925234,18.6235516265575,
0.));
#241644=CARTESIAN_POINT('Ctrl Pts',(-12.7903142925234,18.6235516265575,
12.));
#241645=CARTESIAN_POINT('Ctrl Pts',(-12.7931447451555,18.6282702819371,
0.));
#241646=CARTESIAN_POINT('Ctrl Pts',(-12.7931447451555,18.6282702819371,
12.));
#241647=CARTESIAN_POINT('Ctrl Pts',(-12.7961106222251,18.6332595057006,
0.));
#241648=CARTESIAN_POINT('Ctrl Pts',(-12.7961106222251,18.6332595057006,
12.));
#241649=CARTESIAN_POINT('Ctrl Pts',(-12.7992066625264,18.63851447924,0.));
#241650=CARTESIAN_POINT('Ctrl Pts',(-12.7992066625264,18.63851447924,12.));
#241651=CARTESIAN_POINT('Ctrl Pts',(-12.8024278770152,18.6440306327456,
0.));
#241652=CARTESIAN_POINT('Ctrl Pts',(-12.8024278770152,18.6440306327456,
12.));
#241653=CARTESIAN_POINT('Ctrl Pts',(-12.805769331162,18.6498034438986,0.));
#241654=CARTESIAN_POINT('Ctrl Pts',(-12.805769331162,18.6498034438986,12.));
#241655=CARTESIAN_POINT('Ctrl Pts',(-12.8092261933858,18.6558284825773,
0.));
#241656=CARTESIAN_POINT('Ctrl Pts',(-12.8092261933858,18.6558284825773,
12.));
#241657=CARTESIAN_POINT('Ctrl Pts',(-12.8127937909631,18.6621014624746,
0.));
#241658=CARTESIAN_POINT('Ctrl Pts',(-12.8127937909631,18.6621014624746,
12.));
#241659=CARTESIAN_POINT('Ctrl Pts',(-12.8164676687362,18.6686182952799,
0.));
#241660=CARTESIAN_POINT('Ctrl Pts',(-12.8164676687362,18.6686182952799,
12.));
#241661=CARTESIAN_POINT('Ctrl Pts',(-12.8202436318474,18.6753751301092,
0.));
#241662=CARTESIAN_POINT('Ctrl Pts',(-12.8202436318474,18.6753751301092,
12.));
#241663=CARTESIAN_POINT('Ctrl Pts',(-12.8241176980017,18.6823683094139,
0.));
#241664=CARTESIAN_POINT('Ctrl Pts',(-12.8241176980017,18.6823683094139,
12.));
#241665=CARTESIAN_POINT('Ctrl Pts',(-12.8280860635231,18.6895943376171,
0.));
#241666=CARTESIAN_POINT('Ctrl Pts',(-12.8280860635231,18.6895943376171,
12.));
#241667=CARTESIAN_POINT('Ctrl Pts',(-12.8321450599789,18.6970498410172,
0.));
#241668=CARTESIAN_POINT('Ctrl Pts',(-12.8321450599789,18.6970498410172,
12.));
#241669=CARTESIAN_POINT('Ctrl Pts',(-12.8362911280361,18.7047315436294,
0.));
#241670=CARTESIAN_POINT('Ctrl Pts',(-12.8362911280361,18.7047315436294,
12.));
#241671=CARTESIAN_POINT('Ctrl Pts',(-12.8405208263431,18.7126362754445,
0.));
#241672=CARTESIAN_POINT('Ctrl Pts',(-12.8405208263431,18.7126362754445,
12.));
#241673=CARTESIAN_POINT('Ctrl Pts',(-12.8448308329494,18.7207609737702,
0.));
#241674=CARTESIAN_POINT('Ctrl Pts',(-12.8448308329494,18.7207609737702,
12.));
#241675=CARTESIAN_POINT('Ctrl Pts',(-12.8492179511591,18.7291026886554,
0.));
#241676=CARTESIAN_POINT('Ctrl Pts',(-12.8492179511591,18.7291026886554,
12.));
#241677=CARTESIAN_POINT('Ctrl Pts',(-12.8536791086316,18.7376585820854,
0.));
#241678=CARTESIAN_POINT('Ctrl Pts',(-12.8536791086316,18.7376585820854,
12.));
#241679=CARTESIAN_POINT('Ctrl Pts',(-12.8582113455646,18.7464259171251,
0.));
#241680=CARTESIAN_POINT('Ctrl Pts',(-12.8582113455646,18.7464259171251,
12.));
#241681=CARTESIAN_POINT('Ctrl Pts',(-12.8628118054171,18.7554020493887,
0.));
#241682=CARTESIAN_POINT('Ctrl Pts',(-12.8628118054171,18.7554020493887,
12.));
#241683=CARTESIAN_POINT('Ctrl Pts',(-12.8674777239653,18.7645844169564,
0.));
#241684=CARTESIAN_POINT('Ctrl Pts',(-12.8674777239653,18.7645844169564,
12.));
#241685=CARTESIAN_POINT('Ctrl Pts',(-12.872206421181,18.7739705329022,0.));
#241686=CARTESIAN_POINT('Ctrl Pts',(-12.872206421181,18.7739705329022,12.));
#241687=CARTESIAN_POINT('Ctrl Pts',(-12.8769952998095,18.7835579840477,
0.));
#241688=CARTESIAN_POINT('Ctrl Pts',(-12.8769952998095,18.7835579840477,
12.));
#241689=CARTESIAN_POINT('Ctrl Pts',(-12.8818418427475,18.7933444285868,
0.));
#241690=CARTESIAN_POINT('Ctrl Pts',(-12.8818418427475,18.7933444285868,
12.));
#241691=CARTESIAN_POINT('Ctrl Pts',(-12.8867436109546,18.8033275941943,
0.));
#241692=CARTESIAN_POINT('Ctrl Pts',(-12.8867436109546,18.8033275941943,
12.));
#241693=CARTESIAN_POINT('Ctrl Pts',(-12.8916982409935,18.813505275782,0.));
#241694=CARTESIAN_POINT('Ctrl Pts',(-12.8916982409935,18.813505275782,12.));
#241695=CARTESIAN_POINT('Ctrl Pts',(-12.8967034410755,18.8238753319128,
0.));
#241696=CARTESIAN_POINT('Ctrl Pts',(-12.8967034410755,18.8238753319128,
12.));
#241697=CARTESIAN_POINT('Ctrl Pts',(-12.9017569871738,18.834435681259,0.));
#241698=CARTESIAN_POINT('Ctrl Pts',(-12.9017569871738,18.834435681259,12.));
#241699=CARTESIAN_POINT('Ctrl Pts',(-12.9068567191854,18.8451842990984,
0.));
#241700=CARTESIAN_POINT('Ctrl Pts',(-12.9068567191854,18.8451842990984,
12.));
#241701=CARTESIAN_POINT('Ctrl Pts',(-12.9120005369063,18.8561192136198,
0.));
#241702=CARTESIAN_POINT('Ctrl Pts',(-12.9120005369063,18.8561192136198,
12.));
#241703=CARTESIAN_POINT('Ctrl Pts',(-12.9171863977045,18.8672385038326,
0.));
#241704=CARTESIAN_POINT('Ctrl Pts',(-12.9171863977045,18.8672385038326,
12.));
#241705=CARTESIAN_POINT('Ctrl Pts',(-12.9224123144982,18.8785402977527,
0.));
#241706=CARTESIAN_POINT('Ctrl Pts',(-12.9224123144982,18.8785402977527,
12.));
#241707=CARTESIAN_POINT('Ctrl Pts',(-12.9276763536373,18.8900227704889,
0.));
#241708=CARTESIAN_POINT('Ctrl Pts',(-12.9276763536373,18.8900227704889,
12.));
#241709=CARTESIAN_POINT('Ctrl Pts',(-12.9329766328185,18.9016841423403,
0.));
#241710=CARTESIAN_POINT('Ctrl Pts',(-12.9329766328185,18.9016841423403,
12.));
#241711=CARTESIAN_POINT('Ctrl Pts',(-12.9383113190375,18.9135226769465,
0.));
#241712=CARTESIAN_POINT('Ctrl Pts',(-12.9383113190375,18.9135226769465,
12.));
#241713=CARTESIAN_POINT('Ctrl Pts',(-12.9436786266105,18.9255366795195,
0.));
#241714=CARTESIAN_POINT('Ctrl Pts',(-12.9436786266105,18.9255366795195,
12.));
#241715=CARTESIAN_POINT('Ctrl Pts',(-12.9490768151821,18.9377244950435,
0.));
#241716=CARTESIAN_POINT('Ctrl Pts',(-12.9490768151821,18.9377244950435,
12.));
#241717=CARTESIAN_POINT('Ctrl Pts',(-12.9545041877377,18.9500845064715,
0.));
#241718=CARTESIAN_POINT('Ctrl Pts',(-12.9545041877377,18.9500845064715,
12.));
#241719=CARTESIAN_POINT('Ctrl Pts',(-12.9599590886319,18.9626151329229,
0.));
#241720=CARTESIAN_POINT('Ctrl Pts',(-12.9599590886319,18.9626151329229,
12.));
#241721=CARTESIAN_POINT('Ctrl Pts',(-12.9654399021869,18.9753148284475,
0.));
#241722=CARTESIAN_POINT('Ctrl Pts',(-12.9654399021869,18.9753148284475,
12.));
#241723=CARTESIAN_POINT('Ctrl Pts',(-12.9709450512747,18.9881820807585,
0.));
#241724=CARTESIAN_POINT('Ctrl Pts',(-12.9709450512747,18.9881820807585,
12.));
#241725=CARTESIAN_POINT('Ctrl Pts',(-12.9764729959205,19.0012154099791,
0.));
#241726=CARTESIAN_POINT('Ctrl Pts',(-12.9764729959205,19.0012154099791,
12.));
#241727=CARTESIAN_POINT('Ctrl Pts',(-12.9820222318716,19.0144133673348,
0.));
#241728=CARTESIAN_POINT('Ctrl Pts',(-12.9820222318716,19.0144133673348,
12.));
#241729=CARTESIAN_POINT('Ctrl Pts',(-12.9875912893003,19.0277745339908,
0.));
#241730=CARTESIAN_POINT('Ctrl Pts',(-12.9875912893003,19.0277745339908,
12.));
#241731=CARTESIAN_POINT('Ctrl Pts',(-12.9931787316515,19.0412975200398,
0.));
#241732=CARTESIAN_POINT('Ctrl Pts',(-12.9931787316515,19.0412975200398,
12.));
#241733=CARTESIAN_POINT('Ctrl Pts',(-12.9987831544502,19.0549809634355,
0.));
#241734=CARTESIAN_POINT('Ctrl Pts',(-12.9987831544502,19.0549809634355,
12.));
#241735=CARTESIAN_POINT('Ctrl Pts',(-13.0044031841381,19.0688235289437,
0.));
#241736=CARTESIAN_POINT('Ctrl Pts',(-13.0044031841381,19.0688235289437,
12.));
#241737=CARTESIAN_POINT('Ctrl Pts',(-13.0100374768785,19.0828239070482,
0.));
#241738=CARTESIAN_POINT('Ctrl Pts',(-13.0100374768785,19.0828239070482,
12.));
#241739=CARTESIAN_POINT('Ctrl Pts',(-13.0156847176093,19.0969808131225,
0.));
#241740=CARTESIAN_POINT('Ctrl Pts',(-13.0156847176093,19.0969808131225,
12.));
#241741=CARTESIAN_POINT('Ctrl Pts',(-13.0213436191326,19.1112929866308,
0.));
#241742=CARTESIAN_POINT('Ctrl Pts',(-13.0213436191326,19.1112929866308,
12.));
#241743=CARTESIAN_POINT('Ctrl Pts',(-13.0270129211976,19.1257591903099,
0.));
#241744=CARTESIAN_POINT('Ctrl Pts',(-13.0270129211976,19.1257591903099,
12.));
#241745=CARTESIAN_POINT('Ctrl Pts',(-13.0326913895841,19.1403782093389,
0.));
#241746=CARTESIAN_POINT('Ctrl Pts',(-13.0326913895841,19.1403782093389,
12.));
#241747=CARTESIAN_POINT('Ctrl Pts',(-13.0383778152072,19.1551488505233,
0.));
#241748=CARTESIAN_POINT('Ctrl Pts',(-13.0383778152072,19.1551488505233,
12.));
#241749=CARTESIAN_POINT('Ctrl Pts',(-13.0440710133775,19.1700699416625,
0.));
#241750=CARTESIAN_POINT('Ctrl Pts',(-13.0440710133775,19.1700699416625,
12.));
#241751=CARTESIAN_POINT('Ctrl Pts',(-13.0497698230442,19.1851403308825,
0.));
#241752=CARTESIAN_POINT('Ctrl Pts',(-13.0497698230442,19.1851403308825,
12.));
#241753=CARTESIAN_POINT('Ctrl Pts',(-13.0554731060537,19.2003588859771,
0.));
#241754=CARTESIAN_POINT('Ctrl Pts',(-13.0554731060537,19.2003588859771,
12.));
#241755=CARTESIAN_POINT('Ctrl Pts',(-13.0611797463913,19.2157244937141,
0.));
#241756=CARTESIAN_POINT('Ctrl Pts',(-13.0611797463913,19.2157244937141,
12.));
#241757=CARTESIAN_POINT('Ctrl Pts',(-13.0668886494791,19.2312360592031,
0.));
#241758=CARTESIAN_POINT('Ctrl Pts',(-13.0668886494791,19.2312360592031,
12.));
#241759=CARTESIAN_POINT('Ctrl Pts',(-13.0725987415856,19.2468925053988,
0.));
#241760=CARTESIAN_POINT('Ctrl Pts',(-13.0725987415856,19.2468925053988,
12.));
#241761=CARTESIAN_POINT('Ctrl Pts',(-13.0783089692118,19.2626927725596,
0.));
#241762=CARTESIAN_POINT('Ctrl Pts',(-13.0783089692118,19.2626927725596,
12.));
#241763=CARTESIAN_POINT('Ctrl Pts',(-13.0840182984949,19.2786358177198,
0.));
#241764=CARTESIAN_POINT('Ctrl Pts',(-13.0840182984949,19.2786358177198,
12.));
#241765=CARTESIAN_POINT('Ctrl Pts',(-13.089725714597,19.2947206141246,0.));
#241766=CARTESIAN_POINT('Ctrl Pts',(-13.089725714597,19.2947206141246,12.));
#241767=CARTESIAN_POINT('Ctrl Pts',(-13.095430221148,19.3109461507358,0.));
#241768=CARTESIAN_POINT('Ctrl Pts',(-13.095430221148,19.3109461507358,12.));
#241769=CARTESIAN_POINT('Ctrl Pts',(-13.1011308397592,19.3273114318268,
0.));
#241770=CARTESIAN_POINT('Ctrl Pts',(-13.1011308397592,19.3273114318268,
12.));
#241771=CARTESIAN_POINT('Ctrl Pts',(-13.1068266095186,19.3438154765395,
0.));
#241772=CARTESIAN_POINT('Ctrl Pts',(-13.1068266095186,19.3438154765395,
12.));
#241773=CARTESIAN_POINT('Ctrl Pts',(-13.1125165865021,19.3604573184516,
0.));
#241774=CARTESIAN_POINT('Ctrl Pts',(-13.1125165865021,19.3604573184516,
12.));
#241775=CARTESIAN_POINT('Ctrl Pts',(-13.118199843271,19.3772360051093,0.));
#241776=CARTESIAN_POINT('Ctrl Pts',(-13.118199843271,19.3772360051093,12.));
#241777=CARTESIAN_POINT('Ctrl Pts',(-13.1238754684177,19.3941505976267,
0.));
#241778=CARTESIAN_POINT('Ctrl Pts',(-13.1238754684177,19.3941505976267,
12.));
#241779=CARTESIAN_POINT('Ctrl Pts',(-13.1295425661635,19.4112001703561,
0.));
#241780=CARTESIAN_POINT('Ctrl Pts',(-13.1295425661635,19.4112001703561,
12.));
#241781=CARTESIAN_POINT('Ctrl Pts',(-13.1352002559439,19.4283838105265,
0.));
#241782=CARTESIAN_POINT('Ctrl Pts',(-13.1352002559439,19.4283838105265,
12.));
#241783=CARTESIAN_POINT('Ctrl Pts',(-13.140847672006,19.4457006178875,0.));
#241784=CARTESIAN_POINT('Ctrl Pts',(-13.140847672006,19.4457006178875,12.));
#241785=CARTESIAN_POINT('Ctrl Pts',(-13.1464839629966,19.463149704325,0.));
#241786=CARTESIAN_POINT('Ctrl Pts',(-13.1464839629966,19.463149704325,12.));
#241787=CARTESIAN_POINT('Ctrl Pts',(-13.1521082915846,19.4807301935256,
0.));
#241788=CARTESIAN_POINT('Ctrl Pts',(-13.1521082915846,19.4807301935256,
12.));
#241789=CARTESIAN_POINT('Ctrl Pts',(-13.1577198341238,19.498441220707,0.));
#241790=CARTESIAN_POINT('Ctrl Pts',(-13.1577198341238,19.498441220707,12.));
#241791=CARTESIAN_POINT('Ctrl Pts',(-13.1633177803097,19.5162819323207,
0.));
#241792=CARTESIAN_POINT('Ctrl Pts',(-13.1633177803097,19.5162819323207,
12.));
#241793=CARTESIAN_POINT('Ctrl Pts',(-13.1689013328432,19.5342514857564,
0.));
#241794=CARTESIAN_POINT('Ctrl Pts',(-13.1689013328432,19.5342514857564,
12.));
#241795=CARTESIAN_POINT('Ctrl Pts',(-13.1744697070918,19.5523490490254,
0.));
#241796=CARTESIAN_POINT('Ctrl Pts',(-13.1744697070918,19.5523490490254,
12.));
#241797=CARTESIAN_POINT('Ctrl Pts',(-13.1800221307683,19.5705738004682,
0.));
#241798=CARTESIAN_POINT('Ctrl Pts',(-13.1800221307683,19.5705738004682,
12.));
#241799=CARTESIAN_POINT('Ctrl Pts',(-13.1855578436479,19.5889249285351,
0.));
#241800=CARTESIAN_POINT('Ctrl Pts',(-13.1855578436479,19.5889249285351,
12.));
#241801=CARTESIAN_POINT('Ctrl Pts',(-13.1910760972818,19.6074016315421,
0.));
#241802=CARTESIAN_POINT('Ctrl Pts',(-13.1910760972818,19.6074016315421,
12.));
#241803=CARTESIAN_POINT('Ctrl Pts',(-13.196576154715,19.6260031174244,0.));
#241804=CARTESIAN_POINT('Ctrl Pts',(-13.196576154715,19.6260031174244,12.));
#241805=CARTESIAN_POINT('Ctrl Pts',(-13.202057290206,19.6447286034764,0.));
#241806=CARTESIAN_POINT('Ctrl Pts',(-13.202057290206,19.6447286034764,12.));
#241807=CARTESIAN_POINT('Ctrl Pts',(-13.2075187889522,19.6635773160924,
0.));
#241808=CARTESIAN_POINT('Ctrl Pts',(-13.2075187889522,19.6635773160924,
12.));
#241809=CARTESIAN_POINT('Ctrl Pts',(-13.2129599468478,19.6825484905812,
0.));
#241810=CARTESIAN_POINT('Ctrl Pts',(-13.2129599468478,19.6825484905812,
12.));
#241811=CARTESIAN_POINT('Ctrl Pts',(-13.2183800702431,19.7016413709678,
0.));
#241812=CARTESIAN_POINT('Ctrl Pts',(-13.2183800702431,19.7016413709678,
12.));
#241813=CARTESIAN_POINT('Ctrl Pts',(-13.2237784757065,19.7208552097867,
0.));
#241814=CARTESIAN_POINT('Ctrl Pts',(-13.2237784757065,19.7208552097867,
12.));
#241815=CARTESIAN_POINT('Ctrl Pts',(-13.2291544897902,19.7401892678701,
0.));
#241816=CARTESIAN_POINT('Ctrl Pts',(-13.2291544897902,19.7401892678701,
12.));
#241817=CARTESIAN_POINT('Ctrl Pts',(-13.2345074487968,19.7596428141176,
0.));
#241818=CARTESIAN_POINT('Ctrl Pts',(-13.2345074487968,19.7596428141176,
12.));
#241819=CARTESIAN_POINT('Ctrl Pts',(-13.239836698568,19.7792151253297,0.));
#241820=CARTESIAN_POINT('Ctrl Pts',(-13.239836698568,19.7792151253297,12.));
#241821=CARTESIAN_POINT('Ctrl Pts',(-13.2451415942809,19.7989054860501,
0.));
#241822=CARTESIAN_POINT('Ctrl Pts',(-13.2451415942809,19.7989054860501,
12.));
#241823=CARTESIAN_POINT('Ctrl Pts',(-13.2504215002458,19.8187131883919,
0.));
#241824=CARTESIAN_POINT('Ctrl Pts',(-13.2504215002458,19.8187131883919,
12.));
#241825=CARTESIAN_POINT('Ctrl Pts',(-13.2556757897085,19.8386375318632,
0.));
#241826=CARTESIAN_POINT('Ctrl Pts',(-13.2556757897085,19.8386375318632,
12.));
#241827=CARTESIAN_POINT('Ctrl Pts',(-13.2609038446525,19.8586778231711,
0.));
#241828=CARTESIAN_POINT('Ctrl Pts',(-13.2609038446525,19.8586778231711,
12.));
#241829=CARTESIAN_POINT('Ctrl Pts',(-13.2661050556128,19.8788333760571,
0.));
#241830=CARTESIAN_POINT('Ctrl Pts',(-13.2661050556128,19.8788333760571,
12.));
#241831=CARTESIAN_POINT('Ctrl Pts',(-13.2712788215015,19.8991035111739,
0.));
#241832=CARTESIAN_POINT('Ctrl Pts',(-13.2712788215015,19.8991035111739,
12.));
#241833=CARTESIAN_POINT('Ctrl Pts',(-13.2764245494354,19.9194875559419,
0.));
#241834=CARTESIAN_POINT('Ctrl Pts',(-13.2764245494354,19.9194875559419,
12.));
#241835=CARTESIAN_POINT('Ctrl Pts',(-13.2815416545663,19.9399848444019,
0.));
#241836=CARTESIAN_POINT('Ctrl Pts',(-13.2815416545663,19.9399848444019,
12.));
#241837=CARTESIAN_POINT('Ctrl Pts',(-13.2866295599152,19.9605947170589,
0.));
#241838=CARTESIAN_POINT('Ctrl Pts',(-13.2866295599152,19.9605947170589,
12.));
#241839=CARTESIAN_POINT('Ctrl Pts',(-13.2916876962098,19.9813165207174,
0.));
#241840=CARTESIAN_POINT('Ctrl Pts',(-13.2916876962098,19.9813165207174,
12.));
#241841=CARTESIAN_POINT('Ctrl Pts',(-13.296715501731,20.0021496083742,0.));
#241842=CARTESIAN_POINT('Ctrl Pts',(-13.296715501731,20.0021496083742,12.));
#241843=CARTESIAN_POINT('Ctrl Pts',(-13.3017124221639,20.0230933391039,
0.));
#241844=CARTESIAN_POINT('Ctrl Pts',(-13.3017124221639,20.0230933391039,
12.));
#241845=CARTESIAN_POINT('Ctrl Pts',(-13.3066779104515,20.0441470779345,
0.));
#241846=CARTESIAN_POINT('Ctrl Pts',(-13.3066779104515,20.0441470779345,
12.));
#241847=CARTESIAN_POINT('Ctrl Pts',(-13.3116114266514,20.0653101957188,
0.));
#241848=CARTESIAN_POINT('Ctrl Pts',(-13.3116114266514,20.0653101957188,
12.));
#241849=CARTESIAN_POINT('Ctrl Pts',(-13.3165124377963,20.0865820689883,
0.));
#241850=CARTESIAN_POINT('Ctrl Pts',(-13.3165124377963,20.0865820689883,
12.));
#241851=CARTESIAN_POINT('Ctrl Pts',(-13.3213804177588,20.1079620798377,
0.));
#241852=CARTESIAN_POINT('Ctrl Pts',(-13.3213804177588,20.1079620798377,
12.));
#241853=CARTESIAN_POINT('Ctrl Pts',(-13.3262148471228,20.1294496158405,
0.));
#241854=CARTESIAN_POINT('Ctrl Pts',(-13.3262148471228,20.1294496158405,
12.));
#241855=CARTESIAN_POINT('Ctrl Pts',(-13.3310152130565,20.1510440699477,
0.));
#241856=CARTESIAN_POINT('Ctrl Pts',(-13.3310152130565,20.1510440699477,
12.));
#241857=CARTESIAN_POINT('Ctrl Pts',(-13.3357810091903,20.1727448403818,
0.));
#241858=CARTESIAN_POINT('Ctrl Pts',(-13.3357810091903,20.1727448403818,
12.));
#241859=CARTESIAN_POINT('Ctrl Pts',(-13.3405117354969,20.1945513305233,
0.));
#241860=CARTESIAN_POINT('Ctrl Pts',(-13.3405117354969,20.1945513305233,
12.));
#241861=CARTESIAN_POINT('Ctrl Pts',(-13.3452068981763,20.2164629487855,
0.));
#241862=CARTESIAN_POINT('Ctrl Pts',(-13.3452068981763,20.2164629487855,
12.));
#241863=CARTESIAN_POINT('Ctrl Pts',(-13.3498660095382,20.2384791085354,
0.));
#241864=CARTESIAN_POINT('Ctrl Pts',(-13.3498660095382,20.2384791085354,
12.));
#241865=CARTESIAN_POINT('Ctrl Pts',(-13.3544885878886,20.2605992280117,
0.));
#241866=CARTESIAN_POINT('Ctrl Pts',(-13.3544885878886,20.2605992280117,
12.));
#241867=CARTESIAN_POINT('Ctrl Pts',(-13.3590741574194,20.2828227302337,
0.));
#241868=CARTESIAN_POINT('Ctrl Pts',(-13.3590741574194,20.2828227302337,
12.));
#241869=CARTESIAN_POINT('Ctrl Pts',(-13.3636222481017,20.3051490429049,
0.));
#241870=CARTESIAN_POINT('Ctrl Pts',(-13.3636222481017,20.3051490429049,
12.));
#241871=CARTESIAN_POINT('Ctrl Pts',(-13.3681323955828,20.3275775983032,
0.));
#241872=CARTESIAN_POINT('Ctrl Pts',(-13.3681323955828,20.3275775983032,
12.));
#241873=CARTESIAN_POINT('Ctrl Pts',(-13.3726041410869,20.3501078331818,
0.));
#241874=CARTESIAN_POINT('Ctrl Pts',(-13.3726041410869,20.3501078331818,
12.));
#241875=CARTESIAN_POINT('Ctrl Pts',(-13.377037031319,20.3727391887187,0.));
#241876=CARTESIAN_POINT('Ctrl Pts',(-13.377037031319,20.3727391887187,12.));
#241877=CARTESIAN_POINT('Ctrl Pts',(-13.3814306183721,20.3954711104504,
0.));
#241878=CARTESIAN_POINT('Ctrl Pts',(-13.3814306183721,20.3954711104504,
12.));
#241879=CARTESIAN_POINT('Ctrl Pts',(-13.3857844596387,20.4183030482002,
0.));
#241880=CARTESIAN_POINT('Ctrl Pts',(-13.3857844596387,20.4183030482002,
12.));
#241881=CARTESIAN_POINT('Ctrl Pts',(-13.3900981177254,20.4412344560007,
0.));
#241882=CARTESIAN_POINT('Ctrl Pts',(-13.3900981177254,20.4412344560007,
12.));
#241883=CARTESIAN_POINT('Ctrl Pts',(-13.3943711603739,20.4642647920038,
0.));
#241884=CARTESIAN_POINT('Ctrl Pts',(-13.3943711603739,20.4642647920038,
12.));
#241885=CARTESIAN_POINT('Ctrl Pts',(-13.3986031603716,20.4873935184041,
0.));
#241886=CARTESIAN_POINT('Ctrl Pts',(-13.3986031603716,20.4873935184041,
12.));
#241887=CARTESIAN_POINT('Ctrl Pts',(-13.4027936954529,20.5106201013755,
0.));
#241888=CARTESIAN_POINT('Ctrl Pts',(-13.4027936954529,20.5106201013755,
12.));
#241889=CARTESIAN_POINT('Ctrl Pts',(-13.4069423482076,20.5339440109957,
0.));
#241890=CARTESIAN_POINT('Ctrl Pts',(-13.4069423482076,20.5339440109957,
12.));
#241891=CARTESIAN_POINT('Ctrl Pts',(-13.4110487059912,20.557364721164,0.));
#241892=CARTESIAN_POINT('Ctrl Pts',(-13.4110487059912,20.557364721164,12.));
#241893=CARTESIAN_POINT('Ctrl Pts',(-13.4151123608411,20.5808817095155,
0.));
#241894=CARTESIAN_POINT('Ctrl Pts',(-13.4151123608411,20.5808817095155,
12.));
#241895=CARTESIAN_POINT('Ctrl Pts',(-13.4191329093932,20.6044944573151,
0.));
#241896=CARTESIAN_POINT('Ctrl Pts',(-13.4191329093932,20.6044944573151,
12.));
#241897=CARTESIAN_POINT('Ctrl Pts',(-13.4231099528178,20.6282024494234,
0.));
#241898=CARTESIAN_POINT('Ctrl Pts',(-13.4231099528178,20.6282024494234,
12.));
#241899=CARTESIAN_POINT('Ctrl Pts',(-13.427043096765,20.6520051742867,0.));
#241900=CARTESIAN_POINT('Ctrl Pts',(-13.427043096765,20.6520051742867,12.));
#241901=CARTESIAN_POINT('Ctrl Pts',(-13.4309319513119,20.6759021239102,
0.));
#241902=CARTESIAN_POINT('Ctrl Pts',(-13.4309319513119,20.6759021239102,
12.));
#241903=CARTESIAN_POINT('Ctrl Pts',(-13.4347761309154,20.6998927938288,
0.));
#241904=CARTESIAN_POINT('Ctrl Pts',(-13.4347761309154,20.6998927938288,
12.));
#241905=CARTESIAN_POINT('Ctrl Pts',(-13.4385752543663,20.7239766830675,
0.));
#241906=CARTESIAN_POINT('Ctrl Pts',(-13.4385752543663,20.7239766830675,
12.));
#241907=CARTESIAN_POINT('Ctrl Pts',(-13.4423289447561,20.7481532941014,
0.));
#241908=CARTESIAN_POINT('Ctrl Pts',(-13.4423289447561,20.7481532941014,
12.));
#241909=CARTESIAN_POINT('Ctrl Pts',(-13.4460368293689,20.7724221327609,
0.));
#241910=CARTESIAN_POINT('Ctrl Pts',(-13.4460368293689,20.7724221327609,
12.));
#241911=CARTESIAN_POINT('Ctrl Pts',(-13.4496985395637,20.7967827081228,
0.));
#241912=CARTESIAN_POINT('Ctrl Pts',(-13.4496985395637,20.7967827081228,
12.));
#241913=CARTESIAN_POINT('Ctrl Pts',(-13.4533137106667,20.821234532398,0.));
#241914=CARTESIAN_POINT('Ctrl Pts',(-13.4533137106667,20.821234532398,12.));
#241915=CARTESIAN_POINT('Ctrl Pts',(-13.4568819818631,20.8457771208083,
0.));
#241916=CARTESIAN_POINT('Ctrl Pts',(-13.4568819818631,20.8457771208083,
12.));
#241917=CARTESIAN_POINT('Ctrl Pts',(-13.4604029960983,20.8704099914641,
0.));
#241918=CARTESIAN_POINT('Ctrl Pts',(-13.4604029960983,20.8704099914641,
12.));
#241919=CARTESIAN_POINT('Ctrl Pts',(-13.4638763999725,20.8951326652158,
0.));
#241920=CARTESIAN_POINT('Ctrl Pts',(-13.4638763999725,20.8951326652158,
12.));
#241921=CARTESIAN_POINT('Ctrl Pts',(-13.4673018437717,20.9199446657583,
0.));
#241922=CARTESIAN_POINT('Ctrl Pts',(-13.4673018437717,20.9199446657583,
12.));
#241923=CARTESIAN_POINT('Ctrl Pts',(-13.4706789815166,20.9448455197557,
0.));
#241924=CARTESIAN_POINT('Ctrl Pts',(-13.4706789815166,20.9448455197557,
12.));
#241925=CARTESIAN_POINT('Ctrl Pts',(-13.4740074710086,20.9698347569476,
0.));
#241926=CARTESIAN_POINT('Ctrl Pts',(-13.4740074710086,20.9698347569476,
12.));
#241927=CARTESIAN_POINT('Ctrl Pts',(-13.4772869738879,20.9949119102592,
0.));
#241928=CARTESIAN_POINT('Ctrl Pts',(-13.4772869738879,20.9949119102592,
12.));
#241929=CARTESIAN_POINT('Ctrl Pts',(-13.4805171556822,21.0200765158884,
0.));
#241930=CARTESIAN_POINT('Ctrl Pts',(-13.4805171556822,21.0200765158884,
12.));
#241931=CARTESIAN_POINT('Ctrl Pts',(-13.4836976858912,21.0453281134245,
0.));
#241932=CARTESIAN_POINT('Ctrl Pts',(-13.4836976858912,21.0453281134245,
12.));
#241933=CARTESIAN_POINT('Ctrl Pts',(-13.4868282377191,21.0706662455199,
0.));
#241934=CARTESIAN_POINT('Ctrl Pts',(-13.4868282377191,21.0706662455199,
12.));
#241935=CARTESIAN_POINT('Ctrl Pts',(-13.4899084877717,21.0960904575046,
0.));
#241936=CARTESIAN_POINT('Ctrl Pts',(-13.4899084877717,21.0960904575046,
12.));
#241937=CARTESIAN_POINT('Ctrl Pts',(-13.4929381157778,21.1216002970207,
0.));
#241938=CARTESIAN_POINT('Ctrl Pts',(-13.4929381157778,21.1216002970207,
12.));
#241939=CARTESIAN_POINT('Ctrl Pts',(-13.4959168042934,21.1471953136209,
0.));
#241940=CARTESIAN_POINT('Ctrl Pts',(-13.4959168042934,21.1471953136209,
12.));
#241941=CARTESIAN_POINT('Ctrl Pts',(-13.4988442384491,21.1728750584175,
0.));
#241942=CARTESIAN_POINT('Ctrl Pts',(-13.4988442384491,21.1728750584175,
12.));
#241943=CARTESIAN_POINT('Ctrl Pts',(-13.5017201056088,21.1986390835828,
0.));
#241944=CARTESIAN_POINT('Ctrl Pts',(-13.5017201056088,21.1986390835828,
12.));
#241945=CARTESIAN_POINT('Ctrl Pts',(-13.5045440957404,21.2244869429332,
0.));
#241946=CARTESIAN_POINT('Ctrl Pts',(-13.5045440957404,21.2244869429332,
12.));
#241947=CARTESIAN_POINT('Ctrl Pts',(-13.5073159019452,21.250418192743,0.));
#241948=CARTESIAN_POINT('Ctrl Pts',(-13.5073159019452,21.250418192743,12.));
#241949=CARTESIAN_POINT('Ctrl Pts',(-13.5100352209205,21.2764323924442,
0.));
#241950=CARTESIAN_POINT('Ctrl Pts',(-13.5100352209205,21.2764323924442,
12.));
#241951=CARTESIAN_POINT('Ctrl Pts',(-13.5127017534971,21.3025291054235,
0.));
#241952=CARTESIAN_POINT('Ctrl Pts',(-13.5127017534971,21.3025291054235,
12.));
#241953=CARTESIAN_POINT('Ctrl Pts',(-13.5153152050555,21.328707899634,0.));
#241954=CARTESIAN_POINT('Ctrl Pts',(-13.5153152050555,21.328707899634,12.));
#241955=CARTESIAN_POINT('Ctrl Pts',(-13.5178752862466,21.3549683486222,
0.));
#241956=CARTESIAN_POINT('Ctrl Pts',(-13.5178752862466,21.3549683486222,
12.));
#241957=CARTESIAN_POINT('Ctrl Pts',(-13.5203817122504,21.3813100304973,
0.));
#241958=CARTESIAN_POINT('Ctrl Pts',(-13.5203817122504,21.3813100304973,
12.));
#241959=CARTESIAN_POINT('Ctrl Pts',(-13.5228342013516,21.4077325259324,
0.));
#241960=CARTESIAN_POINT('Ctrl Pts',(-13.5228342013516,21.4077325259324,
12.));
#241961=CARTESIAN_POINT('Ctrl Pts',(-13.5252324737802,21.4342354165259,
0.));
#241962=CARTESIAN_POINT('Ctrl Pts',(-13.5252324737802,21.4342354165259,
12.));
#241963=CARTESIAN_POINT('Ctrl Pts',(-13.5275762503555,21.4608182828697,
0.));
#241964=CARTESIAN_POINT('Ctrl Pts',(-13.5275762503555,21.4608182828697,
12.));
#241965=CARTESIAN_POINT('Ctrl Pts',(-13.5298652514355,21.4874807030468,
0.));
#241966=CARTESIAN_POINT('Ctrl Pts',(-13.5298652514355,21.4874807030468,
12.));
#241967=CARTESIAN_POINT('Ctrl Pts',(-13.5320991952138,21.5142222501666,
0.));
#241968=CARTESIAN_POINT('Ctrl Pts',(-13.5320991952138,21.5142222501666,
12.));
#241969=CARTESIAN_POINT('Ctrl Pts',(-13.5342777983215,21.5410424932503,
0.));
#241970=CARTESIAN_POINT('Ctrl Pts',(-13.5342777983215,21.5410424932503,
12.));
#241971=CARTESIAN_POINT('Ctrl Pts',(-13.536400779028,21.5679410019001,0.));
#241972=CARTESIAN_POINT('Ctrl Pts',(-13.536400779028,21.5679410019001,12.));
#241973=CARTESIAN_POINT('Ctrl Pts',(-13.5384678597195,21.5949173499013,
0.));
#241974=CARTESIAN_POINT('Ctrl Pts',(-13.5384678597195,21.5949173499013,
12.));
#241975=CARTESIAN_POINT('Ctrl Pts',(-13.5404787697792,21.6219711193946,
0.));
#241976=CARTESIAN_POINT('Ctrl Pts',(-13.5404787697792,21.6219711193946,
12.));
#241977=CARTESIAN_POINT('Ctrl Pts',(-13.5424332480699,21.6491019044648,
0.));
#241978=CARTESIAN_POINT('Ctrl Pts',(-13.5424332480699,21.6491019044648,
12.));
#241979=CARTESIAN_POINT('Ctrl Pts',(-13.5443310461526,21.6763093157699,
0.));
#241980=CARTESIAN_POINT('Ctrl Pts',(-13.5443310461526,21.6763093157699,
12.));
#241981=CARTESIAN_POINT('Ctrl Pts',(-13.5461719295048,21.7035929822955,
0.));
#241982=CARTESIAN_POINT('Ctrl Pts',(-13.5461719295048,21.7035929822955,
12.));
#241983=CARTESIAN_POINT('Ctrl Pts',(-13.5479556704481,21.7309525412281,
0.));
#241984=CARTESIAN_POINT('Ctrl Pts',(-13.5479556704481,21.7309525412281,
12.));
#241985=CARTESIAN_POINT('Ctrl Pts',(-13.5496820422211,21.7583876294554,
0.));
#241986=CARTESIAN_POINT('Ctrl Pts',(-13.5496820422211,21.7583876294554,
12.));
#241987=CARTESIAN_POINT('Ctrl Pts',(-13.551350812725,21.7858978745865,0.));
#241988=CARTESIAN_POINT('Ctrl Pts',(-13.551350812725,21.7858978745865,12.));
#241989=CARTESIAN_POINT('Ctrl Pts',(-13.5529617381573,21.8134828857967,
0.));
#241990=CARTESIAN_POINT('Ctrl Pts',(-13.5529617381573,21.8134828857967,
12.));
#241991=CARTESIAN_POINT('Ctrl Pts',(-13.5545145573031,21.8411422456075,
0.));
#241992=CARTESIAN_POINT('Ctrl Pts',(-13.5545145573031,21.8411422456075,
12.));
#241993=CARTESIAN_POINT('Ctrl Pts',(-13.5560089839385,21.8688754989365,
0.));
#241994=CARTESIAN_POINT('Ctrl Pts',(-13.5560089839385,21.8688754989365,
12.));
#241995=CARTESIAN_POINT('Ctrl Pts',(-13.5574447178424,21.8966821688824,
0.));
#241996=CARTESIAN_POINT('Ctrl Pts',(-13.5574447178424,21.8966821688824,
12.));
#241997=CARTESIAN_POINT('Ctrl Pts',(-13.5588214586604,21.9245617765769,
0.));
#241998=CARTESIAN_POINT('Ctrl Pts',(-13.5588214586604,21.9245617765769,
12.));
#241999=CARTESIAN_POINT('Ctrl Pts',(-13.5601389185257,21.9525138592813,
0.));
#242000=CARTESIAN_POINT('Ctrl Pts',(-13.5601389185257,21.9525138592813,
12.));
#242001=CARTESIAN_POINT('Ctrl Pts',(-13.5613968357561,21.9805379899168,
0.));
#242002=CARTESIAN_POINT('Ctrl Pts',(-13.5613968357561,21.9805379899168,
12.));
#242003=CARTESIAN_POINT('Ctrl Pts',(-13.5625949868333,22.0086337943449,
0.));
#242004=CARTESIAN_POINT('Ctrl Pts',(-13.5625949868333,22.0086337943449,
12.));
#242005=CARTESIAN_POINT('Ctrl Pts',(-13.5637332022473,22.0368009736295,
0.));
#242006=CARTESIAN_POINT('Ctrl Pts',(-13.5637332022473,22.0368009736295,
12.));
#242007=CARTESIAN_POINT('Ctrl Pts',(-13.5648113689033,22.0650393089609,
0.));
#242008=CARTESIAN_POINT('Ctrl Pts',(-13.5648113689033,22.0650393089609,
12.));
#242009=CARTESIAN_POINT('Ctrl Pts',(-13.5658294169284,22.0933486464593,
0.));
#242010=CARTESIAN_POINT('Ctrl Pts',(-13.5658294169284,22.0933486464593,
12.));
#242011=CARTESIAN_POINT('Ctrl Pts',(-13.5667873105359,22.1217288871975,
0.));
#242012=CARTESIAN_POINT('Ctrl Pts',(-13.5667873105359,22.1217288871975,
12.));
#242013=CARTESIAN_POINT('Ctrl Pts',(-13.5675054919061,22.1444897575194,
0.));
#242014=CARTESIAN_POINT('Ctrl Pts',(-13.5675054919061,22.1444897575194,
12.));
#242015=CARTESIAN_POINT('Ctrl Pts',(-13.5680170531805,22.1615922805008,
0.));
#242016=CARTESIAN_POINT('Ctrl Pts',(-13.5680170531805,22.1615922805008,
12.));
#242017=CARTESIAN_POINT('Ctrl Pts',(-13.5683460612942,22.1730081264608,
0.));
#242018=CARTESIAN_POINT('Ctrl Pts',(-13.5683460612942,22.1730081264608,
12.));
#242019=CARTESIAN_POINT('Ctrl Pts',(-13.5685075571671,22.1787195904339,
0.));
#242020=CARTESIAN_POINT('Ctrl Pts',(-13.5685075571671,22.1787195904339,
12.));
#242021=CARTESIAN_POINT('',(-13.5685075571671,22.1787195904339,0.));
#242022=CARTESIAN_POINT('Ctrl Pts',(-12.7689476255363,18.5896416359912,
0.));
#242023=CARTESIAN_POINT('Ctrl Pts',(-12.7689524524483,18.5896460962964,
0.));
#242024=CARTESIAN_POINT('Ctrl Pts',(-12.768986426692,18.5896919669165,0.));
#242025=CARTESIAN_POINT('Ctrl Pts',(-12.769110348199,18.589871621843,0.));
#242026=CARTESIAN_POINT('Ctrl Pts',(-12.7694215127919,18.5903328777227,
0.));
#242027=CARTESIAN_POINT('Ctrl Pts',(-12.7700520897173,18.5912775137806,
0.));
#242028=CARTESIAN_POINT('Ctrl Pts',(-12.7709195951156,18.5925859134579,
0.));
#242029=CARTESIAN_POINT('Ctrl Pts',(-12.7720142287172,18.5942490615407,
0.));
#242030=CARTESIAN_POINT('Ctrl Pts',(-12.7733231262108,18.5962551167772,
0.));
#242031=CARTESIAN_POINT('Ctrl Pts',(-12.7748328937638,18.598591752595,0.));
#242032=CARTESIAN_POINT('Ctrl Pts',(-12.7765325225081,18.6012488486709,
0.));
#242033=CARTESIAN_POINT('Ctrl Pts',(-12.7784139605066,18.6042190183704,
0.));
#242034=CARTESIAN_POINT('Ctrl Pts',(-12.7804705387658,18.6074961535723,
0.));
#242035=CARTESIAN_POINT('Ctrl Pts',(-12.7826959526925,18.6110744826219,
0.));
#242036=CARTESIAN_POINT('Ctrl Pts',(-12.7850831657901,18.6149475565188,
0.));
#242037=CARTESIAN_POINT('Ctrl Pts',(-12.7876249657834,18.6191087624752,
0.));
#242038=CARTESIAN_POINT('Ctrl Pts',(-12.7903142925234,18.6235516265575,
0.));
#242039=CARTESIAN_POINT('Ctrl Pts',(-12.7931447451555,18.6282702819371,
0.));
#242040=CARTESIAN_POINT('Ctrl Pts',(-12.7961106222251,18.6332595057006,
0.));
#242041=CARTESIAN_POINT('Ctrl Pts',(-12.7992066625264,18.63851447924,0.));
#242042=CARTESIAN_POINT('Ctrl Pts',(-12.8024278770152,18.6440306327456,
0.));
#242043=CARTESIAN_POINT('Ctrl Pts',(-12.805769331162,18.6498034438986,0.));
#242044=CARTESIAN_POINT('Ctrl Pts',(-12.8092261933858,18.6558284825773,
0.));
#242045=CARTESIAN_POINT('Ctrl Pts',(-12.8127937909631,18.6621014624746,
0.));
#242046=CARTESIAN_POINT('Ctrl Pts',(-12.8164676687362,18.6686182952799,
0.));
#242047=CARTESIAN_POINT('Ctrl Pts',(-12.8202436318474,18.6753751301092,
0.));
#242048=CARTESIAN_POINT('Ctrl Pts',(-12.8241176980017,18.6823683094139,
0.));
#242049=CARTESIAN_POINT('Ctrl Pts',(-12.8280860635231,18.6895943376171,
0.));
#242050=CARTESIAN_POINT('Ctrl Pts',(-12.8321450599789,18.6970498410172,
0.));
#242051=CARTESIAN_POINT('Ctrl Pts',(-12.8362911280361,18.7047315436294,
0.));
#242052=CARTESIAN_POINT('Ctrl Pts',(-12.8405208263431,18.7126362754445,
0.));
#242053=CARTESIAN_POINT('Ctrl Pts',(-12.8448308329494,18.7207609737702,
0.));
#242054=CARTESIAN_POINT('Ctrl Pts',(-12.8492179511591,18.7291026886554,
0.));
#242055=CARTESIAN_POINT('Ctrl Pts',(-12.8536791086316,18.7376585820854,
0.));
#242056=CARTESIAN_POINT('Ctrl Pts',(-12.8582113455646,18.7464259171251,
0.));
#242057=CARTESIAN_POINT('Ctrl Pts',(-12.8628118054171,18.7554020493887,
0.));
#242058=CARTESIAN_POINT('Ctrl Pts',(-12.8674777239653,18.7645844169564,
0.));
#242059=CARTESIAN_POINT('Ctrl Pts',(-12.872206421181,18.7739705329022,0.));
#242060=CARTESIAN_POINT('Ctrl Pts',(-12.8769952998095,18.7835579840477,
0.));
#242061=CARTESIAN_POINT('Ctrl Pts',(-12.8818418427475,18.7933444285868,
0.));
#242062=CARTESIAN_POINT('Ctrl Pts',(-12.8867436109546,18.8033275941943,
0.));
#242063=CARTESIAN_POINT('Ctrl Pts',(-12.8916982409935,18.813505275782,0.));
#242064=CARTESIAN_POINT('Ctrl Pts',(-12.8967034410755,18.8238753319128,
0.));
#242065=CARTESIAN_POINT('Ctrl Pts',(-12.9017569871738,18.834435681259,0.));
#242066=CARTESIAN_POINT('Ctrl Pts',(-12.9068567191854,18.8451842990984,
0.));
#242067=CARTESIAN_POINT('Ctrl Pts',(-12.9120005369063,18.8561192136198,
0.));
#242068=CARTESIAN_POINT('Ctrl Pts',(-12.9171863977045,18.8672385038326,
0.));
#242069=CARTESIAN_POINT('Ctrl Pts',(-12.9224123144982,18.8785402977527,
0.));
#242070=CARTESIAN_POINT('Ctrl Pts',(-12.9276763536373,18.8900227704889,
0.));
#242071=CARTESIAN_POINT('Ctrl Pts',(-12.9329766328185,18.9016841423403,
0.));
#242072=CARTESIAN_POINT('Ctrl Pts',(-12.9383113190375,18.9135226769465,
0.));
#242073=CARTESIAN_POINT('Ctrl Pts',(-12.9436786266105,18.9255366795195,
0.));
#242074=CARTESIAN_POINT('Ctrl Pts',(-12.9490768151821,18.9377244950435,
0.));
#242075=CARTESIAN_POINT('Ctrl Pts',(-12.9545041877377,18.9500845064715,
0.));
#242076=CARTESIAN_POINT('Ctrl Pts',(-12.9599590886319,18.9626151329229,
0.));
#242077=CARTESIAN_POINT('Ctrl Pts',(-12.9654399021869,18.9753148284475,
0.));
#242078=CARTESIAN_POINT('Ctrl Pts',(-12.9709450512747,18.9881820807585,
0.));
#242079=CARTESIAN_POINT('Ctrl Pts',(-12.9764729959205,19.0012154099791,
0.));
#242080=CARTESIAN_POINT('Ctrl Pts',(-12.9820222318716,19.0144133673348,
0.));
#242081=CARTESIAN_POINT('Ctrl Pts',(-12.9875912893003,19.0277745339908,
0.));
#242082=CARTESIAN_POINT('Ctrl Pts',(-12.9931787316515,19.0412975200398,
0.));
#242083=CARTESIAN_POINT('Ctrl Pts',(-12.9987831544502,19.0549809634355,
0.));
#242084=CARTESIAN_POINT('Ctrl Pts',(-13.0044031841381,19.0688235289437,
0.));
#242085=CARTESIAN_POINT('Ctrl Pts',(-13.0100374768785,19.0828239070482,
0.));
#242086=CARTESIAN_POINT('Ctrl Pts',(-13.0156847176093,19.0969808131225,
0.));
#242087=CARTESIAN_POINT('Ctrl Pts',(-13.0213436191326,19.1112929866308,
0.));
#242088=CARTESIAN_POINT('Ctrl Pts',(-13.0270129211976,19.1257591903099,
0.));
#242089=CARTESIAN_POINT('Ctrl Pts',(-13.0326913895841,19.1403782093389,
0.));
#242090=CARTESIAN_POINT('Ctrl Pts',(-13.0383778152072,19.1551488505233,
0.));
#242091=CARTESIAN_POINT('Ctrl Pts',(-13.0440710133775,19.1700699416625,
0.));
#242092=CARTESIAN_POINT('Ctrl Pts',(-13.0497698230442,19.1851403308825,
0.));
#242093=CARTESIAN_POINT('Ctrl Pts',(-13.0554731060537,19.2003588859771,
0.));
#242094=CARTESIAN_POINT('Ctrl Pts',(-13.0611797463913,19.2157244937141,
0.));
#242095=CARTESIAN_POINT('Ctrl Pts',(-13.0668886494791,19.2312360592031,
0.));
#242096=CARTESIAN_POINT('Ctrl Pts',(-13.0725987415856,19.2468925053988,
0.));
#242097=CARTESIAN_POINT('Ctrl Pts',(-13.0783089692118,19.2626927725596,
0.));
#242098=CARTESIAN_POINT('Ctrl Pts',(-13.0840182984949,19.2786358177198,
0.));
#242099=CARTESIAN_POINT('Ctrl Pts',(-13.089725714597,19.2947206141246,0.));
#242100=CARTESIAN_POINT('Ctrl Pts',(-13.095430221148,19.3109461507358,0.));
#242101=CARTESIAN_POINT('Ctrl Pts',(-13.1011308397592,19.3273114318268,
0.));
#242102=CARTESIAN_POINT('Ctrl Pts',(-13.1068266095186,19.3438154765395,
0.));
#242103=CARTESIAN_POINT('Ctrl Pts',(-13.1125165865021,19.3604573184516,
0.));
#242104=CARTESIAN_POINT('Ctrl Pts',(-13.118199843271,19.3772360051093,0.));
#242105=CARTESIAN_POINT('Ctrl Pts',(-13.1238754684177,19.3941505976267,
0.));
#242106=CARTESIAN_POINT('Ctrl Pts',(-13.1295425661635,19.4112001703561,
0.));
#242107=CARTESIAN_POINT('Ctrl Pts',(-13.1352002559439,19.4283838105265,
0.));
#242108=CARTESIAN_POINT('Ctrl Pts',(-13.140847672006,19.4457006178875,0.));
#242109=CARTESIAN_POINT('Ctrl Pts',(-13.1464839629966,19.463149704325,0.));
#242110=CARTESIAN_POINT('Ctrl Pts',(-13.1521082915846,19.4807301935256,
0.));
#242111=CARTESIAN_POINT('Ctrl Pts',(-13.1577198341238,19.498441220707,0.));
#242112=CARTESIAN_POINT('Ctrl Pts',(-13.1633177803097,19.5162819323207,
0.));
#242113=CARTESIAN_POINT('Ctrl Pts',(-13.1689013328432,19.5342514857564,
0.));
#242114=CARTESIAN_POINT('Ctrl Pts',(-13.1744697070918,19.5523490490254,
0.));
#242115=CARTESIAN_POINT('Ctrl Pts',(-13.1800221307683,19.5705738004682,
0.));
#242116=CARTESIAN_POINT('Ctrl Pts',(-13.1855578436479,19.5889249285351,
0.));
#242117=CARTESIAN_POINT('Ctrl Pts',(-13.1910760972818,19.6074016315421,
0.));
#242118=CARTESIAN_POINT('Ctrl Pts',(-13.196576154715,19.6260031174244,0.));
#242119=CARTESIAN_POINT('Ctrl Pts',(-13.202057290206,19.6447286034764,0.));
#242120=CARTESIAN_POINT('Ctrl Pts',(-13.2075187889522,19.6635773160924,
0.));
#242121=CARTESIAN_POINT('Ctrl Pts',(-13.2129599468478,19.6825484905812,
0.));
#242122=CARTESIAN_POINT('Ctrl Pts',(-13.2183800702431,19.7016413709678,
0.));
#242123=CARTESIAN_POINT('Ctrl Pts',(-13.2237784757065,19.7208552097867,
0.));
#242124=CARTESIAN_POINT('Ctrl Pts',(-13.2291544897902,19.7401892678701,
0.));
#242125=CARTESIAN_POINT('Ctrl Pts',(-13.2345074487968,19.7596428141176,
0.));
#242126=CARTESIAN_POINT('Ctrl Pts',(-13.239836698568,19.7792151253297,0.));
#242127=CARTESIAN_POINT('Ctrl Pts',(-13.2451415942809,19.7989054860501,
0.));
#242128=CARTESIAN_POINT('Ctrl Pts',(-13.2504215002458,19.8187131883919,
0.));
#242129=CARTESIAN_POINT('Ctrl Pts',(-13.2556757897085,19.8386375318632,
0.));
#242130=CARTESIAN_POINT('Ctrl Pts',(-13.2609038446525,19.8586778231711,
0.));
#242131=CARTESIAN_POINT('Ctrl Pts',(-13.2661050556128,19.8788333760571,
0.));
#242132=CARTESIAN_POINT('Ctrl Pts',(-13.2712788215015,19.8991035111739,
0.));
#242133=CARTESIAN_POINT('Ctrl Pts',(-13.2764245494354,19.9194875559419,
0.));
#242134=CARTESIAN_POINT('Ctrl Pts',(-13.2815416545663,19.9399848444019,
0.));
#242135=CARTESIAN_POINT('Ctrl Pts',(-13.2866295599152,19.9605947170589,
0.));
#242136=CARTESIAN_POINT('Ctrl Pts',(-13.2916876962098,19.9813165207174,
0.));
#242137=CARTESIAN_POINT('Ctrl Pts',(-13.296715501731,20.0021496083742,0.));
#242138=CARTESIAN_POINT('Ctrl Pts',(-13.3017124221639,20.0230933391039,
0.));
#242139=CARTESIAN_POINT('Ctrl Pts',(-13.3066779104515,20.0441470779345,
0.));
#242140=CARTESIAN_POINT('Ctrl Pts',(-13.3116114266514,20.0653101957188,
0.));
#242141=CARTESIAN_POINT('Ctrl Pts',(-13.3165124377963,20.0865820689883,
0.));
#242142=CARTESIAN_POINT('Ctrl Pts',(-13.3213804177588,20.1079620798377,
0.));
#242143=CARTESIAN_POINT('Ctrl Pts',(-13.3262148471228,20.1294496158405,
0.));
#242144=CARTESIAN_POINT('Ctrl Pts',(-13.3310152130565,20.1510440699477,
0.));
#242145=CARTESIAN_POINT('Ctrl Pts',(-13.3357810091903,20.1727448403818,
0.));
#242146=CARTESIAN_POINT('Ctrl Pts',(-13.3405117354969,20.1945513305233,
0.));
#242147=CARTESIAN_POINT('Ctrl Pts',(-13.3452068981763,20.2164629487855,
0.));
#242148=CARTESIAN_POINT('Ctrl Pts',(-13.3498660095382,20.2384791085354,
0.));
#242149=CARTESIAN_POINT('Ctrl Pts',(-13.3544885878886,20.2605992280117,
0.));
#242150=CARTESIAN_POINT('Ctrl Pts',(-13.3590741574194,20.2828227302337,
0.));
#242151=CARTESIAN_POINT('Ctrl Pts',(-13.3636222481017,20.3051490429049,
0.));
#242152=CARTESIAN_POINT('Ctrl Pts',(-13.3681323955828,20.3275775983032,
0.));
#242153=CARTESIAN_POINT('Ctrl Pts',(-13.3726041410869,20.3501078331818,
0.));
#242154=CARTESIAN_POINT('Ctrl Pts',(-13.377037031319,20.3727391887187,0.));
#242155=CARTESIAN_POINT('Ctrl Pts',(-13.3814306183721,20.3954711104504,
0.));
#242156=CARTESIAN_POINT('Ctrl Pts',(-13.3857844596387,20.4183030482002,
0.));
#242157=CARTESIAN_POINT('Ctrl Pts',(-13.3900981177254,20.4412344560007,
0.));
#242158=CARTESIAN_POINT('Ctrl Pts',(-13.3943711603739,20.4642647920038,
0.));
#242159=CARTESIAN_POINT('Ctrl Pts',(-13.3986031603716,20.4873935184041,
0.));
#242160=CARTESIAN_POINT('Ctrl Pts',(-13.4027936954529,20.5106201013755,
0.));
#242161=CARTESIAN_POINT('Ctrl Pts',(-13.4069423482076,20.5339440109957,
0.));
#242162=CARTESIAN_POINT('Ctrl Pts',(-13.4110487059912,20.557364721164,0.));
#242163=CARTESIAN_POINT('Ctrl Pts',(-13.4151123608411,20.5808817095155,
0.));
#242164=CARTESIAN_POINT('Ctrl Pts',(-13.4191329093932,20.6044944573151,
0.));
#242165=CARTESIAN_POINT('Ctrl Pts',(-13.4231099528178,20.6282024494234,
0.));
#242166=CARTESIAN_POINT('Ctrl Pts',(-13.427043096765,20.6520051742867,0.));
#242167=CARTESIAN_POINT('Ctrl Pts',(-13.4309319513119,20.6759021239102,
0.));
#242168=CARTESIAN_POINT('Ctrl Pts',(-13.4347761309154,20.6998927938288,
0.));
#242169=CARTESIAN_POINT('Ctrl Pts',(-13.4385752543663,20.7239766830675,
0.));
#242170=CARTESIAN_POINT('Ctrl Pts',(-13.4423289447561,20.7481532941014,
0.));
#242171=CARTESIAN_POINT('Ctrl Pts',(-13.4460368293689,20.7724221327609,
0.));
#242172=CARTESIAN_POINT('Ctrl Pts',(-13.4496985395637,20.7967827081228,
0.));
#242173=CARTESIAN_POINT('Ctrl Pts',(-13.4533137106667,20.821234532398,0.));
#242174=CARTESIAN_POINT('Ctrl Pts',(-13.4568819818631,20.8457771208083,
0.));
#242175=CARTESIAN_POINT('Ctrl Pts',(-13.4604029960983,20.8704099914641,
0.));
#242176=CARTESIAN_POINT('Ctrl Pts',(-13.4638763999725,20.8951326652158,
0.));
#242177=CARTESIAN_POINT('Ctrl Pts',(-13.4673018437717,20.9199446657583,
0.));
#242178=CARTESIAN_POINT('Ctrl Pts',(-13.4706789815166,20.9448455197557,
0.));
#242179=CARTESIAN_POINT('Ctrl Pts',(-13.4740074710086,20.9698347569476,
0.));
#242180=CARTESIAN_POINT('Ctrl Pts',(-13.4772869738879,20.9949119102592,
0.));
#242181=CARTESIAN_POINT('Ctrl Pts',(-13.4805171556822,21.0200765158884,
0.));
#242182=CARTESIAN_POINT('Ctrl Pts',(-13.4836976858912,21.0453281134245,
0.));
#242183=CARTESIAN_POINT('Ctrl Pts',(-13.4868282377191,21.0706662455199,
0.));
#242184=CARTESIAN_POINT('Ctrl Pts',(-13.4899084877717,21.0960904575046,
0.));
#242185=CARTESIAN_POINT('Ctrl Pts',(-13.4929381157778,21.1216002970207,
0.));
#242186=CARTESIAN_POINT('Ctrl Pts',(-13.4959168042934,21.1471953136209,
0.));
#242187=CARTESIAN_POINT('Ctrl Pts',(-13.4988442384491,21.1728750584175,
0.));
#242188=CARTESIAN_POINT('Ctrl Pts',(-13.5017201056088,21.1986390835828,
0.));
#242189=CARTESIAN_POINT('Ctrl Pts',(-13.5045440957404,21.2244869429332,
0.));
#242190=CARTESIAN_POINT('Ctrl Pts',(-13.5073159019452,21.250418192743,0.));
#242191=CARTESIAN_POINT('Ctrl Pts',(-13.5100352209205,21.2764323924442,
0.));
#242192=CARTESIAN_POINT('Ctrl Pts',(-13.5127017534971,21.3025291054235,
0.));
#242193=CARTESIAN_POINT('Ctrl Pts',(-13.5153152050555,21.328707899634,0.));
#242194=CARTESIAN_POINT('Ctrl Pts',(-13.5178752862466,21.3549683486222,
0.));
#242195=CARTESIAN_POINT('Ctrl Pts',(-13.5203817122504,21.3813100304973,
0.));
#242196=CARTESIAN_POINT('Ctrl Pts',(-13.5228342013516,21.4077325259324,
0.));
#242197=CARTESIAN_POINT('Ctrl Pts',(-13.5252324737802,21.4342354165259,
0.));
#242198=CARTESIAN_POINT('Ctrl Pts',(-13.5275762503555,21.4608182828697,
0.));
#242199=CARTESIAN_POINT('Ctrl Pts',(-13.5298652514355,21.4874807030468,
0.));
#242200=CARTESIAN_POINT('Ctrl Pts',(-13.5320991952138,21.5142222501666,
0.));
#242201=CARTESIAN_POINT('Ctrl Pts',(-13.5342777983215,21.5410424932503,
0.));
#242202=CARTESIAN_POINT('Ctrl Pts',(-13.536400779028,21.5679410019001,0.));
#242203=CARTESIAN_POINT('Ctrl Pts',(-13.5384678597195,21.5949173499013,
0.));
#242204=CARTESIAN_POINT('Ctrl Pts',(-13.5404787697792,21.6219711193946,
0.));
#242205=CARTESIAN_POINT('Ctrl Pts',(-13.5424332480699,21.6491019044648,
0.));
#242206=CARTESIAN_POINT('Ctrl Pts',(-13.5443310461526,21.6763093157699,
0.));
#242207=CARTESIAN_POINT('Ctrl Pts',(-13.5461719295048,21.7035929822955,
0.));
#242208=CARTESIAN_POINT('Ctrl Pts',(-13.5479556704481,21.7309525412281,
0.));
#242209=CARTESIAN_POINT('Ctrl Pts',(-13.5496820422211,21.7583876294554,
0.));
#242210=CARTESIAN_POINT('Ctrl Pts',(-13.551350812725,21.7858978745865,0.));
#242211=CARTESIAN_POINT('Ctrl Pts',(-13.5529617381573,21.8134828857967,
0.));
#242212=CARTESIAN_POINT('Ctrl Pts',(-13.5545145573031,21.8411422456075,
0.));
#242213=CARTESIAN_POINT('Ctrl Pts',(-13.5560089839385,21.8688754989365,
0.));
#242214=CARTESIAN_POINT('Ctrl Pts',(-13.5574447178424,21.8966821688824,
0.));
#242215=CARTESIAN_POINT('Ctrl Pts',(-13.5588214586604,21.9245617765769,
0.));
#242216=CARTESIAN_POINT('Ctrl Pts',(-13.5601389185257,21.9525138592813,
0.));
#242217=CARTESIAN_POINT('Ctrl Pts',(-13.5613968357561,21.9805379899168,
0.));
#242218=CARTESIAN_POINT('Ctrl Pts',(-13.5625949868333,22.0086337943449,
0.));
#242219=CARTESIAN_POINT('Ctrl Pts',(-13.5637332022473,22.0368009736295,
0.));
#242220=CARTESIAN_POINT('Ctrl Pts',(-13.5648113689033,22.0650393089609,
0.));
#242221=CARTESIAN_POINT('Ctrl Pts',(-13.5658294169284,22.0933486464593,
0.));
#242222=CARTESIAN_POINT('Ctrl Pts',(-13.5667873105359,22.1217288871975,
0.));
#242223=CARTESIAN_POINT('Ctrl Pts',(-13.5675054919061,22.1444897575194,
0.));
#242224=CARTESIAN_POINT('Ctrl Pts',(-13.5680170531805,22.1615922805008,
0.));
#242225=CARTESIAN_POINT('Ctrl Pts',(-13.5683460612942,22.1730081264608,
0.));
#242226=CARTESIAN_POINT('Ctrl Pts',(-13.5685075571671,22.1787195904339,
0.));
#242227=CARTESIAN_POINT('',(-13.5685075571671,22.1787195904339,12.));
#242228=CARTESIAN_POINT('Ctrl Pts',(-13.5685075571671,22.1787195904339,
12.));
#242229=CARTESIAN_POINT('Ctrl Pts',(-13.5683460612942,22.1730081264608,
12.));
#242230=CARTESIAN_POINT('Ctrl Pts',(-13.5680170531805,22.1615922805008,
12.));
#242231=CARTESIAN_POINT('Ctrl Pts',(-13.5675054919061,22.1444897575194,
12.));
#242232=CARTESIAN_POINT('Ctrl Pts',(-13.5667873105359,22.1217288871975,
12.));
#242233=CARTESIAN_POINT('Ctrl Pts',(-13.5658294169284,22.0933486464593,
12.));
#242234=CARTESIAN_POINT('Ctrl Pts',(-13.5648113689033,22.0650393089609,
12.));
#242235=CARTESIAN_POINT('Ctrl Pts',(-13.5637332022473,22.0368009736295,
12.));
#242236=CARTESIAN_POINT('Ctrl Pts',(-13.5625949868333,22.0086337943449,
12.));
#242237=CARTESIAN_POINT('Ctrl Pts',(-13.5613968357561,21.9805379899168,
12.));
#242238=CARTESIAN_POINT('Ctrl Pts',(-13.5601389185257,21.9525138592813,
12.));
#242239=CARTESIAN_POINT('Ctrl Pts',(-13.5588214586604,21.9245617765769,
12.));
#242240=CARTESIAN_POINT('Ctrl Pts',(-13.5574447178424,21.8966821688824,
12.));
#242241=CARTESIAN_POINT('Ctrl Pts',(-13.5560089839385,21.8688754989365,
12.));
#242242=CARTESIAN_POINT('Ctrl Pts',(-13.5545145573031,21.8411422456075,
12.));
#242243=CARTESIAN_POINT('Ctrl Pts',(-13.5529617381573,21.8134828857967,
12.));
#242244=CARTESIAN_POINT('Ctrl Pts',(-13.551350812725,21.7858978745865,12.));
#242245=CARTESIAN_POINT('Ctrl Pts',(-13.5496820422211,21.7583876294554,
12.));
#242246=CARTESIAN_POINT('Ctrl Pts',(-13.5479556704481,21.7309525412281,
12.));
#242247=CARTESIAN_POINT('Ctrl Pts',(-13.5461719295048,21.7035929822955,
12.));
#242248=CARTESIAN_POINT('Ctrl Pts',(-13.5443310461526,21.6763093157699,
12.));
#242249=CARTESIAN_POINT('Ctrl Pts',(-13.5424332480699,21.6491019044648,
12.));
#242250=CARTESIAN_POINT('Ctrl Pts',(-13.5404787697792,21.6219711193946,
12.));
#242251=CARTESIAN_POINT('Ctrl Pts',(-13.5384678597195,21.5949173499013,
12.));
#242252=CARTESIAN_POINT('Ctrl Pts',(-13.536400779028,21.5679410019001,12.));
#242253=CARTESIAN_POINT('Ctrl Pts',(-13.5342777983215,21.5410424932503,
12.));
#242254=CARTESIAN_POINT('Ctrl Pts',(-13.5320991952138,21.5142222501666,
12.));
#242255=CARTESIAN_POINT('Ctrl Pts',(-13.5298652514355,21.4874807030468,
12.));
#242256=CARTESIAN_POINT('Ctrl Pts',(-13.5275762503555,21.4608182828697,
12.));
#242257=CARTESIAN_POINT('Ctrl Pts',(-13.5252324737802,21.4342354165259,
12.));
#242258=CARTESIAN_POINT('Ctrl Pts',(-13.5228342013516,21.4077325259324,
12.));
#242259=CARTESIAN_POINT('Ctrl Pts',(-13.5203817122504,21.3813100304973,
12.));
#242260=CARTESIAN_POINT('Ctrl Pts',(-13.5178752862466,21.3549683486222,
12.));
#242261=CARTESIAN_POINT('Ctrl Pts',(-13.5153152050555,21.328707899634,12.));
#242262=CARTESIAN_POINT('Ctrl Pts',(-13.5127017534971,21.3025291054235,
12.));
#242263=CARTESIAN_POINT('Ctrl Pts',(-13.5100352209205,21.2764323924442,
12.));
#242264=CARTESIAN_POINT('Ctrl Pts',(-13.5073159019452,21.250418192743,12.));
#242265=CARTESIAN_POINT('Ctrl Pts',(-13.5045440957404,21.2244869429332,
12.));
#242266=CARTESIAN_POINT('Ctrl Pts',(-13.5017201056088,21.1986390835828,
12.));
#242267=CARTESIAN_POINT('Ctrl Pts',(-13.4988442384491,21.1728750584175,
12.));
#242268=CARTESIAN_POINT('Ctrl Pts',(-13.4959168042934,21.1471953136209,
12.));
#242269=CARTESIAN_POINT('Ctrl Pts',(-13.4929381157778,21.1216002970207,
12.));
#242270=CARTESIAN_POINT('Ctrl Pts',(-13.4899084877717,21.0960904575046,
12.));
#242271=CARTESIAN_POINT('Ctrl Pts',(-13.4868282377191,21.0706662455199,
12.));
#242272=CARTESIAN_POINT('Ctrl Pts',(-13.4836976858912,21.0453281134245,
12.));
#242273=CARTESIAN_POINT('Ctrl Pts',(-13.4805171556822,21.0200765158884,
12.));
#242274=CARTESIAN_POINT('Ctrl Pts',(-13.4772869738879,20.9949119102592,
12.));
#242275=CARTESIAN_POINT('Ctrl Pts',(-13.4740074710086,20.9698347569476,
12.));
#242276=CARTESIAN_POINT('Ctrl Pts',(-13.4706789815166,20.9448455197557,
12.));
#242277=CARTESIAN_POINT('Ctrl Pts',(-13.4673018437717,20.9199446657583,
12.));
#242278=CARTESIAN_POINT('Ctrl Pts',(-13.4638763999725,20.8951326652158,
12.));
#242279=CARTESIAN_POINT('Ctrl Pts',(-13.4604029960983,20.8704099914641,
12.));
#242280=CARTESIAN_POINT('Ctrl Pts',(-13.4568819818631,20.8457771208083,
12.));
#242281=CARTESIAN_POINT('Ctrl Pts',(-13.4533137106667,20.821234532398,12.));
#242282=CARTESIAN_POINT('Ctrl Pts',(-13.4496985395637,20.7967827081228,
12.));
#242283=CARTESIAN_POINT('Ctrl Pts',(-13.4460368293689,20.7724221327609,
12.));
#242284=CARTESIAN_POINT('Ctrl Pts',(-13.4423289447561,20.7481532941014,
12.));
#242285=CARTESIAN_POINT('Ctrl Pts',(-13.4385752543663,20.7239766830675,
12.));
#242286=CARTESIAN_POINT('Ctrl Pts',(-13.4347761309154,20.6998927938288,
12.));
#242287=CARTESIAN_POINT('Ctrl Pts',(-13.4309319513119,20.6759021239102,
12.));
#242288=CARTESIAN_POINT('Ctrl Pts',(-13.427043096765,20.6520051742867,12.));
#242289=CARTESIAN_POINT('Ctrl Pts',(-13.4231099528178,20.6282024494234,
12.));
#242290=CARTESIAN_POINT('Ctrl Pts',(-13.4191329093932,20.6044944573151,
12.));
#242291=CARTESIAN_POINT('Ctrl Pts',(-13.4151123608411,20.5808817095155,
12.));
#242292=CARTESIAN_POINT('Ctrl Pts',(-13.4110487059912,20.557364721164,12.));
#242293=CARTESIAN_POINT('Ctrl Pts',(-13.4069423482076,20.5339440109957,
12.));
#242294=CARTESIAN_POINT('Ctrl Pts',(-13.4027936954529,20.5106201013755,
12.));
#242295=CARTESIAN_POINT('Ctrl Pts',(-13.3986031603716,20.4873935184041,
12.));
#242296=CARTESIAN_POINT('Ctrl Pts',(-13.3943711603739,20.4642647920038,
12.));
#242297=CARTESIAN_POINT('Ctrl Pts',(-13.3900981177254,20.4412344560007,
12.));
#242298=CARTESIAN_POINT('Ctrl Pts',(-13.3857844596387,20.4183030482002,
12.));
#242299=CARTESIAN_POINT('Ctrl Pts',(-13.3814306183721,20.3954711104504,
12.));
#242300=CARTESIAN_POINT('Ctrl Pts',(-13.377037031319,20.3727391887187,12.));
#242301=CARTESIAN_POINT('Ctrl Pts',(-13.3726041410869,20.3501078331818,
12.));
#242302=CARTESIAN_POINT('Ctrl Pts',(-13.3681323955828,20.3275775983032,
12.));
#242303=CARTESIAN_POINT('Ctrl Pts',(-13.3636222481017,20.3051490429049,
12.));
#242304=CARTESIAN_POINT('Ctrl Pts',(-13.3590741574194,20.2828227302337,
12.));
#242305=CARTESIAN_POINT('Ctrl Pts',(-13.3544885878886,20.2605992280117,
12.));
#242306=CARTESIAN_POINT('Ctrl Pts',(-13.3498660095382,20.2384791085354,
12.));
#242307=CARTESIAN_POINT('Ctrl Pts',(-13.3452068981763,20.2164629487855,
12.));
#242308=CARTESIAN_POINT('Ctrl Pts',(-13.3405117354969,20.1945513305233,
12.));
#242309=CARTESIAN_POINT('Ctrl Pts',(-13.3357810091903,20.1727448403818,
12.));
#242310=CARTESIAN_POINT('Ctrl Pts',(-13.3310152130565,20.1510440699477,
12.));
#242311=CARTESIAN_POINT('Ctrl Pts',(-13.3262148471228,20.1294496158405,
12.));
#242312=CARTESIAN_POINT('Ctrl Pts',(-13.3213804177588,20.1079620798377,
12.));
#242313=CARTESIAN_POINT('Ctrl Pts',(-13.3165124377963,20.0865820689883,
12.));
#242314=CARTESIAN_POINT('Ctrl Pts',(-13.3116114266514,20.0653101957188,
12.));
#242315=CARTESIAN_POINT('Ctrl Pts',(-13.3066779104515,20.0441470779345,
12.));
#242316=CARTESIAN_POINT('Ctrl Pts',(-13.3017124221639,20.0230933391039,
12.));
#242317=CARTESIAN_POINT('Ctrl Pts',(-13.296715501731,20.0021496083742,12.));
#242318=CARTESIAN_POINT('Ctrl Pts',(-13.2916876962098,19.9813165207174,
12.));
#242319=CARTESIAN_POINT('Ctrl Pts',(-13.2866295599152,19.9605947170589,
12.));
#242320=CARTESIAN_POINT('Ctrl Pts',(-13.2815416545663,19.9399848444019,
12.));
#242321=CARTESIAN_POINT('Ctrl Pts',(-13.2764245494354,19.9194875559419,
12.));
#242322=CARTESIAN_POINT('Ctrl Pts',(-13.2712788215015,19.8991035111739,
12.));
#242323=CARTESIAN_POINT('Ctrl Pts',(-13.2661050556128,19.8788333760571,
12.));
#242324=CARTESIAN_POINT('Ctrl Pts',(-13.2609038446525,19.8586778231711,
12.));
#242325=CARTESIAN_POINT('Ctrl Pts',(-13.2556757897085,19.8386375318632,
12.));
#242326=CARTESIAN_POINT('Ctrl Pts',(-13.2504215002458,19.8187131883919,
12.));
#242327=CARTESIAN_POINT('Ctrl Pts',(-13.2451415942809,19.7989054860501,
12.));
#242328=CARTESIAN_POINT('Ctrl Pts',(-13.239836698568,19.7792151253297,12.));
#242329=CARTESIAN_POINT('Ctrl Pts',(-13.2345074487968,19.7596428141176,
12.));
#242330=CARTESIAN_POINT('Ctrl Pts',(-13.2291544897902,19.7401892678701,
12.));
#242331=CARTESIAN_POINT('Ctrl Pts',(-13.2237784757065,19.7208552097867,
12.));
#242332=CARTESIAN_POINT('Ctrl Pts',(-13.2183800702431,19.7016413709678,
12.));
#242333=CARTESIAN_POINT('Ctrl Pts',(-13.2129599468478,19.6825484905812,
12.));
#242334=CARTESIAN_POINT('Ctrl Pts',(-13.2075187889522,19.6635773160924,
12.));
#242335=CARTESIAN_POINT('Ctrl Pts',(-13.202057290206,19.6447286034764,12.));
#242336=CARTESIAN_POINT('Ctrl Pts',(-13.196576154715,19.6260031174244,12.));
#242337=CARTESIAN_POINT('Ctrl Pts',(-13.1910760972818,19.6074016315421,
12.));
#242338=CARTESIAN_POINT('Ctrl Pts',(-13.1855578436479,19.5889249285351,
12.));
#242339=CARTESIAN_POINT('Ctrl Pts',(-13.1800221307683,19.5705738004682,
12.));
#242340=CARTESIAN_POINT('Ctrl Pts',(-13.1744697070918,19.5523490490254,
12.));
#242341=CARTESIAN_POINT('Ctrl Pts',(-13.1689013328432,19.5342514857564,
12.));
#242342=CARTESIAN_POINT('Ctrl Pts',(-13.1633177803097,19.5162819323207,
12.));
#242343=CARTESIAN_POINT('Ctrl Pts',(-13.1577198341238,19.498441220707,12.));
#242344=CARTESIAN_POINT('Ctrl Pts',(-13.1521082915846,19.4807301935256,
12.));
#242345=CARTESIAN_POINT('Ctrl Pts',(-13.1464839629966,19.463149704325,12.));
#242346=CARTESIAN_POINT('Ctrl Pts',(-13.140847672006,19.4457006178875,12.));
#242347=CARTESIAN_POINT('Ctrl Pts',(-13.1352002559439,19.4283838105265,
12.));
#242348=CARTESIAN_POINT('Ctrl Pts',(-13.1295425661635,19.4112001703561,
12.));
#242349=CARTESIAN_POINT('Ctrl Pts',(-13.1238754684177,19.3941505976267,
12.));
#242350=CARTESIAN_POINT('Ctrl Pts',(-13.118199843271,19.3772360051093,12.));
#242351=CARTESIAN_POINT('Ctrl Pts',(-13.1125165865021,19.3604573184516,
12.));
#242352=CARTESIAN_POINT('Ctrl Pts',(-13.1068266095186,19.3438154765395,
12.));
#242353=CARTESIAN_POINT('Ctrl Pts',(-13.1011308397592,19.3273114318268,
12.));
#242354=CARTESIAN_POINT('Ctrl Pts',(-13.095430221148,19.3109461507358,12.));
#242355=CARTESIAN_POINT('Ctrl Pts',(-13.089725714597,19.2947206141246,12.));
#242356=CARTESIAN_POINT('Ctrl Pts',(-13.0840182984949,19.2786358177198,
12.));
#242357=CARTESIAN_POINT('Ctrl Pts',(-13.0783089692118,19.2626927725596,
12.));
#242358=CARTESIAN_POINT('Ctrl Pts',(-13.0725987415856,19.2468925053988,
12.));
#242359=CARTESIAN_POINT('Ctrl Pts',(-13.0668886494791,19.2312360592031,
12.));
#242360=CARTESIAN_POINT('Ctrl Pts',(-13.0611797463913,19.2157244937141,
12.));
#242361=CARTESIAN_POINT('Ctrl Pts',(-13.0554731060537,19.2003588859771,
12.));
#242362=CARTESIAN_POINT('Ctrl Pts',(-13.0497698230442,19.1851403308825,
12.));
#242363=CARTESIAN_POINT('Ctrl Pts',(-13.0440710133775,19.1700699416625,
12.));
#242364=CARTESIAN_POINT('Ctrl Pts',(-13.0383778152072,19.1551488505233,
12.));
#242365=CARTESIAN_POINT('Ctrl Pts',(-13.0326913895841,19.1403782093389,
12.));
#242366=CARTESIAN_POINT('Ctrl Pts',(-13.0270129211976,19.1257591903099,
12.));
#242367=CARTESIAN_POINT('Ctrl Pts',(-13.0213436191326,19.1112929866308,
12.));
#242368=CARTESIAN_POINT('Ctrl Pts',(-13.0156847176093,19.0969808131225,
12.));
#242369=CARTESIAN_POINT('Ctrl Pts',(-13.0100374768785,19.0828239070482,
12.));
#242370=CARTESIAN_POINT('Ctrl Pts',(-13.0044031841381,19.0688235289437,
12.));
#242371=CARTESIAN_POINT('Ctrl Pts',(-12.9987831544502,19.0549809634355,
12.));
#242372=CARTESIAN_POINT('Ctrl Pts',(-12.9931787316515,19.0412975200398,
12.));
#242373=CARTESIAN_POINT('Ctrl Pts',(-12.9875912893003,19.0277745339908,
12.));
#242374=CARTESIAN_POINT('Ctrl Pts',(-12.9820222318716,19.0144133673348,
12.));
#242375=CARTESIAN_POINT('Ctrl Pts',(-12.9764729959205,19.0012154099791,
12.));
#242376=CARTESIAN_POINT('Ctrl Pts',(-12.9709450512747,18.9881820807585,
12.));
#242377=CARTESIAN_POINT('Ctrl Pts',(-12.9654399021869,18.9753148284475,
12.));
#242378=CARTESIAN_POINT('Ctrl Pts',(-12.9599590886319,18.9626151329229,
12.));
#242379=CARTESIAN_POINT('Ctrl Pts',(-12.9545041877377,18.9500845064715,
12.));
#242380=CARTESIAN_POINT('Ctrl Pts',(-12.9490768151821,18.9377244950435,
12.));
#242381=CARTESIAN_POINT('Ctrl Pts',(-12.9436786266105,18.9255366795195,
12.));
#242382=CARTESIAN_POINT('Ctrl Pts',(-12.9383113190375,18.9135226769465,
12.));
#242383=CARTESIAN_POINT('Ctrl Pts',(-12.9329766328185,18.9016841423403,
12.));
#242384=CARTESIAN_POINT('Ctrl Pts',(-12.9276763536373,18.8900227704889,
12.));
#242385=CARTESIAN_POINT('Ctrl Pts',(-12.9224123144982,18.8785402977527,
12.));
#242386=CARTESIAN_POINT('Ctrl Pts',(-12.9171863977045,18.8672385038326,
12.));
#242387=CARTESIAN_POINT('Ctrl Pts',(-12.9120005369063,18.8561192136198,
12.));
#242388=CARTESIAN_POINT('Ctrl Pts',(-12.9068567191854,18.8451842990984,
12.));
#242389=CARTESIAN_POINT('Ctrl Pts',(-12.9017569871738,18.834435681259,12.));
#242390=CARTESIAN_POINT('Ctrl Pts',(-12.8967034410755,18.8238753319128,
12.));
#242391=CARTESIAN_POINT('Ctrl Pts',(-12.8916982409935,18.813505275782,12.));
#242392=CARTESIAN_POINT('Ctrl Pts',(-12.8867436109546,18.8033275941943,
12.));
#242393=CARTESIAN_POINT('Ctrl Pts',(-12.8818418427475,18.7933444285868,
12.));
#242394=CARTESIAN_POINT('Ctrl Pts',(-12.8769952998095,18.7835579840477,
12.));
#242395=CARTESIAN_POINT('Ctrl Pts',(-12.872206421181,18.7739705329022,12.));
#242396=CARTESIAN_POINT('Ctrl Pts',(-12.8674777239653,18.7645844169564,
12.));
#242397=CARTESIAN_POINT('Ctrl Pts',(-12.8628118054171,18.7554020493887,
12.));
#242398=CARTESIAN_POINT('Ctrl Pts',(-12.8582113455646,18.7464259171251,
12.));
#242399=CARTESIAN_POINT('Ctrl Pts',(-12.8536791086316,18.7376585820854,
12.));
#242400=CARTESIAN_POINT('Ctrl Pts',(-12.8492179511591,18.7291026886554,
12.));
#242401=CARTESIAN_POINT('Ctrl Pts',(-12.8448308329494,18.7207609737702,
12.));
#242402=CARTESIAN_POINT('Ctrl Pts',(-12.8405208263431,18.7126362754445,
12.));
#242403=CARTESIAN_POINT('Ctrl Pts',(-12.8362911280361,18.7047315436294,
12.));
#242404=CARTESIAN_POINT('Ctrl Pts',(-12.8321450599789,18.6970498410172,
12.));
#242405=CARTESIAN_POINT('Ctrl Pts',(-12.8280860635231,18.6895943376171,
12.));
#242406=CARTESIAN_POINT('Ctrl Pts',(-12.8241176980017,18.6823683094139,
12.));
#242407=CARTESIAN_POINT('Ctrl Pts',(-12.8202436318474,18.6753751301092,
12.));
#242408=CARTESIAN_POINT('Ctrl Pts',(-12.8164676687362,18.6686182952799,
12.));
#242409=CARTESIAN_POINT('Ctrl Pts',(-12.8127937909631,18.6621014624746,
12.));
#242410=CARTESIAN_POINT('Ctrl Pts',(-12.8092261933858,18.6558284825773,
12.));
#242411=CARTESIAN_POINT('Ctrl Pts',(-12.805769331162,18.6498034438986,12.));
#242412=CARTESIAN_POINT('Ctrl Pts',(-12.8024278770152,18.6440306327456,
12.));
#242413=CARTESIAN_POINT('Ctrl Pts',(-12.7992066625264,18.63851447924,12.));
#242414=CARTESIAN_POINT('Ctrl Pts',(-12.7961106222251,18.6332595057006,
12.));
#242415=CARTESIAN_POINT('Ctrl Pts',(-12.7931447451555,18.6282702819371,
12.));
#242416=CARTESIAN_POINT('Ctrl Pts',(-12.7903142925234,18.6235516265575,
12.));
#242417=CARTESIAN_POINT('Ctrl Pts',(-12.7876249657834,18.6191087624752,
12.));
#242418=CARTESIAN_POINT('Ctrl Pts',(-12.7850831657901,18.6149475565188,
12.));
#242419=CARTESIAN_POINT('Ctrl Pts',(-12.7826959526925,18.6110744826219,
12.));
#242420=CARTESIAN_POINT('Ctrl Pts',(-12.7804705387658,18.6074961535723,
12.));
#242421=CARTESIAN_POINT('Ctrl Pts',(-12.7784139605066,18.6042190183704,
12.));
#242422=CARTESIAN_POINT('Ctrl Pts',(-12.7765325225081,18.6012488486709,
12.));
#242423=CARTESIAN_POINT('Ctrl Pts',(-12.7748328937638,18.598591752595,12.));
#242424=CARTESIAN_POINT('Ctrl Pts',(-12.7733231262108,18.5962551167772,
12.));
#242425=CARTESIAN_POINT('Ctrl Pts',(-12.7720142287172,18.5942490615407,
12.));
#242426=CARTESIAN_POINT('Ctrl Pts',(-12.7709195951156,18.5925859134579,
12.));
#242427=CARTESIAN_POINT('Ctrl Pts',(-12.7700520897173,18.5912775137806,
12.));
#242428=CARTESIAN_POINT('Ctrl Pts',(-12.7694215127919,18.5903328777227,
12.));
#242429=CARTESIAN_POINT('Ctrl Pts',(-12.769110348199,18.589871621843,12.));
#242430=CARTESIAN_POINT('Ctrl Pts',(-12.768986426692,18.5896919669165,12.));
#242431=CARTESIAN_POINT('Ctrl Pts',(-12.7689524524483,18.5896460962964,
12.));
#242432=CARTESIAN_POINT('Ctrl Pts',(-12.7689476255363,18.5896416359912,
12.));
#242433=CARTESIAN_POINT('',(-13.5685075571671,22.1787195904339,0.));
#242434=CARTESIAN_POINT('Origin',(-7.17139709155223,20.2687213152502,0.));
#242435=CARTESIAN_POINT('',(-7.52250298901264,21.2610617890679,12.));
#242436=CARTESIAN_POINT('',(-3.58569854577611,10.1343606576251,12.));
#242437=CARTESIAN_POINT('',(-7.52250298901264,21.2610617890679,0.));
#242438=CARTESIAN_POINT('',(-7.52250298901264,21.2610617890679,0.));
#242439=CARTESIAN_POINT('',(-3.58569854577611,10.1343606576251,0.));
#242440=CARTESIAN_POINT('Ctrl Pts',(-12.4230808101438,22.8400320311648,
0.));
#242441=CARTESIAN_POINT('Ctrl Pts',(-12.4230808101438,22.8400320311648,
12.));
#242442=CARTESIAN_POINT('Ctrl Pts',(-12.418215285186,22.8370364396459,0.));
#242443=CARTESIAN_POINT('Ctrl Pts',(-12.418215285186,22.8370364396459,12.));
#242444=CARTESIAN_POINT('Ctrl Pts',(-12.4084933766347,22.8310435872747,
0.));
#242445=CARTESIAN_POINT('Ctrl Pts',(-12.4084933766347,22.8310435872747,
12.));
#242446=CARTESIAN_POINT('Ctrl Pts',(-12.3939379378998,22.8220493007173,
0.));
#242447=CARTESIAN_POINT('Ctrl Pts',(-12.3939379378998,22.8220493007173,
12.));
#242448=CARTESIAN_POINT('Ctrl Pts',(-12.374585536673,22.81004690224,0.));
#242449=CARTESIAN_POINT('Ctrl Pts',(-12.374585536673,22.81004690224,12.));
#242450=CARTESIAN_POINT('Ctrl Pts',(-12.3504864740319,22.795027221673,0.));
#242451=CARTESIAN_POINT('Ctrl Pts',(-12.3504864740319,22.795027221673,12.));
#242452=CARTESIAN_POINT('Ctrl Pts',(-12.3264788926075,22.7799908974768,
0.));
#242453=CARTESIAN_POINT('Ctrl Pts',(-12.3264788926075,22.7799908974768,
12.));
#242454=CARTESIAN_POINT('Ctrl Pts',(-12.3025628601792,22.764938010105,0.));
#242455=CARTESIAN_POINT('Ctrl Pts',(-12.3025628601792,22.764938010105,12.));
#242456=CARTESIAN_POINT('Ctrl Pts',(-12.2787384750742,22.7498686970069,
0.));
#242457=CARTESIAN_POINT('Ctrl Pts',(-12.2787384750742,22.7498686970069,
12.));
#242458=CARTESIAN_POINT('Ctrl Pts',(-12.2550058702395,22.7347831655287,
0.));
#242459=CARTESIAN_POINT('Ctrl Pts',(-12.2550058702395,22.7347831655287,
12.));
#242460=CARTESIAN_POINT('Ctrl Pts',(-12.2313652198061,22.7196817119374,
0.));
#242461=CARTESIAN_POINT('Ctrl Pts',(-12.2313652198061,22.7196817119374,
12.));
#242462=CARTESIAN_POINT('Ctrl Pts',(-12.2078167360284,22.7045647168747,
0.));
#242463=CARTESIAN_POINT('Ctrl Pts',(-12.2078167360284,22.7045647168747,
12.));
#242464=CARTESIAN_POINT('Ctrl Pts',(-12.1843606579262,22.6894326205037,
0.));
#242465=CARTESIAN_POINT('Ctrl Pts',(-12.1843606579262,22.6894326205037,
12.));
#242466=CARTESIAN_POINT('Ctrl Pts',(-12.1609972423099,22.6742859034944,
0.));
#242467=CARTESIAN_POINT('Ctrl Pts',(-12.1609972423099,22.6742859034944,
12.));
#242468=CARTESIAN_POINT('Ctrl Pts',(-12.1377267537145,22.6591250653965,
0.));
#242469=CARTESIAN_POINT('Ctrl Pts',(-12.1377267537145,22.6591250653965,
12.));
#242470=CARTESIAN_POINT('Ctrl Pts',(-12.1145494550383,22.6439506046605,
0.));
#242471=CARTESIAN_POINT('Ctrl Pts',(-12.1145494550383,22.6439506046605,
12.));
#242472=CARTESIAN_POINT('Ctrl Pts',(-12.0914655972823,22.6287629967056,
0.));
#242473=CARTESIAN_POINT('Ctrl Pts',(-12.0914655972823,22.6287629967056,
12.));
#242474=CARTESIAN_POINT('Ctrl Pts',(-12.0684754113862,22.6135626764898,
0.));
#242475=CARTESIAN_POINT('Ctrl Pts',(-12.0684754113862,22.6135626764898,
12.));
#242476=CARTESIAN_POINT('Ctrl Pts',(-12.0455791139128,22.5983500505644,
0.));
#242477=CARTESIAN_POINT('Ctrl Pts',(-12.0455791139128,22.5983500505644,
12.));
#242478=CARTESIAN_POINT('Ctrl Pts',(-12.0227769113127,22.5831255061282,
0.));
#242479=CARTESIAN_POINT('Ctrl Pts',(-12.0227769113127,22.5831255061282,
12.));
#242480=CARTESIAN_POINT('Ctrl Pts',(-12.0000690046695,22.5678894211181,
0.));
#242481=CARTESIAN_POINT('Ctrl Pts',(-12.0000690046695,22.5678894211181,
12.));
#242482=CARTESIAN_POINT('Ctrl Pts',(-11.9774555943496,22.5526421741158,
0.));
#242483=CARTESIAN_POINT('Ctrl Pts',(-11.9774555943496,22.5526421741158,
12.));
#242484=CARTESIAN_POINT('Ctrl Pts',(-11.9549368843997,22.5373841537307,
0.));
#242485=CARTESIAN_POINT('Ctrl Pts',(-11.9549368843997,22.5373841537307,
12.));
#242486=CARTESIAN_POINT('Ctrl Pts',(-11.9325130877803,22.5221157697883,
0.));
#242487=CARTESIAN_POINT('Ctrl Pts',(-11.9325130877803,22.5221157697883,
12.));
#242488=CARTESIAN_POINT('Ctrl Pts',(-11.9101844254557,22.5068374513973,
0.));
#242489=CARTESIAN_POINT('Ctrl Pts',(-11.9101844254557,22.5068374513973,
12.));
#242490=CARTESIAN_POINT('Ctrl Pts',(-11.8879511239943,22.4915496418485,
0.));
#242491=CARTESIAN_POINT('Ctrl Pts',(-11.8879511239943,22.4915496418485,
12.));
#242492=CARTESIAN_POINT('Ctrl Pts',(-11.8658134137019,22.4762527946702,
0.));
#242493=CARTESIAN_POINT('Ctrl Pts',(-11.8658134137019,22.4762527946702,
12.));
#242494=CARTESIAN_POINT('Ctrl Pts',(-11.8437715264487,22.4609473690471,
0.));
#242495=CARTESIAN_POINT('Ctrl Pts',(-11.8437715264487,22.4609473690471,
12.));
#242496=CARTESIAN_POINT('Ctrl Pts',(-11.8218256937889,22.4456338258735,
0.));
#242497=CARTESIAN_POINT('Ctrl Pts',(-11.8218256937889,22.4456338258735,
12.));
#242498=CARTESIAN_POINT('Ctrl Pts',(-11.7999761445173,22.430312622646,0.));
#242499=CARTESIAN_POINT('Ctrl Pts',(-11.7999761445173,22.430312622646,12.));
#242500=CARTESIAN_POINT('Ctrl Pts',(-11.7782231042039,22.4149842125008,
0.));
#242501=CARTESIAN_POINT('Ctrl Pts',(-11.7782231042039,22.4149842125008,
12.));
#242502=CARTESIAN_POINT('Ctrl Pts',(-11.7565667964764,22.3996490469191,
0.));
#242503=CARTESIAN_POINT('Ctrl Pts',(-11.7565667964764,22.3996490469191,
12.));
#242504=CARTESIAN_POINT('Ctrl Pts',(-11.7350074437961,22.3843075773899,
0.));
#242505=CARTESIAN_POINT('Ctrl Pts',(-11.7350074437961,22.3843075773899,
12.));
#242506=CARTESIAN_POINT('Ctrl Pts',(-11.7135452684532,22.3689602575491,
0.));
#242507=CARTESIAN_POINT('Ctrl Pts',(-11.7135452684532,22.3689602575491,
12.));
#242508=CARTESIAN_POINT('Ctrl Pts',(-11.6921804934056,22.3536075450029,
0.));
#242509=CARTESIAN_POINT('Ctrl Pts',(-11.6921804934056,22.3536075450029,
12.));
#242510=CARTESIAN_POINT('Ctrl Pts',(-11.6709133432985,22.3382499035619,
0.));
#242511=CARTESIAN_POINT('Ctrl Pts',(-11.6709133432985,22.3382499035619,
12.));
#242512=CARTESIAN_POINT('Ctrl Pts',(-11.6497440449857,22.3228878043976,
0.));
#242513=CARTESIAN_POINT('Ctrl Pts',(-11.6497440449857,22.3228878043976,
12.));
#242514=CARTESIAN_POINT('Ctrl Pts',(-11.6286728270009,22.3075217249049,
0.));
#242515=CARTESIAN_POINT('Ctrl Pts',(-11.6286728270009,22.3075217249049,
12.));
#242516=CARTESIAN_POINT('Ctrl Pts',(-11.6076999192357,22.2921521480356,
0.));
#242517=CARTESIAN_POINT('Ctrl Pts',(-11.6076999192357,22.2921521480356,
12.));
#242518=CARTESIAN_POINT('Ctrl Pts',(-11.5868255525188,22.2767795614348,
0.));
#242519=CARTESIAN_POINT('Ctrl Pts',(-11.5868255525188,22.2767795614348,
12.));
#242520=CARTESIAN_POINT('Ctrl Pts',(-11.5660499582403,22.2614044566898,
0.));
#242521=CARTESIAN_POINT('Ctrl Pts',(-11.5660499582403,22.2614044566898,
12.));
#242522=CARTESIAN_POINT('Ctrl Pts',(-11.5453733679121,22.2460273284654,
0.));
#242523=CARTESIAN_POINT('Ctrl Pts',(-11.5453733679121,22.2460273284654,
12.));
#242524=CARTESIAN_POINT('Ctrl Pts',(-11.5247960128477,22.2306486738901,
0.));
#242525=CARTESIAN_POINT('Ctrl Pts',(-11.5247960128477,22.2306486738901,
12.));
#242526=CARTESIAN_POINT('Ctrl Pts',(-11.5043181244242,22.2152689931022,
0.));
#242527=CARTESIAN_POINT('Ctrl Pts',(-11.5043181244242,22.2152689931022,
12.));
#242528=CARTESIAN_POINT('Ctrl Pts',(-11.483939934259,22.1998887896436,0.));
#242529=CARTESIAN_POINT('Ctrl Pts',(-11.483939934259,22.1998887896436,12.));
#242530=CARTESIAN_POINT('Ctrl Pts',(-11.463661674411,22.184508570917,0.));
#242531=CARTESIAN_POINT('Ctrl Pts',(-11.463661674411,22.184508570917,12.));
#242532=CARTESIAN_POINT('Ctrl Pts',(-11.443483577557,22.1691288486096,0.));
#242533=CARTESIAN_POINT('Ctrl Pts',(-11.443483577557,22.1691288486096,12.));
#242534=CARTESIAN_POINT('Ctrl Pts',(-11.4234058771742,22.1537501391487,
0.));
#242535=CARTESIAN_POINT('Ctrl Pts',(-11.4234058771742,22.1537501391487,
12.));
#242536=CARTESIAN_POINT('Ctrl Pts',(-11.4034288076908,22.1383729640964,
0.));
#242537=CARTESIAN_POINT('Ctrl Pts',(-11.4034288076908,22.1383729640964,
12.));
#242538=CARTESIAN_POINT('Ctrl Pts',(-11.3835526044256,22.1229978500186,
0.));
#242539=CARTESIAN_POINT('Ctrl Pts',(-11.3835526044256,22.1229978500186,
12.));
#242540=CARTESIAN_POINT('Ctrl Pts',(-11.3637775035367,22.1076253283979,
0.));
#242541=CARTESIAN_POINT('Ctrl Pts',(-11.3637775035367,22.1076253283979,
12.));
#242542=CARTESIAN_POINT('Ctrl Pts',(-11.3441037419553,22.0922559355294,
0.));
#242543=CARTESIAN_POINT('Ctrl Pts',(-11.3441037419553,22.0922559355294,
12.));
#242544=CARTESIAN_POINT('Ctrl Pts',(-11.3245315573168,22.0768902124267,
0.));
#242545=CARTESIAN_POINT('Ctrl Pts',(-11.3245315573168,22.0768902124267,
12.));
#242546=CARTESIAN_POINT('Ctrl Pts',(-11.3050611878771,22.0615287047179,
0.));
#242547=CARTESIAN_POINT('Ctrl Pts',(-11.3050611878771,22.0615287047179,
12.));
#242548=CARTESIAN_POINT('Ctrl Pts',(-11.2856928724374,22.046171962566,0.));
#242549=CARTESIAN_POINT('Ctrl Pts',(-11.2856928724374,22.046171962566,12.));
#242550=CARTESIAN_POINT('Ctrl Pts',(-11.2664268504206,22.030820540835,0.));
#242551=CARTESIAN_POINT('Ctrl Pts',(-11.2664268504206,22.030820540835,12.));
#242552=CARTESIAN_POINT('Ctrl Pts',(-11.2472633619275,22.0154749992363,
0.));
#242553=CARTESIAN_POINT('Ctrl Pts',(-11.2472633619275,22.0154749992363,
12.));
#242554=CARTESIAN_POINT('Ctrl Pts',(-11.2282026477896,22.0001359024839,
0.));
#242555=CARTESIAN_POINT('Ctrl Pts',(-11.2282026477896,22.0001359024839,
12.));
#242556=CARTESIAN_POINT('Ctrl Pts',(-11.2092449496125,21.9848038204439,
0.));
#242557=CARTESIAN_POINT('Ctrl Pts',(-11.2092449496125,21.9848038204439,
12.));
#242558=CARTESIAN_POINT('Ctrl Pts',(-11.190390509811,21.9694793282914,0.));
#242559=CARTESIAN_POINT('Ctrl Pts',(-11.190390509811,21.9694793282914,12.));
#242560=CARTESIAN_POINT('Ctrl Pts',(-11.1716395716376,21.9541630066506,
0.));
#242561=CARTESIAN_POINT('Ctrl Pts',(-11.1716395716376,21.9541630066506,
12.));
#242562=CARTESIAN_POINT('Ctrl Pts',(-11.1529923792003,21.9388554416439,
0.));
#242563=CARTESIAN_POINT('Ctrl Pts',(-11.1529923792003,21.9388554416439,
12.));
#242564=CARTESIAN_POINT('Ctrl Pts',(-11.1344491774741,21.923557224952,0.));
#242565=CARTESIAN_POINT('Ctrl Pts',(-11.1344491774741,21.923557224952,12.));
#242566=CARTESIAN_POINT('Ctrl Pts',(-11.1160102123024,21.9082689538688,
0.));
#242567=CARTESIAN_POINT('Ctrl Pts',(-11.1160102123024,21.9082689538688,
12.));
#242568=CARTESIAN_POINT('Ctrl Pts',(-11.0976757303944,21.8929912313608,
0.));
#242569=CARTESIAN_POINT('Ctrl Pts',(-11.0976757303944,21.8929912313608,
12.));
#242570=CARTESIAN_POINT('Ctrl Pts',(-11.0794459793057,21.877724666119,0.));
#242571=CARTESIAN_POINT('Ctrl Pts',(-11.0794459793057,21.877724666119,12.));
#242572=CARTESIAN_POINT('Ctrl Pts',(-11.0613212074363,21.8624698726318,
0.));
#242573=CARTESIAN_POINT('Ctrl Pts',(-11.0613212074363,21.8624698726318,
12.));
#242574=CARTESIAN_POINT('Ctrl Pts',(-11.0433016640807,21.8472274713103,
0.));
#242575=CARTESIAN_POINT('Ctrl Pts',(-11.0433016640807,21.8472274713103,
12.));
#242576=CARTESIAN_POINT('Ctrl Pts',(-11.0253875994598,21.8319980886033,
0.));
#242577=CARTESIAN_POINT('Ctrl Pts',(-11.0253875994598,21.8319980886033,
12.));
#242578=CARTESIAN_POINT('Ctrl Pts',(-11.0075792647477,21.8167823571168,
0.));
#242579=CARTESIAN_POINT('Ctrl Pts',(-11.0075792647477,21.8167823571168,
12.));
#242580=CARTESIAN_POINT('Ctrl Pts',(-10.9898769120912,21.8015809157301,
0.));
#242581=CARTESIAN_POINT('Ctrl Pts',(-10.9898769120912,21.8015809157301,
12.));
#242582=CARTESIAN_POINT('Ctrl Pts',(-10.9722807946156,21.7863944097141,
0.));
#242583=CARTESIAN_POINT('Ctrl Pts',(-10.9722807946156,21.7863944097141,
12.));
#242584=CARTESIAN_POINT('Ctrl Pts',(-10.9547911664455,21.7712234908464,
0.));
#242585=CARTESIAN_POINT('Ctrl Pts',(-10.9547911664455,21.7712234908464,
12.));
#242586=CARTESIAN_POINT('Ctrl Pts',(-10.9374082827444,21.7560688175247,
0.));
#242587=CARTESIAN_POINT('Ctrl Pts',(-10.9374082827444,21.7560688175247,
12.));
#242588=CARTESIAN_POINT('Ctrl Pts',(-10.9201323997384,21.7409310548797,
0.));
#242589=CARTESIAN_POINT('Ctrl Pts',(-10.9201323997384,21.7409310548797,
12.));
#242590=CARTESIAN_POINT('Ctrl Pts',(-10.902963774734,21.7258108748873,0.));
#242591=CARTESIAN_POINT('Ctrl Pts',(-10.902963774734,21.7258108748873,12.));
#242592=CARTESIAN_POINT('Ctrl Pts',(-10.8859026661293,21.7107089564825,
0.));
#242593=CARTESIAN_POINT('Ctrl Pts',(-10.8859026661293,21.7107089564825,
12.));
#242594=CARTESIAN_POINT('Ctrl Pts',(-10.8689493334095,21.6956259856672,
0.));
#242595=CARTESIAN_POINT('Ctrl Pts',(-10.8689493334095,21.6956259856672,
12.));
#242596=CARTESIAN_POINT('Ctrl Pts',(-10.8521040371835,21.6805626556467,
0.));
#242597=CARTESIAN_POINT('Ctrl Pts',(-10.8521040371835,21.6805626556467,
12.));
#242598=CARTESIAN_POINT('Ctrl Pts',(-10.8353670392272,21.6655196669732,
0.));
#242599=CARTESIAN_POINT('Ctrl Pts',(-10.8353670392272,21.6655196669732,
12.));
#242600=CARTESIAN_POINT('Ctrl Pts',(-10.8187386025136,21.6504977276866,
0.));
#242601=CARTESIAN_POINT('Ctrl Pts',(-10.8187386025136,21.6504977276866,
12.));
#242602=CARTESIAN_POINT('Ctrl Pts',(-10.8022189912369,21.6354975534557,
0.));
#242603=CARTESIAN_POINT('Ctrl Pts',(-10.8022189912369,21.6354975534557,
12.));
#242604=CARTESIAN_POINT('Ctrl Pts',(-10.7858084708261,21.6205198677173,
0.));
#242605=CARTESIAN_POINT('Ctrl Pts',(-10.7858084708261,21.6205198677173,
12.));
#242606=CARTESIAN_POINT('Ctrl Pts',(-10.7695073079552,21.6055654018176,
0.));
#242607=CARTESIAN_POINT('Ctrl Pts',(-10.7695073079552,21.6055654018176,
12.));
#242608=CARTESIAN_POINT('Ctrl Pts',(-10.7533157705941,21.5906348951743,
0.));
#242609=CARTESIAN_POINT('Ctrl Pts',(-10.7533157705941,21.5906348951743,
12.));
#242610=CARTESIAN_POINT('Ctrl Pts',(-10.7372341280467,21.5757290954371,
0.));
#242611=CARTESIAN_POINT('Ctrl Pts',(-10.7372341280467,21.5757290954371,
12.));
#242612=CARTESIAN_POINT('Ctrl Pts',(-10.7212626509816,21.5608487586468,
0.));
#242613=CARTESIAN_POINT('Ctrl Pts',(-10.7212626509816,21.5608487586468,
12.));
#242614=CARTESIAN_POINT('Ctrl Pts',(-10.7054016114571,21.5459946493955,
0.));
#242615=CARTESIAN_POINT('Ctrl Pts',(-10.7054016114571,21.5459946493955,
12.));
#242616=CARTESIAN_POINT('Ctrl Pts',(-10.689651282929,21.5311675409807,0.));
#242617=CARTESIAN_POINT('Ctrl Pts',(-10.689651282929,21.5311675409807,12.));
#242618=CARTESIAN_POINT('Ctrl Pts',(-10.6740119402834,21.51636821558,0.));
#242619=CARTESIAN_POINT('Ctrl Pts',(-10.6740119402834,21.51636821558,12.));
#242620=CARTESIAN_POINT('Ctrl Pts',(-10.6584838598939,21.5015974644449,
0.));
#242621=CARTESIAN_POINT('Ctrl Pts',(-10.6584838598939,21.5015974644449,
12.));
#242622=CARTESIAN_POINT('Ctrl Pts',(-10.6430673196607,21.4868560880889,
0.));
#242623=CARTESIAN_POINT('Ctrl Pts',(-10.6430673196607,21.4868560880889,
12.));
#242624=CARTESIAN_POINT('Ctrl Pts',(-10.6277625990456,21.4721448964766,
0.));
#242625=CARTESIAN_POINT('Ctrl Pts',(-10.6277625990456,21.4721448964766,
12.));
#242626=CARTESIAN_POINT('Ctrl Pts',(-10.6125699790961,21.4574647092097,
0.));
#242627=CARTESIAN_POINT('Ctrl Pts',(-10.6125699790961,21.4574647092097,
12.));
#242628=CARTESIAN_POINT('Ctrl Pts',(-10.5974897424622,21.4428163557144,
0.));
#242629=CARTESIAN_POINT('Ctrl Pts',(-10.5974897424622,21.4428163557144,
12.));
#242630=CARTESIAN_POINT('Ctrl Pts',(-10.5825221734573,21.4282006754631,
0.));
#242631=CARTESIAN_POINT('Ctrl Pts',(-10.5825221734573,21.4282006754631,
12.));
#242632=CARTESIAN_POINT('Ctrl Pts',(-10.5676675581108,21.4136185181979,
0.));
#242633=CARTESIAN_POINT('Ctrl Pts',(-10.5676675581108,21.4136185181979,
12.));
#242634=CARTESIAN_POINT('Ctrl Pts',(-10.5529261842108,21.3990707441497,
0.));
#242635=CARTESIAN_POINT('Ctrl Pts',(-10.5529261842108,21.3990707441497,
12.));
#242636=CARTESIAN_POINT('Ctrl Pts',(-10.5382983413421,21.3845582242602,
0.));
#242637=CARTESIAN_POINT('Ctrl Pts',(-10.5382983413421,21.3845582242602,
12.));
#242638=CARTESIAN_POINT('Ctrl Pts',(-10.5237843209057,21.3700818403936,
0.));
#242639=CARTESIAN_POINT('Ctrl Pts',(-10.5237843209057,21.3700818403936,
12.));
#242640=CARTESIAN_POINT('Ctrl Pts',(-10.5093844161685,21.3556424855814,
0.));
#242641=CARTESIAN_POINT('Ctrl Pts',(-10.5093844161685,21.3556424855814,
12.));
#242642=CARTESIAN_POINT('Ctrl Pts',(-10.4950989223337,21.3412410642904,
0.));
#242643=CARTESIAN_POINT('Ctrl Pts',(-10.4950989223337,21.3412410642904,
12.));
#242644=CARTESIAN_POINT('Ctrl Pts',(-10.4809281365931,21.3268784926819,
0.));
#242645=CARTESIAN_POINT('Ctrl Pts',(-10.4809281365931,21.3268784926819,
12.));
#242646=CARTESIAN_POINT('Ctrl Pts',(-10.4668723581768,21.3125556988731,
0.));
#242647=CARTESIAN_POINT('Ctrl Pts',(-10.4668723581768,21.3125556988731,
12.));
#242648=CARTESIAN_POINT('Ctrl Pts',(-10.4529318883874,21.2982736231931,
0.));
#242649=CARTESIAN_POINT('Ctrl Pts',(-10.4529318883874,21.2982736231931,
12.));
#242650=CARTESIAN_POINT('Ctrl Pts',(-10.4391070306391,21.2840332184483,
0.));
#242651=CARTESIAN_POINT('Ctrl Pts',(-10.4391070306391,21.2840332184483,
12.));
#242652=CARTESIAN_POINT('Ctrl Pts',(-10.42539809054,21.2698354502403,0.));
#242653=CARTESIAN_POINT('Ctrl Pts',(-10.42539809054,21.2698354502403,12.));
#242654=CARTESIAN_POINT('Ctrl Pts',(-10.4118053759588,21.255681297275,0.));
#242655=CARTESIAN_POINT('Ctrl Pts',(-10.4118053759588,21.255681297275,12.));
#242656=CARTESIAN_POINT('Ctrl Pts',(-10.3983291970846,21.2415717516714,
0.));
#242657=CARTESIAN_POINT('Ctrl Pts',(-10.3983291970846,21.2415717516714,
12.));
#242658=CARTESIAN_POINT('Ctrl Pts',(-10.3849698664786,21.22750781927,0.));
#242659=CARTESIAN_POINT('Ctrl Pts',(-10.3849698664786,21.22750781927,12.));
#242660=CARTESIAN_POINT('Ctrl Pts',(-10.371727699113,21.2134905199345,0.));
#242661=CARTESIAN_POINT('Ctrl Pts',(-10.371727699113,21.2134905199345,12.));
#242662=CARTESIAN_POINT('Ctrl Pts',(-10.3586030124587,21.199520887919,0.));
#242663=CARTESIAN_POINT('Ctrl Pts',(-10.3586030124587,21.199520887919,12.));
#242664=CARTESIAN_POINT('Ctrl Pts',(-10.3455961265701,21.1855999722416,
0.));
#242665=CARTESIAN_POINT('Ctrl Pts',(-10.3455961265701,21.1855999722416,
12.));
#242666=CARTESIAN_POINT('Ctrl Pts',(-10.3327073641572,21.1717288370509,
0.));
#242667=CARTESIAN_POINT('Ctrl Pts',(-10.3327073641572,21.1717288370509,
12.));
#242668=CARTESIAN_POINT('Ctrl Pts',(-10.3199370506544,21.1579085619965,
0.));
#242669=CARTESIAN_POINT('Ctrl Pts',(-10.3199370506544,21.1579085619965,
12.));
#242670=CARTESIAN_POINT('Ctrl Pts',(-10.3072855142687,21.1441402425843,
0.));
#242671=CARTESIAN_POINT('Ctrl Pts',(-10.3072855142687,21.1441402425843,
12.));
#242672=CARTESIAN_POINT('Ctrl Pts',(-10.2947530860721,21.1304249906002,
0.));
#242673=CARTESIAN_POINT('Ctrl Pts',(-10.2947530860721,21.1304249906002,
12.));
#242674=CARTESIAN_POINT('Ctrl Pts',(-10.2823401001072,21.1167639345631,
0.));
#242675=CARTESIAN_POINT('Ctrl Pts',(-10.2823401001072,21.1167639345631,
12.));
#242676=CARTESIAN_POINT('Ctrl Pts',(-10.2700468934744,21.1031582201627,
0.));
#242677=CARTESIAN_POINT('Ctrl Pts',(-10.2700468934744,21.1031582201627,
12.));
#242678=CARTESIAN_POINT('Ctrl Pts',(-10.2578738064181,21.0896090107063,
0.));
#242679=CARTESIAN_POINT('Ctrl Pts',(-10.2578738064181,21.0896090107063,
12.));
#242680=CARTESIAN_POINT('Ctrl Pts',(-10.2458211823912,21.0761174875445,
0.));
#242681=CARTESIAN_POINT('Ctrl Pts',(-10.2458211823912,21.0761174875445,
12.));
#242682=CARTESIAN_POINT('Ctrl Pts',(-10.2338893681567,21.0626848505663,
0.));
#242683=CARTESIAN_POINT('Ctrl Pts',(-10.2338893681567,21.0626848505663,
12.));
#242684=CARTESIAN_POINT('Ctrl Pts',(-10.2220787139155,21.0493123187483,
0.));
#242685=CARTESIAN_POINT('Ctrl Pts',(-10.2220787139155,21.0493123187483,
12.));
#242686=CARTESIAN_POINT('Ctrl Pts',(-10.2103895734123,21.0360011306815,
0.));
#242687=CARTESIAN_POINT('Ctrl Pts',(-10.2103895734123,21.0360011306815,
12.));
#242688=CARTESIAN_POINT('Ctrl Pts',(-10.1988223040425,21.0227525451107,
0.));
#242689=CARTESIAN_POINT('Ctrl Pts',(-10.1988223040425,21.0227525451107,
12.));
#242690=CARTESIAN_POINT('Ctrl Pts',(-10.187377266936,21.0095678414486,0.));
#242691=CARTESIAN_POINT('Ctrl Pts',(-10.187377266936,21.0095678414486,12.));
#242692=CARTESIAN_POINT('Ctrl Pts',(-10.1760548270767,20.9964483203686,
0.));
#242693=CARTESIAN_POINT('Ctrl Pts',(-10.1760548270767,20.9964483203686,
12.));
#242694=CARTESIAN_POINT('Ctrl Pts',(-10.1648553534568,20.9833953044736,
0.));
#242695=CARTESIAN_POINT('Ctrl Pts',(-10.1648553534568,20.9833953044736,
12.));
#242696=CARTESIAN_POINT('Ctrl Pts',(-10.1537792192065,20.9704101389369,
0.));
#242697=CARTESIAN_POINT('Ctrl Pts',(-10.1537792192065,20.9704101389369,
12.));
#242698=CARTESIAN_POINT('Ctrl Pts',(-10.1428268017256,20.9574941921591,
0.));
#242699=CARTESIAN_POINT('Ctrl Pts',(-10.1428268017256,20.9574941921591,
12.));
#242700=CARTESIAN_POINT('Ctrl Pts',(-10.1319984827908,20.9446488563933,
0.));
#242701=CARTESIAN_POINT('Ctrl Pts',(-10.1319984827908,20.9446488563933,
12.));
#242702=CARTESIAN_POINT('Ctrl Pts',(-10.1212946487057,20.9318755484734,
0.));
#242703=CARTESIAN_POINT('Ctrl Pts',(-10.1212946487057,20.9318755484734,
12.));
#242704=CARTESIAN_POINT('Ctrl Pts',(-10.1107156904836,20.919175710627,0.));
#242705=CARTESIAN_POINT('Ctrl Pts',(-10.1107156904836,20.919175710627,12.));
#242706=CARTESIAN_POINT('Ctrl Pts',(-10.1002620040076,20.9065508112557,
0.));
#242707=CARTESIAN_POINT('Ctrl Pts',(-10.1002620040076,20.9065508112557,
12.));
#242708=CARTESIAN_POINT('Ctrl Pts',(-10.0899339901916,20.894002345737,0.));
#242709=CARTESIAN_POINT('Ctrl Pts',(-10.0899339901916,20.894002345737,12.));
#242710=CARTESIAN_POINT('Ctrl Pts',(-10.0797320551154,20.881531837184,0.));
#242711=CARTESIAN_POINT('Ctrl Pts',(-10.0797320551154,20.881531837184,12.));
#242712=CARTESIAN_POINT('Ctrl Pts',(-10.0696566102218,20.86914083737,0.));
#242713=CARTESIAN_POINT('Ctrl Pts',(-10.0696566102218,20.86914083737,12.));
#242714=CARTESIAN_POINT('Ctrl Pts',(-10.0597080725375,20.8568309277316,
0.));
#242715=CARTESIAN_POINT('Ctrl Pts',(-10.0597080725375,20.8568309277316,
12.));
#242716=CARTESIAN_POINT('Ctrl Pts',(-10.0498868648733,20.8446037203402,
0.));
#242717=CARTESIAN_POINT('Ctrl Pts',(-10.0498868648733,20.8446037203402,
12.));
#242718=CARTESIAN_POINT('Ctrl Pts',(-10.0401934160234,20.8324608588909,
0.));
#242719=CARTESIAN_POINT('Ctrl Pts',(-10.0401934160234,20.8324608588909,
12.));
#242720=CARTESIAN_POINT('Ctrl Pts',(-10.0306281609435,20.8204040196602,
0.));
#242721=CARTESIAN_POINT('Ctrl Pts',(-10.0306281609435,20.8204040196602,
12.));
#242722=CARTESIAN_POINT('Ctrl Pts',(-10.0211915410095,20.8084349126888,
0.));
#242723=CARTESIAN_POINT('Ctrl Pts',(-10.0211915410095,20.8084349126888,
12.));
#242724=CARTESIAN_POINT('Ctrl Pts',(-10.0118840042786,20.7965552829908,
0.));
#242725=CARTESIAN_POINT('Ctrl Pts',(-10.0118840042786,20.7965552829908,
12.));
#242726=CARTESIAN_POINT('Ctrl Pts',(-10.0027060057389,20.7847669117568,
0.));
#242727=CARTESIAN_POINT('Ctrl Pts',(-10.0027060057389,20.7847669117568,
12.));
#242728=CARTESIAN_POINT('Ctrl Pts',(-9.9936580075464,20.7730716175417,0.));
#242729=CARTESIAN_POINT('Ctrl Pts',(-9.9936580075464,20.7730716175417,12.));
#242730=CARTESIAN_POINT('Ctrl Pts',(-9.98474047926852,20.761471257499,0.));
#242731=CARTESIAN_POINT('Ctrl Pts',(-9.98474047926852,20.761471257499,12.));
#242732=CARTESIAN_POINT('Ctrl Pts',(-9.9759538982347,20.7499677289627,0.));
#242733=CARTESIAN_POINT('Ctrl Pts',(-9.9759538982347,20.7499677289627,12.));
#242734=CARTESIAN_POINT('Ctrl Pts',(-9.96729874986202,20.7385629709795,
0.));
#242735=CARTESIAN_POINT('Ctrl Pts',(-9.96729874986202,20.7385629709795,
12.));
#242736=CARTESIAN_POINT('Ctrl Pts',(-9.95877552798398,20.7272589658751,
0.));
#242737=CARTESIAN_POINT('Ctrl Pts',(-9.95877552798398,20.7272589658751,
12.));
#242738=CARTESIAN_POINT('Ctrl Pts',(-9.95038473514949,20.7160577407579,
0.));
#242739=CARTESIAN_POINT('Ctrl Pts',(-9.95038473514949,20.7160577407579,
12.));
#242740=CARTESIAN_POINT('Ctrl Pts',(-9.94212688298236,20.7049613692234,
0.));
#242741=CARTESIAN_POINT('Ctrl Pts',(-9.94212688298236,20.7049613692234,
12.));
#242742=CARTESIAN_POINT('Ctrl Pts',(-9.9340024925973,20.6939719732484,0.));
#242743=CARTESIAN_POINT('Ctrl Pts',(-9.9340024925973,20.6939719732484,12.));
#242744=CARTESIAN_POINT('Ctrl Pts',(-9.92601209498749,20.6830917250255,
0.));
#242745=CARTESIAN_POINT('Ctrl Pts',(-9.92601209498749,20.6830917250255,
12.));
#242746=CARTESIAN_POINT('Ctrl Pts',(-9.91815623141289,20.6723228488263,
0.));
#242747=CARTESIAN_POINT('Ctrl Pts',(-9.91815623141289,20.6723228488263,
12.));
#242748=CARTESIAN_POINT('Ctrl Pts',(-9.91043545377007,20.6616676228315,
0.));
#242749=CARTESIAN_POINT('Ctrl Pts',(-9.91043545377007,20.6616676228315,
12.));
#242750=CARTESIAN_POINT('Ctrl Pts',(-9.90285032516693,20.6511283817414,
0.));
#242751=CARTESIAN_POINT('Ctrl Pts',(-9.90285032516693,20.6511283817414,
12.));
#242752=CARTESIAN_POINT('Ctrl Pts',(-9.8954014204912,20.6407075193976,0.));
#242753=CARTESIAN_POINT('Ctrl Pts',(-9.8954014204912,20.6407075193976,12.));
#242754=CARTESIAN_POINT('Ctrl Pts',(-9.88808932697306,20.6304074914087,
0.));
#242755=CARTESIAN_POINT('Ctrl Pts',(-9.88808932697306,20.6304074914087,
12.));
#242756=CARTESIAN_POINT('Ctrl Pts',(-9.88091464472676,20.6202308177474,
0.));
#242757=CARTESIAN_POINT('Ctrl Pts',(-9.88091464472676,20.6202308177474,
12.));
#242758=CARTESIAN_POINT('Ctrl Pts',(-9.87387798732956,20.6101800854494,
0.));
#242759=CARTESIAN_POINT('Ctrl Pts',(-9.87387798732956,20.6101800854494,
12.));
#242760=CARTESIAN_POINT('Ctrl Pts',(-9.86697998242623,20.6002579513699,
0.));
#242761=CARTESIAN_POINT('Ctrl Pts',(-9.86697998242623,20.6002579513699,
12.));
#242762=CARTESIAN_POINT('Ctrl Pts',(-9.86022127232748,20.5904671449754,
0.));
#242763=CARTESIAN_POINT('Ctrl Pts',(-9.86022127232748,20.5904671449754,
12.));
#242764=CARTESIAN_POINT('Ctrl Pts',(-9.85360251456981,20.5808104710015,
0.));
#242765=CARTESIAN_POINT('Ctrl Pts',(-9.85360251456981,20.5808104710015,
12.));
#242766=CARTESIAN_POINT('Ctrl Pts',(-9.84712438256278,20.5712908125139,
0.));
#242767=CARTESIAN_POINT('Ctrl Pts',(-9.84712438256278,20.5712908125139,
12.));
#242768=CARTESIAN_POINT('Ctrl Pts',(-9.84078756677565,20.5619111362402,
0.));
#242769=CARTESIAN_POINT('Ctrl Pts',(-9.84078756677565,20.5619111362402,
12.));
#242770=CARTESIAN_POINT('Ctrl Pts',(-9.83459277585315,20.552674497646,0.));
#242771=CARTESIAN_POINT('Ctrl Pts',(-9.83459277585315,20.552674497646,12.));
#242772=CARTESIAN_POINT('Ctrl Pts',(-9.82854073773877,20.5435840460721,
0.));
#242773=CARTESIAN_POINT('Ctrl Pts',(-9.82854073773877,20.5435840460721,
12.));
#242774=CARTESIAN_POINT('Ctrl Pts',(-9.82263220080363,20.5346430299517,
0.));
#242775=CARTESIAN_POINT('Ctrl Pts',(-9.82263220080363,20.5346430299517,
12.));
#242776=CARTESIAN_POINT('Ctrl Pts',(-9.81686793455943,20.5258548000629,
0.));
#242777=CARTESIAN_POINT('Ctrl Pts',(-9.81686793455943,20.5258548000629,
12.));
#242778=CARTESIAN_POINT('Ctrl Pts',(-9.81124873025282,20.517222812284,0.));
#242779=CARTESIAN_POINT('Ctrl Pts',(-9.81124873025282,20.517222812284,12.));
#242780=CARTESIAN_POINT('Ctrl Pts',(-9.80577540161088,20.5087506310505,
0.));
#242781=CARTESIAN_POINT('Ctrl Pts',(-9.80577540161088,20.5087506310505,
12.));
#242782=CARTESIAN_POINT('Ctrl Pts',(-9.80044878520949,20.5004419312107,
0.));
#242783=CARTESIAN_POINT('Ctrl Pts',(-9.80044878520949,20.5004419312107,
12.));
#242784=CARTESIAN_POINT('Ctrl Pts',(-9.79526974288331,20.4923005087943,
0.));
#242785=CARTESIAN_POINT('Ctrl Pts',(-9.79526974288331,20.4923005087943,
12.));
#242786=CARTESIAN_POINT('Ctrl Pts',(-9.79023916498656,20.4843302955329,
0.));
#242787=CARTESIAN_POINT('Ctrl Pts',(-9.79023916498656,20.4843302955329,
12.));
#242788=CARTESIAN_POINT('Ctrl Pts',(-9.78535797314167,20.4765353711586,
0.));
#242789=CARTESIAN_POINT('Ctrl Pts',(-9.78535797314167,20.4765353711586,
12.));
#242790=CARTESIAN_POINT('Ctrl Pts',(-9.78062712373321,20.4689199790669,
0.));
#242791=CARTESIAN_POINT('Ctrl Pts',(-9.78062712373321,20.4689199790669,
12.));
#242792=CARTESIAN_POINT('Ctrl Pts',(-9.77604760815529,20.4614885274975,
0.));
#242793=CARTESIAN_POINT('Ctrl Pts',(-9.77604760815529,20.4614885274975,
12.));
#242794=CARTESIAN_POINT('Ctrl Pts',(-9.7716204510407,20.4542455817527,0.));
#242795=CARTESIAN_POINT('Ctrl Pts',(-9.7716204510407,20.4542455817527,12.));
#242796=CARTESIAN_POINT('Ctrl Pts',(-9.76734670980892,20.447195862298,0.));
#242797=CARTESIAN_POINT('Ctrl Pts',(-9.76734670980892,20.447195862298,12.));
#242798=CARTESIAN_POINT('Ctrl Pts',(-9.76322747195495,20.44034423294,0.));
#242799=CARTESIAN_POINT('Ctrl Pts',(-9.76322747195495,20.44034423294,12.));
#242800=CARTESIAN_POINT('Ctrl Pts',(-9.75926386289923,20.4336957355473,
0.));
#242801=CARTESIAN_POINT('Ctrl Pts',(-9.75926386289923,20.4336957355473,
12.));
#242802=CARTESIAN_POINT('Ctrl Pts',(-9.75545705902418,20.4272556476629,
0.));
#242803=CARTESIAN_POINT('Ctrl Pts',(-9.75545705902418,20.4272556476629,
12.));
#242804=CARTESIAN_POINT('Ctrl Pts',(-9.7518082978643,20.4210295275817,0.));
#242805=CARTESIAN_POINT('Ctrl Pts',(-9.7518082978643,20.4210295275817,12.));
#242806=CARTESIAN_POINT('Ctrl Pts',(-9.74831889242174,20.4150232777393,
0.));
#242807=CARTESIAN_POINT('Ctrl Pts',(-9.74831889242174,20.4150232777393,
12.));
#242808=CARTESIAN_POINT('Ctrl Pts',(-9.74499021838538,20.4092430879861,
0.));
#242809=CARTESIAN_POINT('Ctrl Pts',(-9.74499021838538,20.4092430879861,
12.));
#242810=CARTESIAN_POINT('Ctrl Pts',(-9.74182369656272,20.4036953576549,
0.));
#242811=CARTESIAN_POINT('Ctrl Pts',(-9.74182369656272,20.4036953576549,
12.));
#242812=CARTESIAN_POINT('Ctrl Pts',(-9.73882077613201,20.3983866213331,
0.));
#242813=CARTESIAN_POINT('Ctrl Pts',(-9.73882077613201,20.3983866213331,
12.));
#242814=CARTESIAN_POINT('Ctrl Pts',(-9.73598292014243,20.3933234845647,
0.));
#242815=CARTESIAN_POINT('Ctrl Pts',(-9.73598292014243,20.3933234845647,
12.));
#242816=CARTESIAN_POINT('Ctrl Pts',(-9.73331167102808,20.3885129129912,
0.));
#242817=CARTESIAN_POINT('Ctrl Pts',(-9.73331167102808,20.3885129129912,
12.));
#242818=CARTESIAN_POINT('Ctrl Pts',(-9.73080870123727,20.3839624556742,
0.));
#242819=CARTESIAN_POINT('Ctrl Pts',(-9.73080870123727,20.3839624556742,
12.));
#242820=CARTESIAN_POINT('Ctrl Pts',(-9.72847589116542,20.3796805893304,
0.));
#242821=CARTESIAN_POINT('Ctrl Pts',(-9.72847589116542,20.3796805893304,
12.));
#242822=CARTESIAN_POINT('Ctrl Pts',(-9.7263153173288,20.3756766651951,0.));
#242823=CARTESIAN_POINT('Ctrl Pts',(-9.7263153173288,20.3756766651951,12.));
#242824=CARTESIAN_POINT('Ctrl Pts',(-9.72432910043194,20.371960235676,0.));
#242825=CARTESIAN_POINT('Ctrl Pts',(-9.72432910043194,20.371960235676,12.));
#242826=CARTESIAN_POINT('Ctrl Pts',(-9.7225193072249,20.3685406190576,0.));
#242827=CARTESIAN_POINT('Ctrl Pts',(-9.7225193072249,20.3685406190576,12.));
#242828=CARTESIAN_POINT('Ctrl Pts',(-9.72088778381081,20.3654261611056,
0.));
#242829=CARTESIAN_POINT('Ctrl Pts',(-9.72088778381081,20.3654261611056,
12.));
#242830=CARTESIAN_POINT('Ctrl Pts',(-9.71943648548099,20.3626256913981,
0.));
#242831=CARTESIAN_POINT('Ctrl Pts',(-9.71943648548099,20.3626256913981,
12.));
#242832=CARTESIAN_POINT('Ctrl Pts',(-9.71816778328006,20.3601498764344,
0.));
#242833=CARTESIAN_POINT('Ctrl Pts',(-9.71816778328006,20.3601498764344,
12.));
#242834=CARTESIAN_POINT('Ctrl Pts',(-9.71708493723096,20.3580133103356,
0.));
#242835=CARTESIAN_POINT('Ctrl Pts',(-9.71708493723096,20.3580133103356,
12.));
#242836=CARTESIAN_POINT('Ctrl Pts',(-9.71619192554186,20.3562337557875,
0.));
#242837=CARTESIAN_POINT('Ctrl Pts',(-9.71619192554186,20.3562337557875,
12.));
#242838=CARTESIAN_POINT('Ctrl Pts',(-9.71549257088172,20.3548282742361,
0.));
#242839=CARTESIAN_POINT('Ctrl Pts',(-9.71549257088172,20.3548282742361,
12.));
#242840=CARTESIAN_POINT('Ctrl Pts',(-9.71498978052021,20.3538098605706,
0.));
#242841=CARTESIAN_POINT('Ctrl Pts',(-9.71498978052021,20.3538098605706,
12.));
#242842=CARTESIAN_POINT('Ctrl Pts',(-9.71474590350681,20.3533097561886,
0.));
#242843=CARTESIAN_POINT('Ctrl Pts',(-9.71474590350681,20.3533097561886,
12.));
#242844=CARTESIAN_POINT('Ctrl Pts',(-9.71465227853041,20.3531126095522,
0.));
#242845=CARTESIAN_POINT('Ctrl Pts',(-9.71465227853041,20.3531126095522,
12.));
#242846=CARTESIAN_POINT('Ctrl Pts',(-9.71462954053042,20.353060251684,0.));
#242847=CARTESIAN_POINT('Ctrl Pts',(-9.71462954053042,20.353060251684,12.));
#242848=CARTESIAN_POINT('Ctrl Pts',(-9.71462809124916,20.353053841303,0.));
#242849=CARTESIAN_POINT('Ctrl Pts',(-9.71462809124916,20.353053841303,12.));
#242850=CARTESIAN_POINT('',(-12.4230808101438,22.8400320311648,0.));
#242851=CARTESIAN_POINT('Ctrl Pts',(-12.4230808101438,22.8400320311648,
0.));
#242852=CARTESIAN_POINT('Ctrl Pts',(-12.418215285186,22.8370364396459,0.));
#242853=CARTESIAN_POINT('Ctrl Pts',(-12.4084933766347,22.8310435872747,
0.));
#242854=CARTESIAN_POINT('Ctrl Pts',(-12.3939379378998,22.8220493007173,
0.));
#242855=CARTESIAN_POINT('Ctrl Pts',(-12.374585536673,22.81004690224,0.));
#242856=CARTESIAN_POINT('Ctrl Pts',(-12.3504864740319,22.795027221673,0.));
#242857=CARTESIAN_POINT('Ctrl Pts',(-12.3264788926075,22.7799908974768,
0.));
#242858=CARTESIAN_POINT('Ctrl Pts',(-12.3025628601792,22.764938010105,0.));
#242859=CARTESIAN_POINT('Ctrl Pts',(-12.2787384750742,22.7498686970069,
0.));
#242860=CARTESIAN_POINT('Ctrl Pts',(-12.2550058702395,22.7347831655287,
0.));
#242861=CARTESIAN_POINT('Ctrl Pts',(-12.2313652198061,22.7196817119374,
0.));
#242862=CARTESIAN_POINT('Ctrl Pts',(-12.2078167360284,22.7045647168747,
0.));
#242863=CARTESIAN_POINT('Ctrl Pts',(-12.1843606579262,22.6894326205037,
0.));
#242864=CARTESIAN_POINT('Ctrl Pts',(-12.1609972423099,22.6742859034944,
0.));
#242865=CARTESIAN_POINT('Ctrl Pts',(-12.1377267537145,22.6591250653965,
0.));
#242866=CARTESIAN_POINT('Ctrl Pts',(-12.1145494550383,22.6439506046605,
0.));
#242867=CARTESIAN_POINT('Ctrl Pts',(-12.0914655972823,22.6287629967056,
0.));
#242868=CARTESIAN_POINT('Ctrl Pts',(-12.0684754113862,22.6135626764898,
0.));
#242869=CARTESIAN_POINT('Ctrl Pts',(-12.0455791139128,22.5983500505644,
0.));
#242870=CARTESIAN_POINT('Ctrl Pts',(-12.0227769113127,22.5831255061282,
0.));
#242871=CARTESIAN_POINT('Ctrl Pts',(-12.0000690046695,22.5678894211181,
0.));
#242872=CARTESIAN_POINT('Ctrl Pts',(-11.9774555943496,22.5526421741158,
0.));
#242873=CARTESIAN_POINT('Ctrl Pts',(-11.9549368843997,22.5373841537307,
0.));
#242874=CARTESIAN_POINT('Ctrl Pts',(-11.9325130877803,22.5221157697883,
0.));
#242875=CARTESIAN_POINT('Ctrl Pts',(-11.9101844254557,22.5068374513973,
0.));
#242876=CARTESIAN_POINT('Ctrl Pts',(-11.8879511239943,22.4915496418485,
0.));
#242877=CARTESIAN_POINT('Ctrl Pts',(-11.8658134137019,22.4762527946702,
0.));
#242878=CARTESIAN_POINT('Ctrl Pts',(-11.8437715264487,22.4609473690471,
0.));
#242879=CARTESIAN_POINT('Ctrl Pts',(-11.8218256937889,22.4456338258735,
0.));
#242880=CARTESIAN_POINT('Ctrl Pts',(-11.7999761445173,22.430312622646,0.));
#242881=CARTESIAN_POINT('Ctrl Pts',(-11.7782231042039,22.4149842125008,
0.));
#242882=CARTESIAN_POINT('Ctrl Pts',(-11.7565667964764,22.3996490469191,
0.));
#242883=CARTESIAN_POINT('Ctrl Pts',(-11.7350074437961,22.3843075773899,
0.));
#242884=CARTESIAN_POINT('Ctrl Pts',(-11.7135452684532,22.3689602575491,
0.));
#242885=CARTESIAN_POINT('Ctrl Pts',(-11.6921804934056,22.3536075450029,
0.));
#242886=CARTESIAN_POINT('Ctrl Pts',(-11.6709133432985,22.3382499035619,
0.));
#242887=CARTESIAN_POINT('Ctrl Pts',(-11.6497440449857,22.3228878043976,
0.));
#242888=CARTESIAN_POINT('Ctrl Pts',(-11.6286728270009,22.3075217249049,
0.));
#242889=CARTESIAN_POINT('Ctrl Pts',(-11.6076999192357,22.2921521480356,
0.));
#242890=CARTESIAN_POINT('Ctrl Pts',(-11.5868255525188,22.2767795614348,
0.));
#242891=CARTESIAN_POINT('Ctrl Pts',(-11.5660499582403,22.2614044566898,
0.));
#242892=CARTESIAN_POINT('Ctrl Pts',(-11.5453733679121,22.2460273284654,
0.));
#242893=CARTESIAN_POINT('Ctrl Pts',(-11.5247960128477,22.2306486738901,
0.));
#242894=CARTESIAN_POINT('Ctrl Pts',(-11.5043181244242,22.2152689931022,
0.));
#242895=CARTESIAN_POINT('Ctrl Pts',(-11.483939934259,22.1998887896436,0.));
#242896=CARTESIAN_POINT('Ctrl Pts',(-11.463661674411,22.184508570917,0.));
#242897=CARTESIAN_POINT('Ctrl Pts',(-11.443483577557,22.1691288486096,0.));
#242898=CARTESIAN_POINT('Ctrl Pts',(-11.4234058771742,22.1537501391487,
0.));
#242899=CARTESIAN_POINT('Ctrl Pts',(-11.4034288076908,22.1383729640964,
0.));
#242900=CARTESIAN_POINT('Ctrl Pts',(-11.3835526044256,22.1229978500186,
0.));
#242901=CARTESIAN_POINT('Ctrl Pts',(-11.3637775035367,22.1076253283979,
0.));
#242902=CARTESIAN_POINT('Ctrl Pts',(-11.3441037419553,22.0922559355294,
0.));
#242903=CARTESIAN_POINT('Ctrl Pts',(-11.3245315573168,22.0768902124267,
0.));
#242904=CARTESIAN_POINT('Ctrl Pts',(-11.3050611878771,22.0615287047179,
0.));
#242905=CARTESIAN_POINT('Ctrl Pts',(-11.2856928724374,22.046171962566,0.));
#242906=CARTESIAN_POINT('Ctrl Pts',(-11.2664268504206,22.030820540835,0.));
#242907=CARTESIAN_POINT('Ctrl Pts',(-11.2472633619275,22.0154749992363,
0.));
#242908=CARTESIAN_POINT('Ctrl Pts',(-11.2282026477896,22.0001359024839,
0.));
#242909=CARTESIAN_POINT('Ctrl Pts',(-11.2092449496125,21.9848038204439,
0.));
#242910=CARTESIAN_POINT('Ctrl Pts',(-11.190390509811,21.9694793282914,0.));
#242911=CARTESIAN_POINT('Ctrl Pts',(-11.1716395716376,21.9541630066506,
0.));
#242912=CARTESIAN_POINT('Ctrl Pts',(-11.1529923792003,21.9388554416439,
0.));
#242913=CARTESIAN_POINT('Ctrl Pts',(-11.1344491774741,21.923557224952,0.));
#242914=CARTESIAN_POINT('Ctrl Pts',(-11.1160102123024,21.9082689538688,
0.));
#242915=CARTESIAN_POINT('Ctrl Pts',(-11.0976757303944,21.8929912313608,
0.));
#242916=CARTESIAN_POINT('Ctrl Pts',(-11.0794459793057,21.877724666119,0.));
#242917=CARTESIAN_POINT('Ctrl Pts',(-11.0613212074363,21.8624698726318,
0.));
#242918=CARTESIAN_POINT('Ctrl Pts',(-11.0433016640807,21.8472274713103,
0.));
#242919=CARTESIAN_POINT('Ctrl Pts',(-11.0253875994598,21.8319980886033,
0.));
#242920=CARTESIAN_POINT('Ctrl Pts',(-11.0075792647477,21.8167823571168,
0.));
#242921=CARTESIAN_POINT('Ctrl Pts',(-10.9898769120912,21.8015809157301,
0.));
#242922=CARTESIAN_POINT('Ctrl Pts',(-10.9722807946156,21.7863944097141,
0.));
#242923=CARTESIAN_POINT('Ctrl Pts',(-10.9547911664455,21.7712234908464,
0.));
#242924=CARTESIAN_POINT('Ctrl Pts',(-10.9374082827444,21.7560688175247,
0.));
#242925=CARTESIAN_POINT('Ctrl Pts',(-10.9201323997384,21.7409310548797,
0.));
#242926=CARTESIAN_POINT('Ctrl Pts',(-10.902963774734,21.7258108748873,0.));
#242927=CARTESIAN_POINT('Ctrl Pts',(-10.8859026661293,21.7107089564825,
0.));
#242928=CARTESIAN_POINT('Ctrl Pts',(-10.8689493334095,21.6956259856672,
0.));
#242929=CARTESIAN_POINT('Ctrl Pts',(-10.8521040371835,21.6805626556467,
0.));
#242930=CARTESIAN_POINT('Ctrl Pts',(-10.8353670392272,21.6655196669732,
0.));
#242931=CARTESIAN_POINT('Ctrl Pts',(-10.8187386025136,21.6504977276866,
0.));
#242932=CARTESIAN_POINT('Ctrl Pts',(-10.8022189912369,21.6354975534557,
0.));
#242933=CARTESIAN_POINT('Ctrl Pts',(-10.7858084708261,21.6205198677173,
0.));
#242934=CARTESIAN_POINT('Ctrl Pts',(-10.7695073079552,21.6055654018176,
0.));
#242935=CARTESIAN_POINT('Ctrl Pts',(-10.7533157705941,21.5906348951743,
0.));
#242936=CARTESIAN_POINT('Ctrl Pts',(-10.7372341280467,21.5757290954371,
0.));
#242937=CARTESIAN_POINT('Ctrl Pts',(-10.7212626509816,21.5608487586468,
0.));
#242938=CARTESIAN_POINT('Ctrl Pts',(-10.7054016114571,21.5459946493955,
0.));
#242939=CARTESIAN_POINT('Ctrl Pts',(-10.689651282929,21.5311675409807,0.));
#242940=CARTESIAN_POINT('Ctrl Pts',(-10.6740119402834,21.51636821558,0.));
#242941=CARTESIAN_POINT('Ctrl Pts',(-10.6584838598939,21.5015974644449,
0.));
#242942=CARTESIAN_POINT('Ctrl Pts',(-10.6430673196607,21.4868560880889,
0.));
#242943=CARTESIAN_POINT('Ctrl Pts',(-10.6277625990456,21.4721448964766,
0.));
#242944=CARTESIAN_POINT('Ctrl Pts',(-10.6125699790961,21.4574647092097,
0.));
#242945=CARTESIAN_POINT('Ctrl Pts',(-10.5974897424622,21.4428163557144,
0.));
#242946=CARTESIAN_POINT('Ctrl Pts',(-10.5825221734573,21.4282006754631,
0.));
#242947=CARTESIAN_POINT('Ctrl Pts',(-10.5676675581108,21.4136185181979,
0.));
#242948=CARTESIAN_POINT('Ctrl Pts',(-10.5529261842108,21.3990707441497,
0.));
#242949=CARTESIAN_POINT('Ctrl Pts',(-10.5382983413421,21.3845582242602,
0.));
#242950=CARTESIAN_POINT('Ctrl Pts',(-10.5237843209057,21.3700818403936,
0.));
#242951=CARTESIAN_POINT('Ctrl Pts',(-10.5093844161685,21.3556424855814,
0.));
#242952=CARTESIAN_POINT('Ctrl Pts',(-10.4950989223337,21.3412410642904,
0.));
#242953=CARTESIAN_POINT('Ctrl Pts',(-10.4809281365931,21.3268784926819,
0.));
#242954=CARTESIAN_POINT('Ctrl Pts',(-10.4668723581768,21.3125556988731,
0.));
#242955=CARTESIAN_POINT('Ctrl Pts',(-10.4529318883874,21.2982736231931,
0.));
#242956=CARTESIAN_POINT('Ctrl Pts',(-10.4391070306391,21.2840332184483,
0.));
#242957=CARTESIAN_POINT('Ctrl Pts',(-10.42539809054,21.2698354502403,0.));
#242958=CARTESIAN_POINT('Ctrl Pts',(-10.4118053759588,21.255681297275,0.));
#242959=CARTESIAN_POINT('Ctrl Pts',(-10.3983291970846,21.2415717516714,
0.));
#242960=CARTESIAN_POINT('Ctrl Pts',(-10.3849698664786,21.22750781927,0.));
#242961=CARTESIAN_POINT('Ctrl Pts',(-10.371727699113,21.2134905199345,0.));
#242962=CARTESIAN_POINT('Ctrl Pts',(-10.3586030124587,21.199520887919,0.));
#242963=CARTESIAN_POINT('Ctrl Pts',(-10.3455961265701,21.1855999722416,
0.));
#242964=CARTESIAN_POINT('Ctrl Pts',(-10.3327073641572,21.1717288370509,
0.));
#242965=CARTESIAN_POINT('Ctrl Pts',(-10.3199370506544,21.1579085619965,
0.));
#242966=CARTESIAN_POINT('Ctrl Pts',(-10.3072855142687,21.1441402425843,
0.));
#242967=CARTESIAN_POINT('Ctrl Pts',(-10.2947530860721,21.1304249906002,
0.));
#242968=CARTESIAN_POINT('Ctrl Pts',(-10.2823401001072,21.1167639345631,
0.));
#242969=CARTESIAN_POINT('Ctrl Pts',(-10.2700468934744,21.1031582201627,
0.));
#242970=CARTESIAN_POINT('Ctrl Pts',(-10.2578738064181,21.0896090107063,
0.));
#242971=CARTESIAN_POINT('Ctrl Pts',(-10.2458211823912,21.0761174875445,
0.));
#242972=CARTESIAN_POINT('Ctrl Pts',(-10.2338893681567,21.0626848505663,
0.));
#242973=CARTESIAN_POINT('Ctrl Pts',(-10.2220787139155,21.0493123187483,
0.));
#242974=CARTESIAN_POINT('Ctrl Pts',(-10.2103895734123,21.0360011306815,
0.));
#242975=CARTESIAN_POINT('Ctrl Pts',(-10.1988223040425,21.0227525451107,
0.));
#242976=CARTESIAN_POINT('Ctrl Pts',(-10.187377266936,21.0095678414486,0.));
#242977=CARTESIAN_POINT('Ctrl Pts',(-10.1760548270767,20.9964483203686,
0.));
#242978=CARTESIAN_POINT('Ctrl Pts',(-10.1648553534568,20.9833953044736,
0.));
#242979=CARTESIAN_POINT('Ctrl Pts',(-10.1537792192065,20.9704101389369,
0.));
#242980=CARTESIAN_POINT('Ctrl Pts',(-10.1428268017256,20.9574941921591,
0.));
#242981=CARTESIAN_POINT('Ctrl Pts',(-10.1319984827908,20.9446488563933,
0.));
#242982=CARTESIAN_POINT('Ctrl Pts',(-10.1212946487057,20.9318755484734,
0.));
#242983=CARTESIAN_POINT('Ctrl Pts',(-10.1107156904836,20.919175710627,0.));
#242984=CARTESIAN_POINT('Ctrl Pts',(-10.1002620040076,20.9065508112557,
0.));
#242985=CARTESIAN_POINT('Ctrl Pts',(-10.0899339901916,20.894002345737,0.));
#242986=CARTESIAN_POINT('Ctrl Pts',(-10.0797320551154,20.881531837184,0.));
#242987=CARTESIAN_POINT('Ctrl Pts',(-10.0696566102218,20.86914083737,0.));
#242988=CARTESIAN_POINT('Ctrl Pts',(-10.0597080725375,20.8568309277316,
0.));
#242989=CARTESIAN_POINT('Ctrl Pts',(-10.0498868648733,20.8446037203402,
0.));
#242990=CARTESIAN_POINT('Ctrl Pts',(-10.0401934160234,20.8324608588909,
0.));
#242991=CARTESIAN_POINT('Ctrl Pts',(-10.0306281609435,20.8204040196602,
0.));
#242992=CARTESIAN_POINT('Ctrl Pts',(-10.0211915410095,20.8084349126888,
0.));
#242993=CARTESIAN_POINT('Ctrl Pts',(-10.0118840042786,20.7965552829908,
0.));
#242994=CARTESIAN_POINT('Ctrl Pts',(-10.0027060057389,20.7847669117568,
0.));
#242995=CARTESIAN_POINT('Ctrl Pts',(-9.9936580075464,20.7730716175417,0.));
#242996=CARTESIAN_POINT('Ctrl Pts',(-9.98474047926852,20.761471257499,0.));
#242997=CARTESIAN_POINT('Ctrl Pts',(-9.9759538982347,20.7499677289627,0.));
#242998=CARTESIAN_POINT('Ctrl Pts',(-9.96729874986202,20.7385629709795,
0.));
#242999=CARTESIAN_POINT('Ctrl Pts',(-9.95877552798398,20.7272589658751,
0.));
#243000=CARTESIAN_POINT('Ctrl Pts',(-9.95038473514949,20.7160577407579,
0.));
#243001=CARTESIAN_POINT('Ctrl Pts',(-9.94212688298236,20.7049613692234,
0.));
#243002=CARTESIAN_POINT('Ctrl Pts',(-9.9340024925973,20.6939719732484,0.));
#243003=CARTESIAN_POINT('Ctrl Pts',(-9.92601209498749,20.6830917250255,
0.));
#243004=CARTESIAN_POINT('Ctrl Pts',(-9.91815623141289,20.6723228488263,
0.));
#243005=CARTESIAN_POINT('Ctrl Pts',(-9.91043545377007,20.6616676228315,
0.));
#243006=CARTESIAN_POINT('Ctrl Pts',(-9.90285032516693,20.6511283817414,
0.));
#243007=CARTESIAN_POINT('Ctrl Pts',(-9.8954014204912,20.6407075193976,0.));
#243008=CARTESIAN_POINT('Ctrl Pts',(-9.88808932697306,20.6304074914087,
0.));
#243009=CARTESIAN_POINT('Ctrl Pts',(-9.88091464472676,20.6202308177474,
0.));
#243010=CARTESIAN_POINT('Ctrl Pts',(-9.87387798732956,20.6101800854494,
0.));
#243011=CARTESIAN_POINT('Ctrl Pts',(-9.86697998242623,20.6002579513699,
0.));
#243012=CARTESIAN_POINT('Ctrl Pts',(-9.86022127232748,20.5904671449754,
0.));
#243013=CARTESIAN_POINT('Ctrl Pts',(-9.85360251456981,20.5808104710015,
0.));
#243014=CARTESIAN_POINT('Ctrl Pts',(-9.84712438256278,20.5712908125139,
0.));
#243015=CARTESIAN_POINT('Ctrl Pts',(-9.84078756677565,20.5619111362402,
0.));
#243016=CARTESIAN_POINT('Ctrl Pts',(-9.83459277585315,20.552674497646,0.));
#243017=CARTESIAN_POINT('Ctrl Pts',(-9.82854073773877,20.5435840460721,
0.));
#243018=CARTESIAN_POINT('Ctrl Pts',(-9.82263220080363,20.5346430299517,
0.));
#243019=CARTESIAN_POINT('Ctrl Pts',(-9.81686793455943,20.5258548000629,
0.));
#243020=CARTESIAN_POINT('Ctrl Pts',(-9.81124873025282,20.517222812284,0.));
#243021=CARTESIAN_POINT('Ctrl Pts',(-9.80577540161088,20.5087506310505,
0.));
#243022=CARTESIAN_POINT('Ctrl Pts',(-9.80044878520949,20.5004419312107,
0.));
#243023=CARTESIAN_POINT('Ctrl Pts',(-9.79526974288331,20.4923005087943,
0.));
#243024=CARTESIAN_POINT('Ctrl Pts',(-9.79023916498656,20.4843302955329,
0.));
#243025=CARTESIAN_POINT('Ctrl Pts',(-9.78535797314167,20.4765353711586,
0.));
#243026=CARTESIAN_POINT('Ctrl Pts',(-9.78062712373321,20.4689199790669,
0.));
#243027=CARTESIAN_POINT('Ctrl Pts',(-9.77604760815529,20.4614885274975,
0.));
#243028=CARTESIAN_POINT('Ctrl Pts',(-9.7716204510407,20.4542455817527,0.));
#243029=CARTESIAN_POINT('Ctrl Pts',(-9.76734670980892,20.447195862298,0.));
#243030=CARTESIAN_POINT('Ctrl Pts',(-9.76322747195495,20.44034423294,0.));
#243031=CARTESIAN_POINT('Ctrl Pts',(-9.75926386289923,20.4336957355473,
0.));
#243032=CARTESIAN_POINT('Ctrl Pts',(-9.75545705902418,20.4272556476629,
0.));
#243033=CARTESIAN_POINT('Ctrl Pts',(-9.7518082978643,20.4210295275817,0.));
#243034=CARTESIAN_POINT('Ctrl Pts',(-9.74831889242174,20.4150232777393,
0.));
#243035=CARTESIAN_POINT('Ctrl Pts',(-9.74499021838538,20.4092430879861,
0.));
#243036=CARTESIAN_POINT('Ctrl Pts',(-9.74182369656272,20.4036953576549,
0.));
#243037=CARTESIAN_POINT('Ctrl Pts',(-9.73882077613201,20.3983866213331,
0.));
#243038=CARTESIAN_POINT('Ctrl Pts',(-9.73598292014243,20.3933234845647,
0.));
#243039=CARTESIAN_POINT('Ctrl Pts',(-9.73331167102808,20.3885129129912,
0.));
#243040=CARTESIAN_POINT('Ctrl Pts',(-9.73080870123727,20.3839624556742,
0.));
#243041=CARTESIAN_POINT('Ctrl Pts',(-9.72847589116542,20.3796805893304,
0.));
#243042=CARTESIAN_POINT('Ctrl Pts',(-9.7263153173288,20.3756766651951,0.));
#243043=CARTESIAN_POINT('Ctrl Pts',(-9.72432910043194,20.371960235676,0.));
#243044=CARTESIAN_POINT('Ctrl Pts',(-9.7225193072249,20.3685406190576,0.));
#243045=CARTESIAN_POINT('Ctrl Pts',(-9.72088778381081,20.3654261611056,
0.));
#243046=CARTESIAN_POINT('Ctrl Pts',(-9.71943648548099,20.3626256913981,
0.));
#243047=CARTESIAN_POINT('Ctrl Pts',(-9.71816778328006,20.3601498764344,
0.));
#243048=CARTESIAN_POINT('Ctrl Pts',(-9.71708493723096,20.3580133103356,
0.));
#243049=CARTESIAN_POINT('Ctrl Pts',(-9.71619192554186,20.3562337557875,
0.));
#243050=CARTESIAN_POINT('Ctrl Pts',(-9.71549257088172,20.3548282742361,
0.));
#243051=CARTESIAN_POINT('Ctrl Pts',(-9.71498978052021,20.3538098605706,
0.));
#243052=CARTESIAN_POINT('Ctrl Pts',(-9.71474590350681,20.3533097561886,
0.));
#243053=CARTESIAN_POINT('Ctrl Pts',(-9.71465227853041,20.3531126095522,
0.));
#243054=CARTESIAN_POINT('Ctrl Pts',(-9.71462954053042,20.353060251684,0.));
#243055=CARTESIAN_POINT('Ctrl Pts',(-9.71462809124916,20.353053841303,0.));
#243056=CARTESIAN_POINT('',(-12.4230808101438,22.8400320311648,12.));
#243057=CARTESIAN_POINT('',(-12.4230808101438,22.8400320311648,0.));
#243058=CARTESIAN_POINT('Ctrl Pts',(-9.71462809124916,20.353053841303,12.));
#243059=CARTESIAN_POINT('Ctrl Pts',(-9.71462954053042,20.353060251684,12.));
#243060=CARTESIAN_POINT('Ctrl Pts',(-9.71465227853041,20.3531126095522,
12.));
#243061=CARTESIAN_POINT('Ctrl Pts',(-9.71474590350681,20.3533097561886,
12.));
#243062=CARTESIAN_POINT('Ctrl Pts',(-9.71498978052021,20.3538098605706,
12.));
#243063=CARTESIAN_POINT('Ctrl Pts',(-9.71549257088172,20.3548282742361,
12.));
#243064=CARTESIAN_POINT('Ctrl Pts',(-9.71619192554186,20.3562337557875,
12.));
#243065=CARTESIAN_POINT('Ctrl Pts',(-9.71708493723096,20.3580133103356,
12.));
#243066=CARTESIAN_POINT('Ctrl Pts',(-9.71816778328006,20.3601498764344,
12.));
#243067=CARTESIAN_POINT('Ctrl Pts',(-9.71943648548099,20.3626256913981,
12.));
#243068=CARTESIAN_POINT('Ctrl Pts',(-9.72088778381081,20.3654261611056,
12.));
#243069=CARTESIAN_POINT('Ctrl Pts',(-9.7225193072249,20.3685406190576,12.));
#243070=CARTESIAN_POINT('Ctrl Pts',(-9.72432910043194,20.371960235676,12.));
#243071=CARTESIAN_POINT('Ctrl Pts',(-9.7263153173288,20.3756766651951,12.));
#243072=CARTESIAN_POINT('Ctrl Pts',(-9.72847589116542,20.3796805893304,
12.));
#243073=CARTESIAN_POINT('Ctrl Pts',(-9.73080870123727,20.3839624556742,
12.));
#243074=CARTESIAN_POINT('Ctrl Pts',(-9.73331167102808,20.3885129129912,
12.));
#243075=CARTESIAN_POINT('Ctrl Pts',(-9.73598292014243,20.3933234845647,
12.));
#243076=CARTESIAN_POINT('Ctrl Pts',(-9.73882077613201,20.3983866213331,
12.));
#243077=CARTESIAN_POINT('Ctrl Pts',(-9.74182369656272,20.4036953576549,
12.));
#243078=CARTESIAN_POINT('Ctrl Pts',(-9.74499021838538,20.4092430879861,
12.));
#243079=CARTESIAN_POINT('Ctrl Pts',(-9.74831889242174,20.4150232777393,
12.));
#243080=CARTESIAN_POINT('Ctrl Pts',(-9.7518082978643,20.4210295275817,12.));
#243081=CARTESIAN_POINT('Ctrl Pts',(-9.75545705902418,20.4272556476629,
12.));
#243082=CARTESIAN_POINT('Ctrl Pts',(-9.75926386289923,20.4336957355473,
12.));
#243083=CARTESIAN_POINT('Ctrl Pts',(-9.76322747195495,20.44034423294,12.));
#243084=CARTESIAN_POINT('Ctrl Pts',(-9.76734670980892,20.447195862298,12.));
#243085=CARTESIAN_POINT('Ctrl Pts',(-9.7716204510407,20.4542455817527,12.));
#243086=CARTESIAN_POINT('Ctrl Pts',(-9.77604760815529,20.4614885274975,
12.));
#243087=CARTESIAN_POINT('Ctrl Pts',(-9.78062712373321,20.4689199790669,
12.));
#243088=CARTESIAN_POINT('Ctrl Pts',(-9.78535797314167,20.4765353711586,
12.));
#243089=CARTESIAN_POINT('Ctrl Pts',(-9.79023916498656,20.4843302955329,
12.));
#243090=CARTESIAN_POINT('Ctrl Pts',(-9.79526974288331,20.4923005087943,
12.));
#243091=CARTESIAN_POINT('Ctrl Pts',(-9.80044878520949,20.5004419312107,
12.));
#243092=CARTESIAN_POINT('Ctrl Pts',(-9.80577540161088,20.5087506310505,
12.));
#243093=CARTESIAN_POINT('Ctrl Pts',(-9.81124873025282,20.517222812284,12.));
#243094=CARTESIAN_POINT('Ctrl Pts',(-9.81686793455943,20.5258548000629,
12.));
#243095=CARTESIAN_POINT('Ctrl Pts',(-9.82263220080363,20.5346430299517,
12.));
#243096=CARTESIAN_POINT('Ctrl Pts',(-9.82854073773877,20.5435840460721,
12.));
#243097=CARTESIAN_POINT('Ctrl Pts',(-9.83459277585315,20.552674497646,12.));
#243098=CARTESIAN_POINT('Ctrl Pts',(-9.84078756677565,20.5619111362402,
12.));
#243099=CARTESIAN_POINT('Ctrl Pts',(-9.84712438256278,20.5712908125139,
12.));
#243100=CARTESIAN_POINT('Ctrl Pts',(-9.85360251456981,20.5808104710015,
12.));
#243101=CARTESIAN_POINT('Ctrl Pts',(-9.86022127232748,20.5904671449754,
12.));
#243102=CARTESIAN_POINT('Ctrl Pts',(-9.86697998242623,20.6002579513699,
12.));
#243103=CARTESIAN_POINT('Ctrl Pts',(-9.87387798732956,20.6101800854494,
12.));
#243104=CARTESIAN_POINT('Ctrl Pts',(-9.88091464472676,20.6202308177474,
12.));
#243105=CARTESIAN_POINT('Ctrl Pts',(-9.88808932697306,20.6304074914087,
12.));
#243106=CARTESIAN_POINT('Ctrl Pts',(-9.8954014204912,20.6407075193976,12.));
#243107=CARTESIAN_POINT('Ctrl Pts',(-9.90285032516693,20.6511283817414,
12.));
#243108=CARTESIAN_POINT('Ctrl Pts',(-9.91043545377007,20.6616676228315,
12.));
#243109=CARTESIAN_POINT('Ctrl Pts',(-9.91815623141289,20.6723228488263,
12.));
#243110=CARTESIAN_POINT('Ctrl Pts',(-9.92601209498749,20.6830917250255,
12.));
#243111=CARTESIAN_POINT('Ctrl Pts',(-9.9340024925973,20.6939719732484,12.));
#243112=CARTESIAN_POINT('Ctrl Pts',(-9.94212688298236,20.7049613692234,
12.));
#243113=CARTESIAN_POINT('Ctrl Pts',(-9.95038473514949,20.7160577407579,
12.));
#243114=CARTESIAN_POINT('Ctrl Pts',(-9.95877552798398,20.7272589658751,
12.));
#243115=CARTESIAN_POINT('Ctrl Pts',(-9.96729874986202,20.7385629709795,
12.));
#243116=CARTESIAN_POINT('Ctrl Pts',(-9.9759538982347,20.7499677289627,12.));
#243117=CARTESIAN_POINT('Ctrl Pts',(-9.98474047926852,20.761471257499,12.));
#243118=CARTESIAN_POINT('Ctrl Pts',(-9.9936580075464,20.7730716175417,12.));
#243119=CARTESIAN_POINT('Ctrl Pts',(-10.0027060057389,20.7847669117568,
12.));
#243120=CARTESIAN_POINT('Ctrl Pts',(-10.0118840042786,20.7965552829908,
12.));
#243121=CARTESIAN_POINT('Ctrl Pts',(-10.0211915410095,20.8084349126888,
12.));
#243122=CARTESIAN_POINT('Ctrl Pts',(-10.0306281609435,20.8204040196602,
12.));
#243123=CARTESIAN_POINT('Ctrl Pts',(-10.0401934160234,20.8324608588909,
12.));
#243124=CARTESIAN_POINT('Ctrl Pts',(-10.0498868648733,20.8446037203402,
12.));
#243125=CARTESIAN_POINT('Ctrl Pts',(-10.0597080725375,20.8568309277316,
12.));
#243126=CARTESIAN_POINT('Ctrl Pts',(-10.0696566102218,20.86914083737,12.));
#243127=CARTESIAN_POINT('Ctrl Pts',(-10.0797320551154,20.881531837184,12.));
#243128=CARTESIAN_POINT('Ctrl Pts',(-10.0899339901916,20.894002345737,12.));
#243129=CARTESIAN_POINT('Ctrl Pts',(-10.1002620040076,20.9065508112557,
12.));
#243130=CARTESIAN_POINT('Ctrl Pts',(-10.1107156904836,20.919175710627,12.));
#243131=CARTESIAN_POINT('Ctrl Pts',(-10.1212946487057,20.9318755484734,
12.));
#243132=CARTESIAN_POINT('Ctrl Pts',(-10.1319984827908,20.9446488563933,
12.));
#243133=CARTESIAN_POINT('Ctrl Pts',(-10.1428268017256,20.9574941921591,
12.));
#243134=CARTESIAN_POINT('Ctrl Pts',(-10.1537792192065,20.9704101389369,
12.));
#243135=CARTESIAN_POINT('Ctrl Pts',(-10.1648553534568,20.9833953044736,
12.));
#243136=CARTESIAN_POINT('Ctrl Pts',(-10.1760548270767,20.9964483203686,
12.));
#243137=CARTESIAN_POINT('Ctrl Pts',(-10.187377266936,21.0095678414486,12.));
#243138=CARTESIAN_POINT('Ctrl Pts',(-10.1988223040425,21.0227525451107,
12.));
#243139=CARTESIAN_POINT('Ctrl Pts',(-10.2103895734123,21.0360011306815,
12.));
#243140=CARTESIAN_POINT('Ctrl Pts',(-10.2220787139155,21.0493123187483,
12.));
#243141=CARTESIAN_POINT('Ctrl Pts',(-10.2338893681567,21.0626848505663,
12.));
#243142=CARTESIAN_POINT('Ctrl Pts',(-10.2458211823912,21.0761174875445,
12.));
#243143=CARTESIAN_POINT('Ctrl Pts',(-10.2578738064181,21.0896090107063,
12.));
#243144=CARTESIAN_POINT('Ctrl Pts',(-10.2700468934744,21.1031582201627,
12.));
#243145=CARTESIAN_POINT('Ctrl Pts',(-10.2823401001072,21.1167639345631,
12.));
#243146=CARTESIAN_POINT('Ctrl Pts',(-10.2947530860721,21.1304249906002,
12.));
#243147=CARTESIAN_POINT('Ctrl Pts',(-10.3072855142687,21.1441402425843,
12.));
#243148=CARTESIAN_POINT('Ctrl Pts',(-10.3199370506544,21.1579085619965,
12.));
#243149=CARTESIAN_POINT('Ctrl Pts',(-10.3327073641572,21.1717288370509,
12.));
#243150=CARTESIAN_POINT('Ctrl Pts',(-10.3455961265701,21.1855999722416,
12.));
#243151=CARTESIAN_POINT('Ctrl Pts',(-10.3586030124587,21.199520887919,12.));
#243152=CARTESIAN_POINT('Ctrl Pts',(-10.371727699113,21.2134905199345,12.));
#243153=CARTESIAN_POINT('Ctrl Pts',(-10.3849698664786,21.22750781927,12.));
#243154=CARTESIAN_POINT('Ctrl Pts',(-10.3983291970846,21.2415717516714,
12.));
#243155=CARTESIAN_POINT('Ctrl Pts',(-10.4118053759588,21.255681297275,12.));
#243156=CARTESIAN_POINT('Ctrl Pts',(-10.42539809054,21.2698354502403,12.));
#243157=CARTESIAN_POINT('Ctrl Pts',(-10.4391070306391,21.2840332184483,
12.));
#243158=CARTESIAN_POINT('Ctrl Pts',(-10.4529318883874,21.2982736231931,
12.));
#243159=CARTESIAN_POINT('Ctrl Pts',(-10.4668723581768,21.3125556988731,
12.));
#243160=CARTESIAN_POINT('Ctrl Pts',(-10.4809281365931,21.3268784926819,
12.));
#243161=CARTESIAN_POINT('Ctrl Pts',(-10.4950989223337,21.3412410642904,
12.));
#243162=CARTESIAN_POINT('Ctrl Pts',(-10.5093844161685,21.3556424855814,
12.));
#243163=CARTESIAN_POINT('Ctrl Pts',(-10.5237843209057,21.3700818403936,
12.));
#243164=CARTESIAN_POINT('Ctrl Pts',(-10.5382983413421,21.3845582242602,
12.));
#243165=CARTESIAN_POINT('Ctrl Pts',(-10.5529261842108,21.3990707441497,
12.));
#243166=CARTESIAN_POINT('Ctrl Pts',(-10.5676675581108,21.4136185181979,
12.));
#243167=CARTESIAN_POINT('Ctrl Pts',(-10.5825221734573,21.4282006754631,
12.));
#243168=CARTESIAN_POINT('Ctrl Pts',(-10.5974897424622,21.4428163557144,
12.));
#243169=CARTESIAN_POINT('Ctrl Pts',(-10.6125699790961,21.4574647092097,
12.));
#243170=CARTESIAN_POINT('Ctrl Pts',(-10.6277625990456,21.4721448964766,
12.));
#243171=CARTESIAN_POINT('Ctrl Pts',(-10.6430673196607,21.4868560880889,
12.));
#243172=CARTESIAN_POINT('Ctrl Pts',(-10.6584838598939,21.5015974644449,
12.));
#243173=CARTESIAN_POINT('Ctrl Pts',(-10.6740119402834,21.51636821558,12.));
#243174=CARTESIAN_POINT('Ctrl Pts',(-10.689651282929,21.5311675409807,12.));
#243175=CARTESIAN_POINT('Ctrl Pts',(-10.7054016114571,21.5459946493955,
12.));
#243176=CARTESIAN_POINT('Ctrl Pts',(-10.7212626509816,21.5608487586468,
12.));
#243177=CARTESIAN_POINT('Ctrl Pts',(-10.7372341280467,21.5757290954371,
12.));
#243178=CARTESIAN_POINT('Ctrl Pts',(-10.7533157705941,21.5906348951743,
12.));
#243179=CARTESIAN_POINT('Ctrl Pts',(-10.7695073079552,21.6055654018176,
12.));
#243180=CARTESIAN_POINT('Ctrl Pts',(-10.7858084708261,21.6205198677173,
12.));
#243181=CARTESIAN_POINT('Ctrl Pts',(-10.8022189912369,21.6354975534557,
12.));
#243182=CARTESIAN_POINT('Ctrl Pts',(-10.8187386025136,21.6504977276866,
12.));
#243183=CARTESIAN_POINT('Ctrl Pts',(-10.8353670392272,21.6655196669732,
12.));
#243184=CARTESIAN_POINT('Ctrl Pts',(-10.8521040371835,21.6805626556467,
12.));
#243185=CARTESIAN_POINT('Ctrl Pts',(-10.8689493334095,21.6956259856672,
12.));
#243186=CARTESIAN_POINT('Ctrl Pts',(-10.8859026661293,21.7107089564825,
12.));
#243187=CARTESIAN_POINT('Ctrl Pts',(-10.902963774734,21.7258108748873,12.));
#243188=CARTESIAN_POINT('Ctrl Pts',(-10.9201323997384,21.7409310548797,
12.));
#243189=CARTESIAN_POINT('Ctrl Pts',(-10.9374082827444,21.7560688175247,
12.));
#243190=CARTESIAN_POINT('Ctrl Pts',(-10.9547911664455,21.7712234908464,
12.));
#243191=CARTESIAN_POINT('Ctrl Pts',(-10.9722807946156,21.7863944097141,
12.));
#243192=CARTESIAN_POINT('Ctrl Pts',(-10.9898769120912,21.8015809157301,
12.));
#243193=CARTESIAN_POINT('Ctrl Pts',(-11.0075792647477,21.8167823571168,
12.));
#243194=CARTESIAN_POINT('Ctrl Pts',(-11.0253875994598,21.8319980886033,
12.));
#243195=CARTESIAN_POINT('Ctrl Pts',(-11.0433016640807,21.8472274713103,
12.));
#243196=CARTESIAN_POINT('Ctrl Pts',(-11.0613212074363,21.8624698726318,
12.));
#243197=CARTESIAN_POINT('Ctrl Pts',(-11.0794459793057,21.877724666119,12.));
#243198=CARTESIAN_POINT('Ctrl Pts',(-11.0976757303944,21.8929912313608,
12.));
#243199=CARTESIAN_POINT('Ctrl Pts',(-11.1160102123024,21.9082689538688,
12.));
#243200=CARTESIAN_POINT('Ctrl Pts',(-11.1344491774741,21.923557224952,12.));
#243201=CARTESIAN_POINT('Ctrl Pts',(-11.1529923792003,21.9388554416439,
12.));
#243202=CARTESIAN_POINT('Ctrl Pts',(-11.1716395716376,21.9541630066506,
12.));
#243203=CARTESIAN_POINT('Ctrl Pts',(-11.190390509811,21.9694793282914,12.));
#243204=CARTESIAN_POINT('Ctrl Pts',(-11.2092449496125,21.9848038204439,
12.));
#243205=CARTESIAN_POINT('Ctrl Pts',(-11.2282026477896,22.0001359024839,
12.));
#243206=CARTESIAN_POINT('Ctrl Pts',(-11.2472633619275,22.0154749992363,
12.));
#243207=CARTESIAN_POINT('Ctrl Pts',(-11.2664268504206,22.030820540835,12.));
#243208=CARTESIAN_POINT('Ctrl Pts',(-11.2856928724374,22.046171962566,12.));
#243209=CARTESIAN_POINT('Ctrl Pts',(-11.3050611878771,22.0615287047179,
12.));
#243210=CARTESIAN_POINT('Ctrl Pts',(-11.3245315573168,22.0768902124267,
12.));
#243211=CARTESIAN_POINT('Ctrl Pts',(-11.3441037419553,22.0922559355294,
12.));
#243212=CARTESIAN_POINT('Ctrl Pts',(-11.3637775035367,22.1076253283979,
12.));
#243213=CARTESIAN_POINT('Ctrl Pts',(-11.3835526044256,22.1229978500186,
12.));
#243214=CARTESIAN_POINT('Ctrl Pts',(-11.4034288076908,22.1383729640964,
12.));
#243215=CARTESIAN_POINT('Ctrl Pts',(-11.4234058771742,22.1537501391487,
12.));
#243216=CARTESIAN_POINT('Ctrl Pts',(-11.443483577557,22.1691288486096,12.));
#243217=CARTESIAN_POINT('Ctrl Pts',(-11.463661674411,22.184508570917,12.));
#243218=CARTESIAN_POINT('Ctrl Pts',(-11.483939934259,22.1998887896436,12.));
#243219=CARTESIAN_POINT('Ctrl Pts',(-11.5043181244242,22.2152689931022,
12.));
#243220=CARTESIAN_POINT('Ctrl Pts',(-11.5247960128477,22.2306486738901,
12.));
#243221=CARTESIAN_POINT('Ctrl Pts',(-11.5453733679121,22.2460273284654,
12.));
#243222=CARTESIAN_POINT('Ctrl Pts',(-11.5660499582403,22.2614044566898,
12.));
#243223=CARTESIAN_POINT('Ctrl Pts',(-11.5868255525188,22.2767795614348,
12.));
#243224=CARTESIAN_POINT('Ctrl Pts',(-11.6076999192357,22.2921521480356,
12.));
#243225=CARTESIAN_POINT('Ctrl Pts',(-11.6286728270009,22.3075217249049,
12.));
#243226=CARTESIAN_POINT('Ctrl Pts',(-11.6497440449857,22.3228878043976,
12.));
#243227=CARTESIAN_POINT('Ctrl Pts',(-11.6709133432985,22.3382499035619,
12.));
#243228=CARTESIAN_POINT('Ctrl Pts',(-11.6921804934056,22.3536075450029,
12.));
#243229=CARTESIAN_POINT('Ctrl Pts',(-11.7135452684532,22.3689602575491,
12.));
#243230=CARTESIAN_POINT('Ctrl Pts',(-11.7350074437961,22.3843075773899,
12.));
#243231=CARTESIAN_POINT('Ctrl Pts',(-11.7565667964764,22.3996490469191,
12.));
#243232=CARTESIAN_POINT('Ctrl Pts',(-11.7782231042039,22.4149842125008,
12.));
#243233=CARTESIAN_POINT('Ctrl Pts',(-11.7999761445173,22.430312622646,12.));
#243234=CARTESIAN_POINT('Ctrl Pts',(-11.8218256937889,22.4456338258735,
12.));
#243235=CARTESIAN_POINT('Ctrl Pts',(-11.8437715264487,22.4609473690471,
12.));
#243236=CARTESIAN_POINT('Ctrl Pts',(-11.8658134137019,22.4762527946702,
12.));
#243237=CARTESIAN_POINT('Ctrl Pts',(-11.8879511239943,22.4915496418485,
12.));
#243238=CARTESIAN_POINT('Ctrl Pts',(-11.9101844254557,22.5068374513973,
12.));
#243239=CARTESIAN_POINT('Ctrl Pts',(-11.9325130877803,22.5221157697883,
12.));
#243240=CARTESIAN_POINT('Ctrl Pts',(-11.9549368843997,22.5373841537307,
12.));
#243241=CARTESIAN_POINT('Ctrl Pts',(-11.9774555943496,22.5526421741158,
12.));
#243242=CARTESIAN_POINT('Ctrl Pts',(-12.0000690046695,22.5678894211181,
12.));
#243243=CARTESIAN_POINT('Ctrl Pts',(-12.0227769113127,22.5831255061282,
12.));
#243244=CARTESIAN_POINT('Ctrl Pts',(-12.0455791139128,22.5983500505644,
12.));
#243245=CARTESIAN_POINT('Ctrl Pts',(-12.0684754113862,22.6135626764898,
12.));
#243246=CARTESIAN_POINT('Ctrl Pts',(-12.0914655972823,22.6287629967056,
12.));
#243247=CARTESIAN_POINT('Ctrl Pts',(-12.1145494550383,22.6439506046605,
12.));
#243248=CARTESIAN_POINT('Ctrl Pts',(-12.1377267537145,22.6591250653965,
12.));
#243249=CARTESIAN_POINT('Ctrl Pts',(-12.1609972423099,22.6742859034944,
12.));
#243250=CARTESIAN_POINT('Ctrl Pts',(-12.1843606579262,22.6894326205037,
12.));
#243251=CARTESIAN_POINT('Ctrl Pts',(-12.2078167360284,22.7045647168747,
12.));
#243252=CARTESIAN_POINT('Ctrl Pts',(-12.2313652198061,22.7196817119374,
12.));
#243253=CARTESIAN_POINT('Ctrl Pts',(-12.2550058702395,22.7347831655287,
12.));
#243254=CARTESIAN_POINT('Ctrl Pts',(-12.2787384750742,22.7498686970069,
12.));
#243255=CARTESIAN_POINT('Ctrl Pts',(-12.3025628601792,22.764938010105,12.));
#243256=CARTESIAN_POINT('Ctrl Pts',(-12.3264788926075,22.7799908974768,
12.));
#243257=CARTESIAN_POINT('Ctrl Pts',(-12.3504864740319,22.795027221673,12.));
#243258=CARTESIAN_POINT('Ctrl Pts',(-12.374585536673,22.81004690224,12.));
#243259=CARTESIAN_POINT('Ctrl Pts',(-12.3939379378998,22.8220493007173,
12.));
#243260=CARTESIAN_POINT('Ctrl Pts',(-12.4084933766347,22.8310435872747,
12.));
#243261=CARTESIAN_POINT('Ctrl Pts',(-12.418215285186,22.8370364396459,12.));
#243262=CARTESIAN_POINT('Ctrl Pts',(-12.4230808101438,22.8400320311648,
12.));
#243263=CARTESIAN_POINT('Ctrl Pts',(-7.52250298901264,21.2610617890679,
0.));
#243264=CARTESIAN_POINT('Ctrl Pts',(-7.52250298901264,21.2610617890679,
12.));
#243265=CARTESIAN_POINT('Ctrl Pts',(-7.5225064970397,21.2610673466886,0.));
#243266=CARTESIAN_POINT('Ctrl Pts',(-7.5225064970397,21.2610673466886,12.));
#243267=CARTESIAN_POINT('Ctrl Pts',(-7.52252744144904,21.2611204474866,
0.));
#243268=CARTESIAN_POINT('Ctrl Pts',(-7.52252744144904,21.2611204474866,
12.));
#243269=CARTESIAN_POINT('Ctrl Pts',(-7.52260064231661,21.261326054066,0.));
#243270=CARTESIAN_POINT('Ctrl Pts',(-7.52260064231661,21.261326054066,12.));
#243271=CARTESIAN_POINT('Ctrl Pts',(-7.5227818224267,21.2618521283555,0.));
#243272=CARTESIAN_POINT('Ctrl Pts',(-7.5227818224267,21.2618521283555,12.));
#243273=CARTESIAN_POINT('Ctrl Pts',(-7.52314642316199,21.262927782038,0.));
#243274=CARTESIAN_POINT('Ctrl Pts',(-7.52314642316199,21.262927782038,12.));
#243275=CARTESIAN_POINT('Ctrl Pts',(-7.52364573027553,21.2644161259962,
0.));
#243276=CARTESIAN_POINT('Ctrl Pts',(-7.52364573027553,21.2644161259962,
12.));
#243277=CARTESIAN_POINT('Ctrl Pts',(-7.52427261074298,21.2663059157058,
0.));
#243278=CARTESIAN_POINT('Ctrl Pts',(-7.52427261074298,21.2663059157058,
12.));
#243279=CARTESIAN_POINT('Ctrl Pts',(-7.5250177033353,21.2685823838671,0.));
#243280=CARTESIAN_POINT('Ctrl Pts',(-7.5250177033353,21.2685823838671,12.));
#243281=CARTESIAN_POINT('Ctrl Pts',(-7.5258712609553,21.2712301573466,0.));
#243282=CARTESIAN_POINT('Ctrl Pts',(-7.5258712609553,21.2712301573466,12.));
#243283=CARTESIAN_POINT('Ctrl Pts',(-7.52682526918541,21.2742366113579,
0.));
#243284=CARTESIAN_POINT('Ctrl Pts',(-7.52682526918541,21.2742366113579,
12.));
#243285=CARTESIAN_POINT('Ctrl Pts',(-7.52787386225333,21.2775925269652,
0.));
#243286=CARTESIAN_POINT('Ctrl Pts',(-7.52787386225333,21.2775925269652,
12.));
#243287=CARTESIAN_POINT('Ctrl Pts',(-7.52901217930408,21.2812902781143,
0.));
#243288=CARTESIAN_POINT('Ctrl Pts',(-7.52901217930408,21.2812902781143,
12.));
#243289=CARTESIAN_POINT('Ctrl Pts',(-7.53023562438229,21.2853226580657,
0.));
#243290=CARTESIAN_POINT('Ctrl Pts',(-7.53023562438229,21.2853226580657,
12.));
#243291=CARTESIAN_POINT('Ctrl Pts',(-7.53153906987855,21.2896816163842,
0.));
#243292=CARTESIAN_POINT('Ctrl Pts',(-7.53153906987855,21.2896816163842,
12.));
#243293=CARTESIAN_POINT('Ctrl Pts',(-7.53291726078527,21.2943588989331,
0.));
#243294=CARTESIAN_POINT('Ctrl Pts',(-7.53291726078527,21.2943588989331,
12.));
#243295=CARTESIAN_POINT('Ctrl Pts',(-7.53436505309943,21.2993464250717,
0.));
#243296=CARTESIAN_POINT('Ctrl Pts',(-7.53436505309943,21.2993464250717,
12.));
#243297=CARTESIAN_POINT('Ctrl Pts',(-7.53587778251736,21.3046368712157,
0.));
#243298=CARTESIAN_POINT('Ctrl Pts',(-7.53587778251736,21.3046368712157,
12.));
#243299=CARTESIAN_POINT('Ctrl Pts',(-7.53745129364616,21.310223716773,0.));
#243300=CARTESIAN_POINT('Ctrl Pts',(-7.53745129364616,21.310223716773,12.));
#243301=CARTESIAN_POINT('Ctrl Pts',(-7.53908175169898,21.3161009456256,
0.));
#243302=CARTESIAN_POINT('Ctrl Pts',(-7.53908175169898,21.3161009456256,
12.));
#243303=CARTESIAN_POINT('Ctrl Pts',(-7.54076552038279,21.3222628524165,
0.));
#243304=CARTESIAN_POINT('Ctrl Pts',(-7.54076552038279,21.3222628524165,
12.));
#243305=CARTESIAN_POINT('Ctrl Pts',(-7.54249900377031,21.328703791771,0.));
#243306=CARTESIAN_POINT('Ctrl Pts',(-7.54249900377031,21.328703791771,12.));
#243307=CARTESIAN_POINT('Ctrl Pts',(-7.54427868151268,21.3354182340149,
0.));
#243308=CARTESIAN_POINT('Ctrl Pts',(-7.54427868151268,21.3354182340149,
12.));
#243309=CARTESIAN_POINT('Ctrl Pts',(-7.54610114948347,21.3424008295038,
0.));
#243310=CARTESIAN_POINT('Ctrl Pts',(-7.54610114948347,21.3424008295038,
12.));
#243311=CARTESIAN_POINT('Ctrl Pts',(-7.5479631624633,21.3496464761531,0.));
#243312=CARTESIAN_POINT('Ctrl Pts',(-7.5479631624633,21.3496464761531,12.));
#243313=CARTESIAN_POINT('Ctrl Pts',(-7.5498616652131,21.3571503685855,0.));
#243314=CARTESIAN_POINT('Ctrl Pts',(-7.5498616652131,21.3571503685855,12.));
#243315=CARTESIAN_POINT('Ctrl Pts',(-7.55179375777444,21.3649079431865,
0.));
#243316=CARTESIAN_POINT('Ctrl Pts',(-7.55179375777444,21.3649079431865,
12.));
#243317=CARTESIAN_POINT('Ctrl Pts',(-7.55375667080029,21.3729148390243,
0.));
#243318=CARTESIAN_POINT('Ctrl Pts',(-7.55375667080029,21.3729148390243,
12.));
#243319=CARTESIAN_POINT('Ctrl Pts',(-7.55574773403503,21.3811668478932,
0.));
#243320=CARTESIAN_POINT('Ctrl Pts',(-7.55574773403503,21.3811668478932,
12.));
#243321=CARTESIAN_POINT('Ctrl Pts',(-7.55776435731417,21.3896598842117,
0.));
#243322=CARTESIAN_POINT('Ctrl Pts',(-7.55776435731417,21.3896598842117,
12.));
#243323=CARTESIAN_POINT('Ctrl Pts',(-7.55980403700611,21.3983899952987,
0.));
#243324=CARTESIAN_POINT('Ctrl Pts',(-7.55980403700611,21.3983899952987,
12.));
#243325=CARTESIAN_POINT('Ctrl Pts',(-7.56186435703622,21.4073533630365,
0.));
#243326=CARTESIAN_POINT('Ctrl Pts',(-7.56186435703622,21.4073533630365,
12.));
#243327=CARTESIAN_POINT('Ctrl Pts',(-7.56394299313685,21.4165463106254,
0.));
#243328=CARTESIAN_POINT('Ctrl Pts',(-7.56394299313685,21.4165463106254,
12.));
#243329=CARTESIAN_POINT('Ctrl Pts',(-7.56603771218712,21.4259653015736,
0.));
#243330=CARTESIAN_POINT('Ctrl Pts',(-7.56603771218712,21.4259653015736,
12.));
#243331=CARTESIAN_POINT('Ctrl Pts',(-7.56814636360847,21.4356069261513,
0.));
#243332=CARTESIAN_POINT('Ctrl Pts',(-7.56814636360847,21.4356069261513,
12.));
#243333=CARTESIAN_POINT('Ctrl Pts',(-7.57026687261166,21.4454678907509,
0.));
#243334=CARTESIAN_POINT('Ctrl Pts',(-7.57026687261166,21.4454678907509,
12.));
#243335=CARTESIAN_POINT('Ctrl Pts',(-7.57239723223506,21.4555450053142,
0.));
#243336=CARTESIAN_POINT('Ctrl Pts',(-7.57239723223506,21.4555450053142,
12.));
#243337=CARTESIAN_POINT('Ctrl Pts',(-7.57453549743412,21.4658351740128,
0.));
#243338=CARTESIAN_POINT('Ctrl Pts',(-7.57453549743412,21.4658351740128,
12.));
#243339=CARTESIAN_POINT('Ctrl Pts',(-7.57667978402987,21.4763353936762,
0.));
#243340=CARTESIAN_POINT('Ctrl Pts',(-7.57667978402987,21.4763353936762,
12.));
#243341=CARTESIAN_POINT('Ctrl Pts',(-7.57882826679132,21.4870427508194,
0.));
#243342=CARTESIAN_POINT('Ctrl Pts',(-7.57882826679132,21.4870427508194,
12.));
#243343=CARTESIAN_POINT('Ctrl Pts',(-7.58097917790744,21.4979544192744,
0.));
#243344=CARTESIAN_POINT('Ctrl Pts',(-7.58097917790744,21.4979544192744,
12.));
#243345=CARTESIAN_POINT('Ctrl Pts',(-7.5831308051918,21.5090676573873,0.));
#243346=CARTESIAN_POINT('Ctrl Pts',(-7.5831308051918,21.5090676573873,12.));
#243347=CARTESIAN_POINT('Ctrl Pts',(-7.5852814891913,21.5203798035299,0.));
#243348=CARTESIAN_POINT('Ctrl Pts',(-7.5852814891913,21.5203798035299,12.));
#243349=CARTESIAN_POINT('Ctrl Pts',(-7.58742962034834,21.5318882716736,
0.));
#243350=CARTESIAN_POINT('Ctrl Pts',(-7.58742962034834,21.5318882716736,
12.));
#243351=CARTESIAN_POINT('Ctrl Pts',(-7.58957363620014,21.543590547011,0.));
#243352=CARTESIAN_POINT('Ctrl Pts',(-7.58957363620014,21.543590547011,12.));
#243353=CARTESIAN_POINT('Ctrl Pts',(-7.59171201844777,21.5554841813462,
0.));
#243354=CARTESIAN_POINT('Ctrl Pts',(-7.59171201844777,21.5554841813462,
12.));
#243355=CARTESIAN_POINT('Ctrl Pts',(-7.59384329124918,21.5675667904726,
0.));
#243356=CARTESIAN_POINT('Ctrl Pts',(-7.59384329124918,21.5675667904726,
12.));
#243357=CARTESIAN_POINT('Ctrl Pts',(-7.59596601973584,21.5798360518978,
0.));
#243358=CARTESIAN_POINT('Ctrl Pts',(-7.59596601973584,21.5798360518978,
12.));
#243359=CARTESIAN_POINT('Ctrl Pts',(-7.59807880846195,21.5922897024466,
0.));
#243360=CARTESIAN_POINT('Ctrl Pts',(-7.59807880846195,21.5922897024466,
12.));
#243361=CARTESIAN_POINT('Ctrl Pts',(-7.60018029988241,21.6049255358843,
0.));
#243362=CARTESIAN_POINT('Ctrl Pts',(-7.60018029988241,21.6049255358843,
12.));
#243363=CARTESIAN_POINT('Ctrl Pts',(-7.60226917285429,21.617741400599,0.));
#243364=CARTESIAN_POINT('Ctrl Pts',(-7.60226917285429,21.617741400599,12.));
#243365=CARTESIAN_POINT('Ctrl Pts',(-7.60434414118296,21.6307351973822,
0.));
#243366=CARTESIAN_POINT('Ctrl Pts',(-7.60434414118296,21.6307351973822,
12.));
#243367=CARTESIAN_POINT('Ctrl Pts',(-7.60640395216357,21.6439048771743,
0.));
#243368=CARTESIAN_POINT('Ctrl Pts',(-7.60640395216357,21.6439048771743,
12.));
#243369=CARTESIAN_POINT('Ctrl Pts',(-7.60844738512874,21.6572484388081,
0.));
#243370=CARTESIAN_POINT('Ctrl Pts',(-7.60844738512874,21.6572484388081,
12.));
#243371=CARTESIAN_POINT('Ctrl Pts',(-7.61047325000956,21.6707639267576,
0.));
#243372=CARTESIAN_POINT('Ctrl Pts',(-7.61047325000956,21.6707639267576,
12.));
#243373=CARTESIAN_POINT('Ctrl Pts',(-7.61248038630268,21.6844494295815,
0.));
#243374=CARTESIAN_POINT('Ctrl Pts',(-7.61248038630268,21.6844494295815,
12.));
#243375=CARTESIAN_POINT('Ctrl Pts',(-7.61446766202787,21.6983030783322,
0.));
#243376=CARTESIAN_POINT('Ctrl Pts',(-7.61446766202787,21.6983030783322,
12.));
#243377=CARTESIAN_POINT('Ctrl Pts',(-7.61643397270421,21.7123230449834,
0.));
#243378=CARTESIAN_POINT('Ctrl Pts',(-7.61643397270421,21.7123230449834,
12.));
#243379=CARTESIAN_POINT('Ctrl Pts',(-7.61837824030538,21.7265075407975,
0.));
#243380=CARTESIAN_POINT('Ctrl Pts',(-7.61837824030538,21.7265075407975,
12.));
#243381=CARTESIAN_POINT('Ctrl Pts',(-7.62029941230855,21.7408548148656,
0.));
#243382=CARTESIAN_POINT('Ctrl Pts',(-7.62029941230855,21.7408548148656,
12.));
#243383=CARTESIAN_POINT('Ctrl Pts',(-7.62219646084228,21.7553631528328,
0.));
#243384=CARTESIAN_POINT('Ctrl Pts',(-7.62219646084228,21.7553631528328,
12.));
#243385=CARTESIAN_POINT('Ctrl Pts',(-7.62406838181166,21.7700308755584,
0.));
#243386=CARTESIAN_POINT('Ctrl Pts',(-7.62406838181166,21.7700308755584,
12.));
#243387=CARTESIAN_POINT('Ctrl Pts',(-7.62591419404512,21.7848563378021,
0.));
#243388=CARTESIAN_POINT('Ctrl Pts',(-7.62591419404512,21.7848563378021,
12.));
#243389=CARTESIAN_POINT('Ctrl Pts',(-7.62773293842389,21.799837926858,0.));
#243390=CARTESIAN_POINT('Ctrl Pts',(-7.62773293842389,21.799837926858,12.));
#243391=CARTESIAN_POINT('Ctrl Pts',(-7.62952367718127,21.814974061509,0.));
#243392=CARTESIAN_POINT('Ctrl Pts',(-7.62952367718127,21.814974061509,12.));
#243393=CARTESIAN_POINT('Ctrl Pts',(-7.63128549323023,21.8302631910195,
0.));
#243394=CARTESIAN_POINT('Ctrl Pts',(-7.63128549323023,21.8302631910195,
12.));
#243395=CARTESIAN_POINT('Ctrl Pts',(-7.63301748948936,21.8457037941084,
0.));
#243396=CARTESIAN_POINT('Ctrl Pts',(-7.63301748948936,21.8457037941084,
12.));
#243397=CARTESIAN_POINT('Ctrl Pts',(-7.63471878821226,21.8612943779089,
0.));
#243398=CARTESIAN_POINT('Ctrl Pts',(-7.63471878821226,21.8612943779089,
12.));
#243399=CARTESIAN_POINT('Ctrl Pts',(-7.636388530334,21.8770334769496,0.));
#243400=CARTESIAN_POINT('Ctrl Pts',(-7.636388530334,21.8770334769496,12.));
#243401=CARTESIAN_POINT('Ctrl Pts',(-7.63802587492035,21.8929196523514,
0.));
#243402=CARTESIAN_POINT('Ctrl Pts',(-7.63802587492035,21.8929196523514,
12.));
#243403=CARTESIAN_POINT('Ctrl Pts',(-7.63962999860927,21.9089514909874,
0.));
#243404=CARTESIAN_POINT('Ctrl Pts',(-7.63962999860927,21.9089514909874,
12.));
#243405=CARTESIAN_POINT('Ctrl Pts',(-7.64120009506532,21.9251276046546,
0.));
#243406=CARTESIAN_POINT('Ctrl Pts',(-7.64120009506532,21.9251276046546,
12.));
#243407=CARTESIAN_POINT('Ctrl Pts',(-7.64273537442682,21.9414466292072,
0.));
#243408=CARTESIAN_POINT('Ctrl Pts',(-7.64273537442682,21.9414466292072,
12.));
#243409=CARTESIAN_POINT('Ctrl Pts',(-7.64423506279123,21.9579072237651,
0.));
#243410=CARTESIAN_POINT('Ctrl Pts',(-7.64423506279123,21.9579072237651,
12.));
#243411=CARTESIAN_POINT('Ctrl Pts',(-7.64569840177336,21.9745080700798,
0.));
#243412=CARTESIAN_POINT('Ctrl Pts',(-7.64569840177336,21.9745080700798,
12.));
#243413=CARTESIAN_POINT('Ctrl Pts',(-7.6471246480525,21.9912478718542,0.));
#243414=CARTESIAN_POINT('Ctrl Pts',(-7.6471246480525,21.9912478718542,12.));
#243415=CARTESIAN_POINT('Ctrl Pts',(-7.64851307293352,22.0081253540774,
0.));
#243416=CARTESIAN_POINT('Ctrl Pts',(-7.64851307293352,22.0081253540774,
12.));
#243417=CARTESIAN_POINT('Ctrl Pts',(-7.64986296190168,22.0251392623209,
0.));
#243418=CARTESIAN_POINT('Ctrl Pts',(-7.64986296190168,22.0251392623209,
12.));
#243419=CARTESIAN_POINT('Ctrl Pts',(-7.65117361421358,22.0422883621174,
0.));
#243420=CARTESIAN_POINT('Ctrl Pts',(-7.65117361421358,22.0422883621174,
12.));
#243421=CARTESIAN_POINT('Ctrl Pts',(-7.65244434253113,22.0595714384431,
0.));
#243422=CARTESIAN_POINT('Ctrl Pts',(-7.65244434253113,22.0595714384431,
12.));
#243423=CARTESIAN_POINT('Ctrl Pts',(-7.65367447254949,22.0769872951596,
0.));
#243424=CARTESIAN_POINT('Ctrl Pts',(-7.65367447254949,22.0769872951596,
12.));
#243425=CARTESIAN_POINT('Ctrl Pts',(-7.65486334263644,22.094534754469,0.));
#243426=CARTESIAN_POINT('Ctrl Pts',(-7.65486334263644,22.094534754469,12.));
#243427=CARTESIAN_POINT('Ctrl Pts',(-7.65601030346807,22.1122126563329,
0.));
#243428=CARTESIAN_POINT('Ctrl Pts',(-7.65601030346807,22.1122126563329,
12.));
#243429=CARTESIAN_POINT('Ctrl Pts',(-7.65711471769397,22.1300198579675,
0.));
#243430=CARTESIAN_POINT('Ctrl Pts',(-7.65711471769397,22.1300198579675,
12.));
#243431=CARTESIAN_POINT('Ctrl Pts',(-7.65817595963349,22.1479552334211,
0.));
#243432=CARTESIAN_POINT('Ctrl Pts',(-7.65817595963349,22.1479552334211,
12.));
#243433=CARTESIAN_POINT('Ctrl Pts',(-7.6591934149693,22.1660176731178,0.));
#243434=CARTESIAN_POINT('Ctrl Pts',(-7.6591934149693,22.1660176731178,12.));
#243435=CARTESIAN_POINT('Ctrl Pts',(-7.66016648045005,22.1842060834091,
0.));
#243436=CARTESIAN_POINT('Ctrl Pts',(-7.66016648045005,22.1842060834091,
12.));
#243437=CARTESIAN_POINT('Ctrl Pts',(-7.66109456359271,22.2025193860964,
0.));
#243438=CARTESIAN_POINT('Ctrl Pts',(-7.66109456359271,22.2025193860964,
12.));
#243439=CARTESIAN_POINT('Ctrl Pts',(-7.661977082404,22.2209565180085,0.));
#243440=CARTESIAN_POINT('Ctrl Pts',(-7.661977082404,22.2209565180085,12.));
#243441=CARTESIAN_POINT('Ctrl Pts',(-7.66281346512509,22.2395164306547,
0.));
#243442=CARTESIAN_POINT('Ctrl Pts',(-7.66281346512509,22.2395164306547,
12.));
#243443=CARTESIAN_POINT('Ctrl Pts',(-7.66360314997641,22.258198089848,0.));
#243444=CARTESIAN_POINT('Ctrl Pts',(-7.66360314997641,22.258198089848,12.));
#243445=CARTESIAN_POINT('Ctrl Pts',(-7.66434558490979,22.2770004753335,
0.));
#243446=CARTESIAN_POINT('Ctrl Pts',(-7.66434558490979,22.2770004753335,
12.));
#243447=CARTESIAN_POINT('Ctrl Pts',(-7.66504022736299,22.2959225803937,
0.));
#243448=CARTESIAN_POINT('Ctrl Pts',(-7.66504022736299,22.2959225803937,
12.));
#243449=CARTESIAN_POINT('Ctrl Pts',(-7.66568654402494,22.314963411484,0.));
#243450=CARTESIAN_POINT('Ctrl Pts',(-7.66568654402494,22.314963411484,12.));
#243451=CARTESIAN_POINT('Ctrl Pts',(-7.66628401061952,22.3341219879469,
0.));
#243452=CARTESIAN_POINT('Ctrl Pts',(-7.66628401061952,22.3341219879469,
12.));
#243453=CARTESIAN_POINT('Ctrl Pts',(-7.66683211169158,22.3533973417021,
0.));
#243454=CARTESIAN_POINT('Ctrl Pts',(-7.66683211169158,22.3533973417021,
12.));
#243455=CARTESIAN_POINT('Ctrl Pts',(-7.66733034039883,22.372788516936,0.));
#243456=CARTESIAN_POINT('Ctrl Pts',(-7.66733034039883,22.372788516936,12.));
#243457=CARTESIAN_POINT('Ctrl Pts',(-7.6677781983079,22.3922945697773,0.));
#243458=CARTESIAN_POINT('Ctrl Pts',(-7.6677781983079,22.3922945697773,12.));
#243459=CARTESIAN_POINT('Ctrl Pts',(-7.6681751951964,22.4119145679758,0.));
#243460=CARTESIAN_POINT('Ctrl Pts',(-7.6681751951964,22.4119145679758,12.));
#243461=CARTESIAN_POINT('Ctrl Pts',(-7.66852084886704,22.4316475906603,
0.));
#243462=CARTESIAN_POINT('Ctrl Pts',(-7.66852084886704,22.4316475906603,
12.));
#243463=CARTESIAN_POINT('Ctrl Pts',(-7.66881468496635,22.4514927280855,
0.));
#243464=CARTESIAN_POINT('Ctrl Pts',(-7.66881468496635,22.4514927280855,
12.));
#243465=CARTESIAN_POINT('Ctrl Pts',(-7.66905623680831,22.47144908137,0.));
#243466=CARTESIAN_POINT('Ctrl Pts',(-7.66905623680831,22.47144908137,12.));
#243467=CARTESIAN_POINT('Ctrl Pts',(-7.66924504520315,22.4915157622312,
0.));
#243468=CARTESIAN_POINT('Ctrl Pts',(-7.66924504520315,22.4915157622312,
12.));
#243469=CARTESIAN_POINT('Ctrl Pts',(-7.66938065829108,22.5116918927031,
0.));
#243470=CARTESIAN_POINT('Ctrl Pts',(-7.66938065829108,22.5116918927031,
12.));
#243471=CARTESIAN_POINT('Ctrl Pts',(-7.66946263138144,22.53197660492,0.));
#243472=CARTESIAN_POINT('Ctrl Pts',(-7.66946263138144,22.53197660492,12.));
#243473=CARTESIAN_POINT('Ctrl Pts',(-7.66949052679693,22.5523690409116,
0.));
#243474=CARTESIAN_POINT('Ctrl Pts',(-7.66949052679693,22.5523690409116,
12.));
#243475=CARTESIAN_POINT('Ctrl Pts',(-7.66946391372306,22.5728683523831,
0.));
#243476=CARTESIAN_POINT('Ctrl Pts',(-7.66946391372306,22.5728683523831,
12.));
#243477=CARTESIAN_POINT('Ctrl Pts',(-7.66938236806233,22.5934737004953,
0.));
#243478=CARTESIAN_POINT('Ctrl Pts',(-7.66938236806233,22.5934737004953,
12.));
#243479=CARTESIAN_POINT('Ctrl Pts',(-7.66924547229414,22.6141842556243,
0.));
#243480=CARTESIAN_POINT('Ctrl Pts',(-7.66924547229414,22.6141842556243,
12.));
#243481=CARTESIAN_POINT('Ctrl Pts',(-7.66905281533715,22.6349991971541,
0.));
#243482=CARTESIAN_POINT('Ctrl Pts',(-7.66905281533715,22.6349991971541,
12.));
#243483=CARTESIAN_POINT('Ctrl Pts',(-7.66880399241323,22.6559177133127,
0.));
#243484=CARTESIAN_POINT('Ctrl Pts',(-7.66880399241323,22.6559177133127,
12.));
#243485=CARTESIAN_POINT('Ctrl Pts',(-7.66849860491743,22.6769390009885,
0.));
#243486=CARTESIAN_POINT('Ctrl Pts',(-7.66849860491743,22.6769390009885,
12.));
#243487=CARTESIAN_POINT('Ctrl Pts',(-7.66813626029275,22.6980622655446,
0.));
#243488=CARTESIAN_POINT('Ctrl Pts',(-7.66813626029275,22.6980622655446,
12.));
#243489=CARTESIAN_POINT('Ctrl Pts',(-7.66771657191027,22.7192867206245,
0.));
#243490=CARTESIAN_POINT('Ctrl Pts',(-7.66771657191027,22.7192867206245,
12.));
#243491=CARTESIAN_POINT('Ctrl Pts',(-7.6672391589544,22.7406115879513,0.));
#243492=CARTESIAN_POINT('Ctrl Pts',(-7.6672391589544,22.7406115879513,12.));
#243493=CARTESIAN_POINT('Ctrl Pts',(-7.66670364630299,22.7620360971843,
0.));
#243494=CARTESIAN_POINT('Ctrl Pts',(-7.66670364630299,22.7620360971843,
12.));
#243495=CARTESIAN_POINT('Ctrl Pts',(-7.66610966441273,22.7835594857699,
0.));
#243496=CARTESIAN_POINT('Ctrl Pts',(-7.66610966441273,22.7835594857699,
12.));
#243497=CARTESIAN_POINT('Ctrl Pts',(-7.66545684920987,22.8051809987833,
0.));
#243498=CARTESIAN_POINT('Ctrl Pts',(-7.66545684920987,22.8051809987833,
12.));
#243499=CARTESIAN_POINT('Ctrl Pts',(-7.66474484198549,22.8268998887678,
0.));
#243500=CARTESIAN_POINT('Ctrl Pts',(-7.66474484198549,22.8268998887678,
12.));
#243501=CARTESIAN_POINT('Ctrl Pts',(-7.66397328929803,22.848715415557,0.));
#243502=CARTESIAN_POINT('Ctrl Pts',(-7.66397328929803,22.848715415557,12.));
#243503=CARTESIAN_POINT('Ctrl Pts',(-7.66314184287337,22.8706268461283,
0.));
#243504=CARTESIAN_POINT('Ctrl Pts',(-7.66314184287337,22.8706268461283,
12.));
#243505=CARTESIAN_POINT('Ctrl Pts',(-7.66225015950156,22.8926334544883,
0.));
#243506=CARTESIAN_POINT('Ctrl Pts',(-7.66225015950156,22.8926334544883,
12.));
#243507=CARTESIAN_POINT('Ctrl Pts',(-7.66129790094108,22.9147345215421,
0.));
#243508=CARTESIAN_POINT('Ctrl Pts',(-7.66129790094108,22.9147345215421,
12.));
#243509=CARTESIAN_POINT('Ctrl Pts',(-7.66028473382778,22.9369293349593,
0.));
#243510=CARTESIAN_POINT('Ctrl Pts',(-7.66028473382778,22.9369293349593,
12.));
#243511=CARTESIAN_POINT('Ctrl Pts',(-7.65921032958902,22.959217189033,0.));
#243512=CARTESIAN_POINT('Ctrl Pts',(-7.65921032958902,22.959217189033,12.));
#243513=CARTESIAN_POINT('Ctrl Pts',(-7.65807436436432,22.9815973845296,
0.));
#243514=CARTESIAN_POINT('Ctrl Pts',(-7.65807436436432,22.9815973845296,
12.));
#243515=CARTESIAN_POINT('Ctrl Pts',(-7.65687651891304,23.0040692285814,
0.));
#243516=CARTESIAN_POINT('Ctrl Pts',(-7.65687651891304,23.0040692285814,
12.));
#243517=CARTESIAN_POINT('Ctrl Pts',(-7.65561647852534,23.0266320345787,
0.));
#243518=CARTESIAN_POINT('Ctrl Pts',(-7.65561647852534,23.0266320345787,
12.));
#243519=CARTESIAN_POINT('Ctrl Pts',(-7.65429393293946,23.0492851220528,
0.));
#243520=CARTESIAN_POINT('Ctrl Pts',(-7.65429393293946,23.0492851220528,
12.));
#243521=CARTESIAN_POINT('Ctrl Pts',(-7.65290857626358,23.072027816555,0.));
#243522=CARTESIAN_POINT('Ctrl Pts',(-7.65290857626358,23.072027816555,12.));
#243523=CARTESIAN_POINT('Ctrl Pts',(-7.65146010690476,23.094859449525,0.));
#243524=CARTESIAN_POINT('Ctrl Pts',(-7.65146010690476,23.094859449525,12.));
#243525=CARTESIAN_POINT('Ctrl Pts',(-7.6499482274986,23.1177793581679,0.));
#243526=CARTESIAN_POINT('Ctrl Pts',(-7.6499482274986,23.1177793581679,12.));
#243527=CARTESIAN_POINT('Ctrl Pts',(-7.64837264482943,23.1407868853819,
0.));
#243528=CARTESIAN_POINT('Ctrl Pts',(-7.64837264482943,23.1407868853819,
12.));
#243529=CARTESIAN_POINT('Ctrl Pts',(-7.64673306975805,23.1638813796694,
0.));
#243530=CARTESIAN_POINT('Ctrl Pts',(-7.64673306975805,23.1638813796694,
12.));
#243531=CARTESIAN_POINT('Ctrl Pts',(-7.64502921715483,23.1870621950452,
0.));
#243532=CARTESIAN_POINT('Ctrl Pts',(-7.64502921715483,23.1870621950452,
12.));
#243533=CARTESIAN_POINT('Ctrl Pts',(-7.6432608058368,23.2103286909398,0.));
#243534=CARTESIAN_POINT('Ctrl Pts',(-7.6432608058368,23.2103286909398,12.));
#243535=CARTESIAN_POINT('Ctrl Pts',(-7.64142755851504,23.2336802320912,
0.));
#243536=CARTESIAN_POINT('Ctrl Pts',(-7.64142755851504,23.2336802320912,
12.));
#243537=CARTESIAN_POINT('Ctrl Pts',(-7.63952920172835,23.2571161884488,
0.));
#243538=CARTESIAN_POINT('Ctrl Pts',(-7.63952920172835,23.2571161884488,
12.));
#243539=CARTESIAN_POINT('Ctrl Pts',(-7.63756546576374,23.2806359350855,
0.));
#243540=CARTESIAN_POINT('Ctrl Pts',(-7.63756546576374,23.2806359350855,
12.));
#243541=CARTESIAN_POINT('Ctrl Pts',(-7.63553608458783,23.3042388521022,
0.));
#243542=CARTESIAN_POINT('Ctrl Pts',(-7.63553608458783,23.3042388521022,
12.));
#243543=CARTESIAN_POINT('Ctrl Pts',(-7.63344079578161,23.3279243245241,
0.));
#243544=CARTESIAN_POINT('Ctrl Pts',(-7.63344079578161,23.3279243245241,
12.));
#243545=CARTESIAN_POINT('Ctrl Pts',(-7.63127934048136,23.3516917421972,
0.));
#243546=CARTESIAN_POINT('Ctrl Pts',(-7.63127934048136,23.3516917421972,
12.));
#243547=CARTESIAN_POINT('Ctrl Pts',(-7.62905146332593,23.3755404996636,
0.));
#243548=CARTESIAN_POINT('Ctrl Pts',(-7.62905146332593,23.3755404996636,
12.));
#243549=CARTESIAN_POINT('Ctrl Pts',(-7.62675691240329,23.399469996112,0.));
#243550=CARTESIAN_POINT('Ctrl Pts',(-7.62675691240329,23.399469996112,12.));
#243551=CARTESIAN_POINT('Ctrl Pts',(-7.6243954392005,23.4234796353542,0.));
#243552=CARTESIAN_POINT('Ctrl Pts',(-7.6243954392005,23.4234796353542,12.));
#243553=CARTESIAN_POINT('Ctrl Pts',(-7.62196679855955,23.4475688257854,
0.));
#243554=CARTESIAN_POINT('Ctrl Pts',(-7.62196679855955,23.4475688257854,
12.));
#243555=CARTESIAN_POINT('Ctrl Pts',(-7.61947074863977,23.4717369803438,
0.));
#243556=CARTESIAN_POINT('Ctrl Pts',(-7.61947074863977,23.4717369803438,
12.));
#243557=CARTESIAN_POINT('Ctrl Pts',(-7.61690705088319,23.4959835164609,
0.));
#243558=CARTESIAN_POINT('Ctrl Pts',(-7.61690705088319,23.4959835164609,
12.));
#243559=CARTESIAN_POINT('Ctrl Pts',(-7.61427546999298,23.5203078560129,
0.));
#243560=CARTESIAN_POINT('Ctrl Pts',(-7.61427546999298,23.5203078560129,
12.));
#243561=CARTESIAN_POINT('Ctrl Pts',(-7.61157577385372,23.544709425203,0.));
#243562=CARTESIAN_POINT('Ctrl Pts',(-7.61157577385372,23.544709425203,12.));
#243563=CARTESIAN_POINT('Ctrl Pts',(-7.608807733446,23.5691876544244,0.));
#243564=CARTESIAN_POINT('Ctrl Pts',(-7.608807733446,23.5691876544244,12.));
#243565=CARTESIAN_POINT('Ctrl Pts',(-7.60597112277094,23.5937419781245,
0.));
#243566=CARTESIAN_POINT('Ctrl Pts',(-7.60597112277094,23.5937419781245,
12.));
#243567=CARTESIAN_POINT('Ctrl Pts',(-7.60306571877806,23.6183718346576,
0.));
#243568=CARTESIAN_POINT('Ctrl Pts',(-7.60306571877806,23.6183718346576,
12.));
#243569=CARTESIAN_POINT('Ctrl Pts',(-7.60009130130126,23.6430766661418,
0.));
#243570=CARTESIAN_POINT('Ctrl Pts',(-7.60009130130126,23.6430766661418,
12.));
#243571=CARTESIAN_POINT('Ctrl Pts',(-7.59704765299567,23.6678559182875,
0.));
#243572=CARTESIAN_POINT('Ctrl Pts',(-7.59704765299567,23.6678559182875,
12.));
#243573=CARTESIAN_POINT('Ctrl Pts',(-7.59393455934035,23.6927090405066,
0.));
#243574=CARTESIAN_POINT('Ctrl Pts',(-7.59393455934035,23.6927090405066,
12.));
#243575=CARTESIAN_POINT('Ctrl Pts',(-7.5907518086532,23.7176354860456,0.));
#243576=CARTESIAN_POINT('Ctrl Pts',(-7.5907518086532,23.7176354860456,12.));
#243577=CARTESIAN_POINT('Ctrl Pts',(-7.58749919210826,23.7426347121006,
0.));
#243578=CARTESIAN_POINT('Ctrl Pts',(-7.58749919210826,23.7426347121006,
12.));
#243579=CARTESIAN_POINT('Ctrl Pts',(-7.58417650376271,23.7677061799376,
0.));
#243580=CARTESIAN_POINT('Ctrl Pts',(-7.58417650376271,23.7677061799376,
12.));
#243581=CARTESIAN_POINT('Ctrl Pts',(-7.58078354058213,23.7928493549908,
0.));
#243582=CARTESIAN_POINT('Ctrl Pts',(-7.58078354058213,23.7928493549908,
12.));
#243583=CARTESIAN_POINT('Ctrl Pts',(-7.57732010249066,23.8180637069976,
0.));
#243584=CARTESIAN_POINT('Ctrl Pts',(-7.57732010249066,23.8180637069976,
12.));
#243585=CARTESIAN_POINT('Ctrl Pts',(-7.57378599219814,23.8433487096132,
0.));
#243586=CARTESIAN_POINT('Ctrl Pts',(-7.57378599219814,23.8433487096132,
12.));
#243587=CARTESIAN_POINT('Ctrl Pts',(-7.57018101500709,23.8687038399595,
0.));
#243588=CARTESIAN_POINT('Ctrl Pts',(-7.57018101500709,23.8687038399595,
12.));
#243589=CARTESIAN_POINT('Ctrl Pts',(-7.56650497863791,23.8941285782002,
0.));
#243590=CARTESIAN_POINT('Ctrl Pts',(-7.56650497863791,23.8941285782002,
12.));
#243591=CARTESIAN_POINT('Ctrl Pts',(-7.56275769304773,23.9196224070759,
0.));
#243592=CARTESIAN_POINT('Ctrl Pts',(-7.56275769304773,23.9196224070759,
12.));
#243593=CARTESIAN_POINT('Ctrl Pts',(-7.5589389702768,23.9451848115002,0.));
#243594=CARTESIAN_POINT('Ctrl Pts',(-7.5589389702768,23.9451848115002,12.));
#243595=CARTESIAN_POINT('Ctrl Pts',(-7.55504862424808,23.9708152779886,
0.));
#243596=CARTESIAN_POINT('Ctrl Pts',(-7.55504862424808,23.9708152779886,
12.));
#243597=CARTESIAN_POINT('Ctrl Pts',(-7.55108647097432,23.9965132953187,
0.));
#243598=CARTESIAN_POINT('Ctrl Pts',(-7.55108647097432,23.9965132953187,
12.));
#243599=CARTESIAN_POINT('Ctrl Pts',(-7.54705232885895,24.0222783554531,
0.));
#243600=CARTESIAN_POINT('Ctrl Pts',(-7.54705232885895,24.0222783554531,
12.));
#243601=CARTESIAN_POINT('Ctrl Pts',(-7.54294601896128,24.0481099543353,
0.));
#243602=CARTESIAN_POINT('Ctrl Pts',(-7.54294601896128,24.0481099543353,
12.));
#243603=CARTESIAN_POINT('Ctrl Pts',(-7.53876736531005,24.0740075927984,
0.));
#243604=CARTESIAN_POINT('Ctrl Pts',(-7.53876736531005,24.0740075927984,
12.));
#243605=CARTESIAN_POINT('Ctrl Pts',(-7.53451619514658,24.0999707772643,
0.));
#243606=CARTESIAN_POINT('Ctrl Pts',(-7.53451619514658,24.0999707772643,
12.));
#243607=CARTESIAN_POINT('Ctrl Pts',(-7.53019233935536,24.1259990209211,
0.));
#243608=CARTESIAN_POINT('Ctrl Pts',(-7.53019233935536,24.1259990209211,
12.));
#243609=CARTESIAN_POINT('Ctrl Pts',(-7.52579563201479,24.152091842537,0.));
#243610=CARTESIAN_POINT('Ctrl Pts',(-7.52579563201479,24.152091842537,12.));
#243611=CARTESIAN_POINT('Ctrl Pts',(-7.52132590953862,24.1782487641602,
0.));
#243612=CARTESIAN_POINT('Ctrl Pts',(-7.52132590953862,24.1782487641602,
12.));
#243613=CARTESIAN_POINT('Ctrl Pts',(-7.51678300997998,24.2044693092356,
0.));
#243614=CARTESIAN_POINT('Ctrl Pts',(-7.51678300997998,24.2044693092356,
12.));
#243615=CARTESIAN_POINT('Ctrl Pts',(-7.51216677222199,24.230753000389,0.));
#243616=CARTESIAN_POINT('Ctrl Pts',(-7.51216677222199,24.230753000389,12.));
#243617=CARTESIAN_POINT('Ctrl Pts',(-7.50747703535115,24.2570993577032,
0.));
#243618=CARTESIAN_POINT('Ctrl Pts',(-7.50747703535115,24.2570993577032,
12.));
#243619=CARTESIAN_POINT('Ctrl Pts',(-7.50271363765098,24.2835078958966,
0.));
#243620=CARTESIAN_POINT('Ctrl Pts',(-7.50271363765098,24.2835078958966,
12.));
#243621=CARTESIAN_POINT('Ctrl Pts',(-7.49787641695359,24.3099781253345,
0.));
#243622=CARTESIAN_POINT('Ctrl Pts',(-7.49787641695359,24.3099781253345,
12.));
#243623=CARTESIAN_POINT('Ctrl Pts',(-7.4929652125233,24.3365095573673,0.));
#243624=CARTESIAN_POINT('Ctrl Pts',(-7.4929652125233,24.3365095573673,12.));
#243625=CARTESIAN_POINT('Ctrl Pts',(-7.48797986651828,24.3631017084513,
0.));
#243626=CARTESIAN_POINT('Ctrl Pts',(-7.48797986651828,24.3631017084513,
12.));
#243627=CARTESIAN_POINT('Ctrl Pts',(-7.48292022569254,24.3897541049248,
0.));
#243628=CARTESIAN_POINT('Ctrl Pts',(-7.48292022569254,24.3897541049248,
12.));
#243629=CARTESIAN_POINT('Ctrl Pts',(-7.47778614286573,24.4164662871165,
0.));
#243630=CARTESIAN_POINT('Ctrl Pts',(-7.47778614286573,24.4164662871165,
12.));
#243631=CARTESIAN_POINT('Ctrl Pts',(-7.47257747883319,24.4432378146501,
0.));
#243632=CARTESIAN_POINT('Ctrl Pts',(-7.47257747883319,24.4432378146501,
12.));
#243633=CARTESIAN_POINT('Ctrl Pts',(-7.46729410308923,24.4700682684544,
0.));
#243634=CARTESIAN_POINT('Ctrl Pts',(-7.46729410308923,24.4700682684544,
12.));
#243635=CARTESIAN_POINT('Ctrl Pts',(-7.46193588961642,24.4969572391509,
0.));
#243636=CARTESIAN_POINT('Ctrl Pts',(-7.46193588961642,24.4969572391509,
12.));
#243637=CARTESIAN_POINT('Ctrl Pts',(-7.45650271336045,24.52390431731,0.));
#243638=CARTESIAN_POINT('Ctrl Pts',(-7.45650271336045,24.52390431731,12.));
#243639=CARTESIAN_POINT('Ctrl Pts',(-7.45099444651296,24.5509090831579,
0.));
#243640=CARTESIAN_POINT('Ctrl Pts',(-7.45099444651296,24.5509090831579,
12.));
#243641=CARTESIAN_POINT('Ctrl Pts',(-7.44541095473163,24.5779710960865,
0.));
#243642=CARTESIAN_POINT('Ctrl Pts',(-7.44541095473163,24.5779710960865,
12.));
#243643=CARTESIAN_POINT('Ctrl Pts',(-7.43975209375375,24.6050898852349,
0.));
#243644=CARTESIAN_POINT('Ctrl Pts',(-7.43975209375375,24.6050898852349,
12.));
#243645=CARTESIAN_POINT('Ctrl Pts',(-7.4340177048922,24.6322649369472,0.));
#243646=CARTESIAN_POINT('Ctrl Pts',(-7.4340177048922,24.6322649369472,12.));
#243647=CARTESIAN_POINT('Ctrl Pts',(-7.42820762158681,24.659495712869,0.));
#243648=CARTESIAN_POINT('Ctrl Pts',(-7.42820762158681,24.659495712869,12.));
#243649=CARTESIAN_POINT('Ctrl Pts',(-7.42232167765763,24.6867816727118,
0.));
#243650=CARTESIAN_POINT('Ctrl Pts',(-7.42232167765763,24.6867816727118,
12.));
#243651=CARTESIAN_POINT('Ctrl Pts',(-7.41635971481243,24.7141222949988,
0.));
#243652=CARTESIAN_POINT('Ctrl Pts',(-7.41635971481243,24.7141222949988,
12.));
#243653=CARTESIAN_POINT('Ctrl Pts',(-7.41032159082173,24.7415170994754,
0.));
#243654=CARTESIAN_POINT('Ctrl Pts',(-7.41032159082173,24.7415170994754,
12.));
#243655=CARTESIAN_POINT('Ctrl Pts',(-7.40420718661754,24.7689656669005,
0.));
#243656=CARTESIAN_POINT('Ctrl Pts',(-7.40420718661754,24.7689656669005,
12.));
#243657=CARTESIAN_POINT('Ctrl Pts',(-7.39801641583612,24.7964676646518,
0.));
#243658=CARTESIAN_POINT('Ctrl Pts',(-7.39801641583612,24.7964676646518,
12.));
#243659=CARTESIAN_POINT('Ctrl Pts',(-7.39174922586841,24.8240228521042,
0.));
#243660=CARTESIAN_POINT('Ctrl Pts',(-7.39174922586841,24.8240228521042,
12.));
#243661=CARTESIAN_POINT('Ctrl Pts',(-7.38540558904946,24.8516310625367,
0.));
#243662=CARTESIAN_POINT('Ctrl Pts',(-7.38540558904946,24.8516310625367,
12.));
#243663=CARTESIAN_POINT('Ctrl Pts',(-7.3789854964161,24.8792921911309,0.));
#243664=CARTESIAN_POINT('Ctrl Pts',(-7.3789854964161,24.8792921911309,12.));
#243665=CARTESIAN_POINT('Ctrl Pts',(-7.37378825962718,24.9014633826201,
0.));
#243666=CARTESIAN_POINT('Ctrl Pts',(-7.37378825962718,24.9014633826201,
12.));
#243667=CARTESIAN_POINT('Ctrl Pts',(-7.36985593120696,24.9181155530631,
0.));
#243668=CARTESIAN_POINT('Ctrl Pts',(-7.36985593120696,24.9181155530631,
12.));
#243669=CARTESIAN_POINT('Ctrl Pts',(-7.3672190902906,24.9292275670705,0.));
#243670=CARTESIAN_POINT('Ctrl Pts',(-7.3672190902906,24.9292275670705,12.));
#243671=CARTESIAN_POINT('Ctrl Pts',(-7.36589684767344,24.9347862158358,
0.));
#243672=CARTESIAN_POINT('Ctrl Pts',(-7.36589684767344,24.9347862158358,
12.));
#243673=CARTESIAN_POINT('',(-7.36589684767344,24.9347862158358,0.));
#243674=CARTESIAN_POINT('Ctrl Pts',(-7.52250298901264,21.2610617890679,
0.));
#243675=CARTESIAN_POINT('Ctrl Pts',(-7.5225064970397,21.2610673466886,0.));
#243676=CARTESIAN_POINT('Ctrl Pts',(-7.52252744144904,21.2611204474866,
0.));
#243677=CARTESIAN_POINT('Ctrl Pts',(-7.52260064231661,21.261326054066,0.));
#243678=CARTESIAN_POINT('Ctrl Pts',(-7.5227818224267,21.2618521283555,0.));
#243679=CARTESIAN_POINT('Ctrl Pts',(-7.52314642316199,21.262927782038,0.));
#243680=CARTESIAN_POINT('Ctrl Pts',(-7.52364573027553,21.2644161259962,
0.));
#243681=CARTESIAN_POINT('Ctrl Pts',(-7.52427261074298,21.2663059157058,
0.));
#243682=CARTESIAN_POINT('Ctrl Pts',(-7.5250177033353,21.2685823838671,0.));
#243683=CARTESIAN_POINT('Ctrl Pts',(-7.5258712609553,21.2712301573466,0.));
#243684=CARTESIAN_POINT('Ctrl Pts',(-7.52682526918541,21.2742366113579,
0.));
#243685=CARTESIAN_POINT('Ctrl Pts',(-7.52787386225333,21.2775925269652,
0.));
#243686=CARTESIAN_POINT('Ctrl Pts',(-7.52901217930408,21.2812902781143,
0.));
#243687=CARTESIAN_POINT('Ctrl Pts',(-7.53023562438229,21.2853226580657,
0.));
#243688=CARTESIAN_POINT('Ctrl Pts',(-7.53153906987855,21.2896816163842,
0.));
#243689=CARTESIAN_POINT('Ctrl Pts',(-7.53291726078527,21.2943588989331,
0.));
#243690=CARTESIAN_POINT('Ctrl Pts',(-7.53436505309943,21.2993464250717,
0.));
#243691=CARTESIAN_POINT('Ctrl Pts',(-7.53587778251736,21.3046368712157,
0.));
#243692=CARTESIAN_POINT('Ctrl Pts',(-7.53745129364616,21.310223716773,0.));
#243693=CARTESIAN_POINT('Ctrl Pts',(-7.53908175169898,21.3161009456256,
0.));
#243694=CARTESIAN_POINT('Ctrl Pts',(-7.54076552038279,21.3222628524165,
0.));
#243695=CARTESIAN_POINT('Ctrl Pts',(-7.54249900377031,21.328703791771,0.));
#243696=CARTESIAN_POINT('Ctrl Pts',(-7.54427868151268,21.3354182340149,
0.));
#243697=CARTESIAN_POINT('Ctrl Pts',(-7.54610114948347,21.3424008295038,
0.));
#243698=CARTESIAN_POINT('Ctrl Pts',(-7.5479631624633,21.3496464761531,0.));
#243699=CARTESIAN_POINT('Ctrl Pts',(-7.5498616652131,21.3571503685855,0.));
#243700=CARTESIAN_POINT('Ctrl Pts',(-7.55179375777444,21.3649079431865,
0.));
#243701=CARTESIAN_POINT('Ctrl Pts',(-7.55375667080029,21.3729148390243,
0.));
#243702=CARTESIAN_POINT('Ctrl Pts',(-7.55574773403503,21.3811668478932,
0.));
#243703=CARTESIAN_POINT('Ctrl Pts',(-7.55776435731417,21.3896598842117,
0.));
#243704=CARTESIAN_POINT('Ctrl Pts',(-7.55980403700611,21.3983899952987,
0.));
#243705=CARTESIAN_POINT('Ctrl Pts',(-7.56186435703622,21.4073533630365,
0.));
#243706=CARTESIAN_POINT('Ctrl Pts',(-7.56394299313685,21.4165463106254,
0.));
#243707=CARTESIAN_POINT('Ctrl Pts',(-7.56603771218712,21.4259653015736,
0.));
#243708=CARTESIAN_POINT('Ctrl Pts',(-7.56814636360847,21.4356069261513,
0.));
#243709=CARTESIAN_POINT('Ctrl Pts',(-7.57026687261166,21.4454678907509,
0.));
#243710=CARTESIAN_POINT('Ctrl Pts',(-7.57239723223506,21.4555450053142,
0.));
#243711=CARTESIAN_POINT('Ctrl Pts',(-7.57453549743412,21.4658351740128,
0.));
#243712=CARTESIAN_POINT('Ctrl Pts',(-7.57667978402987,21.4763353936762,
0.));
#243713=CARTESIAN_POINT('Ctrl Pts',(-7.57882826679132,21.4870427508194,
0.));
#243714=CARTESIAN_POINT('Ctrl Pts',(-7.58097917790744,21.4979544192744,
0.));
#243715=CARTESIAN_POINT('Ctrl Pts',(-7.5831308051918,21.5090676573873,0.));
#243716=CARTESIAN_POINT('Ctrl Pts',(-7.5852814891913,21.5203798035299,0.));
#243717=CARTESIAN_POINT('Ctrl Pts',(-7.58742962034834,21.5318882716736,
0.));
#243718=CARTESIAN_POINT('Ctrl Pts',(-7.58957363620014,21.543590547011,0.));
#243719=CARTESIAN_POINT('Ctrl Pts',(-7.59171201844777,21.5554841813462,
0.));
#243720=CARTESIAN_POINT('Ctrl Pts',(-7.59384329124918,21.5675667904726,
0.));
#243721=CARTESIAN_POINT('Ctrl Pts',(-7.59596601973584,21.5798360518978,
0.));
#243722=CARTESIAN_POINT('Ctrl Pts',(-7.59807880846195,21.5922897024466,
0.));
#243723=CARTESIAN_POINT('Ctrl Pts',(-7.60018029988241,21.6049255358843,
0.));
#243724=CARTESIAN_POINT('Ctrl Pts',(-7.60226917285429,21.617741400599,0.));
#243725=CARTESIAN_POINT('Ctrl Pts',(-7.60434414118296,21.6307351973822,
0.));
#243726=CARTESIAN_POINT('Ctrl Pts',(-7.60640395216357,21.6439048771743,
0.));
#243727=CARTESIAN_POINT('Ctrl Pts',(-7.60844738512874,21.6572484388081,
0.));
#243728=CARTESIAN_POINT('Ctrl Pts',(-7.61047325000956,21.6707639267576,
0.));
#243729=CARTESIAN_POINT('Ctrl Pts',(-7.61248038630268,21.6844494295815,
0.));
#243730=CARTESIAN_POINT('Ctrl Pts',(-7.61446766202787,21.6983030783322,
0.));
#243731=CARTESIAN_POINT('Ctrl Pts',(-7.61643397270421,21.7123230449834,
0.));
#243732=CARTESIAN_POINT('Ctrl Pts',(-7.61837824030538,21.7265075407975,
0.));
#243733=CARTESIAN_POINT('Ctrl Pts',(-7.62029941230855,21.7408548148656,
0.));
#243734=CARTESIAN_POINT('Ctrl Pts',(-7.62219646084228,21.7553631528328,
0.));
#243735=CARTESIAN_POINT('Ctrl Pts',(-7.62406838181166,21.7700308755584,
0.));
#243736=CARTESIAN_POINT('Ctrl Pts',(-7.62591419404512,21.7848563378021,
0.));
#243737=CARTESIAN_POINT('Ctrl Pts',(-7.62773293842389,21.799837926858,0.));
#243738=CARTESIAN_POINT('Ctrl Pts',(-7.62952367718127,21.814974061509,0.));
#243739=CARTESIAN_POINT('Ctrl Pts',(-7.63128549323023,21.8302631910195,
0.));
#243740=CARTESIAN_POINT('Ctrl Pts',(-7.63301748948936,21.8457037941084,
0.));
#243741=CARTESIAN_POINT('Ctrl Pts',(-7.63471878821226,21.8612943779089,
0.));
#243742=CARTESIAN_POINT('Ctrl Pts',(-7.636388530334,21.8770334769496,0.));
#243743=CARTESIAN_POINT('Ctrl Pts',(-7.63802587492035,21.8929196523514,
0.));
#243744=CARTESIAN_POINT('Ctrl Pts',(-7.63962999860927,21.9089514909874,
0.));
#243745=CARTESIAN_POINT('Ctrl Pts',(-7.64120009506532,21.9251276046546,
0.));
#243746=CARTESIAN_POINT('Ctrl Pts',(-7.64273537442682,21.9414466292072,
0.));
#243747=CARTESIAN_POINT('Ctrl Pts',(-7.64423506279123,21.9579072237651,
0.));
#243748=CARTESIAN_POINT('Ctrl Pts',(-7.64569840177336,21.9745080700798,
0.));
#243749=CARTESIAN_POINT('Ctrl Pts',(-7.6471246480525,21.9912478718542,0.));
#243750=CARTESIAN_POINT('Ctrl Pts',(-7.64851307293352,22.0081253540774,
0.));
#243751=CARTESIAN_POINT('Ctrl Pts',(-7.64986296190168,22.0251392623209,
0.));
#243752=CARTESIAN_POINT('Ctrl Pts',(-7.65117361421358,22.0422883621174,
0.));
#243753=CARTESIAN_POINT('Ctrl Pts',(-7.65244434253113,22.0595714384431,
0.));
#243754=CARTESIAN_POINT('Ctrl Pts',(-7.65367447254949,22.0769872951596,
0.));
#243755=CARTESIAN_POINT('Ctrl Pts',(-7.65486334263644,22.094534754469,0.));
#243756=CARTESIAN_POINT('Ctrl Pts',(-7.65601030346807,22.1122126563329,
0.));
#243757=CARTESIAN_POINT('Ctrl Pts',(-7.65711471769397,22.1300198579675,
0.));
#243758=CARTESIAN_POINT('Ctrl Pts',(-7.65817595963349,22.1479552334211,
0.));
#243759=CARTESIAN_POINT('Ctrl Pts',(-7.6591934149693,22.1660176731178,0.));
#243760=CARTESIAN_POINT('Ctrl Pts',(-7.66016648045005,22.1842060834091,
0.));
#243761=CARTESIAN_POINT('Ctrl Pts',(-7.66109456359271,22.2025193860964,
0.));
#243762=CARTESIAN_POINT('Ctrl Pts',(-7.661977082404,22.2209565180085,0.));
#243763=CARTESIAN_POINT('Ctrl Pts',(-7.66281346512509,22.2395164306547,
0.));
#243764=CARTESIAN_POINT('Ctrl Pts',(-7.66360314997641,22.258198089848,0.));
#243765=CARTESIAN_POINT('Ctrl Pts',(-7.66434558490979,22.2770004753335,
0.));
#243766=CARTESIAN_POINT('Ctrl Pts',(-7.66504022736299,22.2959225803937,
0.));
#243767=CARTESIAN_POINT('Ctrl Pts',(-7.66568654402494,22.314963411484,0.));
#243768=CARTESIAN_POINT('Ctrl Pts',(-7.66628401061952,22.3341219879469,
0.));
#243769=CARTESIAN_POINT('Ctrl Pts',(-7.66683211169158,22.3533973417021,
0.));
#243770=CARTESIAN_POINT('Ctrl Pts',(-7.66733034039883,22.372788516936,0.));
#243771=CARTESIAN_POINT('Ctrl Pts',(-7.6677781983079,22.3922945697773,0.));
#243772=CARTESIAN_POINT('Ctrl Pts',(-7.6681751951964,22.4119145679758,0.));
#243773=CARTESIAN_POINT('Ctrl Pts',(-7.66852084886704,22.4316475906603,
0.));
#243774=CARTESIAN_POINT('Ctrl Pts',(-7.66881468496635,22.4514927280855,
0.));
#243775=CARTESIAN_POINT('Ctrl Pts',(-7.66905623680831,22.47144908137,0.));
#243776=CARTESIAN_POINT('Ctrl Pts',(-7.66924504520315,22.4915157622312,
0.));
#243777=CARTESIAN_POINT('Ctrl Pts',(-7.66938065829108,22.5116918927031,
0.));
#243778=CARTESIAN_POINT('Ctrl Pts',(-7.66946263138144,22.53197660492,0.));
#243779=CARTESIAN_POINT('Ctrl Pts',(-7.66949052679693,22.5523690409116,
0.));
#243780=CARTESIAN_POINT('Ctrl Pts',(-7.66946391372306,22.5728683523831,
0.));
#243781=CARTESIAN_POINT('Ctrl Pts',(-7.66938236806233,22.5934737004953,
0.));
#243782=CARTESIAN_POINT('Ctrl Pts',(-7.66924547229414,22.6141842556243,
0.));
#243783=CARTESIAN_POINT('Ctrl Pts',(-7.66905281533715,22.6349991971541,
0.));
#243784=CARTESIAN_POINT('Ctrl Pts',(-7.66880399241323,22.6559177133127,
0.));
#243785=CARTESIAN_POINT('Ctrl Pts',(-7.66849860491743,22.6769390009885,
0.));
#243786=CARTESIAN_POINT('Ctrl Pts',(-7.66813626029275,22.6980622655446,
0.));
#243787=CARTESIAN_POINT('Ctrl Pts',(-7.66771657191027,22.7192867206245,
0.));
#243788=CARTESIAN_POINT('Ctrl Pts',(-7.6672391589544,22.7406115879513,0.));
#243789=CARTESIAN_POINT('Ctrl Pts',(-7.66670364630299,22.7620360971843,
0.));
#243790=CARTESIAN_POINT('Ctrl Pts',(-7.66610966441273,22.7835594857699,
0.));
#243791=CARTESIAN_POINT('Ctrl Pts',(-7.66545684920987,22.8051809987833,
0.));
#243792=CARTESIAN_POINT('Ctrl Pts',(-7.66474484198549,22.8268998887678,
0.));
#243793=CARTESIAN_POINT('Ctrl Pts',(-7.66397328929803,22.848715415557,0.));
#243794=CARTESIAN_POINT('Ctrl Pts',(-7.66314184287337,22.8706268461283,
0.));
#243795=CARTESIAN_POINT('Ctrl Pts',(-7.66225015950156,22.8926334544883,
0.));
#243796=CARTESIAN_POINT('Ctrl Pts',(-7.66129790094108,22.9147345215421,
0.));
#243797=CARTESIAN_POINT('Ctrl Pts',(-7.66028473382778,22.9369293349593,
0.));
#243798=CARTESIAN_POINT('Ctrl Pts',(-7.65921032958902,22.959217189033,0.));
#243799=CARTESIAN_POINT('Ctrl Pts',(-7.65807436436432,22.9815973845296,
0.));
#243800=CARTESIAN_POINT('Ctrl Pts',(-7.65687651891304,23.0040692285814,
0.));
#243801=CARTESIAN_POINT('Ctrl Pts',(-7.65561647852534,23.0266320345787,
0.));
#243802=CARTESIAN_POINT('Ctrl Pts',(-7.65429393293946,23.0492851220528,
0.));
#243803=CARTESIAN_POINT('Ctrl Pts',(-7.65290857626358,23.072027816555,0.));
#243804=CARTESIAN_POINT('Ctrl Pts',(-7.65146010690476,23.094859449525,0.));
#243805=CARTESIAN_POINT('Ctrl Pts',(-7.6499482274986,23.1177793581679,0.));
#243806=CARTESIAN_POINT('Ctrl Pts',(-7.64837264482943,23.1407868853819,
0.));
#243807=CARTESIAN_POINT('Ctrl Pts',(-7.64673306975805,23.1638813796694,
0.));
#243808=CARTESIAN_POINT('Ctrl Pts',(-7.64502921715483,23.1870621950452,
0.));
#243809=CARTESIAN_POINT('Ctrl Pts',(-7.6432608058368,23.2103286909398,0.));
#243810=CARTESIAN_POINT('Ctrl Pts',(-7.64142755851504,23.2336802320912,
0.));
#243811=CARTESIAN_POINT('Ctrl Pts',(-7.63952920172835,23.2571161884488,
0.));
#243812=CARTESIAN_POINT('Ctrl Pts',(-7.63756546576374,23.2806359350855,
0.));
#243813=CARTESIAN_POINT('Ctrl Pts',(-7.63553608458783,23.3042388521022,
0.));
#243814=CARTESIAN_POINT('Ctrl Pts',(-7.63344079578161,23.3279243245241,
0.));
#243815=CARTESIAN_POINT('Ctrl Pts',(-7.63127934048136,23.3516917421972,
0.));
#243816=CARTESIAN_POINT('Ctrl Pts',(-7.62905146332593,23.3755404996636,
0.));
#243817=CARTESIAN_POINT('Ctrl Pts',(-7.62675691240329,23.399469996112,0.));
#243818=CARTESIAN_POINT('Ctrl Pts',(-7.6243954392005,23.4234796353542,0.));
#243819=CARTESIAN_POINT('Ctrl Pts',(-7.62196679855955,23.4475688257854,
0.));
#243820=CARTESIAN_POINT('Ctrl Pts',(-7.61947074863977,23.4717369803438,
0.));
#243821=CARTESIAN_POINT('Ctrl Pts',(-7.61690705088319,23.4959835164609,
0.));
#243822=CARTESIAN_POINT('Ctrl Pts',(-7.61427546999298,23.5203078560129,
0.));
#243823=CARTESIAN_POINT('Ctrl Pts',(-7.61157577385372,23.544709425203,0.));
#243824=CARTESIAN_POINT('Ctrl Pts',(-7.608807733446,23.5691876544244,0.));
#243825=CARTESIAN_POINT('Ctrl Pts',(-7.60597112277094,23.5937419781245,
0.));
#243826=CARTESIAN_POINT('Ctrl Pts',(-7.60306571877806,23.6183718346576,
0.));
#243827=CARTESIAN_POINT('Ctrl Pts',(-7.60009130130126,23.6430766661418,
0.));
#243828=CARTESIAN_POINT('Ctrl Pts',(-7.59704765299567,23.6678559182875,
0.));
#243829=CARTESIAN_POINT('Ctrl Pts',(-7.59393455934035,23.6927090405066,
0.));
#243830=CARTESIAN_POINT('Ctrl Pts',(-7.5907518086532,23.7176354860456,0.));
#243831=CARTESIAN_POINT('Ctrl Pts',(-7.58749919210826,23.7426347121006,
0.));
#243832=CARTESIAN_POINT('Ctrl Pts',(-7.58417650376271,23.7677061799376,
0.));
#243833=CARTESIAN_POINT('Ctrl Pts',(-7.58078354058213,23.7928493549908,
0.));
#243834=CARTESIAN_POINT('Ctrl Pts',(-7.57732010249066,23.8180637069976,
0.));
#243835=CARTESIAN_POINT('Ctrl Pts',(-7.57378599219814,23.8433487096132,
0.));
#243836=CARTESIAN_POINT('Ctrl Pts',(-7.57018101500709,23.8687038399595,
0.));
#243837=CARTESIAN_POINT('Ctrl Pts',(-7.56650497863791,23.8941285782002,
0.));
#243838=CARTESIAN_POINT('Ctrl Pts',(-7.56275769304773,23.9196224070759,
0.));
#243839=CARTESIAN_POINT('Ctrl Pts',(-7.5589389702768,23.9451848115002,0.));
#243840=CARTESIAN_POINT('Ctrl Pts',(-7.55504862424808,23.9708152779886,
0.));
#243841=CARTESIAN_POINT('Ctrl Pts',(-7.55108647097432,23.9965132953187,
0.));
#243842=CARTESIAN_POINT('Ctrl Pts',(-7.54705232885895,24.0222783554531,
0.));
#243843=CARTESIAN_POINT('Ctrl Pts',(-7.54294601896128,24.0481099543353,
0.));
#243844=CARTESIAN_POINT('Ctrl Pts',(-7.53876736531005,24.0740075927984,
0.));
#243845=CARTESIAN_POINT('Ctrl Pts',(-7.53451619514658,24.0999707772643,
0.));
#243846=CARTESIAN_POINT('Ctrl Pts',(-7.53019233935536,24.1259990209211,
0.));
#243847=CARTESIAN_POINT('Ctrl Pts',(-7.52579563201479,24.152091842537,0.));
#243848=CARTESIAN_POINT('Ctrl Pts',(-7.52132590953862,24.1782487641602,
0.));
#243849=CARTESIAN_POINT('Ctrl Pts',(-7.51678300997998,24.2044693092356,
0.));
#243850=CARTESIAN_POINT('Ctrl Pts',(-7.51216677222199,24.230753000389,0.));
#243851=CARTESIAN_POINT('Ctrl Pts',(-7.50747703535115,24.2570993577032,
0.));
#243852=CARTESIAN_POINT('Ctrl Pts',(-7.50271363765098,24.2835078958966,
0.));
#243853=CARTESIAN_POINT('Ctrl Pts',(-7.49787641695359,24.3099781253345,
0.));
#243854=CARTESIAN_POINT('Ctrl Pts',(-7.4929652125233,24.3365095573673,0.));
#243855=CARTESIAN_POINT('Ctrl Pts',(-7.48797986651828,24.3631017084513,
0.));
#243856=CARTESIAN_POINT('Ctrl Pts',(-7.48292022569254,24.3897541049248,
0.));
#243857=CARTESIAN_POINT('Ctrl Pts',(-7.47778614286573,24.4164662871165,
0.));
#243858=CARTESIAN_POINT('Ctrl Pts',(-7.47257747883319,24.4432378146501,
0.));
#243859=CARTESIAN_POINT('Ctrl Pts',(-7.46729410308923,24.4700682684544,
0.));
#243860=CARTESIAN_POINT('Ctrl Pts',(-7.46193588961642,24.4969572391509,
0.));
#243861=CARTESIAN_POINT('Ctrl Pts',(-7.45650271336045,24.52390431731,0.));
#243862=CARTESIAN_POINT('Ctrl Pts',(-7.45099444651296,24.5509090831579,
0.));
#243863=CARTESIAN_POINT('Ctrl Pts',(-7.44541095473163,24.5779710960865,
0.));
#243864=CARTESIAN_POINT('Ctrl Pts',(-7.43975209375375,24.6050898852349,
0.));
#243865=CARTESIAN_POINT('Ctrl Pts',(-7.4340177048922,24.6322649369472,0.));
#243866=CARTESIAN_POINT('Ctrl Pts',(-7.42820762158681,24.659495712869,0.));
#243867=CARTESIAN_POINT('Ctrl Pts',(-7.42232167765763,24.6867816727118,
0.));
#243868=CARTESIAN_POINT('Ctrl Pts',(-7.41635971481243,24.7141222949988,
0.));
#243869=CARTESIAN_POINT('Ctrl Pts',(-7.41032159082173,24.7415170994754,
0.));
#243870=CARTESIAN_POINT('Ctrl Pts',(-7.40420718661754,24.7689656669005,
0.));
#243871=CARTESIAN_POINT('Ctrl Pts',(-7.39801641583612,24.7964676646518,
0.));
#243872=CARTESIAN_POINT('Ctrl Pts',(-7.39174922586841,24.8240228521042,
0.));
#243873=CARTESIAN_POINT('Ctrl Pts',(-7.38540558904946,24.8516310625367,
0.));
#243874=CARTESIAN_POINT('Ctrl Pts',(-7.3789854964161,24.8792921911309,0.));
#243875=CARTESIAN_POINT('Ctrl Pts',(-7.37378825962718,24.9014633826201,
0.));
#243876=CARTESIAN_POINT('Ctrl Pts',(-7.36985593120696,24.9181155530631,
0.));
#243877=CARTESIAN_POINT('Ctrl Pts',(-7.3672190902906,24.9292275670705,0.));
#243878=CARTESIAN_POINT('Ctrl Pts',(-7.36589684767344,24.9347862158358,
0.));
#243879=CARTESIAN_POINT('',(-7.36589684767344,24.9347862158358,12.));
#243880=CARTESIAN_POINT('Ctrl Pts',(-7.36589684767344,24.9347862158358,
12.));
#243881=CARTESIAN_POINT('Ctrl Pts',(-7.3672190902906,24.9292275670705,12.));
#243882=CARTESIAN_POINT('Ctrl Pts',(-7.36985593120696,24.9181155530631,
12.));
#243883=CARTESIAN_POINT('Ctrl Pts',(-7.37378825962718,24.9014633826201,
12.));
#243884=CARTESIAN_POINT('Ctrl Pts',(-7.3789854964161,24.8792921911309,12.));
#243885=CARTESIAN_POINT('Ctrl Pts',(-7.38540558904946,24.8516310625367,
12.));
#243886=CARTESIAN_POINT('Ctrl Pts',(-7.39174922586841,24.8240228521042,
12.));
#243887=CARTESIAN_POINT('Ctrl Pts',(-7.39801641583612,24.7964676646518,
12.));
#243888=CARTESIAN_POINT('Ctrl Pts',(-7.40420718661754,24.7689656669005,
12.));
#243889=CARTESIAN_POINT('Ctrl Pts',(-7.41032159082173,24.7415170994754,
12.));
#243890=CARTESIAN_POINT('Ctrl Pts',(-7.41635971481243,24.7141222949988,
12.));
#243891=CARTESIAN_POINT('Ctrl Pts',(-7.42232167765763,24.6867816727118,
12.));
#243892=CARTESIAN_POINT('Ctrl Pts',(-7.42820762158681,24.659495712869,12.));
#243893=CARTESIAN_POINT('Ctrl Pts',(-7.4340177048922,24.6322649369472,12.));
#243894=CARTESIAN_POINT('Ctrl Pts',(-7.43975209375375,24.6050898852349,
12.));
#243895=CARTESIAN_POINT('Ctrl Pts',(-7.44541095473163,24.5779710960865,
12.));
#243896=CARTESIAN_POINT('Ctrl Pts',(-7.45099444651296,24.5509090831579,
12.));
#243897=CARTESIAN_POINT('Ctrl Pts',(-7.45650271336045,24.52390431731,12.));
#243898=CARTESIAN_POINT('Ctrl Pts',(-7.46193588961642,24.4969572391509,
12.));
#243899=CARTESIAN_POINT('Ctrl Pts',(-7.46729410308923,24.4700682684544,
12.));
#243900=CARTESIAN_POINT('Ctrl Pts',(-7.47257747883319,24.4432378146501,
12.));
#243901=CARTESIAN_POINT('Ctrl Pts',(-7.47778614286573,24.4164662871165,
12.));
#243902=CARTESIAN_POINT('Ctrl Pts',(-7.48292022569254,24.3897541049248,
12.));
#243903=CARTESIAN_POINT('Ctrl Pts',(-7.48797986651828,24.3631017084513,
12.));
#243904=CARTESIAN_POINT('Ctrl Pts',(-7.4929652125233,24.3365095573673,12.));
#243905=CARTESIAN_POINT('Ctrl Pts',(-7.49787641695359,24.3099781253345,
12.));
#243906=CARTESIAN_POINT('Ctrl Pts',(-7.50271363765098,24.2835078958966,
12.));
#243907=CARTESIAN_POINT('Ctrl Pts',(-7.50747703535115,24.2570993577032,
12.));
#243908=CARTESIAN_POINT('Ctrl Pts',(-7.51216677222199,24.230753000389,12.));
#243909=CARTESIAN_POINT('Ctrl Pts',(-7.51678300997998,24.2044693092356,
12.));
#243910=CARTESIAN_POINT('Ctrl Pts',(-7.52132590953862,24.1782487641602,
12.));
#243911=CARTESIAN_POINT('Ctrl Pts',(-7.52579563201479,24.152091842537,12.));
#243912=CARTESIAN_POINT('Ctrl Pts',(-7.53019233935536,24.1259990209211,
12.));
#243913=CARTESIAN_POINT('Ctrl Pts',(-7.53451619514658,24.0999707772643,
12.));
#243914=CARTESIAN_POINT('Ctrl Pts',(-7.53876736531005,24.0740075927984,
12.));
#243915=CARTESIAN_POINT('Ctrl Pts',(-7.54294601896128,24.0481099543353,
12.));
#243916=CARTESIAN_POINT('Ctrl Pts',(-7.54705232885895,24.0222783554531,
12.));
#243917=CARTESIAN_POINT('Ctrl Pts',(-7.55108647097432,23.9965132953187,
12.));
#243918=CARTESIAN_POINT('Ctrl Pts',(-7.55504862424808,23.9708152779886,
12.));
#243919=CARTESIAN_POINT('Ctrl Pts',(-7.5589389702768,23.9451848115002,12.));
#243920=CARTESIAN_POINT('Ctrl Pts',(-7.56275769304773,23.9196224070759,
12.));
#243921=CARTESIAN_POINT('Ctrl Pts',(-7.56650497863791,23.8941285782002,
12.));
#243922=CARTESIAN_POINT('Ctrl Pts',(-7.57018101500709,23.8687038399595,
12.));
#243923=CARTESIAN_POINT('Ctrl Pts',(-7.57378599219814,23.8433487096132,
12.));
#243924=CARTESIAN_POINT('Ctrl Pts',(-7.57732010249066,23.8180637069976,
12.));
#243925=CARTESIAN_POINT('Ctrl Pts',(-7.58078354058213,23.7928493549908,
12.));
#243926=CARTESIAN_POINT('Ctrl Pts',(-7.58417650376271,23.7677061799376,
12.));
#243927=CARTESIAN_POINT('Ctrl Pts',(-7.58749919210826,23.7426347121006,
12.));
#243928=CARTESIAN_POINT('Ctrl Pts',(-7.5907518086532,23.7176354860456,12.));
#243929=CARTESIAN_POINT('Ctrl Pts',(-7.59393455934035,23.6927090405066,
12.));
#243930=CARTESIAN_POINT('Ctrl Pts',(-7.59704765299567,23.6678559182875,
12.));
#243931=CARTESIAN_POINT('Ctrl Pts',(-7.60009130130126,23.6430766661418,
12.));
#243932=CARTESIAN_POINT('Ctrl Pts',(-7.60306571877806,23.6183718346576,
12.));
#243933=CARTESIAN_POINT('Ctrl Pts',(-7.60597112277094,23.5937419781245,
12.));
#243934=CARTESIAN_POINT('Ctrl Pts',(-7.608807733446,23.5691876544244,12.));
#243935=CARTESIAN_POINT('Ctrl Pts',(-7.61157577385372,23.544709425203,12.));
#243936=CARTESIAN_POINT('Ctrl Pts',(-7.61427546999298,23.5203078560129,
12.));
#243937=CARTESIAN_POINT('Ctrl Pts',(-7.61690705088319,23.4959835164609,
12.));
#243938=CARTESIAN_POINT('Ctrl Pts',(-7.61947074863977,23.4717369803438,
12.));
#243939=CARTESIAN_POINT('Ctrl Pts',(-7.62196679855955,23.4475688257854,
12.));
#243940=CARTESIAN_POINT('Ctrl Pts',(-7.6243954392005,23.4234796353542,12.));
#243941=CARTESIAN_POINT('Ctrl Pts',(-7.62675691240329,23.399469996112,12.));
#243942=CARTESIAN_POINT('Ctrl Pts',(-7.62905146332593,23.3755404996636,
12.));
#243943=CARTESIAN_POINT('Ctrl Pts',(-7.63127934048136,23.3516917421972,
12.));
#243944=CARTESIAN_POINT('Ctrl Pts',(-7.63344079578161,23.3279243245241,
12.));
#243945=CARTESIAN_POINT('Ctrl Pts',(-7.63553608458783,23.3042388521022,
12.));
#243946=CARTESIAN_POINT('Ctrl Pts',(-7.63756546576374,23.2806359350855,
12.));
#243947=CARTESIAN_POINT('Ctrl Pts',(-7.63952920172835,23.2571161884488,
12.));
#243948=CARTESIAN_POINT('Ctrl Pts',(-7.64142755851504,23.2336802320912,
12.));
#243949=CARTESIAN_POINT('Ctrl Pts',(-7.6432608058368,23.2103286909398,12.));
#243950=CARTESIAN_POINT('Ctrl Pts',(-7.64502921715483,23.1870621950452,
12.));
#243951=CARTESIAN_POINT('Ctrl Pts',(-7.64673306975805,23.1638813796694,
12.));
#243952=CARTESIAN_POINT('Ctrl Pts',(-7.64837264482943,23.1407868853819,
12.));
#243953=CARTESIAN_POINT('Ctrl Pts',(-7.6499482274986,23.1177793581679,12.));
#243954=CARTESIAN_POINT('Ctrl Pts',(-7.65146010690476,23.094859449525,12.));
#243955=CARTESIAN_POINT('Ctrl Pts',(-7.65290857626358,23.072027816555,12.));
#243956=CARTESIAN_POINT('Ctrl Pts',(-7.65429393293946,23.0492851220528,
12.));
#243957=CARTESIAN_POINT('Ctrl Pts',(-7.65561647852534,23.0266320345787,
12.));
#243958=CARTESIAN_POINT('Ctrl Pts',(-7.65687651891304,23.0040692285814,
12.));
#243959=CARTESIAN_POINT('Ctrl Pts',(-7.65807436436432,22.9815973845296,
12.));
#243960=CARTESIAN_POINT('Ctrl Pts',(-7.65921032958902,22.959217189033,12.));
#243961=CARTESIAN_POINT('Ctrl Pts',(-7.66028473382778,22.9369293349593,
12.));
#243962=CARTESIAN_POINT('Ctrl Pts',(-7.66129790094108,22.9147345215421,
12.));
#243963=CARTESIAN_POINT('Ctrl Pts',(-7.66225015950156,22.8926334544883,
12.));
#243964=CARTESIAN_POINT('Ctrl Pts',(-7.66314184287337,22.8706268461283,
12.));
#243965=CARTESIAN_POINT('Ctrl Pts',(-7.66397328929803,22.848715415557,12.));
#243966=CARTESIAN_POINT('Ctrl Pts',(-7.66474484198549,22.8268998887678,
12.));
#243967=CARTESIAN_POINT('Ctrl Pts',(-7.66545684920987,22.8051809987833,
12.));
#243968=CARTESIAN_POINT('Ctrl Pts',(-7.66610966441273,22.7835594857699,
12.));
#243969=CARTESIAN_POINT('Ctrl Pts',(-7.66670364630299,22.7620360971843,
12.));
#243970=CARTESIAN_POINT('Ctrl Pts',(-7.6672391589544,22.7406115879513,12.));
#243971=CARTESIAN_POINT('Ctrl Pts',(-7.66771657191027,22.7192867206245,
12.));
#243972=CARTESIAN_POINT('Ctrl Pts',(-7.66813626029275,22.6980622655446,
12.));
#243973=CARTESIAN_POINT('Ctrl Pts',(-7.66849860491743,22.6769390009885,
12.));
#243974=CARTESIAN_POINT('Ctrl Pts',(-7.66880399241323,22.6559177133127,
12.));
#243975=CARTESIAN_POINT('Ctrl Pts',(-7.66905281533715,22.6349991971541,
12.));
#243976=CARTESIAN_POINT('Ctrl Pts',(-7.66924547229414,22.6141842556243,
12.));
#243977=CARTESIAN_POINT('Ctrl Pts',(-7.66938236806233,22.5934737004953,
12.));
#243978=CARTESIAN_POINT('Ctrl Pts',(-7.66946391372306,22.5728683523831,
12.));
#243979=CARTESIAN_POINT('Ctrl Pts',(-7.66949052679693,22.5523690409116,
12.));
#243980=CARTESIAN_POINT('Ctrl Pts',(-7.66946263138144,22.53197660492,12.));
#243981=CARTESIAN_POINT('Ctrl Pts',(-7.66938065829108,22.5116918927031,
12.));
#243982=CARTESIAN_POINT('Ctrl Pts',(-7.66924504520315,22.4915157622312,
12.));
#243983=CARTESIAN_POINT('Ctrl Pts',(-7.66905623680831,22.47144908137,12.));
#243984=CARTESIAN_POINT('Ctrl Pts',(-7.66881468496635,22.4514927280855,
12.));
#243985=CARTESIAN_POINT('Ctrl Pts',(-7.66852084886704,22.4316475906603,
12.));
#243986=CARTESIAN_POINT('Ctrl Pts',(-7.6681751951964,22.4119145679758,12.));
#243987=CARTESIAN_POINT('Ctrl Pts',(-7.6677781983079,22.3922945697773,12.));
#243988=CARTESIAN_POINT('Ctrl Pts',(-7.66733034039883,22.372788516936,12.));
#243989=CARTESIAN_POINT('Ctrl Pts',(-7.66683211169158,22.3533973417021,
12.));
#243990=CARTESIAN_POINT('Ctrl Pts',(-7.66628401061952,22.3341219879469,
12.));
#243991=CARTESIAN_POINT('Ctrl Pts',(-7.66568654402494,22.314963411484,12.));
#243992=CARTESIAN_POINT('Ctrl Pts',(-7.66504022736299,22.2959225803937,
12.));
#243993=CARTESIAN_POINT('Ctrl Pts',(-7.66434558490979,22.2770004753335,
12.));
#243994=CARTESIAN_POINT('Ctrl Pts',(-7.66360314997641,22.258198089848,12.));
#243995=CARTESIAN_POINT('Ctrl Pts',(-7.66281346512509,22.2395164306547,
12.));
#243996=CARTESIAN_POINT('Ctrl Pts',(-7.661977082404,22.2209565180085,12.));
#243997=CARTESIAN_POINT('Ctrl Pts',(-7.66109456359271,22.2025193860964,
12.));
#243998=CARTESIAN_POINT('Ctrl Pts',(-7.66016648045005,22.1842060834091,
12.));
#243999=CARTESIAN_POINT('Ctrl Pts',(-7.6591934149693,22.1660176731178,12.));
#244000=CARTESIAN_POINT('Ctrl Pts',(-7.65817595963349,22.1479552334211,
12.));
#244001=CARTESIAN_POINT('Ctrl Pts',(-7.65711471769397,22.1300198579675,
12.));
#244002=CARTESIAN_POINT('Ctrl Pts',(-7.65601030346807,22.1122126563329,
12.));
#244003=CARTESIAN_POINT('Ctrl Pts',(-7.65486334263644,22.094534754469,12.));
#244004=CARTESIAN_POINT('Ctrl Pts',(-7.65367447254949,22.0769872951596,
12.));
#244005=CARTESIAN_POINT('Ctrl Pts',(-7.65244434253113,22.0595714384431,
12.));
#244006=CARTESIAN_POINT('Ctrl Pts',(-7.65117361421358,22.0422883621174,
12.));
#244007=CARTESIAN_POINT('Ctrl Pts',(-7.64986296190168,22.0251392623209,
12.));
#244008=CARTESIAN_POINT('Ctrl Pts',(-7.64851307293352,22.0081253540774,
12.));
#244009=CARTESIAN_POINT('Ctrl Pts',(-7.6471246480525,21.9912478718542,12.));
#244010=CARTESIAN_POINT('Ctrl Pts',(-7.64569840177336,21.9745080700798,
12.));
#244011=CARTESIAN_POINT('Ctrl Pts',(-7.64423506279123,21.9579072237651,
12.));
#244012=CARTESIAN_POINT('Ctrl Pts',(-7.64273537442682,21.9414466292072,
12.));
#244013=CARTESIAN_POINT('Ctrl Pts',(-7.64120009506532,21.9251276046546,
12.));
#244014=CARTESIAN_POINT('Ctrl Pts',(-7.63962999860927,21.9089514909874,
12.));
#244015=CARTESIAN_POINT('Ctrl Pts',(-7.63802587492035,21.8929196523514,
12.));
#244016=CARTESIAN_POINT('Ctrl Pts',(-7.636388530334,21.8770334769496,12.));
#244017=CARTESIAN_POINT('Ctrl Pts',(-7.63471878821226,21.8612943779089,
12.));
#244018=CARTESIAN_POINT('Ctrl Pts',(-7.63301748948936,21.8457037941084,
12.));
#244019=CARTESIAN_POINT('Ctrl Pts',(-7.63128549323023,21.8302631910195,
12.));
#244020=CARTESIAN_POINT('Ctrl Pts',(-7.62952367718127,21.814974061509,12.));
#244021=CARTESIAN_POINT('Ctrl Pts',(-7.62773293842389,21.799837926858,12.));
#244022=CARTESIAN_POINT('Ctrl Pts',(-7.62591419404512,21.7848563378021,
12.));
#244023=CARTESIAN_POINT('Ctrl Pts',(-7.62406838181166,21.7700308755584,
12.));
#244024=CARTESIAN_POINT('Ctrl Pts',(-7.62219646084228,21.7553631528328,
12.));
#244025=CARTESIAN_POINT('Ctrl Pts',(-7.62029941230855,21.7408548148656,
12.));
#244026=CARTESIAN_POINT('Ctrl Pts',(-7.61837824030538,21.7265075407975,
12.));
#244027=CARTESIAN_POINT('Ctrl Pts',(-7.61643397270421,21.7123230449834,
12.));
#244028=CARTESIAN_POINT('Ctrl Pts',(-7.61446766202787,21.6983030783322,
12.));
#244029=CARTESIAN_POINT('Ctrl Pts',(-7.61248038630268,21.6844494295815,
12.));
#244030=CARTESIAN_POINT('Ctrl Pts',(-7.61047325000956,21.6707639267576,
12.));
#244031=CARTESIAN_POINT('Ctrl Pts',(-7.60844738512874,21.6572484388081,
12.));
#244032=CARTESIAN_POINT('Ctrl Pts',(-7.60640395216357,21.6439048771743,
12.));
#244033=CARTESIAN_POINT('Ctrl Pts',(-7.60434414118296,21.6307351973822,
12.));
#244034=CARTESIAN_POINT('Ctrl Pts',(-7.60226917285429,21.617741400599,12.));
#244035=CARTESIAN_POINT('Ctrl Pts',(-7.60018029988241,21.6049255358843,
12.));
#244036=CARTESIAN_POINT('Ctrl Pts',(-7.59807880846195,21.5922897024466,
12.));
#244037=CARTESIAN_POINT('Ctrl Pts',(-7.59596601973584,21.5798360518978,
12.));
#244038=CARTESIAN_POINT('Ctrl Pts',(-7.59384329124918,21.5675667904726,
12.));
#244039=CARTESIAN_POINT('Ctrl Pts',(-7.59171201844777,21.5554841813462,
12.));
#244040=CARTESIAN_POINT('Ctrl Pts',(-7.58957363620014,21.543590547011,12.));
#244041=CARTESIAN_POINT('Ctrl Pts',(-7.58742962034834,21.5318882716736,
12.));
#244042=CARTESIAN_POINT('Ctrl Pts',(-7.5852814891913,21.5203798035299,12.));
#244043=CARTESIAN_POINT('Ctrl Pts',(-7.5831308051918,21.5090676573873,12.));
#244044=CARTESIAN_POINT('Ctrl Pts',(-7.58097917790744,21.4979544192744,
12.));
#244045=CARTESIAN_POINT('Ctrl Pts',(-7.57882826679132,21.4870427508194,
12.));
#244046=CARTESIAN_POINT('Ctrl Pts',(-7.57667978402987,21.4763353936762,
12.));
#244047=CARTESIAN_POINT('Ctrl Pts',(-7.57453549743412,21.4658351740128,
12.));
#244048=CARTESIAN_POINT('Ctrl Pts',(-7.57239723223506,21.4555450053142,
12.));
#244049=CARTESIAN_POINT('Ctrl Pts',(-7.57026687261166,21.4454678907509,
12.));
#244050=CARTESIAN_POINT('Ctrl Pts',(-7.56814636360847,21.4356069261513,
12.));
#244051=CARTESIAN_POINT('Ctrl Pts',(-7.56603771218712,21.4259653015736,
12.));
#244052=CARTESIAN_POINT('Ctrl Pts',(-7.56394299313685,21.4165463106254,
12.));
#244053=CARTESIAN_POINT('Ctrl Pts',(-7.56186435703622,21.4073533630365,
12.));
#244054=CARTESIAN_POINT('Ctrl Pts',(-7.55980403700611,21.3983899952987,
12.));
#244055=CARTESIAN_POINT('Ctrl Pts',(-7.55776435731417,21.3896598842117,
12.));
#244056=CARTESIAN_POINT('Ctrl Pts',(-7.55574773403503,21.3811668478932,
12.));
#244057=CARTESIAN_POINT('Ctrl Pts',(-7.55375667080029,21.3729148390243,
12.));
#244058=CARTESIAN_POINT('Ctrl Pts',(-7.55179375777444,21.3649079431865,
12.));
#244059=CARTESIAN_POINT('Ctrl Pts',(-7.5498616652131,21.3571503685855,12.));
#244060=CARTESIAN_POINT('Ctrl Pts',(-7.5479631624633,21.3496464761531,12.));
#244061=CARTESIAN_POINT('Ctrl Pts',(-7.54610114948347,21.3424008295038,
12.));
#244062=CARTESIAN_POINT('Ctrl Pts',(-7.54427868151268,21.3354182340149,
12.));
#244063=CARTESIAN_POINT('Ctrl Pts',(-7.54249900377031,21.328703791771,12.));
#244064=CARTESIAN_POINT('Ctrl Pts',(-7.54076552038279,21.3222628524165,
12.));
#244065=CARTESIAN_POINT('Ctrl Pts',(-7.53908175169898,21.3161009456256,
12.));
#244066=CARTESIAN_POINT('Ctrl Pts',(-7.53745129364616,21.310223716773,12.));
#244067=CARTESIAN_POINT('Ctrl Pts',(-7.53587778251736,21.3046368712157,
12.));
#244068=CARTESIAN_POINT('Ctrl Pts',(-7.53436505309943,21.2993464250717,
12.));
#244069=CARTESIAN_POINT('Ctrl Pts',(-7.53291726078527,21.2943588989331,
12.));
#244070=CARTESIAN_POINT('Ctrl Pts',(-7.53153906987855,21.2896816163842,
12.));
#244071=CARTESIAN_POINT('Ctrl Pts',(-7.53023562438229,21.2853226580657,
12.));
#244072=CARTESIAN_POINT('Ctrl Pts',(-7.52901217930408,21.2812902781143,
12.));
#244073=CARTESIAN_POINT('Ctrl Pts',(-7.52787386225333,21.2775925269652,
12.));
#244074=CARTESIAN_POINT('Ctrl Pts',(-7.52682526918541,21.2742366113579,
12.));
#244075=CARTESIAN_POINT('Ctrl Pts',(-7.5258712609553,21.2712301573466,12.));
#244076=CARTESIAN_POINT('Ctrl Pts',(-7.5250177033353,21.2685823838671,12.));
#244077=CARTESIAN_POINT('Ctrl Pts',(-7.52427261074298,21.2663059157058,
12.));
#244078=CARTESIAN_POINT('Ctrl Pts',(-7.52364573027553,21.2644161259962,
12.));
#244079=CARTESIAN_POINT('Ctrl Pts',(-7.52314642316199,21.262927782038,12.));
#244080=CARTESIAN_POINT('Ctrl Pts',(-7.5227818224267,21.2618521283555,12.));
#244081=CARTESIAN_POINT('Ctrl Pts',(-7.52260064231661,21.261326054066,12.));
#244082=CARTESIAN_POINT('Ctrl Pts',(-7.52252744144904,21.2611204474866,
12.));
#244083=CARTESIAN_POINT('Ctrl Pts',(-7.5225064970397,21.2610673466886,12.));
#244084=CARTESIAN_POINT('Ctrl Pts',(-7.52250298901264,21.2610617890679,
12.));
#244085=CARTESIAN_POINT('',(-7.36589684767344,24.9347862158358,0.));
#244086=CARTESIAN_POINT('Origin',(-1.68110656504246,21.4341755315424,0.));
#244087=CARTESIAN_POINT('',(-1.76341220531179,22.4835757167854,12.));
#244088=CARTESIAN_POINT('',(-0.840553282521227,10.7170877657712,12.));
#244089=CARTESIAN_POINT('',(-1.76341220531179,22.4835757167854,0.));
#244090=CARTESIAN_POINT('',(-1.76341220531179,22.4835757167854,0.));
#244091=CARTESIAN_POINT('',(-0.840553282521227,10.7170877657712,0.));
#244092=CARTESIAN_POINT('Ctrl Pts',(-6.08833931617698,25.2771067246846,
0.));
#244093=CARTESIAN_POINT('Ctrl Pts',(-6.08833931617698,25.2771067246846,
12.));
#244094=CARTESIAN_POINT('Ctrl Pts',(-6.08441489609824,25.2729539149479,
0.));
#244095=CARTESIAN_POINT('Ctrl Pts',(-6.08441489609824,25.2729539149479,
12.));
#244096=CARTESIAN_POINT('Ctrl Pts',(-6.07657531787578,25.2646490489816,
0.));
#244097=CARTESIAN_POINT('Ctrl Pts',(-6.07657531787578,25.2646490489816,
12.));
#244098=CARTESIAN_POINT('Ctrl Pts',(-6.06484373634697,25.2521940105523,
0.));
#244099=CARTESIAN_POINT('Ctrl Pts',(-6.06484373634697,25.2521940105523,
12.));
#244100=CARTESIAN_POINT('Ctrl Pts',(-6.04925720151412,25.2355918138798,
0.));
#244101=CARTESIAN_POINT('Ctrl Pts',(-6.04925720151412,25.2355918138798,
12.));
#244102=CARTESIAN_POINT('Ctrl Pts',(-6.02986667390187,25.2148466201368,
0.));
#244103=CARTESIAN_POINT('Ctrl Pts',(-6.02986667390187,25.2148466201368,
12.));
#244104=CARTESIAN_POINT('Ctrl Pts',(-6.0105688180476,25.1941090269638,0.));
#244105=CARTESIAN_POINT('Ctrl Pts',(-6.0105688180476,25.1941090269638,12.));
#244106=CARTESIAN_POINT('Ctrl Pts',(-5.99136367859838,25.1733791296154,
0.));
#244107=CARTESIAN_POINT('Ctrl Pts',(-5.99136367859838,25.1733791296154,
12.));
#244108=CARTESIAN_POINT('Ctrl Pts',(-5.97225131495636,25.1526570863065,
0.));
#244109=CARTESIAN_POINT('Ctrl Pts',(-5.97225131495636,25.1526570863065,
12.));
#244110=CARTESIAN_POINT('Ctrl Pts',(-5.95323180187348,25.1319431317273,
0.));
#244111=CARTESIAN_POINT('Ctrl Pts',(-5.95323180187348,25.1319431317273,
12.));
#244112=CARTESIAN_POINT('Ctrl Pts',(-5.93430523086776,25.1112375971182,
0.));
#244113=CARTESIAN_POINT('Ctrl Pts',(-5.93430523086776,25.1112375971182,
12.));
#244114=CARTESIAN_POINT('Ctrl Pts',(-5.91547170844382,25.0905409050863,
0.));
#244115=CARTESIAN_POINT('Ctrl Pts',(-5.91547170844382,25.0905409050863,
12.));
#244116=CARTESIAN_POINT('Ctrl Pts',(-5.89673135155459,25.0698535426593,
0.));
#244117=CARTESIAN_POINT('Ctrl Pts',(-5.89673135155459,25.0698535426593,
12.));
#244118=CARTESIAN_POINT('Ctrl Pts',(-5.87808428385329,25.0491760405965,
0.));
#244119=CARTESIAN_POINT('Ctrl Pts',(-5.87808428385329,25.0491760405965,
12.));
#244120=CARTESIAN_POINT('Ctrl Pts',(-5.8595306315681,25.0285089498922,0.));
#244121=CARTESIAN_POINT('Ctrl Pts',(-5.8595306315681,25.0285089498922,12.));
#244122=CARTESIAN_POINT('Ctrl Pts',(-5.84107051963073,25.0078528200558,
0.));
#244123=CARTESIAN_POINT('Ctrl Pts',(-5.84107051963073,25.0078528200558,
12.));
#244124=CARTESIAN_POINT('Ctrl Pts',(-5.82270406744214,24.9872081752709,
0.));
#244125=CARTESIAN_POINT('Ctrl Pts',(-5.82270406744214,24.9872081752709,
12.));
#244126=CARTESIAN_POINT('Ctrl Pts',(-5.80443138549747,24.9665754954462,
0.));
#244127=CARTESIAN_POINT('Ctrl Pts',(-5.80443138549747,24.9665754954462,
12.));
#244128=CARTESIAN_POINT('Ctrl Pts',(-5.78625257775703,24.9459552293308,
0.));
#244129=CARTESIAN_POINT('Ctrl Pts',(-5.78625257775703,24.9459552293308,
12.));
#244130=CARTESIAN_POINT('Ctrl Pts',(-5.76816774342236,24.9253478043632,
0.));
#244131=CARTESIAN_POINT('Ctrl Pts',(-5.76816774342236,24.9253478043632,
12.));
#244132=CARTESIAN_POINT('Ctrl Pts',(-5.75017697890813,24.9047536376467,
0.));
#244133=CARTESIAN_POINT('Ctrl Pts',(-5.75017697890813,24.9047536376467,
12.));
#244134=CARTESIAN_POINT('Ctrl Pts',(-5.73228037976927,24.8841731467219,
0.));
#244135=CARTESIAN_POINT('Ctrl Pts',(-5.73228037976927,24.8841731467219,
12.));
#244136=CARTESIAN_POINT('Ctrl Pts',(-5.71447804252019,24.8636067597677,
0.));
#244137=CARTESIAN_POINT('Ctrl Pts',(-5.71447804252019,24.8636067597677,
12.));
#244138=CARTESIAN_POINT('Ctrl Pts',(-5.69677006679429,24.8430549277634,
0.));
#244139=CARTESIAN_POINT('Ctrl Pts',(-5.69677006679429,24.8430549277634,
12.));
#244140=CARTESIAN_POINT('Ctrl Pts',(-5.67915655496524,24.822518122386,0.));
#244141=CARTESIAN_POINT('Ctrl Pts',(-5.67915655496524,24.822518122386,12.));
#244142=CARTESIAN_POINT('Ctrl Pts',(-5.66163761114903,24.8019968304618,
0.));
#244143=CARTESIAN_POINT('Ctrl Pts',(-5.66163761114903,24.8019968304618,
12.));
#244144=CARTESIAN_POINT('Ctrl Pts',(-5.64421334042248,24.7814915496728,
0.));
#244145=CARTESIAN_POINT('Ctrl Pts',(-5.64421334042248,24.7814915496728,
12.));
#244146=CARTESIAN_POINT('Ctrl Pts',(-5.62688384790919,24.76100278357,0.));
#244147=CARTESIAN_POINT('Ctrl Pts',(-5.62688384790919,24.76100278357,12.));
#244148=CARTESIAN_POINT('Ctrl Pts',(-5.60964923798495,24.7405310372736,
0.));
#244149=CARTESIAN_POINT('Ctrl Pts',(-5.60964923798495,24.7405310372736,
12.));
#244150=CARTESIAN_POINT('Ctrl Pts',(-5.59250961323995,24.7200768119079,
0.));
#244151=CARTESIAN_POINT('Ctrl Pts',(-5.59250961323995,24.7200768119079,
12.));
#244152=CARTESIAN_POINT('Ctrl Pts',(-5.57546507427767,24.6996406035507,
0.));
#244153=CARTESIAN_POINT('Ctrl Pts',(-5.57546507427767,24.6996406035507,
12.));
#244154=CARTESIAN_POINT('Ctrl Pts',(-5.55851572025389,24.6792229061785,
0.));
#244155=CARTESIAN_POINT('Ctrl Pts',(-5.55851572025389,24.6792229061785,
12.));
#244156=CARTESIAN_POINT('Ctrl Pts',(-5.54166164919593,24.6588242134733,
0.));
#244157=CARTESIAN_POINT('Ctrl Pts',(-5.54166164919593,24.6588242134733,
12.));
#244158=CARTESIAN_POINT('Ctrl Pts',(-5.52490295840996,24.6384450211466,
0.));
#244159=CARTESIAN_POINT('Ctrl Pts',(-5.52490295840996,24.6384450211466,
12.));
#244160=CARTESIAN_POINT('Ctrl Pts',(-5.50823974481959,24.618085828918,0.));
#244161=CARTESIAN_POINT('Ctrl Pts',(-5.50823974481959,24.618085828918,12.));
#244162=CARTESIAN_POINT('Ctrl Pts',(-5.49167210537235,24.5977471429365,
0.));
#244163=CARTESIAN_POINT('Ctrl Pts',(-5.49167210537235,24.5977471429365,
12.));
#244164=CARTESIAN_POINT('Ctrl Pts',(-5.47520013724403,24.5774294770329,
0.));
#244165=CARTESIAN_POINT('Ctrl Pts',(-5.47520013724403,24.5774294770329,
12.));
#244166=CARTESIAN_POINT('Ctrl Pts',(-5.45882393762244,24.5571333514841,
0.));
#244167=CARTESIAN_POINT('Ctrl Pts',(-5.45882393762244,24.5571333514841,
12.));
#244168=CARTESIAN_POINT('Ctrl Pts',(-5.44254360356865,24.5368592922861,
0.));
#244169=CARTESIAN_POINT('Ctrl Pts',(-5.44254360356865,24.5368592922861,
12.));
#244170=CARTESIAN_POINT('Ctrl Pts',(-5.42635923183411,24.5166078302107,
0.));
#244171=CARTESIAN_POINT('Ctrl Pts',(-5.42635923183411,24.5166078302107,
12.));
#244172=CARTESIAN_POINT('Ctrl Pts',(-5.41027091869242,24.4963794999831,
0.));
#244173=CARTESIAN_POINT('Ctrl Pts',(-5.41027091869242,24.4963794999831,
12.));
#244174=CARTESIAN_POINT('Ctrl Pts',(-5.3942787597383,24.4761748393322,0.));
#244175=CARTESIAN_POINT('Ctrl Pts',(-5.3942787597383,24.4761748393322,12.));
#244176=CARTESIAN_POINT('Ctrl Pts',(-5.37838284973706,24.4559943883159,
0.));
#244177=CARTESIAN_POINT('Ctrl Pts',(-5.37838284973706,24.4559943883159,
12.));
#244178=CARTESIAN_POINT('Ctrl Pts',(-5.36258328273639,24.4358386899152,
0.));
#244179=CARTESIAN_POINT('Ctrl Pts',(-5.36258328273639,24.4358386899152,
12.));
#244180=CARTESIAN_POINT('Ctrl Pts',(-5.34688015213546,24.4157082904615,
0.));
#244181=CARTESIAN_POINT('Ctrl Pts',(-5.34688015213546,24.4157082904615,
12.));
#244182=CARTESIAN_POINT('Ctrl Pts',(-5.33127355076037,24.3956037401293,
0.));
#244183=CARTESIAN_POINT('Ctrl Pts',(-5.33127355076037,24.3956037401293,
12.));
#244184=CARTESIAN_POINT('Ctrl Pts',(-5.31576357092524,24.3755255933917,
0.));
#244185=CARTESIAN_POINT('Ctrl Pts',(-5.31576357092524,24.3755255933917,
12.));
#244186=CARTESIAN_POINT('Ctrl Pts',(-5.30035030449059,24.3554744095075,
0.));
#244187=CARTESIAN_POINT('Ctrl Pts',(-5.30035030449059,24.3554744095075,
12.));
#244188=CARTESIAN_POINT('Ctrl Pts',(-5.28503384290644,24.3354507529415,
0.));
#244189=CARTESIAN_POINT('Ctrl Pts',(-5.28503384290644,24.3354507529415,
12.));
#244190=CARTESIAN_POINT('Ctrl Pts',(-5.26981427718796,24.3154551932222,
0.));
#244191=CARTESIAN_POINT('Ctrl Pts',(-5.26981427718796,24.3154551932222,
12.));
#244192=CARTESIAN_POINT('Ctrl Pts',(-5.25469169788856,24.2954883048448,
0.));
#244193=CARTESIAN_POINT('Ctrl Pts',(-5.25469169788856,24.2954883048448,
12.));
#244194=CARTESIAN_POINT('Ctrl Pts',(-5.23966619506289,24.2755506671526,
0.));
#244195=CARTESIAN_POINT('Ctrl Pts',(-5.23966619506289,24.2755506671526,
12.));
#244196=CARTESIAN_POINT('Ctrl Pts',(-5.22473785822441,24.2556428642294,
0.));
#244197=CARTESIAN_POINT('Ctrl Pts',(-5.22473785822441,24.2556428642294,
12.));
#244198=CARTESIAN_POINT('Ctrl Pts',(-5.20990677629173,24.2357654847765,
0.));
#244199=CARTESIAN_POINT('Ctrl Pts',(-5.20990677629173,24.2357654847765,
12.));
#244200=CARTESIAN_POINT('Ctrl Pts',(-5.19517303753643,24.215919122017,0.));
#244201=CARTESIAN_POINT('Ctrl Pts',(-5.19517303753643,24.215919122017,12.));
#244202=CARTESIAN_POINT('Ctrl Pts',(-5.18053672961392,24.1961043738754,
0.));
#244203=CARTESIAN_POINT('Ctrl Pts',(-5.18053672961392,24.1961043738754,
12.));
#244204=CARTESIAN_POINT('Ctrl Pts',(-5.16599793957979,24.1763218431343,
0.));
#244205=CARTESIAN_POINT('Ctrl Pts',(-5.16599793957979,24.1763218431343,
12.));
#244206=CARTESIAN_POINT('Ctrl Pts',(-5.15155675390075,24.156572137597,0.));
#244207=CARTESIAN_POINT('Ctrl Pts',(-5.15155675390075,24.156572137597,12.));
#244208=CARTESIAN_POINT('Ctrl Pts',(-5.13721325845745,24.1368558702443,
0.));
#244209=CARTESIAN_POINT('Ctrl Pts',(-5.13721325845745,24.1368558702443,
12.));
#244210=CARTESIAN_POINT('Ctrl Pts',(-5.12296753853859,24.117173659394,0.));
#244211=CARTESIAN_POINT('Ctrl Pts',(-5.12296753853859,24.117173659394,12.));
#244212=CARTESIAN_POINT('Ctrl Pts',(-5.10881967883132,24.0975261288446,
0.));
#244213=CARTESIAN_POINT('Ctrl Pts',(-5.10881967883132,24.0975261288446,
12.));
#244214=CARTESIAN_POINT('Ctrl Pts',(-5.09476976342625,24.0779139079266,
0.));
#244215=CARTESIAN_POINT('Ctrl Pts',(-5.09476976342625,24.0779139079266,
12.));
#244216=CARTESIAN_POINT('Ctrl Pts',(-5.08081787581276,24.0583376315638,
0.));
#244217=CARTESIAN_POINT('Ctrl Pts',(-5.08081787581276,24.0583376315638,
12.));
#244218=CARTESIAN_POINT('Ctrl Pts',(-5.06696409886641,24.0387979403268,
0.));
#244219=CARTESIAN_POINT('Ctrl Pts',(-5.06696409886641,24.0387979403268,
12.));
#244220=CARTESIAN_POINT('Ctrl Pts',(-5.05320851483065,24.0192954804896,
0.));
#244221=CARTESIAN_POINT('Ctrl Pts',(-5.05320851483065,24.0192954804896,
12.));
#244222=CARTESIAN_POINT('Ctrl Pts',(-5.03955120528521,23.9998309040746,
0.));
#244223=CARTESIAN_POINT('Ctrl Pts',(-5.03955120528521,23.9998309040746,
12.));
#244224=CARTESIAN_POINT('Ctrl Pts',(-5.02599225112454,23.9804048689227,
0.));
#244225=CARTESIAN_POINT('Ctrl Pts',(-5.02599225112454,23.9804048689227,
12.));
#244226=CARTESIAN_POINT('Ctrl Pts',(-5.01253173257453,23.9610180388271,
0.));
#244227=CARTESIAN_POINT('Ctrl Pts',(-5.01253173257453,23.9610180388271,
12.));
#244228=CARTESIAN_POINT('Ctrl Pts',(-4.99916972919307,23.9416710836529,
0.));
#244229=CARTESIAN_POINT('Ctrl Pts',(-4.99916972919307,23.9416710836529,
12.));
#244230=CARTESIAN_POINT('Ctrl Pts',(-4.98590631986533,23.9223646794592,
0.));
#244231=CARTESIAN_POINT('Ctrl Pts',(-4.98590631986533,23.9223646794592,
12.));
#244232=CARTESIAN_POINT('Ctrl Pts',(-4.97274158279227,23.9030995086163,
0.));
#244233=CARTESIAN_POINT('Ctrl Pts',(-4.97274158279227,23.9030995086163,
12.));
#244234=CARTESIAN_POINT('Ctrl Pts',(-4.95967559546561,23.8838762599218,
0.));
#244235=CARTESIAN_POINT('Ctrl Pts',(-4.95967559546561,23.8838762599218,
12.));
#244236=CARTESIAN_POINT('Ctrl Pts',(-4.9467084346586,23.8646956287168,0.));
#244237=CARTESIAN_POINT('Ctrl Pts',(-4.9467084346586,23.8646956287168,12.));
#244238=CARTESIAN_POINT('Ctrl Pts',(-4.93384017643432,23.8455583170057,
0.));
#244239=CARTESIAN_POINT('Ctrl Pts',(-4.93384017643432,23.8455583170057,
12.));
#244240=CARTESIAN_POINT('Ctrl Pts',(-4.92107089613969,23.8264650335717,
0.));
#244241=CARTESIAN_POINT('Ctrl Pts',(-4.92107089613969,23.8264650335717,
12.));
#244242=CARTESIAN_POINT('Ctrl Pts',(-4.90840066839344,23.8074164940896,
0.));
#244243=CARTESIAN_POINT('Ctrl Pts',(-4.90840066839344,23.8074164940896,
12.));
#244244=CARTESIAN_POINT('Ctrl Pts',(-4.89582956706775,23.7884134212384,
0.));
#244245=CARTESIAN_POINT('Ctrl Pts',(-4.89582956706775,23.7884134212384,
12.));
#244246=CARTESIAN_POINT('Ctrl Pts',(-4.88335766525573,23.7694565448049,
0.));
#244247=CARTESIAN_POINT('Ctrl Pts',(-4.88335766525573,23.7694565448049,
12.));
#244248=CARTESIAN_POINT('Ctrl Pts',(-4.87098503527152,23.7505466018245,
0.));
#244249=CARTESIAN_POINT('Ctrl Pts',(-4.87098503527152,23.7505466018245,
12.));
#244250=CARTESIAN_POINT('Ctrl Pts',(-4.85871174865499,23.7316843367313,
0.));
#244251=CARTESIAN_POINT('Ctrl Pts',(-4.85871174865499,23.7316843367313,
12.));
#244252=CARTESIAN_POINT('Ctrl Pts',(-4.84653787616425,23.7128705015017,
0.));
#244253=CARTESIAN_POINT('Ctrl Pts',(-4.84653787616425,23.7128705015017,
12.));
#244254=CARTESIAN_POINT('Ctrl Pts',(-4.83446348776266,23.6941058557971,
0.));
#244255=CARTESIAN_POINT('Ctrl Pts',(-4.83446348776266,23.6941058557971,
12.));
#244256=CARTESIAN_POINT('Ctrl Pts',(-4.82248865259562,23.675391167102,0.));
#244257=CARTESIAN_POINT('Ctrl Pts',(-4.82248865259562,23.675391167102,12.));
#244258=CARTESIAN_POINT('Ctrl Pts',(-4.81061343896432,23.6567272108628,
0.));
#244259=CARTESIAN_POINT('Ctrl Pts',(-4.81061343896432,23.6567272108628,
12.));
#244260=CARTESIAN_POINT('Ctrl Pts',(-4.7988379143322,23.6381147706579,0.));
#244261=CARTESIAN_POINT('Ctrl Pts',(-4.7988379143322,23.6381147706579,12.));
#244262=CARTESIAN_POINT('Ctrl Pts',(-4.78716214532098,23.6195546383624,
0.));
#244263=CARTESIAN_POINT('Ctrl Pts',(-4.78716214532098,23.6195546383624,
12.));
#244264=CARTESIAN_POINT('Ctrl Pts',(-4.77558619769872,23.6010476143099,
0.));
#244265=CARTESIAN_POINT('Ctrl Pts',(-4.77558619769872,23.6010476143099,
12.));
#244266=CARTESIAN_POINT('Ctrl Pts',(-4.76411013636251,23.5825945074535,
0.));
#244267=CARTESIAN_POINT('Ctrl Pts',(-4.76411013636251,23.5825945074535,
12.));
#244268=CARTESIAN_POINT('Ctrl Pts',(-4.75273402530617,23.5641961355168,
0.));
#244269=CARTESIAN_POINT('Ctrl Pts',(-4.75273402530617,23.5641961355168,
12.));
#244270=CARTESIAN_POINT('Ctrl Pts',(-4.74145792760698,23.545853325171,0.));
#244271=CARTESIAN_POINT('Ctrl Pts',(-4.74145792760698,23.545853325171,12.));
#244272=CARTESIAN_POINT('Ctrl Pts',(-4.7302819054303,23.5275669122372,0.));
#244273=CARTESIAN_POINT('Ctrl Pts',(-4.7302819054303,23.5275669122372,12.));
#244274=CARTESIAN_POINT('Ctrl Pts',(-4.71920602001902,23.509337741878,0.));
#244275=CARTESIAN_POINT('Ctrl Pts',(-4.71920602001902,23.509337741878,12.));
#244276=CARTESIAN_POINT('Ctrl Pts',(-4.70823033167819,23.491166668789,0.));
#244277=CARTESIAN_POINT('Ctrl Pts',(-4.70823033167819,23.491166668789,12.));
#244278=CARTESIAN_POINT('Ctrl Pts',(-4.69735489975024,23.4730545573853,
0.));
#244279=CARTESIAN_POINT('Ctrl Pts',(-4.69735489975024,23.4730545573853,
12.));
#244280=CARTESIAN_POINT('Ctrl Pts',(-4.68657978258303,23.455002281986,0.));
#244281=CARTESIAN_POINT('Ctrl Pts',(-4.68657978258303,23.455002281986,12.));
#244282=CARTESIAN_POINT('Ctrl Pts',(-4.67590503753058,23.4370107270451,
0.));
#244283=CARTESIAN_POINT('Ctrl Pts',(-4.67590503753058,23.4370107270451,
12.));
#244284=CARTESIAN_POINT('Ctrl Pts',(-4.6653307209467,23.4190807873803,0.));
#244285=CARTESIAN_POINT('Ctrl Pts',(-4.6653307209467,23.4190807873803,12.));
#244286=CARTESIAN_POINT('Ctrl Pts',(-4.65485688816924,23.4012133683959,
0.));
#244287=CARTESIAN_POINT('Ctrl Pts',(-4.65485688816924,23.4012133683959,
12.));
#244288=CARTESIAN_POINT('Ctrl Pts',(-4.6444835934993,23.3834093863068,0.));
#244289=CARTESIAN_POINT('Ctrl Pts',(-4.6444835934993,23.3834093863068,12.));
#244290=CARTESIAN_POINT('Ctrl Pts',(-4.63421089016541,23.3656697683489,
0.));
#244291=CARTESIAN_POINT('Ctrl Pts',(-4.63421089016541,23.3656697683489,
12.));
#244292=CARTESIAN_POINT('Ctrl Pts',(-4.62403883030805,23.3479954530272,
0.));
#244293=CARTESIAN_POINT('Ctrl Pts',(-4.62403883030805,23.3479954530272,
12.));
#244294=CARTESIAN_POINT('Ctrl Pts',(-4.6139674649783,23.3303873903938,0.));
#244295=CARTESIAN_POINT('Ctrl Pts',(-4.6139674649783,23.3303873903938,12.));
#244296=CARTESIAN_POINT('Ctrl Pts',(-4.60399684412163,23.3128465423115,
0.));
#244297=CARTESIAN_POINT('Ctrl Pts',(-4.60399684412163,23.3128465423115,
12.));
#244298=CARTESIAN_POINT('Ctrl Pts',(-4.5941270165575,23.2953738827191,0.));
#244299=CARTESIAN_POINT('Ctrl Pts',(-4.5941270165575,23.2953738827191,12.));
#244300=CARTESIAN_POINT('Ctrl Pts',(-4.5843580299469,23.2779703978876,0.));
#244301=CARTESIAN_POINT('Ctrl Pts',(-4.5843580299469,23.2779703978876,12.));
#244302=CARTESIAN_POINT('Ctrl Pts',(-4.57468993076097,23.2606370866866,
0.));
#244303=CARTESIAN_POINT('Ctrl Pts',(-4.57468993076097,23.2606370866866,
12.));
#244304=CARTESIAN_POINT('Ctrl Pts',(-4.56512276427839,23.2433749609131,
0.));
#244305=CARTESIAN_POINT('Ctrl Pts',(-4.56512276427839,23.2433749609131,
12.));
#244306=CARTESIAN_POINT('Ctrl Pts',(-4.55565657456975,23.2261850456064,
0.));
#244307=CARTESIAN_POINT('Ctrl Pts',(-4.55565657456975,23.2261850456064,
12.));
#244308=CARTESIAN_POINT('Ctrl Pts',(-4.54629140447544,23.2090683793629,
0.));
#244309=CARTESIAN_POINT('Ctrl Pts',(-4.54629140447544,23.2090683793629,
12.));
#244310=CARTESIAN_POINT('Ctrl Pts',(-4.53702729557566,23.1920260146465,
0.));
#244311=CARTESIAN_POINT('Ctrl Pts',(-4.53702729557566,23.1920260146465,
12.));
#244312=CARTESIAN_POINT('Ctrl Pts',(-4.52786428815015,23.1750590180908,
0.));
#244313=CARTESIAN_POINT('Ctrl Pts',(-4.52786428815015,23.1750590180908,
12.));
#244314=CARTESIAN_POINT('Ctrl Pts',(-4.51880242116748,23.1581684708761,
0.));
#244315=CARTESIAN_POINT('Ctrl Pts',(-4.51880242116748,23.1581684708761,
12.));
#244316=CARTESIAN_POINT('Ctrl Pts',(-4.5098417322706,23.1413554691123,0.));
#244317=CARTESIAN_POINT('Ctrl Pts',(-4.5098417322706,23.1413554691123,12.));
#244318=CARTESIAN_POINT('Ctrl Pts',(-4.50098225775171,23.1246211242115,
0.));
#244319=CARTESIAN_POINT('Ctrl Pts',(-4.50098225775171,23.1246211242115,
12.));
#244320=CARTESIAN_POINT('Ctrl Pts',(-4.49222403252216,23.1079665632636,
0.));
#244321=CARTESIAN_POINT('Ctrl Pts',(-4.49222403252216,23.1079665632636,
12.));
#244322=CARTESIAN_POINT('Ctrl Pts',(-4.48356709006788,23.0913929293922,
0.));
#244323=CARTESIAN_POINT('Ctrl Pts',(-4.48356709006788,23.0913929293922,
12.));
#244324=CARTESIAN_POINT('Ctrl Pts',(-4.47501146242856,23.0749013821881,
0.));
#244325=CARTESIAN_POINT('Ctrl Pts',(-4.47501146242856,23.0749013821881,
12.));
#244326=CARTESIAN_POINT('Ctrl Pts',(-4.4665571801823,23.0584930981732,0.));
#244327=CARTESIAN_POINT('Ctrl Pts',(-4.4665571801823,23.0584930981732,12.));
#244328=CARTESIAN_POINT('Ctrl Pts',(-4.45820427241683,23.0421692712467,
0.));
#244329=CARTESIAN_POINT('Ctrl Pts',(-4.45820427241683,23.0421692712467,
12.));
#244330=CARTESIAN_POINT('Ctrl Pts',(-4.44995276669686,23.0259311131392,
0.));
#244331=CARTESIAN_POINT('Ctrl Pts',(-4.44995276669686,23.0259311131392,
12.));
#244332=CARTESIAN_POINT('Ctrl Pts',(-4.44180268901643,23.0097798538395,
0.));
#244333=CARTESIAN_POINT('Ctrl Pts',(-4.44180268901643,23.0097798538395,
12.));
#244334=CARTESIAN_POINT('Ctrl Pts',(-4.43375406376879,22.9937167421006,
0.));
#244335=CARTESIAN_POINT('Ctrl Pts',(-4.43375406376879,22.9937167421006,
12.));
#244336=CARTESIAN_POINT('Ctrl Pts',(-4.42580691372751,22.977743046002,0.));
#244337=CARTESIAN_POINT('Ctrl Pts',(-4.42580691372751,22.977743046002,12.));
#244338=CARTESIAN_POINT('Ctrl Pts',(-4.41796126001302,22.9618600534866,
0.));
#244339=CARTESIAN_POINT('Ctrl Pts',(-4.41796126001302,22.9618600534866,
12.));
#244340=CARTESIAN_POINT('Ctrl Pts',(-4.41021712205553,22.9460690729093,
0.));
#244341=CARTESIAN_POINT('Ctrl Pts',(-4.41021712205553,22.9460690729093,
12.));
#244342=CARTESIAN_POINT('Ctrl Pts',(-4.40257451754323,22.930371433555,0.));
#244343=CARTESIAN_POINT('Ctrl Pts',(-4.40257451754323,22.930371433555,12.));
#244344=CARTESIAN_POINT('Ctrl Pts',(-4.39503346238473,22.9147684862426,
0.));
#244345=CARTESIAN_POINT('Ctrl Pts',(-4.39503346238473,22.9147684862426,
12.));
#244346=CARTESIAN_POINT('Ctrl Pts',(-4.38759397068406,22.8992616040108,
0.));
#244347=CARTESIAN_POINT('Ctrl Pts',(-4.38759397068406,22.8992616040108,
12.));
#244348=CARTESIAN_POINT('Ctrl Pts',(-4.38025605470093,22.8838521827701,
0.));
#244349=CARTESIAN_POINT('Ctrl Pts',(-4.38025605470093,22.8838521827701,
12.));
#244350=CARTESIAN_POINT('Ctrl Pts',(-4.37301972480746,22.8685416419725,
0.));
#244351=CARTESIAN_POINT('Ctrl Pts',(-4.37301972480746,22.8685416419725,
12.));
#244352=CARTESIAN_POINT('Ctrl Pts',(-4.36588498942997,22.8533314252422,
0.));
#244353=CARTESIAN_POINT('Ctrl Pts',(-4.36588498942997,22.8533314252422,
12.));
#244354=CARTESIAN_POINT('Ctrl Pts',(-4.35885185500546,22.8382230011184,
0.));
#244355=CARTESIAN_POINT('Ctrl Pts',(-4.35885185500546,22.8382230011184,
12.));
#244356=CARTESIAN_POINT('Ctrl Pts',(-4.35192032594791,22.8232178638876,
0.));
#244357=CARTESIAN_POINT('Ctrl Pts',(-4.35192032594791,22.8232178638876,
12.));
#244358=CARTESIAN_POINT('Ctrl Pts',(-4.34509040460062,22.8083175343791,
0.));
#244359=CARTESIAN_POINT('Ctrl Pts',(-4.34509040460062,22.8083175343791,
12.));
#244360=CARTESIAN_POINT('Ctrl Pts',(-4.33836209118446,22.7935235607806,
0.));
#244361=CARTESIAN_POINT('Ctrl Pts',(-4.33836209118446,22.7935235607806,
12.));
#244362=CARTESIAN_POINT('Ctrl Pts',(-4.3317353837319,22.7788375194076,0.));
#244363=CARTESIAN_POINT('Ctrl Pts',(-4.3317353837319,22.7788375194076,12.));
#244364=CARTESIAN_POINT('Ctrl Pts',(-4.32521027803754,22.7642610156475,
0.));
#244365=CARTESIAN_POINT('Ctrl Pts',(-4.32521027803754,22.7642610156475,
12.));
#244366=CARTESIAN_POINT('Ctrl Pts',(-4.31878676761235,22.7497956849848,
0.));
#244367=CARTESIAN_POINT('Ctrl Pts',(-4.31878676761235,22.7497956849848,
12.));
#244368=CARTESIAN_POINT('Ctrl Pts',(-4.31246484362549,22.7354431939926,
0.));
#244369=CARTESIAN_POINT('Ctrl Pts',(-4.31246484362549,22.7354431939926,
12.));
#244370=CARTESIAN_POINT('Ctrl Pts',(-4.30624449484069,22.7212052413386,
0.));
#244371=CARTESIAN_POINT('Ctrl Pts',(-4.30624449484069,22.7212052413386,
12.));
#244372=CARTESIAN_POINT('Ctrl Pts',(-4.3001257075406,22.7070835587564,0.));
#244373=CARTESIAN_POINT('Ctrl Pts',(-4.3001257075406,22.7070835587564,12.));
#244374=CARTESIAN_POINT('Ctrl Pts',(-4.29410846547056,22.6930799122548,
0.));
#244375=CARTESIAN_POINT('Ctrl Pts',(-4.29410846547056,22.6930799122548,
12.));
#244376=CARTESIAN_POINT('Ctrl Pts',(-4.28819274977763,22.6791961033538,
0.));
#244377=CARTESIAN_POINT('Ctrl Pts',(-4.28819274977763,22.6791961033538,
12.));
#244378=CARTESIAN_POINT('Ctrl Pts',(-4.28237853894059,22.6654339703109,
0.));
#244379=CARTESIAN_POINT('Ctrl Pts',(-4.28237853894059,22.6654339703109,
12.));
#244380=CARTESIAN_POINT('Ctrl Pts',(-4.2766658086912,22.6517953893303,0.));
#244381=CARTESIAN_POINT('Ctrl Pts',(-4.2766658086912,22.6517953893303,12.));
#244382=CARTESIAN_POINT('Ctrl Pts',(-4.27105453193004,22.6382822758172,
0.));
#244383=CARTESIAN_POINT('Ctrl Pts',(-4.27105453193004,22.6382822758172,
12.));
#244384=CARTESIAN_POINT('Ctrl Pts',(-4.26554467865576,22.6248965859977,
0.));
#244385=CARTESIAN_POINT('Ctrl Pts',(-4.26554467865576,22.6248965859977,
12.));
#244386=CARTESIAN_POINT('Ctrl Pts',(-4.26013621588305,22.6116403184821,
0.));
#244387=CARTESIAN_POINT('Ctrl Pts',(-4.26013621588305,22.6116403184821,
12.));
#244388=CARTESIAN_POINT('Ctrl Pts',(-4.25482910755481,22.5985155158636,
0.));
#244389=CARTESIAN_POINT('Ctrl Pts',(-4.25482910755481,22.5985155158636,
12.));
#244390=CARTESIAN_POINT('Ctrl Pts',(-4.24962331444177,22.5855242662477,
0.));
#244391=CARTESIAN_POINT('Ctrl Pts',(-4.24962331444177,22.5855242662477,
12.));
#244392=CARTESIAN_POINT('Ctrl Pts',(-4.24451879404851,22.572668704992,0.));
#244393=CARTESIAN_POINT('Ctrl Pts',(-4.24451879404851,22.572668704992,12.));
#244394=CARTESIAN_POINT('Ctrl Pts',(-4.23951550052523,22.5599510166429,
0.));
#244395=CARTESIAN_POINT('Ctrl Pts',(-4.23951550052523,22.5599510166429,
12.));
#244396=CARTESIAN_POINT('Ctrl Pts',(-4.23461338456712,22.5473734368086,
0.));
#244397=CARTESIAN_POINT('Ctrl Pts',(-4.23461338456712,22.5473734368086,
12.));
#244398=CARTESIAN_POINT('Ctrl Pts',(-4.22981239330733,22.5349382540588,
0.));
#244399=CARTESIAN_POINT('Ctrl Pts',(-4.22981239330733,22.5349382540588,
12.));
#244400=CARTESIAN_POINT('Ctrl Pts',(-4.22511247020041,22.5226478117886,
0.));
#244401=CARTESIAN_POINT('Ctrl Pts',(-4.22511247020041,22.5226478117886,
12.));
#244402=CARTESIAN_POINT('Ctrl Pts',(-4.22051355490196,22.5105045108881,
0.));
#244403=CARTESIAN_POINT('Ctrl Pts',(-4.22051355490196,22.5105045108881,
12.));
#244404=CARTESIAN_POINT('Ctrl Pts',(-4.21601558313906,22.4985108124228,
0.));
#244405=CARTESIAN_POINT('Ctrl Pts',(-4.21601558313906,22.4985108124228,
12.));
#244406=CARTESIAN_POINT('Ctrl Pts',(-4.21161848657428,22.4866692403147,
0.));
#244407=CARTESIAN_POINT('Ctrl Pts',(-4.21161848657428,22.4866692403147,
12.));
#244408=CARTESIAN_POINT('Ctrl Pts',(-4.20732219265649,22.4749823839917,
0.));
#244409=CARTESIAN_POINT('Ctrl Pts',(-4.20732219265649,22.4749823839917,
12.));
#244410=CARTESIAN_POINT('Ctrl Pts',(-4.20312662448174,22.4634529011437,
0.));
#244411=CARTESIAN_POINT('Ctrl Pts',(-4.20312662448174,22.4634529011437,
12.));
#244412=CARTESIAN_POINT('Ctrl Pts',(-4.19903170066358,22.4520835205422,
0.));
#244413=CARTESIAN_POINT('Ctrl Pts',(-4.19903170066358,22.4520835205422,
12.));
#244414=CARTESIAN_POINT('Ctrl Pts',(-4.1950373351886,22.4408770448917,0.));
#244415=CARTESIAN_POINT('Ctrl Pts',(-4.1950373351886,22.4408770448917,12.));
#244416=CARTESIAN_POINT('Ctrl Pts',(-4.19114343726932,22.4298363535416,
0.));
#244417=CARTESIAN_POINT('Ctrl Pts',(-4.19114343726932,22.4298363535416,
12.));
#244418=CARTESIAN_POINT('Ctrl Pts',(-4.18734991117707,22.4189644056109,
0.));
#244419=CARTESIAN_POINT('Ctrl Pts',(-4.18734991117707,22.4189644056109,
12.));
#244420=CARTESIAN_POINT('Ctrl Pts',(-4.18365665600839,22.4082642454448,
0.));
#244421=CARTESIAN_POINT('Ctrl Pts',(-4.18365665600839,22.4082642454448,
12.));
#244422=CARTESIAN_POINT('Ctrl Pts',(-4.18006356544879,22.3977390078074,
0.));
#244423=CARTESIAN_POINT('Ctrl Pts',(-4.18006356544879,22.3977390078074,
12.));
#244424=CARTESIAN_POINT('Ctrl Pts',(-4.17657052752834,22.3873919231339,
0.));
#244425=CARTESIAN_POINT('Ctrl Pts',(-4.17657052752834,22.3873919231339,
12.));
#244426=CARTESIAN_POINT('Ctrl Pts',(-4.17317742436162,22.3772263228624,
0.));
#244427=CARTESIAN_POINT('Ctrl Pts',(-4.17317742436162,22.3772263228624,
12.));
#244428=CARTESIAN_POINT('Ctrl Pts',(-4.1698841319947,22.3672456427605,0.));
#244429=CARTESIAN_POINT('Ctrl Pts',(-4.1698841319947,22.3672456427605,12.));
#244430=CARTESIAN_POINT('Ctrl Pts',(-4.16669052026602,22.3574534257397,
0.));
#244431=CARTESIAN_POINT('Ctrl Pts',(-4.16669052026602,22.3574534257397,
12.));
#244432=CARTESIAN_POINT('Ctrl Pts',(-4.1635964526318,22.3478533253886,0.));
#244433=CARTESIAN_POINT('Ctrl Pts',(-4.1635964526318,22.3478533253886,12.));
#244434=CARTESIAN_POINT('Ctrl Pts',(-4.16060178604154,22.3384491078599,
0.));
#244435=CARTESIAN_POINT('Ctrl Pts',(-4.16060178604154,22.3384491078599,
12.));
#244436=CARTESIAN_POINT('Ctrl Pts',(-4.15770637047882,22.3292446628957,
0.));
#244437=CARTESIAN_POINT('Ctrl Pts',(-4.15770637047882,22.3292446628957,
12.));
#244438=CARTESIAN_POINT('Ctrl Pts',(-4.15491004835278,22.3202440186979,
0.));
#244439=CARTESIAN_POINT('Ctrl Pts',(-4.15491004835278,22.3202440186979,
12.));
#244440=CARTESIAN_POINT('Ctrl Pts',(-4.15221265396992,22.3114513545186,
0.));
#244441=CARTESIAN_POINT('Ctrl Pts',(-4.15221265396992,22.3114513545186,
12.));
#244442=CARTESIAN_POINT('Ctrl Pts',(-4.14961401285526,22.3028710166935,
0.));
#244443=CARTESIAN_POINT('Ctrl Pts',(-4.14961401285526,22.3028710166935,
12.));
#244444=CARTESIAN_POINT('Ctrl Pts',(-4.14711394168559,22.2945075198468,
0.));
#244445=CARTESIAN_POINT('Ctrl Pts',(-4.14711394168559,22.2945075198468,
12.));
#244446=CARTESIAN_POINT('Ctrl Pts',(-4.14471224859295,22.2863655389166,
0.));
#244447=CARTESIAN_POINT('Ctrl Pts',(-4.14471224859295,22.2863655389166,
12.));
#244448=CARTESIAN_POINT('Ctrl Pts',(-4.14240873321982,22.2784499072026,
0.));
#244449=CARTESIAN_POINT('Ctrl Pts',(-4.14240873321982,22.2784499072026,
12.));
#244450=CARTESIAN_POINT('Ctrl Pts',(-4.14020318715988,22.2707656042456,
0.));
#244451=CARTESIAN_POINT('Ctrl Pts',(-4.14020318715988,22.2707656042456,
12.));
#244452=CARTESIAN_POINT('Ctrl Pts',(-4.13809539255419,22.263317791397,0.));
#244453=CARTESIAN_POINT('Ctrl Pts',(-4.13809539255419,22.263317791397,12.));
#244454=CARTESIAN_POINT('Ctrl Pts',(-4.13608511977226,22.2561118708422,
0.));
#244455=CARTESIAN_POINT('Ctrl Pts',(-4.13608511977226,22.2561118708422,
12.));
#244456=CARTESIAN_POINT('Ctrl Pts',(-4.13417212558808,22.2491535317789,
0.));
#244457=CARTESIAN_POINT('Ctrl Pts',(-4.13417212558808,22.2491535317789,
12.));
#244458=CARTESIAN_POINT('Ctrl Pts',(-4.1323561506016,22.2424488153523,0.));
#244459=CARTESIAN_POINT('Ctrl Pts',(-4.1323561506016,22.2424488153523,12.));
#244460=CARTESIAN_POINT('Ctrl Pts',(-4.13063692157499,22.2360040565534,
0.));
#244461=CARTESIAN_POINT('Ctrl Pts',(-4.13063692157499,22.2360040565534,
12.));
#244462=CARTESIAN_POINT('Ctrl Pts',(-4.12901415463379,22.2298258043947,
0.));
#244463=CARTESIAN_POINT('Ctrl Pts',(-4.12901415463379,22.2298258043947,
12.));
#244464=CARTESIAN_POINT('Ctrl Pts',(-4.12748755830099,22.2239207458781,
0.));
#244465=CARTESIAN_POINT('Ctrl Pts',(-4.12748755830099,22.2239207458781,
12.));
#244466=CARTESIAN_POINT('Ctrl Pts',(-4.126056836133,22.2182956401341,0.));
#244467=CARTESIAN_POINT('Ctrl Pts',(-4.126056836133,22.2182956401341,12.));
#244468=CARTESIAN_POINT('Ctrl Pts',(-4.12472167516602,22.2129576146671,
0.));
#244469=CARTESIAN_POINT('Ctrl Pts',(-4.12472167516602,22.2129576146671,
12.));
#244470=CARTESIAN_POINT('Ctrl Pts',(-4.12348173702025,22.2079143941719,
0.));
#244471=CARTESIAN_POINT('Ctrl Pts',(-4.12348173702025,22.2079143941719,
12.));
#244472=CARTESIAN_POINT('Ctrl Pts',(-4.12233664408237,22.2031746532106,
0.));
#244473=CARTESIAN_POINT('Ctrl Pts',(-4.12233664408237,22.2031746532106,
12.));
#244474=CARTESIAN_POINT('Ctrl Pts',(-4.12128598183533,22.1987479618246,
0.));
#244475=CARTESIAN_POINT('Ctrl Pts',(-4.12128598183533,22.1987479618246,
12.));
#244476=CARTESIAN_POINT('Ctrl Pts',(-4.12032932637738,22.1946440958098,
0.));
#244477=CARTESIAN_POINT('Ctrl Pts',(-4.12032932637738,22.1946440958098,
12.));
#244478=CARTESIAN_POINT('Ctrl Pts',(-4.11946626228623,22.1908725908525,
0.));
#244479=CARTESIAN_POINT('Ctrl Pts',(-4.11946626228623,22.1908725908525,
12.));
#244480=CARTESIAN_POINT('Ctrl Pts',(-4.11869641271752,22.1874419861496,
0.));
#244481=CARTESIAN_POINT('Ctrl Pts',(-4.11869641271752,22.1874419861496,
12.));
#244482=CARTESIAN_POINT('Ctrl Pts',(-4.11801938107464,22.1843613164855,
0.));
#244483=CARTESIAN_POINT('Ctrl Pts',(-4.11801938107464,22.1843613164855,
12.));
#244484=CARTESIAN_POINT('Ctrl Pts',(-4.11743469691765,22.1816414985788,
0.));
#244485=CARTESIAN_POINT('Ctrl Pts',(-4.11743469691765,22.1816414985788,
12.));
#244486=CARTESIAN_POINT('Ctrl Pts',(-4.11694173195041,22.179297473024,0.));
#244487=CARTESIAN_POINT('Ctrl Pts',(-4.11694173195041,22.179297473024,12.));
#244488=CARTESIAN_POINT('Ctrl Pts',(-4.11653973150558,22.177347426894,0.));
#244489=CARTESIAN_POINT('Ctrl Pts',(-4.11653973150558,22.177347426894,12.));
#244490=CARTESIAN_POINT('Ctrl Pts',(-4.11622797217066,22.1758088296598,
0.));
#244491=CARTESIAN_POINT('Ctrl Pts',(-4.11622797217066,22.1758088296598,
12.));
#244492=CARTESIAN_POINT('Ctrl Pts',(-4.11600589882767,22.1746949858773,
0.));
#244493=CARTESIAN_POINT('Ctrl Pts',(-4.11600589882767,22.1746949858773,
12.));
#244494=CARTESIAN_POINT('Ctrl Pts',(-4.11589976826061,22.174148802123,0.));
#244495=CARTESIAN_POINT('Ctrl Pts',(-4.11589976826061,22.174148802123,12.));
#244496=CARTESIAN_POINT('Ctrl Pts',(-4.1158603587821,22.1739341411684,0.));
#244497=CARTESIAN_POINT('Ctrl Pts',(-4.1158603587821,22.1739341411684,12.));
#244498=CARTESIAN_POINT('Ctrl Pts',(-4.11585194677412,22.1738776823239,
0.));
#244499=CARTESIAN_POINT('Ctrl Pts',(-4.11585194677412,22.1738776823239,
12.));
#244500=CARTESIAN_POINT('Ctrl Pts',(-4.11585220600461,22.1738711152697,
0.));
#244501=CARTESIAN_POINT('Ctrl Pts',(-4.11585220600461,22.1738711152697,
12.));
#244502=CARTESIAN_POINT('',(-6.08833931617698,25.2771067246846,0.));
#244503=CARTESIAN_POINT('Ctrl Pts',(-6.08833931617698,25.2771067246846,
0.));
#244504=CARTESIAN_POINT('Ctrl Pts',(-6.08441489609824,25.2729539149479,
0.));
#244505=CARTESIAN_POINT('Ctrl Pts',(-6.07657531787578,25.2646490489816,
0.));
#244506=CARTESIAN_POINT('Ctrl Pts',(-6.06484373634697,25.2521940105523,
0.));
#244507=CARTESIAN_POINT('Ctrl Pts',(-6.04925720151412,25.2355918138798,
0.));
#244508=CARTESIAN_POINT('Ctrl Pts',(-6.02986667390187,25.2148466201368,
0.));
#244509=CARTESIAN_POINT('Ctrl Pts',(-6.0105688180476,25.1941090269638,0.));
#244510=CARTESIAN_POINT('Ctrl Pts',(-5.99136367859838,25.1733791296154,
0.));
#244511=CARTESIAN_POINT('Ctrl Pts',(-5.97225131495636,25.1526570863065,
0.));
#244512=CARTESIAN_POINT('Ctrl Pts',(-5.95323180187348,25.1319431317273,
0.));
#244513=CARTESIAN_POINT('Ctrl Pts',(-5.93430523086776,25.1112375971182,
0.));
#244514=CARTESIAN_POINT('Ctrl Pts',(-5.91547170844382,25.0905409050863,
0.));
#244515=CARTESIAN_POINT('Ctrl Pts',(-5.89673135155459,25.0698535426593,
0.));
#244516=CARTESIAN_POINT('Ctrl Pts',(-5.87808428385329,25.0491760405965,
0.));
#244517=CARTESIAN_POINT('Ctrl Pts',(-5.8595306315681,25.0285089498922,0.));
#244518=CARTESIAN_POINT('Ctrl Pts',(-5.84107051963073,25.0078528200558,
0.));
#244519=CARTESIAN_POINT('Ctrl Pts',(-5.82270406744214,24.9872081752709,
0.));
#244520=CARTESIAN_POINT('Ctrl Pts',(-5.80443138549747,24.9665754954462,
0.));
#244521=CARTESIAN_POINT('Ctrl Pts',(-5.78625257775703,24.9459552293308,
0.));
#244522=CARTESIAN_POINT('Ctrl Pts',(-5.76816774342236,24.9253478043632,
0.));
#244523=CARTESIAN_POINT('Ctrl Pts',(-5.75017697890813,24.9047536376467,
0.));
#244524=CARTESIAN_POINT('Ctrl Pts',(-5.73228037976927,24.8841731467219,
0.));
#244525=CARTESIAN_POINT('Ctrl Pts',(-5.71447804252019,24.8636067597677,
0.));
#244526=CARTESIAN_POINT('Ctrl Pts',(-5.69677006679429,24.8430549277634,
0.));
#244527=CARTESIAN_POINT('Ctrl Pts',(-5.67915655496524,24.822518122386,0.));
#244528=CARTESIAN_POINT('Ctrl Pts',(-5.66163761114903,24.8019968304618,
0.));
#244529=CARTESIAN_POINT('Ctrl Pts',(-5.64421334042248,24.7814915496728,
0.));
#244530=CARTESIAN_POINT('Ctrl Pts',(-5.62688384790919,24.76100278357,0.));
#244531=CARTESIAN_POINT('Ctrl Pts',(-5.60964923798495,24.7405310372736,
0.));
#244532=CARTESIAN_POINT('Ctrl Pts',(-5.59250961323995,24.7200768119079,
0.));
#244533=CARTESIAN_POINT('Ctrl Pts',(-5.57546507427767,24.6996406035507,
0.));
#244534=CARTESIAN_POINT('Ctrl Pts',(-5.55851572025389,24.6792229061785,
0.));
#244535=CARTESIAN_POINT('Ctrl Pts',(-5.54166164919593,24.6588242134733,
0.));
#244536=CARTESIAN_POINT('Ctrl Pts',(-5.52490295840996,24.6384450211466,
0.));
#244537=CARTESIAN_POINT('Ctrl Pts',(-5.50823974481959,24.618085828918,0.));
#244538=CARTESIAN_POINT('Ctrl Pts',(-5.49167210537235,24.5977471429365,
0.));
#244539=CARTESIAN_POINT('Ctrl Pts',(-5.47520013724403,24.5774294770329,
0.));
#244540=CARTESIAN_POINT('Ctrl Pts',(-5.45882393762244,24.5571333514841,
0.));
#244541=CARTESIAN_POINT('Ctrl Pts',(-5.44254360356865,24.5368592922861,
0.));
#244542=CARTESIAN_POINT('Ctrl Pts',(-5.42635923183411,24.5166078302107,
0.));
#244543=CARTESIAN_POINT('Ctrl Pts',(-5.41027091869242,24.4963794999831,
0.));
#244544=CARTESIAN_POINT('Ctrl Pts',(-5.3942787597383,24.4761748393322,0.));
#244545=CARTESIAN_POINT('Ctrl Pts',(-5.37838284973706,24.4559943883159,
0.));
#244546=CARTESIAN_POINT('Ctrl Pts',(-5.36258328273639,24.4358386899152,
0.));
#244547=CARTESIAN_POINT('Ctrl Pts',(-5.34688015213546,24.4157082904615,
0.));
#244548=CARTESIAN_POINT('Ctrl Pts',(-5.33127355076037,24.3956037401293,
0.));
#244549=CARTESIAN_POINT('Ctrl Pts',(-5.31576357092524,24.3755255933917,
0.));
#244550=CARTESIAN_POINT('Ctrl Pts',(-5.30035030449059,24.3554744095075,
0.));
#244551=CARTESIAN_POINT('Ctrl Pts',(-5.28503384290644,24.3354507529415,
0.));
#244552=CARTESIAN_POINT('Ctrl Pts',(-5.26981427718796,24.3154551932222,
0.));
#244553=CARTESIAN_POINT('Ctrl Pts',(-5.25469169788856,24.2954883048448,
0.));
#244554=CARTESIAN_POINT('Ctrl Pts',(-5.23966619506289,24.2755506671526,
0.));
#244555=CARTESIAN_POINT('Ctrl Pts',(-5.22473785822441,24.2556428642294,
0.));
#244556=CARTESIAN_POINT('Ctrl Pts',(-5.20990677629173,24.2357654847765,
0.));
#244557=CARTESIAN_POINT('Ctrl Pts',(-5.19517303753643,24.215919122017,0.));
#244558=CARTESIAN_POINT('Ctrl Pts',(-5.18053672961392,24.1961043738754,
0.));
#244559=CARTESIAN_POINT('Ctrl Pts',(-5.16599793957979,24.1763218431343,
0.));
#244560=CARTESIAN_POINT('Ctrl Pts',(-5.15155675390075,24.156572137597,0.));
#244561=CARTESIAN_POINT('Ctrl Pts',(-5.13721325845745,24.1368558702443,
0.));
#244562=CARTESIAN_POINT('Ctrl Pts',(-5.12296753853859,24.117173659394,0.));
#244563=CARTESIAN_POINT('Ctrl Pts',(-5.10881967883132,24.0975261288446,
0.));
#244564=CARTESIAN_POINT('Ctrl Pts',(-5.09476976342625,24.0779139079266,
0.));
#244565=CARTESIAN_POINT('Ctrl Pts',(-5.08081787581276,24.0583376315638,
0.));
#244566=CARTESIAN_POINT('Ctrl Pts',(-5.06696409886641,24.0387979403268,
0.));
#244567=CARTESIAN_POINT('Ctrl Pts',(-5.05320851483065,24.0192954804896,
0.));
#244568=CARTESIAN_POINT('Ctrl Pts',(-5.03955120528521,23.9998309040746,
0.));
#244569=CARTESIAN_POINT('Ctrl Pts',(-5.02599225112454,23.9804048689227,
0.));
#244570=CARTESIAN_POINT('Ctrl Pts',(-5.01253173257453,23.9610180388271,
0.));
#244571=CARTESIAN_POINT('Ctrl Pts',(-4.99916972919307,23.9416710836529,
0.));
#244572=CARTESIAN_POINT('Ctrl Pts',(-4.98590631986533,23.9223646794592,
0.));
#244573=CARTESIAN_POINT('Ctrl Pts',(-4.97274158279227,23.9030995086163,
0.));
#244574=CARTESIAN_POINT('Ctrl Pts',(-4.95967559546561,23.8838762599218,
0.));
#244575=CARTESIAN_POINT('Ctrl Pts',(-4.9467084346586,23.8646956287168,0.));
#244576=CARTESIAN_POINT('Ctrl Pts',(-4.93384017643432,23.8455583170057,
0.));
#244577=CARTESIAN_POINT('Ctrl Pts',(-4.92107089613969,23.8264650335717,
0.));
#244578=CARTESIAN_POINT('Ctrl Pts',(-4.90840066839344,23.8074164940896,
0.));
#244579=CARTESIAN_POINT('Ctrl Pts',(-4.89582956706775,23.7884134212384,
0.));
#244580=CARTESIAN_POINT('Ctrl Pts',(-4.88335766525573,23.7694565448049,
0.));
#244581=CARTESIAN_POINT('Ctrl Pts',(-4.87098503527152,23.7505466018245,
0.));
#244582=CARTESIAN_POINT('Ctrl Pts',(-4.85871174865499,23.7316843367313,
0.));
#244583=CARTESIAN_POINT('Ctrl Pts',(-4.84653787616425,23.7128705015017,
0.));
#244584=CARTESIAN_POINT('Ctrl Pts',(-4.83446348776266,23.6941058557971,
0.));
#244585=CARTESIAN_POINT('Ctrl Pts',(-4.82248865259562,23.675391167102,0.));
#244586=CARTESIAN_POINT('Ctrl Pts',(-4.81061343896432,23.6567272108628,
0.));
#244587=CARTESIAN_POINT('Ctrl Pts',(-4.7988379143322,23.6381147706579,0.));
#244588=CARTESIAN_POINT('Ctrl Pts',(-4.78716214532098,23.6195546383624,
0.));
#244589=CARTESIAN_POINT('Ctrl Pts',(-4.77558619769872,23.6010476143099,
0.));
#244590=CARTESIAN_POINT('Ctrl Pts',(-4.76411013636251,23.5825945074535,
0.));
#244591=CARTESIAN_POINT('Ctrl Pts',(-4.75273402530617,23.5641961355168,
0.));
#244592=CARTESIAN_POINT('Ctrl Pts',(-4.74145792760698,23.545853325171,0.));
#244593=CARTESIAN_POINT('Ctrl Pts',(-4.7302819054303,23.5275669122372,0.));
#244594=CARTESIAN_POINT('Ctrl Pts',(-4.71920602001902,23.509337741878,0.));
#244595=CARTESIAN_POINT('Ctrl Pts',(-4.70823033167819,23.491166668789,0.));
#244596=CARTESIAN_POINT('Ctrl Pts',(-4.69735489975024,23.4730545573853,
0.));
#244597=CARTESIAN_POINT('Ctrl Pts',(-4.68657978258303,23.455002281986,0.));
#244598=CARTESIAN_POINT('Ctrl Pts',(-4.67590503753058,23.4370107270451,
0.));
#244599=CARTESIAN_POINT('Ctrl Pts',(-4.6653307209467,23.4190807873803,0.));
#244600=CARTESIAN_POINT('Ctrl Pts',(-4.65485688816924,23.4012133683959,
0.));
#244601=CARTESIAN_POINT('Ctrl Pts',(-4.6444835934993,23.3834093863068,0.));
#244602=CARTESIAN_POINT('Ctrl Pts',(-4.63421089016541,23.3656697683489,
0.));
#244603=CARTESIAN_POINT('Ctrl Pts',(-4.62403883030805,23.3479954530272,
0.));
#244604=CARTESIAN_POINT('Ctrl Pts',(-4.6139674649783,23.3303873903938,0.));
#244605=CARTESIAN_POINT('Ctrl Pts',(-4.60399684412163,23.3128465423115,
0.));
#244606=CARTESIAN_POINT('Ctrl Pts',(-4.5941270165575,23.2953738827191,0.));
#244607=CARTESIAN_POINT('Ctrl Pts',(-4.5843580299469,23.2779703978876,0.));
#244608=CARTESIAN_POINT('Ctrl Pts',(-4.57468993076097,23.2606370866866,
0.));
#244609=CARTESIAN_POINT('Ctrl Pts',(-4.56512276427839,23.2433749609131,
0.));
#244610=CARTESIAN_POINT('Ctrl Pts',(-4.55565657456975,23.2261850456064,
0.));
#244611=CARTESIAN_POINT('Ctrl Pts',(-4.54629140447544,23.2090683793629,
0.));
#244612=CARTESIAN_POINT('Ctrl Pts',(-4.53702729557566,23.1920260146465,
0.));
#244613=CARTESIAN_POINT('Ctrl Pts',(-4.52786428815015,23.1750590180908,
0.));
#244614=CARTESIAN_POINT('Ctrl Pts',(-4.51880242116748,23.1581684708761,
0.));
#244615=CARTESIAN_POINT('Ctrl Pts',(-4.5098417322706,23.1413554691123,0.));
#244616=CARTESIAN_POINT('Ctrl Pts',(-4.50098225775171,23.1246211242115,
0.));
#244617=CARTESIAN_POINT('Ctrl Pts',(-4.49222403252216,23.1079665632636,
0.));
#244618=CARTESIAN_POINT('Ctrl Pts',(-4.48356709006788,23.0913929293922,
0.));
#244619=CARTESIAN_POINT('Ctrl Pts',(-4.47501146242856,23.0749013821881,
0.));
#244620=CARTESIAN_POINT('Ctrl Pts',(-4.4665571801823,23.0584930981732,0.));
#244621=CARTESIAN_POINT('Ctrl Pts',(-4.45820427241683,23.0421692712467,
0.));
#244622=CARTESIAN_POINT('Ctrl Pts',(-4.44995276669686,23.0259311131392,
0.));
#244623=CARTESIAN_POINT('Ctrl Pts',(-4.44180268901643,23.0097798538395,
0.));
#244624=CARTESIAN_POINT('Ctrl Pts',(-4.43375406376879,22.9937167421006,
0.));
#244625=CARTESIAN_POINT('Ctrl Pts',(-4.42580691372751,22.977743046002,0.));
#244626=CARTESIAN_POINT('Ctrl Pts',(-4.41796126001302,22.9618600534866,
0.));
#244627=CARTESIAN_POINT('Ctrl Pts',(-4.41021712205553,22.9460690729093,
0.));
#244628=CARTESIAN_POINT('Ctrl Pts',(-4.40257451754323,22.930371433555,0.));
#244629=CARTESIAN_POINT('Ctrl Pts',(-4.39503346238473,22.9147684862426,
0.));
#244630=CARTESIAN_POINT('Ctrl Pts',(-4.38759397068406,22.8992616040108,
0.));
#244631=CARTESIAN_POINT('Ctrl Pts',(-4.38025605470093,22.8838521827701,
0.));
#244632=CARTESIAN_POINT('Ctrl Pts',(-4.37301972480746,22.8685416419725,
0.));
#244633=CARTESIAN_POINT('Ctrl Pts',(-4.36588498942997,22.8533314252422,
0.));
#244634=CARTESIAN_POINT('Ctrl Pts',(-4.35885185500546,22.8382230011184,
0.));
#244635=CARTESIAN_POINT('Ctrl Pts',(-4.35192032594791,22.8232178638876,
0.));
#244636=CARTESIAN_POINT('Ctrl Pts',(-4.34509040460062,22.8083175343791,
0.));
#244637=CARTESIAN_POINT('Ctrl Pts',(-4.33836209118446,22.7935235607806,
0.));
#244638=CARTESIAN_POINT('Ctrl Pts',(-4.3317353837319,22.7788375194076,0.));
#244639=CARTESIAN_POINT('Ctrl Pts',(-4.32521027803754,22.7642610156475,
0.));
#244640=CARTESIAN_POINT('Ctrl Pts',(-4.31878676761235,22.7497956849848,
0.));
#244641=CARTESIAN_POINT('Ctrl Pts',(-4.31246484362549,22.7354431939926,
0.));
#244642=CARTESIAN_POINT('Ctrl Pts',(-4.30624449484069,22.7212052413386,
0.));
#244643=CARTESIAN_POINT('Ctrl Pts',(-4.3001257075406,22.7070835587564,0.));
#244644=CARTESIAN_POINT('Ctrl Pts',(-4.29410846547056,22.6930799122548,
0.));
#244645=CARTESIAN_POINT('Ctrl Pts',(-4.28819274977763,22.6791961033538,
0.));
#244646=CARTESIAN_POINT('Ctrl Pts',(-4.28237853894059,22.6654339703109,
0.));
#244647=CARTESIAN_POINT('Ctrl Pts',(-4.2766658086912,22.6517953893303,0.));
#244648=CARTESIAN_POINT('Ctrl Pts',(-4.27105453193004,22.6382822758172,
0.));
#244649=CARTESIAN_POINT('Ctrl Pts',(-4.26554467865576,22.6248965859977,
0.));
#244650=CARTESIAN_POINT('Ctrl Pts',(-4.26013621588305,22.6116403184821,
0.));
#244651=CARTESIAN_POINT('Ctrl Pts',(-4.25482910755481,22.5985155158636,
0.));
#244652=CARTESIAN_POINT('Ctrl Pts',(-4.24962331444177,22.5855242662477,
0.));
#244653=CARTESIAN_POINT('Ctrl Pts',(-4.24451879404851,22.572668704992,0.));
#244654=CARTESIAN_POINT('Ctrl Pts',(-4.23951550052523,22.5599510166429,
0.));
#244655=CARTESIAN_POINT('Ctrl Pts',(-4.23461338456712,22.5473734368086,
0.));
#244656=CARTESIAN_POINT('Ctrl Pts',(-4.22981239330733,22.5349382540588,
0.));
#244657=CARTESIAN_POINT('Ctrl Pts',(-4.22511247020041,22.5226478117886,
0.));
#244658=CARTESIAN_POINT('Ctrl Pts',(-4.22051355490196,22.5105045108881,
0.));
#244659=CARTESIAN_POINT('Ctrl Pts',(-4.21601558313906,22.4985108124228,
0.));
#244660=CARTESIAN_POINT('Ctrl Pts',(-4.21161848657428,22.4866692403147,
0.));
#244661=CARTESIAN_POINT('Ctrl Pts',(-4.20732219265649,22.4749823839917,
0.));
#244662=CARTESIAN_POINT('Ctrl Pts',(-4.20312662448174,22.4634529011437,
0.));
#244663=CARTESIAN_POINT('Ctrl Pts',(-4.19903170066358,22.4520835205422,
0.));
#244664=CARTESIAN_POINT('Ctrl Pts',(-4.1950373351886,22.4408770448917,0.));
#244665=CARTESIAN_POINT('Ctrl Pts',(-4.19114343726932,22.4298363535416,
0.));
#244666=CARTESIAN_POINT('Ctrl Pts',(-4.18734991117707,22.4189644056109,
0.));
#244667=CARTESIAN_POINT('Ctrl Pts',(-4.18365665600839,22.4082642454448,
0.));
#244668=CARTESIAN_POINT('Ctrl Pts',(-4.18006356544879,22.3977390078074,
0.));
#244669=CARTESIAN_POINT('Ctrl Pts',(-4.17657052752834,22.3873919231339,
0.));
#244670=CARTESIAN_POINT('Ctrl Pts',(-4.17317742436162,22.3772263228624,
0.));
#244671=CARTESIAN_POINT('Ctrl Pts',(-4.1698841319947,22.3672456427605,0.));
#244672=CARTESIAN_POINT('Ctrl Pts',(-4.16669052026602,22.3574534257397,
0.));
#244673=CARTESIAN_POINT('Ctrl Pts',(-4.1635964526318,22.3478533253886,0.));
#244674=CARTESIAN_POINT('Ctrl Pts',(-4.16060178604154,22.3384491078599,
0.));
#244675=CARTESIAN_POINT('Ctrl Pts',(-4.15770637047882,22.3292446628957,
0.));
#244676=CARTESIAN_POINT('Ctrl Pts',(-4.15491004835278,22.3202440186979,
0.));
#244677=CARTESIAN_POINT('Ctrl Pts',(-4.15221265396992,22.3114513545186,
0.));
#244678=CARTESIAN_POINT('Ctrl Pts',(-4.14961401285526,22.3028710166935,
0.));
#244679=CARTESIAN_POINT('Ctrl Pts',(-4.14711394168559,22.2945075198468,
0.));
#244680=CARTESIAN_POINT('Ctrl Pts',(-4.14471224859295,22.2863655389166,
0.));
#244681=CARTESIAN_POINT('Ctrl Pts',(-4.14240873321982,22.2784499072026,
0.));
#244682=CARTESIAN_POINT('Ctrl Pts',(-4.14020318715988,22.2707656042456,
0.));
#244683=CARTESIAN_POINT('Ctrl Pts',(-4.13809539255419,22.263317791397,0.));
#244684=CARTESIAN_POINT('Ctrl Pts',(-4.13608511977226,22.2561118708422,
0.));
#244685=CARTESIAN_POINT('Ctrl Pts',(-4.13417212558808,22.2491535317789,
0.));
#244686=CARTESIAN_POINT('Ctrl Pts',(-4.1323561506016,22.2424488153523,0.));
#244687=CARTESIAN_POINT('Ctrl Pts',(-4.13063692157499,22.2360040565534,
0.));
#244688=CARTESIAN_POINT('Ctrl Pts',(-4.12901415463379,22.2298258043947,
0.));
#244689=CARTESIAN_POINT('Ctrl Pts',(-4.12748755830099,22.2239207458781,
0.));
#244690=CARTESIAN_POINT('Ctrl Pts',(-4.126056836133,22.2182956401341,0.));
#244691=CARTESIAN_POINT('Ctrl Pts',(-4.12472167516602,22.2129576146671,
0.));
#244692=CARTESIAN_POINT('Ctrl Pts',(-4.12348173702025,22.2079143941719,
0.));
#244693=CARTESIAN_POINT('Ctrl Pts',(-4.12233664408237,22.2031746532106,
0.));
#244694=CARTESIAN_POINT('Ctrl Pts',(-4.12128598183533,22.1987479618246,
0.));
#244695=CARTESIAN_POINT('Ctrl Pts',(-4.12032932637738,22.1946440958098,
0.));
#244696=CARTESIAN_POINT('Ctrl Pts',(-4.11946626228623,22.1908725908525,
0.));
#244697=CARTESIAN_POINT('Ctrl Pts',(-4.11869641271752,22.1874419861496,
0.));
#244698=CARTESIAN_POINT('Ctrl Pts',(-4.11801938107464,22.1843613164855,
0.));
#244699=CARTESIAN_POINT('Ctrl Pts',(-4.11743469691765,22.1816414985788,
0.));
#244700=CARTESIAN_POINT('Ctrl Pts',(-4.11694173195041,22.179297473024,0.));
#244701=CARTESIAN_POINT('Ctrl Pts',(-4.11653973150558,22.177347426894,0.));
#244702=CARTESIAN_POINT('Ctrl Pts',(-4.11622797217066,22.1758088296598,
0.));
#244703=CARTESIAN_POINT('Ctrl Pts',(-4.11600589882767,22.1746949858773,
0.));
#244704=CARTESIAN_POINT('Ctrl Pts',(-4.11589976826061,22.174148802123,0.));
#244705=CARTESIAN_POINT('Ctrl Pts',(-4.1158603587821,22.1739341411684,0.));
#244706=CARTESIAN_POINT('Ctrl Pts',(-4.11585194677412,22.1738776823239,
0.));
#244707=CARTESIAN_POINT('Ctrl Pts',(-4.11585220600461,22.1738711152697,
0.));
#244708=CARTESIAN_POINT('',(-6.08833931617698,25.2771067246846,12.));
#244709=CARTESIAN_POINT('',(-6.08833931617698,25.2771067246846,0.));
#244710=CARTESIAN_POINT('Ctrl Pts',(-4.11585220600461,22.1738711152697,
12.));
#244711=CARTESIAN_POINT('Ctrl Pts',(-4.11585194677412,22.1738776823239,
12.));
#244712=CARTESIAN_POINT('Ctrl Pts',(-4.1158603587821,22.1739341411684,12.));
#244713=CARTESIAN_POINT('Ctrl Pts',(-4.11589976826061,22.174148802123,12.));
#244714=CARTESIAN_POINT('Ctrl Pts',(-4.11600589882767,22.1746949858773,
12.));
#244715=CARTESIAN_POINT('Ctrl Pts',(-4.11622797217066,22.1758088296598,
12.));
#244716=CARTESIAN_POINT('Ctrl Pts',(-4.11653973150558,22.177347426894,12.));
#244717=CARTESIAN_POINT('Ctrl Pts',(-4.11694173195041,22.179297473024,12.));
#244718=CARTESIAN_POINT('Ctrl Pts',(-4.11743469691765,22.1816414985788,
12.));
#244719=CARTESIAN_POINT('Ctrl Pts',(-4.11801938107464,22.1843613164855,
12.));
#244720=CARTESIAN_POINT('Ctrl Pts',(-4.11869641271752,22.1874419861496,
12.));
#244721=CARTESIAN_POINT('Ctrl Pts',(-4.11946626228623,22.1908725908525,
12.));
#244722=CARTESIAN_POINT('Ctrl Pts',(-4.12032932637738,22.1946440958098,
12.));
#244723=CARTESIAN_POINT('Ctrl Pts',(-4.12128598183533,22.1987479618246,
12.));
#244724=CARTESIAN_POINT('Ctrl Pts',(-4.12233664408237,22.2031746532106,
12.));
#244725=CARTESIAN_POINT('Ctrl Pts',(-4.12348173702025,22.2079143941719,
12.));
#244726=CARTESIAN_POINT('Ctrl Pts',(-4.12472167516602,22.2129576146671,
12.));
#244727=CARTESIAN_POINT('Ctrl Pts',(-4.126056836133,22.2182956401341,12.));
#244728=CARTESIAN_POINT('Ctrl Pts',(-4.12748755830099,22.2239207458781,
12.));
#244729=CARTESIAN_POINT('Ctrl Pts',(-4.12901415463379,22.2298258043947,
12.));
#244730=CARTESIAN_POINT('Ctrl Pts',(-4.13063692157499,22.2360040565534,
12.));
#244731=CARTESIAN_POINT('Ctrl Pts',(-4.1323561506016,22.2424488153523,12.));
#244732=CARTESIAN_POINT('Ctrl Pts',(-4.13417212558808,22.2491535317789,
12.));
#244733=CARTESIAN_POINT('Ctrl Pts',(-4.13608511977226,22.2561118708422,
12.));
#244734=CARTESIAN_POINT('Ctrl Pts',(-4.13809539255419,22.263317791397,12.));
#244735=CARTESIAN_POINT('Ctrl Pts',(-4.14020318715988,22.2707656042456,
12.));
#244736=CARTESIAN_POINT('Ctrl Pts',(-4.14240873321982,22.2784499072026,
12.));
#244737=CARTESIAN_POINT('Ctrl Pts',(-4.14471224859295,22.2863655389166,
12.));
#244738=CARTESIAN_POINT('Ctrl Pts',(-4.14711394168559,22.2945075198468,
12.));
#244739=CARTESIAN_POINT('Ctrl Pts',(-4.14961401285526,22.3028710166935,
12.));
#244740=CARTESIAN_POINT('Ctrl Pts',(-4.15221265396992,22.3114513545186,
12.));
#244741=CARTESIAN_POINT('Ctrl Pts',(-4.15491004835278,22.3202440186979,
12.));
#244742=CARTESIAN_POINT('Ctrl Pts',(-4.15770637047882,22.3292446628957,
12.));
#244743=CARTESIAN_POINT('Ctrl Pts',(-4.16060178604154,22.3384491078599,
12.));
#244744=CARTESIAN_POINT('Ctrl Pts',(-4.1635964526318,22.3478533253886,12.));
#244745=CARTESIAN_POINT('Ctrl Pts',(-4.16669052026602,22.3574534257397,
12.));
#244746=CARTESIAN_POINT('Ctrl Pts',(-4.1698841319947,22.3672456427605,12.));
#244747=CARTESIAN_POINT('Ctrl Pts',(-4.17317742436162,22.3772263228624,
12.));
#244748=CARTESIAN_POINT('Ctrl Pts',(-4.17657052752834,22.3873919231339,
12.));
#244749=CARTESIAN_POINT('Ctrl Pts',(-4.18006356544879,22.3977390078074,
12.));
#244750=CARTESIAN_POINT('Ctrl Pts',(-4.18365665600839,22.4082642454448,
12.));
#244751=CARTESIAN_POINT('Ctrl Pts',(-4.18734991117707,22.4189644056109,
12.));
#244752=CARTESIAN_POINT('Ctrl Pts',(-4.19114343726932,22.4298363535416,
12.));
#244753=CARTESIAN_POINT('Ctrl Pts',(-4.1950373351886,22.4408770448917,12.));
#244754=CARTESIAN_POINT('Ctrl Pts',(-4.19903170066358,22.4520835205422,
12.));
#244755=CARTESIAN_POINT('Ctrl Pts',(-4.20312662448174,22.4634529011437,
12.));
#244756=CARTESIAN_POINT('Ctrl Pts',(-4.20732219265649,22.4749823839917,
12.));
#244757=CARTESIAN_POINT('Ctrl Pts',(-4.21161848657428,22.4866692403147,
12.));
#244758=CARTESIAN_POINT('Ctrl Pts',(-4.21601558313906,22.4985108124228,
12.));
#244759=CARTESIAN_POINT('Ctrl Pts',(-4.22051355490196,22.5105045108881,
12.));
#244760=CARTESIAN_POINT('Ctrl Pts',(-4.22511247020041,22.5226478117886,
12.));
#244761=CARTESIAN_POINT('Ctrl Pts',(-4.22981239330733,22.5349382540588,
12.));
#244762=CARTESIAN_POINT('Ctrl Pts',(-4.23461338456712,22.5473734368086,
12.));
#244763=CARTESIAN_POINT('Ctrl Pts',(-4.23951550052523,22.5599510166429,
12.));
#244764=CARTESIAN_POINT('Ctrl Pts',(-4.24451879404851,22.572668704992,12.));
#244765=CARTESIAN_POINT('Ctrl Pts',(-4.24962331444177,22.5855242662477,
12.));
#244766=CARTESIAN_POINT('Ctrl Pts',(-4.25482910755481,22.5985155158636,
12.));
#244767=CARTESIAN_POINT('Ctrl Pts',(-4.26013621588305,22.6116403184821,
12.));
#244768=CARTESIAN_POINT('Ctrl Pts',(-4.26554467865576,22.6248965859977,
12.));
#244769=CARTESIAN_POINT('Ctrl Pts',(-4.27105453193004,22.6382822758172,
12.));
#244770=CARTESIAN_POINT('Ctrl Pts',(-4.2766658086912,22.6517953893303,12.));
#244771=CARTESIAN_POINT('Ctrl Pts',(-4.28237853894059,22.6654339703109,
12.));
#244772=CARTESIAN_POINT('Ctrl Pts',(-4.28819274977763,22.6791961033538,
12.));
#244773=CARTESIAN_POINT('Ctrl Pts',(-4.29410846547056,22.6930799122548,
12.));
#244774=CARTESIAN_POINT('Ctrl Pts',(-4.3001257075406,22.7070835587564,12.));
#244775=CARTESIAN_POINT('Ctrl Pts',(-4.30624449484069,22.7212052413386,
12.));
#244776=CARTESIAN_POINT('Ctrl Pts',(-4.31246484362549,22.7354431939926,
12.));
#244777=CARTESIAN_POINT('Ctrl Pts',(-4.31878676761235,22.7497956849848,
12.));
#244778=CARTESIAN_POINT('Ctrl Pts',(-4.32521027803754,22.7642610156475,
12.));
#244779=CARTESIAN_POINT('Ctrl Pts',(-4.3317353837319,22.7788375194076,12.));
#244780=CARTESIAN_POINT('Ctrl Pts',(-4.33836209118446,22.7935235607806,
12.));
#244781=CARTESIAN_POINT('Ctrl Pts',(-4.34509040460062,22.8083175343791,
12.));
#244782=CARTESIAN_POINT('Ctrl Pts',(-4.35192032594791,22.8232178638876,
12.));
#244783=CARTESIAN_POINT('Ctrl Pts',(-4.35885185500546,22.8382230011184,
12.));
#244784=CARTESIAN_POINT('Ctrl Pts',(-4.36588498942997,22.8533314252422,
12.));
#244785=CARTESIAN_POINT('Ctrl Pts',(-4.37301972480746,22.8685416419725,
12.));
#244786=CARTESIAN_POINT('Ctrl Pts',(-4.38025605470093,22.8838521827701,
12.));
#244787=CARTESIAN_POINT('Ctrl Pts',(-4.38759397068406,22.8992616040108,
12.));
#244788=CARTESIAN_POINT('Ctrl Pts',(-4.39503346238473,22.9147684862426,
12.));
#244789=CARTESIAN_POINT('Ctrl Pts',(-4.40257451754323,22.930371433555,12.));
#244790=CARTESIAN_POINT('Ctrl Pts',(-4.41021712205553,22.9460690729093,
12.));
#244791=CARTESIAN_POINT('Ctrl Pts',(-4.41796126001302,22.9618600534866,
12.));
#244792=CARTESIAN_POINT('Ctrl Pts',(-4.42580691372751,22.977743046002,12.));
#244793=CARTESIAN_POINT('Ctrl Pts',(-4.43375406376879,22.9937167421006,
12.));
#244794=CARTESIAN_POINT('Ctrl Pts',(-4.44180268901643,23.0097798538395,
12.));
#244795=CARTESIAN_POINT('Ctrl Pts',(-4.44995276669686,23.0259311131392,
12.));
#244796=CARTESIAN_POINT('Ctrl Pts',(-4.45820427241683,23.0421692712467,
12.));
#244797=CARTESIAN_POINT('Ctrl Pts',(-4.4665571801823,23.0584930981732,12.));
#244798=CARTESIAN_POINT('Ctrl Pts',(-4.47501146242856,23.0749013821881,
12.));
#244799=CARTESIAN_POINT('Ctrl Pts',(-4.48356709006788,23.0913929293922,
12.));
#244800=CARTESIAN_POINT('Ctrl Pts',(-4.49222403252216,23.1079665632636,
12.));
#244801=CARTESIAN_POINT('Ctrl Pts',(-4.50098225775171,23.1246211242115,
12.));
#244802=CARTESIAN_POINT('Ctrl Pts',(-4.5098417322706,23.1413554691123,12.));
#244803=CARTESIAN_POINT('Ctrl Pts',(-4.51880242116748,23.1581684708761,
12.));
#244804=CARTESIAN_POINT('Ctrl Pts',(-4.52786428815015,23.1750590180908,
12.));
#244805=CARTESIAN_POINT('Ctrl Pts',(-4.53702729557566,23.1920260146465,
12.));
#244806=CARTESIAN_POINT('Ctrl Pts',(-4.54629140447544,23.2090683793629,
12.));
#244807=CARTESIAN_POINT('Ctrl Pts',(-4.55565657456975,23.2261850456064,
12.));
#244808=CARTESIAN_POINT('Ctrl Pts',(-4.56512276427839,23.2433749609131,
12.));
#244809=CARTESIAN_POINT('Ctrl Pts',(-4.57468993076097,23.2606370866866,
12.));
#244810=CARTESIAN_POINT('Ctrl Pts',(-4.5843580299469,23.2779703978876,12.));
#244811=CARTESIAN_POINT('Ctrl Pts',(-4.5941270165575,23.2953738827191,12.));
#244812=CARTESIAN_POINT('Ctrl Pts',(-4.60399684412163,23.3128465423115,
12.));
#244813=CARTESIAN_POINT('Ctrl Pts',(-4.6139674649783,23.3303873903938,12.));
#244814=CARTESIAN_POINT('Ctrl Pts',(-4.62403883030805,23.3479954530272,
12.));
#244815=CARTESIAN_POINT('Ctrl Pts',(-4.63421089016541,23.3656697683489,
12.));
#244816=CARTESIAN_POINT('Ctrl Pts',(-4.6444835934993,23.3834093863068,12.));
#244817=CARTESIAN_POINT('Ctrl Pts',(-4.65485688816924,23.4012133683959,
12.));
#244818=CARTESIAN_POINT('Ctrl Pts',(-4.6653307209467,23.4190807873803,12.));
#244819=CARTESIAN_POINT('Ctrl Pts',(-4.67590503753058,23.4370107270451,
12.));
#244820=CARTESIAN_POINT('Ctrl Pts',(-4.68657978258303,23.455002281986,12.));
#244821=CARTESIAN_POINT('Ctrl Pts',(-4.69735489975024,23.4730545573853,
12.));
#244822=CARTESIAN_POINT('Ctrl Pts',(-4.70823033167819,23.491166668789,12.));
#244823=CARTESIAN_POINT('Ctrl Pts',(-4.71920602001902,23.509337741878,12.));
#244824=CARTESIAN_POINT('Ctrl Pts',(-4.7302819054303,23.5275669122372,12.));
#244825=CARTESIAN_POINT('Ctrl Pts',(-4.74145792760698,23.545853325171,12.));
#244826=CARTESIAN_POINT('Ctrl Pts',(-4.75273402530617,23.5641961355168,
12.));
#244827=CARTESIAN_POINT('Ctrl Pts',(-4.76411013636251,23.5825945074535,
12.));
#244828=CARTESIAN_POINT('Ctrl Pts',(-4.77558619769872,23.6010476143099,
12.));
#244829=CARTESIAN_POINT('Ctrl Pts',(-4.78716214532098,23.6195546383624,
12.));
#244830=CARTESIAN_POINT('Ctrl Pts',(-4.7988379143322,23.6381147706579,12.));
#244831=CARTESIAN_POINT('Ctrl Pts',(-4.81061343896432,23.6567272108628,
12.));
#244832=CARTESIAN_POINT('Ctrl Pts',(-4.82248865259562,23.675391167102,12.));
#244833=CARTESIAN_POINT('Ctrl Pts',(-4.83446348776266,23.6941058557971,
12.));
#244834=CARTESIAN_POINT('Ctrl Pts',(-4.84653787616425,23.7128705015017,
12.));
#244835=CARTESIAN_POINT('Ctrl Pts',(-4.85871174865499,23.7316843367313,
12.));
#244836=CARTESIAN_POINT('Ctrl Pts',(-4.87098503527152,23.7505466018245,
12.));
#244837=CARTESIAN_POINT('Ctrl Pts',(-4.88335766525573,23.7694565448049,
12.));
#244838=CARTESIAN_POINT('Ctrl Pts',(-4.89582956706775,23.7884134212384,
12.));
#244839=CARTESIAN_POINT('Ctrl Pts',(-4.90840066839344,23.8074164940896,
12.));
#244840=CARTESIAN_POINT('Ctrl Pts',(-4.92107089613969,23.8264650335717,
12.));
#244841=CARTESIAN_POINT('Ctrl Pts',(-4.93384017643432,23.8455583170057,
12.));
#244842=CARTESIAN_POINT('Ctrl Pts',(-4.9467084346586,23.8646956287168,12.));
#244843=CARTESIAN_POINT('Ctrl Pts',(-4.95967559546561,23.8838762599218,
12.));
#244844=CARTESIAN_POINT('Ctrl Pts',(-4.97274158279227,23.9030995086163,
12.));
#244845=CARTESIAN_POINT('Ctrl Pts',(-4.98590631986533,23.9223646794592,
12.));
#244846=CARTESIAN_POINT('Ctrl Pts',(-4.99916972919307,23.9416710836529,
12.));
#244847=CARTESIAN_POINT('Ctrl Pts',(-5.01253173257453,23.9610180388271,
12.));
#244848=CARTESIAN_POINT('Ctrl Pts',(-5.02599225112454,23.9804048689227,
12.));
#244849=CARTESIAN_POINT('Ctrl Pts',(-5.03955120528521,23.9998309040746,
12.));
#244850=CARTESIAN_POINT('Ctrl Pts',(-5.05320851483065,24.0192954804896,
12.));
#244851=CARTESIAN_POINT('Ctrl Pts',(-5.06696409886641,24.0387979403268,
12.));
#244852=CARTESIAN_POINT('Ctrl Pts',(-5.08081787581276,24.0583376315638,
12.));
#244853=CARTESIAN_POINT('Ctrl Pts',(-5.09476976342625,24.0779139079266,
12.));
#244854=CARTESIAN_POINT('Ctrl Pts',(-5.10881967883132,24.0975261288446,
12.));
#244855=CARTESIAN_POINT('Ctrl Pts',(-5.12296753853859,24.117173659394,12.));
#244856=CARTESIAN_POINT('Ctrl Pts',(-5.13721325845745,24.1368558702443,
12.));
#244857=CARTESIAN_POINT('Ctrl Pts',(-5.15155675390075,24.156572137597,12.));
#244858=CARTESIAN_POINT('Ctrl Pts',(-5.16599793957979,24.1763218431343,
12.));
#244859=CARTESIAN_POINT('Ctrl Pts',(-5.18053672961392,24.1961043738754,
12.));
#244860=CARTESIAN_POINT('Ctrl Pts',(-5.19517303753643,24.215919122017,12.));
#244861=CARTESIAN_POINT('Ctrl Pts',(-5.20990677629173,24.2357654847765,
12.));
#244862=CARTESIAN_POINT('Ctrl Pts',(-5.22473785822441,24.2556428642294,
12.));
#244863=CARTESIAN_POINT('Ctrl Pts',(-5.23966619506289,24.2755506671526,
12.));
#244864=CARTESIAN_POINT('Ctrl Pts',(-5.25469169788856,24.2954883048448,
12.));
#244865=CARTESIAN_POINT('Ctrl Pts',(-5.26981427718796,24.3154551932222,
12.));
#244866=CARTESIAN_POINT('Ctrl Pts',(-5.28503384290644,24.3354507529415,
12.));
#244867=CARTESIAN_POINT('Ctrl Pts',(-5.30035030449059,24.3554744095075,
12.));
#244868=CARTESIAN_POINT('Ctrl Pts',(-5.31576357092524,24.3755255933917,
12.));
#244869=CARTESIAN_POINT('Ctrl Pts',(-5.33127355076037,24.3956037401293,
12.));
#244870=CARTESIAN_POINT('Ctrl Pts',(-5.34688015213546,24.4157082904615,
12.));
#244871=CARTESIAN_POINT('Ctrl Pts',(-5.36258328273639,24.4358386899152,
12.));
#244872=CARTESIAN_POINT('Ctrl Pts',(-5.37838284973706,24.4559943883159,
12.));
#244873=CARTESIAN_POINT('Ctrl Pts',(-5.3942787597383,24.4761748393322,12.));
#244874=CARTESIAN_POINT('Ctrl Pts',(-5.41027091869242,24.4963794999831,
12.));
#244875=CARTESIAN_POINT('Ctrl Pts',(-5.42635923183411,24.5166078302107,
12.));
#244876=CARTESIAN_POINT('Ctrl Pts',(-5.44254360356865,24.5368592922861,
12.));
#244877=CARTESIAN_POINT('Ctrl Pts',(-5.45882393762244,24.5571333514841,
12.));
#244878=CARTESIAN_POINT('Ctrl Pts',(-5.47520013724403,24.5774294770329,
12.));
#244879=CARTESIAN_POINT('Ctrl Pts',(-5.49167210537235,24.5977471429365,
12.));
#244880=CARTESIAN_POINT('Ctrl Pts',(-5.50823974481959,24.618085828918,12.));
#244881=CARTESIAN_POINT('Ctrl Pts',(-5.52490295840996,24.6384450211466,
12.));
#244882=CARTESIAN_POINT('Ctrl Pts',(-5.54166164919593,24.6588242134733,
12.));
#244883=CARTESIAN_POINT('Ctrl Pts',(-5.55851572025389,24.6792229061785,
12.));
#244884=CARTESIAN_POINT('Ctrl Pts',(-5.57546507427767,24.6996406035507,
12.));
#244885=CARTESIAN_POINT('Ctrl Pts',(-5.59250961323995,24.7200768119079,
12.));
#244886=CARTESIAN_POINT('Ctrl Pts',(-5.60964923798495,24.7405310372736,
12.));
#244887=CARTESIAN_POINT('Ctrl Pts',(-5.62688384790919,24.76100278357,12.));
#244888=CARTESIAN_POINT('Ctrl Pts',(-5.64421334042248,24.7814915496728,
12.));
#244889=CARTESIAN_POINT('Ctrl Pts',(-5.66163761114903,24.8019968304618,
12.));
#244890=CARTESIAN_POINT('Ctrl Pts',(-5.67915655496524,24.822518122386,12.));
#244891=CARTESIAN_POINT('Ctrl Pts',(-5.69677006679429,24.8430549277634,
12.));
#244892=CARTESIAN_POINT('Ctrl Pts',(-5.71447804252019,24.8636067597677,
12.));
#244893=CARTESIAN_POINT('Ctrl Pts',(-5.73228037976927,24.8841731467219,
12.));
#244894=CARTESIAN_POINT('Ctrl Pts',(-5.75017697890813,24.9047536376467,
12.));
#244895=CARTESIAN_POINT('Ctrl Pts',(-5.76816774342236,24.9253478043632,
12.));
#244896=CARTESIAN_POINT('Ctrl Pts',(-5.78625257775703,24.9459552293308,
12.));
#244897=CARTESIAN_POINT('Ctrl Pts',(-5.80443138549747,24.9665754954462,
12.));
#244898=CARTESIAN_POINT('Ctrl Pts',(-5.82270406744214,24.9872081752709,
12.));
#244899=CARTESIAN_POINT('Ctrl Pts',(-5.84107051963073,25.0078528200558,
12.));
#244900=CARTESIAN_POINT('Ctrl Pts',(-5.8595306315681,25.0285089498922,12.));
#244901=CARTESIAN_POINT('Ctrl Pts',(-5.87808428385329,25.0491760405965,
12.));
#244902=CARTESIAN_POINT('Ctrl Pts',(-5.89673135155459,25.0698535426593,
12.));
#244903=CARTESIAN_POINT('Ctrl Pts',(-5.91547170844382,25.0905409050863,
12.));
#244904=CARTESIAN_POINT('Ctrl Pts',(-5.93430523086776,25.1112375971182,
12.));
#244905=CARTESIAN_POINT('Ctrl Pts',(-5.95323180187348,25.1319431317273,
12.));
#244906=CARTESIAN_POINT('Ctrl Pts',(-5.97225131495636,25.1526570863065,
12.));
#244907=CARTESIAN_POINT('Ctrl Pts',(-5.99136367859838,25.1733791296154,
12.));
#244908=CARTESIAN_POINT('Ctrl Pts',(-6.0105688180476,25.1941090269638,12.));
#244909=CARTESIAN_POINT('Ctrl Pts',(-6.02986667390187,25.2148466201368,
12.));
#244910=CARTESIAN_POINT('Ctrl Pts',(-6.04925720151412,25.2355918138798,
12.));
#244911=CARTESIAN_POINT('Ctrl Pts',(-6.06484373634697,25.2521940105523,
12.));
#244912=CARTESIAN_POINT('Ctrl Pts',(-6.07657531787578,25.2646490489816,
12.));
#244913=CARTESIAN_POINT('Ctrl Pts',(-6.08441489609824,25.2729539149479,
12.));
#244914=CARTESIAN_POINT('Ctrl Pts',(-6.08833931617698,25.2771067246846,
12.));
#244915=CARTESIAN_POINT('Ctrl Pts',(-1.76341220531179,22.4835757167854,
0.));
#244916=CARTESIAN_POINT('Ctrl Pts',(-1.76341220531179,22.4835757167854,
12.));
#244917=CARTESIAN_POINT('Ctrl Pts',(-1.76341415538764,22.483581992979,0.));
#244918=CARTESIAN_POINT('Ctrl Pts',(-1.76341415538764,22.483581992979,12.));
#244919=CARTESIAN_POINT('Ctrl Pts',(-1.7634206426357,22.4836387052232,0.));
#244920=CARTESIAN_POINT('Ctrl Pts',(-1.7634206426357,22.4836387052232,12.));
#244921=CARTESIAN_POINT('Ctrl Pts',(-1.76343813434565,22.483856251707,0.));
#244922=CARTESIAN_POINT('Ctrl Pts',(-1.76343813434565,22.483856251707,12.));
#244923=CARTESIAN_POINT('Ctrl Pts',(-1.76347698284792,22.4844112933129,
0.));
#244924=CARTESIAN_POINT('Ctrl Pts',(-1.76347698284792,22.4844112933129,
12.));
#244925=CARTESIAN_POINT('Ctrl Pts',(-1.76355076045546,22.4855446605991,
0.));
#244926=CARTESIAN_POINT('Ctrl Pts',(-1.76355076045546,22.4855446605991,
12.));
#244927=CARTESIAN_POINT('Ctrl Pts',(-1.76364784232963,22.4871115206571,
0.));
#244928=CARTESIAN_POINT('Ctrl Pts',(-1.76364784232963,22.4871115206571,
12.));
#244929=CARTESIAN_POINT('Ctrl Pts',(-1.76376424879505,22.4890991659478,
0.));
#244930=CARTESIAN_POINT('Ctrl Pts',(-1.76376424879505,22.4890991659478,
12.));
#244931=CARTESIAN_POINT('Ctrl Pts',(-1.76389475965724,22.4914909094908,
0.));
#244932=CARTESIAN_POINT('Ctrl Pts',(-1.76389475965724,22.4914909094908,
12.));
#244933=CARTESIAN_POINT('Ctrl Pts',(-1.76403393880301,22.4942693792449,
0.));
#244934=CARTESIAN_POINT('Ctrl Pts',(-1.76403393880301,22.4942693792449,
12.));
#244935=CARTESIAN_POINT('Ctrl Pts',(-1.76417731243462,22.4974203063191,
0.));
#244936=CARTESIAN_POINT('Ctrl Pts',(-1.76417731243462,22.4974203063191,
12.));
#244937=CARTESIAN_POINT('Ctrl Pts',(-1.76432160068725,22.5009332677316,
0.));
#244938=CARTESIAN_POINT('Ctrl Pts',(-1.76432160068725,22.5009332677316,
12.));
#244939=CARTESIAN_POINT('Ctrl Pts',(-1.76446408210366,22.5047996391978,
0.));
#244940=CARTESIAN_POINT('Ctrl Pts',(-1.76446408210366,22.5047996391978,
12.));
#244941=CARTESIAN_POINT('Ctrl Pts',(-1.76460218257323,22.5090112700212,
0.));
#244942=CARTESIAN_POINT('Ctrl Pts',(-1.76460218257323,22.5090112700212,
12.));
#244943=CARTESIAN_POINT('Ctrl Pts',(-1.76473303281159,22.5135590569554,
0.));
#244944=CARTESIAN_POINT('Ctrl Pts',(-1.76473303281159,22.5135590569554,
12.));
#244945=CARTESIAN_POINT('Ctrl Pts',(-1.76485369319896,22.5184336670207,
0.));
#244946=CARTESIAN_POINT('Ctrl Pts',(-1.76485369319896,22.5184336670207,
12.));
#244947=CARTESIAN_POINT('Ctrl Pts',(-1.76496128643369,22.5236259635515,
0.));
#244948=CARTESIAN_POINT('Ctrl Pts',(-1.76496128643369,22.5236259635515,
12.));
#244949=CARTESIAN_POINT('Ctrl Pts',(-1.76505320262752,22.529127665298,0.));
#244950=CARTESIAN_POINT('Ctrl Pts',(-1.76505320262752,22.529127665298,12.));
#244951=CARTESIAN_POINT('Ctrl Pts',(-1.7651271156325,22.5349313983571,0.));
#244952=CARTESIAN_POINT('Ctrl Pts',(-1.7651271156325,22.5349313983571,12.));
#244953=CARTESIAN_POINT('Ctrl Pts',(-1.76518087841493,22.5410303590891,
0.));
#244954=CARTESIAN_POINT('Ctrl Pts',(-1.76518087841493,22.5410303590891,
12.));
#244955=CARTESIAN_POINT('Ctrl Pts',(-1.76521245524047,22.5474180954006,
0.));
#244956=CARTESIAN_POINT('Ctrl Pts',(-1.76521245524047,22.5474180954006,
12.));
#244957=CARTESIAN_POINT('Ctrl Pts',(-1.76521983384063,22.5540882235837,
0.));
#244958=CARTESIAN_POINT('Ctrl Pts',(-1.76521983384063,22.5540882235837,
12.));
#244959=CARTESIAN_POINT('Ctrl Pts',(-1.76520104500449,22.5610344912501,
0.));
#244960=CARTESIAN_POINT('Ctrl Pts',(-1.76520104500449,22.5610344912501,
12.));
#244961=CARTESIAN_POINT('Ctrl Pts',(-1.76515418518829,22.5682508499873,
0.));
#244962=CARTESIAN_POINT('Ctrl Pts',(-1.76515418518829,22.5682508499873,
12.));
#244963=CARTESIAN_POINT('Ctrl Pts',(-1.76507744026747,22.5757315316355,
0.));
#244964=CARTESIAN_POINT('Ctrl Pts',(-1.76507744026747,22.5757315316355,
12.));
#244965=CARTESIAN_POINT('Ctrl Pts',(-1.76496910283088,22.5834711038024,
0.));
#244966=CARTESIAN_POINT('Ctrl Pts',(-1.76496910283088,22.5834711038024,
12.));
#244967=CARTESIAN_POINT('Ctrl Pts',(-1.76482755288411,22.5914644078106,
0.));
#244968=CARTESIAN_POINT('Ctrl Pts',(-1.76482755288411,22.5914644078106,
12.));
#244969=CARTESIAN_POINT('Ctrl Pts',(-1.76465124413556,22.5997065145638,
0.));
#244970=CARTESIAN_POINT('Ctrl Pts',(-1.76465124413556,22.5997065145638,
12.));
#244971=CARTESIAN_POINT('Ctrl Pts',(-1.76443868648015,22.6081926681342,
0.));
#244972=CARTESIAN_POINT('Ctrl Pts',(-1.76443868648015,22.6081926681342,
12.));
#244973=CARTESIAN_POINT('Ctrl Pts',(-1.76418843543739,22.6169182517693,
0.));
#244974=CARTESIAN_POINT('Ctrl Pts',(-1.76418843543739,22.6169182517693,
12.));
#244975=CARTESIAN_POINT('Ctrl Pts',(-1.76389909571402,22.6258787994847,
0.));
#244976=CARTESIAN_POINT('Ctrl Pts',(-1.76389909571402,22.6258787994847,
12.));
#244977=CARTESIAN_POINT('Ctrl Pts',(-1.76356932176272,22.635069997936,0.));
#244978=CARTESIAN_POINT('Ctrl Pts',(-1.76356932176272,22.635069997936,12.));
#244979=CARTESIAN_POINT('Ctrl Pts',(-1.76319782013914,22.6444876940425,
0.));
#244980=CARTESIAN_POINT('Ctrl Pts',(-1.76319782013914,22.6444876940425,
12.));
#244981=CARTESIAN_POINT('Ctrl Pts',(-1.76278334912559,22.6541278938413,
0.));
#244982=CARTESIAN_POINT('Ctrl Pts',(-1.76278334912559,22.6541278938413,
12.));
#244983=CARTESIAN_POINT('Ctrl Pts',(-1.76232471392567,22.6639867471756,
0.));
#244984=CARTESIAN_POINT('Ctrl Pts',(-1.76232471392567,22.6639867471756,
12.));
#244985=CARTESIAN_POINT('Ctrl Pts',(-1.76182076289525,22.6740605356699,
0.));
#244986=CARTESIAN_POINT('Ctrl Pts',(-1.76182076289525,22.6740605356699,
12.));
#244987=CARTESIAN_POINT('Ctrl Pts',(-1.76127038310613,22.6843456585245,
0.));
#244988=CARTESIAN_POINT('Ctrl Pts',(-1.76127038310613,22.6843456585245,
12.));
#244989=CARTESIAN_POINT('Ctrl Pts',(-1.76067249704884,22.6948386219843,
0.));
#244990=CARTESIAN_POINT('Ctrl Pts',(-1.76067249704884,22.6948386219843,
12.));
#244991=CARTESIAN_POINT('Ctrl Pts',(-1.76002606202399,22.7055360375481,
0.));
#244992=CARTESIAN_POINT('Ctrl Pts',(-1.76002606202399,22.7055360375481,
12.));
#244993=CARTESIAN_POINT('Ctrl Pts',(-1.75933006905924,22.7164346186007,
0.));
#244994=CARTESIAN_POINT('Ctrl Pts',(-1.75933006905924,22.7164346186007,
12.));
#244995=CARTESIAN_POINT('Ctrl Pts',(-1.75858354204635,22.7275311777305,
0.));
#244996=CARTESIAN_POINT('Ctrl Pts',(-1.75858354204635,22.7275311777305,
12.));
#244997=CARTESIAN_POINT('Ctrl Pts',(-1.75778553673249,22.7388226235565,
0.));
#244998=CARTESIAN_POINT('Ctrl Pts',(-1.75778553673249,22.7388226235565,
12.));
#244999=CARTESIAN_POINT('Ctrl Pts',(-1.75693513908911,22.7503059556455,
0.));
#245000=CARTESIAN_POINT('Ctrl Pts',(-1.75693513908911,22.7503059556455,
12.));
#245001=CARTESIAN_POINT('Ctrl Pts',(-1.7560314637164,22.7619782595013,0.));
#245002=CARTESIAN_POINT('Ctrl Pts',(-1.7560314637164,22.7619782595013,12.));
#245003=CARTESIAN_POINT('Ctrl Pts',(-1.75507365227127,22.7738367016115,
0.));
#245004=CARTESIAN_POINT('Ctrl Pts',(-1.75507365227127,22.7738367016115,
12.));
#245005=CARTESIAN_POINT('Ctrl Pts',(-1.7540608718293,22.7858785242358,0.));
#245006=CARTESIAN_POINT('Ctrl Pts',(-1.7540608718293,22.7858785242358,12.));
#245007=CARTESIAN_POINT('Ctrl Pts',(-1.75299231391461,22.7981010424312,
0.));
#245008=CARTESIAN_POINT('Ctrl Pts',(-1.75299231391461,22.7981010424312,
12.));
#245009=CARTESIAN_POINT('Ctrl Pts',(-1.7518671936559,22.8105016414712,0.));
#245010=CARTESIAN_POINT('Ctrl Pts',(-1.7518671936559,22.8105016414712,12.));
#245011=CARTESIAN_POINT('Ctrl Pts',(-1.75068474890884,22.8230777741285,
0.));
#245012=CARTESIAN_POINT('Ctrl Pts',(-1.75068474890884,22.8230777741285,
12.));
#245013=CARTESIAN_POINT('Ctrl Pts',(-1.74944423940117,22.8358269579854,
0.));
#245014=CARTESIAN_POINT('Ctrl Pts',(-1.74944423940117,22.8358269579854,
12.));
#245015=CARTESIAN_POINT('Ctrl Pts',(-1.74814494588492,22.8487467728075,
0.));
#245016=CARTESIAN_POINT('Ctrl Pts',(-1.74814494588492,22.8487467728075,
12.));
#245017=CARTESIAN_POINT('Ctrl Pts',(-1.74678616930663,22.8618348580234,
0.));
#245018=CARTESIAN_POINT('Ctrl Pts',(-1.74678616930663,22.8618348580234,
12.));
#245019=CARTESIAN_POINT('Ctrl Pts',(-1.745367229982,22.8750889101696,0.));
#245020=CARTESIAN_POINT('Ctrl Pts',(-1.745367229982,22.8750889101696,12.));
#245021=CARTESIAN_POINT('Ctrl Pts',(-1.74388746677702,22.8885066803351,
0.));
#245022=CARTESIAN_POINT('Ctrl Pts',(-1.74388746677702,22.8885066803351,
12.));
#245023=CARTESIAN_POINT('Ctrl Pts',(-1.74234623630079,22.9020859716144,
0.));
#245024=CARTESIAN_POINT('Ctrl Pts',(-1.74234623630079,22.9020859716144,
12.));
#245025=CARTESIAN_POINT('Ctrl Pts',(-1.74074291231057,22.9158246373365,
0.));
#245026=CARTESIAN_POINT('Ctrl Pts',(-1.74074291231057,22.9158246373365,
12.));
#245027=CARTESIAN_POINT('Ctrl Pts',(-1.73907688511664,22.9297205792587,
0.));
#245028=CARTESIAN_POINT('Ctrl Pts',(-1.73907688511664,22.9297205792587,
12.));
#245029=CARTESIAN_POINT('Ctrl Pts',(-1.73734756100038,22.9437717457825,
0.));
#245030=CARTESIAN_POINT('Ctrl Pts',(-1.73734756100038,22.9437717457825,
12.));
#245031=CARTESIAN_POINT('Ctrl Pts',(-1.73555436162771,22.9579761301062,
0.));
#245032=CARTESIAN_POINT('Ctrl Pts',(-1.73555436162771,22.9579761301062,
12.));
#245033=CARTESIAN_POINT('Ctrl Pts',(-1.73369672350818,22.9723317685688,
0.));
#245034=CARTESIAN_POINT('Ctrl Pts',(-1.73369672350818,22.9723317685688,
12.));
#245035=CARTESIAN_POINT('Ctrl Pts',(-1.73177409750194,22.9868367391978,
0.));
#245036=CARTESIAN_POINT('Ctrl Pts',(-1.73177409750194,22.9868367391978,
12.));
#245037=CARTESIAN_POINT('Ctrl Pts',(-1.72978594832137,23.0014891601891,
0.));
#245038=CARTESIAN_POINT('Ctrl Pts',(-1.72978594832137,23.0014891601891,
12.));
#245039=CARTESIAN_POINT('Ctrl Pts',(-1.72773175404703,23.0162871884167,
0.));
#245040=CARTESIAN_POINT('Ctrl Pts',(-1.72773175404703,23.0162871884167,
12.));
#245041=CARTESIAN_POINT('Ctrl Pts',(-1.72561100564033,23.031229017888,0.));
#245042=CARTESIAN_POINT('Ctrl Pts',(-1.72561100564033,23.031229017888,12.));
#245043=CARTESIAN_POINT('Ctrl Pts',(-1.72342320653731,23.0463128785528,
0.));
#245044=CARTESIAN_POINT('Ctrl Pts',(-1.72342320653731,23.0463128785528,
12.));
#245045=CARTESIAN_POINT('Ctrl Pts',(-1.7211678722598,23.061537035156,0.));
#245046=CARTESIAN_POINT('Ctrl Pts',(-1.7211678722598,23.061537035156,12.));
#245047=CARTESIAN_POINT('Ctrl Pts',(-1.71884453003027,23.0768997860709,
0.));
#245048=CARTESIAN_POINT('Ctrl Pts',(-1.71884453003027,23.0768997860709,
12.));
#245049=CARTESIAN_POINT('Ctrl Pts',(-1.71645271839311,23.0923994621216,
0.));
#245050=CARTESIAN_POINT('Ctrl Pts',(-1.71645271839311,23.0923994621216,
12.));
#245051=CARTESIAN_POINT('Ctrl Pts',(-1.71399198684725,23.1080344254291,
0.));
#245052=CARTESIAN_POINT('Ctrl Pts',(-1.71399198684725,23.1080344254291,
12.));
#245053=CARTESIAN_POINT('Ctrl Pts',(-1.71146189552192,23.1238030684929,
0.));
#245054=CARTESIAN_POINT('Ctrl Pts',(-1.71146189552192,23.1238030684929,
12.));
#245055=CARTESIAN_POINT('Ctrl Pts',(-1.7088620148546,23.1397038132358,0.));
#245056=CARTESIAN_POINT('Ctrl Pts',(-1.7088620148546,23.1397038132358,12.));
#245057=CARTESIAN_POINT('Ctrl Pts',(-1.70619192527847,23.1557351100613,
0.));
#245058=CARTESIAN_POINT('Ctrl Pts',(-1.70619192527847,23.1557351100613,
12.));
#245059=CARTESIAN_POINT('Ctrl Pts',(-1.70345121691259,23.1718954368749,
0.));
#245060=CARTESIAN_POINT('Ctrl Pts',(-1.70345121691259,23.1718954368749,
12.));
#245061=CARTESIAN_POINT('Ctrl Pts',(-1.70063948926987,23.1881832981848,
0.));
#245062=CARTESIAN_POINT('Ctrl Pts',(-1.70063948926987,23.1881832981848,
12.));
#245063=CARTESIAN_POINT('Ctrl Pts',(-1.69775635099425,23.2045972243765,
0.));
#245064=CARTESIAN_POINT('Ctrl Pts',(-1.69775635099425,23.2045972243765,
12.));
#245065=CARTESIAN_POINT('Ctrl Pts',(-1.69480141959946,23.2211357709374,
0.));
#245066=CARTESIAN_POINT('Ctrl Pts',(-1.69480141959946,23.2211357709374,
12.));
#245067=CARTESIAN_POINT('Ctrl Pts',(-1.69177432121716,23.2377975177014,
0.));
#245068=CARTESIAN_POINT('Ctrl Pts',(-1.69177432121716,23.2377975177014,
12.));
#245069=CARTESIAN_POINT('Ctrl Pts',(-1.6886746903491,23.2545810680536,0.));
#245070=CARTESIAN_POINT('Ctrl Pts',(-1.6886746903491,23.2545810680536,12.));
#245071=CARTESIAN_POINT('Ctrl Pts',(-1.68550216963275,23.2714850482245,
0.));
#245072=CARTESIAN_POINT('Ctrl Pts',(-1.68550216963275,23.2714850482245,
12.));
#245073=CARTESIAN_POINT('Ctrl Pts',(-1.68225640962181,23.2885081066949,
0.));
#245074=CARTESIAN_POINT('Ctrl Pts',(-1.68225640962181,23.2885081066949,
12.));
#245075=CARTESIAN_POINT('Ctrl Pts',(-1.67893706857123,23.3056489135611,
0.));
#245076=CARTESIAN_POINT('Ctrl Pts',(-1.67893706857123,23.3056489135611,
12.));
#245077=CARTESIAN_POINT('Ctrl Pts',(-1.67554381222987,23.3229061599145,
0.));
#245078=CARTESIAN_POINT('Ctrl Pts',(-1.67554381222987,23.3229061599145,
12.));
#245079=CARTESIAN_POINT('Ctrl Pts',(-1.67207631363905,23.3402785571866,
0.));
#245080=CARTESIAN_POINT('Ctrl Pts',(-1.67207631363905,23.3402785571866,
12.));
#245081=CARTESIAN_POINT('Ctrl Pts',(-1.66853425293978,23.3577648365747,
0.));
#245082=CARTESIAN_POINT('Ctrl Pts',(-1.66853425293978,23.3577648365747,
12.));
#245083=CARTESIAN_POINT('Ctrl Pts',(-1.66491731718864,23.375363748555,0.));
#245084=CARTESIAN_POINT('Ctrl Pts',(-1.66491731718864,23.375363748555,12.));
#245085=CARTESIAN_POINT('Ctrl Pts',(-1.66122520018008,23.3930740623622,
0.));
#245086=CARTESIAN_POINT('Ctrl Pts',(-1.66122520018008,23.3930740623622,
12.));
#245087=CARTESIAN_POINT('Ctrl Pts',(-1.65745760227507,23.4108945654803,
0.));
#245088=CARTESIAN_POINT('Ctrl Pts',(-1.65745760227507,23.4108945654803,
12.));
#245089=CARTESIAN_POINT('Ctrl Pts',(-1.6536142302373,23.4288240631034,0.));
#245090=CARTESIAN_POINT('Ctrl Pts',(-1.6536142302373,23.4288240631034,12.));
#245091=CARTESIAN_POINT('Ctrl Pts',(-1.6496947970734,23.446861377656,0.));
#245092=CARTESIAN_POINT('Ctrl Pts',(-1.6496947970734,23.446861377656,12.));
#245093=CARTESIAN_POINT('Ctrl Pts',(-1.64569902187608,23.4650053483919,
0.));
#245094=CARTESIAN_POINT('Ctrl Pts',(-1.64569902187608,23.4650053483919,
12.));
#245095=CARTESIAN_POINT('Ctrl Pts',(-1.64162662967525,23.4832548309638,
0.));
#245096=CARTESIAN_POINT('Ctrl Pts',(-1.64162662967525,23.4832548309638,
12.));
#245097=CARTESIAN_POINT('Ctrl Pts',(-1.63747735129474,23.5016086970006,
0.));
#245098=CARTESIAN_POINT('Ctrl Pts',(-1.63747735129474,23.5016086970006,
12.));
#245099=CARTESIAN_POINT('Ctrl Pts',(-1.63325092321731,23.5200658336624,
0.));
#245100=CARTESIAN_POINT('Ctrl Pts',(-1.63325092321731,23.5200658336624,
12.));
#245101=CARTESIAN_POINT('Ctrl Pts',(-1.62894708745231,23.5386251432278,
0.));
#245102=CARTESIAN_POINT('Ctrl Pts',(-1.62894708745231,23.5386251432278,
12.));
#245103=CARTESIAN_POINT('Ctrl Pts',(-1.62456559140072,23.5572855427617,
0.));
#245104=CARTESIAN_POINT('Ctrl Pts',(-1.62456559140072,23.5572855427617,
12.));
#245105=CARTESIAN_POINT('Ctrl Pts',(-1.62010618772869,23.5760459637608,
0.));
#245106=CARTESIAN_POINT('Ctrl Pts',(-1.62010618772869,23.5760459637608,
12.));
#245107=CARTESIAN_POINT('Ctrl Pts',(-1.61556863424697,23.5949053517996,
0.));
#245108=CARTESIAN_POINT('Ctrl Pts',(-1.61556863424697,23.5949053517996,
12.));
#245109=CARTESIAN_POINT('Ctrl Pts',(-1.61095269379773,23.6138626661644,
0.));
#245110=CARTESIAN_POINT('Ctrl Pts',(-1.61095269379773,23.6138626661644,
12.));
#245111=CARTESIAN_POINT('Ctrl Pts',(-1.60625813414666,23.6329168794916,
0.));
#245112=CARTESIAN_POINT('Ctrl Pts',(-1.60625813414666,23.6329168794916,
12.));
#245113=CARTESIAN_POINT('Ctrl Pts',(-1.60148472786588,23.6520669774863,
0.));
#245114=CARTESIAN_POINT('Ctrl Pts',(-1.60148472786588,23.6520669774863,
12.));
#245115=CARTESIAN_POINT('Ctrl Pts',(-1.59663225222458,23.6713119586302,
0.));
#245116=CARTESIAN_POINT('Ctrl Pts',(-1.59663225222458,23.6713119586302,
12.));
#245117=CARTESIAN_POINT('Ctrl Pts',(-1.59170048908632,23.6906508338833,
0.));
#245118=CARTESIAN_POINT('Ctrl Pts',(-1.59170048908632,23.6906508338833,
12.));
#245119=CARTESIAN_POINT('Ctrl Pts',(-1.58668922481222,23.7100826263835,
0.));
#245120=CARTESIAN_POINT('Ctrl Pts',(-1.58668922481222,23.7100826263835,
12.));
#245121=CARTESIAN_POINT('Ctrl Pts',(-1.58159825017362,23.7296063711308,
0.));
#245122=CARTESIAN_POINT('Ctrl Pts',(-1.58159825017362,23.7296063711308,
12.));
#245123=CARTESIAN_POINT('Ctrl Pts',(-1.57642736025251,23.7492211147369,
0.));
#245124=CARTESIAN_POINT('Ctrl Pts',(-1.57642736025251,23.7492211147369,
12.));
#245125=CARTESIAN_POINT('Ctrl Pts',(-1.57117635434412,23.7689259151869,
0.));
#245126=CARTESIAN_POINT('Ctrl Pts',(-1.57117635434412,23.7689259151869,
12.));
#245127=CARTESIAN_POINT('Ctrl Pts',(-1.56584503586844,23.788719841588,0.));
#245128=CARTESIAN_POINT('Ctrl Pts',(-1.56584503586844,23.788719841588,12.));
#245129=CARTESIAN_POINT('Ctrl Pts',(-1.56043321228631,23.8086019739192,
0.));
#245130=CARTESIAN_POINT('Ctrl Pts',(-1.56043321228631,23.8086019739192,
12.));
#245131=CARTESIAN_POINT('Ctrl Pts',(-1.55494069502628,23.8285714027631,
0.));
#245132=CARTESIAN_POINT('Ctrl Pts',(-1.55494069502628,23.8285714027631,
12.));
#245133=CARTESIAN_POINT('Ctrl Pts',(-1.5493672994053,23.8486272290698,0.));
#245134=CARTESIAN_POINT('Ctrl Pts',(-1.5493672994053,23.8486272290698,12.));
#245135=CARTESIAN_POINT('Ctrl Pts',(-1.54371284453978,23.8687685639635,
0.));
#245136=CARTESIAN_POINT('Ctrl Pts',(-1.54371284453978,23.8687685639635,
12.));
#245137=CARTESIAN_POINT('Ctrl Pts',(-1.53797715326748,23.8889945285313,
0.));
#245138=CARTESIAN_POINT('Ctrl Pts',(-1.53797715326748,23.8889945285313,
12.));
#245139=CARTESIAN_POINT('Ctrl Pts',(-1.53216005207462,23.9093042536119,
0.));
#245140=CARTESIAN_POINT('Ctrl Pts',(-1.53216005207462,23.9093042536119,
12.));
#245141=CARTESIAN_POINT('Ctrl Pts',(-1.5262613710304,23.9296968795761,0.));
#245142=CARTESIAN_POINT('Ctrl Pts',(-1.5262613710304,23.9296968795761,12.));
#245143=CARTESIAN_POINT('Ctrl Pts',(-1.52028094372806,23.9501715561038,
0.));
#245144=CARTESIAN_POINT('Ctrl Pts',(-1.52028094372806,23.9501715561038,
12.));
#245145=CARTESIAN_POINT('Ctrl Pts',(-1.51421860720628,23.9707274420145,
0.));
#245146=CARTESIAN_POINT('Ctrl Pts',(-1.51421860720628,23.9707274420145,
12.));
#245147=CARTESIAN_POINT('Ctrl Pts',(-1.50807420187703,23.991363705093,0.));
#245148=CARTESIAN_POINT('Ctrl Pts',(-1.50807420187703,23.991363705093,12.));
#245149=CARTESIAN_POINT('Ctrl Pts',(-1.50184757146099,24.0120795219086,
0.));
#245150=CARTESIAN_POINT('Ctrl Pts',(-1.50184757146099,24.0120795219086,
12.));
#245151=CARTESIAN_POINT('Ctrl Pts',(-1.49553856292798,24.0328740776331,
0.));
#245152=CARTESIAN_POINT('Ctrl Pts',(-1.49553856292798,24.0328740776331,
12.));
#245153=CARTESIAN_POINT('Ctrl Pts',(-1.48914702644883,24.053746565843,0.));
#245154=CARTESIAN_POINT('Ctrl Pts',(-1.48914702644883,24.053746565843,12.));
#245155=CARTESIAN_POINT('Ctrl Pts',(-1.4826728153368,24.074696188353,0.));
#245156=CARTESIAN_POINT('Ctrl Pts',(-1.4826728153368,24.074696188353,12.));
#245157=CARTESIAN_POINT('Ctrl Pts',(-1.47611578597741,24.0957221550782,
0.));
#245158=CARTESIAN_POINT('Ctrl Pts',(-1.47611578597741,24.0957221550782,
12.));
#245159=CARTESIAN_POINT('Ctrl Pts',(-1.46947579776992,24.1168236838827,
0.));
#245160=CARTESIAN_POINT('Ctrl Pts',(-1.46947579776992,24.1168236838827,
12.));
#245161=CARTESIAN_POINT('Ctrl Pts',(-1.46275271307398,24.1380000004272,
0.));
#245162=CARTESIAN_POINT('Ctrl Pts',(-1.46275271307398,24.1380000004272,
12.));
#245163=CARTESIAN_POINT('Ctrl Pts',(-1.45594639716314,24.1592503380105,
0.));
#245164=CARTESIAN_POINT('Ctrl Pts',(-1.45594639716314,24.1592503380105,
12.));
#245165=CARTESIAN_POINT('Ctrl Pts',(-1.44905671818721,24.1805739374033,
0.));
#245166=CARTESIAN_POINT('Ctrl Pts',(-1.44905671818721,24.1805739374033,
12.));
#245167=CARTESIAN_POINT('Ctrl Pts',(-1.44208354711074,24.2019700467214,
0.));
#245168=CARTESIAN_POINT('Ctrl Pts',(-1.44208354711074,24.2019700467214,
12.));
#245169=CARTESIAN_POINT('Ctrl Pts',(-1.43502675765502,24.2234379212978,
0.));
#245170=CARTESIAN_POINT('Ctrl Pts',(-1.43502675765502,24.2234379212978,
12.));
#245171=CARTESIAN_POINT('Ctrl Pts',(-1.42788622624851,24.2449768235485,
0.));
#245172=CARTESIAN_POINT('Ctrl Pts',(-1.42788622624851,24.2449768235485,
12.));
#245173=CARTESIAN_POINT('Ctrl Pts',(-1.42066183198252,24.2665860228357,
0.));
#245174=CARTESIAN_POINT('Ctrl Pts',(-1.42066183198252,24.2665860228357,
12.));
#245175=CARTESIAN_POINT('Ctrl Pts',(-1.41335345657685,24.2882647953214,
0.));
#245176=CARTESIAN_POINT('Ctrl Pts',(-1.41335345657685,24.2882647953214,
12.));
#245177=CARTESIAN_POINT('Ctrl Pts',(-1.40596098434341,24.3100124238316,
0.));
#245178=CARTESIAN_POINT('Ctrl Pts',(-1.40596098434341,24.3100124238316,
12.));
#245179=CARTESIAN_POINT('Ctrl Pts',(-1.3984843021281,24.3318281977647,0.));
#245180=CARTESIAN_POINT('Ctrl Pts',(-1.3984843021281,24.3318281977647,12.));
#245181=CARTESIAN_POINT('Ctrl Pts',(-1.3909232992639,24.3537114129877,0.));
#245182=CARTESIAN_POINT('Ctrl Pts',(-1.3909232992639,24.3537114129877,12.));
#245183=CARTESIAN_POINT('Ctrl Pts',(-1.38327786752998,24.37566137173,0.));
#245184=CARTESIAN_POINT('Ctrl Pts',(-1.38327786752998,24.37566137173,12.));
#245185=CARTESIAN_POINT('Ctrl Pts',(-1.37554790111608,24.3976773824731,
0.));
#245186=CARTESIAN_POINT('Ctrl Pts',(-1.37554790111608,24.3976773824731,
12.));
#245187=CARTESIAN_POINT('Ctrl Pts',(-1.36773329659954,24.4197587598337,
0.));
#245188=CARTESIAN_POINT('Ctrl Pts',(-1.36773329659954,24.4197587598337,
12.));
#245189=CARTESIAN_POINT('Ctrl Pts',(-1.35983395290624,24.4419048244524,
0.));
#245190=CARTESIAN_POINT('Ctrl Pts',(-1.35983395290624,24.4419048244524,
12.));
#245191=CARTESIAN_POINT('Ctrl Pts',(-1.35184977125645,24.4641149028894,
0.));
#245192=CARTESIAN_POINT('Ctrl Pts',(-1.35184977125645,24.4641149028894,
12.));
#245193=CARTESIAN_POINT('Ctrl Pts',(-1.34378065512335,24.4863883275135,
0.));
#245194=CARTESIAN_POINT('Ctrl Pts',(-1.34378065512335,24.4863883275135,
12.));
#245195=CARTESIAN_POINT('Ctrl Pts',(-1.33562651019684,24.5087244363856,
0.));
#245196=CARTESIAN_POINT('Ctrl Pts',(-1.33562651019684,24.5087244363856,
12.));
#245197=CARTESIAN_POINT('Ctrl Pts',(-1.32738724435326,24.5311225731434,
0.));
#245198=CARTESIAN_POINT('Ctrl Pts',(-1.32738724435326,24.5311225731434,
12.));
#245199=CARTESIAN_POINT('Ctrl Pts',(-1.31906276763669,24.5535820868671,
0.));
#245200=CARTESIAN_POINT('Ctrl Pts',(-1.31906276763669,24.5535820868671,
12.));
#245201=CARTESIAN_POINT('Ctrl Pts',(-1.31065299222023,24.576102332018,0.));
#245202=CARTESIAN_POINT('Ctrl Pts',(-1.31065299222023,24.576102332018,12.));
#245203=CARTESIAN_POINT('Ctrl Pts',(-1.30215783236364,24.5986826684025,
0.));
#245204=CARTESIAN_POINT('Ctrl Pts',(-1.30215783236364,24.5986826684025,
12.));
#245205=CARTESIAN_POINT('Ctrl Pts',(-1.29357720438108,24.6213224611228,
0.));
#245206=CARTESIAN_POINT('Ctrl Pts',(-1.29357720438108,24.6213224611228,
12.));
#245207=CARTESIAN_POINT('Ctrl Pts',(-1.28491102661514,24.6440210805278,
0.));
#245208=CARTESIAN_POINT('Ctrl Pts',(-1.28491102661514,24.6440210805278,
12.));
#245209=CARTESIAN_POINT('Ctrl Pts',(-1.2761592194164,24.666777902156,0.));
#245210=CARTESIAN_POINT('Ctrl Pts',(-1.2761592194164,24.666777902156,12.));
#245211=CARTESIAN_POINT('Ctrl Pts',(-1.26732170513497,24.6895923066837,
0.));
#245212=CARTESIAN_POINT('Ctrl Pts',(-1.26732170513497,24.6895923066837,
12.));
#245213=CARTESIAN_POINT('Ctrl Pts',(-1.25839840807415,24.7124636797895,
0.));
#245214=CARTESIAN_POINT('Ctrl Pts',(-1.25839840807415,24.7124636797895,
12.));
#245215=CARTESIAN_POINT('Ctrl Pts',(-1.24938925444324,24.7353914120012,
0.));
#245216=CARTESIAN_POINT('Ctrl Pts',(-1.24938925444324,24.7353914120012,
12.));
#245217=CARTESIAN_POINT('Ctrl Pts',(-1.24029417231988,24.7583748985439,
0.));
#245218=CARTESIAN_POINT('Ctrl Pts',(-1.24029417231988,24.7583748985439,
12.));
#245219=CARTESIAN_POINT('Ctrl Pts',(-1.23111309161843,24.78141353918,0.));
#245220=CARTESIAN_POINT('Ctrl Pts',(-1.23111309161843,24.78141353918,12.));
#245221=CARTESIAN_POINT('Ctrl Pts',(-1.22184594406526,24.8045067380536,
0.));
#245222=CARTESIAN_POINT('Ctrl Pts',(-1.22184594406526,24.8045067380536,
12.));
#245223=CARTESIAN_POINT('Ctrl Pts',(-1.21249266318205,24.8276539035092,
0.));
#245224=CARTESIAN_POINT('Ctrl Pts',(-1.21249266318205,24.8276539035092,
12.));
#245225=CARTESIAN_POINT('Ctrl Pts',(-1.20305318426015,24.8508544481973,
0.));
#245226=CARTESIAN_POINT('Ctrl Pts',(-1.20305318426015,24.8508544481973,
12.));
#245227=CARTESIAN_POINT('Ctrl Pts',(-1.19352744434059,24.8741077892074,
0.));
#245228=CARTESIAN_POINT('Ctrl Pts',(-1.19352744434059,24.8741077892074,
12.));
#245229=CARTESIAN_POINT('Ctrl Pts',(-1.18391538220098,24.8974133481829,
0.));
#245230=CARTESIAN_POINT('Ctrl Pts',(-1.18391538220098,24.8974133481829,
12.));
#245231=CARTESIAN_POINT('Ctrl Pts',(-1.17421693835039,24.9207705514449,
0.));
#245232=CARTESIAN_POINT('Ctrl Pts',(-1.17421693835039,24.9207705514449,
12.));
#245233=CARTESIAN_POINT('Ctrl Pts',(-1.16443205502852,24.9441788300932,
0.));
#245234=CARTESIAN_POINT('Ctrl Pts',(-1.16443205502852,24.9441788300932,
12.));
#245235=CARTESIAN_POINT('Ctrl Pts',(-1.15456067621894,24.9676376201501,
0.));
#245236=CARTESIAN_POINT('Ctrl Pts',(-1.15456067621894,24.9676376201501,
12.));
#245237=CARTESIAN_POINT('Ctrl Pts',(-1.14460274758206,24.9911463621431,
0.));
#245238=CARTESIAN_POINT('Ctrl Pts',(-1.14460274758206,24.9911463621431,
12.));
#245239=CARTESIAN_POINT('Ctrl Pts',(-1.13455821638536,25.0147045006193,
0.));
#245240=CARTESIAN_POINT('Ctrl Pts',(-1.13455821638536,25.0147045006193,
12.));
#245241=CARTESIAN_POINT('Ctrl Pts',(-1.12442703144455,25.0383114836898,
0.));
#245242=CARTESIAN_POINT('Ctrl Pts',(-1.12442703144455,25.0383114836898,
12.));
#245243=CARTESIAN_POINT('Ctrl Pts',(-1.1142091430689,25.0619667625336,0.));
#245244=CARTESIAN_POINT('Ctrl Pts',(-1.1142091430689,25.0619667625336,12.));
#245245=CARTESIAN_POINT('Ctrl Pts',(-1.1039045030174,25.085669790968,0.));
#245246=CARTESIAN_POINT('Ctrl Pts',(-1.1039045030174,25.085669790968,12.));
#245247=CARTESIAN_POINT('Ctrl Pts',(-1.09351306445299,25.1094200248448,
0.));
#245248=CARTESIAN_POINT('Ctrl Pts',(-1.09351306445299,25.1094200248448,
12.));
#245249=CARTESIAN_POINT('Ctrl Pts',(-1.08303478197174,25.1332169227415,
0.));
#245250=CARTESIAN_POINT('Ctrl Pts',(-1.08303478197174,25.1332169227415,
12.));
#245251=CARTESIAN_POINT('Ctrl Pts',(-1.0724696116546,25.1570599469311,0.));
#245252=CARTESIAN_POINT('Ctrl Pts',(-1.0724696116546,25.1570599469311,12.));
#245253=CARTESIAN_POINT('Ctrl Pts',(-1.06181751111754,25.1809485642191,
0.));
#245254=CARTESIAN_POINT('Ctrl Pts',(-1.06181751111754,25.1809485642191,
12.));
#245255=CARTESIAN_POINT('Ctrl Pts',(-1.05107843957926,25.2048822469027,
0.));
#245256=CARTESIAN_POINT('Ctrl Pts',(-1.05107843957926,25.2048822469027,
12.));
#245257=CARTESIAN_POINT('Ctrl Pts',(-1.04025235791515,25.2288604735087,
0.));
#245258=CARTESIAN_POINT('Ctrl Pts',(-1.04025235791515,25.2288604735087,
12.));
#245259=CARTESIAN_POINT('Ctrl Pts',(-1.0293392287683,25.2528827300427,0.));
#245260=CARTESIAN_POINT('Ctrl Pts',(-1.0293392287683,25.2528827300427,12.));
#245261=CARTESIAN_POINT('Ctrl Pts',(-1.01833901642272,25.2769485087268,
0.));
#245262=CARTESIAN_POINT('Ctrl Pts',(-1.01833901642272,25.2769485087268,
12.));
#245263=CARTESIAN_POINT('Ctrl Pts',(-1.00725168656934,25.3010573055557,
0.));
#245264=CARTESIAN_POINT('Ctrl Pts',(-1.00725168656934,25.3010573055557,
12.));
#245265=CARTESIAN_POINT('Ctrl Pts',(-0.99607720612092,25.3252086182976,
0.));
#245266=CARTESIAN_POINT('Ctrl Pts',(-0.99607720612092,25.3252086182976,
12.));
#245267=CARTESIAN_POINT('Ctrl Pts',(-0.984815543004092,25.3494019441444,
0.));
#245268=CARTESIAN_POINT('Ctrl Pts',(-0.984815543004092,25.3494019441444,
12.));
#245269=CARTESIAN_POINT('Ctrl Pts',(-0.973466666000049,25.3736367778842,
0.));
#245270=CARTESIAN_POINT('Ctrl Pts',(-0.973466666000049,25.3736367778842,
12.));
#245271=CARTESIAN_POINT('Ctrl Pts',(-0.962030544502803,25.3979126089155,
0.));
#245272=CARTESIAN_POINT('Ctrl Pts',(-0.962030544502803,25.3979126089155,
12.));
#245273=CARTESIAN_POINT('Ctrl Pts',(-0.95050714859697,25.4222289223155,
0.));
#245274=CARTESIAN_POINT('Ctrl Pts',(-0.95050714859697,25.4222289223155,
12.));
#245275=CARTESIAN_POINT('Ctrl Pts',(-0.938896449495633,25.4465852044835,
0.));
#245276=CARTESIAN_POINT('Ctrl Pts',(-0.938896449495633,25.4465852044835,
12.));
#245277=CARTESIAN_POINT('Ctrl Pts',(-0.927198419885605,25.4709809474996,
0.));
#245278=CARTESIAN_POINT('Ctrl Pts',(-0.927198419885605,25.4709809474996,
12.));
#245279=CARTESIAN_POINT('Ctrl Pts',(-0.915413034335334,25.4954156541787,
0.));
#245280=CARTESIAN_POINT('Ctrl Pts',(-0.915413034335334,25.4954156541787,
12.));
#245281=CARTESIAN_POINT('Ctrl Pts',(-0.903540269651155,25.5198888424195,
0.));
#245282=CARTESIAN_POINT('Ctrl Pts',(-0.903540269651155,25.5198888424195,
12.));
#245283=CARTESIAN_POINT('Ctrl Pts',(-0.891580105349468,25.5444000508223,
0.));
#245284=CARTESIAN_POINT('Ctrl Pts',(-0.891580105349468,25.5444000508223,
12.));
#245285=CARTESIAN_POINT('Ctrl Pts',(-0.879532523835092,25.568948840818,
0.));
#245286=CARTESIAN_POINT('Ctrl Pts',(-0.879532523835092,25.568948840818,
12.));
#245287=CARTESIAN_POINT('Ctrl Pts',(-0.86739750933947,25.5935347843616,
0.));
#245288=CARTESIAN_POINT('Ctrl Pts',(-0.86739750933947,25.5935347843616,
12.));
#245289=CARTESIAN_POINT('Ctrl Pts',(-0.855175047037615,25.618157453608,
0.));
#245290=CARTESIAN_POINT('Ctrl Pts',(-0.855175047037615,25.618157453608,
12.));
#245291=CARTESIAN_POINT('Ctrl Pts',(-0.842865122121547,25.6428164100078,
0.));
#245292=CARTESIAN_POINT('Ctrl Pts',(-0.842865122121547,25.6428164100078,
12.));
#245293=CARTESIAN_POINT('Ctrl Pts',(-0.830467718864369,25.6675111931957,
0.));
#245294=CARTESIAN_POINT('Ctrl Pts',(-0.830467718864369,25.6675111931957,
12.));
#245295=CARTESIAN_POINT('Ctrl Pts',(-0.81798281978672,25.6922413110172,
0.));
#245296=CARTESIAN_POINT('Ctrl Pts',(-0.81798281978672,25.6922413110172,
12.));
#245297=CARTESIAN_POINT('Ctrl Pts',(-0.805410404552596,25.7170062262474,
0.));
#245298=CARTESIAN_POINT('Ctrl Pts',(-0.805410404552596,25.7170062262474,
12.));
#245299=CARTESIAN_POINT('Ctrl Pts',(-0.792750451613536,25.7418053757671,
0.));
#245300=CARTESIAN_POINT('Ctrl Pts',(-0.792750451613536,25.7418053757671,
12.));
#245301=CARTESIAN_POINT('Ctrl Pts',(-0.780002940289027,25.7666381946871,
0.));
#245302=CARTESIAN_POINT('Ctrl Pts',(-0.780002940289027,25.7666381946871,
12.));
#245303=CARTESIAN_POINT('Ctrl Pts',(-0.767167852648641,25.7915041383304,
0.));
#245304=CARTESIAN_POINT('Ctrl Pts',(-0.767167852648641,25.7915041383304,
12.));
#245305=CARTESIAN_POINT('Ctrl Pts',(-0.75424517560829,25.816402705995,0.));
#245306=CARTESIAN_POINT('Ctrl Pts',(-0.75424517560829,25.816402705995,12.));
#245307=CARTESIAN_POINT('Ctrl Pts',(-0.741234902664698,25.841333461908,
0.));
#245308=CARTESIAN_POINT('Ctrl Pts',(-0.741234902664698,25.841333461908,
12.));
#245309=CARTESIAN_POINT('Ctrl Pts',(-0.728137036485879,25.8662960624285,
0.));
#245310=CARTESIAN_POINT('Ctrl Pts',(-0.728137036485879,25.8662960624285,
12.));
#245311=CARTESIAN_POINT('Ctrl Pts',(-0.714951588533753,25.8912902615141,
0.));
#245312=CARTESIAN_POINT('Ctrl Pts',(-0.714951588533753,25.8912902615141,
12.));
#245313=CARTESIAN_POINT('Ctrl Pts',(-0.701678575236603,25.9163158909645,
0.));
#245314=CARTESIAN_POINT('Ctrl Pts',(-0.701678575236603,25.9163158909645,
12.));
#245315=CARTESIAN_POINT('Ctrl Pts',(-0.688318015065679,25.941372847213,
0.));
#245316=CARTESIAN_POINT('Ctrl Pts',(-0.688318015065679,25.941372847213,
12.));
#245317=CARTESIAN_POINT('Ctrl Pts',(-0.677559543215903,25.9614434298092,
0.));
#245318=CARTESIAN_POINT('Ctrl Pts',(-0.677559543215903,25.9614434298092,
12.));
#245319=CARTESIAN_POINT('Ctrl Pts',(-0.669451306784418,25.9765104298171,
0.));
#245320=CARTESIAN_POINT('Ctrl Pts',(-0.669451306784418,25.9765104298171,
12.));
#245321=CARTESIAN_POINT('Ctrl Pts',(-0.664028313188914,25.9865613464809,
0.));
#245322=CARTESIAN_POINT('Ctrl Pts',(-0.664028313188914,25.9865613464809,
12.));
#245323=CARTESIAN_POINT('Ctrl Pts',(-0.661312440730891,25.991588367311,
0.));
#245324=CARTESIAN_POINT('Ctrl Pts',(-0.661312440730891,25.991588367311,
12.));
#245325=CARTESIAN_POINT('',(-0.661312440730891,25.991588367311,0.));
#245326=CARTESIAN_POINT('Ctrl Pts',(-1.76341220531179,22.4835757167854,
0.));
#245327=CARTESIAN_POINT('Ctrl Pts',(-1.76341415538764,22.483581992979,0.));
#245328=CARTESIAN_POINT('Ctrl Pts',(-1.7634206426357,22.4836387052232,0.));
#245329=CARTESIAN_POINT('Ctrl Pts',(-1.76343813434565,22.483856251707,0.));
#245330=CARTESIAN_POINT('Ctrl Pts',(-1.76347698284792,22.4844112933129,
0.));
#245331=CARTESIAN_POINT('Ctrl Pts',(-1.76355076045546,22.4855446605991,
0.));
#245332=CARTESIAN_POINT('Ctrl Pts',(-1.76364784232963,22.4871115206571,
0.));
#245333=CARTESIAN_POINT('Ctrl Pts',(-1.76376424879505,22.4890991659478,
0.));
#245334=CARTESIAN_POINT('Ctrl Pts',(-1.76389475965724,22.4914909094908,
0.));
#245335=CARTESIAN_POINT('Ctrl Pts',(-1.76403393880301,22.4942693792449,
0.));
#245336=CARTESIAN_POINT('Ctrl Pts',(-1.76417731243462,22.4974203063191,
0.));
#245337=CARTESIAN_POINT('Ctrl Pts',(-1.76432160068725,22.5009332677316,
0.));
#245338=CARTESIAN_POINT('Ctrl Pts',(-1.76446408210366,22.5047996391978,
0.));
#245339=CARTESIAN_POINT('Ctrl Pts',(-1.76460218257323,22.5090112700212,
0.));
#245340=CARTESIAN_POINT('Ctrl Pts',(-1.76473303281159,22.5135590569554,
0.));
#245341=CARTESIAN_POINT('Ctrl Pts',(-1.76485369319896,22.5184336670207,
0.));
#245342=CARTESIAN_POINT('Ctrl Pts',(-1.76496128643369,22.5236259635515,
0.));
#245343=CARTESIAN_POINT('Ctrl Pts',(-1.76505320262752,22.529127665298,0.));
#245344=CARTESIAN_POINT('Ctrl Pts',(-1.7651271156325,22.5349313983571,0.));
#245345=CARTESIAN_POINT('Ctrl Pts',(-1.76518087841493,22.5410303590891,
0.));
#245346=CARTESIAN_POINT('Ctrl Pts',(-1.76521245524047,22.5474180954006,
0.));
#245347=CARTESIAN_POINT('Ctrl Pts',(-1.76521983384063,22.5540882235837,
0.));
#245348=CARTESIAN_POINT('Ctrl Pts',(-1.76520104500449,22.5610344912501,
0.));
#245349=CARTESIAN_POINT('Ctrl Pts',(-1.76515418518829,22.5682508499873,
0.));
#245350=CARTESIAN_POINT('Ctrl Pts',(-1.76507744026747,22.5757315316355,
0.));
#245351=CARTESIAN_POINT('Ctrl Pts',(-1.76496910283088,22.5834711038024,
0.));
#245352=CARTESIAN_POINT('Ctrl Pts',(-1.76482755288411,22.5914644078106,
0.));
#245353=CARTESIAN_POINT('Ctrl Pts',(-1.76465124413556,22.5997065145638,
0.));
#245354=CARTESIAN_POINT('Ctrl Pts',(-1.76443868648015,22.6081926681342,
0.));
#245355=CARTESIAN_POINT('Ctrl Pts',(-1.76418843543739,22.6169182517693,
0.));
#245356=CARTESIAN_POINT('Ctrl Pts',(-1.76389909571402,22.6258787994847,
0.));
#245357=CARTESIAN_POINT('Ctrl Pts',(-1.76356932176272,22.635069997936,0.));
#245358=CARTESIAN_POINT('Ctrl Pts',(-1.76319782013914,22.6444876940425,
0.));
#245359=CARTESIAN_POINT('Ctrl Pts',(-1.76278334912559,22.6541278938413,
0.));
#245360=CARTESIAN_POINT('Ctrl Pts',(-1.76232471392567,22.6639867471756,
0.));
#245361=CARTESIAN_POINT('Ctrl Pts',(-1.76182076289525,22.6740605356699,
0.));
#245362=CARTESIAN_POINT('Ctrl Pts',(-1.76127038310613,22.6843456585245,
0.));
#245363=CARTESIAN_POINT('Ctrl Pts',(-1.76067249704884,22.6948386219843,
0.));
#245364=CARTESIAN_POINT('Ctrl Pts',(-1.76002606202399,22.7055360375481,
0.));
#245365=CARTESIAN_POINT('Ctrl Pts',(-1.75933006905924,22.7164346186007,
0.));
#245366=CARTESIAN_POINT('Ctrl Pts',(-1.75858354204635,22.7275311777305,
0.));
#245367=CARTESIAN_POINT('Ctrl Pts',(-1.75778553673249,22.7388226235565,
0.));
#245368=CARTESIAN_POINT('Ctrl Pts',(-1.75693513908911,22.7503059556455,
0.));
#245369=CARTESIAN_POINT('Ctrl Pts',(-1.7560314637164,22.7619782595013,0.));
#245370=CARTESIAN_POINT('Ctrl Pts',(-1.75507365227127,22.7738367016115,
0.));
#245371=CARTESIAN_POINT('Ctrl Pts',(-1.7540608718293,22.7858785242358,0.));
#245372=CARTESIAN_POINT('Ctrl Pts',(-1.75299231391461,22.7981010424312,
0.));
#245373=CARTESIAN_POINT('Ctrl Pts',(-1.7518671936559,22.8105016414712,0.));
#245374=CARTESIAN_POINT('Ctrl Pts',(-1.75068474890884,22.8230777741285,
0.));
#245375=CARTESIAN_POINT('Ctrl Pts',(-1.74944423940117,22.8358269579854,
0.));
#245376=CARTESIAN_POINT('Ctrl Pts',(-1.74814494588492,22.8487467728075,
0.));
#245377=CARTESIAN_POINT('Ctrl Pts',(-1.74678616930663,22.8618348580234,
0.));
#245378=CARTESIAN_POINT('Ctrl Pts',(-1.745367229982,22.8750889101696,0.));
#245379=CARTESIAN_POINT('Ctrl Pts',(-1.74388746677702,22.8885066803351,
0.));
#245380=CARTESIAN_POINT('Ctrl Pts',(-1.74234623630079,22.9020859716144,
0.));
#245381=CARTESIAN_POINT('Ctrl Pts',(-1.74074291231057,22.9158246373365,
0.));
#245382=CARTESIAN_POINT('Ctrl Pts',(-1.73907688511664,22.9297205792587,
0.));
#245383=CARTESIAN_POINT('Ctrl Pts',(-1.73734756100038,22.9437717457825,
0.));
#245384=CARTESIAN_POINT('Ctrl Pts',(-1.73555436162771,22.9579761301062,
0.));
#245385=CARTESIAN_POINT('Ctrl Pts',(-1.73369672350818,22.9723317685688,
0.));
#245386=CARTESIAN_POINT('Ctrl Pts',(-1.73177409750194,22.9868367391978,
0.));
#245387=CARTESIAN_POINT('Ctrl Pts',(-1.72978594832137,23.0014891601891,
0.));
#245388=CARTESIAN_POINT('Ctrl Pts',(-1.72773175404703,23.0162871884167,
0.));
#245389=CARTESIAN_POINT('Ctrl Pts',(-1.72561100564033,23.031229017888,0.));
#245390=CARTESIAN_POINT('Ctrl Pts',(-1.72342320653731,23.0463128785528,
0.));
#245391=CARTESIAN_POINT('Ctrl Pts',(-1.7211678722598,23.061537035156,0.));
#245392=CARTESIAN_POINT('Ctrl Pts',(-1.71884453003027,23.0768997860709,
0.));
#245393=CARTESIAN_POINT('Ctrl Pts',(-1.71645271839311,23.0923994621216,
0.));
#245394=CARTESIAN_POINT('Ctrl Pts',(-1.71399198684725,23.1080344254291,
0.));
#245395=CARTESIAN_POINT('Ctrl Pts',(-1.71146189552192,23.1238030684929,
0.));
#245396=CARTESIAN_POINT('Ctrl Pts',(-1.7088620148546,23.1397038132358,0.));
#245397=CARTESIAN_POINT('Ctrl Pts',(-1.70619192527847,23.1557351100613,
0.));
#245398=CARTESIAN_POINT('Ctrl Pts',(-1.70345121691259,23.1718954368749,
0.));
#245399=CARTESIAN_POINT('Ctrl Pts',(-1.70063948926987,23.1881832981848,
0.));
#245400=CARTESIAN_POINT('Ctrl Pts',(-1.69775635099425,23.2045972243765,
0.));
#245401=CARTESIAN_POINT('Ctrl Pts',(-1.69480141959946,23.2211357709374,
0.));
#245402=CARTESIAN_POINT('Ctrl Pts',(-1.69177432121716,23.2377975177014,
0.));
#245403=CARTESIAN_POINT('Ctrl Pts',(-1.6886746903491,23.2545810680536,0.));
#245404=CARTESIAN_POINT('Ctrl Pts',(-1.68550216963275,23.2714850482245,
0.));
#245405=CARTESIAN_POINT('Ctrl Pts',(-1.68225640962181,23.2885081066949,
0.));
#245406=CARTESIAN_POINT('Ctrl Pts',(-1.67893706857123,23.3056489135611,
0.));
#245407=CARTESIAN_POINT('Ctrl Pts',(-1.67554381222987,23.3229061599145,
0.));
#245408=CARTESIAN_POINT('Ctrl Pts',(-1.67207631363905,23.3402785571866,
0.));
#245409=CARTESIAN_POINT('Ctrl Pts',(-1.66853425293978,23.3577648365747,
0.));
#245410=CARTESIAN_POINT('Ctrl Pts',(-1.66491731718864,23.375363748555,0.));
#245411=CARTESIAN_POINT('Ctrl Pts',(-1.66122520018008,23.3930740623622,
0.));
#245412=CARTESIAN_POINT('Ctrl Pts',(-1.65745760227507,23.4108945654803,
0.));
#245413=CARTESIAN_POINT('Ctrl Pts',(-1.6536142302373,23.4288240631034,0.));
#245414=CARTESIAN_POINT('Ctrl Pts',(-1.6496947970734,23.446861377656,0.));
#245415=CARTESIAN_POINT('Ctrl Pts',(-1.64569902187608,23.4650053483919,
0.));
#245416=CARTESIAN_POINT('Ctrl Pts',(-1.64162662967525,23.4832548309638,
0.));
#245417=CARTESIAN_POINT('Ctrl Pts',(-1.63747735129474,23.5016086970006,
0.));
#245418=CARTESIAN_POINT('Ctrl Pts',(-1.63325092321731,23.5200658336624,
0.));
#245419=CARTESIAN_POINT('Ctrl Pts',(-1.62894708745231,23.5386251432278,
0.));
#245420=CARTESIAN_POINT('Ctrl Pts',(-1.62456559140072,23.5572855427617,
0.));
#245421=CARTESIAN_POINT('Ctrl Pts',(-1.62010618772869,23.5760459637608,
0.));
#245422=CARTESIAN_POINT('Ctrl Pts',(-1.61556863424697,23.5949053517996,
0.));
#245423=CARTESIAN_POINT('Ctrl Pts',(-1.61095269379773,23.6138626661644,
0.));
#245424=CARTESIAN_POINT('Ctrl Pts',(-1.60625813414666,23.6329168794916,
0.));
#245425=CARTESIAN_POINT('Ctrl Pts',(-1.60148472786588,23.6520669774863,
0.));
#245426=CARTESIAN_POINT('Ctrl Pts',(-1.59663225222458,23.6713119586302,
0.));
#245427=CARTESIAN_POINT('Ctrl Pts',(-1.59170048908632,23.6906508338833,
0.));
#245428=CARTESIAN_POINT('Ctrl Pts',(-1.58668922481222,23.7100826263835,
0.));
#245429=CARTESIAN_POINT('Ctrl Pts',(-1.58159825017362,23.7296063711308,
0.));
#245430=CARTESIAN_POINT('Ctrl Pts',(-1.57642736025251,23.7492211147369,
0.));
#245431=CARTESIAN_POINT('Ctrl Pts',(-1.57117635434412,23.7689259151869,
0.));
#245432=CARTESIAN_POINT('Ctrl Pts',(-1.56584503586844,23.788719841588,0.));
#245433=CARTESIAN_POINT('Ctrl Pts',(-1.56043321228631,23.8086019739192,
0.));
#245434=CARTESIAN_POINT('Ctrl Pts',(-1.55494069502628,23.8285714027631,
0.));
#245435=CARTESIAN_POINT('Ctrl Pts',(-1.5493672994053,23.8486272290698,0.));
#245436=CARTESIAN_POINT('Ctrl Pts',(-1.54371284453978,23.8687685639635,
0.));
#245437=CARTESIAN_POINT('Ctrl Pts',(-1.53797715326748,23.8889945285313,
0.));
#245438=CARTESIAN_POINT('Ctrl Pts',(-1.53216005207462,23.9093042536119,
0.));
#245439=CARTESIAN_POINT('Ctrl Pts',(-1.5262613710304,23.9296968795761,0.));
#245440=CARTESIAN_POINT('Ctrl Pts',(-1.52028094372806,23.9501715561038,
0.));
#245441=CARTESIAN_POINT('Ctrl Pts',(-1.51421860720628,23.9707274420145,
0.));
#245442=CARTESIAN_POINT('Ctrl Pts',(-1.50807420187703,23.991363705093,0.));
#245443=CARTESIAN_POINT('Ctrl Pts',(-1.50184757146099,24.0120795219086,
0.));
#245444=CARTESIAN_POINT('Ctrl Pts',(-1.49553856292798,24.0328740776331,
0.));
#245445=CARTESIAN_POINT('Ctrl Pts',(-1.48914702644883,24.053746565843,0.));
#245446=CARTESIAN_POINT('Ctrl Pts',(-1.4826728153368,24.074696188353,0.));
#245447=CARTESIAN_POINT('Ctrl Pts',(-1.47611578597741,24.0957221550782,
0.));
#245448=CARTESIAN_POINT('Ctrl Pts',(-1.46947579776992,24.1168236838827,
0.));
#245449=CARTESIAN_POINT('Ctrl Pts',(-1.46275271307398,24.1380000004272,
0.));
#245450=CARTESIAN_POINT('Ctrl Pts',(-1.45594639716314,24.1592503380105,
0.));
#245451=CARTESIAN_POINT('Ctrl Pts',(-1.44905671818721,24.1805739374033,
0.));
#245452=CARTESIAN_POINT('Ctrl Pts',(-1.44208354711074,24.2019700467214,
0.));
#245453=CARTESIAN_POINT('Ctrl Pts',(-1.43502675765502,24.2234379212978,
0.));
#245454=CARTESIAN_POINT('Ctrl Pts',(-1.42788622624851,24.2449768235485,
0.));
#245455=CARTESIAN_POINT('Ctrl Pts',(-1.42066183198252,24.2665860228357,
0.));
#245456=CARTESIAN_POINT('Ctrl Pts',(-1.41335345657685,24.2882647953214,
0.));
#245457=CARTESIAN_POINT('Ctrl Pts',(-1.40596098434341,24.3100124238316,
0.));
#245458=CARTESIAN_POINT('Ctrl Pts',(-1.3984843021281,24.3318281977647,0.));
#245459=CARTESIAN_POINT('Ctrl Pts',(-1.3909232992639,24.3537114129877,0.));
#245460=CARTESIAN_POINT('Ctrl Pts',(-1.38327786752998,24.37566137173,0.));
#245461=CARTESIAN_POINT('Ctrl Pts',(-1.37554790111608,24.3976773824731,
0.));
#245462=CARTESIAN_POINT('Ctrl Pts',(-1.36773329659954,24.4197587598337,
0.));
#245463=CARTESIAN_POINT('Ctrl Pts',(-1.35983395290624,24.4419048244524,
0.));
#245464=CARTESIAN_POINT('Ctrl Pts',(-1.35184977125645,24.4641149028894,
0.));
#245465=CARTESIAN_POINT('Ctrl Pts',(-1.34378065512335,24.4863883275135,
0.));
#245466=CARTESIAN_POINT('Ctrl Pts',(-1.33562651019684,24.5087244363856,
0.));
#245467=CARTESIAN_POINT('Ctrl Pts',(-1.32738724435326,24.5311225731434,
0.));
#245468=CARTESIAN_POINT('Ctrl Pts',(-1.31906276763669,24.5535820868671,
0.));
#245469=CARTESIAN_POINT('Ctrl Pts',(-1.31065299222023,24.576102332018,0.));
#245470=CARTESIAN_POINT('Ctrl Pts',(-1.30215783236364,24.5986826684025,
0.));
#245471=CARTESIAN_POINT('Ctrl Pts',(-1.29357720438108,24.6213224611228,
0.));
#245472=CARTESIAN_POINT('Ctrl Pts',(-1.28491102661514,24.6440210805278,
0.));
#245473=CARTESIAN_POINT('Ctrl Pts',(-1.2761592194164,24.666777902156,0.));
#245474=CARTESIAN_POINT('Ctrl Pts',(-1.26732170513497,24.6895923066837,
0.));
#245475=CARTESIAN_POINT('Ctrl Pts',(-1.25839840807415,24.7124636797895,
0.));
#245476=CARTESIAN_POINT('Ctrl Pts',(-1.24938925444324,24.7353914120012,
0.));
#245477=CARTESIAN_POINT('Ctrl Pts',(-1.24029417231988,24.7583748985439,
0.));
#245478=CARTESIAN_POINT('Ctrl Pts',(-1.23111309161843,24.78141353918,0.));
#245479=CARTESIAN_POINT('Ctrl Pts',(-1.22184594406526,24.8045067380536,
0.));
#245480=CARTESIAN_POINT('Ctrl Pts',(-1.21249266318205,24.8276539035092,
0.));
#245481=CARTESIAN_POINT('Ctrl Pts',(-1.20305318426015,24.8508544481973,
0.));
#245482=CARTESIAN_POINT('Ctrl Pts',(-1.19352744434059,24.8741077892074,
0.));
#245483=CARTESIAN_POINT('Ctrl Pts',(-1.18391538220098,24.8974133481829,
0.));
#245484=CARTESIAN_POINT('Ctrl Pts',(-1.17421693835039,24.9207705514449,
0.));
#245485=CARTESIAN_POINT('Ctrl Pts',(-1.16443205502852,24.9441788300932,
0.));
#245486=CARTESIAN_POINT('Ctrl Pts',(-1.15456067621894,24.9676376201501,
0.));
#245487=CARTESIAN_POINT('Ctrl Pts',(-1.14460274758206,24.9911463621431,
0.));
#245488=CARTESIAN_POINT('Ctrl Pts',(-1.13455821638536,25.0147045006193,
0.));
#245489=CARTESIAN_POINT('Ctrl Pts',(-1.12442703144455,25.0383114836898,
0.));
#245490=CARTESIAN_POINT('Ctrl Pts',(-1.1142091430689,25.0619667625336,0.));
#245491=CARTESIAN_POINT('Ctrl Pts',(-1.1039045030174,25.085669790968,0.));
#245492=CARTESIAN_POINT('Ctrl Pts',(-1.09351306445299,25.1094200248448,
0.));
#245493=CARTESIAN_POINT('Ctrl Pts',(-1.08303478197174,25.1332169227415,
0.));
#245494=CARTESIAN_POINT('Ctrl Pts',(-1.0724696116546,25.1570599469311,0.));
#245495=CARTESIAN_POINT('Ctrl Pts',(-1.06181751111754,25.1809485642191,
0.));
#245496=CARTESIAN_POINT('Ctrl Pts',(-1.05107843957926,25.2048822469027,
0.));
#245497=CARTESIAN_POINT('Ctrl Pts',(-1.04025235791515,25.2288604735087,
0.));
#245498=CARTESIAN_POINT('Ctrl Pts',(-1.0293392287683,25.2528827300427,0.));
#245499=CARTESIAN_POINT('Ctrl Pts',(-1.01833901642272,25.2769485087268,
0.));
#245500=CARTESIAN_POINT('Ctrl Pts',(-1.00725168656934,25.3010573055557,
0.));
#245501=CARTESIAN_POINT('Ctrl Pts',(-0.99607720612092,25.3252086182976,
0.));
#245502=CARTESIAN_POINT('Ctrl Pts',(-0.984815543004092,25.3494019441444,
0.));
#245503=CARTESIAN_POINT('Ctrl Pts',(-0.973466666000049,25.3736367778842,
0.));
#245504=CARTESIAN_POINT('Ctrl Pts',(-0.962030544502803,25.3979126089155,
0.));
#245505=CARTESIAN_POINT('Ctrl Pts',(-0.95050714859697,25.4222289223155,
0.));
#245506=CARTESIAN_POINT('Ctrl Pts',(-0.938896449495633,25.4465852044835,
0.));
#245507=CARTESIAN_POINT('Ctrl Pts',(-0.927198419885605,25.4709809474996,
0.));
#245508=CARTESIAN_POINT('Ctrl Pts',(-0.915413034335334,25.4954156541787,
0.));
#245509=CARTESIAN_POINT('Ctrl Pts',(-0.903540269651155,25.5198888424195,
0.));
#245510=CARTESIAN_POINT('Ctrl Pts',(-0.891580105349468,25.5444000508223,
0.));
#245511=CARTESIAN_POINT('Ctrl Pts',(-0.879532523835092,25.568948840818,
0.));
#245512=CARTESIAN_POINT('Ctrl Pts',(-0.86739750933947,25.5935347843616,
0.));
#245513=CARTESIAN_POINT('Ctrl Pts',(-0.855175047037615,25.618157453608,
0.));
#245514=CARTESIAN_POINT('Ctrl Pts',(-0.842865122121547,25.6428164100078,
0.));
#245515=CARTESIAN_POINT('Ctrl Pts',(-0.830467718864369,25.6675111931957,
0.));
#245516=CARTESIAN_POINT('Ctrl Pts',(-0.81798281978672,25.6922413110172,
0.));
#245517=CARTESIAN_POINT('Ctrl Pts',(-0.805410404552596,25.7170062262474,
0.));
#245518=CARTESIAN_POINT('Ctrl Pts',(-0.792750451613536,25.7418053757671,
0.));
#245519=CARTESIAN_POINT('Ctrl Pts',(-0.780002940289027,25.7666381946871,
0.));
#245520=CARTESIAN_POINT('Ctrl Pts',(-0.767167852648641,25.7915041383304,
0.));
#245521=CARTESIAN_POINT('Ctrl Pts',(-0.75424517560829,25.816402705995,0.));
#245522=CARTESIAN_POINT('Ctrl Pts',(-0.741234902664698,25.841333461908,
0.));
#245523=CARTESIAN_POINT('Ctrl Pts',(-0.728137036485879,25.8662960624285,
0.));
#245524=CARTESIAN_POINT('Ctrl Pts',(-0.714951588533753,25.8912902615141,
0.));
#245525=CARTESIAN_POINT('Ctrl Pts',(-0.701678575236603,25.9163158909645,
0.));
#245526=CARTESIAN_POINT('Ctrl Pts',(-0.688318015065679,25.941372847213,
0.));
#245527=CARTESIAN_POINT('Ctrl Pts',(-0.677559543215903,25.9614434298092,
0.));
#245528=CARTESIAN_POINT('Ctrl Pts',(-0.669451306784418,25.9765104298171,
0.));
#245529=CARTESIAN_POINT('Ctrl Pts',(-0.664028313188914,25.9865613464809,
0.));
#245530=CARTESIAN_POINT('Ctrl Pts',(-0.661312440730891,25.991588367311,
0.));
#245531=CARTESIAN_POINT('',(-0.661312440730891,25.991588367311,12.));
#245532=CARTESIAN_POINT('Ctrl Pts',(-0.661312440730891,25.991588367311,
12.));
#245533=CARTESIAN_POINT('Ctrl Pts',(-0.664028313188914,25.9865613464809,
12.));
#245534=CARTESIAN_POINT('Ctrl Pts',(-0.669451306784418,25.9765104298171,
12.));
#245535=CARTESIAN_POINT('Ctrl Pts',(-0.677559543215903,25.9614434298092,
12.));
#245536=CARTESIAN_POINT('Ctrl Pts',(-0.688318015065679,25.941372847213,
12.));
#245537=CARTESIAN_POINT('Ctrl Pts',(-0.701678575236603,25.9163158909645,
12.));
#245538=CARTESIAN_POINT('Ctrl Pts',(-0.714951588533753,25.8912902615141,
12.));
#245539=CARTESIAN_POINT('Ctrl Pts',(-0.728137036485879,25.8662960624285,
12.));
#245540=CARTESIAN_POINT('Ctrl Pts',(-0.741234902664698,25.841333461908,
12.));
#245541=CARTESIAN_POINT('Ctrl Pts',(-0.75424517560829,25.816402705995,12.));
#245542=CARTESIAN_POINT('Ctrl Pts',(-0.767167852648641,25.7915041383304,
12.));
#245543=CARTESIAN_POINT('Ctrl Pts',(-0.780002940289027,25.7666381946871,
12.));
#245544=CARTESIAN_POINT('Ctrl Pts',(-0.792750451613536,25.7418053757671,
12.));
#245545=CARTESIAN_POINT('Ctrl Pts',(-0.805410404552596,25.7170062262474,
12.));
#245546=CARTESIAN_POINT('Ctrl Pts',(-0.81798281978672,25.6922413110172,
12.));
#245547=CARTESIAN_POINT('Ctrl Pts',(-0.830467718864369,25.6675111931957,
12.));
#245548=CARTESIAN_POINT('Ctrl Pts',(-0.842865122121547,25.6428164100078,
12.));
#245549=CARTESIAN_POINT('Ctrl Pts',(-0.855175047037615,25.618157453608,
12.));
#245550=CARTESIAN_POINT('Ctrl Pts',(-0.86739750933947,25.5935347843616,
12.));
#245551=CARTESIAN_POINT('Ctrl Pts',(-0.879532523835092,25.568948840818,
12.));
#245552=CARTESIAN_POINT('Ctrl Pts',(-0.891580105349468,25.5444000508223,
12.));
#245553=CARTESIAN_POINT('Ctrl Pts',(-0.903540269651155,25.5198888424195,
12.));
#245554=CARTESIAN_POINT('Ctrl Pts',(-0.915413034335334,25.4954156541787,
12.));
#245555=CARTESIAN_POINT('Ctrl Pts',(-0.927198419885605,25.4709809474996,
12.));
#245556=CARTESIAN_POINT('Ctrl Pts',(-0.938896449495633,25.4465852044835,
12.));
#245557=CARTESIAN_POINT('Ctrl Pts',(-0.95050714859697,25.4222289223155,
12.));
#245558=CARTESIAN_POINT('Ctrl Pts',(-0.962030544502803,25.3979126089155,
12.));
#245559=CARTESIAN_POINT('Ctrl Pts',(-0.973466666000049,25.3736367778842,
12.));
#245560=CARTESIAN_POINT('Ctrl Pts',(-0.984815543004092,25.3494019441444,
12.));
#245561=CARTESIAN_POINT('Ctrl Pts',(-0.99607720612092,25.3252086182976,
12.));
#245562=CARTESIAN_POINT('Ctrl Pts',(-1.00725168656934,25.3010573055557,
12.));
#245563=CARTESIAN_POINT('Ctrl Pts',(-1.01833901642272,25.2769485087268,
12.));
#245564=CARTESIAN_POINT('Ctrl Pts',(-1.0293392287683,25.2528827300427,12.));
#245565=CARTESIAN_POINT('Ctrl Pts',(-1.04025235791515,25.2288604735087,
12.));
#245566=CARTESIAN_POINT('Ctrl Pts',(-1.05107843957926,25.2048822469027,
12.));
#245567=CARTESIAN_POINT('Ctrl Pts',(-1.06181751111754,25.1809485642191,
12.));
#245568=CARTESIAN_POINT('Ctrl Pts',(-1.0724696116546,25.1570599469311,12.));
#245569=CARTESIAN_POINT('Ctrl Pts',(-1.08303478197174,25.1332169227415,
12.));
#245570=CARTESIAN_POINT('Ctrl Pts',(-1.09351306445299,25.1094200248448,
12.));
#245571=CARTESIAN_POINT('Ctrl Pts',(-1.1039045030174,25.085669790968,12.));
#245572=CARTESIAN_POINT('Ctrl Pts',(-1.1142091430689,25.0619667625336,12.));
#245573=CARTESIAN_POINT('Ctrl Pts',(-1.12442703144455,25.0383114836898,
12.));
#245574=CARTESIAN_POINT('Ctrl Pts',(-1.13455821638536,25.0147045006193,
12.));
#245575=CARTESIAN_POINT('Ctrl Pts',(-1.14460274758206,24.9911463621431,
12.));
#245576=CARTESIAN_POINT('Ctrl Pts',(-1.15456067621894,24.9676376201501,
12.));
#245577=CARTESIAN_POINT('Ctrl Pts',(-1.16443205502852,24.9441788300932,
12.));
#245578=CARTESIAN_POINT('Ctrl Pts',(-1.17421693835039,24.9207705514449,
12.));
#245579=CARTESIAN_POINT('Ctrl Pts',(-1.18391538220098,24.8974133481829,
12.));
#245580=CARTESIAN_POINT('Ctrl Pts',(-1.19352744434059,24.8741077892074,
12.));
#245581=CARTESIAN_POINT('Ctrl Pts',(-1.20305318426015,24.8508544481973,
12.));
#245582=CARTESIAN_POINT('Ctrl Pts',(-1.21249266318205,24.8276539035092,
12.));
#245583=CARTESIAN_POINT('Ctrl Pts',(-1.22184594406526,24.8045067380536,
12.));
#245584=CARTESIAN_POINT('Ctrl Pts',(-1.23111309161843,24.78141353918,12.));
#245585=CARTESIAN_POINT('Ctrl Pts',(-1.24029417231988,24.7583748985439,
12.));
#245586=CARTESIAN_POINT('Ctrl Pts',(-1.24938925444324,24.7353914120012,
12.));
#245587=CARTESIAN_POINT('Ctrl Pts',(-1.25839840807415,24.7124636797895,
12.));
#245588=CARTESIAN_POINT('Ctrl Pts',(-1.26732170513497,24.6895923066837,
12.));
#245589=CARTESIAN_POINT('Ctrl Pts',(-1.2761592194164,24.666777902156,12.));
#245590=CARTESIAN_POINT('Ctrl Pts',(-1.28491102661514,24.6440210805278,
12.));
#245591=CARTESIAN_POINT('Ctrl Pts',(-1.29357720438108,24.6213224611228,
12.));
#245592=CARTESIAN_POINT('Ctrl Pts',(-1.30215783236364,24.5986826684025,
12.));
#245593=CARTESIAN_POINT('Ctrl Pts',(-1.31065299222023,24.576102332018,12.));
#245594=CARTESIAN_POINT('Ctrl Pts',(-1.31906276763669,24.5535820868671,
12.));
#245595=CARTESIAN_POINT('Ctrl Pts',(-1.32738724435326,24.5311225731434,
12.));
#245596=CARTESIAN_POINT('Ctrl Pts',(-1.33562651019684,24.5087244363856,
12.));
#245597=CARTESIAN_POINT('Ctrl Pts',(-1.34378065512335,24.4863883275135,
12.));
#245598=CARTESIAN_POINT('Ctrl Pts',(-1.35184977125645,24.4641149028894,
12.));
#245599=CARTESIAN_POINT('Ctrl Pts',(-1.35983395290624,24.4419048244524,
12.));
#245600=CARTESIAN_POINT('Ctrl Pts',(-1.36773329659954,24.4197587598337,
12.));
#245601=CARTESIAN_POINT('Ctrl Pts',(-1.37554790111608,24.3976773824731,
12.));
#245602=CARTESIAN_POINT('Ctrl Pts',(-1.38327786752998,24.37566137173,12.));
#245603=CARTESIAN_POINT('Ctrl Pts',(-1.3909232992639,24.3537114129877,12.));
#245604=CARTESIAN_POINT('Ctrl Pts',(-1.3984843021281,24.3318281977647,12.));
#245605=CARTESIAN_POINT('Ctrl Pts',(-1.40596098434341,24.3100124238316,
12.));
#245606=CARTESIAN_POINT('Ctrl Pts',(-1.41335345657685,24.2882647953214,
12.));
#245607=CARTESIAN_POINT('Ctrl Pts',(-1.42066183198252,24.2665860228357,
12.));
#245608=CARTESIAN_POINT('Ctrl Pts',(-1.42788622624851,24.2449768235485,
12.));
#245609=CARTESIAN_POINT('Ctrl Pts',(-1.43502675765502,24.2234379212978,
12.));
#245610=CARTESIAN_POINT('Ctrl Pts',(-1.44208354711074,24.2019700467214,
12.));
#245611=CARTESIAN_POINT('Ctrl Pts',(-1.44905671818721,24.1805739374033,
12.));
#245612=CARTESIAN_POINT('Ctrl Pts',(-1.45594639716314,24.1592503380105,
12.));
#245613=CARTESIAN_POINT('Ctrl Pts',(-1.46275271307398,24.1380000004272,
12.));
#245614=CARTESIAN_POINT('Ctrl Pts',(-1.46947579776992,24.1168236838827,
12.));
#245615=CARTESIAN_POINT('Ctrl Pts',(-1.47611578597741,24.0957221550782,
12.));
#245616=CARTESIAN_POINT('Ctrl Pts',(-1.4826728153368,24.074696188353,12.));
#245617=CARTESIAN_POINT('Ctrl Pts',(-1.48914702644883,24.053746565843,12.));
#245618=CARTESIAN_POINT('Ctrl Pts',(-1.49553856292798,24.0328740776331,
12.));
#245619=CARTESIAN_POINT('Ctrl Pts',(-1.50184757146099,24.0120795219086,
12.));
#245620=CARTESIAN_POINT('Ctrl Pts',(-1.50807420187703,23.991363705093,12.));
#245621=CARTESIAN_POINT('Ctrl Pts',(-1.51421860720628,23.9707274420145,
12.));
#245622=CARTESIAN_POINT('Ctrl Pts',(-1.52028094372806,23.9501715561038,
12.));
#245623=CARTESIAN_POINT('Ctrl Pts',(-1.5262613710304,23.9296968795761,12.));
#245624=CARTESIAN_POINT('Ctrl Pts',(-1.53216005207462,23.9093042536119,
12.));
#245625=CARTESIAN_POINT('Ctrl Pts',(-1.53797715326748,23.8889945285313,
12.));
#245626=CARTESIAN_POINT('Ctrl Pts',(-1.54371284453978,23.8687685639635,
12.));
#245627=CARTESIAN_POINT('Ctrl Pts',(-1.5493672994053,23.8486272290698,12.));
#245628=CARTESIAN_POINT('Ctrl Pts',(-1.55494069502628,23.8285714027631,
12.));
#245629=CARTESIAN_POINT('Ctrl Pts',(-1.56043321228631,23.8086019739192,
12.));
#245630=CARTESIAN_POINT('Ctrl Pts',(-1.56584503586844,23.788719841588,12.));
#245631=CARTESIAN_POINT('Ctrl Pts',(-1.57117635434412,23.7689259151869,
12.));
#245632=CARTESIAN_POINT('Ctrl Pts',(-1.57642736025251,23.7492211147369,
12.));
#245633=CARTESIAN_POINT('Ctrl Pts',(-1.58159825017362,23.7296063711308,
12.));
#245634=CARTESIAN_POINT('Ctrl Pts',(-1.58668922481222,23.7100826263835,
12.));
#245635=CARTESIAN_POINT('Ctrl Pts',(-1.59170048908632,23.6906508338833,
12.));
#245636=CARTESIAN_POINT('Ctrl Pts',(-1.59663225222458,23.6713119586302,
12.));
#245637=CARTESIAN_POINT('Ctrl Pts',(-1.60148472786588,23.6520669774863,
12.));
#245638=CARTESIAN_POINT('Ctrl Pts',(-1.60625813414666,23.6329168794916,
12.));
#245639=CARTESIAN_POINT('Ctrl Pts',(-1.61095269379773,23.6138626661644,
12.));
#245640=CARTESIAN_POINT('Ctrl Pts',(-1.61556863424697,23.5949053517996,
12.));
#245641=CARTESIAN_POINT('Ctrl Pts',(-1.62010618772869,23.5760459637608,
12.));
#245642=CARTESIAN_POINT('Ctrl Pts',(-1.62456559140072,23.5572855427617,
12.));
#245643=CARTESIAN_POINT('Ctrl Pts',(-1.62894708745231,23.5386251432278,
12.));
#245644=CARTESIAN_POINT('Ctrl Pts',(-1.63325092321731,23.5200658336624,
12.));
#245645=CARTESIAN_POINT('Ctrl Pts',(-1.63747735129474,23.5016086970006,
12.));
#245646=CARTESIAN_POINT('Ctrl Pts',(-1.64162662967525,23.4832548309638,
12.));
#245647=CARTESIAN_POINT('Ctrl Pts',(-1.64569902187608,23.4650053483919,
12.));
#245648=CARTESIAN_POINT('Ctrl Pts',(-1.6496947970734,23.446861377656,12.));
#245649=CARTESIAN_POINT('Ctrl Pts',(-1.6536142302373,23.4288240631034,12.));
#245650=CARTESIAN_POINT('Ctrl Pts',(-1.65745760227507,23.4108945654803,
12.));
#245651=CARTESIAN_POINT('Ctrl Pts',(-1.66122520018008,23.3930740623622,
12.));
#245652=CARTESIAN_POINT('Ctrl Pts',(-1.66491731718864,23.375363748555,12.));
#245653=CARTESIAN_POINT('Ctrl Pts',(-1.66853425293978,23.3577648365747,
12.));
#245654=CARTESIAN_POINT('Ctrl Pts',(-1.67207631363905,23.3402785571866,
12.));
#245655=CARTESIAN_POINT('Ctrl Pts',(-1.67554381222987,23.3229061599145,
12.));
#245656=CARTESIAN_POINT('Ctrl Pts',(-1.67893706857123,23.3056489135611,
12.));
#245657=CARTESIAN_POINT('Ctrl Pts',(-1.68225640962181,23.2885081066949,
12.));
#245658=CARTESIAN_POINT('Ctrl Pts',(-1.68550216963275,23.2714850482245,
12.));
#245659=CARTESIAN_POINT('Ctrl Pts',(-1.6886746903491,23.2545810680536,12.));
#245660=CARTESIAN_POINT('Ctrl Pts',(-1.69177432121716,23.2377975177014,
12.));
#245661=CARTESIAN_POINT('Ctrl Pts',(-1.69480141959946,23.2211357709374,
12.));
#245662=CARTESIAN_POINT('Ctrl Pts',(-1.69775635099425,23.2045972243765,
12.));
#245663=CARTESIAN_POINT('Ctrl Pts',(-1.70063948926987,23.1881832981848,
12.));
#245664=CARTESIAN_POINT('Ctrl Pts',(-1.70345121691259,23.1718954368749,
12.));
#245665=CARTESIAN_POINT('Ctrl Pts',(-1.70619192527847,23.1557351100613,
12.));
#245666=CARTESIAN_POINT('Ctrl Pts',(-1.7088620148546,23.1397038132358,12.));
#245667=CARTESIAN_POINT('Ctrl Pts',(-1.71146189552192,23.1238030684929,
12.));
#245668=CARTESIAN_POINT('Ctrl Pts',(-1.71399198684725,23.1080344254291,
12.));
#245669=CARTESIAN_POINT('Ctrl Pts',(-1.71645271839311,23.0923994621216,
12.));
#245670=CARTESIAN_POINT('Ctrl Pts',(-1.71884453003027,23.0768997860709,
12.));
#245671=CARTESIAN_POINT('Ctrl Pts',(-1.7211678722598,23.061537035156,12.));
#245672=CARTESIAN_POINT('Ctrl Pts',(-1.72342320653731,23.0463128785528,
12.));
#245673=CARTESIAN_POINT('Ctrl Pts',(-1.72561100564033,23.031229017888,12.));
#245674=CARTESIAN_POINT('Ctrl Pts',(-1.72773175404703,23.0162871884167,
12.));
#245675=CARTESIAN_POINT('Ctrl Pts',(-1.72978594832137,23.0014891601891,
12.));
#245676=CARTESIAN_POINT('Ctrl Pts',(-1.73177409750194,22.9868367391978,
12.));
#245677=CARTESIAN_POINT('Ctrl Pts',(-1.73369672350818,22.9723317685688,
12.));
#245678=CARTESIAN_POINT('Ctrl Pts',(-1.73555436162771,22.9579761301062,
12.));
#245679=CARTESIAN_POINT('Ctrl Pts',(-1.73734756100038,22.9437717457825,
12.));
#245680=CARTESIAN_POINT('Ctrl Pts',(-1.73907688511664,22.9297205792587,
12.));
#245681=CARTESIAN_POINT('Ctrl Pts',(-1.74074291231057,22.9158246373365,
12.));
#245682=CARTESIAN_POINT('Ctrl Pts',(-1.74234623630079,22.9020859716144,
12.));
#245683=CARTESIAN_POINT('Ctrl Pts',(-1.74388746677702,22.8885066803351,
12.));
#245684=CARTESIAN_POINT('Ctrl Pts',(-1.745367229982,22.8750889101696,12.));
#245685=CARTESIAN_POINT('Ctrl Pts',(-1.74678616930663,22.8618348580234,
12.));
#245686=CARTESIAN_POINT('Ctrl Pts',(-1.74814494588492,22.8487467728075,
12.));
#245687=CARTESIAN_POINT('Ctrl Pts',(-1.74944423940117,22.8358269579854,
12.));
#245688=CARTESIAN_POINT('Ctrl Pts',(-1.75068474890884,22.8230777741285,
12.));
#245689=CARTESIAN_POINT('Ctrl Pts',(-1.7518671936559,22.8105016414712,12.));
#245690=CARTESIAN_POINT('Ctrl Pts',(-1.75299231391461,22.7981010424312,
12.));
#245691=CARTESIAN_POINT('Ctrl Pts',(-1.7540608718293,22.7858785242358,12.));
#245692=CARTESIAN_POINT('Ctrl Pts',(-1.75507365227127,22.7738367016115,
12.));
#245693=CARTESIAN_POINT('Ctrl Pts',(-1.7560314637164,22.7619782595013,12.));
#245694=CARTESIAN_POINT('Ctrl Pts',(-1.75693513908911,22.7503059556455,
12.));
#245695=CARTESIAN_POINT('Ctrl Pts',(-1.75778553673249,22.7388226235565,
12.));
#245696=CARTESIAN_POINT('Ctrl Pts',(-1.75858354204635,22.7275311777305,
12.));
#245697=CARTESIAN_POINT('Ctrl Pts',(-1.75933006905924,22.7164346186007,
12.));
#245698=CARTESIAN_POINT('Ctrl Pts',(-1.76002606202399,22.7055360375481,
12.));
#245699=CARTESIAN_POINT('Ctrl Pts',(-1.76067249704884,22.6948386219843,
12.));
#245700=CARTESIAN_POINT('Ctrl Pts',(-1.76127038310613,22.6843456585245,
12.));
#245701=CARTESIAN_POINT('Ctrl Pts',(-1.76182076289525,22.6740605356699,
12.));
#245702=CARTESIAN_POINT('Ctrl Pts',(-1.76232471392567,22.6639867471756,
12.));
#245703=CARTESIAN_POINT('Ctrl Pts',(-1.76278334912559,22.6541278938413,
12.));
#245704=CARTESIAN_POINT('Ctrl Pts',(-1.76319782013914,22.6444876940425,
12.));
#245705=CARTESIAN_POINT('Ctrl Pts',(-1.76356932176272,22.635069997936,12.));
#245706=CARTESIAN_POINT('Ctrl Pts',(-1.76389909571402,22.6258787994847,
12.));
#245707=CARTESIAN_POINT('Ctrl Pts',(-1.76418843543739,22.6169182517693,
12.));
#245708=CARTESIAN_POINT('Ctrl Pts',(-1.76443868648015,22.6081926681342,
12.));
#245709=CARTESIAN_POINT('Ctrl Pts',(-1.76465124413556,22.5997065145638,
12.));
#245710=CARTESIAN_POINT('Ctrl Pts',(-1.76482755288411,22.5914644078106,
12.));
#245711=CARTESIAN_POINT('Ctrl Pts',(-1.76496910283088,22.5834711038024,
12.));
#245712=CARTESIAN_POINT('Ctrl Pts',(-1.76507744026747,22.5757315316355,
12.));
#245713=CARTESIAN_POINT('Ctrl Pts',(-1.76515418518829,22.5682508499873,
12.));
#245714=CARTESIAN_POINT('Ctrl Pts',(-1.76520104500449,22.5610344912501,
12.));
#245715=CARTESIAN_POINT('Ctrl Pts',(-1.76521983384063,22.5540882235837,
12.));
#245716=CARTESIAN_POINT('Ctrl Pts',(-1.76521245524047,22.5474180954006,
12.));
#245717=CARTESIAN_POINT('Ctrl Pts',(-1.76518087841493,22.5410303590891,
12.));
#245718=CARTESIAN_POINT('Ctrl Pts',(-1.7651271156325,22.5349313983571,12.));
#245719=CARTESIAN_POINT('Ctrl Pts',(-1.76505320262752,22.529127665298,12.));
#245720=CARTESIAN_POINT('Ctrl Pts',(-1.76496128643369,22.5236259635515,
12.));
#245721=CARTESIAN_POINT('Ctrl Pts',(-1.76485369319896,22.5184336670207,
12.));
#245722=CARTESIAN_POINT('Ctrl Pts',(-1.76473303281159,22.5135590569554,
12.));
#245723=CARTESIAN_POINT('Ctrl Pts',(-1.76460218257323,22.5090112700212,
12.));
#245724=CARTESIAN_POINT('Ctrl Pts',(-1.76446408210366,22.5047996391978,
12.));
#245725=CARTESIAN_POINT('Ctrl Pts',(-1.76432160068725,22.5009332677316,
12.));
#245726=CARTESIAN_POINT('Ctrl Pts',(-1.76417731243462,22.4974203063191,
12.));
#245727=CARTESIAN_POINT('Ctrl Pts',(-1.76403393880301,22.4942693792449,
12.));
#245728=CARTESIAN_POINT('Ctrl Pts',(-1.76389475965724,22.4914909094908,
12.));
#245729=CARTESIAN_POINT('Ctrl Pts',(-1.76376424879505,22.4890991659478,
12.));
#245730=CARTESIAN_POINT('Ctrl Pts',(-1.76364784232963,22.4871115206571,
12.));
#245731=CARTESIAN_POINT('Ctrl Pts',(-1.76355076045546,22.4855446605991,
12.));
#245732=CARTESIAN_POINT('Ctrl Pts',(-1.76347698284792,22.4844112933129,
12.));
#245733=CARTESIAN_POINT('Ctrl Pts',(-1.76343813434565,22.483856251707,12.));
#245734=CARTESIAN_POINT('Ctrl Pts',(-1.7634206426357,22.4836387052232,12.));
#245735=CARTESIAN_POINT('Ctrl Pts',(-1.76341415538764,22.483581992979,12.));
#245736=CARTESIAN_POINT('Ctrl Pts',(-1.76341220531179,22.4835757167854,
12.));
#245737=CARTESIAN_POINT('',(-0.661312440730891,25.991588367311,0.));
#245738=CARTESIAN_POINT('Origin',(3.92374859571501,21.1389261070099,0.));
#245739=CARTESIAN_POINT('',(4.11585220600461,22.1738711152697,12.));
#245740=CARTESIAN_POINT('',(1.96187429785751,10.5694630535049,12.));
#245741=CARTESIAN_POINT('',(4.11585220600461,22.1738711152697,0.));
#245742=CARTESIAN_POINT('',(4.11585220600461,22.1738711152697,0.));
#245743=CARTESIAN_POINT('',(1.96187429785751,10.5694630535049,0.));
#245744=CARTESIAN_POINT('Ctrl Pts',(0.661312440730901,25.991588367311,0.));
#245745=CARTESIAN_POINT('Ctrl Pts',(0.661312440730901,25.991588367311,12.));
#245746=CARTESIAN_POINT('Ctrl Pts',(0.664028313187627,25.9865613464773,
0.));
#245747=CARTESIAN_POINT('Ctrl Pts',(0.664028313187627,25.9865613464773,
12.));
#245748=CARTESIAN_POINT('Ctrl Pts',(0.669451306780825,25.9765104298071,
0.));
#245749=CARTESIAN_POINT('Ctrl Pts',(0.669451306780825,25.9765104298071,
12.));
#245750=CARTESIAN_POINT('Ctrl Pts',(0.677559543209725,25.9614434297919,
0.));
#245751=CARTESIAN_POINT('Ctrl Pts',(0.677559543209725,25.9614434297919,
12.));
#245752=CARTESIAN_POINT('Ctrl Pts',(0.688318015057729,25.9413728471909,
0.));
#245753=CARTESIAN_POINT('Ctrl Pts',(0.688318015057729,25.9413728471909,
12.));
#245754=CARTESIAN_POINT('Ctrl Pts',(0.701678575228756,25.9163158909426,
0.));
#245755=CARTESIAN_POINT('Ctrl Pts',(0.701678575228756,25.9163158909426,
12.));
#245756=CARTESIAN_POINT('Ctrl Pts',(0.714951588527638,25.891290261497,0.));
#245757=CARTESIAN_POINT('Ctrl Pts',(0.714951588527638,25.891290261497,12.));
#245758=CARTESIAN_POINT('Ctrl Pts',(0.728137036482335,25.8662960624185,
0.));
#245759=CARTESIAN_POINT('Ctrl Pts',(0.728137036482335,25.8662960624185,
12.));
#245760=CARTESIAN_POINT('Ctrl Pts',(0.741234902663807,25.8413334619055,
0.));
#245761=CARTESIAN_POINT('Ctrl Pts',(0.741234902663807,25.8413334619055,
12.));
#245762=CARTESIAN_POINT('Ctrl Pts',(0.754245175609524,25.8164027059984,
0.));
#245763=CARTESIAN_POINT('Ctrl Pts',(0.754245175609524,25.8164027059984,
12.));
#245764=CARTESIAN_POINT('Ctrl Pts',(0.767167852651168,25.7915041383376,
0.));
#245765=CARTESIAN_POINT('Ctrl Pts',(0.767167852651168,25.7915041383376,
12.));
#245766=CARTESIAN_POINT('Ctrl Pts',(0.780002940291965,25.7666381946955,
0.));
#245767=CARTESIAN_POINT('Ctrl Pts',(0.780002940291965,25.7666381946955,
12.));
#245768=CARTESIAN_POINT('Ctrl Pts',(0.792750451616127,25.7418053757746,
0.));
#245769=CARTESIAN_POINT('Ctrl Pts',(0.792750451616127,25.7418053757746,
12.));
#245770=CARTESIAN_POINT('Ctrl Pts',(0.805410404554352,25.7170062262525,
0.));
#245771=CARTESIAN_POINT('Ctrl Pts',(0.805410404554352,25.7170062262525,
12.));
#245772=CARTESIAN_POINT('Ctrl Pts',(0.817982819787464,25.6922413110194,
0.));
#245773=CARTESIAN_POINT('Ctrl Pts',(0.817982819787464,25.6922413110194,
12.));
#245774=CARTESIAN_POINT('Ctrl Pts',(0.830467718864205,25.6675111931952,
0.));
#245775=CARTESIAN_POINT('Ctrl Pts',(0.830467718864205,25.6675111931952,
12.));
#245776=CARTESIAN_POINT('Ctrl Pts',(0.842865122120758,25.6428164100055,
0.));
#245777=CARTESIAN_POINT('Ctrl Pts',(0.842865122120758,25.6428164100055,
12.));
#245778=CARTESIAN_POINT('Ctrl Pts',(0.855175047036549,25.6181574536049,
0.));
#245779=CARTESIAN_POINT('Ctrl Pts',(0.855175047036549,25.6181574536049,
12.));
#245780=CARTESIAN_POINT('Ctrl Pts',(0.867397509338431,25.5935347843585,
0.));
#245781=CARTESIAN_POINT('Ctrl Pts',(0.867397509338431,25.5935347843585,
12.));
#245782=CARTESIAN_POINT('Ctrl Pts',(0.879532523834294,25.5689488408156,
0.));
#245783=CARTESIAN_POINT('Ctrl Pts',(0.879532523834294,25.5689488408156,
12.));
#245784=CARTESIAN_POINT('Ctrl Pts',(0.89158010534904,25.5444000508211,0.));
#245785=CARTESIAN_POINT('Ctrl Pts',(0.89158010534904,25.5444000508211,12.));
#245786=CARTESIAN_POINT('Ctrl Pts',(0.903540269651106,25.5198888424194,
0.));
#245787=CARTESIAN_POINT('Ctrl Pts',(0.903540269651106,25.5198888424194,
12.));
#245788=CARTESIAN_POINT('Ctrl Pts',(0.915413034335613,25.4954156541795,
0.));
#245789=CARTESIAN_POINT('Ctrl Pts',(0.915413034335613,25.4954156541795,
12.));
#245790=CARTESIAN_POINT('Ctrl Pts',(0.927198419886094,25.4709809475009,
0.));
#245791=CARTESIAN_POINT('Ctrl Pts',(0.927198419886094,25.4709809475009,
12.));
#245792=CARTESIAN_POINT('Ctrl Pts',(0.938896449496192,25.4465852044849,
0.));
#245793=CARTESIAN_POINT('Ctrl Pts',(0.938896449496192,25.4465852044849,
12.));
#245794=CARTESIAN_POINT('Ctrl Pts',(0.950507148597468,25.4222289223167,
0.));
#245795=CARTESIAN_POINT('Ctrl Pts',(0.950507148597468,25.4222289223167,
12.));
#245796=CARTESIAN_POINT('Ctrl Pts',(0.962030544503142,25.3979126089163,
0.));
#245797=CARTESIAN_POINT('Ctrl Pts',(0.962030544503142,25.3979126089163,
12.));
#245798=CARTESIAN_POINT('Ctrl Pts',(0.973466666000163,25.3736367778845,
0.));
#245799=CARTESIAN_POINT('Ctrl Pts',(0.973466666000163,25.3736367778845,
12.));
#245800=CARTESIAN_POINT('Ctrl Pts',(0.984815543003973,25.3494019441441,
0.));
#245801=CARTESIAN_POINT('Ctrl Pts',(0.984815543003973,25.3494019441441,
12.));
#245802=CARTESIAN_POINT('Ctrl Pts',(0.996077206120624,25.3252086182968,
0.));
#245803=CARTESIAN_POINT('Ctrl Pts',(0.996077206120624,25.3252086182968,
12.));
#245804=CARTESIAN_POINT('Ctrl Pts',(1.00725168656896,25.3010573055547,0.));
#245805=CARTESIAN_POINT('Ctrl Pts',(1.00725168656896,25.3010573055547,12.));
#245806=CARTESIAN_POINT('Ctrl Pts',(1.01833901642237,25.276948508726,0.));
#245807=CARTESIAN_POINT('Ctrl Pts',(1.01833901642237,25.276948508726,12.));
#245808=CARTESIAN_POINT('Ctrl Pts',(1.02933922876806,25.2528827300422,0.));
#245809=CARTESIAN_POINT('Ctrl Pts',(1.02933922876806,25.2528827300422,12.));
#245810=CARTESIAN_POINT('Ctrl Pts',(1.04025235791507,25.2288604735086,0.));
#245811=CARTESIAN_POINT('Ctrl Pts',(1.04025235791507,25.2288604735086,12.));
#245812=CARTESIAN_POINT('Ctrl Pts',(1.05107843957931,25.2048822469028,0.));
#245813=CARTESIAN_POINT('Ctrl Pts',(1.05107843957931,25.2048822469028,12.));
#245814=CARTESIAN_POINT('Ctrl Pts',(1.06181751111768,25.1809485642192,0.));
#245815=CARTESIAN_POINT('Ctrl Pts',(1.06181751111768,25.1809485642192,12.));
#245816=CARTESIAN_POINT('Ctrl Pts',(1.07246961165475,25.157059946931,0.));
#245817=CARTESIAN_POINT('Ctrl Pts',(1.07246961165475,25.157059946931,12.));
#245818=CARTESIAN_POINT('Ctrl Pts',(1.08303478197187,25.1332169227413,0.));
#245819=CARTESIAN_POINT('Ctrl Pts',(1.08303478197187,25.1332169227413,12.));
#245820=CARTESIAN_POINT('Ctrl Pts',(1.09351306445308,25.1094200248446,0.));
#245821=CARTESIAN_POINT('Ctrl Pts',(1.09351306445308,25.1094200248446,12.));
#245822=CARTESIAN_POINT('Ctrl Pts',(1.10390450301745,25.0856697909679,0.));
#245823=CARTESIAN_POINT('Ctrl Pts',(1.10390450301745,25.0856697909679,12.));
#245824=CARTESIAN_POINT('Ctrl Pts',(1.11420914306889,25.0619667625336,0.));
#245825=CARTESIAN_POINT('Ctrl Pts',(1.11420914306889,25.0619667625336,12.));
#245826=CARTESIAN_POINT('Ctrl Pts',(1.12442703144451,25.0383114836899,0.));
#245827=CARTESIAN_POINT('Ctrl Pts',(1.12442703144451,25.0383114836899,12.));
#245828=CARTESIAN_POINT('Ctrl Pts',(1.1345582163853,25.0147045006196,0.));
#245829=CARTESIAN_POINT('Ctrl Pts',(1.1345582163853,25.0147045006196,12.));
#245830=CARTESIAN_POINT('Ctrl Pts',(1.144602747582,24.9911463621433,0.));
#245831=CARTESIAN_POINT('Ctrl Pts',(1.144602747582,24.9911463621433,12.));
#245832=CARTESIAN_POINT('Ctrl Pts',(1.15456067621889,24.9676376201502,0.));
#245833=CARTESIAN_POINT('Ctrl Pts',(1.15456067621889,24.9676376201502,12.));
#245834=CARTESIAN_POINT('Ctrl Pts',(1.16443205502849,24.9441788300932,0.));
#245835=CARTESIAN_POINT('Ctrl Pts',(1.16443205502849,24.9441788300932,12.));
#245836=CARTESIAN_POINT('Ctrl Pts',(1.17421693835041,24.9207705514449,0.));
#245837=CARTESIAN_POINT('Ctrl Pts',(1.17421693835041,24.9207705514449,12.));
#245838=CARTESIAN_POINT('Ctrl Pts',(1.18391538220103,24.8974133481829,0.));
#245839=CARTESIAN_POINT('Ctrl Pts',(1.18391538220103,24.8974133481829,12.));
#245840=CARTESIAN_POINT('Ctrl Pts',(1.19352744434064,24.8741077892075,0.));
#245841=CARTESIAN_POINT('Ctrl Pts',(1.19352744434064,24.8741077892075,12.));
#245842=CARTESIAN_POINT('Ctrl Pts',(1.2030531842602,24.8508544481974,0.));
#245843=CARTESIAN_POINT('Ctrl Pts',(1.2030531842602,24.8508544481974,12.));
#245844=CARTESIAN_POINT('Ctrl Pts',(1.21249266318208,24.8276539035092,0.));
#245845=CARTESIAN_POINT('Ctrl Pts',(1.21249266318208,24.8276539035092,12.));
#245846=CARTESIAN_POINT('Ctrl Pts',(1.22184594406528,24.8045067380536,0.));
#245847=CARTESIAN_POINT('Ctrl Pts',(1.22184594406528,24.8045067380536,12.));
#245848=CARTESIAN_POINT('Ctrl Pts',(1.23111309161843,24.7814135391799,0.));
#245849=CARTESIAN_POINT('Ctrl Pts',(1.23111309161843,24.7814135391799,12.));
#245850=CARTESIAN_POINT('Ctrl Pts',(1.24029417231989,24.7583748985438,0.));
#245851=CARTESIAN_POINT('Ctrl Pts',(1.24029417231989,24.7583748985438,12.));
#245852=CARTESIAN_POINT('Ctrl Pts',(1.24938925444325,24.7353914120011,0.));
#245853=CARTESIAN_POINT('Ctrl Pts',(1.24938925444325,24.7353914120011,12.));
#245854=CARTESIAN_POINT('Ctrl Pts',(1.25839840807418,24.7124636797894,0.));
#245855=CARTESIAN_POINT('Ctrl Pts',(1.25839840807418,24.7124636797894,12.));
#245856=CARTESIAN_POINT('Ctrl Pts',(1.267321705135,24.6895923066836,0.));
#245857=CARTESIAN_POINT('Ctrl Pts',(1.267321705135,24.6895923066836,12.));
#245858=CARTESIAN_POINT('Ctrl Pts',(1.27615921941642,24.666777902156,0.));
#245859=CARTESIAN_POINT('Ctrl Pts',(1.27615921941642,24.666777902156,12.));
#245860=CARTESIAN_POINT('Ctrl Pts',(1.28491102661514,24.6440210805278,0.));
#245861=CARTESIAN_POINT('Ctrl Pts',(1.28491102661514,24.6440210805278,12.));
#245862=CARTESIAN_POINT('Ctrl Pts',(1.29357720438107,24.6213224611229,0.));
#245863=CARTESIAN_POINT('Ctrl Pts',(1.29357720438107,24.6213224611229,12.));
#245864=CARTESIAN_POINT('Ctrl Pts',(1.30215783236362,24.5986826684027,0.));
#245865=CARTESIAN_POINT('Ctrl Pts',(1.30215783236362,24.5986826684027,12.));
#245866=CARTESIAN_POINT('Ctrl Pts',(1.31065299222021,24.5761023320183,0.));
#245867=CARTESIAN_POINT('Ctrl Pts',(1.31065299222021,24.5761023320183,12.));
#245868=CARTESIAN_POINT('Ctrl Pts',(1.31906276763668,24.5535820868674,0.));
#245869=CARTESIAN_POINT('Ctrl Pts',(1.31906276763668,24.5535820868674,12.));
#245870=CARTESIAN_POINT('Ctrl Pts',(1.32738724435326,24.5311225731435,0.));
#245871=CARTESIAN_POINT('Ctrl Pts',(1.32738724435326,24.5311225731435,12.));
#245872=CARTESIAN_POINT('Ctrl Pts',(1.33562651019686,24.5087244363856,0.));
#245873=CARTESIAN_POINT('Ctrl Pts',(1.33562651019686,24.5087244363856,12.));
#245874=CARTESIAN_POINT('Ctrl Pts',(1.34378065512337,24.4863883275134,0.));
#245875=CARTESIAN_POINT('Ctrl Pts',(1.34378065512337,24.4863883275134,12.));
#245876=CARTESIAN_POINT('Ctrl Pts',(1.35184977125648,24.4641149028892,0.));
#245877=CARTESIAN_POINT('Ctrl Pts',(1.35184977125648,24.4641149028892,12.));
#245878=CARTESIAN_POINT('Ctrl Pts',(1.35983395290627,24.4419048244523,0.));
#245879=CARTESIAN_POINT('Ctrl Pts',(1.35983395290627,24.4419048244523,12.));
#245880=CARTESIAN_POINT('Ctrl Pts',(1.36773329659956,24.4197587598337,0.));
#245881=CARTESIAN_POINT('Ctrl Pts',(1.36773329659956,24.4197587598337,12.));
#245882=CARTESIAN_POINT('Ctrl Pts',(1.37554790111609,24.3976773824732,0.));
#245883=CARTESIAN_POINT('Ctrl Pts',(1.37554790111609,24.3976773824732,12.));
#245884=CARTESIAN_POINT('Ctrl Pts',(1.38327786752998,24.3756613717299,0.));
#245885=CARTESIAN_POINT('Ctrl Pts',(1.38327786752998,24.3756613717299,12.));
#245886=CARTESIAN_POINT('Ctrl Pts',(1.39092329926388,24.3537114129875,0.));
#245887=CARTESIAN_POINT('Ctrl Pts',(1.39092329926388,24.3537114129875,12.));
#245888=CARTESIAN_POINT('Ctrl Pts',(1.39848430212807,24.3318281977643,0.));
#245889=CARTESIAN_POINT('Ctrl Pts',(1.39848430212807,24.3318281977643,12.));
#245890=CARTESIAN_POINT('Ctrl Pts',(1.40596098434337,24.3100124238311,0.));
#245891=CARTESIAN_POINT('Ctrl Pts',(1.40596098434337,24.3100124238311,12.));
#245892=CARTESIAN_POINT('Ctrl Pts',(1.41335345657682,24.288264795321,0.));
#245893=CARTESIAN_POINT('Ctrl Pts',(1.41335345657682,24.288264795321,12.));
#245894=CARTESIAN_POINT('Ctrl Pts',(1.42066183198252,24.2665860228356,0.));
#245895=CARTESIAN_POINT('Ctrl Pts',(1.42066183198252,24.2665860228356,12.));
#245896=CARTESIAN_POINT('Ctrl Pts',(1.42788622624854,24.2449768235488,0.));
#245897=CARTESIAN_POINT('Ctrl Pts',(1.42788622624854,24.2449768235488,12.));
#245898=CARTESIAN_POINT('Ctrl Pts',(1.43502675765508,24.2234379212984,0.));
#245899=CARTESIAN_POINT('Ctrl Pts',(1.43502675765508,24.2234379212984,12.));
#245900=CARTESIAN_POINT('Ctrl Pts',(1.44208354711082,24.201970046722,0.));
#245901=CARTESIAN_POINT('Ctrl Pts',(1.44208354711082,24.201970046722,12.));
#245902=CARTESIAN_POINT('Ctrl Pts',(1.44905671818727,24.1805739374038,0.));
#245903=CARTESIAN_POINT('Ctrl Pts',(1.44905671818727,24.1805739374038,12.));
#245904=CARTESIAN_POINT('Ctrl Pts',(1.45594639716317,24.1592503380107,0.));
#245905=CARTESIAN_POINT('Ctrl Pts',(1.45594639716317,24.1592503380107,12.));
#245906=CARTESIAN_POINT('Ctrl Pts',(1.46275271307397,24.1380000004272,0.));
#245907=CARTESIAN_POINT('Ctrl Pts',(1.46275271307397,24.1380000004272,12.));
#245908=CARTESIAN_POINT('Ctrl Pts',(1.46947579776991,24.1168236838824,0.));
#245909=CARTESIAN_POINT('Ctrl Pts',(1.46947579776991,24.1168236838824,12.));
#245910=CARTESIAN_POINT('Ctrl Pts',(1.47611578597742,24.0957221550778,0.));
#245911=CARTESIAN_POINT('Ctrl Pts',(1.47611578597742,24.0957221550778,12.));
#245912=CARTESIAN_POINT('Ctrl Pts',(1.48267281533683,24.0746961883528,0.));
#245913=CARTESIAN_POINT('Ctrl Pts',(1.48267281533683,24.0746961883528,12.));
#245914=CARTESIAN_POINT('Ctrl Pts',(1.48914702644887,24.0537465658429,0.));
#245915=CARTESIAN_POINT('Ctrl Pts',(1.48914702644887,24.0537465658429,12.));
#245916=CARTESIAN_POINT('Ctrl Pts',(1.49553856292801,24.0328740776331,0.));
#245917=CARTESIAN_POINT('Ctrl Pts',(1.49553856292801,24.0328740776331,12.));
#245918=CARTESIAN_POINT('Ctrl Pts',(1.50184757146098,24.0120795219086,0.));
#245919=CARTESIAN_POINT('Ctrl Pts',(1.50184757146098,24.0120795219086,12.));
#245920=CARTESIAN_POINT('Ctrl Pts',(1.50807420187694,23.9913637050927,0.));
#245921=CARTESIAN_POINT('Ctrl Pts',(1.50807420187694,23.9913637050927,12.));
#245922=CARTESIAN_POINT('Ctrl Pts',(1.51421860720614,23.970727442014,0.));
#245923=CARTESIAN_POINT('Ctrl Pts',(1.51421860720614,23.970727442014,12.));
#245924=CARTESIAN_POINT('Ctrl Pts',(1.52028094372792,23.9501715561033,0.));
#245925=CARTESIAN_POINT('Ctrl Pts',(1.52028094372792,23.9501715561033,12.));
#245926=CARTESIAN_POINT('Ctrl Pts',(1.52626137103032,23.9296968795757,0.));
#245927=CARTESIAN_POINT('Ctrl Pts',(1.52626137103032,23.9296968795757,12.));
#245928=CARTESIAN_POINT('Ctrl Pts',(1.53216005207463,23.9093042536119,0.));
#245929=CARTESIAN_POINT('Ctrl Pts',(1.53216005207463,23.9093042536119,12.));
#245930=CARTESIAN_POINT('Ctrl Pts',(1.53797715326758,23.8889945285318,0.));
#245931=CARTESIAN_POINT('Ctrl Pts',(1.53797715326758,23.8889945285318,12.));
#245932=CARTESIAN_POINT('Ctrl Pts',(1.5437128445399,23.8687685639642,0.));
#245933=CARTESIAN_POINT('Ctrl Pts',(1.5437128445399,23.8687685639642,12.));
#245934=CARTESIAN_POINT('Ctrl Pts',(1.54936729940541,23.8486272290705,0.));
#245935=CARTESIAN_POINT('Ctrl Pts',(1.54936729940541,23.8486272290705,12.));
#245936=CARTESIAN_POINT('Ctrl Pts',(1.55494069502635,23.8285714027636,0.));
#245937=CARTESIAN_POINT('Ctrl Pts',(1.55494069502635,23.8285714027636,12.));
#245938=CARTESIAN_POINT('Ctrl Pts',(1.56043321228633,23.8086019739194,0.));
#245939=CARTESIAN_POINT('Ctrl Pts',(1.56043321228633,23.8086019739194,12.));
#245940=CARTESIAN_POINT('Ctrl Pts',(1.56584503586843,23.7887198415878,0.));
#245941=CARTESIAN_POINT('Ctrl Pts',(1.56584503586843,23.7887198415878,12.));
#245942=CARTESIAN_POINT('Ctrl Pts',(1.57117635434408,23.7689259151862,0.));
#245943=CARTESIAN_POINT('Ctrl Pts',(1.57117635434408,23.7689259151862,12.));
#245944=CARTESIAN_POINT('Ctrl Pts',(1.57642736025246,23.749221114736,0.));
#245945=CARTESIAN_POINT('Ctrl Pts',(1.57642736025246,23.749221114736,12.));
#245946=CARTESIAN_POINT('Ctrl Pts',(1.58159825017358,23.72960637113,0.));
#245947=CARTESIAN_POINT('Ctrl Pts',(1.58159825017358,23.72960637113,12.));
#245948=CARTESIAN_POINT('Ctrl Pts',(1.58668922481221,23.710082626383,0.));
#245949=CARTESIAN_POINT('Ctrl Pts',(1.58668922481221,23.710082626383,12.));
#245950=CARTESIAN_POINT('Ctrl Pts',(1.59170048908633,23.6906508338833,0.));
#245951=CARTESIAN_POINT('Ctrl Pts',(1.59170048908633,23.6906508338833,12.));
#245952=CARTESIAN_POINT('Ctrl Pts',(1.59663225222463,23.671311958631,0.));
#245953=CARTESIAN_POINT('Ctrl Pts',(1.59663225222463,23.671311958631,12.));
#245954=CARTESIAN_POINT('Ctrl Pts',(1.60148472786595,23.6520669774876,0.));
#245955=CARTESIAN_POINT('Ctrl Pts',(1.60148472786595,23.6520669774876,12.));
#245956=CARTESIAN_POINT('Ctrl Pts',(1.60625813414672,23.6329168794929,0.));
#245957=CARTESIAN_POINT('Ctrl Pts',(1.60625813414672,23.6329168794929,12.));
#245958=CARTESIAN_POINT('Ctrl Pts',(1.61095269379778,23.6138626661653,0.));
#245959=CARTESIAN_POINT('Ctrl Pts',(1.61095269379778,23.6138626661653,12.));
#245960=CARTESIAN_POINT('Ctrl Pts',(1.61556863424698,23.5949053517997,0.));
#245961=CARTESIAN_POINT('Ctrl Pts',(1.61556863424698,23.5949053517997,12.));
#245962=CARTESIAN_POINT('Ctrl Pts',(1.62010618772866,23.57604596376,0.));
#245963=CARTESIAN_POINT('Ctrl Pts',(1.62010618772866,23.57604596376,12.));
#245964=CARTESIAN_POINT('Ctrl Pts',(1.62456559140064,23.5572855427601,0.));
#245965=CARTESIAN_POINT('Ctrl Pts',(1.62456559140064,23.5572855427601,12.));
#245966=CARTESIAN_POINT('Ctrl Pts',(1.62894708745223,23.538625143226,0.));
#245967=CARTESIAN_POINT('Ctrl Pts',(1.62894708745223,23.538625143226,12.));
#245968=CARTESIAN_POINT('Ctrl Pts',(1.63325092321725,23.5200658336612,0.));
#245969=CARTESIAN_POINT('Ctrl Pts',(1.63325092321725,23.5200658336612,12.));
#245970=CARTESIAN_POINT('Ctrl Pts',(1.63747735129474,23.5016086970003,0.));
#245971=CARTESIAN_POINT('Ctrl Pts',(1.63747735129474,23.5016086970003,12.));
#245972=CARTESIAN_POINT('Ctrl Pts',(1.64162662967528,23.4832548309645,0.));
#245973=CARTESIAN_POINT('Ctrl Pts',(1.64162662967528,23.4832548309645,12.));
#245974=CARTESIAN_POINT('Ctrl Pts',(1.64569902187611,23.4650053483932,0.));
#245975=CARTESIAN_POINT('Ctrl Pts',(1.64569902187611,23.4650053483932,12.));
#245976=CARTESIAN_POINT('Ctrl Pts',(1.6496947970734,23.4468613776574,0.));
#245977=CARTESIAN_POINT('Ctrl Pts',(1.6496947970734,23.4468613776574,12.));
#245978=CARTESIAN_POINT('Ctrl Pts',(1.65361423023728,23.4288240631043,0.));
#245979=CARTESIAN_POINT('Ctrl Pts',(1.65361423023728,23.4288240631043,12.));
#245980=CARTESIAN_POINT('Ctrl Pts',(1.65745760227505,23.4108945654805,0.));
#245981=CARTESIAN_POINT('Ctrl Pts',(1.65745760227505,23.4108945654805,12.));
#245982=CARTESIAN_POINT('Ctrl Pts',(1.66122520018011,23.3930740623619,0.));
#245983=CARTESIAN_POINT('Ctrl Pts',(1.66122520018011,23.3930740623619,12.));
#245984=CARTESIAN_POINT('Ctrl Pts',(1.66491731718876,23.3753637485545,0.));
#245985=CARTESIAN_POINT('Ctrl Pts',(1.66491731718876,23.3753637485545,12.));
#245986=CARTESIAN_POINT('Ctrl Pts',(1.66853425293995,23.3577648365744,0.));
#245987=CARTESIAN_POINT('Ctrl Pts',(1.66853425293995,23.3577648365744,12.));
#245988=CARTESIAN_POINT('Ctrl Pts',(1.67207631363921,23.3402785571865,0.));
#245989=CARTESIAN_POINT('Ctrl Pts',(1.67207631363921,23.3402785571865,12.));
#245990=CARTESIAN_POINT('Ctrl Pts',(1.67554381222994,23.3229061599145,0.));
#245991=CARTESIAN_POINT('Ctrl Pts',(1.67554381222994,23.3229061599145,12.));
#245992=CARTESIAN_POINT('Ctrl Pts',(1.67893706857117,23.3056489135611,0.));
#245993=CARTESIAN_POINT('Ctrl Pts',(1.67893706857117,23.3056489135611,12.));
#245994=CARTESIAN_POINT('Ctrl Pts',(1.68225640962168,23.2885081066951,0.));
#245995=CARTESIAN_POINT('Ctrl Pts',(1.68225640962168,23.2885081066951,12.));
#245996=CARTESIAN_POINT('Ctrl Pts',(1.68550216963258,23.2714850482246,0.));
#245997=CARTESIAN_POINT('Ctrl Pts',(1.68550216963258,23.2714850482246,12.));
#245998=CARTESIAN_POINT('Ctrl Pts',(1.68867469034896,23.2545810680537,0.));
#245999=CARTESIAN_POINT('Ctrl Pts',(1.68867469034896,23.2545810680537,12.));
#246000=CARTESIAN_POINT('Ctrl Pts',(1.69177432121711,23.2377975177013,0.));
#246001=CARTESIAN_POINT('Ctrl Pts',(1.69177432121711,23.2377975177013,12.));
#246002=CARTESIAN_POINT('Ctrl Pts',(1.69480141959953,23.2211357709374,0.));
#246003=CARTESIAN_POINT('Ctrl Pts',(1.69480141959953,23.2211357709374,12.));
#246004=CARTESIAN_POINT('Ctrl Pts',(1.69775635099443,23.2045972243767,0.));
#246005=CARTESIAN_POINT('Ctrl Pts',(1.69775635099443,23.2045972243767,12.));
#246006=CARTESIAN_POINT('Ctrl Pts',(1.7006394892701,23.1881832981851,0.));
#246007=CARTESIAN_POINT('Ctrl Pts',(1.7006394892701,23.1881832981851,12.));
#246008=CARTESIAN_POINT('Ctrl Pts',(1.70345121691276,23.1718954368751,0.));
#246009=CARTESIAN_POINT('Ctrl Pts',(1.70345121691276,23.1718954368751,12.));
#246010=CARTESIAN_POINT('Ctrl Pts',(1.70619192527852,23.1557351100614,0.));
#246011=CARTESIAN_POINT('Ctrl Pts',(1.70619192527852,23.1557351100614,12.));
#246012=CARTESIAN_POINT('Ctrl Pts',(1.70886201485452,23.1397038132356,0.));
#246013=CARTESIAN_POINT('Ctrl Pts',(1.70886201485452,23.1397038132356,12.));
#246014=CARTESIAN_POINT('Ctrl Pts',(1.71146189552174,23.1238030684925,0.));
#246015=CARTESIAN_POINT('Ctrl Pts',(1.71146189552174,23.1238030684925,12.));
#246016=CARTESIAN_POINT('Ctrl Pts',(1.71399198684704,23.1080344254286,0.));
#246017=CARTESIAN_POINT('Ctrl Pts',(1.71399198684704,23.1080344254286,12.));
#246018=CARTESIAN_POINT('Ctrl Pts',(1.71645271839296,23.0923994621213,0.));
#246019=CARTESIAN_POINT('Ctrl Pts',(1.71645271839296,23.0923994621213,12.));
#246020=CARTESIAN_POINT('Ctrl Pts',(1.71884453003027,23.0768997860709,0.));
#246021=CARTESIAN_POINT('Ctrl Pts',(1.71884453003027,23.0768997860709,12.));
#246022=CARTESIAN_POINT('Ctrl Pts',(1.72116787225991,23.0615370351562,0.));
#246023=CARTESIAN_POINT('Ctrl Pts',(1.72116787225991,23.0615370351562,12.));
#246024=CARTESIAN_POINT('Ctrl Pts',(1.72342320653746,23.0463128785531,0.));
#246025=CARTESIAN_POINT('Ctrl Pts',(1.72342320653746,23.0463128785531,12.));
#246026=CARTESIAN_POINT('Ctrl Pts',(1.72561100564045,23.0312290178883,0.));
#246027=CARTESIAN_POINT('Ctrl Pts',(1.72561100564045,23.0312290178883,12.));
#246028=CARTESIAN_POINT('Ctrl Pts',(1.72773175404708,23.0162871884168,0.));
#246029=CARTESIAN_POINT('Ctrl Pts',(1.72773175404708,23.0162871884168,12.));
#246030=CARTESIAN_POINT('Ctrl Pts',(1.72978594832136,23.001489160189,0.));
#246031=CARTESIAN_POINT('Ctrl Pts',(1.72978594832136,23.001489160189,12.));
#246032=CARTESIAN_POINT('Ctrl Pts',(1.7317740975019,22.9868367391978,0.));
#246033=CARTESIAN_POINT('Ctrl Pts',(1.7317740975019,22.9868367391978,12.));
#246034=CARTESIAN_POINT('Ctrl Pts',(1.73369672350814,22.9723317685688,0.));
#246035=CARTESIAN_POINT('Ctrl Pts',(1.73369672350814,22.9723317685688,12.));
#246036=CARTESIAN_POINT('Ctrl Pts',(1.73555436162769,22.9579761301063,0.));
#246037=CARTESIAN_POINT('Ctrl Pts',(1.73555436162769,22.9579761301063,12.));
#246038=CARTESIAN_POINT('Ctrl Pts',(1.73734756100039,22.9437717457826,0.));
#246039=CARTESIAN_POINT('Ctrl Pts',(1.73734756100039,22.9437717457826,12.));
#246040=CARTESIAN_POINT('Ctrl Pts',(1.73907688511666,22.9297205792586,0.));
#246041=CARTESIAN_POINT('Ctrl Pts',(1.73907688511666,22.9297205792586,12.));
#246042=CARTESIAN_POINT('Ctrl Pts',(1.74074291231058,22.9158246373363,0.));
#246043=CARTESIAN_POINT('Ctrl Pts',(1.74074291231058,22.9158246373363,12.));
#246044=CARTESIAN_POINT('Ctrl Pts',(1.7423462363008,22.9020859716141,0.));
#246045=CARTESIAN_POINT('Ctrl Pts',(1.7423462363008,22.9020859716141,12.));
#246046=CARTESIAN_POINT('Ctrl Pts',(1.74388746677702,22.888506680335,0.));
#246047=CARTESIAN_POINT('Ctrl Pts',(1.74388746677702,22.888506680335,12.));
#246048=CARTESIAN_POINT('Ctrl Pts',(1.74536722998201,22.8750889101696,0.));
#246049=CARTESIAN_POINT('Ctrl Pts',(1.74536722998201,22.8750889101696,12.));
#246050=CARTESIAN_POINT('Ctrl Pts',(1.74678616930664,22.8618348580235,0.));
#246051=CARTESIAN_POINT('Ctrl Pts',(1.74678616930664,22.8618348580235,12.));
#246052=CARTESIAN_POINT('Ctrl Pts',(1.74814494588492,22.8487467728076,0.));
#246053=CARTESIAN_POINT('Ctrl Pts',(1.74814494588492,22.8487467728076,12.));
#246054=CARTESIAN_POINT('Ctrl Pts',(1.74944423940115,22.8358269579853,0.));
#246055=CARTESIAN_POINT('Ctrl Pts',(1.74944423940115,22.8358269579853,12.));
#246056=CARTESIAN_POINT('Ctrl Pts',(1.75068474890883,22.8230777741284,0.));
#246057=CARTESIAN_POINT('Ctrl Pts',(1.75068474890883,22.8230777741284,12.));
#246058=CARTESIAN_POINT('Ctrl Pts',(1.75186719365592,22.8105016414713,0.));
#246059=CARTESIAN_POINT('Ctrl Pts',(1.75186719365592,22.8105016414713,12.));
#246060=CARTESIAN_POINT('Ctrl Pts',(1.75299231391466,22.7981010424314,0.));
#246061=CARTESIAN_POINT('Ctrl Pts',(1.75299231391466,22.7981010424314,12.));
#246062=CARTESIAN_POINT('Ctrl Pts',(1.75406087182936,22.7858785242361,0.));
#246063=CARTESIAN_POINT('Ctrl Pts',(1.75406087182936,22.7858785242361,12.));
#246064=CARTESIAN_POINT('Ctrl Pts',(1.75507365227131,22.7738367016118,0.));
#246065=CARTESIAN_POINT('Ctrl Pts',(1.75507365227131,22.7738367016118,12.));
#246066=CARTESIAN_POINT('Ctrl Pts',(1.75603146371641,22.7619782595013,0.));
#246067=CARTESIAN_POINT('Ctrl Pts',(1.75603146371641,22.7619782595013,12.));
#246068=CARTESIAN_POINT('Ctrl Pts',(1.75693513908907,22.750305955645,0.));
#246069=CARTESIAN_POINT('Ctrl Pts',(1.75693513908907,22.750305955645,12.));
#246070=CARTESIAN_POINT('Ctrl Pts',(1.75778553673244,22.7388226235559,0.));
#246071=CARTESIAN_POINT('Ctrl Pts',(1.75778553673244,22.7388226235559,12.));
#246072=CARTESIAN_POINT('Ctrl Pts',(1.75858354204633,22.72753117773,0.));
#246073=CARTESIAN_POINT('Ctrl Pts',(1.75858354204633,22.72753117773,12.));
#246074=CARTESIAN_POINT('Ctrl Pts',(1.75933006905925,22.7164346186006,0.));
#246075=CARTESIAN_POINT('Ctrl Pts',(1.75933006905925,22.7164346186006,12.));
#246076=CARTESIAN_POINT('Ctrl Pts',(1.76002606202401,22.7055360375485,0.));
#246077=CARTESIAN_POINT('Ctrl Pts',(1.76002606202401,22.7055360375485,12.));
#246078=CARTESIAN_POINT('Ctrl Pts',(1.76067249704886,22.6948386219851,0.));
#246079=CARTESIAN_POINT('Ctrl Pts',(1.76067249704886,22.6948386219851,12.));
#246080=CARTESIAN_POINT('Ctrl Pts',(1.76127038310614,22.684345658525,0.));
#246081=CARTESIAN_POINT('Ctrl Pts',(1.76127038310614,22.684345658525,12.));
#246082=CARTESIAN_POINT('Ctrl Pts',(1.76182076289525,22.67406053567,0.));
#246083=CARTESIAN_POINT('Ctrl Pts',(1.76182076289525,22.67406053567,12.));
#246084=CARTESIAN_POINT('Ctrl Pts',(1.76232471392568,22.6639867471753,0.));
#246085=CARTESIAN_POINT('Ctrl Pts',(1.76232471392568,22.6639867471753,12.));
#246086=CARTESIAN_POINT('Ctrl Pts',(1.76278334912561,22.6541278938409,0.));
#246087=CARTESIAN_POINT('Ctrl Pts',(1.76278334912561,22.6541278938409,12.));
#246088=CARTESIAN_POINT('Ctrl Pts',(1.76319782013916,22.6444876940423,0.));
#246089=CARTESIAN_POINT('Ctrl Pts',(1.76319782013916,22.6444876940423,12.));
#246090=CARTESIAN_POINT('Ctrl Pts',(1.76356932176273,22.6350699979359,0.));
#246091=CARTESIAN_POINT('Ctrl Pts',(1.76356932176273,22.6350699979359,12.));
#246092=CARTESIAN_POINT('Ctrl Pts',(1.76389909571403,22.6258787994848,0.));
#246093=CARTESIAN_POINT('Ctrl Pts',(1.76389909571403,22.6258787994848,12.));
#246094=CARTESIAN_POINT('Ctrl Pts',(1.76418843543739,22.6169182517694,0.));
#246095=CARTESIAN_POINT('Ctrl Pts',(1.76418843543739,22.6169182517694,12.));
#246096=CARTESIAN_POINT('Ctrl Pts',(1.76443868648015,22.6081926681343,0.));
#246097=CARTESIAN_POINT('Ctrl Pts',(1.76443868648015,22.6081926681343,12.));
#246098=CARTESIAN_POINT('Ctrl Pts',(1.76465124413557,22.5997065145638,0.));
#246099=CARTESIAN_POINT('Ctrl Pts',(1.76465124413557,22.5997065145638,12.));
#246100=CARTESIAN_POINT('Ctrl Pts',(1.76482755288411,22.5914644078106,0.));
#246101=CARTESIAN_POINT('Ctrl Pts',(1.76482755288411,22.5914644078106,12.));
#246102=CARTESIAN_POINT('Ctrl Pts',(1.76496910283088,22.5834711038022,0.));
#246103=CARTESIAN_POINT('Ctrl Pts',(1.76496910283088,22.5834711038022,12.));
#246104=CARTESIAN_POINT('Ctrl Pts',(1.76507744026746,22.5757315316353,0.));
#246105=CARTESIAN_POINT('Ctrl Pts',(1.76507744026746,22.5757315316353,12.));
#246106=CARTESIAN_POINT('Ctrl Pts',(1.76515418518831,22.5682508499873,0.));
#246107=CARTESIAN_POINT('Ctrl Pts',(1.76515418518831,22.5682508499873,12.));
#246108=CARTESIAN_POINT('Ctrl Pts',(1.7652010450045,22.5610344912501,0.));
#246109=CARTESIAN_POINT('Ctrl Pts',(1.7652010450045,22.5610344912501,12.));
#246110=CARTESIAN_POINT('Ctrl Pts',(1.76521983384062,22.5540882235837,0.));
#246111=CARTESIAN_POINT('Ctrl Pts',(1.76521983384062,22.5540882235837,12.));
#246112=CARTESIAN_POINT('Ctrl Pts',(1.76521245524047,22.5474180954006,0.));
#246113=CARTESIAN_POINT('Ctrl Pts',(1.76521245524047,22.5474180954006,12.));
#246114=CARTESIAN_POINT('Ctrl Pts',(1.76518087841493,22.5410303590892,0.));
#246115=CARTESIAN_POINT('Ctrl Pts',(1.76518087841493,22.5410303590892,12.));
#246116=CARTESIAN_POINT('Ctrl Pts',(1.76512711563254,22.5349313983571,0.));
#246117=CARTESIAN_POINT('Ctrl Pts',(1.76512711563254,22.5349313983571,12.));
#246118=CARTESIAN_POINT('Ctrl Pts',(1.76505320262759,22.529127665298,0.));
#246119=CARTESIAN_POINT('Ctrl Pts',(1.76505320262759,22.529127665298,12.));
#246120=CARTESIAN_POINT('Ctrl Pts',(1.76496128643375,22.5236259635515,0.));
#246121=CARTESIAN_POINT('Ctrl Pts',(1.76496128643375,22.5236259635515,12.));
#246122=CARTESIAN_POINT('Ctrl Pts',(1.76485369319895,22.5184336670207,0.));
#246123=CARTESIAN_POINT('Ctrl Pts',(1.76485369319895,22.5184336670207,12.));
#246124=CARTESIAN_POINT('Ctrl Pts',(1.76473303281149,22.5135590569554,0.));
#246125=CARTESIAN_POINT('Ctrl Pts',(1.76473303281149,22.5135590569554,12.));
#246126=CARTESIAN_POINT('Ctrl Pts',(1.76460218257313,22.5090112700212,0.));
#246127=CARTESIAN_POINT('Ctrl Pts',(1.76460218257313,22.5090112700212,12.));
#246128=CARTESIAN_POINT('Ctrl Pts',(1.76446408210364,22.5047996391978,0.));
#246129=CARTESIAN_POINT('Ctrl Pts',(1.76446408210364,22.5047996391978,12.));
#246130=CARTESIAN_POINT('Ctrl Pts',(1.76432160068737,22.5009332677316,0.));
#246131=CARTESIAN_POINT('Ctrl Pts',(1.76432160068737,22.5009332677316,12.));
#246132=CARTESIAN_POINT('Ctrl Pts',(1.76417731243483,22.4974203063191,0.));
#246133=CARTESIAN_POINT('Ctrl Pts',(1.76417731243483,22.4974203063191,12.));
#246134=CARTESIAN_POINT('Ctrl Pts',(1.76403393880316,22.4942693792449,0.));
#246135=CARTESIAN_POINT('Ctrl Pts',(1.76403393880316,22.4942693792449,12.));
#246136=CARTESIAN_POINT('Ctrl Pts',(1.76389475965714,22.4914909094908,0.));
#246137=CARTESIAN_POINT('Ctrl Pts',(1.76389475965714,22.4914909094908,12.));
#246138=CARTESIAN_POINT('Ctrl Pts',(1.76376424879468,22.4890991659479,0.));
#246139=CARTESIAN_POINT('Ctrl Pts',(1.76376424879468,22.4890991659479,12.));
#246140=CARTESIAN_POINT('Ctrl Pts',(1.76364784232925,22.4871115206572,0.));
#246141=CARTESIAN_POINT('Ctrl Pts',(1.76364784232925,22.4871115206572,12.));
#246142=CARTESIAN_POINT('Ctrl Pts',(1.76355076045549,22.4855446605991,0.));
#246143=CARTESIAN_POINT('Ctrl Pts',(1.76355076045549,22.4855446605991,12.));
#246144=CARTESIAN_POINT('Ctrl Pts',(1.76347698284861,22.4844112933125,0.));
#246145=CARTESIAN_POINT('Ctrl Pts',(1.76347698284861,22.4844112933125,12.));
#246146=CARTESIAN_POINT('Ctrl Pts',(1.76343813434659,22.4838562517064,0.));
#246147=CARTESIAN_POINT('Ctrl Pts',(1.76343813434659,22.4838562517064,12.));
#246148=CARTESIAN_POINT('Ctrl Pts',(1.76342064263637,22.4836387052228,0.));
#246149=CARTESIAN_POINT('Ctrl Pts',(1.76342064263637,22.4836387052228,12.));
#246150=CARTESIAN_POINT('Ctrl Pts',(1.7634141553879,22.4835819929788,0.));
#246151=CARTESIAN_POINT('Ctrl Pts',(1.7634141553879,22.4835819929788,12.));
#246152=CARTESIAN_POINT('Ctrl Pts',(1.7634122053118,22.4835757167854,0.));
#246153=CARTESIAN_POINT('Ctrl Pts',(1.7634122053118,22.4835757167854,12.));
#246154=CARTESIAN_POINT('',(0.661312440730901,25.991588367311,0.));
#246155=CARTESIAN_POINT('Ctrl Pts',(0.661312440730901,25.991588367311,0.));
#246156=CARTESIAN_POINT('Ctrl Pts',(0.664028313187627,25.9865613464773,
0.));
#246157=CARTESIAN_POINT('Ctrl Pts',(0.669451306780825,25.9765104298071,
0.));
#246158=CARTESIAN_POINT('Ctrl Pts',(0.677559543209725,25.9614434297919,
0.));
#246159=CARTESIAN_POINT('Ctrl Pts',(0.688318015057729,25.9413728471909,
0.));
#246160=CARTESIAN_POINT('Ctrl Pts',(0.701678575228756,25.9163158909426,
0.));
#246161=CARTESIAN_POINT('Ctrl Pts',(0.714951588527638,25.891290261497,0.));
#246162=CARTESIAN_POINT('Ctrl Pts',(0.728137036482335,25.8662960624185,
0.));
#246163=CARTESIAN_POINT('Ctrl Pts',(0.741234902663807,25.8413334619055,
0.));
#246164=CARTESIAN_POINT('Ctrl Pts',(0.754245175609524,25.8164027059984,
0.));
#246165=CARTESIAN_POINT('Ctrl Pts',(0.767167852651168,25.7915041383376,
0.));
#246166=CARTESIAN_POINT('Ctrl Pts',(0.780002940291965,25.7666381946955,
0.));
#246167=CARTESIAN_POINT('Ctrl Pts',(0.792750451616127,25.7418053757746,
0.));
#246168=CARTESIAN_POINT('Ctrl Pts',(0.805410404554352,25.7170062262525,
0.));
#246169=CARTESIAN_POINT('Ctrl Pts',(0.817982819787464,25.6922413110194,
0.));
#246170=CARTESIAN_POINT('Ctrl Pts',(0.830467718864205,25.6675111931952,
0.));
#246171=CARTESIAN_POINT('Ctrl Pts',(0.842865122120758,25.6428164100055,
0.));
#246172=CARTESIAN_POINT('Ctrl Pts',(0.855175047036549,25.6181574536049,
0.));
#246173=CARTESIAN_POINT('Ctrl Pts',(0.867397509338431,25.5935347843585,
0.));
#246174=CARTESIAN_POINT('Ctrl Pts',(0.879532523834294,25.5689488408156,
0.));
#246175=CARTESIAN_POINT('Ctrl Pts',(0.89158010534904,25.5444000508211,0.));
#246176=CARTESIAN_POINT('Ctrl Pts',(0.903540269651106,25.5198888424194,
0.));
#246177=CARTESIAN_POINT('Ctrl Pts',(0.915413034335613,25.4954156541795,
0.));
#246178=CARTESIAN_POINT('Ctrl Pts',(0.927198419886094,25.4709809475009,
0.));
#246179=CARTESIAN_POINT('Ctrl Pts',(0.938896449496192,25.4465852044849,
0.));
#246180=CARTESIAN_POINT('Ctrl Pts',(0.950507148597468,25.4222289223167,
0.));
#246181=CARTESIAN_POINT('Ctrl Pts',(0.962030544503142,25.3979126089163,
0.));
#246182=CARTESIAN_POINT('Ctrl Pts',(0.973466666000163,25.3736367778845,
0.));
#246183=CARTESIAN_POINT('Ctrl Pts',(0.984815543003973,25.3494019441441,
0.));
#246184=CARTESIAN_POINT('Ctrl Pts',(0.996077206120624,25.3252086182968,
0.));
#246185=CARTESIAN_POINT('Ctrl Pts',(1.00725168656896,25.3010573055547,0.));
#246186=CARTESIAN_POINT('Ctrl Pts',(1.01833901642237,25.276948508726,0.));
#246187=CARTESIAN_POINT('Ctrl Pts',(1.02933922876806,25.2528827300422,0.));
#246188=CARTESIAN_POINT('Ctrl Pts',(1.04025235791507,25.2288604735086,0.));
#246189=CARTESIAN_POINT('Ctrl Pts',(1.05107843957931,25.2048822469028,0.));
#246190=CARTESIAN_POINT('Ctrl Pts',(1.06181751111768,25.1809485642192,0.));
#246191=CARTESIAN_POINT('Ctrl Pts',(1.07246961165475,25.157059946931,0.));
#246192=CARTESIAN_POINT('Ctrl Pts',(1.08303478197187,25.1332169227413,0.));
#246193=CARTESIAN_POINT('Ctrl Pts',(1.09351306445308,25.1094200248446,0.));
#246194=CARTESIAN_POINT('Ctrl Pts',(1.10390450301745,25.0856697909679,0.));
#246195=CARTESIAN_POINT('Ctrl Pts',(1.11420914306889,25.0619667625336,0.));
#246196=CARTESIAN_POINT('Ctrl Pts',(1.12442703144451,25.0383114836899,0.));
#246197=CARTESIAN_POINT('Ctrl Pts',(1.1345582163853,25.0147045006196,0.));
#246198=CARTESIAN_POINT('Ctrl Pts',(1.144602747582,24.9911463621433,0.));
#246199=CARTESIAN_POINT('Ctrl Pts',(1.15456067621889,24.9676376201502,0.));
#246200=CARTESIAN_POINT('Ctrl Pts',(1.16443205502849,24.9441788300932,0.));
#246201=CARTESIAN_POINT('Ctrl Pts',(1.17421693835041,24.9207705514449,0.));
#246202=CARTESIAN_POINT('Ctrl Pts',(1.18391538220103,24.8974133481829,0.));
#246203=CARTESIAN_POINT('Ctrl Pts',(1.19352744434064,24.8741077892075,0.));
#246204=CARTESIAN_POINT('Ctrl Pts',(1.2030531842602,24.8508544481974,0.));
#246205=CARTESIAN_POINT('Ctrl Pts',(1.21249266318208,24.8276539035092,0.));
#246206=CARTESIAN_POINT('Ctrl Pts',(1.22184594406528,24.8045067380536,0.));
#246207=CARTESIAN_POINT('Ctrl Pts',(1.23111309161843,24.7814135391799,0.));
#246208=CARTESIAN_POINT('Ctrl Pts',(1.24029417231989,24.7583748985438,0.));
#246209=CARTESIAN_POINT('Ctrl Pts',(1.24938925444325,24.7353914120011,0.));
#246210=CARTESIAN_POINT('Ctrl Pts',(1.25839840807418,24.7124636797894,0.));
#246211=CARTESIAN_POINT('Ctrl Pts',(1.267321705135,24.6895923066836,0.));
#246212=CARTESIAN_POINT('Ctrl Pts',(1.27615921941642,24.666777902156,0.));
#246213=CARTESIAN_POINT('Ctrl Pts',(1.28491102661514,24.6440210805278,0.));
#246214=CARTESIAN_POINT('Ctrl Pts',(1.29357720438107,24.6213224611229,0.));
#246215=CARTESIAN_POINT('Ctrl Pts',(1.30215783236362,24.5986826684027,0.));
#246216=CARTESIAN_POINT('Ctrl Pts',(1.31065299222021,24.5761023320183,0.));
#246217=CARTESIAN_POINT('Ctrl Pts',(1.31906276763668,24.5535820868674,0.));
#246218=CARTESIAN_POINT('Ctrl Pts',(1.32738724435326,24.5311225731435,0.));
#246219=CARTESIAN_POINT('Ctrl Pts',(1.33562651019686,24.5087244363856,0.));
#246220=CARTESIAN_POINT('Ctrl Pts',(1.34378065512337,24.4863883275134,0.));
#246221=CARTESIAN_POINT('Ctrl Pts',(1.35184977125648,24.4641149028892,0.));
#246222=CARTESIAN_POINT('Ctrl Pts',(1.35983395290627,24.4419048244523,0.));
#246223=CARTESIAN_POINT('Ctrl Pts',(1.36773329659956,24.4197587598337,0.));
#246224=CARTESIAN_POINT('Ctrl Pts',(1.37554790111609,24.3976773824732,0.));
#246225=CARTESIAN_POINT('Ctrl Pts',(1.38327786752998,24.3756613717299,0.));
#246226=CARTESIAN_POINT('Ctrl Pts',(1.39092329926388,24.3537114129875,0.));
#246227=CARTESIAN_POINT('Ctrl Pts',(1.39848430212807,24.3318281977643,0.));
#246228=CARTESIAN_POINT('Ctrl Pts',(1.40596098434337,24.3100124238311,0.));
#246229=CARTESIAN_POINT('Ctrl Pts',(1.41335345657682,24.288264795321,0.));
#246230=CARTESIAN_POINT('Ctrl Pts',(1.42066183198252,24.2665860228356,0.));
#246231=CARTESIAN_POINT('Ctrl Pts',(1.42788622624854,24.2449768235488,0.));
#246232=CARTESIAN_POINT('Ctrl Pts',(1.43502675765508,24.2234379212984,0.));
#246233=CARTESIAN_POINT('Ctrl Pts',(1.44208354711082,24.201970046722,0.));
#246234=CARTESIAN_POINT('Ctrl Pts',(1.44905671818727,24.1805739374038,0.));
#246235=CARTESIAN_POINT('Ctrl Pts',(1.45594639716317,24.1592503380107,0.));
#246236=CARTESIAN_POINT('Ctrl Pts',(1.46275271307397,24.1380000004272,0.));
#246237=CARTESIAN_POINT('Ctrl Pts',(1.46947579776991,24.1168236838824,0.));
#246238=CARTESIAN_POINT('Ctrl Pts',(1.47611578597742,24.0957221550778,0.));
#246239=CARTESIAN_POINT('Ctrl Pts',(1.48267281533683,24.0746961883528,0.));
#246240=CARTESIAN_POINT('Ctrl Pts',(1.48914702644887,24.0537465658429,0.));
#246241=CARTESIAN_POINT('Ctrl Pts',(1.49553856292801,24.0328740776331,0.));
#246242=CARTESIAN_POINT('Ctrl Pts',(1.50184757146098,24.0120795219086,0.));
#246243=CARTESIAN_POINT('Ctrl Pts',(1.50807420187694,23.9913637050927,0.));
#246244=CARTESIAN_POINT('Ctrl Pts',(1.51421860720614,23.970727442014,0.));
#246245=CARTESIAN_POINT('Ctrl Pts',(1.52028094372792,23.9501715561033,0.));
#246246=CARTESIAN_POINT('Ctrl Pts',(1.52626137103032,23.9296968795757,0.));
#246247=CARTESIAN_POINT('Ctrl Pts',(1.53216005207463,23.9093042536119,0.));
#246248=CARTESIAN_POINT('Ctrl Pts',(1.53797715326758,23.8889945285318,0.));
#246249=CARTESIAN_POINT('Ctrl Pts',(1.5437128445399,23.8687685639642,0.));
#246250=CARTESIAN_POINT('Ctrl Pts',(1.54936729940541,23.8486272290705,0.));
#246251=CARTESIAN_POINT('Ctrl Pts',(1.55494069502635,23.8285714027636,0.));
#246252=CARTESIAN_POINT('Ctrl Pts',(1.56043321228633,23.8086019739194,0.));
#246253=CARTESIAN_POINT('Ctrl Pts',(1.56584503586843,23.7887198415878,0.));
#246254=CARTESIAN_POINT('Ctrl Pts',(1.57117635434408,23.7689259151862,0.));
#246255=CARTESIAN_POINT('Ctrl Pts',(1.57642736025246,23.749221114736,0.));
#246256=CARTESIAN_POINT('Ctrl Pts',(1.58159825017358,23.72960637113,0.));
#246257=CARTESIAN_POINT('Ctrl Pts',(1.58668922481221,23.710082626383,0.));
#246258=CARTESIAN_POINT('Ctrl Pts',(1.59170048908633,23.6906508338833,0.));
#246259=CARTESIAN_POINT('Ctrl Pts',(1.59663225222463,23.671311958631,0.));
#246260=CARTESIAN_POINT('Ctrl Pts',(1.60148472786595,23.6520669774876,0.));
#246261=CARTESIAN_POINT('Ctrl Pts',(1.60625813414672,23.6329168794929,0.));
#246262=CARTESIAN_POINT('Ctrl Pts',(1.61095269379778,23.6138626661653,0.));
#246263=CARTESIAN_POINT('Ctrl Pts',(1.61556863424698,23.5949053517997,0.));
#246264=CARTESIAN_POINT('Ctrl Pts',(1.62010618772866,23.57604596376,0.));
#246265=CARTESIAN_POINT('Ctrl Pts',(1.62456559140064,23.5572855427601,0.));
#246266=CARTESIAN_POINT('Ctrl Pts',(1.62894708745223,23.538625143226,0.));
#246267=CARTESIAN_POINT('Ctrl Pts',(1.63325092321725,23.5200658336612,0.));
#246268=CARTESIAN_POINT('Ctrl Pts',(1.63747735129474,23.5016086970003,0.));
#246269=CARTESIAN_POINT('Ctrl Pts',(1.64162662967528,23.4832548309645,0.));
#246270=CARTESIAN_POINT('Ctrl Pts',(1.64569902187611,23.4650053483932,0.));
#246271=CARTESIAN_POINT('Ctrl Pts',(1.6496947970734,23.4468613776574,0.));
#246272=CARTESIAN_POINT('Ctrl Pts',(1.65361423023728,23.4288240631043,0.));
#246273=CARTESIAN_POINT('Ctrl Pts',(1.65745760227505,23.4108945654805,0.));
#246274=CARTESIAN_POINT('Ctrl Pts',(1.66122520018011,23.3930740623619,0.));
#246275=CARTESIAN_POINT('Ctrl Pts',(1.66491731718876,23.3753637485545,0.));
#246276=CARTESIAN_POINT('Ctrl Pts',(1.66853425293995,23.3577648365744,0.));
#246277=CARTESIAN_POINT('Ctrl Pts',(1.67207631363921,23.3402785571865,0.));
#246278=CARTESIAN_POINT('Ctrl Pts',(1.67554381222994,23.3229061599145,0.));
#246279=CARTESIAN_POINT('Ctrl Pts',(1.67893706857117,23.3056489135611,0.));
#246280=CARTESIAN_POINT('Ctrl Pts',(1.68225640962168,23.2885081066951,0.));
#246281=CARTESIAN_POINT('Ctrl Pts',(1.68550216963258,23.2714850482246,0.));
#246282=CARTESIAN_POINT('Ctrl Pts',(1.68867469034896,23.2545810680537,0.));
#246283=CARTESIAN_POINT('Ctrl Pts',(1.69177432121711,23.2377975177013,0.));
#246284=CARTESIAN_POINT('Ctrl Pts',(1.69480141959953,23.2211357709374,0.));
#246285=CARTESIAN_POINT('Ctrl Pts',(1.69775635099443,23.2045972243767,0.));
#246286=CARTESIAN_POINT('Ctrl Pts',(1.7006394892701,23.1881832981851,0.));
#246287=CARTESIAN_POINT('Ctrl Pts',(1.70345121691276,23.1718954368751,0.));
#246288=CARTESIAN_POINT('Ctrl Pts',(1.70619192527852,23.1557351100614,0.));
#246289=CARTESIAN_POINT('Ctrl Pts',(1.70886201485452,23.1397038132356,0.));
#246290=CARTESIAN_POINT('Ctrl Pts',(1.71146189552174,23.1238030684925,0.));
#246291=CARTESIAN_POINT('Ctrl Pts',(1.71399198684704,23.1080344254286,0.));
#246292=CARTESIAN_POINT('Ctrl Pts',(1.71645271839296,23.0923994621213,0.));
#246293=CARTESIAN_POINT('Ctrl Pts',(1.71884453003027,23.0768997860709,0.));
#246294=CARTESIAN_POINT('Ctrl Pts',(1.72116787225991,23.0615370351562,0.));
#246295=CARTESIAN_POINT('Ctrl Pts',(1.72342320653746,23.0463128785531,0.));
#246296=CARTESIAN_POINT('Ctrl Pts',(1.72561100564045,23.0312290178883,0.));
#246297=CARTESIAN_POINT('Ctrl Pts',(1.72773175404708,23.0162871884168,0.));
#246298=CARTESIAN_POINT('Ctrl Pts',(1.72978594832136,23.001489160189,0.));
#246299=CARTESIAN_POINT('Ctrl Pts',(1.7317740975019,22.9868367391978,0.));
#246300=CARTESIAN_POINT('Ctrl Pts',(1.73369672350814,22.9723317685688,0.));
#246301=CARTESIAN_POINT('Ctrl Pts',(1.73555436162769,22.9579761301063,0.));
#246302=CARTESIAN_POINT('Ctrl Pts',(1.73734756100039,22.9437717457826,0.));
#246303=CARTESIAN_POINT('Ctrl Pts',(1.73907688511666,22.9297205792586,0.));
#246304=CARTESIAN_POINT('Ctrl Pts',(1.74074291231058,22.9158246373363,0.));
#246305=CARTESIAN_POINT('Ctrl Pts',(1.7423462363008,22.9020859716141,0.));
#246306=CARTESIAN_POINT('Ctrl Pts',(1.74388746677702,22.888506680335,0.));
#246307=CARTESIAN_POINT('Ctrl Pts',(1.74536722998201,22.8750889101696,0.));
#246308=CARTESIAN_POINT('Ctrl Pts',(1.74678616930664,22.8618348580235,0.));
#246309=CARTESIAN_POINT('Ctrl Pts',(1.74814494588492,22.8487467728076,0.));
#246310=CARTESIAN_POINT('Ctrl Pts',(1.74944423940115,22.8358269579853,0.));
#246311=CARTESIAN_POINT('Ctrl Pts',(1.75068474890883,22.8230777741284,0.));
#246312=CARTESIAN_POINT('Ctrl Pts',(1.75186719365592,22.8105016414713,0.));
#246313=CARTESIAN_POINT('Ctrl Pts',(1.75299231391466,22.7981010424314,0.));
#246314=CARTESIAN_POINT('Ctrl Pts',(1.75406087182936,22.7858785242361,0.));
#246315=CARTESIAN_POINT('Ctrl Pts',(1.75507365227131,22.7738367016118,0.));
#246316=CARTESIAN_POINT('Ctrl Pts',(1.75603146371641,22.7619782595013,0.));
#246317=CARTESIAN_POINT('Ctrl Pts',(1.75693513908907,22.750305955645,0.));
#246318=CARTESIAN_POINT('Ctrl Pts',(1.75778553673244,22.7388226235559,0.));
#246319=CARTESIAN_POINT('Ctrl Pts',(1.75858354204633,22.72753117773,0.));
#246320=CARTESIAN_POINT('Ctrl Pts',(1.75933006905925,22.7164346186006,0.));
#246321=CARTESIAN_POINT('Ctrl Pts',(1.76002606202401,22.7055360375485,0.));
#246322=CARTESIAN_POINT('Ctrl Pts',(1.76067249704886,22.6948386219851,0.));
#246323=CARTESIAN_POINT('Ctrl Pts',(1.76127038310614,22.684345658525,0.));
#246324=CARTESIAN_POINT('Ctrl Pts',(1.76182076289525,22.67406053567,0.));
#246325=CARTESIAN_POINT('Ctrl Pts',(1.76232471392568,22.6639867471753,0.));
#246326=CARTESIAN_POINT('Ctrl Pts',(1.76278334912561,22.6541278938409,0.));
#246327=CARTESIAN_POINT('Ctrl Pts',(1.76319782013916,22.6444876940423,0.));
#246328=CARTESIAN_POINT('Ctrl Pts',(1.76356932176273,22.6350699979359,0.));
#246329=CARTESIAN_POINT('Ctrl Pts',(1.76389909571403,22.6258787994848,0.));
#246330=CARTESIAN_POINT('Ctrl Pts',(1.76418843543739,22.6169182517694,0.));
#246331=CARTESIAN_POINT('Ctrl Pts',(1.76443868648015,22.6081926681343,0.));
#246332=CARTESIAN_POINT('Ctrl Pts',(1.76465124413557,22.5997065145638,0.));
#246333=CARTESIAN_POINT('Ctrl Pts',(1.76482755288411,22.5914644078106,0.));
#246334=CARTESIAN_POINT('Ctrl Pts',(1.76496910283088,22.5834711038022,0.));
#246335=CARTESIAN_POINT('Ctrl Pts',(1.76507744026746,22.5757315316353,0.));
#246336=CARTESIAN_POINT('Ctrl Pts',(1.76515418518831,22.5682508499873,0.));
#246337=CARTESIAN_POINT('Ctrl Pts',(1.7652010450045,22.5610344912501,0.));
#246338=CARTESIAN_POINT('Ctrl Pts',(1.76521983384062,22.5540882235837,0.));
#246339=CARTESIAN_POINT('Ctrl Pts',(1.76521245524047,22.5474180954006,0.));
#246340=CARTESIAN_POINT('Ctrl Pts',(1.76518087841493,22.5410303590892,0.));
#246341=CARTESIAN_POINT('Ctrl Pts',(1.76512711563254,22.5349313983571,0.));
#246342=CARTESIAN_POINT('Ctrl Pts',(1.76505320262759,22.529127665298,0.));
#246343=CARTESIAN_POINT('Ctrl Pts',(1.76496128643375,22.5236259635515,0.));
#246344=CARTESIAN_POINT('Ctrl Pts',(1.76485369319895,22.5184336670207,0.));
#246345=CARTESIAN_POINT('Ctrl Pts',(1.76473303281149,22.5135590569554,0.));
#246346=CARTESIAN_POINT('Ctrl Pts',(1.76460218257313,22.5090112700212,0.));
#246347=CARTESIAN_POINT('Ctrl Pts',(1.76446408210364,22.5047996391978,0.));
#246348=CARTESIAN_POINT('Ctrl Pts',(1.76432160068737,22.5009332677316,0.));
#246349=CARTESIAN_POINT('Ctrl Pts',(1.76417731243483,22.4974203063191,0.));
#246350=CARTESIAN_POINT('Ctrl Pts',(1.76403393880316,22.4942693792449,0.));
#246351=CARTESIAN_POINT('Ctrl Pts',(1.76389475965714,22.4914909094908,0.));
#246352=CARTESIAN_POINT('Ctrl Pts',(1.76376424879468,22.4890991659479,0.));
#246353=CARTESIAN_POINT('Ctrl Pts',(1.76364784232925,22.4871115206572,0.));
#246354=CARTESIAN_POINT('Ctrl Pts',(1.76355076045549,22.4855446605991,0.));
#246355=CARTESIAN_POINT('Ctrl Pts',(1.76347698284861,22.4844112933125,0.));
#246356=CARTESIAN_POINT('Ctrl Pts',(1.76343813434659,22.4838562517064,0.));
#246357=CARTESIAN_POINT('Ctrl Pts',(1.76342064263637,22.4836387052228,0.));
#246358=CARTESIAN_POINT('Ctrl Pts',(1.7634141553879,22.4835819929788,0.));
#246359=CARTESIAN_POINT('Ctrl Pts',(1.7634122053118,22.4835757167854,0.));
#246360=CARTESIAN_POINT('',(0.661312440730901,25.991588367311,12.));
#246361=CARTESIAN_POINT('',(0.661312440730901,25.991588367311,0.));
#246362=CARTESIAN_POINT('Ctrl Pts',(1.7634122053118,22.4835757167854,12.));
#246363=CARTESIAN_POINT('Ctrl Pts',(1.7634141553879,22.4835819929788,12.));
#246364=CARTESIAN_POINT('Ctrl Pts',(1.76342064263637,22.4836387052228,12.));
#246365=CARTESIAN_POINT('Ctrl Pts',(1.76343813434659,22.4838562517064,12.));
#246366=CARTESIAN_POINT('Ctrl Pts',(1.76347698284861,22.4844112933125,12.));
#246367=CARTESIAN_POINT('Ctrl Pts',(1.76355076045549,22.4855446605991,12.));
#246368=CARTESIAN_POINT('Ctrl Pts',(1.76364784232925,22.4871115206572,12.));
#246369=CARTESIAN_POINT('Ctrl Pts',(1.76376424879468,22.4890991659479,12.));
#246370=CARTESIAN_POINT('Ctrl Pts',(1.76389475965714,22.4914909094908,12.));
#246371=CARTESIAN_POINT('Ctrl Pts',(1.76403393880316,22.4942693792449,12.));
#246372=CARTESIAN_POINT('Ctrl Pts',(1.76417731243483,22.4974203063191,12.));
#246373=CARTESIAN_POINT('Ctrl Pts',(1.76432160068737,22.5009332677316,12.));
#246374=CARTESIAN_POINT('Ctrl Pts',(1.76446408210364,22.5047996391978,12.));
#246375=CARTESIAN_POINT('Ctrl Pts',(1.76460218257313,22.5090112700212,12.));
#246376=CARTESIAN_POINT('Ctrl Pts',(1.76473303281149,22.5135590569554,12.));
#246377=CARTESIAN_POINT('Ctrl Pts',(1.76485369319895,22.5184336670207,12.));
#246378=CARTESIAN_POINT('Ctrl Pts',(1.76496128643375,22.5236259635515,12.));
#246379=CARTESIAN_POINT('Ctrl Pts',(1.76505320262759,22.529127665298,12.));
#246380=CARTESIAN_POINT('Ctrl Pts',(1.76512711563254,22.5349313983571,12.));
#246381=CARTESIAN_POINT('Ctrl Pts',(1.76518087841493,22.5410303590892,12.));
#246382=CARTESIAN_POINT('Ctrl Pts',(1.76521245524047,22.5474180954006,12.));
#246383=CARTESIAN_POINT('Ctrl Pts',(1.76521983384062,22.5540882235837,12.));
#246384=CARTESIAN_POINT('Ctrl Pts',(1.7652010450045,22.5610344912501,12.));
#246385=CARTESIAN_POINT('Ctrl Pts',(1.76515418518831,22.5682508499873,12.));
#246386=CARTESIAN_POINT('Ctrl Pts',(1.76507744026746,22.5757315316353,12.));
#246387=CARTESIAN_POINT('Ctrl Pts',(1.76496910283088,22.5834711038022,12.));
#246388=CARTESIAN_POINT('Ctrl Pts',(1.76482755288411,22.5914644078106,12.));
#246389=CARTESIAN_POINT('Ctrl Pts',(1.76465124413557,22.5997065145638,12.));
#246390=CARTESIAN_POINT('Ctrl Pts',(1.76443868648015,22.6081926681343,12.));
#246391=CARTESIAN_POINT('Ctrl Pts',(1.76418843543739,22.6169182517694,12.));
#246392=CARTESIAN_POINT('Ctrl Pts',(1.76389909571403,22.6258787994848,12.));
#246393=CARTESIAN_POINT('Ctrl Pts',(1.76356932176273,22.6350699979359,12.));
#246394=CARTESIAN_POINT('Ctrl Pts',(1.76319782013916,22.6444876940423,12.));
#246395=CARTESIAN_POINT('Ctrl Pts',(1.76278334912561,22.6541278938409,12.));
#246396=CARTESIAN_POINT('Ctrl Pts',(1.76232471392568,22.6639867471753,12.));
#246397=CARTESIAN_POINT('Ctrl Pts',(1.76182076289525,22.67406053567,12.));
#246398=CARTESIAN_POINT('Ctrl Pts',(1.76127038310614,22.684345658525,12.));
#246399=CARTESIAN_POINT('Ctrl Pts',(1.76067249704886,22.6948386219851,12.));
#246400=CARTESIAN_POINT('Ctrl Pts',(1.76002606202401,22.7055360375485,12.));
#246401=CARTESIAN_POINT('Ctrl Pts',(1.75933006905925,22.7164346186006,12.));
#246402=CARTESIAN_POINT('Ctrl Pts',(1.75858354204633,22.72753117773,12.));
#246403=CARTESIAN_POINT('Ctrl Pts',(1.75778553673244,22.7388226235559,12.));
#246404=CARTESIAN_POINT('Ctrl Pts',(1.75693513908907,22.750305955645,12.));
#246405=CARTESIAN_POINT('Ctrl Pts',(1.75603146371641,22.7619782595013,12.));
#246406=CARTESIAN_POINT('Ctrl Pts',(1.75507365227131,22.7738367016118,12.));
#246407=CARTESIAN_POINT('Ctrl Pts',(1.75406087182936,22.7858785242361,12.));
#246408=CARTESIAN_POINT('Ctrl Pts',(1.75299231391466,22.7981010424314,12.));
#246409=CARTESIAN_POINT('Ctrl Pts',(1.75186719365592,22.8105016414713,12.));
#246410=CARTESIAN_POINT('Ctrl Pts',(1.75068474890883,22.8230777741284,12.));
#246411=CARTESIAN_POINT('Ctrl Pts',(1.74944423940115,22.8358269579853,12.));
#246412=CARTESIAN_POINT('Ctrl Pts',(1.74814494588492,22.8487467728076,12.));
#246413=CARTESIAN_POINT('Ctrl Pts',(1.74678616930664,22.8618348580235,12.));
#246414=CARTESIAN_POINT('Ctrl Pts',(1.74536722998201,22.8750889101696,12.));
#246415=CARTESIAN_POINT('Ctrl Pts',(1.74388746677702,22.888506680335,12.));
#246416=CARTESIAN_POINT('Ctrl Pts',(1.7423462363008,22.9020859716141,12.));
#246417=CARTESIAN_POINT('Ctrl Pts',(1.74074291231058,22.9158246373363,12.));
#246418=CARTESIAN_POINT('Ctrl Pts',(1.73907688511666,22.9297205792586,12.));
#246419=CARTESIAN_POINT('Ctrl Pts',(1.73734756100039,22.9437717457826,12.));
#246420=CARTESIAN_POINT('Ctrl Pts',(1.73555436162769,22.9579761301063,12.));
#246421=CARTESIAN_POINT('Ctrl Pts',(1.73369672350814,22.9723317685688,12.));
#246422=CARTESIAN_POINT('Ctrl Pts',(1.7317740975019,22.9868367391978,12.));
#246423=CARTESIAN_POINT('Ctrl Pts',(1.72978594832136,23.001489160189,12.));
#246424=CARTESIAN_POINT('Ctrl Pts',(1.72773175404708,23.0162871884168,12.));
#246425=CARTESIAN_POINT('Ctrl Pts',(1.72561100564045,23.0312290178883,12.));
#246426=CARTESIAN_POINT('Ctrl Pts',(1.72342320653746,23.0463128785531,12.));
#246427=CARTESIAN_POINT('Ctrl Pts',(1.72116787225991,23.0615370351562,12.));
#246428=CARTESIAN_POINT('Ctrl Pts',(1.71884453003027,23.0768997860709,12.));
#246429=CARTESIAN_POINT('Ctrl Pts',(1.71645271839296,23.0923994621213,12.));
#246430=CARTESIAN_POINT('Ctrl Pts',(1.71399198684704,23.1080344254286,12.));
#246431=CARTESIAN_POINT('Ctrl Pts',(1.71146189552174,23.1238030684925,12.));
#246432=CARTESIAN_POINT('Ctrl Pts',(1.70886201485452,23.1397038132356,12.));
#246433=CARTESIAN_POINT('Ctrl Pts',(1.70619192527852,23.1557351100614,12.));
#246434=CARTESIAN_POINT('Ctrl Pts',(1.70345121691276,23.1718954368751,12.));
#246435=CARTESIAN_POINT('Ctrl Pts',(1.7006394892701,23.1881832981851,12.));
#246436=CARTESIAN_POINT('Ctrl Pts',(1.69775635099443,23.2045972243767,12.));
#246437=CARTESIAN_POINT('Ctrl Pts',(1.69480141959953,23.2211357709374,12.));
#246438=CARTESIAN_POINT('Ctrl Pts',(1.69177432121711,23.2377975177013,12.));
#246439=CARTESIAN_POINT('Ctrl Pts',(1.68867469034896,23.2545810680537,12.));
#246440=CARTESIAN_POINT('Ctrl Pts',(1.68550216963258,23.2714850482246,12.));
#246441=CARTESIAN_POINT('Ctrl Pts',(1.68225640962168,23.2885081066951,12.));
#246442=CARTESIAN_POINT('Ctrl Pts',(1.67893706857117,23.3056489135611,12.));
#246443=CARTESIAN_POINT('Ctrl Pts',(1.67554381222994,23.3229061599145,12.));
#246444=CARTESIAN_POINT('Ctrl Pts',(1.67207631363921,23.3402785571865,12.));
#246445=CARTESIAN_POINT('Ctrl Pts',(1.66853425293995,23.3577648365744,12.));
#246446=CARTESIAN_POINT('Ctrl Pts',(1.66491731718876,23.3753637485545,12.));
#246447=CARTESIAN_POINT('Ctrl Pts',(1.66122520018011,23.3930740623619,12.));
#246448=CARTESIAN_POINT('Ctrl Pts',(1.65745760227505,23.4108945654805,12.));
#246449=CARTESIAN_POINT('Ctrl Pts',(1.65361423023728,23.4288240631043,12.));
#246450=CARTESIAN_POINT('Ctrl Pts',(1.6496947970734,23.4468613776574,12.));
#246451=CARTESIAN_POINT('Ctrl Pts',(1.64569902187611,23.4650053483932,12.));
#246452=CARTESIAN_POINT('Ctrl Pts',(1.64162662967528,23.4832548309645,12.));
#246453=CARTESIAN_POINT('Ctrl Pts',(1.63747735129474,23.5016086970003,12.));
#246454=CARTESIAN_POINT('Ctrl Pts',(1.63325092321725,23.5200658336612,12.));
#246455=CARTESIAN_POINT('Ctrl Pts',(1.62894708745223,23.538625143226,12.));
#246456=CARTESIAN_POINT('Ctrl Pts',(1.62456559140064,23.5572855427601,12.));
#246457=CARTESIAN_POINT('Ctrl Pts',(1.62010618772866,23.57604596376,12.));
#246458=CARTESIAN_POINT('Ctrl Pts',(1.61556863424698,23.5949053517997,12.));
#246459=CARTESIAN_POINT('Ctrl Pts',(1.61095269379778,23.6138626661653,12.));
#246460=CARTESIAN_POINT('Ctrl Pts',(1.60625813414672,23.6329168794929,12.));
#246461=CARTESIAN_POINT('Ctrl Pts',(1.60148472786595,23.6520669774876,12.));
#246462=CARTESIAN_POINT('Ctrl Pts',(1.59663225222463,23.671311958631,12.));
#246463=CARTESIAN_POINT('Ctrl Pts',(1.59170048908633,23.6906508338833,12.));
#246464=CARTESIAN_POINT('Ctrl Pts',(1.58668922481221,23.710082626383,12.));
#246465=CARTESIAN_POINT('Ctrl Pts',(1.58159825017358,23.72960637113,12.));
#246466=CARTESIAN_POINT('Ctrl Pts',(1.57642736025246,23.749221114736,12.));
#246467=CARTESIAN_POINT('Ctrl Pts',(1.57117635434408,23.7689259151862,12.));
#246468=CARTESIAN_POINT('Ctrl Pts',(1.56584503586843,23.7887198415878,12.));
#246469=CARTESIAN_POINT('Ctrl Pts',(1.56043321228633,23.8086019739194,12.));
#246470=CARTESIAN_POINT('Ctrl Pts',(1.55494069502635,23.8285714027636,12.));
#246471=CARTESIAN_POINT('Ctrl Pts',(1.54936729940541,23.8486272290705,12.));
#246472=CARTESIAN_POINT('Ctrl Pts',(1.5437128445399,23.8687685639642,12.));
#246473=CARTESIAN_POINT('Ctrl Pts',(1.53797715326758,23.8889945285318,12.));
#246474=CARTESIAN_POINT('Ctrl Pts',(1.53216005207463,23.9093042536119,12.));
#246475=CARTESIAN_POINT('Ctrl Pts',(1.52626137103032,23.9296968795757,12.));
#246476=CARTESIAN_POINT('Ctrl Pts',(1.52028094372792,23.9501715561033,12.));
#246477=CARTESIAN_POINT('Ctrl Pts',(1.51421860720614,23.970727442014,12.));
#246478=CARTESIAN_POINT('Ctrl Pts',(1.50807420187694,23.9913637050927,12.));
#246479=CARTESIAN_POINT('Ctrl Pts',(1.50184757146098,24.0120795219086,12.));
#246480=CARTESIAN_POINT('Ctrl Pts',(1.49553856292801,24.0328740776331,12.));
#246481=CARTESIAN_POINT('Ctrl Pts',(1.48914702644887,24.0537465658429,12.));
#246482=CARTESIAN_POINT('Ctrl Pts',(1.48267281533683,24.0746961883528,12.));
#246483=CARTESIAN_POINT('Ctrl Pts',(1.47611578597742,24.0957221550778,12.));
#246484=CARTESIAN_POINT('Ctrl Pts',(1.46947579776991,24.1168236838824,12.));
#246485=CARTESIAN_POINT('Ctrl Pts',(1.46275271307397,24.1380000004272,12.));
#246486=CARTESIAN_POINT('Ctrl Pts',(1.45594639716317,24.1592503380107,12.));
#246487=CARTESIAN_POINT('Ctrl Pts',(1.44905671818727,24.1805739374038,12.));
#246488=CARTESIAN_POINT('Ctrl Pts',(1.44208354711082,24.201970046722,12.));
#246489=CARTESIAN_POINT('Ctrl Pts',(1.43502675765508,24.2234379212984,12.));
#246490=CARTESIAN_POINT('Ctrl Pts',(1.42788622624854,24.2449768235488,12.));
#246491=CARTESIAN_POINT('Ctrl Pts',(1.42066183198252,24.2665860228356,12.));
#246492=CARTESIAN_POINT('Ctrl Pts',(1.41335345657682,24.288264795321,12.));
#246493=CARTESIAN_POINT('Ctrl Pts',(1.40596098434337,24.3100124238311,12.));
#246494=CARTESIAN_POINT('Ctrl Pts',(1.39848430212807,24.3318281977643,12.));
#246495=CARTESIAN_POINT('Ctrl Pts',(1.39092329926388,24.3537114129875,12.));
#246496=CARTESIAN_POINT('Ctrl Pts',(1.38327786752998,24.3756613717299,12.));
#246497=CARTESIAN_POINT('Ctrl Pts',(1.37554790111609,24.3976773824732,12.));
#246498=CARTESIAN_POINT('Ctrl Pts',(1.36773329659956,24.4197587598337,12.));
#246499=CARTESIAN_POINT('Ctrl Pts',(1.35983395290627,24.4419048244523,12.));
#246500=CARTESIAN_POINT('Ctrl Pts',(1.35184977125648,24.4641149028892,12.));
#246501=CARTESIAN_POINT('Ctrl Pts',(1.34378065512337,24.4863883275134,12.));
#246502=CARTESIAN_POINT('Ctrl Pts',(1.33562651019686,24.5087244363856,12.));
#246503=CARTESIAN_POINT('Ctrl Pts',(1.32738724435326,24.5311225731435,12.));
#246504=CARTESIAN_POINT('Ctrl Pts',(1.31906276763668,24.5535820868674,12.));
#246505=CARTESIAN_POINT('Ctrl Pts',(1.31065299222021,24.5761023320183,12.));
#246506=CARTESIAN_POINT('Ctrl Pts',(1.30215783236362,24.5986826684027,12.));
#246507=CARTESIAN_POINT('Ctrl Pts',(1.29357720438107,24.6213224611229,12.));
#246508=CARTESIAN_POINT('Ctrl Pts',(1.28491102661514,24.6440210805278,12.));
#246509=CARTESIAN_POINT('Ctrl Pts',(1.27615921941642,24.666777902156,12.));
#246510=CARTESIAN_POINT('Ctrl Pts',(1.267321705135,24.6895923066836,12.));
#246511=CARTESIAN_POINT('Ctrl Pts',(1.25839840807418,24.7124636797894,12.));
#246512=CARTESIAN_POINT('Ctrl Pts',(1.24938925444325,24.7353914120011,12.));
#246513=CARTESIAN_POINT('Ctrl Pts',(1.24029417231989,24.7583748985438,12.));
#246514=CARTESIAN_POINT('Ctrl Pts',(1.23111309161843,24.7814135391799,12.));
#246515=CARTESIAN_POINT('Ctrl Pts',(1.22184594406528,24.8045067380536,12.));
#246516=CARTESIAN_POINT('Ctrl Pts',(1.21249266318208,24.8276539035092,12.));
#246517=CARTESIAN_POINT('Ctrl Pts',(1.2030531842602,24.8508544481974,12.));
#246518=CARTESIAN_POINT('Ctrl Pts',(1.19352744434064,24.8741077892075,12.));
#246519=CARTESIAN_POINT('Ctrl Pts',(1.18391538220103,24.8974133481829,12.));
#246520=CARTESIAN_POINT('Ctrl Pts',(1.17421693835041,24.9207705514449,12.));
#246521=CARTESIAN_POINT('Ctrl Pts',(1.16443205502849,24.9441788300932,12.));
#246522=CARTESIAN_POINT('Ctrl Pts',(1.15456067621889,24.9676376201502,12.));
#246523=CARTESIAN_POINT('Ctrl Pts',(1.144602747582,24.9911463621433,12.));
#246524=CARTESIAN_POINT('Ctrl Pts',(1.1345582163853,25.0147045006196,12.));
#246525=CARTESIAN_POINT('Ctrl Pts',(1.12442703144451,25.0383114836899,12.));
#246526=CARTESIAN_POINT('Ctrl Pts',(1.11420914306889,25.0619667625336,12.));
#246527=CARTESIAN_POINT('Ctrl Pts',(1.10390450301745,25.0856697909679,12.));
#246528=CARTESIAN_POINT('Ctrl Pts',(1.09351306445308,25.1094200248446,12.));
#246529=CARTESIAN_POINT('Ctrl Pts',(1.08303478197187,25.1332169227413,12.));
#246530=CARTESIAN_POINT('Ctrl Pts',(1.07246961165475,25.157059946931,12.));
#246531=CARTESIAN_POINT('Ctrl Pts',(1.06181751111768,25.1809485642192,12.));
#246532=CARTESIAN_POINT('Ctrl Pts',(1.05107843957931,25.2048822469028,12.));
#246533=CARTESIAN_POINT('Ctrl Pts',(1.04025235791507,25.2288604735086,12.));
#246534=CARTESIAN_POINT('Ctrl Pts',(1.02933922876806,25.2528827300422,12.));
#246535=CARTESIAN_POINT('Ctrl Pts',(1.01833901642237,25.276948508726,12.));
#246536=CARTESIAN_POINT('Ctrl Pts',(1.00725168656896,25.3010573055547,12.));
#246537=CARTESIAN_POINT('Ctrl Pts',(0.996077206120624,25.3252086182968,
12.));
#246538=CARTESIAN_POINT('Ctrl Pts',(0.984815543003973,25.3494019441441,
12.));
#246539=CARTESIAN_POINT('Ctrl Pts',(0.973466666000163,25.3736367778845,
12.));
#246540=CARTESIAN_POINT('Ctrl Pts',(0.962030544503142,25.3979126089163,
12.));
#246541=CARTESIAN_POINT('Ctrl Pts',(0.950507148597468,25.4222289223167,
12.));
#246542=CARTESIAN_POINT('Ctrl Pts',(0.938896449496192,25.4465852044849,
12.));
#246543=CARTESIAN_POINT('Ctrl Pts',(0.927198419886094,25.4709809475009,
12.));
#246544=CARTESIAN_POINT('Ctrl Pts',(0.915413034335613,25.4954156541795,
12.));
#246545=CARTESIAN_POINT('Ctrl Pts',(0.903540269651106,25.5198888424194,
12.));
#246546=CARTESIAN_POINT('Ctrl Pts',(0.89158010534904,25.5444000508211,12.));
#246547=CARTESIAN_POINT('Ctrl Pts',(0.879532523834294,25.5689488408156,
12.));
#246548=CARTESIAN_POINT('Ctrl Pts',(0.867397509338431,25.5935347843585,
12.));
#246549=CARTESIAN_POINT('Ctrl Pts',(0.855175047036549,25.6181574536049,
12.));
#246550=CARTESIAN_POINT('Ctrl Pts',(0.842865122120758,25.6428164100055,
12.));
#246551=CARTESIAN_POINT('Ctrl Pts',(0.830467718864205,25.6675111931952,
12.));
#246552=CARTESIAN_POINT('Ctrl Pts',(0.817982819787464,25.6922413110194,
12.));
#246553=CARTESIAN_POINT('Ctrl Pts',(0.805410404554352,25.7170062262525,
12.));
#246554=CARTESIAN_POINT('Ctrl Pts',(0.792750451616127,25.7418053757746,
12.));
#246555=CARTESIAN_POINT('Ctrl Pts',(0.780002940291965,25.7666381946955,
12.));
#246556=CARTESIAN_POINT('Ctrl Pts',(0.767167852651168,25.7915041383376,
12.));
#246557=CARTESIAN_POINT('Ctrl Pts',(0.754245175609524,25.8164027059984,
12.));
#246558=CARTESIAN_POINT('Ctrl Pts',(0.741234902663807,25.8413334619055,
12.));
#246559=CARTESIAN_POINT('Ctrl Pts',(0.728137036482335,25.8662960624185,
12.));
#246560=CARTESIAN_POINT('Ctrl Pts',(0.714951588527638,25.891290261497,12.));
#246561=CARTESIAN_POINT('Ctrl Pts',(0.701678575228756,25.9163158909426,
12.));
#246562=CARTESIAN_POINT('Ctrl Pts',(0.688318015057729,25.9413728471909,
12.));
#246563=CARTESIAN_POINT('Ctrl Pts',(0.677559543209725,25.9614434297919,
12.));
#246564=CARTESIAN_POINT('Ctrl Pts',(0.669451306780825,25.9765104298071,
12.));
#246565=CARTESIAN_POINT('Ctrl Pts',(0.664028313187627,25.9865613464773,
12.));
#246566=CARTESIAN_POINT('Ctrl Pts',(0.661312440730901,25.991588367311,12.));
#246567=CARTESIAN_POINT('Ctrl Pts',(4.11585220600461,22.1738711152697,0.));
#246568=CARTESIAN_POINT('Ctrl Pts',(4.11585220600461,22.1738711152697,12.));
#246569=CARTESIAN_POINT('Ctrl Pts',(4.11585194677442,22.173877682324,0.));
#246570=CARTESIAN_POINT('Ctrl Pts',(4.11585194677442,22.173877682324,12.));
#246571=CARTESIAN_POINT('Ctrl Pts',(4.11586035878287,22.1739341411687,0.));
#246572=CARTESIAN_POINT('Ctrl Pts',(4.11586035878287,22.1739341411687,12.));
#246573=CARTESIAN_POINT('Ctrl Pts',(4.11589976826166,22.1741488021234,0.));
#246574=CARTESIAN_POINT('Ctrl Pts',(4.11589976826166,22.1741488021234,12.));
#246575=CARTESIAN_POINT('Ctrl Pts',(4.11600589882845,22.1746949858775,0.));
#246576=CARTESIAN_POINT('Ctrl Pts',(4.11600589882845,22.1746949858775,12.));
#246577=CARTESIAN_POINT('Ctrl Pts',(4.11622797217068,22.1758088296598,0.));
#246578=CARTESIAN_POINT('Ctrl Pts',(4.11622797217068,22.1758088296598,12.));
#246579=CARTESIAN_POINT('Ctrl Pts',(4.11653973150518,22.177347426894,0.));
#246580=CARTESIAN_POINT('Ctrl Pts',(4.11653973150518,22.177347426894,12.));
#246581=CARTESIAN_POINT('Ctrl Pts',(4.11694173195003,22.179297473024,0.));
#246582=CARTESIAN_POINT('Ctrl Pts',(4.11694173195003,22.179297473024,12.));
#246583=CARTESIAN_POINT('Ctrl Pts',(4.11743469691756,22.1816414985788,0.));
#246584=CARTESIAN_POINT('Ctrl Pts',(4.11743469691756,22.1816414985788,12.));
#246585=CARTESIAN_POINT('Ctrl Pts',(4.11801938107479,22.1843613164855,0.));
#246586=CARTESIAN_POINT('Ctrl Pts',(4.11801938107479,22.1843613164855,12.));
#246587=CARTESIAN_POINT('Ctrl Pts',(4.11869641271773,22.1874419861496,0.));
#246588=CARTESIAN_POINT('Ctrl Pts',(4.11869641271773,22.1874419861496,12.));
#246589=CARTESIAN_POINT('Ctrl Pts',(4.11946626228636,22.1908725908525,0.));
#246590=CARTESIAN_POINT('Ctrl Pts',(4.11946626228636,22.1908725908525,12.));
#246591=CARTESIAN_POINT('Ctrl Pts',(4.12032932637736,22.1946440958098,0.));
#246592=CARTESIAN_POINT('Ctrl Pts',(4.12032932637736,22.1946440958098,12.));
#246593=CARTESIAN_POINT('Ctrl Pts',(4.12128598183522,22.1987479618246,0.));
#246594=CARTESIAN_POINT('Ctrl Pts',(4.12128598183522,22.1987479618246,12.));
#246595=CARTESIAN_POINT('Ctrl Pts',(4.12233664408227,22.2031746532106,0.));
#246596=CARTESIAN_POINT('Ctrl Pts',(4.12233664408227,22.2031746532106,12.));
#246597=CARTESIAN_POINT('Ctrl Pts',(4.12348173702023,22.2079143941719,0.));
#246598=CARTESIAN_POINT('Ctrl Pts',(4.12348173702023,22.2079143941719,12.));
#246599=CARTESIAN_POINT('Ctrl Pts',(4.12472167516607,22.2129576146671,0.));
#246600=CARTESIAN_POINT('Ctrl Pts',(4.12472167516607,22.2129576146671,12.));
#246601=CARTESIAN_POINT('Ctrl Pts',(4.12605683613307,22.2182956401341,0.));
#246602=CARTESIAN_POINT('Ctrl Pts',(4.12605683613307,22.2182956401341,12.));
#246603=CARTESIAN_POINT('Ctrl Pts',(4.12748755830104,22.2239207458781,0.));
#246604=CARTESIAN_POINT('Ctrl Pts',(4.12748755830104,22.2239207458781,12.));
#246605=CARTESIAN_POINT('Ctrl Pts',(4.12901415463379,22.2298258043947,0.));
#246606=CARTESIAN_POINT('Ctrl Pts',(4.12901415463379,22.2298258043947,12.));
#246607=CARTESIAN_POINT('Ctrl Pts',(4.13063692157498,22.2360040565533,0.));
#246608=CARTESIAN_POINT('Ctrl Pts',(4.13063692157498,22.2360040565533,12.));
#246609=CARTESIAN_POINT('Ctrl Pts',(4.1323561506016,22.2424488153523,0.));
#246610=CARTESIAN_POINT('Ctrl Pts',(4.1323561506016,22.2424488153523,12.));
#246611=CARTESIAN_POINT('Ctrl Pts',(4.1341721255881,22.249153531779,0.));
#246612=CARTESIAN_POINT('Ctrl Pts',(4.1341721255881,22.249153531779,12.));
#246613=CARTESIAN_POINT('Ctrl Pts',(4.13608511977225,22.2561118708421,0.));
#246614=CARTESIAN_POINT('Ctrl Pts',(4.13608511977225,22.2561118708421,12.));
#246615=CARTESIAN_POINT('Ctrl Pts',(4.13809539255421,22.2633177913972,0.));
#246616=CARTESIAN_POINT('Ctrl Pts',(4.13809539255421,22.2633177913972,12.));
#246617=CARTESIAN_POINT('Ctrl Pts',(4.14020318715991,22.2707656042457,0.));
#246618=CARTESIAN_POINT('Ctrl Pts',(4.14020318715991,22.2707656042457,12.));
#246619=CARTESIAN_POINT('Ctrl Pts',(4.14240873321984,22.2784499072027,0.));
#246620=CARTESIAN_POINT('Ctrl Pts',(4.14240873321984,22.2784499072027,12.));
#246621=CARTESIAN_POINT('Ctrl Pts',(4.14471224859295,22.2863655389166,0.));
#246622=CARTESIAN_POINT('Ctrl Pts',(4.14471224859295,22.2863655389166,12.));
#246623=CARTESIAN_POINT('Ctrl Pts',(4.14711394168556,22.2945075198467,0.));
#246624=CARTESIAN_POINT('Ctrl Pts',(4.14711394168556,22.2945075198467,12.));
#246625=CARTESIAN_POINT('Ctrl Pts',(4.14961401285522,22.3028710166933,0.));
#246626=CARTESIAN_POINT('Ctrl Pts',(4.14961401285522,22.3028710166933,12.));
#246627=CARTESIAN_POINT('Ctrl Pts',(4.1522126539699,22.3114513545185,0.));
#246628=CARTESIAN_POINT('Ctrl Pts',(4.1522126539699,22.3114513545185,12.));
#246629=CARTESIAN_POINT('Ctrl Pts',(4.15491004835281,22.3202440186979,0.));
#246630=CARTESIAN_POINT('Ctrl Pts',(4.15491004835281,22.3202440186979,12.));
#246631=CARTESIAN_POINT('Ctrl Pts',(4.15770637047889,22.3292446628959,0.));
#246632=CARTESIAN_POINT('Ctrl Pts',(4.15770637047889,22.3292446628959,12.));
#246633=CARTESIAN_POINT('Ctrl Pts',(4.16060178604164,22.3384491078602,0.));
#246634=CARTESIAN_POINT('Ctrl Pts',(4.16060178604164,22.3384491078602,12.));
#246635=CARTESIAN_POINT('Ctrl Pts',(4.16359645263187,22.3478533253889,0.));
#246636=CARTESIAN_POINT('Ctrl Pts',(4.16359645263187,22.3478533253889,12.));
#246637=CARTESIAN_POINT('Ctrl Pts',(4.166690520266,22.3574534257396,0.));
#246638=CARTESIAN_POINT('Ctrl Pts',(4.166690520266,22.3574534257396,12.));
#246639=CARTESIAN_POINT('Ctrl Pts',(4.16988413199457,22.36724564276,0.));
#246640=CARTESIAN_POINT('Ctrl Pts',(4.16988413199457,22.36724564276,12.));
#246641=CARTESIAN_POINT('Ctrl Pts',(4.17317742436145,22.3772263228617,0.));
#246642=CARTESIAN_POINT('Ctrl Pts',(4.17317742436145,22.3772263228617,12.));
#246643=CARTESIAN_POINT('Ctrl Pts',(4.17657052752825,22.3873919231334,0.));
#246644=CARTESIAN_POINT('Ctrl Pts',(4.17657052752825,22.3873919231334,12.));
#246645=CARTESIAN_POINT('Ctrl Pts',(4.18006356544882,22.3977390078075,0.));
#246646=CARTESIAN_POINT('Ctrl Pts',(4.18006356544882,22.3977390078075,12.));
#246647=CARTESIAN_POINT('Ctrl Pts',(4.1836566560085,22.4082642454453,0.));
#246648=CARTESIAN_POINT('Ctrl Pts',(4.1836566560085,22.4082642454453,12.));
#246649=CARTESIAN_POINT('Ctrl Pts',(4.1873499111772,22.4189644056115,0.));
#246650=CARTESIAN_POINT('Ctrl Pts',(4.1873499111772,22.4189644056115,12.));
#246651=CARTESIAN_POINT('Ctrl Pts',(4.19114343726941,22.4298363535421,0.));
#246652=CARTESIAN_POINT('Ctrl Pts',(4.19114343726941,22.4298363535421,12.));
#246653=CARTESIAN_POINT('Ctrl Pts',(4.1950373351886,22.4408770448917,0.));
#246654=CARTESIAN_POINT('Ctrl Pts',(4.1950373351886,22.4408770448917,12.));
#246655=CARTESIAN_POINT('Ctrl Pts',(4.19903170066354,22.4520835205419,0.));
#246656=CARTESIAN_POINT('Ctrl Pts',(4.19903170066354,22.4520835205419,12.));
#246657=CARTESIAN_POINT('Ctrl Pts',(4.2031266244817,22.4634529011433,0.));
#246658=CARTESIAN_POINT('Ctrl Pts',(4.2031266244817,22.4634529011433,12.));
#246659=CARTESIAN_POINT('Ctrl Pts',(4.20732219265648,22.4749823839915,0.));
#246660=CARTESIAN_POINT('Ctrl Pts',(4.20732219265648,22.4749823839915,12.));
#246661=CARTESIAN_POINT('Ctrl Pts',(4.21161848657428,22.4866692403147,0.));
#246662=CARTESIAN_POINT('Ctrl Pts',(4.21161848657428,22.4866692403147,12.));
#246663=CARTESIAN_POINT('Ctrl Pts',(4.21601558313908,22.4985108124229,0.));
#246664=CARTESIAN_POINT('Ctrl Pts',(4.21601558313908,22.4985108124229,12.));
#246665=CARTESIAN_POINT('Ctrl Pts',(4.22051355490196,22.5105045108882,0.));
#246666=CARTESIAN_POINT('Ctrl Pts',(4.22051355490196,22.5105045108882,12.));
#246667=CARTESIAN_POINT('Ctrl Pts',(4.2251124702004,22.5226478117885,0.));
#246668=CARTESIAN_POINT('Ctrl Pts',(4.2251124702004,22.5226478117885,12.));
#246669=CARTESIAN_POINT('Ctrl Pts',(4.22981239330731,22.5349382540587,0.));
#246670=CARTESIAN_POINT('Ctrl Pts',(4.22981239330731,22.5349382540587,12.));
#246671=CARTESIAN_POINT('Ctrl Pts',(4.23461338456713,22.5473734368086,0.));
#246672=CARTESIAN_POINT('Ctrl Pts',(4.23461338456713,22.5473734368086,12.));
#246673=CARTESIAN_POINT('Ctrl Pts',(4.23951550052526,22.559951016643,0.));
#246674=CARTESIAN_POINT('Ctrl Pts',(4.23951550052526,22.559951016643,12.));
#246675=CARTESIAN_POINT('Ctrl Pts',(4.24451879404858,22.5726687049922,0.));
#246676=CARTESIAN_POINT('Ctrl Pts',(4.24451879404858,22.5726687049922,12.));
#246677=CARTESIAN_POINT('Ctrl Pts',(4.24962331444184,22.5855242662479,0.));
#246678=CARTESIAN_POINT('Ctrl Pts',(4.24962331444184,22.5855242662479,12.));
#246679=CARTESIAN_POINT('Ctrl Pts',(4.25482910755485,22.5985155158637,0.));
#246680=CARTESIAN_POINT('Ctrl Pts',(4.25482910755485,22.5985155158637,12.));
#246681=CARTESIAN_POINT('Ctrl Pts',(4.26013621588303,22.611640318482,0.));
#246682=CARTESIAN_POINT('Ctrl Pts',(4.26013621588303,22.611640318482,12.));
#246683=CARTESIAN_POINT('Ctrl Pts',(4.26554467865571,22.6248965859975,0.));
#246684=CARTESIAN_POINT('Ctrl Pts',(4.26554467865571,22.6248965859975,12.));
#246685=CARTESIAN_POINT('Ctrl Pts',(4.27105453192999,22.6382822758171,0.));
#246686=CARTESIAN_POINT('Ctrl Pts',(4.27105453192999,22.6382822758171,12.));
#246687=CARTESIAN_POINT('Ctrl Pts',(4.27666580869117,22.6517953893303,0.));
#246688=CARTESIAN_POINT('Ctrl Pts',(4.27666580869117,22.6517953893303,12.));
#246689=CARTESIAN_POINT('Ctrl Pts',(4.28237853894059,22.665433970311,0.));
#246690=CARTESIAN_POINT('Ctrl Pts',(4.28237853894059,22.665433970311,12.));
#246691=CARTESIAN_POINT('Ctrl Pts',(4.28819274977766,22.6791961033537,0.));
#246692=CARTESIAN_POINT('Ctrl Pts',(4.28819274977766,22.6791961033537,12.));
#246693=CARTESIAN_POINT('Ctrl Pts',(4.29410846547061,22.6930799122545,0.));
#246694=CARTESIAN_POINT('Ctrl Pts',(4.29410846547061,22.6930799122545,12.));
#246695=CARTESIAN_POINT('Ctrl Pts',(4.30012570754066,22.707083558756,0.));
#246696=CARTESIAN_POINT('Ctrl Pts',(4.30012570754066,22.707083558756,12.));
#246697=CARTESIAN_POINT('Ctrl Pts',(4.30624449484074,22.7212052413384,0.));
#246698=CARTESIAN_POINT('Ctrl Pts',(4.30624449484074,22.7212052413384,12.));
#246699=CARTESIAN_POINT('Ctrl Pts',(4.3124648436255,22.7354431939927,0.));
#246700=CARTESIAN_POINT('Ctrl Pts',(4.3124648436255,22.7354431939927,12.));
#246701=CARTESIAN_POINT('Ctrl Pts',(4.3187867676123,22.7497956849852,0.));
#246702=CARTESIAN_POINT('Ctrl Pts',(4.3187867676123,22.7497956849852,12.));
#246703=CARTESIAN_POINT('Ctrl Pts',(4.32521027803747,22.764261015648,0.));
#246704=CARTESIAN_POINT('Ctrl Pts',(4.32521027803747,22.764261015648,12.));
#246705=CARTESIAN_POINT('Ctrl Pts',(4.33173538373182,22.7788375194081,0.));
#246706=CARTESIAN_POINT('Ctrl Pts',(4.33173538373182,22.7788375194081,12.));
#246707=CARTESIAN_POINT('Ctrl Pts',(4.33836209118442,22.7935235607807,0.));
#246708=CARTESIAN_POINT('Ctrl Pts',(4.33836209118442,22.7935235607807,12.));
#246709=CARTESIAN_POINT('Ctrl Pts',(4.34509040460065,22.808317534379,0.));
#246710=CARTESIAN_POINT('Ctrl Pts',(4.34509040460065,22.808317534379,12.));
#246711=CARTESIAN_POINT('Ctrl Pts',(4.35192032594801,22.8232178638873,0.));
#246712=CARTESIAN_POINT('Ctrl Pts',(4.35192032594801,22.8232178638873,12.));
#246713=CARTESIAN_POINT('Ctrl Pts',(4.35885185500559,22.838223001118,0.));
#246714=CARTESIAN_POINT('Ctrl Pts',(4.35885185500559,22.838223001118,12.));
#246715=CARTESIAN_POINT('Ctrl Pts',(4.36588498943009,22.8533314252419,0.));
#246716=CARTESIAN_POINT('Ctrl Pts',(4.36588498943009,22.8533314252419,12.));
#246717=CARTESIAN_POINT('Ctrl Pts',(4.37301972480752,22.8685416419725,0.));
#246718=CARTESIAN_POINT('Ctrl Pts',(4.37301972480752,22.8685416419725,12.));
#246719=CARTESIAN_POINT('Ctrl Pts',(4.38025605470089,22.8838521827702,0.));
#246720=CARTESIAN_POINT('Ctrl Pts',(4.38025605470089,22.8838521827702,12.));
#246721=CARTESIAN_POINT('Ctrl Pts',(4.38759397068391,22.8992616040108,0.));
#246722=CARTESIAN_POINT('Ctrl Pts',(4.38759397068391,22.8992616040108,12.));
#246723=CARTESIAN_POINT('Ctrl Pts',(4.39503346238454,22.9147684862425,0.));
#246724=CARTESIAN_POINT('Ctrl Pts',(4.39503346238454,22.9147684862425,12.));
#246725=CARTESIAN_POINT('Ctrl Pts',(4.40257451754307,22.9303714335549,0.));
#246726=CARTESIAN_POINT('Ctrl Pts',(4.40257451754307,22.9303714335549,12.));
#246727=CARTESIAN_POINT('Ctrl Pts',(4.41021712205547,22.9460690729093,0.));
#246728=CARTESIAN_POINT('Ctrl Pts',(4.41021712205547,22.9460690729093,12.));
#246729=CARTESIAN_POINT('Ctrl Pts',(4.41796126001309,22.9618600534866,0.));
#246730=CARTESIAN_POINT('Ctrl Pts',(4.41796126001309,22.9618600534866,12.));
#246731=CARTESIAN_POINT('Ctrl Pts',(4.42580691372771,22.9777430460021,0.));
#246732=CARTESIAN_POINT('Ctrl Pts',(4.42580691372771,22.9777430460021,12.));
#246733=CARTESIAN_POINT('Ctrl Pts',(4.43375406376904,22.9937167421009,0.));
#246734=CARTESIAN_POINT('Ctrl Pts',(4.43375406376904,22.9937167421009,12.));
#246735=CARTESIAN_POINT('Ctrl Pts',(4.44180268901666,23.0097798538399,0.));
#246736=CARTESIAN_POINT('Ctrl Pts',(4.44180268901666,23.0097798538399,12.));
#246737=CARTESIAN_POINT('Ctrl Pts',(4.44995276669698,23.0259311131395,0.));
#246738=CARTESIAN_POINT('Ctrl Pts',(4.44995276669698,23.0259311131395,12.));
#246739=CARTESIAN_POINT('Ctrl Pts',(4.45820427241676,23.0421692712466,0.));
#246740=CARTESIAN_POINT('Ctrl Pts',(4.45820427241676,23.0421692712466,12.));
#246741=CARTESIAN_POINT('Ctrl Pts',(4.46655718018205,23.0584930981723,0.));
#246742=CARTESIAN_POINT('Ctrl Pts',(4.46655718018205,23.0584930981723,12.));
#246743=CARTESIAN_POINT('Ctrl Pts',(4.47501146242821,23.0749013821868,0.));
#246744=CARTESIAN_POINT('Ctrl Pts',(4.47501146242821,23.0749013821868,12.));
#246745=CARTESIAN_POINT('Ctrl Pts',(4.48356709006756,23.0913929293909,0.));
#246746=CARTESIAN_POINT('Ctrl Pts',(4.48356709006756,23.0913929293909,12.));
#246747=CARTESIAN_POINT('Ctrl Pts',(4.49222403252201,23.1079665632629,0.));
#246748=CARTESIAN_POINT('Ctrl Pts',(4.49222403252201,23.1079665632629,12.));
#246749=CARTESIAN_POINT('Ctrl Pts',(4.50098225775178,23.1246211242117,0.));
#246750=CARTESIAN_POINT('Ctrl Pts',(4.50098225775178,23.1246211242117,12.));
#246751=CARTESIAN_POINT('Ctrl Pts',(4.50984173227087,23.1413554691136,0.));
#246752=CARTESIAN_POINT('Ctrl Pts',(4.50984173227087,23.1413554691136,12.));
#246753=CARTESIAN_POINT('Ctrl Pts',(4.51880242116785,23.1581684708778,0.));
#246754=CARTESIAN_POINT('Ctrl Pts',(4.51880242116785,23.1581684708778,12.));
#246755=CARTESIAN_POINT('Ctrl Pts',(4.52786428815047,23.1750590180923,0.));
#246756=CARTESIAN_POINT('Ctrl Pts',(4.52786428815047,23.1750590180923,12.));
#246757=CARTESIAN_POINT('Ctrl Pts',(4.53702729557585,23.1920260146474,0.));
#246758=CARTESIAN_POINT('Ctrl Pts',(4.53702729557585,23.1920260146474,12.));
#246759=CARTESIAN_POINT('Ctrl Pts',(4.54629140447542,23.2090683793627,0.));
#246760=CARTESIAN_POINT('Ctrl Pts',(4.54629140447542,23.2090683793627,12.));
#246761=CARTESIAN_POINT('Ctrl Pts',(4.55565657456956,23.2261850456055,0.));
#246762=CARTESIAN_POINT('Ctrl Pts',(4.55565657456956,23.2261850456055,12.));
#246763=CARTESIAN_POINT('Ctrl Pts',(4.5651227642781,23.2433749609117,0.));
#246764=CARTESIAN_POINT('Ctrl Pts',(4.5651227642781,23.2433749609117,12.));
#246765=CARTESIAN_POINT('Ctrl Pts',(4.5746899307607,23.2606370866853,0.));
#246766=CARTESIAN_POINT('Ctrl Pts',(4.5746899307607,23.2606370866853,12.));
#246767=CARTESIAN_POINT('Ctrl Pts',(4.58435802994674,23.2779703978868,0.));
#246768=CARTESIAN_POINT('Ctrl Pts',(4.58435802994674,23.2779703978868,12.));
#246769=CARTESIAN_POINT('Ctrl Pts',(4.59412701655749,23.295373882719,0.));
#246770=CARTESIAN_POINT('Ctrl Pts',(4.59412701655749,23.295373882719,12.));
#246771=CARTESIAN_POINT('Ctrl Pts',(4.60399684412174,23.3128465423119,0.));
#246772=CARTESIAN_POINT('Ctrl Pts',(4.60399684412174,23.3128465423119,12.));
#246773=CARTESIAN_POINT('Ctrl Pts',(4.61396746497848,23.3303873903947,0.));
#246774=CARTESIAN_POINT('Ctrl Pts',(4.61396746497848,23.3303873903947,12.));
#246775=CARTESIAN_POINT('Ctrl Pts',(4.62403883030823,23.3479954530281,0.));
#246776=CARTESIAN_POINT('Ctrl Pts',(4.62403883030823,23.3479954530281,12.));
#246777=CARTESIAN_POINT('Ctrl Pts',(4.63421089016554,23.3656697683496,0.));
#246778=CARTESIAN_POINT('Ctrl Pts',(4.63421089016554,23.3656697683496,12.));
#246779=CARTESIAN_POINT('Ctrl Pts',(4.64448359349935,23.383409386307,0.));
#246780=CARTESIAN_POINT('Ctrl Pts',(4.64448359349935,23.383409386307,12.));
#246781=CARTESIAN_POINT('Ctrl Pts',(4.65485688816921,23.4012133683957,0.));
#246782=CARTESIAN_POINT('Ctrl Pts',(4.65485688816921,23.4012133683957,12.));
#246783=CARTESIAN_POINT('Ctrl Pts',(4.66533072094663,23.4190807873798,0.));
#246784=CARTESIAN_POINT('Ctrl Pts',(4.66533072094663,23.4190807873798,12.));
#246785=CARTESIAN_POINT('Ctrl Pts',(4.6759050375305,23.4370107270444,0.));
#246786=CARTESIAN_POINT('Ctrl Pts',(4.6759050375305,23.4370107270444,12.));
#246787=CARTESIAN_POINT('Ctrl Pts',(4.68657978258297,23.4550022819853,0.));
#246788=CARTESIAN_POINT('Ctrl Pts',(4.68657978258297,23.4550022819853,12.));
#246789=CARTESIAN_POINT('Ctrl Pts',(4.69735489975023,23.4730545573849,0.));
#246790=CARTESIAN_POINT('Ctrl Pts',(4.69735489975023,23.4730545573849,12.));
#246791=CARTESIAN_POINT('Ctrl Pts',(4.7082303316782,23.491166668789,0.));
#246792=CARTESIAN_POINT('Ctrl Pts',(4.7082303316782,23.491166668789,12.));
#246793=CARTESIAN_POINT('Ctrl Pts',(4.71920602001904,23.5093377418784,0.));
#246794=CARTESIAN_POINT('Ctrl Pts',(4.71920602001904,23.5093377418784,12.));
#246795=CARTESIAN_POINT('Ctrl Pts',(4.73028190543031,23.5275669122378,0.));
#246796=CARTESIAN_POINT('Ctrl Pts',(4.73028190543031,23.5275669122378,12.));
#246797=CARTESIAN_POINT('Ctrl Pts',(4.74145792760698,23.5458533251715,0.));
#246798=CARTESIAN_POINT('Ctrl Pts',(4.74145792760698,23.5458533251715,12.));
#246799=CARTESIAN_POINT('Ctrl Pts',(4.75273402530615,23.564196135517,0.));
#246800=CARTESIAN_POINT('Ctrl Pts',(4.75273402530615,23.564196135517,12.));
#246801=CARTESIAN_POINT('Ctrl Pts',(4.7641101363625,23.5825945074535,0.));
#246802=CARTESIAN_POINT('Ctrl Pts',(4.7641101363625,23.5825945074535,12.));
#246803=CARTESIAN_POINT('Ctrl Pts',(4.77558619769875,23.6010476143099,0.));
#246804=CARTESIAN_POINT('Ctrl Pts',(4.77558619769875,23.6010476143099,12.));
#246805=CARTESIAN_POINT('Ctrl Pts',(4.78716214532104,23.6195546383625,0.));
#246806=CARTESIAN_POINT('Ctrl Pts',(4.78716214532104,23.6195546383625,12.));
#246807=CARTESIAN_POINT('Ctrl Pts',(4.79883791433229,23.6381147706581,0.));
#246808=CARTESIAN_POINT('Ctrl Pts',(4.79883791433229,23.6381147706581,12.));
#246809=CARTESIAN_POINT('Ctrl Pts',(4.81061343896442,23.6567272108631,0.));
#246810=CARTESIAN_POINT('Ctrl Pts',(4.81061343896442,23.6567272108631,12.));
#246811=CARTESIAN_POINT('Ctrl Pts',(4.82248865259569,23.6753911671023,0.));
#246812=CARTESIAN_POINT('Ctrl Pts',(4.82248865259569,23.6753911671023,12.));
#246813=CARTESIAN_POINT('Ctrl Pts',(4.83446348776267,23.6941058557971,0.));
#246814=CARTESIAN_POINT('Ctrl Pts',(4.83446348776267,23.6941058557971,12.));
#246815=CARTESIAN_POINT('Ctrl Pts',(4.84653787616422,23.7128705015014,0.));
#246816=CARTESIAN_POINT('Ctrl Pts',(4.84653787616422,23.7128705015014,12.));
#246817=CARTESIAN_POINT('Ctrl Pts',(4.85871174865491,23.7316843367308,0.));
#246818=CARTESIAN_POINT('Ctrl Pts',(4.85871174865491,23.7316843367308,12.));
#246819=CARTESIAN_POINT('Ctrl Pts',(4.87098503527142,23.7505466018239,0.));
#246820=CARTESIAN_POINT('Ctrl Pts',(4.87098503527142,23.7505466018239,12.));
#246821=CARTESIAN_POINT('Ctrl Pts',(4.88335766525565,23.7694565448044,0.));
#246822=CARTESIAN_POINT('Ctrl Pts',(4.88335766525565,23.7694565448044,12.));
#246823=CARTESIAN_POINT('Ctrl Pts',(4.89582956706771,23.7884134212381,0.));
#246824=CARTESIAN_POINT('Ctrl Pts',(4.89582956706771,23.7884134212381,12.));
#246825=CARTESIAN_POINT('Ctrl Pts',(4.90840066839346,23.8074164940897,0.));
#246826=CARTESIAN_POINT('Ctrl Pts',(4.90840066839346,23.8074164940897,12.));
#246827=CARTESIAN_POINT('Ctrl Pts',(4.92107089613976,23.8264650335721,0.));
#246828=CARTESIAN_POINT('Ctrl Pts',(4.92107089613976,23.8264650335721,12.));
#246829=CARTESIAN_POINT('Ctrl Pts',(4.93384017643441,23.8455583170062,0.));
#246830=CARTESIAN_POINT('Ctrl Pts',(4.93384017643441,23.8455583170062,12.));
#246831=CARTESIAN_POINT('Ctrl Pts',(4.94670843465868,23.8646956287172,0.));
#246832=CARTESIAN_POINT('Ctrl Pts',(4.94670843465868,23.8646956287172,12.));
#246833=CARTESIAN_POINT('Ctrl Pts',(4.95967559546565,23.883876259922,0.));
#246834=CARTESIAN_POINT('Ctrl Pts',(4.95967559546565,23.883876259922,12.));
#246835=CARTESIAN_POINT('Ctrl Pts',(4.97274158279228,23.9030995086164,0.));
#246836=CARTESIAN_POINT('Ctrl Pts',(4.97274158279228,23.9030995086164,12.));
#246837=CARTESIAN_POINT('Ctrl Pts',(4.98590631986532,23.9223646794591,0.));
#246838=CARTESIAN_POINT('Ctrl Pts',(4.98590631986532,23.9223646794591,12.));
#246839=CARTESIAN_POINT('Ctrl Pts',(4.99916972919309,23.9416710836529,0.));
#246840=CARTESIAN_POINT('Ctrl Pts',(4.99916972919309,23.9416710836529,12.));
#246841=CARTESIAN_POINT('Ctrl Pts',(5.01253173257458,23.9610180388271,0.));
#246842=CARTESIAN_POINT('Ctrl Pts',(5.01253173257458,23.9610180388271,12.));
#246843=CARTESIAN_POINT('Ctrl Pts',(5.02599225112461,23.9804048689228,0.));
#246844=CARTESIAN_POINT('Ctrl Pts',(5.02599225112461,23.9804048689228,12.));
#246845=CARTESIAN_POINT('Ctrl Pts',(5.03955120528527,23.9998309040747,0.));
#246846=CARTESIAN_POINT('Ctrl Pts',(5.03955120528527,23.9998309040747,12.));
#246847=CARTESIAN_POINT('Ctrl Pts',(5.05320851483068,24.0192954804896,0.));
#246848=CARTESIAN_POINT('Ctrl Pts',(5.05320851483068,24.0192954804896,12.));
#246849=CARTESIAN_POINT('Ctrl Pts',(5.06696409886639,24.0387979403268,0.));
#246850=CARTESIAN_POINT('Ctrl Pts',(5.06696409886639,24.0387979403268,12.));
#246851=CARTESIAN_POINT('Ctrl Pts',(5.0808178758127,24.0583376315636,0.));
#246852=CARTESIAN_POINT('Ctrl Pts',(5.0808178758127,24.0583376315636,12.));
#246853=CARTESIAN_POINT('Ctrl Pts',(5.09476976342616,24.0779139079264,0.));
#246854=CARTESIAN_POINT('Ctrl Pts',(5.09476976342616,24.0779139079264,12.));
#246855=CARTESIAN_POINT('Ctrl Pts',(5.10881967883124,24.0975261288444,0.));
#246856=CARTESIAN_POINT('Ctrl Pts',(5.10881967883124,24.0975261288444,12.));
#246857=CARTESIAN_POINT('Ctrl Pts',(5.12296753853857,24.117173659394,0.));
#246858=CARTESIAN_POINT('Ctrl Pts',(5.12296753853857,24.117173659394,12.));
#246859=CARTESIAN_POINT('Ctrl Pts',(5.13721325845745,24.1368558702443,0.));
#246860=CARTESIAN_POINT('Ctrl Pts',(5.13721325845745,24.1368558702443,12.));
#246861=CARTESIAN_POINT('Ctrl Pts',(5.15155675390079,24.1565721375971,0.));
#246862=CARTESIAN_POINT('Ctrl Pts',(5.15155675390079,24.1565721375971,12.));
#246863=CARTESIAN_POINT('Ctrl Pts',(5.16599793957985,24.1763218431344,0.));
#246864=CARTESIAN_POINT('Ctrl Pts',(5.16599793957985,24.1763218431344,12.));
#246865=CARTESIAN_POINT('Ctrl Pts',(5.18053672961398,24.1961043738756,0.));
#246866=CARTESIAN_POINT('Ctrl Pts',(5.18053672961398,24.1961043738756,12.));
#246867=CARTESIAN_POINT('Ctrl Pts',(5.19517303753647,24.2159191220171,0.));
#246868=CARTESIAN_POINT('Ctrl Pts',(5.19517303753647,24.2159191220171,12.));
#246869=CARTESIAN_POINT('Ctrl Pts',(5.20990677629176,24.2357654847766,0.));
#246870=CARTESIAN_POINT('Ctrl Pts',(5.20990677629176,24.2357654847766,12.));
#246871=CARTESIAN_POINT('Ctrl Pts',(5.22473785822442,24.2556428642294,0.));
#246872=CARTESIAN_POINT('Ctrl Pts',(5.22473785822442,24.2556428642294,12.));
#246873=CARTESIAN_POINT('Ctrl Pts',(5.23966619506289,24.2755506671525,0.));
#246874=CARTESIAN_POINT('Ctrl Pts',(5.23966619506289,24.2755506671525,12.));
#246875=CARTESIAN_POINT('Ctrl Pts',(5.25469169788856,24.2954883048447,0.));
#246876=CARTESIAN_POINT('Ctrl Pts',(5.25469169788856,24.2954883048447,12.));
#246877=CARTESIAN_POINT('Ctrl Pts',(5.26981427718798,24.3154551932221,0.));
#246878=CARTESIAN_POINT('Ctrl Pts',(5.26981427718798,24.3154551932221,12.));
#246879=CARTESIAN_POINT('Ctrl Pts',(5.28503384290648,24.3354507529414,0.));
#246880=CARTESIAN_POINT('Ctrl Pts',(5.28503384290648,24.3354507529414,12.));
#246881=CARTESIAN_POINT('Ctrl Pts',(5.30035030449063,24.3554744095075,0.));
#246882=CARTESIAN_POINT('Ctrl Pts',(5.30035030449063,24.3554744095075,12.));
#246883=CARTESIAN_POINT('Ctrl Pts',(5.31576357092526,24.3755255933917,0.));
#246884=CARTESIAN_POINT('Ctrl Pts',(5.31576357092526,24.3755255933917,12.));
#246885=CARTESIAN_POINT('Ctrl Pts',(5.33127355076033,24.3956037401293,0.));
#246886=CARTESIAN_POINT('Ctrl Pts',(5.33127355076033,24.3956037401293,12.));
#246887=CARTESIAN_POINT('Ctrl Pts',(5.34688015213537,24.4157082904614,0.));
#246888=CARTESIAN_POINT('Ctrl Pts',(5.34688015213537,24.4157082904614,12.));
#246889=CARTESIAN_POINT('Ctrl Pts',(5.36258328273627,24.435838689915,0.));
#246890=CARTESIAN_POINT('Ctrl Pts',(5.36258328273627,24.435838689915,12.));
#246891=CARTESIAN_POINT('Ctrl Pts',(5.37838284973695,24.4559943883157,0.));
#246892=CARTESIAN_POINT('Ctrl Pts',(5.37838284973695,24.4559943883157,12.));
#246893=CARTESIAN_POINT('Ctrl Pts',(5.39427875973824,24.4761748393321,0.));
#246894=CARTESIAN_POINT('Ctrl Pts',(5.39427875973824,24.4761748393321,12.));
#246895=CARTESIAN_POINT('Ctrl Pts',(5.41027091869241,24.4963794999831,0.));
#246896=CARTESIAN_POINT('Ctrl Pts',(5.41027091869241,24.4963794999831,12.));
#246897=CARTESIAN_POINT('Ctrl Pts',(5.42635923183419,24.5166078302108,0.));
#246898=CARTESIAN_POINT('Ctrl Pts',(5.42635923183419,24.5166078302108,12.));
#246899=CARTESIAN_POINT('Ctrl Pts',(5.4425436035688,24.5368592922863,0.));
#246900=CARTESIAN_POINT('Ctrl Pts',(5.4425436035688,24.5368592922863,12.));
#246901=CARTESIAN_POINT('Ctrl Pts',(5.45882393762261,24.5571333514842,0.));
#246902=CARTESIAN_POINT('Ctrl Pts',(5.45882393762261,24.5571333514842,12.));
#246903=CARTESIAN_POINT('Ctrl Pts',(5.47520013724419,24.5774294770329,0.));
#246904=CARTESIAN_POINT('Ctrl Pts',(5.47520013724419,24.5774294770329,12.));
#246905=CARTESIAN_POINT('Ctrl Pts',(5.49167210537246,24.5977471429364,0.));
#246906=CARTESIAN_POINT('Ctrl Pts',(5.49167210537246,24.5977471429364,12.));
#246907=CARTESIAN_POINT('Ctrl Pts',(5.50823974481962,24.6180858289179,0.));
#246908=CARTESIAN_POINT('Ctrl Pts',(5.50823974481962,24.6180858289179,12.));
#246909=CARTESIAN_POINT('Ctrl Pts',(5.52490295840991,24.6384450211467,0.));
#246910=CARTESIAN_POINT('Ctrl Pts',(5.52490295840991,24.6384450211467,12.));
#246911=CARTESIAN_POINT('Ctrl Pts',(5.54166164919583,24.6588242134738,0.));
#246912=CARTESIAN_POINT('Ctrl Pts',(5.54166164919583,24.6588242134738,12.));
#246913=CARTESIAN_POINT('Ctrl Pts',(5.55851572025376,24.6792229061794,0.));
#246914=CARTESIAN_POINT('Ctrl Pts',(5.55851572025376,24.6792229061794,12.));
#246915=CARTESIAN_POINT('Ctrl Pts',(5.57546507427754,24.6996406035517,0.));
#246916=CARTESIAN_POINT('Ctrl Pts',(5.57546507427754,24.6996406035517,12.));
#246917=CARTESIAN_POINT('Ctrl Pts',(5.59250961323987,24.7200768119088,0.));
#246918=CARTESIAN_POINT('Ctrl Pts',(5.59250961323987,24.7200768119088,12.));
#246919=CARTESIAN_POINT('Ctrl Pts',(5.60964923798491,24.7405310372739,0.));
#246920=CARTESIAN_POINT('Ctrl Pts',(5.60964923798491,24.7405310372739,12.));
#246921=CARTESIAN_POINT('Ctrl Pts',(5.62688384790923,24.7610027835697,0.));
#246922=CARTESIAN_POINT('Ctrl Pts',(5.62688384790923,24.7610027835697,12.));
#246923=CARTESIAN_POINT('Ctrl Pts',(5.6442133404226,24.781491549672,0.));
#246924=CARTESIAN_POINT('Ctrl Pts',(5.6442133404226,24.781491549672,12.));
#246925=CARTESIAN_POINT('Ctrl Pts',(5.66163761114921,24.8019968304605,0.));
#246926=CARTESIAN_POINT('Ctrl Pts',(5.66163761114921,24.8019968304605,12.));
#246927=CARTESIAN_POINT('Ctrl Pts',(5.67915655496542,24.8225181223845,0.));
#246928=CARTESIAN_POINT('Ctrl Pts',(5.67915655496542,24.8225181223845,12.));
#246929=CARTESIAN_POINT('Ctrl Pts',(5.69677006679444,24.8430549277621,0.));
#246930=CARTESIAN_POINT('Ctrl Pts',(5.69677006679444,24.8430549277621,12.));
#246931=CARTESIAN_POINT('Ctrl Pts',(5.71447804252027,24.8636067597669,0.));
#246932=CARTESIAN_POINT('Ctrl Pts',(5.71447804252027,24.8636067597669,12.));
#246933=CARTESIAN_POINT('Ctrl Pts',(5.73228037976926,24.884173146722,0.));
#246934=CARTESIAN_POINT('Ctrl Pts',(5.73228037976926,24.884173146722,12.));
#246935=CARTESIAN_POINT('Ctrl Pts',(5.75017697890804,24.904753637648,0.));
#246936=CARTESIAN_POINT('Ctrl Pts',(5.75017697890804,24.904753637648,12.));
#246937=CARTESIAN_POINT('Ctrl Pts',(5.76816774342219,24.9253478043656,0.));
#246938=CARTESIAN_POINT('Ctrl Pts',(5.76816774342219,24.9253478043656,12.));
#246939=CARTESIAN_POINT('Ctrl Pts',(5.78625257775681,24.945955229334,0.));
#246940=CARTESIAN_POINT('Ctrl Pts',(5.78625257775681,24.945955229334,12.));
#246941=CARTESIAN_POINT('Ctrl Pts',(5.80443138549726,24.9665754954496,0.));
#246942=CARTESIAN_POINT('Ctrl Pts',(5.80443138549726,24.9665754954496,12.));
#246943=CARTESIAN_POINT('Ctrl Pts',(5.82270406744198,24.9872081752734,0.));
#246944=CARTESIAN_POINT('Ctrl Pts',(5.82270406744198,24.9872081752734,12.));
#246945=CARTESIAN_POINT('Ctrl Pts',(5.84107051963071,25.0078528200564,0.));
#246946=CARTESIAN_POINT('Ctrl Pts',(5.84107051963071,25.0078528200564,12.));
#246947=CARTESIAN_POINT('Ctrl Pts',(5.85953063156826,25.0285089498899,0.));
#246948=CARTESIAN_POINT('Ctrl Pts',(5.85953063156826,25.0285089498899,12.));
#246949=CARTESIAN_POINT('Ctrl Pts',(5.87808428385365,25.0491760405911,0.));
#246950=CARTESIAN_POINT('Ctrl Pts',(5.87808428385365,25.0491760405911,12.));
#246951=CARTESIAN_POINT('Ctrl Pts',(5.89673135155514,25.0698535426514,0.));
#246952=CARTESIAN_POINT('Ctrl Pts',(5.89673135155514,25.0698535426514,12.));
#246953=CARTESIAN_POINT('Ctrl Pts',(5.91547170844447,25.0905409050773,0.));
#246954=CARTESIAN_POINT('Ctrl Pts',(5.91547170844447,25.0905409050773,12.));
#246955=CARTESIAN_POINT('Ctrl Pts',(5.93430523086834,25.1112375971106,0.));
#246956=CARTESIAN_POINT('Ctrl Pts',(5.93430523086834,25.1112375971106,12.));
#246957=CARTESIAN_POINT('Ctrl Pts',(5.95323180187378,25.1319431317237,0.));
#246958=CARTESIAN_POINT('Ctrl Pts',(5.95323180187378,25.1319431317237,12.));
#246959=CARTESIAN_POINT('Ctrl Pts',(5.97225131495616,25.1526570863092,0.));
#246960=CARTESIAN_POINT('Ctrl Pts',(5.97225131495616,25.1526570863092,12.));
#246961=CARTESIAN_POINT('Ctrl Pts',(5.99136367859754,25.1733791296259,0.));
#246962=CARTESIAN_POINT('Ctrl Pts',(5.99136367859754,25.1733791296259,12.));
#246963=CARTESIAN_POINT('Ctrl Pts',(6.01056881804612,25.1941090269819,0.));
#246964=CARTESIAN_POINT('Ctrl Pts',(6.01056881804612,25.1941090269819,12.));
#246965=CARTESIAN_POINT('Ctrl Pts',(6.02986667389996,25.21484662016,0.));
#246966=CARTESIAN_POINT('Ctrl Pts',(6.02986667389996,25.21484662016,12.));
#246967=CARTESIAN_POINT('Ctrl Pts',(6.04925720151218,25.2355918139032,0.));
#246968=CARTESIAN_POINT('Ctrl Pts',(6.04925720151218,25.2355918139032,12.));
#246969=CARTESIAN_POINT('Ctrl Pts',(6.06484373634546,25.2521940105705,0.));
#246970=CARTESIAN_POINT('Ctrl Pts',(6.06484373634546,25.2521940105705,12.));
#246971=CARTESIAN_POINT('Ctrl Pts',(6.0765753178749,25.2646490489923,0.));
#246972=CARTESIAN_POINT('Ctrl Pts',(6.0765753178749,25.2646490489923,12.));
#246973=CARTESIAN_POINT('Ctrl Pts',(6.08441489609793,25.2729539149517,0.));
#246974=CARTESIAN_POINT('Ctrl Pts',(6.08441489609793,25.2729539149517,12.));
#246975=CARTESIAN_POINT('Ctrl Pts',(6.08833931617699,25.2771067246846,0.));
#246976=CARTESIAN_POINT('Ctrl Pts',(6.08833931617699,25.2771067246846,12.));
#246977=CARTESIAN_POINT('',(6.08833931617699,25.2771067246846,0.));
#246978=CARTESIAN_POINT('Ctrl Pts',(4.11585220600461,22.1738711152697,0.));
#246979=CARTESIAN_POINT('Ctrl Pts',(4.11585194677442,22.173877682324,0.));
#246980=CARTESIAN_POINT('Ctrl Pts',(4.11586035878287,22.1739341411687,0.));
#246981=CARTESIAN_POINT('Ctrl Pts',(4.11589976826166,22.1741488021234,0.));
#246982=CARTESIAN_POINT('Ctrl Pts',(4.11600589882845,22.1746949858775,0.));
#246983=CARTESIAN_POINT('Ctrl Pts',(4.11622797217068,22.1758088296598,0.));
#246984=CARTESIAN_POINT('Ctrl Pts',(4.11653973150518,22.177347426894,0.));
#246985=CARTESIAN_POINT('Ctrl Pts',(4.11694173195003,22.179297473024,0.));
#246986=CARTESIAN_POINT('Ctrl Pts',(4.11743469691756,22.1816414985788,0.));
#246987=CARTESIAN_POINT('Ctrl Pts',(4.11801938107479,22.1843613164855,0.));
#246988=CARTESIAN_POINT('Ctrl Pts',(4.11869641271773,22.1874419861496,0.));
#246989=CARTESIAN_POINT('Ctrl Pts',(4.11946626228636,22.1908725908525,0.));
#246990=CARTESIAN_POINT('Ctrl Pts',(4.12032932637736,22.1946440958098,0.));
#246991=CARTESIAN_POINT('Ctrl Pts',(4.12128598183522,22.1987479618246,0.));
#246992=CARTESIAN_POINT('Ctrl Pts',(4.12233664408227,22.2031746532106,0.));
#246993=CARTESIAN_POINT('Ctrl Pts',(4.12348173702023,22.2079143941719,0.));
#246994=CARTESIAN_POINT('Ctrl Pts',(4.12472167516607,22.2129576146671,0.));
#246995=CARTESIAN_POINT('Ctrl Pts',(4.12605683613307,22.2182956401341,0.));
#246996=CARTESIAN_POINT('Ctrl Pts',(4.12748755830104,22.2239207458781,0.));
#246997=CARTESIAN_POINT('Ctrl Pts',(4.12901415463379,22.2298258043947,0.));
#246998=CARTESIAN_POINT('Ctrl Pts',(4.13063692157498,22.2360040565533,0.));
#246999=CARTESIAN_POINT('Ctrl Pts',(4.1323561506016,22.2424488153523,0.));
#247000=CARTESIAN_POINT('Ctrl Pts',(4.1341721255881,22.249153531779,0.));
#247001=CARTESIAN_POINT('Ctrl Pts',(4.13608511977225,22.2561118708421,0.));
#247002=CARTESIAN_POINT('Ctrl Pts',(4.13809539255421,22.2633177913972,0.));
#247003=CARTESIAN_POINT('Ctrl Pts',(4.14020318715991,22.2707656042457,0.));
#247004=CARTESIAN_POINT('Ctrl Pts',(4.14240873321984,22.2784499072027,0.));
#247005=CARTESIAN_POINT('Ctrl Pts',(4.14471224859295,22.2863655389166,0.));
#247006=CARTESIAN_POINT('Ctrl Pts',(4.14711394168556,22.2945075198467,0.));
#247007=CARTESIAN_POINT('Ctrl Pts',(4.14961401285522,22.3028710166933,0.));
#247008=CARTESIAN_POINT('Ctrl Pts',(4.1522126539699,22.3114513545185,0.));
#247009=CARTESIAN_POINT('Ctrl Pts',(4.15491004835281,22.3202440186979,0.));
#247010=CARTESIAN_POINT('Ctrl Pts',(4.15770637047889,22.3292446628959,0.));
#247011=CARTESIAN_POINT('Ctrl Pts',(4.16060178604164,22.3384491078602,0.));
#247012=CARTESIAN_POINT('Ctrl Pts',(4.16359645263187,22.3478533253889,0.));
#247013=CARTESIAN_POINT('Ctrl Pts',(4.166690520266,22.3574534257396,0.));
#247014=CARTESIAN_POINT('Ctrl Pts',(4.16988413199457,22.36724564276,0.));
#247015=CARTESIAN_POINT('Ctrl Pts',(4.17317742436145,22.3772263228617,0.));
#247016=CARTESIAN_POINT('Ctrl Pts',(4.17657052752825,22.3873919231334,0.));
#247017=CARTESIAN_POINT('Ctrl Pts',(4.18006356544882,22.3977390078075,0.));
#247018=CARTESIAN_POINT('Ctrl Pts',(4.1836566560085,22.4082642454453,0.));
#247019=CARTESIAN_POINT('Ctrl Pts',(4.1873499111772,22.4189644056115,0.));
#247020=CARTESIAN_POINT('Ctrl Pts',(4.19114343726941,22.4298363535421,0.));
#247021=CARTESIAN_POINT('Ctrl Pts',(4.1950373351886,22.4408770448917,0.));
#247022=CARTESIAN_POINT('Ctrl Pts',(4.19903170066354,22.4520835205419,0.));
#247023=CARTESIAN_POINT('Ctrl Pts',(4.2031266244817,22.4634529011433,0.));
#247024=CARTESIAN_POINT('Ctrl Pts',(4.20732219265648,22.4749823839915,0.));
#247025=CARTESIAN_POINT('Ctrl Pts',(4.21161848657428,22.4866692403147,0.));
#247026=CARTESIAN_POINT('Ctrl Pts',(4.21601558313908,22.4985108124229,0.));
#247027=CARTESIAN_POINT('Ctrl Pts',(4.22051355490196,22.5105045108882,0.));
#247028=CARTESIAN_POINT('Ctrl Pts',(4.2251124702004,22.5226478117885,0.));
#247029=CARTESIAN_POINT('Ctrl Pts',(4.22981239330731,22.5349382540587,0.));
#247030=CARTESIAN_POINT('Ctrl Pts',(4.23461338456713,22.5473734368086,0.));
#247031=CARTESIAN_POINT('Ctrl Pts',(4.23951550052526,22.559951016643,0.));
#247032=CARTESIAN_POINT('Ctrl Pts',(4.24451879404858,22.5726687049922,0.));
#247033=CARTESIAN_POINT('Ctrl Pts',(4.24962331444184,22.5855242662479,0.));
#247034=CARTESIAN_POINT('Ctrl Pts',(4.25482910755485,22.5985155158637,0.));
#247035=CARTESIAN_POINT('Ctrl Pts',(4.26013621588303,22.611640318482,0.));
#247036=CARTESIAN_POINT('Ctrl Pts',(4.26554467865571,22.6248965859975,0.));
#247037=CARTESIAN_POINT('Ctrl Pts',(4.27105453192999,22.6382822758171,0.));
#247038=CARTESIAN_POINT('Ctrl Pts',(4.27666580869117,22.6517953893303,0.));
#247039=CARTESIAN_POINT('Ctrl Pts',(4.28237853894059,22.665433970311,0.));
#247040=CARTESIAN_POINT('Ctrl Pts',(4.28819274977766,22.6791961033537,0.));
#247041=CARTESIAN_POINT('Ctrl Pts',(4.29410846547061,22.6930799122545,0.));
#247042=CARTESIAN_POINT('Ctrl Pts',(4.30012570754066,22.707083558756,0.));
#247043=CARTESIAN_POINT('Ctrl Pts',(4.30624449484074,22.7212052413384,0.));
#247044=CARTESIAN_POINT('Ctrl Pts',(4.3124648436255,22.7354431939927,0.));
#247045=CARTESIAN_POINT('Ctrl Pts',(4.3187867676123,22.7497956849852,0.));
#247046=CARTESIAN_POINT('Ctrl Pts',(4.32521027803747,22.764261015648,0.));
#247047=CARTESIAN_POINT('Ctrl Pts',(4.33173538373182,22.7788375194081,0.));
#247048=CARTESIAN_POINT('Ctrl Pts',(4.33836209118442,22.7935235607807,0.));
#247049=CARTESIAN_POINT('Ctrl Pts',(4.34509040460065,22.808317534379,0.));
#247050=CARTESIAN_POINT('Ctrl Pts',(4.35192032594801,22.8232178638873,0.));
#247051=CARTESIAN_POINT('Ctrl Pts',(4.35885185500559,22.838223001118,0.));
#247052=CARTESIAN_POINT('Ctrl Pts',(4.36588498943009,22.8533314252419,0.));
#247053=CARTESIAN_POINT('Ctrl Pts',(4.37301972480752,22.8685416419725,0.));
#247054=CARTESIAN_POINT('Ctrl Pts',(4.38025605470089,22.8838521827702,0.));
#247055=CARTESIAN_POINT('Ctrl Pts',(4.38759397068391,22.8992616040108,0.));
#247056=CARTESIAN_POINT('Ctrl Pts',(4.39503346238454,22.9147684862425,0.));
#247057=CARTESIAN_POINT('Ctrl Pts',(4.40257451754307,22.9303714335549,0.));
#247058=CARTESIAN_POINT('Ctrl Pts',(4.41021712205547,22.9460690729093,0.));
#247059=CARTESIAN_POINT('Ctrl Pts',(4.41796126001309,22.9618600534866,0.));
#247060=CARTESIAN_POINT('Ctrl Pts',(4.42580691372771,22.9777430460021,0.));
#247061=CARTESIAN_POINT('Ctrl Pts',(4.43375406376904,22.9937167421009,0.));
#247062=CARTESIAN_POINT('Ctrl Pts',(4.44180268901666,23.0097798538399,0.));
#247063=CARTESIAN_POINT('Ctrl Pts',(4.44995276669698,23.0259311131395,0.));
#247064=CARTESIAN_POINT('Ctrl Pts',(4.45820427241676,23.0421692712466,0.));
#247065=CARTESIAN_POINT('Ctrl Pts',(4.46655718018205,23.0584930981723,0.));
#247066=CARTESIAN_POINT('Ctrl Pts',(4.47501146242821,23.0749013821868,0.));
#247067=CARTESIAN_POINT('Ctrl Pts',(4.48356709006756,23.0913929293909,0.));
#247068=CARTESIAN_POINT('Ctrl Pts',(4.49222403252201,23.1079665632629,0.));
#247069=CARTESIAN_POINT('Ctrl Pts',(4.50098225775178,23.1246211242117,0.));
#247070=CARTESIAN_POINT('Ctrl Pts',(4.50984173227087,23.1413554691136,0.));
#247071=CARTESIAN_POINT('Ctrl Pts',(4.51880242116785,23.1581684708778,0.));
#247072=CARTESIAN_POINT('Ctrl Pts',(4.52786428815047,23.1750590180923,0.));
#247073=CARTESIAN_POINT('Ctrl Pts',(4.53702729557585,23.1920260146474,0.));
#247074=CARTESIAN_POINT('Ctrl Pts',(4.54629140447542,23.2090683793627,0.));
#247075=CARTESIAN_POINT('Ctrl Pts',(4.55565657456956,23.2261850456055,0.));
#247076=CARTESIAN_POINT('Ctrl Pts',(4.5651227642781,23.2433749609117,0.));
#247077=CARTESIAN_POINT('Ctrl Pts',(4.5746899307607,23.2606370866853,0.));
#247078=CARTESIAN_POINT('Ctrl Pts',(4.58435802994674,23.2779703978868,0.));
#247079=CARTESIAN_POINT('Ctrl Pts',(4.59412701655749,23.295373882719,0.));
#247080=CARTESIAN_POINT('Ctrl Pts',(4.60399684412174,23.3128465423119,0.));
#247081=CARTESIAN_POINT('Ctrl Pts',(4.61396746497848,23.3303873903947,0.));
#247082=CARTESIAN_POINT('Ctrl Pts',(4.62403883030823,23.3479954530281,0.));
#247083=CARTESIAN_POINT('Ctrl Pts',(4.63421089016554,23.3656697683496,0.));
#247084=CARTESIAN_POINT('Ctrl Pts',(4.64448359349935,23.383409386307,0.));
#247085=CARTESIAN_POINT('Ctrl Pts',(4.65485688816921,23.4012133683957,0.));
#247086=CARTESIAN_POINT('Ctrl Pts',(4.66533072094663,23.4190807873798,0.));
#247087=CARTESIAN_POINT('Ctrl Pts',(4.6759050375305,23.4370107270444,0.));
#247088=CARTESIAN_POINT('Ctrl Pts',(4.68657978258297,23.4550022819853,0.));
#247089=CARTESIAN_POINT('Ctrl Pts',(4.69735489975023,23.4730545573849,0.));
#247090=CARTESIAN_POINT('Ctrl Pts',(4.7082303316782,23.491166668789,0.));
#247091=CARTESIAN_POINT('Ctrl Pts',(4.71920602001904,23.5093377418784,0.));
#247092=CARTESIAN_POINT('Ctrl Pts',(4.73028190543031,23.5275669122378,0.));
#247093=CARTESIAN_POINT('Ctrl Pts',(4.74145792760698,23.5458533251715,0.));
#247094=CARTESIAN_POINT('Ctrl Pts',(4.75273402530615,23.564196135517,0.));
#247095=CARTESIAN_POINT('Ctrl Pts',(4.7641101363625,23.5825945074535,0.));
#247096=CARTESIAN_POINT('Ctrl Pts',(4.77558619769875,23.6010476143099,0.));
#247097=CARTESIAN_POINT('Ctrl Pts',(4.78716214532104,23.6195546383625,0.));
#247098=CARTESIAN_POINT('Ctrl Pts',(4.79883791433229,23.6381147706581,0.));
#247099=CARTESIAN_POINT('Ctrl Pts',(4.81061343896442,23.6567272108631,0.));
#247100=CARTESIAN_POINT('Ctrl Pts',(4.82248865259569,23.6753911671023,0.));
#247101=CARTESIAN_POINT('Ctrl Pts',(4.83446348776267,23.6941058557971,0.));
#247102=CARTESIAN_POINT('Ctrl Pts',(4.84653787616422,23.7128705015014,0.));
#247103=CARTESIAN_POINT('Ctrl Pts',(4.85871174865491,23.7316843367308,0.));
#247104=CARTESIAN_POINT('Ctrl Pts',(4.87098503527142,23.7505466018239,0.));
#247105=CARTESIAN_POINT('Ctrl Pts',(4.88335766525565,23.7694565448044,0.));
#247106=CARTESIAN_POINT('Ctrl Pts',(4.89582956706771,23.7884134212381,0.));
#247107=CARTESIAN_POINT('Ctrl Pts',(4.90840066839346,23.8074164940897,0.));
#247108=CARTESIAN_POINT('Ctrl Pts',(4.92107089613976,23.8264650335721,0.));
#247109=CARTESIAN_POINT('Ctrl Pts',(4.93384017643441,23.8455583170062,0.));
#247110=CARTESIAN_POINT('Ctrl Pts',(4.94670843465868,23.8646956287172,0.));
#247111=CARTESIAN_POINT('Ctrl Pts',(4.95967559546565,23.883876259922,0.));
#247112=CARTESIAN_POINT('Ctrl Pts',(4.97274158279228,23.9030995086164,0.));
#247113=CARTESIAN_POINT('Ctrl Pts',(4.98590631986532,23.9223646794591,0.));
#247114=CARTESIAN_POINT('Ctrl Pts',(4.99916972919309,23.9416710836529,0.));
#247115=CARTESIAN_POINT('Ctrl Pts',(5.01253173257458,23.9610180388271,0.));
#247116=CARTESIAN_POINT('Ctrl Pts',(5.02599225112461,23.9804048689228,0.));
#247117=CARTESIAN_POINT('Ctrl Pts',(5.03955120528527,23.9998309040747,0.));
#247118=CARTESIAN_POINT('Ctrl Pts',(5.05320851483068,24.0192954804896,0.));
#247119=CARTESIAN_POINT('Ctrl Pts',(5.06696409886639,24.0387979403268,0.));
#247120=CARTESIAN_POINT('Ctrl Pts',(5.0808178758127,24.0583376315636,0.));
#247121=CARTESIAN_POINT('Ctrl Pts',(5.09476976342616,24.0779139079264,0.));
#247122=CARTESIAN_POINT('Ctrl Pts',(5.10881967883124,24.0975261288444,0.));
#247123=CARTESIAN_POINT('Ctrl Pts',(5.12296753853857,24.117173659394,0.));
#247124=CARTESIAN_POINT('Ctrl Pts',(5.13721325845745,24.1368558702443,0.));
#247125=CARTESIAN_POINT('Ctrl Pts',(5.15155675390079,24.1565721375971,0.));
#247126=CARTESIAN_POINT('Ctrl Pts',(5.16599793957985,24.1763218431344,0.));
#247127=CARTESIAN_POINT('Ctrl Pts',(5.18053672961398,24.1961043738756,0.));
#247128=CARTESIAN_POINT('Ctrl Pts',(5.19517303753647,24.2159191220171,0.));
#247129=CARTESIAN_POINT('Ctrl Pts',(5.20990677629176,24.2357654847766,0.));
#247130=CARTESIAN_POINT('Ctrl Pts',(5.22473785822442,24.2556428642294,0.));
#247131=CARTESIAN_POINT('Ctrl Pts',(5.23966619506289,24.2755506671525,0.));
#247132=CARTESIAN_POINT('Ctrl Pts',(5.25469169788856,24.2954883048447,0.));
#247133=CARTESIAN_POINT('Ctrl Pts',(5.26981427718798,24.3154551932221,0.));
#247134=CARTESIAN_POINT('Ctrl Pts',(5.28503384290648,24.3354507529414,0.));
#247135=CARTESIAN_POINT('Ctrl Pts',(5.30035030449063,24.3554744095075,0.));
#247136=CARTESIAN_POINT('Ctrl Pts',(5.31576357092526,24.3755255933917,0.));
#247137=CARTESIAN_POINT('Ctrl Pts',(5.33127355076033,24.3956037401293,0.));
#247138=CARTESIAN_POINT('Ctrl Pts',(5.34688015213537,24.4157082904614,0.));
#247139=CARTESIAN_POINT('Ctrl Pts',(5.36258328273627,24.435838689915,0.));
#247140=CARTESIAN_POINT('Ctrl Pts',(5.37838284973695,24.4559943883157,0.));
#247141=CARTESIAN_POINT('Ctrl Pts',(5.39427875973824,24.4761748393321,0.));
#247142=CARTESIAN_POINT('Ctrl Pts',(5.41027091869241,24.4963794999831,0.));
#247143=CARTESIAN_POINT('Ctrl Pts',(5.42635923183419,24.5166078302108,0.));
#247144=CARTESIAN_POINT('Ctrl Pts',(5.4425436035688,24.5368592922863,0.));
#247145=CARTESIAN_POINT('Ctrl Pts',(5.45882393762261,24.5571333514842,0.));
#247146=CARTESIAN_POINT('Ctrl Pts',(5.47520013724419,24.5774294770329,0.));
#247147=CARTESIAN_POINT('Ctrl Pts',(5.49167210537246,24.5977471429364,0.));
#247148=CARTESIAN_POINT('Ctrl Pts',(5.50823974481962,24.6180858289179,0.));
#247149=CARTESIAN_POINT('Ctrl Pts',(5.52490295840991,24.6384450211467,0.));
#247150=CARTESIAN_POINT('Ctrl Pts',(5.54166164919583,24.6588242134738,0.));
#247151=CARTESIAN_POINT('Ctrl Pts',(5.55851572025376,24.6792229061794,0.));
#247152=CARTESIAN_POINT('Ctrl Pts',(5.57546507427754,24.6996406035517,0.));
#247153=CARTESIAN_POINT('Ctrl Pts',(5.59250961323987,24.7200768119088,0.));
#247154=CARTESIAN_POINT('Ctrl Pts',(5.60964923798491,24.7405310372739,0.));
#247155=CARTESIAN_POINT('Ctrl Pts',(5.62688384790923,24.7610027835697,0.));
#247156=CARTESIAN_POINT('Ctrl Pts',(5.6442133404226,24.781491549672,0.));
#247157=CARTESIAN_POINT('Ctrl Pts',(5.66163761114921,24.8019968304605,0.));
#247158=CARTESIAN_POINT('Ctrl Pts',(5.67915655496542,24.8225181223845,0.));
#247159=CARTESIAN_POINT('Ctrl Pts',(5.69677006679444,24.8430549277621,0.));
#247160=CARTESIAN_POINT('Ctrl Pts',(5.71447804252027,24.8636067597669,0.));
#247161=CARTESIAN_POINT('Ctrl Pts',(5.73228037976926,24.884173146722,0.));
#247162=CARTESIAN_POINT('Ctrl Pts',(5.75017697890804,24.904753637648,0.));
#247163=CARTESIAN_POINT('Ctrl Pts',(5.76816774342219,24.9253478043656,0.));
#247164=CARTESIAN_POINT('Ctrl Pts',(5.78625257775681,24.945955229334,0.));
#247165=CARTESIAN_POINT('Ctrl Pts',(5.80443138549726,24.9665754954496,0.));
#247166=CARTESIAN_POINT('Ctrl Pts',(5.82270406744198,24.9872081752734,0.));
#247167=CARTESIAN_POINT('Ctrl Pts',(5.84107051963071,25.0078528200564,0.));
#247168=CARTESIAN_POINT('Ctrl Pts',(5.85953063156826,25.0285089498899,0.));
#247169=CARTESIAN_POINT('Ctrl Pts',(5.87808428385365,25.0491760405911,0.));
#247170=CARTESIAN_POINT('Ctrl Pts',(5.89673135155514,25.0698535426514,0.));
#247171=CARTESIAN_POINT('Ctrl Pts',(5.91547170844447,25.0905409050773,0.));
#247172=CARTESIAN_POINT('Ctrl Pts',(5.93430523086834,25.1112375971106,0.));
#247173=CARTESIAN_POINT('Ctrl Pts',(5.95323180187378,25.1319431317237,0.));
#247174=CARTESIAN_POINT('Ctrl Pts',(5.97225131495616,25.1526570863092,0.));
#247175=CARTESIAN_POINT('Ctrl Pts',(5.99136367859754,25.1733791296259,0.));
#247176=CARTESIAN_POINT('Ctrl Pts',(6.01056881804612,25.1941090269819,0.));
#247177=CARTESIAN_POINT('Ctrl Pts',(6.02986667389996,25.21484662016,0.));
#247178=CARTESIAN_POINT('Ctrl Pts',(6.04925720151218,25.2355918139032,0.));
#247179=CARTESIAN_POINT('Ctrl Pts',(6.06484373634546,25.2521940105705,0.));
#247180=CARTESIAN_POINT('Ctrl Pts',(6.0765753178749,25.2646490489923,0.));
#247181=CARTESIAN_POINT('Ctrl Pts',(6.08441489609793,25.2729539149517,0.));
#247182=CARTESIAN_POINT('Ctrl Pts',(6.08833931617699,25.2771067246846,0.));
#247183=CARTESIAN_POINT('',(6.08833931617699,25.2771067246846,12.));
#247184=CARTESIAN_POINT('Ctrl Pts',(6.08833931617699,25.2771067246846,12.));
#247185=CARTESIAN_POINT('Ctrl Pts',(6.08441489609793,25.2729539149517,12.));
#247186=CARTESIAN_POINT('Ctrl Pts',(6.0765753178749,25.2646490489923,12.));
#247187=CARTESIAN_POINT('Ctrl Pts',(6.06484373634546,25.2521940105705,12.));
#247188=CARTESIAN_POINT('Ctrl Pts',(6.04925720151218,25.2355918139032,12.));
#247189=CARTESIAN_POINT('Ctrl Pts',(6.02986667389996,25.21484662016,12.));
#247190=CARTESIAN_POINT('Ctrl Pts',(6.01056881804612,25.1941090269819,12.));
#247191=CARTESIAN_POINT('Ctrl Pts',(5.99136367859754,25.1733791296259,12.));
#247192=CARTESIAN_POINT('Ctrl Pts',(5.97225131495616,25.1526570863092,12.));
#247193=CARTESIAN_POINT('Ctrl Pts',(5.95323180187378,25.1319431317237,12.));
#247194=CARTESIAN_POINT('Ctrl Pts',(5.93430523086834,25.1112375971106,12.));
#247195=CARTESIAN_POINT('Ctrl Pts',(5.91547170844447,25.0905409050773,12.));
#247196=CARTESIAN_POINT('Ctrl Pts',(5.89673135155514,25.0698535426514,12.));
#247197=CARTESIAN_POINT('Ctrl Pts',(5.87808428385365,25.0491760405911,12.));
#247198=CARTESIAN_POINT('Ctrl Pts',(5.85953063156826,25.0285089498899,12.));
#247199=CARTESIAN_POINT('Ctrl Pts',(5.84107051963071,25.0078528200564,12.));
#247200=CARTESIAN_POINT('Ctrl Pts',(5.82270406744198,24.9872081752734,12.));
#247201=CARTESIAN_POINT('Ctrl Pts',(5.80443138549726,24.9665754954496,12.));
#247202=CARTESIAN_POINT('Ctrl Pts',(5.78625257775681,24.945955229334,12.));
#247203=CARTESIAN_POINT('Ctrl Pts',(5.76816774342219,24.9253478043656,12.));
#247204=CARTESIAN_POINT('Ctrl Pts',(5.75017697890804,24.904753637648,12.));
#247205=CARTESIAN_POINT('Ctrl Pts',(5.73228037976926,24.884173146722,12.));
#247206=CARTESIAN_POINT('Ctrl Pts',(5.71447804252027,24.8636067597669,12.));
#247207=CARTESIAN_POINT('Ctrl Pts',(5.69677006679444,24.8430549277621,12.));
#247208=CARTESIAN_POINT('Ctrl Pts',(5.67915655496542,24.8225181223845,12.));
#247209=CARTESIAN_POINT('Ctrl Pts',(5.66163761114921,24.8019968304605,12.));
#247210=CARTESIAN_POINT('Ctrl Pts',(5.6442133404226,24.781491549672,12.));
#247211=CARTESIAN_POINT('Ctrl Pts',(5.62688384790923,24.7610027835697,12.));
#247212=CARTESIAN_POINT('Ctrl Pts',(5.60964923798491,24.7405310372739,12.));
#247213=CARTESIAN_POINT('Ctrl Pts',(5.59250961323987,24.7200768119088,12.));
#247214=CARTESIAN_POINT('Ctrl Pts',(5.57546507427754,24.6996406035517,12.));
#247215=CARTESIAN_POINT('Ctrl Pts',(5.55851572025376,24.6792229061794,12.));
#247216=CARTESIAN_POINT('Ctrl Pts',(5.54166164919583,24.6588242134738,12.));
#247217=CARTESIAN_POINT('Ctrl Pts',(5.52490295840991,24.6384450211467,12.));
#247218=CARTESIAN_POINT('Ctrl Pts',(5.50823974481962,24.6180858289179,12.));
#247219=CARTESIAN_POINT('Ctrl Pts',(5.49167210537246,24.5977471429364,12.));
#247220=CARTESIAN_POINT('Ctrl Pts',(5.47520013724419,24.5774294770329,12.));
#247221=CARTESIAN_POINT('Ctrl Pts',(5.45882393762261,24.5571333514842,12.));
#247222=CARTESIAN_POINT('Ctrl Pts',(5.4425436035688,24.5368592922863,12.));
#247223=CARTESIAN_POINT('Ctrl Pts',(5.42635923183419,24.5166078302108,12.));
#247224=CARTESIAN_POINT('Ctrl Pts',(5.41027091869241,24.4963794999831,12.));
#247225=CARTESIAN_POINT('Ctrl Pts',(5.39427875973824,24.4761748393321,12.));
#247226=CARTESIAN_POINT('Ctrl Pts',(5.37838284973695,24.4559943883157,12.));
#247227=CARTESIAN_POINT('Ctrl Pts',(5.36258328273627,24.435838689915,12.));
#247228=CARTESIAN_POINT('Ctrl Pts',(5.34688015213537,24.4157082904614,12.));
#247229=CARTESIAN_POINT('Ctrl Pts',(5.33127355076033,24.3956037401293,12.));
#247230=CARTESIAN_POINT('Ctrl Pts',(5.31576357092526,24.3755255933917,12.));
#247231=CARTESIAN_POINT('Ctrl Pts',(5.30035030449063,24.3554744095075,12.));
#247232=CARTESIAN_POINT('Ctrl Pts',(5.28503384290648,24.3354507529414,12.));
#247233=CARTESIAN_POINT('Ctrl Pts',(5.26981427718798,24.3154551932221,12.));
#247234=CARTESIAN_POINT('Ctrl Pts',(5.25469169788856,24.2954883048447,12.));
#247235=CARTESIAN_POINT('Ctrl Pts',(5.23966619506289,24.2755506671525,12.));
#247236=CARTESIAN_POINT('Ctrl Pts',(5.22473785822442,24.2556428642294,12.));
#247237=CARTESIAN_POINT('Ctrl Pts',(5.20990677629176,24.2357654847766,12.));
#247238=CARTESIAN_POINT('Ctrl Pts',(5.19517303753647,24.2159191220171,12.));
#247239=CARTESIAN_POINT('Ctrl Pts',(5.18053672961398,24.1961043738756,12.));
#247240=CARTESIAN_POINT('Ctrl Pts',(5.16599793957985,24.1763218431344,12.));
#247241=CARTESIAN_POINT('Ctrl Pts',(5.15155675390079,24.1565721375971,12.));
#247242=CARTESIAN_POINT('Ctrl Pts',(5.13721325845745,24.1368558702443,12.));
#247243=CARTESIAN_POINT('Ctrl Pts',(5.12296753853857,24.117173659394,12.));
#247244=CARTESIAN_POINT('Ctrl Pts',(5.10881967883124,24.0975261288444,12.));
#247245=CARTESIAN_POINT('Ctrl Pts',(5.09476976342616,24.0779139079264,12.));
#247246=CARTESIAN_POINT('Ctrl Pts',(5.0808178758127,24.0583376315636,12.));
#247247=CARTESIAN_POINT('Ctrl Pts',(5.06696409886639,24.0387979403268,12.));
#247248=CARTESIAN_POINT('Ctrl Pts',(5.05320851483068,24.0192954804896,12.));
#247249=CARTESIAN_POINT('Ctrl Pts',(5.03955120528527,23.9998309040747,12.));
#247250=CARTESIAN_POINT('Ctrl Pts',(5.02599225112461,23.9804048689228,12.));
#247251=CARTESIAN_POINT('Ctrl Pts',(5.01253173257458,23.9610180388271,12.));
#247252=CARTESIAN_POINT('Ctrl Pts',(4.99916972919309,23.9416710836529,12.));
#247253=CARTESIAN_POINT('Ctrl Pts',(4.98590631986532,23.9223646794591,12.));
#247254=CARTESIAN_POINT('Ctrl Pts',(4.97274158279228,23.9030995086164,12.));
#247255=CARTESIAN_POINT('Ctrl Pts',(4.95967559546565,23.883876259922,12.));
#247256=CARTESIAN_POINT('Ctrl Pts',(4.94670843465868,23.8646956287172,12.));
#247257=CARTESIAN_POINT('Ctrl Pts',(4.93384017643441,23.8455583170062,12.));
#247258=CARTESIAN_POINT('Ctrl Pts',(4.92107089613976,23.8264650335721,12.));
#247259=CARTESIAN_POINT('Ctrl Pts',(4.90840066839346,23.8074164940897,12.));
#247260=CARTESIAN_POINT('Ctrl Pts',(4.89582956706771,23.7884134212381,12.));
#247261=CARTESIAN_POINT('Ctrl Pts',(4.88335766525565,23.7694565448044,12.));
#247262=CARTESIAN_POINT('Ctrl Pts',(4.87098503527142,23.7505466018239,12.));
#247263=CARTESIAN_POINT('Ctrl Pts',(4.85871174865491,23.7316843367308,12.));
#247264=CARTESIAN_POINT('Ctrl Pts',(4.84653787616422,23.7128705015014,12.));
#247265=CARTESIAN_POINT('Ctrl Pts',(4.83446348776267,23.6941058557971,12.));
#247266=CARTESIAN_POINT('Ctrl Pts',(4.82248865259569,23.6753911671023,12.));
#247267=CARTESIAN_POINT('Ctrl Pts',(4.81061343896442,23.6567272108631,12.));
#247268=CARTESIAN_POINT('Ctrl Pts',(4.79883791433229,23.6381147706581,12.));
#247269=CARTESIAN_POINT('Ctrl Pts',(4.78716214532104,23.6195546383625,12.));
#247270=CARTESIAN_POINT('Ctrl Pts',(4.77558619769875,23.6010476143099,12.));
#247271=CARTESIAN_POINT('Ctrl Pts',(4.7641101363625,23.5825945074535,12.));
#247272=CARTESIAN_POINT('Ctrl Pts',(4.75273402530615,23.564196135517,12.));
#247273=CARTESIAN_POINT('Ctrl Pts',(4.74145792760698,23.5458533251715,12.));
#247274=CARTESIAN_POINT('Ctrl Pts',(4.73028190543031,23.5275669122378,12.));
#247275=CARTESIAN_POINT('Ctrl Pts',(4.71920602001904,23.5093377418784,12.));
#247276=CARTESIAN_POINT('Ctrl Pts',(4.7082303316782,23.491166668789,12.));
#247277=CARTESIAN_POINT('Ctrl Pts',(4.69735489975023,23.4730545573849,12.));
#247278=CARTESIAN_POINT('Ctrl Pts',(4.68657978258297,23.4550022819853,12.));
#247279=CARTESIAN_POINT('Ctrl Pts',(4.6759050375305,23.4370107270444,12.));
#247280=CARTESIAN_POINT('Ctrl Pts',(4.66533072094663,23.4190807873798,12.));
#247281=CARTESIAN_POINT('Ctrl Pts',(4.65485688816921,23.4012133683957,12.));
#247282=CARTESIAN_POINT('Ctrl Pts',(4.64448359349935,23.383409386307,12.));
#247283=CARTESIAN_POINT('Ctrl Pts',(4.63421089016554,23.3656697683496,12.));
#247284=CARTESIAN_POINT('Ctrl Pts',(4.62403883030823,23.3479954530281,12.));
#247285=CARTESIAN_POINT('Ctrl Pts',(4.61396746497848,23.3303873903947,12.));
#247286=CARTESIAN_POINT('Ctrl Pts',(4.60399684412174,23.3128465423119,12.));
#247287=CARTESIAN_POINT('Ctrl Pts',(4.59412701655749,23.295373882719,12.));
#247288=CARTESIAN_POINT('Ctrl Pts',(4.58435802994674,23.2779703978868,12.));
#247289=CARTESIAN_POINT('Ctrl Pts',(4.5746899307607,23.2606370866853,12.));
#247290=CARTESIAN_POINT('Ctrl Pts',(4.5651227642781,23.2433749609117,12.));
#247291=CARTESIAN_POINT('Ctrl Pts',(4.55565657456956,23.2261850456055,12.));
#247292=CARTESIAN_POINT('Ctrl Pts',(4.54629140447542,23.2090683793627,12.));
#247293=CARTESIAN_POINT('Ctrl Pts',(4.53702729557585,23.1920260146474,12.));
#247294=CARTESIAN_POINT('Ctrl Pts',(4.52786428815047,23.1750590180923,12.));
#247295=CARTESIAN_POINT('Ctrl Pts',(4.51880242116785,23.1581684708778,12.));
#247296=CARTESIAN_POINT('Ctrl Pts',(4.50984173227087,23.1413554691136,12.));
#247297=CARTESIAN_POINT('Ctrl Pts',(4.50098225775178,23.1246211242117,12.));
#247298=CARTESIAN_POINT('Ctrl Pts',(4.49222403252201,23.1079665632629,12.));
#247299=CARTESIAN_POINT('Ctrl Pts',(4.48356709006756,23.0913929293909,12.));
#247300=CARTESIAN_POINT('Ctrl Pts',(4.47501146242821,23.0749013821868,12.));
#247301=CARTESIAN_POINT('Ctrl Pts',(4.46655718018205,23.0584930981723,12.));
#247302=CARTESIAN_POINT('Ctrl Pts',(4.45820427241676,23.0421692712466,12.));
#247303=CARTESIAN_POINT('Ctrl Pts',(4.44995276669698,23.0259311131395,12.));
#247304=CARTESIAN_POINT('Ctrl Pts',(4.44180268901666,23.0097798538399,12.));
#247305=CARTESIAN_POINT('Ctrl Pts',(4.43375406376904,22.9937167421009,12.));
#247306=CARTESIAN_POINT('Ctrl Pts',(4.42580691372771,22.9777430460021,12.));
#247307=CARTESIAN_POINT('Ctrl Pts',(4.41796126001309,22.9618600534866,12.));
#247308=CARTESIAN_POINT('Ctrl Pts',(4.41021712205547,22.9460690729093,12.));
#247309=CARTESIAN_POINT('Ctrl Pts',(4.40257451754307,22.9303714335549,12.));
#247310=CARTESIAN_POINT('Ctrl Pts',(4.39503346238454,22.9147684862425,12.));
#247311=CARTESIAN_POINT('Ctrl Pts',(4.38759397068391,22.8992616040108,12.));
#247312=CARTESIAN_POINT('Ctrl Pts',(4.38025605470089,22.8838521827702,12.));
#247313=CARTESIAN_POINT('Ctrl Pts',(4.37301972480752,22.8685416419725,12.));
#247314=CARTESIAN_POINT('Ctrl Pts',(4.36588498943009,22.8533314252419,12.));
#247315=CARTESIAN_POINT('Ctrl Pts',(4.35885185500559,22.838223001118,12.));
#247316=CARTESIAN_POINT('Ctrl Pts',(4.35192032594801,22.8232178638873,12.));
#247317=CARTESIAN_POINT('Ctrl Pts',(4.34509040460065,22.808317534379,12.));
#247318=CARTESIAN_POINT('Ctrl Pts',(4.33836209118442,22.7935235607807,12.));
#247319=CARTESIAN_POINT('Ctrl Pts',(4.33173538373182,22.7788375194081,12.));
#247320=CARTESIAN_POINT('Ctrl Pts',(4.32521027803747,22.764261015648,12.));
#247321=CARTESIAN_POINT('Ctrl Pts',(4.3187867676123,22.7497956849852,12.));
#247322=CARTESIAN_POINT('Ctrl Pts',(4.3124648436255,22.7354431939927,12.));
#247323=CARTESIAN_POINT('Ctrl Pts',(4.30624449484074,22.7212052413384,12.));
#247324=CARTESIAN_POINT('Ctrl Pts',(4.30012570754066,22.707083558756,12.));
#247325=CARTESIAN_POINT('Ctrl Pts',(4.29410846547061,22.6930799122545,12.));
#247326=CARTESIAN_POINT('Ctrl Pts',(4.28819274977766,22.6791961033537,12.));
#247327=CARTESIAN_POINT('Ctrl Pts',(4.28237853894059,22.665433970311,12.));
#247328=CARTESIAN_POINT('Ctrl Pts',(4.27666580869117,22.6517953893303,12.));
#247329=CARTESIAN_POINT('Ctrl Pts',(4.27105453192999,22.6382822758171,12.));
#247330=CARTESIAN_POINT('Ctrl Pts',(4.26554467865571,22.6248965859975,12.));
#247331=CARTESIAN_POINT('Ctrl Pts',(4.26013621588303,22.611640318482,12.));
#247332=CARTESIAN_POINT('Ctrl Pts',(4.25482910755485,22.5985155158637,12.));
#247333=CARTESIAN_POINT('Ctrl Pts',(4.24962331444184,22.5855242662479,12.));
#247334=CARTESIAN_POINT('Ctrl Pts',(4.24451879404858,22.5726687049922,12.));
#247335=CARTESIAN_POINT('Ctrl Pts',(4.23951550052526,22.559951016643,12.));
#247336=CARTESIAN_POINT('Ctrl Pts',(4.23461338456713,22.5473734368086,12.));
#247337=CARTESIAN_POINT('Ctrl Pts',(4.22981239330731,22.5349382540587,12.));
#247338=CARTESIAN_POINT('Ctrl Pts',(4.2251124702004,22.5226478117885,12.));
#247339=CARTESIAN_POINT('Ctrl Pts',(4.22051355490196,22.5105045108882,12.));
#247340=CARTESIAN_POINT('Ctrl Pts',(4.21601558313908,22.4985108124229,12.));
#247341=CARTESIAN_POINT('Ctrl Pts',(4.21161848657428,22.4866692403147,12.));
#247342=CARTESIAN_POINT('Ctrl Pts',(4.20732219265648,22.4749823839915,12.));
#247343=CARTESIAN_POINT('Ctrl Pts',(4.2031266244817,22.4634529011433,12.));
#247344=CARTESIAN_POINT('Ctrl Pts',(4.19903170066354,22.4520835205419,12.));
#247345=CARTESIAN_POINT('Ctrl Pts',(4.1950373351886,22.4408770448917,12.));
#247346=CARTESIAN_POINT('Ctrl Pts',(4.19114343726941,22.4298363535421,12.));
#247347=CARTESIAN_POINT('Ctrl Pts',(4.1873499111772,22.4189644056115,12.));
#247348=CARTESIAN_POINT('Ctrl Pts',(4.1836566560085,22.4082642454453,12.));
#247349=CARTESIAN_POINT('Ctrl Pts',(4.18006356544882,22.3977390078075,12.));
#247350=CARTESIAN_POINT('Ctrl Pts',(4.17657052752825,22.3873919231334,12.));
#247351=CARTESIAN_POINT('Ctrl Pts',(4.17317742436145,22.3772263228617,12.));
#247352=CARTESIAN_POINT('Ctrl Pts',(4.16988413199457,22.36724564276,12.));
#247353=CARTESIAN_POINT('Ctrl Pts',(4.166690520266,22.3574534257396,12.));
#247354=CARTESIAN_POINT('Ctrl Pts',(4.16359645263187,22.3478533253889,12.));
#247355=CARTESIAN_POINT('Ctrl Pts',(4.16060178604164,22.3384491078602,12.));
#247356=CARTESIAN_POINT('Ctrl Pts',(4.15770637047889,22.3292446628959,12.));
#247357=CARTESIAN_POINT('Ctrl Pts',(4.15491004835281,22.3202440186979,12.));
#247358=CARTESIAN_POINT('Ctrl Pts',(4.1522126539699,22.3114513545185,12.));
#247359=CARTESIAN_POINT('Ctrl Pts',(4.14961401285522,22.3028710166933,12.));
#247360=CARTESIAN_POINT('Ctrl Pts',(4.14711394168556,22.2945075198467,12.));
#247361=CARTESIAN_POINT('Ctrl Pts',(4.14471224859295,22.2863655389166,12.));
#247362=CARTESIAN_POINT('Ctrl Pts',(4.14240873321984,22.2784499072027,12.));
#247363=CARTESIAN_POINT('Ctrl Pts',(4.14020318715991,22.2707656042457,12.));
#247364=CARTESIAN_POINT('Ctrl Pts',(4.13809539255421,22.2633177913972,12.));
#247365=CARTESIAN_POINT('Ctrl Pts',(4.13608511977225,22.2561118708421,12.));
#247366=CARTESIAN_POINT('Ctrl Pts',(4.1341721255881,22.249153531779,12.));
#247367=CARTESIAN_POINT('Ctrl Pts',(4.1323561506016,22.2424488153523,12.));
#247368=CARTESIAN_POINT('Ctrl Pts',(4.13063692157498,22.2360040565533,12.));
#247369=CARTESIAN_POINT('Ctrl Pts',(4.12901415463379,22.2298258043947,12.));
#247370=CARTESIAN_POINT('Ctrl Pts',(4.12748755830104,22.2239207458781,12.));
#247371=CARTESIAN_POINT('Ctrl Pts',(4.12605683613307,22.2182956401341,12.));
#247372=CARTESIAN_POINT('Ctrl Pts',(4.12472167516607,22.2129576146671,12.));
#247373=CARTESIAN_POINT('Ctrl Pts',(4.12348173702023,22.2079143941719,12.));
#247374=CARTESIAN_POINT('Ctrl Pts',(4.12233664408227,22.2031746532106,12.));
#247375=CARTESIAN_POINT('Ctrl Pts',(4.12128598183522,22.1987479618246,12.));
#247376=CARTESIAN_POINT('Ctrl Pts',(4.12032932637736,22.1946440958098,12.));
#247377=CARTESIAN_POINT('Ctrl Pts',(4.11946626228636,22.1908725908525,12.));
#247378=CARTESIAN_POINT('Ctrl Pts',(4.11869641271773,22.1874419861496,12.));
#247379=CARTESIAN_POINT('Ctrl Pts',(4.11801938107479,22.1843613164855,12.));
#247380=CARTESIAN_POINT('Ctrl Pts',(4.11743469691756,22.1816414985788,12.));
#247381=CARTESIAN_POINT('Ctrl Pts',(4.11694173195003,22.179297473024,12.));
#247382=CARTESIAN_POINT('Ctrl Pts',(4.11653973150518,22.177347426894,12.));
#247383=CARTESIAN_POINT('Ctrl Pts',(4.11622797217068,22.1758088296598,12.));
#247384=CARTESIAN_POINT('Ctrl Pts',(4.11600589882845,22.1746949858775,12.));
#247385=CARTESIAN_POINT('Ctrl Pts',(4.11589976826166,22.1741488021234,12.));
#247386=CARTESIAN_POINT('Ctrl Pts',(4.11586035878287,22.1739341411687,12.));
#247387=CARTESIAN_POINT('Ctrl Pts',(4.11585194677442,22.173877682324,12.));
#247388=CARTESIAN_POINT('Ctrl Pts',(4.11585220600461,22.1738711152697,12.));
#247389=CARTESIAN_POINT('',(6.08833931617699,25.2771067246846,0.));
#247390=CARTESIAN_POINT('Origin',(9.26120677397564,19.4030938020118,0.));
#247391=CARTESIAN_POINT('',(9.71462809124917,20.353053841303,12.));
#247392=CARTESIAN_POINT('',(4.63060338698782,9.70154690100589,12.));
#247393=CARTESIAN_POINT('',(9.71462809124917,20.353053841303,0.));
#247394=CARTESIAN_POINT('',(9.71462809124917,20.353053841303,0.));
#247395=CARTESIAN_POINT('',(4.63060338698782,9.70154690100589,0.));
#247396=CARTESIAN_POINT('Ctrl Pts',(7.36589684767344,24.9347862158358,0.));
#247397=CARTESIAN_POINT('Ctrl Pts',(7.36589684767344,24.9347862158358,12.));
#247398=CARTESIAN_POINT('Ctrl Pts',(7.36721909028842,24.9292275670674,0.));
#247399=CARTESIAN_POINT('Ctrl Pts',(7.36721909028842,24.9292275670674,12.));
#247400=CARTESIAN_POINT('Ctrl Pts',(7.3698559312009,24.9181155530543,0.));
#247401=CARTESIAN_POINT('Ctrl Pts',(7.3698559312009,24.9181155530543,12.));
#247402=CARTESIAN_POINT('Ctrl Pts',(7.37378825961676,24.901463382605,0.));
#247403=CARTESIAN_POINT('Ctrl Pts',(7.37378825961676,24.901463382605,12.));
#247404=CARTESIAN_POINT('Ctrl Pts',(7.37898549640269,24.8792921911115,0.));
#247405=CARTESIAN_POINT('Ctrl Pts',(7.37898549640269,24.8792921911115,12.));
#247406=CARTESIAN_POINT('Ctrl Pts',(7.3854055890362,24.8516310625176,0.));
#247407=CARTESIAN_POINT('Ctrl Pts',(7.3854055890362,24.8516310625176,12.));
#247408=CARTESIAN_POINT('Ctrl Pts',(7.39174922585808,24.8240228520893,0.));
#247409=CARTESIAN_POINT('Ctrl Pts',(7.39174922585808,24.8240228520893,12.));
#247410=CARTESIAN_POINT('Ctrl Pts',(7.39801641583012,24.7964676646431,0.));
#247411=CARTESIAN_POINT('Ctrl Pts',(7.39801641583012,24.7964676646431,12.));
#247412=CARTESIAN_POINT('Ctrl Pts',(7.40420718661602,24.7689656668983,0.));
#247413=CARTESIAN_POINT('Ctrl Pts',(7.40420718661602,24.7689656668983,12.));
#247414=CARTESIAN_POINT('Ctrl Pts',(7.41032159082381,24.7415170994784,0.));
#247415=CARTESIAN_POINT('Ctrl Pts',(7.41032159082381,24.7415170994784,12.));
#247416=CARTESIAN_POINT('Ctrl Pts',(7.41635971481674,24.7141222950051,0.));
#247417=CARTESIAN_POINT('Ctrl Pts',(7.41635971481674,24.7141222950051,12.));
#247418=CARTESIAN_POINT('Ctrl Pts',(7.42232167766265,24.6867816727192,0.));
#247419=CARTESIAN_POINT('Ctrl Pts',(7.42232167766265,24.6867816727192,12.));
#247420=CARTESIAN_POINT('Ctrl Pts',(7.42820762159125,24.6594957128756,0.));
#247421=CARTESIAN_POINT('Ctrl Pts',(7.42820762159125,24.6594957128756,12.));
#247422=CARTESIAN_POINT('Ctrl Pts',(7.43401770489523,24.6322649369517,0.));
#247423=CARTESIAN_POINT('Ctrl Pts',(7.43401770489523,24.6322649369517,12.));
#247424=CARTESIAN_POINT('Ctrl Pts',(7.43975209375503,24.6050898852368,0.));
#247425=CARTESIAN_POINT('Ctrl Pts',(7.43975209375503,24.6050898852368,12.));
#247426=CARTESIAN_POINT('Ctrl Pts',(7.44541095473134,24.577971096086,0.));
#247427=CARTESIAN_POINT('Ctrl Pts',(7.44541095473134,24.577971096086,12.));
#247428=CARTESIAN_POINT('Ctrl Pts',(7.4509944465116,24.5509090831559,0.));
#247429=CARTESIAN_POINT('Ctrl Pts',(7.4509944465116,24.5509090831559,12.));
#247430=CARTESIAN_POINT('Ctrl Pts',(7.45650271335861,24.5239043173072,0.));
#247431=CARTESIAN_POINT('Ctrl Pts',(7.45650271335861,24.5239043173072,12.));
#247432=CARTESIAN_POINT('Ctrl Pts',(7.46193588961463,24.4969572391483,0.));
#247433=CARTESIAN_POINT('Ctrl Pts',(7.46193588961463,24.4969572391483,12.));
#247434=CARTESIAN_POINT('Ctrl Pts',(7.46729410308786,24.4700682684524,0.));
#247435=CARTESIAN_POINT('Ctrl Pts',(7.46729410308786,24.4700682684524,12.));
#247436=CARTESIAN_POINT('Ctrl Pts',(7.47257747883246,24.443237814649,0.));
#247437=CARTESIAN_POINT('Ctrl Pts',(7.47257747883246,24.443237814649,12.));
#247438=CARTESIAN_POINT('Ctrl Pts',(7.47778614286564,24.4164662871163,0.));
#247439=CARTESIAN_POINT('Ctrl Pts',(7.47778614286564,24.4164662871163,12.));
#247440=CARTESIAN_POINT('Ctrl Pts',(7.482920225693,24.3897541049254,0.));
#247441=CARTESIAN_POINT('Ctrl Pts',(7.482920225693,24.3897541049254,12.));
#247442=CARTESIAN_POINT('Ctrl Pts',(7.48797986651908,24.3631017084524,0.));
#247443=CARTESIAN_POINT('Ctrl Pts',(7.48797986651908,24.3631017084524,12.));
#247444=CARTESIAN_POINT('Ctrl Pts',(7.4929652125242,24.3365095573685,0.));
#247445=CARTESIAN_POINT('Ctrl Pts',(7.4929652125242,24.3365095573685,12.));
#247446=CARTESIAN_POINT('Ctrl Pts',(7.49787641695438,24.3099781253355,0.));
#247447=CARTESIAN_POINT('Ctrl Pts',(7.49787641695438,24.3099781253355,12.));
#247448=CARTESIAN_POINT('Ctrl Pts',(7.50271363765151,24.2835078958973,0.));
#247449=CARTESIAN_POINT('Ctrl Pts',(7.50271363765151,24.2835078958973,12.));
#247450=CARTESIAN_POINT('Ctrl Pts',(7.50747703535133,24.2570993577034,0.));
#247451=CARTESIAN_POINT('Ctrl Pts',(7.50747703535133,24.2570993577034,12.));
#247452=CARTESIAN_POINT('Ctrl Pts',(7.5121667722218,24.2307530003887,0.));
#247453=CARTESIAN_POINT('Ctrl Pts',(7.5121667722218,24.2307530003887,12.));
#247454=CARTESIAN_POINT('Ctrl Pts',(7.51678300997949,24.2044693092349,0.));
#247455=CARTESIAN_POINT('Ctrl Pts',(7.51678300997949,24.2044693092349,12.));
#247456=CARTESIAN_POINT('Ctrl Pts',(7.52132590953801,24.1782487641594,0.));
#247457=CARTESIAN_POINT('Ctrl Pts',(7.52132590953801,24.1782487641594,12.));
#247458=CARTESIAN_POINT('Ctrl Pts',(7.52579563201423,24.1520918425364,0.));
#247459=CARTESIAN_POINT('Ctrl Pts',(7.52579563201423,24.1520918425364,12.));
#247460=CARTESIAN_POINT('Ctrl Pts',(7.53019233935501,24.1259990209207,0.));
#247461=CARTESIAN_POINT('Ctrl Pts',(7.53019233935501,24.1259990209207,12.));
#247462=CARTESIAN_POINT('Ctrl Pts',(7.53451619514649,24.0999707772642,0.));
#247463=CARTESIAN_POINT('Ctrl Pts',(7.53451619514649,24.0999707772642,12.));
#247464=CARTESIAN_POINT('Ctrl Pts',(7.53876736531013,24.0740075927985,0.));
#247465=CARTESIAN_POINT('Ctrl Pts',(7.53876736531013,24.0740075927985,12.));
#247466=CARTESIAN_POINT('Ctrl Pts',(7.54294601896144,24.0481099543353,0.));
#247467=CARTESIAN_POINT('Ctrl Pts',(7.54294601896144,24.0481099543353,12.));
#247468=CARTESIAN_POINT('Ctrl Pts',(7.5470523288591,24.022278355453,0.));
#247469=CARTESIAN_POINT('Ctrl Pts',(7.5470523288591,24.022278355453,12.));
#247470=CARTESIAN_POINT('Ctrl Pts',(7.5510864709744,23.9965132953185,0.));
#247471=CARTESIAN_POINT('Ctrl Pts',(7.5510864709744,23.9965132953185,12.));
#247472=CARTESIAN_POINT('Ctrl Pts',(7.55504862424811,23.9708152779884,0.));
#247473=CARTESIAN_POINT('Ctrl Pts',(7.55504862424811,23.9708152779884,12.));
#247474=CARTESIAN_POINT('Ctrl Pts',(7.55893897027682,23.9451848115,0.));
#247475=CARTESIAN_POINT('Ctrl Pts',(7.55893897027682,23.9451848115,12.));
#247476=CARTESIAN_POINT('Ctrl Pts',(7.56275769304773,23.9196224070759,0.));
#247477=CARTESIAN_POINT('Ctrl Pts',(7.56275769304773,23.9196224070759,12.));
#247478=CARTESIAN_POINT('Ctrl Pts',(7.56650497863791,23.8941285782003,0.));
#247479=CARTESIAN_POINT('Ctrl Pts',(7.56650497863791,23.8941285782003,12.));
#247480=CARTESIAN_POINT('Ctrl Pts',(7.5701810150071,23.8687038399598,0.));
#247481=CARTESIAN_POINT('Ctrl Pts',(7.5701810150071,23.8687038399598,12.));
#247482=CARTESIAN_POINT('Ctrl Pts',(7.57378599219816,23.8433487096134,0.));
#247483=CARTESIAN_POINT('Ctrl Pts',(7.57378599219816,23.8433487096134,12.));
#247484=CARTESIAN_POINT('Ctrl Pts',(7.57732010249065,23.8180637069977,0.));
#247485=CARTESIAN_POINT('Ctrl Pts',(7.57732010249065,23.8180637069977,12.));
#247486=CARTESIAN_POINT('Ctrl Pts',(7.58078354058211,23.7928493549908,0.));
#247487=CARTESIAN_POINT('Ctrl Pts',(7.58078354058211,23.7928493549908,12.));
#247488=CARTESIAN_POINT('Ctrl Pts',(7.58417650376271,23.7677061799376,0.));
#247489=CARTESIAN_POINT('Ctrl Pts',(7.58417650376271,23.7677061799376,12.));
#247490=CARTESIAN_POINT('Ctrl Pts',(7.58749919210831,23.7426347121006,0.));
#247491=CARTESIAN_POINT('Ctrl Pts',(7.58749919210831,23.7426347121006,12.));
#247492=CARTESIAN_POINT('Ctrl Pts',(7.59075180865326,23.7176354860457,0.));
#247493=CARTESIAN_POINT('Ctrl Pts',(7.59075180865326,23.7176354860457,12.));
#247494=CARTESIAN_POINT('Ctrl Pts',(7.59393455934041,23.6927090405067,0.));
#247495=CARTESIAN_POINT('Ctrl Pts',(7.59393455934041,23.6927090405067,12.));
#247496=CARTESIAN_POINT('Ctrl Pts',(7.59704765299572,23.6678559182876,0.));
#247497=CARTESIAN_POINT('Ctrl Pts',(7.59704765299572,23.6678559182876,12.));
#247498=CARTESIAN_POINT('Ctrl Pts',(7.60009130130129,23.6430766661419,0.));
#247499=CARTESIAN_POINT('Ctrl Pts',(7.60009130130129,23.6430766661419,12.));
#247500=CARTESIAN_POINT('Ctrl Pts',(7.60306571877806,23.6183718346576,0.));
#247501=CARTESIAN_POINT('Ctrl Pts',(7.60306571877806,23.6183718346576,12.));
#247502=CARTESIAN_POINT('Ctrl Pts',(7.60597112277094,23.5937419781244,0.));
#247503=CARTESIAN_POINT('Ctrl Pts',(7.60597112277094,23.5937419781244,12.));
#247504=CARTESIAN_POINT('Ctrl Pts',(7.60880773344599,23.5691876544243,0.));
#247505=CARTESIAN_POINT('Ctrl Pts',(7.60880773344599,23.5691876544243,12.));
#247506=CARTESIAN_POINT('Ctrl Pts',(7.61157577385371,23.5447094252029,0.));
#247507=CARTESIAN_POINT('Ctrl Pts',(7.61157577385371,23.5447094252029,12.));
#247508=CARTESIAN_POINT('Ctrl Pts',(7.61427546999298,23.5203078560128,0.));
#247509=CARTESIAN_POINT('Ctrl Pts',(7.61427546999298,23.5203078560128,12.));
#247510=CARTESIAN_POINT('Ctrl Pts',(7.61690705088318,23.4959835164608,0.));
#247511=CARTESIAN_POINT('Ctrl Pts',(7.61690705088318,23.4959835164608,12.));
#247512=CARTESIAN_POINT('Ctrl Pts',(7.61947074863977,23.4717369803438,0.));
#247513=CARTESIAN_POINT('Ctrl Pts',(7.61947074863977,23.4717369803438,12.));
#247514=CARTESIAN_POINT('Ctrl Pts',(7.62196679855957,23.4475688257855,0.));
#247515=CARTESIAN_POINT('Ctrl Pts',(7.62196679855957,23.4475688257855,12.));
#247516=CARTESIAN_POINT('Ctrl Pts',(7.62439543920053,23.4234796353544,0.));
#247517=CARTESIAN_POINT('Ctrl Pts',(7.62439543920053,23.4234796353544,12.));
#247518=CARTESIAN_POINT('Ctrl Pts',(7.62675691240334,23.3994699961122,0.));
#247519=CARTESIAN_POINT('Ctrl Pts',(7.62675691240334,23.3994699961122,12.));
#247520=CARTESIAN_POINT('Ctrl Pts',(7.62905146332597,23.3755404996638,0.));
#247521=CARTESIAN_POINT('Ctrl Pts',(7.62905146332597,23.3755404996638,12.));
#247522=CARTESIAN_POINT('Ctrl Pts',(7.63127934048138,23.3516917421973,0.));
#247523=CARTESIAN_POINT('Ctrl Pts',(7.63127934048138,23.3516917421973,12.));
#247524=CARTESIAN_POINT('Ctrl Pts',(7.63344079578162,23.3279243245241,0.));
#247525=CARTESIAN_POINT('Ctrl Pts',(7.63344079578162,23.3279243245241,12.));
#247526=CARTESIAN_POINT('Ctrl Pts',(7.63553608458783,23.3042388521021,0.));
#247527=CARTESIAN_POINT('Ctrl Pts',(7.63553608458783,23.3042388521021,12.));
#247528=CARTESIAN_POINT('Ctrl Pts',(7.63756546576374,23.2806359350853,0.));
#247529=CARTESIAN_POINT('Ctrl Pts',(7.63756546576374,23.2806359350853,12.));
#247530=CARTESIAN_POINT('Ctrl Pts',(7.63952920172837,23.2571161884487,0.));
#247531=CARTESIAN_POINT('Ctrl Pts',(7.63952920172837,23.2571161884487,12.));
#247532=CARTESIAN_POINT('Ctrl Pts',(7.64142755851507,23.2336802320912,0.));
#247533=CARTESIAN_POINT('Ctrl Pts',(7.64142755851507,23.2336802320912,12.));
#247534=CARTESIAN_POINT('Ctrl Pts',(7.64326080583683,23.2103286909399,0.));
#247535=CARTESIAN_POINT('Ctrl Pts',(7.64326080583683,23.2103286909399,12.));
#247536=CARTESIAN_POINT('Ctrl Pts',(7.64502921715482,23.1870621950452,0.));
#247537=CARTESIAN_POINT('Ctrl Pts',(7.64502921715482,23.1870621950452,12.));
#247538=CARTESIAN_POINT('Ctrl Pts',(7.64673306975796,23.1638813796691,0.));
#247539=CARTESIAN_POINT('Ctrl Pts',(7.64673306975796,23.1638813796691,12.));
#247540=CARTESIAN_POINT('Ctrl Pts',(7.64837264482929,23.1407868853815,0.));
#247541=CARTESIAN_POINT('Ctrl Pts',(7.64837264482929,23.1407868853815,12.));
#247542=CARTESIAN_POINT('Ctrl Pts',(7.64994822749844,23.1177793581674,0.));
#247543=CARTESIAN_POINT('Ctrl Pts',(7.64994822749844,23.1177793581674,12.));
#247544=CARTESIAN_POINT('Ctrl Pts',(7.65146010690464,23.0948594495246,0.));
#247545=CARTESIAN_POINT('Ctrl Pts',(7.65146010690464,23.0948594495246,12.));
#247546=CARTESIAN_POINT('Ctrl Pts',(7.65290857626356,23.072027816555,0.));
#247547=CARTESIAN_POINT('Ctrl Pts',(7.65290857626356,23.072027816555,12.));
#247548=CARTESIAN_POINT('Ctrl Pts',(7.65429393293955,23.049285122053,0.));
#247549=CARTESIAN_POINT('Ctrl Pts',(7.65429393293955,23.049285122053,12.));
#247550=CARTESIAN_POINT('Ctrl Pts',(7.65561647852554,23.0266320345792,0.));
#247551=CARTESIAN_POINT('Ctrl Pts',(7.65561647852554,23.0266320345792,12.));
#247552=CARTESIAN_POINT('Ctrl Pts',(7.6568765189133,23.004069228582,0.));
#247553=CARTESIAN_POINT('Ctrl Pts',(7.6568765189133,23.004069228582,12.));
#247554=CARTESIAN_POINT('Ctrl Pts',(7.65807436436452,22.9815973845301,0.));
#247555=CARTESIAN_POINT('Ctrl Pts',(7.65807436436452,22.9815973845301,12.));
#247556=CARTESIAN_POINT('Ctrl Pts',(7.65921032958911,22.9592171890332,0.));
#247557=CARTESIAN_POINT('Ctrl Pts',(7.65921032958911,22.9592171890332,12.));
#247558=CARTESIAN_POINT('Ctrl Pts',(7.66028473382776,22.9369293349592,0.));
#247559=CARTESIAN_POINT('Ctrl Pts',(7.66028473382776,22.9369293349592,12.));
#247560=CARTESIAN_POINT('Ctrl Pts',(7.66129790094099,22.9147345215418,0.));
#247561=CARTESIAN_POINT('Ctrl Pts',(7.66129790094099,22.9147345215418,12.));
#247562=CARTESIAN_POINT('Ctrl Pts',(7.66225015950147,22.8926334544879,0.));
#247563=CARTESIAN_POINT('Ctrl Pts',(7.66225015950147,22.8926334544879,12.));
#247564=CARTESIAN_POINT('Ctrl Pts',(7.66314184287333,22.870626846128,0.));
#247565=CARTESIAN_POINT('Ctrl Pts',(7.66314184287333,22.870626846128,12.));
#247566=CARTESIAN_POINT('Ctrl Pts',(7.66397328929805,22.8487154155569,0.));
#247567=CARTESIAN_POINT('Ctrl Pts',(7.66397328929805,22.8487154155569,12.));
#247568=CARTESIAN_POINT('Ctrl Pts',(7.66474484198552,22.8268998887679,0.));
#247569=CARTESIAN_POINT('Ctrl Pts',(7.66474484198552,22.8268998887679,12.));
#247570=CARTESIAN_POINT('Ctrl Pts',(7.66545684920987,22.8051809987834,0.));
#247571=CARTESIAN_POINT('Ctrl Pts',(7.66545684920987,22.8051809987834,12.));
#247572=CARTESIAN_POINT('Ctrl Pts',(7.66610966441259,22.7835594857697,0.));
#247573=CARTESIAN_POINT('Ctrl Pts',(7.66610966441259,22.7835594857697,12.));
#247574=CARTESIAN_POINT('Ctrl Pts',(7.66670364630273,22.7620360971839,0.));
#247575=CARTESIAN_POINT('Ctrl Pts',(7.66670364630273,22.7620360971839,12.));
#247576=CARTESIAN_POINT('Ctrl Pts',(7.66723915895412,22.7406115879508,0.));
#247577=CARTESIAN_POINT('Ctrl Pts',(7.66723915895412,22.7406115879508,12.));
#247578=CARTESIAN_POINT('Ctrl Pts',(7.6677165719101,22.7192867206242,0.));
#247579=CARTESIAN_POINT('Ctrl Pts',(7.6677165719101,22.7192867206242,12.));
#247580=CARTESIAN_POINT('Ctrl Pts',(7.66813626029276,22.6980622655446,0.));
#247581=CARTESIAN_POINT('Ctrl Pts',(7.66813626029276,22.6980622655446,12.));
#247582=CARTESIAN_POINT('Ctrl Pts',(7.66849860491762,22.6769390009889,0.));
#247583=CARTESIAN_POINT('Ctrl Pts',(7.66849860491762,22.6769390009889,12.));
#247584=CARTESIAN_POINT('Ctrl Pts',(7.66880399241353,22.6559177133133,0.));
#247585=CARTESIAN_POINT('Ctrl Pts',(7.66880399241353,22.6559177133133,12.));
#247586=CARTESIAN_POINT('Ctrl Pts',(7.66905281533744,22.6349991971548,0.));
#247587=CARTESIAN_POINT('Ctrl Pts',(7.66905281533744,22.6349991971548,12.));
#247588=CARTESIAN_POINT('Ctrl Pts',(7.66924547229434,22.6141842556248,0.));
#247589=CARTESIAN_POINT('Ctrl Pts',(7.66924547229434,22.6141842556248,12.));
#247590=CARTESIAN_POINT('Ctrl Pts',(7.6693823680624,22.5934737004955,0.));
#247591=CARTESIAN_POINT('Ctrl Pts',(7.6693823680624,22.5934737004955,12.));
#247592=CARTESIAN_POINT('Ctrl Pts',(7.66946391372299,22.5728683523829,0.));
#247593=CARTESIAN_POINT('Ctrl Pts',(7.66946391372299,22.5728683523829,12.));
#247594=CARTESIAN_POINT('Ctrl Pts',(7.66949052679671,22.5523690409109,0.));
#247595=CARTESIAN_POINT('Ctrl Pts',(7.66949052679671,22.5523690409109,12.));
#247596=CARTESIAN_POINT('Ctrl Pts',(7.66946263138115,22.5319766049191,0.));
#247597=CARTESIAN_POINT('Ctrl Pts',(7.66946263138115,22.5319766049191,12.));
#247598=CARTESIAN_POINT('Ctrl Pts',(7.66938065829082,22.5116918927023,0.));
#247599=CARTESIAN_POINT('Ctrl Pts',(7.66938065829082,22.5116918927023,12.));
#247600=CARTESIAN_POINT('Ctrl Pts',(7.66924504520301,22.4915157622308,0.));
#247601=CARTESIAN_POINT('Ctrl Pts',(7.66924504520301,22.4915157622308,12.));
#247602=CARTESIAN_POINT('Ctrl Pts',(7.66905623680835,22.47144908137,0.));
#247603=CARTESIAN_POINT('Ctrl Pts',(7.66905623680835,22.47144908137,12.));
#247604=CARTESIAN_POINT('Ctrl Pts',(7.66881468496659,22.4514927280863,0.));
#247605=CARTESIAN_POINT('Ctrl Pts',(7.66881468496659,22.4514927280863,12.));
#247606=CARTESIAN_POINT('Ctrl Pts',(7.66852084886745,22.4316475906616,0.));
#247607=CARTESIAN_POINT('Ctrl Pts',(7.66852084886745,22.4316475906616,12.));
#247608=CARTESIAN_POINT('Ctrl Pts',(7.66817519519681,22.411914567977,0.));
#247609=CARTESIAN_POINT('Ctrl Pts',(7.66817519519681,22.411914567977,12.));
#247610=CARTESIAN_POINT('Ctrl Pts',(7.66777819830819,22.3922945697782,0.));
#247611=CARTESIAN_POINT('Ctrl Pts',(7.66777819830819,22.3922945697782,12.));
#247612=CARTESIAN_POINT('Ctrl Pts',(7.66733034039887,22.3727885169361,0.));
#247613=CARTESIAN_POINT('Ctrl Pts',(7.66733034039887,22.3727885169361,12.));
#247614=CARTESIAN_POINT('Ctrl Pts',(7.66683211169133,22.3533973417013,0.));
#247615=CARTESIAN_POINT('Ctrl Pts',(7.66683211169133,22.3533973417013,12.));
#247616=CARTESIAN_POINT('Ctrl Pts',(7.66628401061905,22.3341219879454,0.));
#247617=CARTESIAN_POINT('Ctrl Pts',(7.66628401061905,22.3341219879454,12.));
#247618=CARTESIAN_POINT('Ctrl Pts',(7.66568654402441,22.3149634114823,0.));
#247619=CARTESIAN_POINT('Ctrl Pts',(7.66568654402441,22.3149634114823,12.));
#247620=CARTESIAN_POINT('Ctrl Pts',(7.66504022736262,22.2959225803925,0.));
#247621=CARTESIAN_POINT('Ctrl Pts',(7.66504022736262,22.2959225803925,12.));
#247622=CARTESIAN_POINT('Ctrl Pts',(7.66434558490972,22.2770004753332,0.));
#247623=CARTESIAN_POINT('Ctrl Pts',(7.66434558490972,22.2770004753332,12.));
#247624=CARTESIAN_POINT('Ctrl Pts',(7.66360314997661,22.2581980898487,0.));
#247625=CARTESIAN_POINT('Ctrl Pts',(7.66360314997661,22.2581980898487,12.));
#247626=CARTESIAN_POINT('Ctrl Pts',(7.66281346512545,22.239516430656,0.));
#247627=CARTESIAN_POINT('Ctrl Pts',(7.66281346512545,22.239516430656,12.));
#247628=CARTESIAN_POINT('Ctrl Pts',(7.66197708240435,22.2209565180098,0.));
#247629=CARTESIAN_POINT('Ctrl Pts',(7.66197708240435,22.2209565180098,12.));
#247630=CARTESIAN_POINT('Ctrl Pts',(7.66109456359292,22.2025193860972,0.));
#247631=CARTESIAN_POINT('Ctrl Pts',(7.66109456359292,22.2025193860972,12.));
#247632=CARTESIAN_POINT('Ctrl Pts',(7.66016648045007,22.1842060834093,0.));
#247633=CARTESIAN_POINT('Ctrl Pts',(7.66016648045007,22.1842060834093,12.));
#247634=CARTESIAN_POINT('Ctrl Pts',(7.65919341496925,22.1660176731174,0.));
#247635=CARTESIAN_POINT('Ctrl Pts',(7.65919341496925,22.1660176731174,12.));
#247636=CARTESIAN_POINT('Ctrl Pts',(7.6581759596335,22.1479552334206,0.));
#247637=CARTESIAN_POINT('Ctrl Pts',(7.6581759596335,22.1479552334206,12.));
#247638=CARTESIAN_POINT('Ctrl Pts',(7.65711471769406,22.1300198579671,0.));
#247639=CARTESIAN_POINT('Ctrl Pts',(7.65711471769406,22.1300198579671,12.));
#247640=CARTESIAN_POINT('Ctrl Pts',(7.65601030346818,22.1122126563327,0.));
#247641=CARTESIAN_POINT('Ctrl Pts',(7.65601030346818,22.1122126563327,12.));
#247642=CARTESIAN_POINT('Ctrl Pts',(7.6548633426365,22.094534754469,0.));
#247643=CARTESIAN_POINT('Ctrl Pts',(7.6548633426365,22.094534754469,12.));
#247644=CARTESIAN_POINT('Ctrl Pts',(7.65367447254944,22.0769872951596,0.));
#247645=CARTESIAN_POINT('Ctrl Pts',(7.65367447254944,22.0769872951596,12.));
#247646=CARTESIAN_POINT('Ctrl Pts',(7.65244434253103,22.0595714384432,0.));
#247647=CARTESIAN_POINT('Ctrl Pts',(7.65244434253103,22.0595714384432,12.));
#247648=CARTESIAN_POINT('Ctrl Pts',(7.65117361421346,22.0422883621176,0.));
#247649=CARTESIAN_POINT('Ctrl Pts',(7.65117361421346,22.0422883621176,12.));
#247650=CARTESIAN_POINT('Ctrl Pts',(7.64986296190156,22.025139262321,0.));
#247651=CARTESIAN_POINT('Ctrl Pts',(7.64986296190156,22.025139262321,12.));
#247652=CARTESIAN_POINT('Ctrl Pts',(7.64851307293345,22.0081253540774,0.));
#247653=CARTESIAN_POINT('Ctrl Pts',(7.64851307293345,22.0081253540774,12.));
#247654=CARTESIAN_POINT('Ctrl Pts',(7.64712464805257,21.9912478718542,0.));
#247655=CARTESIAN_POINT('Ctrl Pts',(7.64712464805257,21.9912478718542,12.));
#247656=CARTESIAN_POINT('Ctrl Pts',(7.64569840177359,21.97450807008,0.));
#247657=CARTESIAN_POINT('Ctrl Pts',(7.64569840177359,21.97450807008,12.));
#247658=CARTESIAN_POINT('Ctrl Pts',(7.64423506279153,21.9579072237653,0.));
#247659=CARTESIAN_POINT('Ctrl Pts',(7.64423506279153,21.9579072237653,12.));
#247660=CARTESIAN_POINT('Ctrl Pts',(7.64273537442706,21.9414466292074,0.));
#247661=CARTESIAN_POINT('Ctrl Pts',(7.64273537442706,21.9414466292074,12.));
#247662=CARTESIAN_POINT('Ctrl Pts',(7.64120009506539,21.9251276046546,0.));
#247663=CARTESIAN_POINT('Ctrl Pts',(7.64120009506539,21.9251276046546,12.));
#247664=CARTESIAN_POINT('Ctrl Pts',(7.63962999860916,21.9089514909873,0.));
#247665=CARTESIAN_POINT('Ctrl Pts',(7.63962999860916,21.9089514909873,12.));
#247666=CARTESIAN_POINT('Ctrl Pts',(7.63802587492007,21.8929196523511,0.));
#247667=CARTESIAN_POINT('Ctrl Pts',(7.63802587492007,21.8929196523511,12.));
#247668=CARTESIAN_POINT('Ctrl Pts',(7.63638853033367,21.8770334769492,0.));
#247669=CARTESIAN_POINT('Ctrl Pts',(7.63638853033367,21.8770334769492,12.));
#247670=CARTESIAN_POINT('Ctrl Pts',(7.63471878821203,21.8612943779086,0.));
#247671=CARTESIAN_POINT('Ctrl Pts',(7.63471878821203,21.8612943779086,12.));
#247672=CARTESIAN_POINT('Ctrl Pts',(7.63301748948936,21.8457037941084,0.));
#247673=CARTESIAN_POINT('Ctrl Pts',(7.63301748948936,21.8457037941084,12.));
#247674=CARTESIAN_POINT('Ctrl Pts',(7.6312854932304,21.8302631910197,0.));
#247675=CARTESIAN_POINT('Ctrl Pts',(7.6312854932304,21.8302631910197,12.));
#247676=CARTESIAN_POINT('Ctrl Pts',(7.62952367718151,21.8149740615093,0.));
#247677=CARTESIAN_POINT('Ctrl Pts',(7.62952367718151,21.8149740615093,12.));
#247678=CARTESIAN_POINT('Ctrl Pts',(7.62773293842409,21.7998379268583,0.));
#247679=CARTESIAN_POINT('Ctrl Pts',(7.62773293842409,21.7998379268583,12.));
#247680=CARTESIAN_POINT('Ctrl Pts',(7.6259141940452,21.7848563378022,0.));
#247681=CARTESIAN_POINT('Ctrl Pts',(7.6259141940452,21.7848563378022,12.));
#247682=CARTESIAN_POINT('Ctrl Pts',(7.62406838181164,21.7700308755584,0.));
#247683=CARTESIAN_POINT('Ctrl Pts',(7.62406838181164,21.7700308755584,12.));
#247684=CARTESIAN_POINT('Ctrl Pts',(7.62219646084225,21.7553631528329,0.));
#247685=CARTESIAN_POINT('Ctrl Pts',(7.62219646084225,21.7553631528329,12.));
#247686=CARTESIAN_POINT('Ctrl Pts',(7.62029941230854,21.7408548148657,0.));
#247687=CARTESIAN_POINT('Ctrl Pts',(7.62029941230854,21.7408548148657,12.));
#247688=CARTESIAN_POINT('Ctrl Pts',(7.61837824030541,21.7265075407977,0.));
#247689=CARTESIAN_POINT('Ctrl Pts',(7.61837824030541,21.7265075407977,12.));
#247690=CARTESIAN_POINT('Ctrl Pts',(7.61643397270424,21.7123230449835,0.));
#247691=CARTESIAN_POINT('Ctrl Pts',(7.61643397270424,21.7123230449835,12.));
#247692=CARTESIAN_POINT('Ctrl Pts',(7.61446766202786,21.6983030783321,0.));
#247693=CARTESIAN_POINT('Ctrl Pts',(7.61446766202786,21.6983030783321,12.));
#247694=CARTESIAN_POINT('Ctrl Pts',(7.61248038630264,21.6844494295813,0.));
#247695=CARTESIAN_POINT('Ctrl Pts',(7.61248038630264,21.6844494295813,12.));
#247696=CARTESIAN_POINT('Ctrl Pts',(7.61047325000949,21.6707639267573,0.));
#247697=CARTESIAN_POINT('Ctrl Pts',(7.61047325000949,21.6707639267573,12.));
#247698=CARTESIAN_POINT('Ctrl Pts',(7.60844738512871,21.6572484388079,0.));
#247699=CARTESIAN_POINT('Ctrl Pts',(7.60844738512871,21.6572484388079,12.));
#247700=CARTESIAN_POINT('Ctrl Pts',(7.60640395216358,21.6439048771743,0.));
#247701=CARTESIAN_POINT('Ctrl Pts',(7.60640395216358,21.6439048771743,12.));
#247702=CARTESIAN_POINT('Ctrl Pts',(7.60434414118299,21.6307351973823,0.));
#247703=CARTESIAN_POINT('Ctrl Pts',(7.60434414118299,21.6307351973823,12.));
#247704=CARTESIAN_POINT('Ctrl Pts',(7.60226917285431,21.6177414005991,0.));
#247705=CARTESIAN_POINT('Ctrl Pts',(7.60226917285431,21.6177414005991,12.));
#247706=CARTESIAN_POINT('Ctrl Pts',(7.60018029988238,21.6049255358843,0.));
#247707=CARTESIAN_POINT('Ctrl Pts',(7.60018029988238,21.6049255358843,12.));
#247708=CARTESIAN_POINT('Ctrl Pts',(7.59807880846192,21.5922897024466,0.));
#247709=CARTESIAN_POINT('Ctrl Pts',(7.59807880846192,21.5922897024466,12.));
#247710=CARTESIAN_POINT('Ctrl Pts',(7.59596601973588,21.5798360518978,0.));
#247711=CARTESIAN_POINT('Ctrl Pts',(7.59596601973588,21.5798360518978,12.));
#247712=CARTESIAN_POINT('Ctrl Pts',(7.59384329124929,21.5675667904728,0.));
#247713=CARTESIAN_POINT('Ctrl Pts',(7.59384329124929,21.5675667904728,12.));
#247714=CARTESIAN_POINT('Ctrl Pts',(7.59171201844792,21.5554841813466,0.));
#247715=CARTESIAN_POINT('Ctrl Pts',(7.59171201844792,21.5554841813466,12.));
#247716=CARTESIAN_POINT('Ctrl Pts',(7.58957363620026,21.5435905470113,0.));
#247717=CARTESIAN_POINT('Ctrl Pts',(7.58957363620026,21.5435905470113,12.));
#247718=CARTESIAN_POINT('Ctrl Pts',(7.58742962034834,21.5318882716736,0.));
#247719=CARTESIAN_POINT('Ctrl Pts',(7.58742962034834,21.5318882716736,12.));
#247720=CARTESIAN_POINT('Ctrl Pts',(7.58528148919113,21.5203798035294,0.));
#247721=CARTESIAN_POINT('Ctrl Pts',(7.58528148919113,21.5203798035294,12.));
#247722=CARTESIAN_POINT('Ctrl Pts',(7.58313080519158,21.5090676573866,0.));
#247723=CARTESIAN_POINT('Ctrl Pts',(7.58313080519158,21.5090676573866,12.));
#247724=CARTESIAN_POINT('Ctrl Pts',(7.58097917790729,21.497954419274,0.));
#247725=CARTESIAN_POINT('Ctrl Pts',(7.58097917790729,21.497954419274,12.));
#247726=CARTESIAN_POINT('Ctrl Pts',(7.57882826679131,21.4870427508193,0.));
#247727=CARTESIAN_POINT('Ctrl Pts',(7.57882826679131,21.4870427508193,12.));
#247728=CARTESIAN_POINT('Ctrl Pts',(7.57667978403001,21.4763353936766,0.));
#247729=CARTESIAN_POINT('Ctrl Pts',(7.57667978403001,21.4763353936766,12.));
#247730=CARTESIAN_POINT('Ctrl Pts',(7.57453549743434,21.4658351740135,0.));
#247731=CARTESIAN_POINT('Ctrl Pts',(7.57453549743434,21.4658351740135,12.));
#247732=CARTESIAN_POINT('Ctrl Pts',(7.57239723223521,21.4555450053147,0.));
#247733=CARTESIAN_POINT('Ctrl Pts',(7.57239723223521,21.4555450053147,12.));
#247734=CARTESIAN_POINT('Ctrl Pts',(7.57026687261169,21.445467890751,0.));
#247735=CARTESIAN_POINT('Ctrl Pts',(7.57026687261169,21.445467890751,12.));
#247736=CARTESIAN_POINT('Ctrl Pts',(7.56814636360841,21.435606926151,0.));
#247737=CARTESIAN_POINT('Ctrl Pts',(7.56814636360841,21.435606926151,12.));
#247738=CARTESIAN_POINT('Ctrl Pts',(7.56603771218706,21.4259653015732,0.));
#247739=CARTESIAN_POINT('Ctrl Pts',(7.56603771218706,21.4259653015732,12.));
#247740=CARTESIAN_POINT('Ctrl Pts',(7.56394299313682,21.4165463106252,0.));
#247741=CARTESIAN_POINT('Ctrl Pts',(7.56394299313682,21.4165463106252,12.));
#247742=CARTESIAN_POINT('Ctrl Pts',(7.56186435703622,21.4073533630364,0.));
#247743=CARTESIAN_POINT('Ctrl Pts',(7.56186435703622,21.4073533630364,12.));
#247744=CARTESIAN_POINT('Ctrl Pts',(7.55980403700614,21.3983899952988,0.));
#247745=CARTESIAN_POINT('Ctrl Pts',(7.55980403700614,21.3983899952988,12.));
#247746=CARTESIAN_POINT('Ctrl Pts',(7.55776435731421,21.3896598842119,0.));
#247747=CARTESIAN_POINT('Ctrl Pts',(7.55776435731421,21.3896598842119,12.));
#247748=CARTESIAN_POINT('Ctrl Pts',(7.55574773403507,21.3811668478933,0.));
#247749=CARTESIAN_POINT('Ctrl Pts',(7.55574773403507,21.3811668478933,12.));
#247750=CARTESIAN_POINT('Ctrl Pts',(7.55375667080031,21.3729148390244,0.));
#247751=CARTESIAN_POINT('Ctrl Pts',(7.55375667080031,21.3729148390244,12.));
#247752=CARTESIAN_POINT('Ctrl Pts',(7.55179375777441,21.3649079431864,0.));
#247753=CARTESIAN_POINT('Ctrl Pts',(7.55179375777441,21.3649079431864,12.));
#247754=CARTESIAN_POINT('Ctrl Pts',(7.54986166521306,21.3571503685853,0.));
#247755=CARTESIAN_POINT('Ctrl Pts',(7.54986166521306,21.3571503685853,12.));
#247756=CARTESIAN_POINT('Ctrl Pts',(7.54796316246326,21.349646476153,0.));
#247757=CARTESIAN_POINT('Ctrl Pts',(7.54796316246326,21.349646476153,12.));
#247758=CARTESIAN_POINT('Ctrl Pts',(7.5461011494835,21.3424008295038,0.));
#247759=CARTESIAN_POINT('Ctrl Pts',(7.5461011494835,21.3424008295038,12.));
#247760=CARTESIAN_POINT('Ctrl Pts',(7.54427868151268,21.3354182340149,0.));
#247761=CARTESIAN_POINT('Ctrl Pts',(7.54427868151268,21.3354182340149,12.));
#247762=CARTESIAN_POINT('Ctrl Pts',(7.54249900377031,21.328703791771,0.));
#247763=CARTESIAN_POINT('Ctrl Pts',(7.54249900377031,21.328703791771,12.));
#247764=CARTESIAN_POINT('Ctrl Pts',(7.54076552038279,21.3222628524165,0.));
#247765=CARTESIAN_POINT('Ctrl Pts',(7.54076552038279,21.3222628524165,12.));
#247766=CARTESIAN_POINT('Ctrl Pts',(7.53908175169898,21.3161009456256,0.));
#247767=CARTESIAN_POINT('Ctrl Pts',(7.53908175169898,21.3161009456256,12.));
#247768=CARTESIAN_POINT('Ctrl Pts',(7.53745129364619,21.3102237167729,0.));
#247769=CARTESIAN_POINT('Ctrl Pts',(7.53745129364619,21.3102237167729,12.));
#247770=CARTESIAN_POINT('Ctrl Pts',(7.53587778251743,21.3046368712157,0.));
#247771=CARTESIAN_POINT('Ctrl Pts',(7.53587778251743,21.3046368712157,12.));
#247772=CARTESIAN_POINT('Ctrl Pts',(7.53436505309948,21.2993464250717,0.));
#247773=CARTESIAN_POINT('Ctrl Pts',(7.53436505309948,21.2993464250717,12.));
#247774=CARTESIAN_POINT('Ctrl Pts',(7.53291726078526,21.2943588989331,0.));
#247775=CARTESIAN_POINT('Ctrl Pts',(7.53291726078526,21.2943588989331,12.));
#247776=CARTESIAN_POINT('Ctrl Pts',(7.53153906987846,21.2896816163843,0.));
#247777=CARTESIAN_POINT('Ctrl Pts',(7.53153906987846,21.2896816163843,12.));
#247778=CARTESIAN_POINT('Ctrl Pts',(7.5302356243822,21.2853226580658,0.));
#247779=CARTESIAN_POINT('Ctrl Pts',(7.5302356243822,21.2853226580658,12.));
#247780=CARTESIAN_POINT('Ctrl Pts',(7.52901217930407,21.2812902781143,0.));
#247781=CARTESIAN_POINT('Ctrl Pts',(7.52901217930407,21.2812902781143,12.));
#247782=CARTESIAN_POINT('Ctrl Pts',(7.52787386225343,21.2775925269652,0.));
#247783=CARTESIAN_POINT('Ctrl Pts',(7.52787386225343,21.2775925269652,12.));
#247784=CARTESIAN_POINT('Ctrl Pts',(7.5268252691856,21.2742366113578,0.));
#247785=CARTESIAN_POINT('Ctrl Pts',(7.5268252691856,21.2742366113578,12.));
#247786=CARTESIAN_POINT('Ctrl Pts',(7.52587126095544,21.2712301573465,0.));
#247787=CARTESIAN_POINT('Ctrl Pts',(7.52587126095544,21.2712301573465,12.));
#247788=CARTESIAN_POINT('Ctrl Pts',(7.52501770333521,21.2685823838672,0.));
#247789=CARTESIAN_POINT('Ctrl Pts',(7.52501770333521,21.2685823838672,12.));
#247790=CARTESIAN_POINT('Ctrl Pts',(7.52427261074263,21.266305915706,0.));
#247791=CARTESIAN_POINT('Ctrl Pts',(7.52427261074263,21.266305915706,12.));
#247792=CARTESIAN_POINT('Ctrl Pts',(7.52364573027521,21.2644161259965,0.));
#247793=CARTESIAN_POINT('Ctrl Pts',(7.52364573027521,21.2644161259965,12.));
#247794=CARTESIAN_POINT('Ctrl Pts',(7.52314642316202,21.262927782038,0.));
#247795=CARTESIAN_POINT('Ctrl Pts',(7.52314642316202,21.262927782038,12.));
#247796=CARTESIAN_POINT('Ctrl Pts',(7.52278182242727,21.261852128355,0.));
#247797=CARTESIAN_POINT('Ctrl Pts',(7.52278182242727,21.261852128355,12.));
#247798=CARTESIAN_POINT('Ctrl Pts',(7.52260064231736,21.2613260540651,0.));
#247799=CARTESIAN_POINT('Ctrl Pts',(7.52260064231736,21.2613260540651,12.));
#247800=CARTESIAN_POINT('Ctrl Pts',(7.52252744144957,21.261120447486,0.));
#247801=CARTESIAN_POINT('Ctrl Pts',(7.52252744144957,21.261120447486,12.));
#247802=CARTESIAN_POINT('Ctrl Pts',(7.52250649703991,21.2610673466883,0.));
#247803=CARTESIAN_POINT('Ctrl Pts',(7.52250649703991,21.2610673466883,12.));
#247804=CARTESIAN_POINT('Ctrl Pts',(7.52250298901265,21.2610617890679,0.));
#247805=CARTESIAN_POINT('Ctrl Pts',(7.52250298901265,21.2610617890679,12.));
#247806=CARTESIAN_POINT('',(7.36589684767344,24.9347862158358,0.));
#247807=CARTESIAN_POINT('Ctrl Pts',(7.36589684767344,24.9347862158358,0.));
#247808=CARTESIAN_POINT('Ctrl Pts',(7.36721909028842,24.9292275670674,0.));
#247809=CARTESIAN_POINT('Ctrl Pts',(7.3698559312009,24.9181155530543,0.));
#247810=CARTESIAN_POINT('Ctrl Pts',(7.37378825961676,24.901463382605,0.));
#247811=CARTESIAN_POINT('Ctrl Pts',(7.37898549640269,24.8792921911115,0.));
#247812=CARTESIAN_POINT('Ctrl Pts',(7.3854055890362,24.8516310625176,0.));
#247813=CARTESIAN_POINT('Ctrl Pts',(7.39174922585808,24.8240228520893,0.));
#247814=CARTESIAN_POINT('Ctrl Pts',(7.39801641583012,24.7964676646431,0.));
#247815=CARTESIAN_POINT('Ctrl Pts',(7.40420718661602,24.7689656668983,0.));
#247816=CARTESIAN_POINT('Ctrl Pts',(7.41032159082381,24.7415170994784,0.));
#247817=CARTESIAN_POINT('Ctrl Pts',(7.41635971481674,24.7141222950051,0.));
#247818=CARTESIAN_POINT('Ctrl Pts',(7.42232167766265,24.6867816727192,0.));
#247819=CARTESIAN_POINT('Ctrl Pts',(7.42820762159125,24.6594957128756,0.));
#247820=CARTESIAN_POINT('Ctrl Pts',(7.43401770489523,24.6322649369517,0.));
#247821=CARTESIAN_POINT('Ctrl Pts',(7.43975209375503,24.6050898852368,0.));
#247822=CARTESIAN_POINT('Ctrl Pts',(7.44541095473134,24.577971096086,0.));
#247823=CARTESIAN_POINT('Ctrl Pts',(7.4509944465116,24.5509090831559,0.));
#247824=CARTESIAN_POINT('Ctrl Pts',(7.45650271335861,24.5239043173072,0.));
#247825=CARTESIAN_POINT('Ctrl Pts',(7.46193588961463,24.4969572391483,0.));
#247826=CARTESIAN_POINT('Ctrl Pts',(7.46729410308786,24.4700682684524,0.));
#247827=CARTESIAN_POINT('Ctrl Pts',(7.47257747883246,24.443237814649,0.));
#247828=CARTESIAN_POINT('Ctrl Pts',(7.47778614286564,24.4164662871163,0.));
#247829=CARTESIAN_POINT('Ctrl Pts',(7.482920225693,24.3897541049254,0.));
#247830=CARTESIAN_POINT('Ctrl Pts',(7.48797986651908,24.3631017084524,0.));
#247831=CARTESIAN_POINT('Ctrl Pts',(7.4929652125242,24.3365095573685,0.));
#247832=CARTESIAN_POINT('Ctrl Pts',(7.49787641695438,24.3099781253355,0.));
#247833=CARTESIAN_POINT('Ctrl Pts',(7.50271363765151,24.2835078958973,0.));
#247834=CARTESIAN_POINT('Ctrl Pts',(7.50747703535133,24.2570993577034,0.));
#247835=CARTESIAN_POINT('Ctrl Pts',(7.5121667722218,24.2307530003887,0.));
#247836=CARTESIAN_POINT('Ctrl Pts',(7.51678300997949,24.2044693092349,0.));
#247837=CARTESIAN_POINT('Ctrl Pts',(7.52132590953801,24.1782487641594,0.));
#247838=CARTESIAN_POINT('Ctrl Pts',(7.52579563201423,24.1520918425364,0.));
#247839=CARTESIAN_POINT('Ctrl Pts',(7.53019233935501,24.1259990209207,0.));
#247840=CARTESIAN_POINT('Ctrl Pts',(7.53451619514649,24.0999707772642,0.));
#247841=CARTESIAN_POINT('Ctrl Pts',(7.53876736531013,24.0740075927985,0.));
#247842=CARTESIAN_POINT('Ctrl Pts',(7.54294601896144,24.0481099543353,0.));
#247843=CARTESIAN_POINT('Ctrl Pts',(7.5470523288591,24.022278355453,0.));
#247844=CARTESIAN_POINT('Ctrl Pts',(7.5510864709744,23.9965132953185,0.));
#247845=CARTESIAN_POINT('Ctrl Pts',(7.55504862424811,23.9708152779884,0.));
#247846=CARTESIAN_POINT('Ctrl Pts',(7.55893897027682,23.9451848115,0.));
#247847=CARTESIAN_POINT('Ctrl Pts',(7.56275769304773,23.9196224070759,0.));
#247848=CARTESIAN_POINT('Ctrl Pts',(7.56650497863791,23.8941285782003,0.));
#247849=CARTESIAN_POINT('Ctrl Pts',(7.5701810150071,23.8687038399598,0.));
#247850=CARTESIAN_POINT('Ctrl Pts',(7.57378599219816,23.8433487096134,0.));
#247851=CARTESIAN_POINT('Ctrl Pts',(7.57732010249065,23.8180637069977,0.));
#247852=CARTESIAN_POINT('Ctrl Pts',(7.58078354058211,23.7928493549908,0.));
#247853=CARTESIAN_POINT('Ctrl Pts',(7.58417650376271,23.7677061799376,0.));
#247854=CARTESIAN_POINT('Ctrl Pts',(7.58749919210831,23.7426347121006,0.));
#247855=CARTESIAN_POINT('Ctrl Pts',(7.59075180865326,23.7176354860457,0.));
#247856=CARTESIAN_POINT('Ctrl Pts',(7.59393455934041,23.6927090405067,0.));
#247857=CARTESIAN_POINT('Ctrl Pts',(7.59704765299572,23.6678559182876,0.));
#247858=CARTESIAN_POINT('Ctrl Pts',(7.60009130130129,23.6430766661419,0.));
#247859=CARTESIAN_POINT('Ctrl Pts',(7.60306571877806,23.6183718346576,0.));
#247860=CARTESIAN_POINT('Ctrl Pts',(7.60597112277094,23.5937419781244,0.));
#247861=CARTESIAN_POINT('Ctrl Pts',(7.60880773344599,23.5691876544243,0.));
#247862=CARTESIAN_POINT('Ctrl Pts',(7.61157577385371,23.5447094252029,0.));
#247863=CARTESIAN_POINT('Ctrl Pts',(7.61427546999298,23.5203078560128,0.));
#247864=CARTESIAN_POINT('Ctrl Pts',(7.61690705088318,23.4959835164608,0.));
#247865=CARTESIAN_POINT('Ctrl Pts',(7.61947074863977,23.4717369803438,0.));
#247866=CARTESIAN_POINT('Ctrl Pts',(7.62196679855957,23.4475688257855,0.));
#247867=CARTESIAN_POINT('Ctrl Pts',(7.62439543920053,23.4234796353544,0.));
#247868=CARTESIAN_POINT('Ctrl Pts',(7.62675691240334,23.3994699961122,0.));
#247869=CARTESIAN_POINT('Ctrl Pts',(7.62905146332597,23.3755404996638,0.));
#247870=CARTESIAN_POINT('Ctrl Pts',(7.63127934048138,23.3516917421973,0.));
#247871=CARTESIAN_POINT('Ctrl Pts',(7.63344079578162,23.3279243245241,0.));
#247872=CARTESIAN_POINT('Ctrl Pts',(7.63553608458783,23.3042388521021,0.));
#247873=CARTESIAN_POINT('Ctrl Pts',(7.63756546576374,23.2806359350853,0.));
#247874=CARTESIAN_POINT('Ctrl Pts',(7.63952920172837,23.2571161884487,0.));
#247875=CARTESIAN_POINT('Ctrl Pts',(7.64142755851507,23.2336802320912,0.));
#247876=CARTESIAN_POINT('Ctrl Pts',(7.64326080583683,23.2103286909399,0.));
#247877=CARTESIAN_POINT('Ctrl Pts',(7.64502921715482,23.1870621950452,0.));
#247878=CARTESIAN_POINT('Ctrl Pts',(7.64673306975796,23.1638813796691,0.));
#247879=CARTESIAN_POINT('Ctrl Pts',(7.64837264482929,23.1407868853815,0.));
#247880=CARTESIAN_POINT('Ctrl Pts',(7.64994822749844,23.1177793581674,0.));
#247881=CARTESIAN_POINT('Ctrl Pts',(7.65146010690464,23.0948594495246,0.));
#247882=CARTESIAN_POINT('Ctrl Pts',(7.65290857626356,23.072027816555,0.));
#247883=CARTESIAN_POINT('Ctrl Pts',(7.65429393293955,23.049285122053,0.));
#247884=CARTESIAN_POINT('Ctrl Pts',(7.65561647852554,23.0266320345792,0.));
#247885=CARTESIAN_POINT('Ctrl Pts',(7.6568765189133,23.004069228582,0.));
#247886=CARTESIAN_POINT('Ctrl Pts',(7.65807436436452,22.9815973845301,0.));
#247887=CARTESIAN_POINT('Ctrl Pts',(7.65921032958911,22.9592171890332,0.));
#247888=CARTESIAN_POINT('Ctrl Pts',(7.66028473382776,22.9369293349592,0.));
#247889=CARTESIAN_POINT('Ctrl Pts',(7.66129790094099,22.9147345215418,0.));
#247890=CARTESIAN_POINT('Ctrl Pts',(7.66225015950147,22.8926334544879,0.));
#247891=CARTESIAN_POINT('Ctrl Pts',(7.66314184287333,22.870626846128,0.));
#247892=CARTESIAN_POINT('Ctrl Pts',(7.66397328929805,22.8487154155569,0.));
#247893=CARTESIAN_POINT('Ctrl Pts',(7.66474484198552,22.8268998887679,0.));
#247894=CARTESIAN_POINT('Ctrl Pts',(7.66545684920987,22.8051809987834,0.));
#247895=CARTESIAN_POINT('Ctrl Pts',(7.66610966441259,22.7835594857697,0.));
#247896=CARTESIAN_POINT('Ctrl Pts',(7.66670364630273,22.7620360971839,0.));
#247897=CARTESIAN_POINT('Ctrl Pts',(7.66723915895412,22.7406115879508,0.));
#247898=CARTESIAN_POINT('Ctrl Pts',(7.6677165719101,22.7192867206242,0.));
#247899=CARTESIAN_POINT('Ctrl Pts',(7.66813626029276,22.6980622655446,0.));
#247900=CARTESIAN_POINT('Ctrl Pts',(7.66849860491762,22.6769390009889,0.));
#247901=CARTESIAN_POINT('Ctrl Pts',(7.66880399241353,22.6559177133133,0.));
#247902=CARTESIAN_POINT('Ctrl Pts',(7.66905281533744,22.6349991971548,0.));
#247903=CARTESIAN_POINT('Ctrl Pts',(7.66924547229434,22.6141842556248,0.));
#247904=CARTESIAN_POINT('Ctrl Pts',(7.6693823680624,22.5934737004955,0.));
#247905=CARTESIAN_POINT('Ctrl Pts',(7.66946391372299,22.5728683523829,0.));
#247906=CARTESIAN_POINT('Ctrl Pts',(7.66949052679671,22.5523690409109,0.));
#247907=CARTESIAN_POINT('Ctrl Pts',(7.66946263138115,22.5319766049191,0.));
#247908=CARTESIAN_POINT('Ctrl Pts',(7.66938065829082,22.5116918927023,0.));
#247909=CARTESIAN_POINT('Ctrl Pts',(7.66924504520301,22.4915157622308,0.));
#247910=CARTESIAN_POINT('Ctrl Pts',(7.66905623680835,22.47144908137,0.));
#247911=CARTESIAN_POINT('Ctrl Pts',(7.66881468496659,22.4514927280863,0.));
#247912=CARTESIAN_POINT('Ctrl Pts',(7.66852084886745,22.4316475906616,0.));
#247913=CARTESIAN_POINT('Ctrl Pts',(7.66817519519681,22.411914567977,0.));
#247914=CARTESIAN_POINT('Ctrl Pts',(7.66777819830819,22.3922945697782,0.));
#247915=CARTESIAN_POINT('Ctrl Pts',(7.66733034039887,22.3727885169361,0.));
#247916=CARTESIAN_POINT('Ctrl Pts',(7.66683211169133,22.3533973417013,0.));
#247917=CARTESIAN_POINT('Ctrl Pts',(7.66628401061905,22.3341219879454,0.));
#247918=CARTESIAN_POINT('Ctrl Pts',(7.66568654402441,22.3149634114823,0.));
#247919=CARTESIAN_POINT('Ctrl Pts',(7.66504022736262,22.2959225803925,0.));
#247920=CARTESIAN_POINT('Ctrl Pts',(7.66434558490972,22.2770004753332,0.));
#247921=CARTESIAN_POINT('Ctrl Pts',(7.66360314997661,22.2581980898487,0.));
#247922=CARTESIAN_POINT('Ctrl Pts',(7.66281346512545,22.239516430656,0.));
#247923=CARTESIAN_POINT('Ctrl Pts',(7.66197708240435,22.2209565180098,0.));
#247924=CARTESIAN_POINT('Ctrl Pts',(7.66109456359292,22.2025193860972,0.));
#247925=CARTESIAN_POINT('Ctrl Pts',(7.66016648045007,22.1842060834093,0.));
#247926=CARTESIAN_POINT('Ctrl Pts',(7.65919341496925,22.1660176731174,0.));
#247927=CARTESIAN_POINT('Ctrl Pts',(7.6581759596335,22.1479552334206,0.));
#247928=CARTESIAN_POINT('Ctrl Pts',(7.65711471769406,22.1300198579671,0.));
#247929=CARTESIAN_POINT('Ctrl Pts',(7.65601030346818,22.1122126563327,0.));
#247930=CARTESIAN_POINT('Ctrl Pts',(7.6548633426365,22.094534754469,0.));
#247931=CARTESIAN_POINT('Ctrl Pts',(7.65367447254944,22.0769872951596,0.));
#247932=CARTESIAN_POINT('Ctrl Pts',(7.65244434253103,22.0595714384432,0.));
#247933=CARTESIAN_POINT('Ctrl Pts',(7.65117361421346,22.0422883621176,0.));
#247934=CARTESIAN_POINT('Ctrl Pts',(7.64986296190156,22.025139262321,0.));
#247935=CARTESIAN_POINT('Ctrl Pts',(7.64851307293345,22.0081253540774,0.));
#247936=CARTESIAN_POINT('Ctrl Pts',(7.64712464805257,21.9912478718542,0.));
#247937=CARTESIAN_POINT('Ctrl Pts',(7.64569840177359,21.97450807008,0.));
#247938=CARTESIAN_POINT('Ctrl Pts',(7.64423506279153,21.9579072237653,0.));
#247939=CARTESIAN_POINT('Ctrl Pts',(7.64273537442706,21.9414466292074,0.));
#247940=CARTESIAN_POINT('Ctrl Pts',(7.64120009506539,21.9251276046546,0.));
#247941=CARTESIAN_POINT('Ctrl Pts',(7.63962999860916,21.9089514909873,0.));
#247942=CARTESIAN_POINT('Ctrl Pts',(7.63802587492007,21.8929196523511,0.));
#247943=CARTESIAN_POINT('Ctrl Pts',(7.63638853033367,21.8770334769492,0.));
#247944=CARTESIAN_POINT('Ctrl Pts',(7.63471878821203,21.8612943779086,0.));
#247945=CARTESIAN_POINT('Ctrl Pts',(7.63301748948936,21.8457037941084,0.));
#247946=CARTESIAN_POINT('Ctrl Pts',(7.6312854932304,21.8302631910197,0.));
#247947=CARTESIAN_POINT('Ctrl Pts',(7.62952367718151,21.8149740615093,0.));
#247948=CARTESIAN_POINT('Ctrl Pts',(7.62773293842409,21.7998379268583,0.));
#247949=CARTESIAN_POINT('Ctrl Pts',(7.6259141940452,21.7848563378022,0.));
#247950=CARTESIAN_POINT('Ctrl Pts',(7.62406838181164,21.7700308755584,0.));
#247951=CARTESIAN_POINT('Ctrl Pts',(7.62219646084225,21.7553631528329,0.));
#247952=CARTESIAN_POINT('Ctrl Pts',(7.62029941230854,21.7408548148657,0.));
#247953=CARTESIAN_POINT('Ctrl Pts',(7.61837824030541,21.7265075407977,0.));
#247954=CARTESIAN_POINT('Ctrl Pts',(7.61643397270424,21.7123230449835,0.));
#247955=CARTESIAN_POINT('Ctrl Pts',(7.61446766202786,21.6983030783321,0.));
#247956=CARTESIAN_POINT('Ctrl Pts',(7.61248038630264,21.6844494295813,0.));
#247957=CARTESIAN_POINT('Ctrl Pts',(7.61047325000949,21.6707639267573,0.));
#247958=CARTESIAN_POINT('Ctrl Pts',(7.60844738512871,21.6572484388079,0.));
#247959=CARTESIAN_POINT('Ctrl Pts',(7.60640395216358,21.6439048771743,0.));
#247960=CARTESIAN_POINT('Ctrl Pts',(7.60434414118299,21.6307351973823,0.));
#247961=CARTESIAN_POINT('Ctrl Pts',(7.60226917285431,21.6177414005991,0.));
#247962=CARTESIAN_POINT('Ctrl Pts',(7.60018029988238,21.6049255358843,0.));
#247963=CARTESIAN_POINT('Ctrl Pts',(7.59807880846192,21.5922897024466,0.));
#247964=CARTESIAN_POINT('Ctrl Pts',(7.59596601973588,21.5798360518978,0.));
#247965=CARTESIAN_POINT('Ctrl Pts',(7.59384329124929,21.5675667904728,0.));
#247966=CARTESIAN_POINT('Ctrl Pts',(7.59171201844792,21.5554841813466,0.));
#247967=CARTESIAN_POINT('Ctrl Pts',(7.58957363620026,21.5435905470113,0.));
#247968=CARTESIAN_POINT('Ctrl Pts',(7.58742962034834,21.5318882716736,0.));
#247969=CARTESIAN_POINT('Ctrl Pts',(7.58528148919113,21.5203798035294,0.));
#247970=CARTESIAN_POINT('Ctrl Pts',(7.58313080519158,21.5090676573866,0.));
#247971=CARTESIAN_POINT('Ctrl Pts',(7.58097917790729,21.497954419274,0.));
#247972=CARTESIAN_POINT('Ctrl Pts',(7.57882826679131,21.4870427508193,0.));
#247973=CARTESIAN_POINT('Ctrl Pts',(7.57667978403001,21.4763353936766,0.));
#247974=CARTESIAN_POINT('Ctrl Pts',(7.57453549743434,21.4658351740135,0.));
#247975=CARTESIAN_POINT('Ctrl Pts',(7.57239723223521,21.4555450053147,0.));
#247976=CARTESIAN_POINT('Ctrl Pts',(7.57026687261169,21.445467890751,0.));
#247977=CARTESIAN_POINT('Ctrl Pts',(7.56814636360841,21.435606926151,0.));
#247978=CARTESIAN_POINT('Ctrl Pts',(7.56603771218706,21.4259653015732,0.));
#247979=CARTESIAN_POINT('Ctrl Pts',(7.56394299313682,21.4165463106252,0.));
#247980=CARTESIAN_POINT('Ctrl Pts',(7.56186435703622,21.4073533630364,0.));
#247981=CARTESIAN_POINT('Ctrl Pts',(7.55980403700614,21.3983899952988,0.));
#247982=CARTESIAN_POINT('Ctrl Pts',(7.55776435731421,21.3896598842119,0.));
#247983=CARTESIAN_POINT('Ctrl Pts',(7.55574773403507,21.3811668478933,0.));
#247984=CARTESIAN_POINT('Ctrl Pts',(7.55375667080031,21.3729148390244,0.));
#247985=CARTESIAN_POINT('Ctrl Pts',(7.55179375777441,21.3649079431864,0.));
#247986=CARTESIAN_POINT('Ctrl Pts',(7.54986166521306,21.3571503685853,0.));
#247987=CARTESIAN_POINT('Ctrl Pts',(7.54796316246326,21.349646476153,0.));
#247988=CARTESIAN_POINT('Ctrl Pts',(7.5461011494835,21.3424008295038,0.));
#247989=CARTESIAN_POINT('Ctrl Pts',(7.54427868151268,21.3354182340149,0.));
#247990=CARTESIAN_POINT('Ctrl Pts',(7.54249900377031,21.328703791771,0.));
#247991=CARTESIAN_POINT('Ctrl Pts',(7.54076552038279,21.3222628524165,0.));
#247992=CARTESIAN_POINT('Ctrl Pts',(7.53908175169898,21.3161009456256,0.));
#247993=CARTESIAN_POINT('Ctrl Pts',(7.53745129364619,21.3102237167729,0.));
#247994=CARTESIAN_POINT('Ctrl Pts',(7.53587778251743,21.3046368712157,0.));
#247995=CARTESIAN_POINT('Ctrl Pts',(7.53436505309948,21.2993464250717,0.));
#247996=CARTESIAN_POINT('Ctrl Pts',(7.53291726078526,21.2943588989331,0.));
#247997=CARTESIAN_POINT('Ctrl Pts',(7.53153906987846,21.2896816163843,0.));
#247998=CARTESIAN_POINT('Ctrl Pts',(7.5302356243822,21.2853226580658,0.));
#247999=CARTESIAN_POINT('Ctrl Pts',(7.52901217930407,21.2812902781143,0.));
#248000=CARTESIAN_POINT('Ctrl Pts',(7.52787386225343,21.2775925269652,0.));
#248001=CARTESIAN_POINT('Ctrl Pts',(7.5268252691856,21.2742366113578,0.));
#248002=CARTESIAN_POINT('Ctrl Pts',(7.52587126095544,21.2712301573465,0.));
#248003=CARTESIAN_POINT('Ctrl Pts',(7.52501770333521,21.2685823838672,0.));
#248004=CARTESIAN_POINT('Ctrl Pts',(7.52427261074263,21.266305915706,0.));
#248005=CARTESIAN_POINT('Ctrl Pts',(7.52364573027521,21.2644161259965,0.));
#248006=CARTESIAN_POINT('Ctrl Pts',(7.52314642316202,21.262927782038,0.));
#248007=CARTESIAN_POINT('Ctrl Pts',(7.52278182242727,21.261852128355,0.));
#248008=CARTESIAN_POINT('Ctrl Pts',(7.52260064231736,21.2613260540651,0.));
#248009=CARTESIAN_POINT('Ctrl Pts',(7.52252744144957,21.261120447486,0.));
#248010=CARTESIAN_POINT('Ctrl Pts',(7.52250649703991,21.2610673466883,0.));
#248011=CARTESIAN_POINT('Ctrl Pts',(7.52250298901265,21.2610617890679,0.));
#248012=CARTESIAN_POINT('',(7.36589684767344,24.9347862158358,12.));
#248013=CARTESIAN_POINT('',(7.36589684767344,24.9347862158358,0.));
#248014=CARTESIAN_POINT('Ctrl Pts',(7.52250298901265,21.2610617890679,12.));
#248015=CARTESIAN_POINT('Ctrl Pts',(7.52250649703991,21.2610673466883,12.));
#248016=CARTESIAN_POINT('Ctrl Pts',(7.52252744144957,21.261120447486,12.));
#248017=CARTESIAN_POINT('Ctrl Pts',(7.52260064231736,21.2613260540651,12.));
#248018=CARTESIAN_POINT('Ctrl Pts',(7.52278182242727,21.261852128355,12.));
#248019=CARTESIAN_POINT('Ctrl Pts',(7.52314642316202,21.262927782038,12.));
#248020=CARTESIAN_POINT('Ctrl Pts',(7.52364573027521,21.2644161259965,12.));
#248021=CARTESIAN_POINT('Ctrl Pts',(7.52427261074263,21.266305915706,12.));
#248022=CARTESIAN_POINT('Ctrl Pts',(7.52501770333521,21.2685823838672,12.));
#248023=CARTESIAN_POINT('Ctrl Pts',(7.52587126095544,21.2712301573465,12.));
#248024=CARTESIAN_POINT('Ctrl Pts',(7.5268252691856,21.2742366113578,12.));
#248025=CARTESIAN_POINT('Ctrl Pts',(7.52787386225343,21.2775925269652,12.));
#248026=CARTESIAN_POINT('Ctrl Pts',(7.52901217930407,21.2812902781143,12.));
#248027=CARTESIAN_POINT('Ctrl Pts',(7.5302356243822,21.2853226580658,12.));
#248028=CARTESIAN_POINT('Ctrl Pts',(7.53153906987846,21.2896816163843,12.));
#248029=CARTESIAN_POINT('Ctrl Pts',(7.53291726078526,21.2943588989331,12.));
#248030=CARTESIAN_POINT('Ctrl Pts',(7.53436505309948,21.2993464250717,12.));
#248031=CARTESIAN_POINT('Ctrl Pts',(7.53587778251743,21.3046368712157,12.));
#248032=CARTESIAN_POINT('Ctrl Pts',(7.53745129364619,21.3102237167729,12.));
#248033=CARTESIAN_POINT('Ctrl Pts',(7.53908175169898,21.3161009456256,12.));
#248034=CARTESIAN_POINT('Ctrl Pts',(7.54076552038279,21.3222628524165,12.));
#248035=CARTESIAN_POINT('Ctrl Pts',(7.54249900377031,21.328703791771,12.));
#248036=CARTESIAN_POINT('Ctrl Pts',(7.54427868151268,21.3354182340149,12.));
#248037=CARTESIAN_POINT('Ctrl Pts',(7.5461011494835,21.3424008295038,12.));
#248038=CARTESIAN_POINT('Ctrl Pts',(7.54796316246326,21.349646476153,12.));
#248039=CARTESIAN_POINT('Ctrl Pts',(7.54986166521306,21.3571503685853,12.));
#248040=CARTESIAN_POINT('Ctrl Pts',(7.55179375777441,21.3649079431864,12.));
#248041=CARTESIAN_POINT('Ctrl Pts',(7.55375667080031,21.3729148390244,12.));
#248042=CARTESIAN_POINT('Ctrl Pts',(7.55574773403507,21.3811668478933,12.));
#248043=CARTESIAN_POINT('Ctrl Pts',(7.55776435731421,21.3896598842119,12.));
#248044=CARTESIAN_POINT('Ctrl Pts',(7.55980403700614,21.3983899952988,12.));
#248045=CARTESIAN_POINT('Ctrl Pts',(7.56186435703622,21.4073533630364,12.));
#248046=CARTESIAN_POINT('Ctrl Pts',(7.56394299313682,21.4165463106252,12.));
#248047=CARTESIAN_POINT('Ctrl Pts',(7.56603771218706,21.4259653015732,12.));
#248048=CARTESIAN_POINT('Ctrl Pts',(7.56814636360841,21.435606926151,12.));
#248049=CARTESIAN_POINT('Ctrl Pts',(7.57026687261169,21.445467890751,12.));
#248050=CARTESIAN_POINT('Ctrl Pts',(7.57239723223521,21.4555450053147,12.));
#248051=CARTESIAN_POINT('Ctrl Pts',(7.57453549743434,21.4658351740135,12.));
#248052=CARTESIAN_POINT('Ctrl Pts',(7.57667978403001,21.4763353936766,12.));
#248053=CARTESIAN_POINT('Ctrl Pts',(7.57882826679131,21.4870427508193,12.));
#248054=CARTESIAN_POINT('Ctrl Pts',(7.58097917790729,21.497954419274,12.));
#248055=CARTESIAN_POINT('Ctrl Pts',(7.58313080519158,21.5090676573866,12.));
#248056=CARTESIAN_POINT('Ctrl Pts',(7.58528148919113,21.5203798035294,12.));
#248057=CARTESIAN_POINT('Ctrl Pts',(7.58742962034834,21.5318882716736,12.));
#248058=CARTESIAN_POINT('Ctrl Pts',(7.58957363620026,21.5435905470113,12.));
#248059=CARTESIAN_POINT('Ctrl Pts',(7.59171201844792,21.5554841813466,12.));
#248060=CARTESIAN_POINT('Ctrl Pts',(7.59384329124929,21.5675667904728,12.));
#248061=CARTESIAN_POINT('Ctrl Pts',(7.59596601973588,21.5798360518978,12.));
#248062=CARTESIAN_POINT('Ctrl Pts',(7.59807880846192,21.5922897024466,12.));
#248063=CARTESIAN_POINT('Ctrl Pts',(7.60018029988238,21.6049255358843,12.));
#248064=CARTESIAN_POINT('Ctrl Pts',(7.60226917285431,21.6177414005991,12.));
#248065=CARTESIAN_POINT('Ctrl Pts',(7.60434414118299,21.6307351973823,12.));
#248066=CARTESIAN_POINT('Ctrl Pts',(7.60640395216358,21.6439048771743,12.));
#248067=CARTESIAN_POINT('Ctrl Pts',(7.60844738512871,21.6572484388079,12.));
#248068=CARTESIAN_POINT('Ctrl Pts',(7.61047325000949,21.6707639267573,12.));
#248069=CARTESIAN_POINT('Ctrl Pts',(7.61248038630264,21.6844494295813,12.));
#248070=CARTESIAN_POINT('Ctrl Pts',(7.61446766202786,21.6983030783321,12.));
#248071=CARTESIAN_POINT('Ctrl Pts',(7.61643397270424,21.7123230449835,12.));
#248072=CARTESIAN_POINT('Ctrl Pts',(7.61837824030541,21.7265075407977,12.));
#248073=CARTESIAN_POINT('Ctrl Pts',(7.62029941230854,21.7408548148657,12.));
#248074=CARTESIAN_POINT('Ctrl Pts',(7.62219646084225,21.7553631528329,12.));
#248075=CARTESIAN_POINT('Ctrl Pts',(7.62406838181164,21.7700308755584,12.));
#248076=CARTESIAN_POINT('Ctrl Pts',(7.6259141940452,21.7848563378022,12.));
#248077=CARTESIAN_POINT('Ctrl Pts',(7.62773293842409,21.7998379268583,12.));
#248078=CARTESIAN_POINT('Ctrl Pts',(7.62952367718151,21.8149740615093,12.));
#248079=CARTESIAN_POINT('Ctrl Pts',(7.6312854932304,21.8302631910197,12.));
#248080=CARTESIAN_POINT('Ctrl Pts',(7.63301748948936,21.8457037941084,12.));
#248081=CARTESIAN_POINT('Ctrl Pts',(7.63471878821203,21.8612943779086,12.));
#248082=CARTESIAN_POINT('Ctrl Pts',(7.63638853033367,21.8770334769492,12.));
#248083=CARTESIAN_POINT('Ctrl Pts',(7.63802587492007,21.8929196523511,12.));
#248084=CARTESIAN_POINT('Ctrl Pts',(7.63962999860916,21.9089514909873,12.));
#248085=CARTESIAN_POINT('Ctrl Pts',(7.64120009506539,21.9251276046546,12.));
#248086=CARTESIAN_POINT('Ctrl Pts',(7.64273537442706,21.9414466292074,12.));
#248087=CARTESIAN_POINT('Ctrl Pts',(7.64423506279153,21.9579072237653,12.));
#248088=CARTESIAN_POINT('Ctrl Pts',(7.64569840177359,21.97450807008,12.));
#248089=CARTESIAN_POINT('Ctrl Pts',(7.64712464805257,21.9912478718542,12.));
#248090=CARTESIAN_POINT('Ctrl Pts',(7.64851307293345,22.0081253540774,12.));
#248091=CARTESIAN_POINT('Ctrl Pts',(7.64986296190156,22.025139262321,12.));
#248092=CARTESIAN_POINT('Ctrl Pts',(7.65117361421346,22.0422883621176,12.));
#248093=CARTESIAN_POINT('Ctrl Pts',(7.65244434253103,22.0595714384432,12.));
#248094=CARTESIAN_POINT('Ctrl Pts',(7.65367447254944,22.0769872951596,12.));
#248095=CARTESIAN_POINT('Ctrl Pts',(7.6548633426365,22.094534754469,12.));
#248096=CARTESIAN_POINT('Ctrl Pts',(7.65601030346818,22.1122126563327,12.));
#248097=CARTESIAN_POINT('Ctrl Pts',(7.65711471769406,22.1300198579671,12.));
#248098=CARTESIAN_POINT('Ctrl Pts',(7.6581759596335,22.1479552334206,12.));
#248099=CARTESIAN_POINT('Ctrl Pts',(7.65919341496925,22.1660176731174,12.));
#248100=CARTESIAN_POINT('Ctrl Pts',(7.66016648045007,22.1842060834093,12.));
#248101=CARTESIAN_POINT('Ctrl Pts',(7.66109456359292,22.2025193860972,12.));
#248102=CARTESIAN_POINT('Ctrl Pts',(7.66197708240435,22.2209565180098,12.));
#248103=CARTESIAN_POINT('Ctrl Pts',(7.66281346512545,22.239516430656,12.));
#248104=CARTESIAN_POINT('Ctrl Pts',(7.66360314997661,22.2581980898487,12.));
#248105=CARTESIAN_POINT('Ctrl Pts',(7.66434558490972,22.2770004753332,12.));
#248106=CARTESIAN_POINT('Ctrl Pts',(7.66504022736262,22.2959225803925,12.));
#248107=CARTESIAN_POINT('Ctrl Pts',(7.66568654402441,22.3149634114823,12.));
#248108=CARTESIAN_POINT('Ctrl Pts',(7.66628401061905,22.3341219879454,12.));
#248109=CARTESIAN_POINT('Ctrl Pts',(7.66683211169133,22.3533973417013,12.));
#248110=CARTESIAN_POINT('Ctrl Pts',(7.66733034039887,22.3727885169361,12.));
#248111=CARTESIAN_POINT('Ctrl Pts',(7.66777819830819,22.3922945697782,12.));
#248112=CARTESIAN_POINT('Ctrl Pts',(7.66817519519681,22.411914567977,12.));
#248113=CARTESIAN_POINT('Ctrl Pts',(7.66852084886745,22.4316475906616,12.));
#248114=CARTESIAN_POINT('Ctrl Pts',(7.66881468496659,22.4514927280863,12.));
#248115=CARTESIAN_POINT('Ctrl Pts',(7.66905623680835,22.47144908137,12.));
#248116=CARTESIAN_POINT('Ctrl Pts',(7.66924504520301,22.4915157622308,12.));
#248117=CARTESIAN_POINT('Ctrl Pts',(7.66938065829082,22.5116918927023,12.));
#248118=CARTESIAN_POINT('Ctrl Pts',(7.66946263138115,22.5319766049191,12.));
#248119=CARTESIAN_POINT('Ctrl Pts',(7.66949052679671,22.5523690409109,12.));
#248120=CARTESIAN_POINT('Ctrl Pts',(7.66946391372299,22.5728683523829,12.));
#248121=CARTESIAN_POINT('Ctrl Pts',(7.6693823680624,22.5934737004955,12.));
#248122=CARTESIAN_POINT('Ctrl Pts',(7.66924547229434,22.6141842556248,12.));
#248123=CARTESIAN_POINT('Ctrl Pts',(7.66905281533744,22.6349991971548,12.));
#248124=CARTESIAN_POINT('Ctrl Pts',(7.66880399241353,22.6559177133133,12.));
#248125=CARTESIAN_POINT('Ctrl Pts',(7.66849860491762,22.6769390009889,12.));
#248126=CARTESIAN_POINT('Ctrl Pts',(7.66813626029276,22.6980622655446,12.));
#248127=CARTESIAN_POINT('Ctrl Pts',(7.6677165719101,22.7192867206242,12.));
#248128=CARTESIAN_POINT('Ctrl Pts',(7.66723915895412,22.7406115879508,12.));
#248129=CARTESIAN_POINT('Ctrl Pts',(7.66670364630273,22.7620360971839,12.));
#248130=CARTESIAN_POINT('Ctrl Pts',(7.66610966441259,22.7835594857697,12.));
#248131=CARTESIAN_POINT('Ctrl Pts',(7.66545684920987,22.8051809987834,12.));
#248132=CARTESIAN_POINT('Ctrl Pts',(7.66474484198552,22.8268998887679,12.));
#248133=CARTESIAN_POINT('Ctrl Pts',(7.66397328929805,22.8487154155569,12.));
#248134=CARTESIAN_POINT('Ctrl Pts',(7.66314184287333,22.870626846128,12.));
#248135=CARTESIAN_POINT('Ctrl Pts',(7.66225015950147,22.8926334544879,12.));
#248136=CARTESIAN_POINT('Ctrl Pts',(7.66129790094099,22.9147345215418,12.));
#248137=CARTESIAN_POINT('Ctrl Pts',(7.66028473382776,22.9369293349592,12.));
#248138=CARTESIAN_POINT('Ctrl Pts',(7.65921032958911,22.9592171890332,12.));
#248139=CARTESIAN_POINT('Ctrl Pts',(7.65807436436452,22.9815973845301,12.));
#248140=CARTESIAN_POINT('Ctrl Pts',(7.6568765189133,23.004069228582,12.));
#248141=CARTESIAN_POINT('Ctrl Pts',(7.65561647852554,23.0266320345792,12.));
#248142=CARTESIAN_POINT('Ctrl Pts',(7.65429393293955,23.049285122053,12.));
#248143=CARTESIAN_POINT('Ctrl Pts',(7.65290857626356,23.072027816555,12.));
#248144=CARTESIAN_POINT('Ctrl Pts',(7.65146010690464,23.0948594495246,12.));
#248145=CARTESIAN_POINT('Ctrl Pts',(7.64994822749844,23.1177793581674,12.));
#248146=CARTESIAN_POINT('Ctrl Pts',(7.64837264482929,23.1407868853815,12.));
#248147=CARTESIAN_POINT('Ctrl Pts',(7.64673306975796,23.1638813796691,12.));
#248148=CARTESIAN_POINT('Ctrl Pts',(7.64502921715482,23.1870621950452,12.));
#248149=CARTESIAN_POINT('Ctrl Pts',(7.64326080583683,23.2103286909399,12.));
#248150=CARTESIAN_POINT('Ctrl Pts',(7.64142755851507,23.2336802320912,12.));
#248151=CARTESIAN_POINT('Ctrl Pts',(7.63952920172837,23.2571161884487,12.));
#248152=CARTESIAN_POINT('Ctrl Pts',(7.63756546576374,23.2806359350853,12.));
#248153=CARTESIAN_POINT('Ctrl Pts',(7.63553608458783,23.3042388521021,12.));
#248154=CARTESIAN_POINT('Ctrl Pts',(7.63344079578162,23.3279243245241,12.));
#248155=CARTESIAN_POINT('Ctrl Pts',(7.63127934048138,23.3516917421973,12.));
#248156=CARTESIAN_POINT('Ctrl Pts',(7.62905146332597,23.3755404996638,12.));
#248157=CARTESIAN_POINT('Ctrl Pts',(7.62675691240334,23.3994699961122,12.));
#248158=CARTESIAN_POINT('Ctrl Pts',(7.62439543920053,23.4234796353544,12.));
#248159=CARTESIAN_POINT('Ctrl Pts',(7.62196679855957,23.4475688257855,12.));
#248160=CARTESIAN_POINT('Ctrl Pts',(7.61947074863977,23.4717369803438,12.));
#248161=CARTESIAN_POINT('Ctrl Pts',(7.61690705088318,23.4959835164608,12.));
#248162=CARTESIAN_POINT('Ctrl Pts',(7.61427546999298,23.5203078560128,12.));
#248163=CARTESIAN_POINT('Ctrl Pts',(7.61157577385371,23.5447094252029,12.));
#248164=CARTESIAN_POINT('Ctrl Pts',(7.60880773344599,23.5691876544243,12.));
#248165=CARTESIAN_POINT('Ctrl Pts',(7.60597112277094,23.5937419781244,12.));
#248166=CARTESIAN_POINT('Ctrl Pts',(7.60306571877806,23.6183718346576,12.));
#248167=CARTESIAN_POINT('Ctrl Pts',(7.60009130130129,23.6430766661419,12.));
#248168=CARTESIAN_POINT('Ctrl Pts',(7.59704765299572,23.6678559182876,12.));
#248169=CARTESIAN_POINT('Ctrl Pts',(7.59393455934041,23.6927090405067,12.));
#248170=CARTESIAN_POINT('Ctrl Pts',(7.59075180865326,23.7176354860457,12.));
#248171=CARTESIAN_POINT('Ctrl Pts',(7.58749919210831,23.7426347121006,12.));
#248172=CARTESIAN_POINT('Ctrl Pts',(7.58417650376271,23.7677061799376,12.));
#248173=CARTESIAN_POINT('Ctrl Pts',(7.58078354058211,23.7928493549908,12.));
#248174=CARTESIAN_POINT('Ctrl Pts',(7.57732010249065,23.8180637069977,12.));
#248175=CARTESIAN_POINT('Ctrl Pts',(7.57378599219816,23.8433487096134,12.));
#248176=CARTESIAN_POINT('Ctrl Pts',(7.5701810150071,23.8687038399598,12.));
#248177=CARTESIAN_POINT('Ctrl Pts',(7.56650497863791,23.8941285782003,12.));
#248178=CARTESIAN_POINT('Ctrl Pts',(7.56275769304773,23.9196224070759,12.));
#248179=CARTESIAN_POINT('Ctrl Pts',(7.55893897027682,23.9451848115,12.));
#248180=CARTESIAN_POINT('Ctrl Pts',(7.55504862424811,23.9708152779884,12.));
#248181=CARTESIAN_POINT('Ctrl Pts',(7.5510864709744,23.9965132953185,12.));
#248182=CARTESIAN_POINT('Ctrl Pts',(7.5470523288591,24.022278355453,12.));
#248183=CARTESIAN_POINT('Ctrl Pts',(7.54294601896144,24.0481099543353,12.));
#248184=CARTESIAN_POINT('Ctrl Pts',(7.53876736531013,24.0740075927985,12.));
#248185=CARTESIAN_POINT('Ctrl Pts',(7.53451619514649,24.0999707772642,12.));
#248186=CARTESIAN_POINT('Ctrl Pts',(7.53019233935501,24.1259990209207,12.));
#248187=CARTESIAN_POINT('Ctrl Pts',(7.52579563201423,24.1520918425364,12.));
#248188=CARTESIAN_POINT('Ctrl Pts',(7.52132590953801,24.1782487641594,12.));
#248189=CARTESIAN_POINT('Ctrl Pts',(7.51678300997949,24.2044693092349,12.));
#248190=CARTESIAN_POINT('Ctrl Pts',(7.5121667722218,24.2307530003887,12.));
#248191=CARTESIAN_POINT('Ctrl Pts',(7.50747703535133,24.2570993577034,12.));
#248192=CARTESIAN_POINT('Ctrl Pts',(7.50271363765151,24.2835078958973,12.));
#248193=CARTESIAN_POINT('Ctrl Pts',(7.49787641695438,24.3099781253355,12.));
#248194=CARTESIAN_POINT('Ctrl Pts',(7.4929652125242,24.3365095573685,12.));
#248195=CARTESIAN_POINT('Ctrl Pts',(7.48797986651908,24.3631017084524,12.));
#248196=CARTESIAN_POINT('Ctrl Pts',(7.482920225693,24.3897541049254,12.));
#248197=CARTESIAN_POINT('Ctrl Pts',(7.47778614286564,24.4164662871163,12.));
#248198=CARTESIAN_POINT('Ctrl Pts',(7.47257747883246,24.443237814649,12.));
#248199=CARTESIAN_POINT('Ctrl Pts',(7.46729410308786,24.4700682684524,12.));
#248200=CARTESIAN_POINT('Ctrl Pts',(7.46193588961463,24.4969572391483,12.));
#248201=CARTESIAN_POINT('Ctrl Pts',(7.45650271335861,24.5239043173072,12.));
#248202=CARTESIAN_POINT('Ctrl Pts',(7.4509944465116,24.5509090831559,12.));
#248203=CARTESIAN_POINT('Ctrl Pts',(7.44541095473134,24.577971096086,12.));
#248204=CARTESIAN_POINT('Ctrl Pts',(7.43975209375503,24.6050898852368,12.));
#248205=CARTESIAN_POINT('Ctrl Pts',(7.43401770489523,24.6322649369517,12.));
#248206=CARTESIAN_POINT('Ctrl Pts',(7.42820762159125,24.6594957128756,12.));
#248207=CARTESIAN_POINT('Ctrl Pts',(7.42232167766265,24.6867816727192,12.));
#248208=CARTESIAN_POINT('Ctrl Pts',(7.41635971481674,24.7141222950051,12.));
#248209=CARTESIAN_POINT('Ctrl Pts',(7.41032159082381,24.7415170994784,12.));
#248210=CARTESIAN_POINT('Ctrl Pts',(7.40420718661602,24.7689656668983,12.));
#248211=CARTESIAN_POINT('Ctrl Pts',(7.39801641583012,24.7964676646431,12.));
#248212=CARTESIAN_POINT('Ctrl Pts',(7.39174922585808,24.8240228520893,12.));
#248213=CARTESIAN_POINT('Ctrl Pts',(7.3854055890362,24.8516310625176,12.));
#248214=CARTESIAN_POINT('Ctrl Pts',(7.37898549640269,24.8792921911115,12.));
#248215=CARTESIAN_POINT('Ctrl Pts',(7.37378825961676,24.901463382605,12.));
#248216=CARTESIAN_POINT('Ctrl Pts',(7.3698559312009,24.9181155530543,12.));
#248217=CARTESIAN_POINT('Ctrl Pts',(7.36721909028842,24.9292275670674,12.));
#248218=CARTESIAN_POINT('Ctrl Pts',(7.36589684767344,24.9347862158358,12.));
#248219=CARTESIAN_POINT('Ctrl Pts',(9.71462809124917,20.353053841303,0.));
#248220=CARTESIAN_POINT('Ctrl Pts',(9.71462809124917,20.353053841303,12.));
#248221=CARTESIAN_POINT('Ctrl Pts',(9.71462954053074,20.353060251684,0.));
#248222=CARTESIAN_POINT('Ctrl Pts',(9.71462954053074,20.353060251684,12.));
#248223=CARTESIAN_POINT('Ctrl Pts',(9.71465227853122,20.3531126095522,0.));
#248224=CARTESIAN_POINT('Ctrl Pts',(9.71465227853122,20.3531126095522,12.));
#248225=CARTESIAN_POINT('Ctrl Pts',(9.71474590350791,20.3533097561886,0.));
#248226=CARTESIAN_POINT('Ctrl Pts',(9.71474590350791,20.3533097561886,12.));
#248227=CARTESIAN_POINT('Ctrl Pts',(9.714989780521,20.3538098605706,0.));
#248228=CARTESIAN_POINT('Ctrl Pts',(9.714989780521,20.3538098605706,12.));
#248229=CARTESIAN_POINT('Ctrl Pts',(9.71549257088174,20.3548282742361,0.));
#248230=CARTESIAN_POINT('Ctrl Pts',(9.71549257088174,20.3548282742361,12.));
#248231=CARTESIAN_POINT('Ctrl Pts',(9.71619192554146,20.3562337557875,0.));
#248232=CARTESIAN_POINT('Ctrl Pts',(9.71619192554146,20.3562337557875,12.));
#248233=CARTESIAN_POINT('Ctrl Pts',(9.71708493723061,20.3580133103357,0.));
#248234=CARTESIAN_POINT('Ctrl Pts',(9.71708493723061,20.3580133103357,12.));
#248235=CARTESIAN_POINT('Ctrl Pts',(9.71816778327998,20.3601498764344,0.));
#248236=CARTESIAN_POINT('Ctrl Pts',(9.71816778327998,20.3601498764344,12.));
#248237=CARTESIAN_POINT('Ctrl Pts',(9.71943648548114,20.362625691398,0.));
#248238=CARTESIAN_POINT('Ctrl Pts',(9.71943648548114,20.362625691398,12.));
#248239=CARTESIAN_POINT('Ctrl Pts',(9.72088778381101,20.3654261611055,0.));
#248240=CARTESIAN_POINT('Ctrl Pts',(9.72088778381101,20.3654261611055,12.));
#248241=CARTESIAN_POINT('Ctrl Pts',(9.72251930722503,20.3685406190576,0.));
#248242=CARTESIAN_POINT('Ctrl Pts',(9.72251930722503,20.3685406190576,12.));
#248243=CARTESIAN_POINT('Ctrl Pts',(9.72432910043192,20.371960235676,0.));
#248244=CARTESIAN_POINT('Ctrl Pts',(9.72432910043192,20.371960235676,12.));
#248245=CARTESIAN_POINT('Ctrl Pts',(9.7263153173287,20.3756766651952,0.));
#248246=CARTESIAN_POINT('Ctrl Pts',(9.7263153173287,20.3756766651952,12.));
#248247=CARTESIAN_POINT('Ctrl Pts',(9.72847589116532,20.3796805893304,0.));
#248248=CARTESIAN_POINT('Ctrl Pts',(9.72847589116532,20.3796805893304,12.));
#248249=CARTESIAN_POINT('Ctrl Pts',(9.73080870123726,20.3839624556742,0.));
#248250=CARTESIAN_POINT('Ctrl Pts',(9.73080870123726,20.3839624556742,12.));
#248251=CARTESIAN_POINT('Ctrl Pts',(9.73331167102812,20.3885129129912,0.));
#248252=CARTESIAN_POINT('Ctrl Pts',(9.73331167102812,20.3885129129912,12.));
#248253=CARTESIAN_POINT('Ctrl Pts',(9.73598292014249,20.3933234845646,0.));
#248254=CARTESIAN_POINT('Ctrl Pts',(9.73598292014249,20.3933234845646,12.));
#248255=CARTESIAN_POINT('Ctrl Pts',(9.73882077613206,20.3983866213331,0.));
#248256=CARTESIAN_POINT('Ctrl Pts',(9.73882077613206,20.3983866213331,12.));
#248257=CARTESIAN_POINT('Ctrl Pts',(9.74182369656272,20.4036953576549,0.));
#248258=CARTESIAN_POINT('Ctrl Pts',(9.74182369656272,20.4036953576549,12.));
#248259=CARTESIAN_POINT('Ctrl Pts',(9.74499021838536,20.4092430879861,0.));
#248260=CARTESIAN_POINT('Ctrl Pts',(9.74499021838536,20.4092430879861,12.));
#248261=CARTESIAN_POINT('Ctrl Pts',(9.74831889242174,20.4150232777393,0.));
#248262=CARTESIAN_POINT('Ctrl Pts',(9.74831889242174,20.4150232777393,12.));
#248263=CARTESIAN_POINT('Ctrl Pts',(9.75180829786433,20.4210295275818,0.));
#248264=CARTESIAN_POINT('Ctrl Pts',(9.75180829786433,20.4210295275818,12.));
#248265=CARTESIAN_POINT('Ctrl Pts',(9.75545705902416,20.4272556476629,0.));
#248266=CARTESIAN_POINT('Ctrl Pts',(9.75545705902416,20.4272556476629,12.));
#248267=CARTESIAN_POINT('Ctrl Pts',(9.75926386289929,20.4336957355474,0.));
#248268=CARTESIAN_POINT('Ctrl Pts',(9.75926386289929,20.4336957355474,12.));
#248269=CARTESIAN_POINT('Ctrl Pts',(9.76322747195502,20.4403442329401,0.));
#248270=CARTESIAN_POINT('Ctrl Pts',(9.76322747195502,20.4403442329401,12.));
#248271=CARTESIAN_POINT('Ctrl Pts',(9.76734670980896,20.447195862298,0.));
#248272=CARTESIAN_POINT('Ctrl Pts',(9.76734670980896,20.447195862298,12.));
#248273=CARTESIAN_POINT('Ctrl Pts',(9.77162045104069,20.4542455817527,0.));
#248274=CARTESIAN_POINT('Ctrl Pts',(9.77162045104069,20.4542455817527,12.));
#248275=CARTESIAN_POINT('Ctrl Pts',(9.77604760815522,20.4614885274973,0.));
#248276=CARTESIAN_POINT('Ctrl Pts',(9.77604760815522,20.4614885274973,12.));
#248277=CARTESIAN_POINT('Ctrl Pts',(9.78062712373313,20.4689199790668,0.));
#248278=CARTESIAN_POINT('Ctrl Pts',(9.78062712373313,20.4689199790668,12.));
#248279=CARTESIAN_POINT('Ctrl Pts',(9.78535797314162,20.4765353711585,0.));
#248280=CARTESIAN_POINT('Ctrl Pts',(9.78535797314162,20.4765353711585,12.));
#248281=CARTESIAN_POINT('Ctrl Pts',(9.79023916498659,20.4843302955329,0.));
#248282=CARTESIAN_POINT('Ctrl Pts',(9.79023916498659,20.4843302955329,12.));
#248283=CARTESIAN_POINT('Ctrl Pts',(9.79526974288343,20.4923005087945,0.));
#248284=CARTESIAN_POINT('Ctrl Pts',(9.79526974288343,20.4923005087945,12.));
#248285=CARTESIAN_POINT('Ctrl Pts',(9.80044878520967,20.500441931211,0.));
#248286=CARTESIAN_POINT('Ctrl Pts',(9.80044878520967,20.500441931211,12.));
#248287=CARTESIAN_POINT('Ctrl Pts',(9.80577540161102,20.5087506310507,0.));
#248288=CARTESIAN_POINT('Ctrl Pts',(9.80577540161102,20.5087506310507,12.));
#248289=CARTESIAN_POINT('Ctrl Pts',(9.81124873025278,20.5172228122839,0.));
#248290=CARTESIAN_POINT('Ctrl Pts',(9.81124873025278,20.5172228122839,12.));
#248291=CARTESIAN_POINT('Ctrl Pts',(9.81686793455918,20.5258548000625,0.));
#248292=CARTESIAN_POINT('Ctrl Pts',(9.81686793455918,20.5258548000625,12.));
#248293=CARTESIAN_POINT('Ctrl Pts',(9.82263220080327,20.534643029951,0.));
#248294=CARTESIAN_POINT('Ctrl Pts',(9.82263220080327,20.534643029951,12.));
#248295=CARTESIAN_POINT('Ctrl Pts',(9.82854073773857,20.5435840460717,0.));
#248296=CARTESIAN_POINT('Ctrl Pts',(9.82854073773857,20.5435840460717,12.));
#248297=CARTESIAN_POINT('Ctrl Pts',(9.8345927758532,20.5526744976461,0.));
#248298=CARTESIAN_POINT('Ctrl Pts',(9.8345927758532,20.5526744976461,12.));
#248299=CARTESIAN_POINT('Ctrl Pts',(9.84078756677589,20.5619111362406,0.));
#248300=CARTESIAN_POINT('Ctrl Pts',(9.84078756677589,20.5619111362406,12.));
#248301=CARTESIAN_POINT('Ctrl Pts',(9.84712438256308,20.5712908125145,0.));
#248302=CARTESIAN_POINT('Ctrl Pts',(9.84712438256308,20.5712908125145,12.));
#248303=CARTESIAN_POINT('Ctrl Pts',(9.85360251457004,20.580810471002,0.));
#248304=CARTESIAN_POINT('Ctrl Pts',(9.85360251457004,20.580810471002,12.));
#248305=CARTESIAN_POINT('Ctrl Pts',(9.86022127232749,20.5904671449755,0.));
#248306=CARTESIAN_POINT('Ctrl Pts',(9.86022127232749,20.5904671449755,12.));
#248307=CARTESIAN_POINT('Ctrl Pts',(9.86697998242612,20.6002579513696,0.));
#248308=CARTESIAN_POINT('Ctrl Pts',(9.86697998242612,20.6002579513696,12.));
#248309=CARTESIAN_POINT('Ctrl Pts',(9.87387798732943,20.6101800854491,0.));
#248310=CARTESIAN_POINT('Ctrl Pts',(9.87387798732943,20.6101800854491,12.));
#248311=CARTESIAN_POINT('Ctrl Pts',(9.88091464472669,20.6202308177472,0.));
#248312=CARTESIAN_POINT('Ctrl Pts',(9.88091464472669,20.6202308177472,12.));
#248313=CARTESIAN_POINT('Ctrl Pts',(9.88808932697304,20.6304074914086,0.));
#248314=CARTESIAN_POINT('Ctrl Pts',(9.88808932697304,20.6304074914086,12.));
#248315=CARTESIAN_POINT('Ctrl Pts',(9.89540142049123,20.6407075193977,0.));
#248316=CARTESIAN_POINT('Ctrl Pts',(9.89540142049123,20.6407075193977,12.));
#248317=CARTESIAN_POINT('Ctrl Pts',(9.90285032516695,20.6511283817415,0.));
#248318=CARTESIAN_POINT('Ctrl Pts',(9.90285032516695,20.6511283817415,12.));
#248319=CARTESIAN_POINT('Ctrl Pts',(9.91043545377004,20.6616676228315,0.));
#248320=CARTESIAN_POINT('Ctrl Pts',(9.91043545377004,20.6616676228315,12.));
#248321=CARTESIAN_POINT('Ctrl Pts',(9.91815623141284,20.6723228488262,0.));
#248322=CARTESIAN_POINT('Ctrl Pts',(9.91815623141284,20.6723228488262,12.));
#248323=CARTESIAN_POINT('Ctrl Pts',(9.9260120949875,20.6830917250255,0.));
#248324=CARTESIAN_POINT('Ctrl Pts',(9.9260120949875,20.6830917250255,12.));
#248325=CARTESIAN_POINT('Ctrl Pts',(9.93400249259736,20.6939719732485,0.));
#248326=CARTESIAN_POINT('Ctrl Pts',(9.93400249259736,20.6939719732485,12.));
#248327=CARTESIAN_POINT('Ctrl Pts',(9.9421268829825,20.7049613692237,0.));
#248328=CARTESIAN_POINT('Ctrl Pts',(9.9421268829825,20.7049613692237,12.));
#248329=CARTESIAN_POINT('Ctrl Pts',(9.95038473514962,20.7160577407581,0.));
#248330=CARTESIAN_POINT('Ctrl Pts',(9.95038473514962,20.7160577407581,12.));
#248331=CARTESIAN_POINT('Ctrl Pts',(9.95877552798403,20.7272589658752,0.));
#248332=CARTESIAN_POINT('Ctrl Pts',(9.95877552798403,20.7272589658752,12.));
#248333=CARTESIAN_POINT('Ctrl Pts',(9.96729874986198,20.7385629709795,0.));
#248334=CARTESIAN_POINT('Ctrl Pts',(9.96729874986198,20.7385629709795,12.));
#248335=CARTESIAN_POINT('Ctrl Pts',(9.97595389823461,20.7499677289626,0.));
#248336=CARTESIAN_POINT('Ctrl Pts',(9.97595389823461,20.7499677289626,12.));
#248337=CARTESIAN_POINT('Ctrl Pts',(9.98474047926846,20.7614712574989,0.));
#248338=CARTESIAN_POINT('Ctrl Pts',(9.98474047926846,20.7614712574989,12.));
#248339=CARTESIAN_POINT('Ctrl Pts',(9.99365800754637,20.7730716175417,0.));
#248340=CARTESIAN_POINT('Ctrl Pts',(9.99365800754637,20.7730716175417,12.));
#248341=CARTESIAN_POINT('Ctrl Pts',(10.0027060057389,20.7847669117568,0.));
#248342=CARTESIAN_POINT('Ctrl Pts',(10.0027060057389,20.7847669117568,12.));
#248343=CARTESIAN_POINT('Ctrl Pts',(10.0118840042786,20.7965552829907,0.));
#248344=CARTESIAN_POINT('Ctrl Pts',(10.0118840042786,20.7965552829907,12.));
#248345=CARTESIAN_POINT('Ctrl Pts',(10.0211915410095,20.8084349126885,0.));
#248346=CARTESIAN_POINT('Ctrl Pts',(10.0211915410095,20.8084349126885,12.));
#248347=CARTESIAN_POINT('Ctrl Pts',(10.0306281609435,20.8204040196599,0.));
#248348=CARTESIAN_POINT('Ctrl Pts',(10.0306281609435,20.8204040196599,12.));
#248349=CARTESIAN_POINT('Ctrl Pts',(10.0401934160234,20.8324608588906,0.));
#248350=CARTESIAN_POINT('Ctrl Pts',(10.0401934160234,20.8324608588906,12.));
#248351=CARTESIAN_POINT('Ctrl Pts',(10.0498868648733,20.8446037203402,0.));
#248352=CARTESIAN_POINT('Ctrl Pts',(10.0498868648733,20.8446037203402,12.));
#248353=CARTESIAN_POINT('Ctrl Pts',(10.0597080725375,20.856830927732,0.));
#248354=CARTESIAN_POINT('Ctrl Pts',(10.0597080725375,20.856830927732,12.));
#248355=CARTESIAN_POINT('Ctrl Pts',(10.0696566102219,20.8691408373705,0.));
#248356=CARTESIAN_POINT('Ctrl Pts',(10.0696566102219,20.8691408373705,12.));
#248357=CARTESIAN_POINT('Ctrl Pts',(10.0797320551154,20.8815318371844,0.));
#248358=CARTESIAN_POINT('Ctrl Pts',(10.0797320551154,20.8815318371844,12.));
#248359=CARTESIAN_POINT('Ctrl Pts',(10.0899339901916,20.8940023457371,0.));
#248360=CARTESIAN_POINT('Ctrl Pts',(10.0899339901916,20.8940023457371,12.));
#248361=CARTESIAN_POINT('Ctrl Pts',(10.1002620040076,20.9065508112556,0.));
#248362=CARTESIAN_POINT('Ctrl Pts',(10.1002620040076,20.9065508112556,12.));
#248363=CARTESIAN_POINT('Ctrl Pts',(10.1107156904836,20.9191757106266,0.));
#248364=CARTESIAN_POINT('Ctrl Pts',(10.1107156904836,20.9191757106266,12.));
#248365=CARTESIAN_POINT('Ctrl Pts',(10.1212946487057,20.931875548473,0.));
#248366=CARTESIAN_POINT('Ctrl Pts',(10.1212946487057,20.931875548473,12.));
#248367=CARTESIAN_POINT('Ctrl Pts',(10.1319984827909,20.944648856393,0.));
#248368=CARTESIAN_POINT('Ctrl Pts',(10.1319984827909,20.944648856393,12.));
#248369=CARTESIAN_POINT('Ctrl Pts',(10.1428268017257,20.9574941921591,0.));
#248370=CARTESIAN_POINT('Ctrl Pts',(10.1428268017257,20.9574941921591,12.));
#248371=CARTESIAN_POINT('Ctrl Pts',(10.1537792192065,20.970410138937,0.));
#248372=CARTESIAN_POINT('Ctrl Pts',(10.1537792192065,20.970410138937,12.));
#248373=CARTESIAN_POINT('Ctrl Pts',(10.1648553534567,20.9833953044737,0.));
#248374=CARTESIAN_POINT('Ctrl Pts',(10.1648553534567,20.9833953044737,12.));
#248375=CARTESIAN_POINT('Ctrl Pts',(10.1760548270765,20.9964483203685,0.));
#248376=CARTESIAN_POINT('Ctrl Pts',(10.1760548270765,20.9964483203685,12.));
#248377=CARTESIAN_POINT('Ctrl Pts',(10.1873772669358,21.0095678414486,0.));
#248378=CARTESIAN_POINT('Ctrl Pts',(10.1873772669358,21.0095678414486,12.));
#248379=CARTESIAN_POINT('Ctrl Pts',(10.1988223040425,21.0227525451107,0.));
#248380=CARTESIAN_POINT('Ctrl Pts',(10.1988223040425,21.0227525451107,12.));
#248381=CARTESIAN_POINT('Ctrl Pts',(10.2103895734123,21.0360011306814,0.));
#248382=CARTESIAN_POINT('Ctrl Pts',(10.2103895734123,21.0360011306814,12.));
#248383=CARTESIAN_POINT('Ctrl Pts',(10.2220787139157,21.0493123187484,0.));
#248384=CARTESIAN_POINT('Ctrl Pts',(10.2220787139157,21.0493123187484,12.));
#248385=CARTESIAN_POINT('Ctrl Pts',(10.233889368157,21.0626848505665,0.));
#248386=CARTESIAN_POINT('Ctrl Pts',(10.233889368157,21.0626848505665,12.));
#248387=CARTESIAN_POINT('Ctrl Pts',(10.2458211823915,21.0761174875448,0.));
#248388=CARTESIAN_POINT('Ctrl Pts',(10.2458211823915,21.0761174875448,12.));
#248389=CARTESIAN_POINT('Ctrl Pts',(10.2578738064183,21.0896090107066,0.));
#248390=CARTESIAN_POINT('Ctrl Pts',(10.2578738064183,21.0896090107066,12.));
#248391=CARTESIAN_POINT('Ctrl Pts',(10.2700468934743,21.1031582201625,0.));
#248392=CARTESIAN_POINT('Ctrl Pts',(10.2700468934743,21.1031582201625,12.));
#248393=CARTESIAN_POINT('Ctrl Pts',(10.2823401001067,21.1167639345623,0.));
#248394=CARTESIAN_POINT('Ctrl Pts',(10.2823401001067,21.1167639345623,12.));
#248395=CARTESIAN_POINT('Ctrl Pts',(10.2947530860714,21.130424990599,0.));
#248396=CARTESIAN_POINT('Ctrl Pts',(10.2947530860714,21.130424990599,12.));
#248397=CARTESIAN_POINT('Ctrl Pts',(10.307285514268,21.1441402425831,0.));
#248398=CARTESIAN_POINT('Ctrl Pts',(10.307285514268,21.1441402425831,12.));
#248399=CARTESIAN_POINT('Ctrl Pts',(10.3199370506541,21.1579085619959,0.));
#248400=CARTESIAN_POINT('Ctrl Pts',(10.3199370506541,21.1579085619959,12.));
#248401=CARTESIAN_POINT('Ctrl Pts',(10.3327073641574,21.1717288370512,0.));
#248402=CARTESIAN_POINT('Ctrl Pts',(10.3327073641574,21.1717288370512,12.));
#248403=CARTESIAN_POINT('Ctrl Pts',(10.3455961265706,21.1855999722427,0.));
#248404=CARTESIAN_POINT('Ctrl Pts',(10.3455961265706,21.1855999722427,12.));
#248405=CARTESIAN_POINT('Ctrl Pts',(10.3586030124595,21.1995208879205,0.));
#248406=CARTESIAN_POINT('Ctrl Pts',(10.3586030124595,21.1995208879205,12.));
#248407=CARTESIAN_POINT('Ctrl Pts',(10.3717276991137,21.2134905199359,0.));
#248408=CARTESIAN_POINT('Ctrl Pts',(10.3717276991137,21.2134905199359,12.));
#248409=CARTESIAN_POINT('Ctrl Pts',(10.384969866479,21.2275078192708,0.));
#248410=CARTESIAN_POINT('Ctrl Pts',(10.384969866479,21.2275078192708,12.));
#248411=CARTESIAN_POINT('Ctrl Pts',(10.3983291970846,21.2415717516713,0.));
#248412=CARTESIAN_POINT('Ctrl Pts',(10.3983291970846,21.2415717516713,12.));
#248413=CARTESIAN_POINT('Ctrl Pts',(10.4118053759584,21.2556812972741,0.));
#248414=CARTESIAN_POINT('Ctrl Pts',(10.4118053759584,21.2556812972741,12.));
#248415=CARTESIAN_POINT('Ctrl Pts',(10.4253980905394,21.2698354502391,0.));
#248416=CARTESIAN_POINT('Ctrl Pts',(10.4253980905394,21.2698354502391,12.));
#248417=CARTESIAN_POINT('Ctrl Pts',(10.4391070306385,21.2840332184471,0.));
#248418=CARTESIAN_POINT('Ctrl Pts',(10.4391070306385,21.2840332184471,12.));
#248419=CARTESIAN_POINT('Ctrl Pts',(10.452931888387,21.2982736231924,0.));
#248420=CARTESIAN_POINT('Ctrl Pts',(10.452931888387,21.2982736231924,12.));
#248421=CARTESIAN_POINT('Ctrl Pts',(10.4668723581768,21.312555698873,0.));
#248422=CARTESIAN_POINT('Ctrl Pts',(10.4668723581768,21.312555698873,12.));
#248423=CARTESIAN_POINT('Ctrl Pts',(10.4809281365933,21.3268784926823,0.));
#248424=CARTESIAN_POINT('Ctrl Pts',(10.4809281365933,21.3268784926823,12.));
#248425=CARTESIAN_POINT('Ctrl Pts',(10.4950989223341,21.3412410642912,0.));
#248426=CARTESIAN_POINT('Ctrl Pts',(10.4950989223341,21.3412410642912,12.));
#248427=CARTESIAN_POINT('Ctrl Pts',(10.5093844161689,21.3556424855822,0.));
#248428=CARTESIAN_POINT('Ctrl Pts',(10.5093844161689,21.3556424855822,12.));
#248429=CARTESIAN_POINT('Ctrl Pts',(10.523784320906,21.3700818403942,0.));
#248430=CARTESIAN_POINT('Ctrl Pts',(10.523784320906,21.3700818403942,12.));
#248431=CARTESIAN_POINT('Ctrl Pts',(10.5382983413422,21.3845582242604,0.));
#248432=CARTESIAN_POINT('Ctrl Pts',(10.5382983413422,21.3845582242604,12.));
#248433=CARTESIAN_POINT('Ctrl Pts',(10.5529261842107,21.3990707441495,0.));
#248434=CARTESIAN_POINT('Ctrl Pts',(10.5529261842107,21.3990707441495,12.));
#248435=CARTESIAN_POINT('Ctrl Pts',(10.5676675581106,21.4136185181974,0.));
#248436=CARTESIAN_POINT('Ctrl Pts',(10.5676675581106,21.4136185181974,12.));
#248437=CARTESIAN_POINT('Ctrl Pts',(10.582522173457,21.4282006754624,0.));
#248438=CARTESIAN_POINT('Ctrl Pts',(10.582522173457,21.4282006754624,12.));
#248439=CARTESIAN_POINT('Ctrl Pts',(10.597489742462,21.4428163557137,0.));
#248440=CARTESIAN_POINT('Ctrl Pts',(10.597489742462,21.4428163557137,12.));
#248441=CARTESIAN_POINT('Ctrl Pts',(10.612569979096,21.4574647092093,0.));
#248442=CARTESIAN_POINT('Ctrl Pts',(10.612569979096,21.4574647092093,12.));
#248443=CARTESIAN_POINT('Ctrl Pts',(10.6277625990456,21.4721448964766,0.));
#248444=CARTESIAN_POINT('Ctrl Pts',(10.6277625990456,21.4721448964766,12.));
#248445=CARTESIAN_POINT('Ctrl Pts',(10.6430673196609,21.4868560880893,0.));
#248446=CARTESIAN_POINT('Ctrl Pts',(10.6430673196609,21.4868560880893,12.));
#248447=CARTESIAN_POINT('Ctrl Pts',(10.658483859894,21.5015974644454,0.));
#248448=CARTESIAN_POINT('Ctrl Pts',(10.658483859894,21.5015974644454,12.));
#248449=CARTESIAN_POINT('Ctrl Pts',(10.6740119402835,21.5163682155805,0.));
#248450=CARTESIAN_POINT('Ctrl Pts',(10.6740119402835,21.5163682155805,12.));
#248451=CARTESIAN_POINT('Ctrl Pts',(10.689651282929,21.531167540981,0.));
#248452=CARTESIAN_POINT('Ctrl Pts',(10.689651282929,21.531167540981,12.));
#248453=CARTESIAN_POINT('Ctrl Pts',(10.7054016114571,21.5459946493955,0.));
#248454=CARTESIAN_POINT('Ctrl Pts',(10.7054016114571,21.5459946493955,12.));
#248455=CARTESIAN_POINT('Ctrl Pts',(10.7212626509816,21.5608487586467,0.));
#248456=CARTESIAN_POINT('Ctrl Pts',(10.7212626509816,21.5608487586467,12.));
#248457=CARTESIAN_POINT('Ctrl Pts',(10.7372341280468,21.5757290954372,0.));
#248458=CARTESIAN_POINT('Ctrl Pts',(10.7372341280468,21.5757290954372,12.));
#248459=CARTESIAN_POINT('Ctrl Pts',(10.7533157705943,21.5906348951745,0.));
#248460=CARTESIAN_POINT('Ctrl Pts',(10.7533157705943,21.5906348951745,12.));
#248461=CARTESIAN_POINT('Ctrl Pts',(10.7695073079554,21.6055654018179,0.));
#248462=CARTESIAN_POINT('Ctrl Pts',(10.7695073079554,21.6055654018179,12.));
#248463=CARTESIAN_POINT('Ctrl Pts',(10.7858084708262,21.6205198677176,0.));
#248464=CARTESIAN_POINT('Ctrl Pts',(10.7858084708262,21.6205198677176,12.));
#248465=CARTESIAN_POINT('Ctrl Pts',(10.8022189912369,21.6354975534558,0.));
#248466=CARTESIAN_POINT('Ctrl Pts',(10.8022189912369,21.6354975534558,12.));
#248467=CARTESIAN_POINT('Ctrl Pts',(10.8187386025135,21.6504977276864,0.));
#248468=CARTESIAN_POINT('Ctrl Pts',(10.8187386025135,21.6504977276864,12.));
#248469=CARTESIAN_POINT('Ctrl Pts',(10.835367039227,21.6655196669727,0.));
#248470=CARTESIAN_POINT('Ctrl Pts',(10.835367039227,21.6655196669727,12.));
#248471=CARTESIAN_POINT('Ctrl Pts',(10.8521040371832,21.6805626556461,0.));
#248472=CARTESIAN_POINT('Ctrl Pts',(10.8521040371832,21.6805626556461,12.));
#248473=CARTESIAN_POINT('Ctrl Pts',(10.8689493334093,21.6956259856667,0.));
#248474=CARTESIAN_POINT('Ctrl Pts',(10.8689493334093,21.6956259856667,12.));
#248475=CARTESIAN_POINT('Ctrl Pts',(10.8859026661292,21.7107089564822,0.));
#248476=CARTESIAN_POINT('Ctrl Pts',(10.8859026661292,21.7107089564822,12.));
#248477=CARTESIAN_POINT('Ctrl Pts',(10.9029637747341,21.7258108748874,0.));
#248478=CARTESIAN_POINT('Ctrl Pts',(10.9029637747341,21.7258108748874,12.));
#248479=CARTESIAN_POINT('Ctrl Pts',(10.9201323997386,21.74093105488,0.));
#248480=CARTESIAN_POINT('Ctrl Pts',(10.9201323997386,21.74093105488,12.));
#248481=CARTESIAN_POINT('Ctrl Pts',(10.9374082827446,21.7560688175252,0.));
#248482=CARTESIAN_POINT('Ctrl Pts',(10.9374082827446,21.7560688175252,12.));
#248483=CARTESIAN_POINT('Ctrl Pts',(10.9547911664457,21.7712234908468,0.));
#248484=CARTESIAN_POINT('Ctrl Pts',(10.9547911664457,21.7712234908468,12.));
#248485=CARTESIAN_POINT('Ctrl Pts',(10.9722807946157,21.7863944097143,0.));
#248486=CARTESIAN_POINT('Ctrl Pts',(10.9722807946157,21.7863944097143,12.));
#248487=CARTESIAN_POINT('Ctrl Pts',(10.9898769120913,21.8015809157302,0.));
#248488=CARTESIAN_POINT('Ctrl Pts',(10.9898769120913,21.8015809157302,12.));
#248489=CARTESIAN_POINT('Ctrl Pts',(11.0075792647477,21.8167823571168,0.));
#248490=CARTESIAN_POINT('Ctrl Pts',(11.0075792647477,21.8167823571168,12.));
#248491=CARTESIAN_POINT('Ctrl Pts',(11.0253875994598,21.8319980886033,0.));
#248492=CARTESIAN_POINT('Ctrl Pts',(11.0253875994598,21.8319980886033,12.));
#248493=CARTESIAN_POINT('Ctrl Pts',(11.0433016640808,21.8472274713103,0.));
#248494=CARTESIAN_POINT('Ctrl Pts',(11.0433016640808,21.8472274713103,12.));
#248495=CARTESIAN_POINT('Ctrl Pts',(11.0613212074364,21.8624698726319,0.));
#248496=CARTESIAN_POINT('Ctrl Pts',(11.0613212074364,21.8624698726319,12.));
#248497=CARTESIAN_POINT('Ctrl Pts',(11.0794459793058,21.8777246661191,0.));
#248498=CARTESIAN_POINT('Ctrl Pts',(11.0794459793058,21.8777246661191,12.));
#248499=CARTESIAN_POINT('Ctrl Pts',(11.0976757303944,21.8929912313608,0.));
#248500=CARTESIAN_POINT('Ctrl Pts',(11.0976757303944,21.8929912313608,12.));
#248501=CARTESIAN_POINT('Ctrl Pts',(11.1160102123024,21.9082689538687,0.));
#248502=CARTESIAN_POINT('Ctrl Pts',(11.1160102123024,21.9082689538687,12.));
#248503=CARTESIAN_POINT('Ctrl Pts',(11.134449177474,21.9235572249518,0.));
#248504=CARTESIAN_POINT('Ctrl Pts',(11.134449177474,21.9235572249518,12.));
#248505=CARTESIAN_POINT('Ctrl Pts',(11.1529923792002,21.9388554416437,0.));
#248506=CARTESIAN_POINT('Ctrl Pts',(11.1529923792002,21.9388554416437,12.));
#248507=CARTESIAN_POINT('Ctrl Pts',(11.1716395716375,21.9541630066504,0.));
#248508=CARTESIAN_POINT('Ctrl Pts',(11.1716395716375,21.9541630066504,12.));
#248509=CARTESIAN_POINT('Ctrl Pts',(11.1903905098109,21.9694793282913,0.));
#248510=CARTESIAN_POINT('Ctrl Pts',(11.1903905098109,21.9694793282913,12.));
#248511=CARTESIAN_POINT('Ctrl Pts',(11.2092449496125,21.9848038204439,0.));
#248512=CARTESIAN_POINT('Ctrl Pts',(11.2092449496125,21.9848038204439,12.));
#248513=CARTESIAN_POINT('Ctrl Pts',(11.2282026477897,22.000135902484,0.));
#248514=CARTESIAN_POINT('Ctrl Pts',(11.2282026477897,22.000135902484,12.));
#248515=CARTESIAN_POINT('Ctrl Pts',(11.2472633619276,22.0154749992364,0.));
#248516=CARTESIAN_POINT('Ctrl Pts',(11.2472633619276,22.0154749992364,12.));
#248517=CARTESIAN_POINT('Ctrl Pts',(11.2664268504207,22.0308205408351,0.));
#248518=CARTESIAN_POINT('Ctrl Pts',(11.2664268504207,22.0308205408351,12.));
#248519=CARTESIAN_POINT('Ctrl Pts',(11.2856928724374,22.0461719625661,0.));
#248520=CARTESIAN_POINT('Ctrl Pts',(11.2856928724374,22.0461719625661,12.));
#248521=CARTESIAN_POINT('Ctrl Pts',(11.3050611878771,22.0615287047179,0.));
#248522=CARTESIAN_POINT('Ctrl Pts',(11.3050611878771,22.0615287047179,12.));
#248523=CARTESIAN_POINT('Ctrl Pts',(11.3245315573168,22.0768902124267,0.));
#248524=CARTESIAN_POINT('Ctrl Pts',(11.3245315573168,22.0768902124267,12.));
#248525=CARTESIAN_POINT('Ctrl Pts',(11.3441037419553,22.0922559355293,0.));
#248526=CARTESIAN_POINT('Ctrl Pts',(11.3441037419553,22.0922559355293,12.));
#248527=CARTESIAN_POINT('Ctrl Pts',(11.3637775035367,22.1076253283978,0.));
#248528=CARTESIAN_POINT('Ctrl Pts',(11.3637775035367,22.1076253283978,12.));
#248529=CARTESIAN_POINT('Ctrl Pts',(11.3835526044256,22.1229978500185,0.));
#248530=CARTESIAN_POINT('Ctrl Pts',(11.3835526044256,22.1229978500185,12.));
#248531=CARTESIAN_POINT('Ctrl Pts',(11.4034288076908,22.1383729640963,0.));
#248532=CARTESIAN_POINT('Ctrl Pts',(11.4034288076908,22.1383729640963,12.));
#248533=CARTESIAN_POINT('Ctrl Pts',(11.4234058771742,22.1537501391486,0.));
#248534=CARTESIAN_POINT('Ctrl Pts',(11.4234058771742,22.1537501391486,12.));
#248535=CARTESIAN_POINT('Ctrl Pts',(11.443483577557,22.1691288486096,0.));
#248536=CARTESIAN_POINT('Ctrl Pts',(11.443483577557,22.1691288486096,12.));
#248537=CARTESIAN_POINT('Ctrl Pts',(11.463661674411,22.184508570917,0.));
#248538=CARTESIAN_POINT('Ctrl Pts',(11.463661674411,22.184508570917,12.));
#248539=CARTESIAN_POINT('Ctrl Pts',(11.4839399342589,22.1998887896435,0.));
#248540=CARTESIAN_POINT('Ctrl Pts',(11.4839399342589,22.1998887896435,12.));
#248541=CARTESIAN_POINT('Ctrl Pts',(11.504318124424,22.215268993102,0.));
#248542=CARTESIAN_POINT('Ctrl Pts',(11.504318124424,22.215268993102,12.));
#248543=CARTESIAN_POINT('Ctrl Pts',(11.5247960128476,22.2306486738899,0.));
#248544=CARTESIAN_POINT('Ctrl Pts',(11.5247960128476,22.2306486738899,12.));
#248545=CARTESIAN_POINT('Ctrl Pts',(11.545373367912,22.2460273284653,0.));
#248546=CARTESIAN_POINT('Ctrl Pts',(11.545373367912,22.2460273284653,12.));
#248547=CARTESIAN_POINT('Ctrl Pts',(11.5660499582403,22.2614044566898,0.));
#248548=CARTESIAN_POINT('Ctrl Pts',(11.5660499582403,22.2614044566898,12.));
#248549=CARTESIAN_POINT('Ctrl Pts',(11.5868255525189,22.2767795614349,0.));
#248550=CARTESIAN_POINT('Ctrl Pts',(11.5868255525189,22.2767795614349,12.));
#248551=CARTESIAN_POINT('Ctrl Pts',(11.6076999192359,22.2921521480358,0.));
#248552=CARTESIAN_POINT('Ctrl Pts',(11.6076999192359,22.2921521480358,12.));
#248553=CARTESIAN_POINT('Ctrl Pts',(11.6286728270011,22.3075217249049,0.));
#248554=CARTESIAN_POINT('Ctrl Pts',(11.6286728270011,22.3075217249049,12.));
#248555=CARTESIAN_POINT('Ctrl Pts',(11.6497440449858,22.3228878043976,0.));
#248556=CARTESIAN_POINT('Ctrl Pts',(11.6497440449858,22.3228878043976,12.));
#248557=CARTESIAN_POINT('Ctrl Pts',(11.6709133432986,22.3382499035618,0.));
#248558=CARTESIAN_POINT('Ctrl Pts',(11.6709133432986,22.3382499035618,12.));
#248559=CARTESIAN_POINT('Ctrl Pts',(11.6921804934056,22.3536075450028,0.));
#248560=CARTESIAN_POINT('Ctrl Pts',(11.6921804934056,22.3536075450028,12.));
#248561=CARTESIAN_POINT('Ctrl Pts',(11.7135452684532,22.3689602575492,0.));
#248562=CARTESIAN_POINT('Ctrl Pts',(11.7135452684532,22.3689602575492,12.));
#248563=CARTESIAN_POINT('Ctrl Pts',(11.7350074437961,22.3843075773905,0.));
#248564=CARTESIAN_POINT('Ctrl Pts',(11.7350074437961,22.3843075773905,12.));
#248565=CARTESIAN_POINT('Ctrl Pts',(11.7565667964765,22.39964904692,0.));
#248566=CARTESIAN_POINT('Ctrl Pts',(11.7565667964765,22.39964904692,12.));
#248567=CARTESIAN_POINT('Ctrl Pts',(11.7782231042041,22.4149842125018,0.));
#248568=CARTESIAN_POINT('Ctrl Pts',(11.7782231042041,22.4149842125018,12.));
#248569=CARTESIAN_POINT('Ctrl Pts',(11.7999761445175,22.4303126226468,0.));
#248570=CARTESIAN_POINT('Ctrl Pts',(11.7999761445175,22.4303126226468,12.));
#248571=CARTESIAN_POINT('Ctrl Pts',(11.8218256937889,22.4456338258738,0.));
#248572=CARTESIAN_POINT('Ctrl Pts',(11.8218256937889,22.4456338258738,12.));
#248573=CARTESIAN_POINT('Ctrl Pts',(11.8437715264487,22.4609473690469,0.));
#248574=CARTESIAN_POINT('Ctrl Pts',(11.8437715264487,22.4609473690469,12.));
#248575=CARTESIAN_POINT('Ctrl Pts',(11.8658134137018,22.4762527946694,0.));
#248576=CARTESIAN_POINT('Ctrl Pts',(11.8658134137018,22.4762527946694,12.));
#248577=CARTESIAN_POINT('Ctrl Pts',(11.8879511239941,22.4915496418472,0.));
#248578=CARTESIAN_POINT('Ctrl Pts',(11.8879511239941,22.4915496418472,12.));
#248579=CARTESIAN_POINT('Ctrl Pts',(11.9101844254555,22.5068374513958,0.));
#248580=CARTESIAN_POINT('Ctrl Pts',(11.9101844254555,22.5068374513958,12.));
#248581=CARTESIAN_POINT('Ctrl Pts',(11.9325130877801,22.5221157697869,0.));
#248582=CARTESIAN_POINT('Ctrl Pts',(11.9325130877801,22.5221157697869,12.));
#248583=CARTESIAN_POINT('Ctrl Pts',(11.9549368843996,22.5373841537299,0.));
#248584=CARTESIAN_POINT('Ctrl Pts',(11.9549368843996,22.5373841537299,12.));
#248585=CARTESIAN_POINT('Ctrl Pts',(11.9774555943496,22.5526421741159,0.));
#248586=CARTESIAN_POINT('Ctrl Pts',(11.9774555943496,22.5526421741159,12.));
#248587=CARTESIAN_POINT('Ctrl Pts',(12.0000690046697,22.5678894211194,0.));
#248588=CARTESIAN_POINT('Ctrl Pts',(12.0000690046697,22.5678894211194,12.));
#248589=CARTESIAN_POINT('Ctrl Pts',(12.0227769113132,22.5831255061306,0.));
#248590=CARTESIAN_POINT('Ctrl Pts',(12.0227769113132,22.5831255061306,12.));
#248591=CARTESIAN_POINT('Ctrl Pts',(12.0455791139135,22.5983500505675,0.));
#248592=CARTESIAN_POINT('Ctrl Pts',(12.0455791139135,22.5983500505675,12.));
#248593=CARTESIAN_POINT('Ctrl Pts',(12.0684754113869,22.613562676493,0.));
#248594=CARTESIAN_POINT('Ctrl Pts',(12.0684754113869,22.613562676493,12.));
#248595=CARTESIAN_POINT('Ctrl Pts',(12.0914655972828,22.628762996708,0.));
#248596=CARTESIAN_POINT('Ctrl Pts',(12.0914655972828,22.628762996708,12.));
#248597=CARTESIAN_POINT('Ctrl Pts',(12.1145494550384,22.6439506046611,0.));
#248598=CARTESIAN_POINT('Ctrl Pts',(12.1145494550384,22.6439506046611,12.));
#248599=CARTESIAN_POINT('Ctrl Pts',(12.1377267537141,22.6591250653942,0.));
#248600=CARTESIAN_POINT('Ctrl Pts',(12.1377267537141,22.6591250653942,12.));
#248601=CARTESIAN_POINT('Ctrl Pts',(12.1609972423088,22.6742859034891,0.));
#248602=CARTESIAN_POINT('Ctrl Pts',(12.1609972423088,22.6742859034891,12.));
#248603=CARTESIAN_POINT('Ctrl Pts',(12.1843606579246,22.6894326204959,0.));
#248604=CARTESIAN_POINT('Ctrl Pts',(12.1843606579246,22.6894326204959,12.));
#248605=CARTESIAN_POINT('Ctrl Pts',(12.2078167360267,22.7045647168659,0.));
#248606=CARTESIAN_POINT('Ctrl Pts',(12.2078167360267,22.7045647168659,12.));
#248607=CARTESIAN_POINT('Ctrl Pts',(12.2313652198047,22.7196817119299,0.));
#248608=CARTESIAN_POINT('Ctrl Pts',(12.2313652198047,22.7196817119299,12.));
#248609=CARTESIAN_POINT('Ctrl Pts',(12.2550058702389,22.7347831655251,0.));
#248610=CARTESIAN_POINT('Ctrl Pts',(12.2550058702389,22.7347831655251,12.));
#248611=CARTESIAN_POINT('Ctrl Pts',(12.2787384750747,22.7498686970096,0.));
#248612=CARTESIAN_POINT('Ctrl Pts',(12.2787384750747,22.7498686970096,12.));
#248613=CARTESIAN_POINT('Ctrl Pts',(12.3025628601811,22.7649380101154,0.));
#248614=CARTESIAN_POINT('Ctrl Pts',(12.3025628601811,22.7649380101154,12.));
#248615=CARTESIAN_POINT('Ctrl Pts',(12.3264788926108,22.7799908974947,0.));
#248616=CARTESIAN_POINT('Ctrl Pts',(12.3264788926108,22.7799908974947,12.));
#248617=CARTESIAN_POINT('Ctrl Pts',(12.3504864740361,22.7950272216959,0.));
#248618=CARTESIAN_POINT('Ctrl Pts',(12.3504864740361,22.7950272216959,12.));
#248619=CARTESIAN_POINT('Ctrl Pts',(12.3745855366772,22.8100469022632,0.));
#248620=CARTESIAN_POINT('Ctrl Pts',(12.3745855366772,22.8100469022632,12.));
#248621=CARTESIAN_POINT('Ctrl Pts',(12.393937937903,22.8220493007353,0.));
#248622=CARTESIAN_POINT('Ctrl Pts',(12.393937937903,22.8220493007353,12.));
#248623=CARTESIAN_POINT('Ctrl Pts',(12.4084933766366,22.8310435872852,0.));
#248624=CARTESIAN_POINT('Ctrl Pts',(12.4084933766366,22.8310435872852,12.));
#248625=CARTESIAN_POINT('Ctrl Pts',(12.4182152851867,22.8370364396497,0.));
#248626=CARTESIAN_POINT('Ctrl Pts',(12.4182152851867,22.8370364396497,12.));
#248627=CARTESIAN_POINT('Ctrl Pts',(12.4230808101438,22.8400320311648,0.));
#248628=CARTESIAN_POINT('Ctrl Pts',(12.4230808101438,22.8400320311648,12.));
#248629=CARTESIAN_POINT('',(12.4230808101438,22.8400320311648,0.));
#248630=CARTESIAN_POINT('Ctrl Pts',(9.71462809124917,20.353053841303,0.));
#248631=CARTESIAN_POINT('Ctrl Pts',(9.71462954053074,20.353060251684,0.));
#248632=CARTESIAN_POINT('Ctrl Pts',(9.71465227853122,20.3531126095522,0.));
#248633=CARTESIAN_POINT('Ctrl Pts',(9.71474590350791,20.3533097561886,0.));
#248634=CARTESIAN_POINT('Ctrl Pts',(9.714989780521,20.3538098605706,0.));
#248635=CARTESIAN_POINT('Ctrl Pts',(9.71549257088174,20.3548282742361,0.));
#248636=CARTESIAN_POINT('Ctrl Pts',(9.71619192554146,20.3562337557875,0.));
#248637=CARTESIAN_POINT('Ctrl Pts',(9.71708493723061,20.3580133103357,0.));
#248638=CARTESIAN_POINT('Ctrl Pts',(9.71816778327998,20.3601498764344,0.));
#248639=CARTESIAN_POINT('Ctrl Pts',(9.71943648548114,20.362625691398,0.));
#248640=CARTESIAN_POINT('Ctrl Pts',(9.72088778381101,20.3654261611055,0.));
#248641=CARTESIAN_POINT('Ctrl Pts',(9.72251930722503,20.3685406190576,0.));
#248642=CARTESIAN_POINT('Ctrl Pts',(9.72432910043192,20.371960235676,0.));
#248643=CARTESIAN_POINT('Ctrl Pts',(9.7263153173287,20.3756766651952,0.));
#248644=CARTESIAN_POINT('Ctrl Pts',(9.72847589116532,20.3796805893304,0.));
#248645=CARTESIAN_POINT('Ctrl Pts',(9.73080870123726,20.3839624556742,0.));
#248646=CARTESIAN_POINT('Ctrl Pts',(9.73331167102812,20.3885129129912,0.));
#248647=CARTESIAN_POINT('Ctrl Pts',(9.73598292014249,20.3933234845646,0.));
#248648=CARTESIAN_POINT('Ctrl Pts',(9.73882077613206,20.3983866213331,0.));
#248649=CARTESIAN_POINT('Ctrl Pts',(9.74182369656272,20.4036953576549,0.));
#248650=CARTESIAN_POINT('Ctrl Pts',(9.74499021838536,20.4092430879861,0.));
#248651=CARTESIAN_POINT('Ctrl Pts',(9.74831889242174,20.4150232777393,0.));
#248652=CARTESIAN_POINT('Ctrl Pts',(9.75180829786433,20.4210295275818,0.));
#248653=CARTESIAN_POINT('Ctrl Pts',(9.75545705902416,20.4272556476629,0.));
#248654=CARTESIAN_POINT('Ctrl Pts',(9.75926386289929,20.4336957355474,0.));
#248655=CARTESIAN_POINT('Ctrl Pts',(9.76322747195502,20.4403442329401,0.));
#248656=CARTESIAN_POINT('Ctrl Pts',(9.76734670980896,20.447195862298,0.));
#248657=CARTESIAN_POINT('Ctrl Pts',(9.77162045104069,20.4542455817527,0.));
#248658=CARTESIAN_POINT('Ctrl Pts',(9.77604760815522,20.4614885274973,0.));
#248659=CARTESIAN_POINT('Ctrl Pts',(9.78062712373313,20.4689199790668,0.));
#248660=CARTESIAN_POINT('Ctrl Pts',(9.78535797314162,20.4765353711585,0.));
#248661=CARTESIAN_POINT('Ctrl Pts',(9.79023916498659,20.4843302955329,0.));
#248662=CARTESIAN_POINT('Ctrl Pts',(9.79526974288343,20.4923005087945,0.));
#248663=CARTESIAN_POINT('Ctrl Pts',(9.80044878520967,20.500441931211,0.));
#248664=CARTESIAN_POINT('Ctrl Pts',(9.80577540161102,20.5087506310507,0.));
#248665=CARTESIAN_POINT('Ctrl Pts',(9.81124873025278,20.5172228122839,0.));
#248666=CARTESIAN_POINT('Ctrl Pts',(9.81686793455918,20.5258548000625,0.));
#248667=CARTESIAN_POINT('Ctrl Pts',(9.82263220080327,20.534643029951,0.));
#248668=CARTESIAN_POINT('Ctrl Pts',(9.82854073773857,20.5435840460717,0.));
#248669=CARTESIAN_POINT('Ctrl Pts',(9.8345927758532,20.5526744976461,0.));
#248670=CARTESIAN_POINT('Ctrl Pts',(9.84078756677589,20.5619111362406,0.));
#248671=CARTESIAN_POINT('Ctrl Pts',(9.84712438256308,20.5712908125145,0.));
#248672=CARTESIAN_POINT('Ctrl Pts',(9.85360251457004,20.580810471002,0.));
#248673=CARTESIAN_POINT('Ctrl Pts',(9.86022127232749,20.5904671449755,0.));
#248674=CARTESIAN_POINT('Ctrl Pts',(9.86697998242612,20.6002579513696,0.));
#248675=CARTESIAN_POINT('Ctrl Pts',(9.87387798732943,20.6101800854491,0.));
#248676=CARTESIAN_POINT('Ctrl Pts',(9.88091464472669,20.6202308177472,0.));
#248677=CARTESIAN_POINT('Ctrl Pts',(9.88808932697304,20.6304074914086,0.));
#248678=CARTESIAN_POINT('Ctrl Pts',(9.89540142049123,20.6407075193977,0.));
#248679=CARTESIAN_POINT('Ctrl Pts',(9.90285032516695,20.6511283817415,0.));
#248680=CARTESIAN_POINT('Ctrl Pts',(9.91043545377004,20.6616676228315,0.));
#248681=CARTESIAN_POINT('Ctrl Pts',(9.91815623141284,20.6723228488262,0.));
#248682=CARTESIAN_POINT('Ctrl Pts',(9.9260120949875,20.6830917250255,0.));
#248683=CARTESIAN_POINT('Ctrl Pts',(9.93400249259736,20.6939719732485,0.));
#248684=CARTESIAN_POINT('Ctrl Pts',(9.9421268829825,20.7049613692237,0.));
#248685=CARTESIAN_POINT('Ctrl Pts',(9.95038473514962,20.7160577407581,0.));
#248686=CARTESIAN_POINT('Ctrl Pts',(9.95877552798403,20.7272589658752,0.));
#248687=CARTESIAN_POINT('Ctrl Pts',(9.96729874986198,20.7385629709795,0.));
#248688=CARTESIAN_POINT('Ctrl Pts',(9.97595389823461,20.7499677289626,0.));
#248689=CARTESIAN_POINT('Ctrl Pts',(9.98474047926846,20.7614712574989,0.));
#248690=CARTESIAN_POINT('Ctrl Pts',(9.99365800754637,20.7730716175417,0.));
#248691=CARTESIAN_POINT('Ctrl Pts',(10.0027060057389,20.7847669117568,0.));
#248692=CARTESIAN_POINT('Ctrl Pts',(10.0118840042786,20.7965552829907,0.));
#248693=CARTESIAN_POINT('Ctrl Pts',(10.0211915410095,20.8084349126885,0.));
#248694=CARTESIAN_POINT('Ctrl Pts',(10.0306281609435,20.8204040196599,0.));
#248695=CARTESIAN_POINT('Ctrl Pts',(10.0401934160234,20.8324608588906,0.));
#248696=CARTESIAN_POINT('Ctrl Pts',(10.0498868648733,20.8446037203402,0.));
#248697=CARTESIAN_POINT('Ctrl Pts',(10.0597080725375,20.856830927732,0.));
#248698=CARTESIAN_POINT('Ctrl Pts',(10.0696566102219,20.8691408373705,0.));
#248699=CARTESIAN_POINT('Ctrl Pts',(10.0797320551154,20.8815318371844,0.));
#248700=CARTESIAN_POINT('Ctrl Pts',(10.0899339901916,20.8940023457371,0.));
#248701=CARTESIAN_POINT('Ctrl Pts',(10.1002620040076,20.9065508112556,0.));
#248702=CARTESIAN_POINT('Ctrl Pts',(10.1107156904836,20.9191757106266,0.));
#248703=CARTESIAN_POINT('Ctrl Pts',(10.1212946487057,20.931875548473,0.));
#248704=CARTESIAN_POINT('Ctrl Pts',(10.1319984827909,20.944648856393,0.));
#248705=CARTESIAN_POINT('Ctrl Pts',(10.1428268017257,20.9574941921591,0.));
#248706=CARTESIAN_POINT('Ctrl Pts',(10.1537792192065,20.970410138937,0.));
#248707=CARTESIAN_POINT('Ctrl Pts',(10.1648553534567,20.9833953044737,0.));
#248708=CARTESIAN_POINT('Ctrl Pts',(10.1760548270765,20.9964483203685,0.));
#248709=CARTESIAN_POINT('Ctrl Pts',(10.1873772669358,21.0095678414486,0.));
#248710=CARTESIAN_POINT('Ctrl Pts',(10.1988223040425,21.0227525451107,0.));
#248711=CARTESIAN_POINT('Ctrl Pts',(10.2103895734123,21.0360011306814,0.));
#248712=CARTESIAN_POINT('Ctrl Pts',(10.2220787139157,21.0493123187484,0.));
#248713=CARTESIAN_POINT('Ctrl Pts',(10.233889368157,21.0626848505665,0.));
#248714=CARTESIAN_POINT('Ctrl Pts',(10.2458211823915,21.0761174875448,0.));
#248715=CARTESIAN_POINT('Ctrl Pts',(10.2578738064183,21.0896090107066,0.));
#248716=CARTESIAN_POINT('Ctrl Pts',(10.2700468934743,21.1031582201625,0.));
#248717=CARTESIAN_POINT('Ctrl Pts',(10.2823401001067,21.1167639345623,0.));
#248718=CARTESIAN_POINT('Ctrl Pts',(10.2947530860714,21.130424990599,0.));
#248719=CARTESIAN_POINT('Ctrl Pts',(10.307285514268,21.1441402425831,0.));
#248720=CARTESIAN_POINT('Ctrl Pts',(10.3199370506541,21.1579085619959,0.));
#248721=CARTESIAN_POINT('Ctrl Pts',(10.3327073641574,21.1717288370512,0.));
#248722=CARTESIAN_POINT('Ctrl Pts',(10.3455961265706,21.1855999722427,0.));
#248723=CARTESIAN_POINT('Ctrl Pts',(10.3586030124595,21.1995208879205,0.));
#248724=CARTESIAN_POINT('Ctrl Pts',(10.3717276991137,21.2134905199359,0.));
#248725=CARTESIAN_POINT('Ctrl Pts',(10.384969866479,21.2275078192708,0.));
#248726=CARTESIAN_POINT('Ctrl Pts',(10.3983291970846,21.2415717516713,0.));
#248727=CARTESIAN_POINT('Ctrl Pts',(10.4118053759584,21.2556812972741,0.));
#248728=CARTESIAN_POINT('Ctrl Pts',(10.4253980905394,21.2698354502391,0.));
#248729=CARTESIAN_POINT('Ctrl Pts',(10.4391070306385,21.2840332184471,0.));
#248730=CARTESIAN_POINT('Ctrl Pts',(10.452931888387,21.2982736231924,0.));
#248731=CARTESIAN_POINT('Ctrl Pts',(10.4668723581768,21.312555698873,0.));
#248732=CARTESIAN_POINT('Ctrl Pts',(10.4809281365933,21.3268784926823,0.));
#248733=CARTESIAN_POINT('Ctrl Pts',(10.4950989223341,21.3412410642912,0.));
#248734=CARTESIAN_POINT('Ctrl Pts',(10.5093844161689,21.3556424855822,0.));
#248735=CARTESIAN_POINT('Ctrl Pts',(10.523784320906,21.3700818403942,0.));
#248736=CARTESIAN_POINT('Ctrl Pts',(10.5382983413422,21.3845582242604,0.));
#248737=CARTESIAN_POINT('Ctrl Pts',(10.5529261842107,21.3990707441495,0.));
#248738=CARTESIAN_POINT('Ctrl Pts',(10.5676675581106,21.4136185181974,0.));
#248739=CARTESIAN_POINT('Ctrl Pts',(10.582522173457,21.4282006754624,0.));
#248740=CARTESIAN_POINT('Ctrl Pts',(10.597489742462,21.4428163557137,0.));
#248741=CARTESIAN_POINT('Ctrl Pts',(10.612569979096,21.4574647092093,0.));
#248742=CARTESIAN_POINT('Ctrl Pts',(10.6277625990456,21.4721448964766,0.));
#248743=CARTESIAN_POINT('Ctrl Pts',(10.6430673196609,21.4868560880893,0.));
#248744=CARTESIAN_POINT('Ctrl Pts',(10.658483859894,21.5015974644454,0.));
#248745=CARTESIAN_POINT('Ctrl Pts',(10.6740119402835,21.5163682155805,0.));
#248746=CARTESIAN_POINT('Ctrl Pts',(10.689651282929,21.531167540981,0.));
#248747=CARTESIAN_POINT('Ctrl Pts',(10.7054016114571,21.5459946493955,0.));
#248748=CARTESIAN_POINT('Ctrl Pts',(10.7212626509816,21.5608487586467,0.));
#248749=CARTESIAN_POINT('Ctrl Pts',(10.7372341280468,21.5757290954372,0.));
#248750=CARTESIAN_POINT('Ctrl Pts',(10.7533157705943,21.5906348951745,0.));
#248751=CARTESIAN_POINT('Ctrl Pts',(10.7695073079554,21.6055654018179,0.));
#248752=CARTESIAN_POINT('Ctrl Pts',(10.7858084708262,21.6205198677176,0.));
#248753=CARTESIAN_POINT('Ctrl Pts',(10.8022189912369,21.6354975534558,0.));
#248754=CARTESIAN_POINT('Ctrl Pts',(10.8187386025135,21.6504977276864,0.));
#248755=CARTESIAN_POINT('Ctrl Pts',(10.835367039227,21.6655196669727,0.));
#248756=CARTESIAN_POINT('Ctrl Pts',(10.8521040371832,21.6805626556461,0.));
#248757=CARTESIAN_POINT('Ctrl Pts',(10.8689493334093,21.6956259856667,0.));
#248758=CARTESIAN_POINT('Ctrl Pts',(10.8859026661292,21.7107089564822,0.));
#248759=CARTESIAN_POINT('Ctrl Pts',(10.9029637747341,21.7258108748874,0.));
#248760=CARTESIAN_POINT('Ctrl Pts',(10.9201323997386,21.74093105488,0.));
#248761=CARTESIAN_POINT('Ctrl Pts',(10.9374082827446,21.7560688175252,0.));
#248762=CARTESIAN_POINT('Ctrl Pts',(10.9547911664457,21.7712234908468,0.));
#248763=CARTESIAN_POINT('Ctrl Pts',(10.9722807946157,21.7863944097143,0.));
#248764=CARTESIAN_POINT('Ctrl Pts',(10.9898769120913,21.8015809157302,0.));
#248765=CARTESIAN_POINT('Ctrl Pts',(11.0075792647477,21.8167823571168,0.));
#248766=CARTESIAN_POINT('Ctrl Pts',(11.0253875994598,21.8319980886033,0.));
#248767=CARTESIAN_POINT('Ctrl Pts',(11.0433016640808,21.8472274713103,0.));
#248768=CARTESIAN_POINT('Ctrl Pts',(11.0613212074364,21.8624698726319,0.));
#248769=CARTESIAN_POINT('Ctrl Pts',(11.0794459793058,21.8777246661191,0.));
#248770=CARTESIAN_POINT('Ctrl Pts',(11.0976757303944,21.8929912313608,0.));
#248771=CARTESIAN_POINT('Ctrl Pts',(11.1160102123024,21.9082689538687,0.));
#248772=CARTESIAN_POINT('Ctrl Pts',(11.134449177474,21.9235572249518,0.));
#248773=CARTESIAN_POINT('Ctrl Pts',(11.1529923792002,21.9388554416437,0.));
#248774=CARTESIAN_POINT('Ctrl Pts',(11.1716395716375,21.9541630066504,0.));
#248775=CARTESIAN_POINT('Ctrl Pts',(11.1903905098109,21.9694793282913,0.));
#248776=CARTESIAN_POINT('Ctrl Pts',(11.2092449496125,21.9848038204439,0.));
#248777=CARTESIAN_POINT('Ctrl Pts',(11.2282026477897,22.000135902484,0.));
#248778=CARTESIAN_POINT('Ctrl Pts',(11.2472633619276,22.0154749992364,0.));
#248779=CARTESIAN_POINT('Ctrl Pts',(11.2664268504207,22.0308205408351,0.));
#248780=CARTESIAN_POINT('Ctrl Pts',(11.2856928724374,22.0461719625661,0.));
#248781=CARTESIAN_POINT('Ctrl Pts',(11.3050611878771,22.0615287047179,0.));
#248782=CARTESIAN_POINT('Ctrl Pts',(11.3245315573168,22.0768902124267,0.));
#248783=CARTESIAN_POINT('Ctrl Pts',(11.3441037419553,22.0922559355293,0.));
#248784=CARTESIAN_POINT('Ctrl Pts',(11.3637775035367,22.1076253283978,0.));
#248785=CARTESIAN_POINT('Ctrl Pts',(11.3835526044256,22.1229978500185,0.));
#248786=CARTESIAN_POINT('Ctrl Pts',(11.4034288076908,22.1383729640963,0.));
#248787=CARTESIAN_POINT('Ctrl Pts',(11.4234058771742,22.1537501391486,0.));
#248788=CARTESIAN_POINT('Ctrl Pts',(11.443483577557,22.1691288486096,0.));
#248789=CARTESIAN_POINT('Ctrl Pts',(11.463661674411,22.184508570917,0.));
#248790=CARTESIAN_POINT('Ctrl Pts',(11.4839399342589,22.1998887896435,0.));
#248791=CARTESIAN_POINT('Ctrl Pts',(11.504318124424,22.215268993102,0.));
#248792=CARTESIAN_POINT('Ctrl Pts',(11.5247960128476,22.2306486738899,0.));
#248793=CARTESIAN_POINT('Ctrl Pts',(11.545373367912,22.2460273284653,0.));
#248794=CARTESIAN_POINT('Ctrl Pts',(11.5660499582403,22.2614044566898,0.));
#248795=CARTESIAN_POINT('Ctrl Pts',(11.5868255525189,22.2767795614349,0.));
#248796=CARTESIAN_POINT('Ctrl Pts',(11.6076999192359,22.2921521480358,0.));
#248797=CARTESIAN_POINT('Ctrl Pts',(11.6286728270011,22.3075217249049,0.));
#248798=CARTESIAN_POINT('Ctrl Pts',(11.6497440449858,22.3228878043976,0.));
#248799=CARTESIAN_POINT('Ctrl Pts',(11.6709133432986,22.3382499035618,0.));
#248800=CARTESIAN_POINT('Ctrl Pts',(11.6921804934056,22.3536075450028,0.));
#248801=CARTESIAN_POINT('Ctrl Pts',(11.7135452684532,22.3689602575492,0.));
#248802=CARTESIAN_POINT('Ctrl Pts',(11.7350074437961,22.3843075773905,0.));
#248803=CARTESIAN_POINT('Ctrl Pts',(11.7565667964765,22.39964904692,0.));
#248804=CARTESIAN_POINT('Ctrl Pts',(11.7782231042041,22.4149842125018,0.));
#248805=CARTESIAN_POINT('Ctrl Pts',(11.7999761445175,22.4303126226468,0.));
#248806=CARTESIAN_POINT('Ctrl Pts',(11.8218256937889,22.4456338258738,0.));
#248807=CARTESIAN_POINT('Ctrl Pts',(11.8437715264487,22.4609473690469,0.));
#248808=CARTESIAN_POINT('Ctrl Pts',(11.8658134137018,22.4762527946694,0.));
#248809=CARTESIAN_POINT('Ctrl Pts',(11.8879511239941,22.4915496418472,0.));
#248810=CARTESIAN_POINT('Ctrl Pts',(11.9101844254555,22.5068374513958,0.));
#248811=CARTESIAN_POINT('Ctrl Pts',(11.9325130877801,22.5221157697869,0.));
#248812=CARTESIAN_POINT('Ctrl Pts',(11.9549368843996,22.5373841537299,0.));
#248813=CARTESIAN_POINT('Ctrl Pts',(11.9774555943496,22.5526421741159,0.));
#248814=CARTESIAN_POINT('Ctrl Pts',(12.0000690046697,22.5678894211194,0.));
#248815=CARTESIAN_POINT('Ctrl Pts',(12.0227769113132,22.5831255061306,0.));
#248816=CARTESIAN_POINT('Ctrl Pts',(12.0455791139135,22.5983500505675,0.));
#248817=CARTESIAN_POINT('Ctrl Pts',(12.0684754113869,22.613562676493,0.));
#248818=CARTESIAN_POINT('Ctrl Pts',(12.0914655972828,22.628762996708,0.));
#248819=CARTESIAN_POINT('Ctrl Pts',(12.1145494550384,22.6439506046611,0.));
#248820=CARTESIAN_POINT('Ctrl Pts',(12.1377267537141,22.6591250653942,0.));
#248821=CARTESIAN_POINT('Ctrl Pts',(12.1609972423088,22.6742859034891,0.));
#248822=CARTESIAN_POINT('Ctrl Pts',(12.1843606579246,22.6894326204959,0.));
#248823=CARTESIAN_POINT('Ctrl Pts',(12.2078167360267,22.7045647168659,0.));
#248824=CARTESIAN_POINT('Ctrl Pts',(12.2313652198047,22.7196817119299,0.));
#248825=CARTESIAN_POINT('Ctrl Pts',(12.2550058702389,22.7347831655251,0.));
#248826=CARTESIAN_POINT('Ctrl Pts',(12.2787384750747,22.7498686970096,0.));
#248827=CARTESIAN_POINT('Ctrl Pts',(12.3025628601811,22.7649380101154,0.));
#248828=CARTESIAN_POINT('Ctrl Pts',(12.3264788926108,22.7799908974947,0.));
#248829=CARTESIAN_POINT('Ctrl Pts',(12.3504864740361,22.7950272216959,0.));
#248830=CARTESIAN_POINT('Ctrl Pts',(12.3745855366772,22.8100469022632,0.));
#248831=CARTESIAN_POINT('Ctrl Pts',(12.393937937903,22.8220493007353,0.));
#248832=CARTESIAN_POINT('Ctrl Pts',(12.4084933766366,22.8310435872852,0.));
#248833=CARTESIAN_POINT('Ctrl Pts',(12.4182152851867,22.8370364396497,0.));
#248834=CARTESIAN_POINT('Ctrl Pts',(12.4230808101438,22.8400320311648,0.));
#248835=CARTESIAN_POINT('',(12.4230808101438,22.8400320311648,12.));
#248836=CARTESIAN_POINT('Ctrl Pts',(12.4230808101438,22.8400320311648,12.));
#248837=CARTESIAN_POINT('Ctrl Pts',(12.4182152851867,22.8370364396497,12.));
#248838=CARTESIAN_POINT('Ctrl Pts',(12.4084933766366,22.8310435872852,12.));
#248839=CARTESIAN_POINT('Ctrl Pts',(12.393937937903,22.8220493007353,12.));
#248840=CARTESIAN_POINT('Ctrl Pts',(12.3745855366772,22.8100469022632,12.));
#248841=CARTESIAN_POINT('Ctrl Pts',(12.3504864740361,22.7950272216959,12.));
#248842=CARTESIAN_POINT('Ctrl Pts',(12.3264788926108,22.7799908974947,12.));
#248843=CARTESIAN_POINT('Ctrl Pts',(12.3025628601811,22.7649380101154,12.));
#248844=CARTESIAN_POINT('Ctrl Pts',(12.2787384750747,22.7498686970096,12.));
#248845=CARTESIAN_POINT('Ctrl Pts',(12.2550058702389,22.7347831655251,12.));
#248846=CARTESIAN_POINT('Ctrl Pts',(12.2313652198047,22.7196817119299,12.));
#248847=CARTESIAN_POINT('Ctrl Pts',(12.2078167360267,22.7045647168659,12.));
#248848=CARTESIAN_POINT('Ctrl Pts',(12.1843606579246,22.6894326204959,12.));
#248849=CARTESIAN_POINT('Ctrl Pts',(12.1609972423088,22.6742859034891,12.));
#248850=CARTESIAN_POINT('Ctrl Pts',(12.1377267537141,22.6591250653942,12.));
#248851=CARTESIAN_POINT('Ctrl Pts',(12.1145494550384,22.6439506046611,12.));
#248852=CARTESIAN_POINT('Ctrl Pts',(12.0914655972828,22.628762996708,12.));
#248853=CARTESIAN_POINT('Ctrl Pts',(12.0684754113869,22.613562676493,12.));
#248854=CARTESIAN_POINT('Ctrl Pts',(12.0455791139135,22.5983500505675,12.));
#248855=CARTESIAN_POINT('Ctrl Pts',(12.0227769113132,22.5831255061306,12.));
#248856=CARTESIAN_POINT('Ctrl Pts',(12.0000690046697,22.5678894211194,12.));
#248857=CARTESIAN_POINT('Ctrl Pts',(11.9774555943496,22.5526421741159,12.));
#248858=CARTESIAN_POINT('Ctrl Pts',(11.9549368843996,22.5373841537299,12.));
#248859=CARTESIAN_POINT('Ctrl Pts',(11.9325130877801,22.5221157697869,12.));
#248860=CARTESIAN_POINT('Ctrl Pts',(11.9101844254555,22.5068374513958,12.));
#248861=CARTESIAN_POINT('Ctrl Pts',(11.8879511239941,22.4915496418472,12.));
#248862=CARTESIAN_POINT('Ctrl Pts',(11.8658134137018,22.4762527946694,12.));
#248863=CARTESIAN_POINT('Ctrl Pts',(11.8437715264487,22.4609473690469,12.));
#248864=CARTESIAN_POINT('Ctrl Pts',(11.8218256937889,22.4456338258738,12.));
#248865=CARTESIAN_POINT('Ctrl Pts',(11.7999761445175,22.4303126226468,12.));
#248866=CARTESIAN_POINT('Ctrl Pts',(11.7782231042041,22.4149842125018,12.));
#248867=CARTESIAN_POINT('Ctrl Pts',(11.7565667964765,22.39964904692,12.));
#248868=CARTESIAN_POINT('Ctrl Pts',(11.7350074437961,22.3843075773905,12.));
#248869=CARTESIAN_POINT('Ctrl Pts',(11.7135452684532,22.3689602575492,12.));
#248870=CARTESIAN_POINT('Ctrl Pts',(11.6921804934056,22.3536075450028,12.));
#248871=CARTESIAN_POINT('Ctrl Pts',(11.6709133432986,22.3382499035618,12.));
#248872=CARTESIAN_POINT('Ctrl Pts',(11.6497440449858,22.3228878043976,12.));
#248873=CARTESIAN_POINT('Ctrl Pts',(11.6286728270011,22.3075217249049,12.));
#248874=CARTESIAN_POINT('Ctrl Pts',(11.6076999192359,22.2921521480358,12.));
#248875=CARTESIAN_POINT('Ctrl Pts',(11.5868255525189,22.2767795614349,12.));
#248876=CARTESIAN_POINT('Ctrl Pts',(11.5660499582403,22.2614044566898,12.));
#248877=CARTESIAN_POINT('Ctrl Pts',(11.545373367912,22.2460273284653,12.));
#248878=CARTESIAN_POINT('Ctrl Pts',(11.5247960128476,22.2306486738899,12.));
#248879=CARTESIAN_POINT('Ctrl Pts',(11.504318124424,22.215268993102,12.));
#248880=CARTESIAN_POINT('Ctrl Pts',(11.4839399342589,22.1998887896435,12.));
#248881=CARTESIAN_POINT('Ctrl Pts',(11.463661674411,22.184508570917,12.));
#248882=CARTESIAN_POINT('Ctrl Pts',(11.443483577557,22.1691288486096,12.));
#248883=CARTESIAN_POINT('Ctrl Pts',(11.4234058771742,22.1537501391486,12.));
#248884=CARTESIAN_POINT('Ctrl Pts',(11.4034288076908,22.1383729640963,12.));
#248885=CARTESIAN_POINT('Ctrl Pts',(11.3835526044256,22.1229978500185,12.));
#248886=CARTESIAN_POINT('Ctrl Pts',(11.3637775035367,22.1076253283978,12.));
#248887=CARTESIAN_POINT('Ctrl Pts',(11.3441037419553,22.0922559355293,12.));
#248888=CARTESIAN_POINT('Ctrl Pts',(11.3245315573168,22.0768902124267,12.));
#248889=CARTESIAN_POINT('Ctrl Pts',(11.3050611878771,22.0615287047179,12.));
#248890=CARTESIAN_POINT('Ctrl Pts',(11.2856928724374,22.0461719625661,12.));
#248891=CARTESIAN_POINT('Ctrl Pts',(11.2664268504207,22.0308205408351,12.));
#248892=CARTESIAN_POINT('Ctrl Pts',(11.2472633619276,22.0154749992364,12.));
#248893=CARTESIAN_POINT('Ctrl Pts',(11.2282026477897,22.000135902484,12.));
#248894=CARTESIAN_POINT('Ctrl Pts',(11.2092449496125,21.9848038204439,12.));
#248895=CARTESIAN_POINT('Ctrl Pts',(11.1903905098109,21.9694793282913,12.));
#248896=CARTESIAN_POINT('Ctrl Pts',(11.1716395716375,21.9541630066504,12.));
#248897=CARTESIAN_POINT('Ctrl Pts',(11.1529923792002,21.9388554416437,12.));
#248898=CARTESIAN_POINT('Ctrl Pts',(11.134449177474,21.9235572249518,12.));
#248899=CARTESIAN_POINT('Ctrl Pts',(11.1160102123024,21.9082689538687,12.));
#248900=CARTESIAN_POINT('Ctrl Pts',(11.0976757303944,21.8929912313608,12.));
#248901=CARTESIAN_POINT('Ctrl Pts',(11.0794459793058,21.8777246661191,12.));
#248902=CARTESIAN_POINT('Ctrl Pts',(11.0613212074364,21.8624698726319,12.));
#248903=CARTESIAN_POINT('Ctrl Pts',(11.0433016640808,21.8472274713103,12.));
#248904=CARTESIAN_POINT('Ctrl Pts',(11.0253875994598,21.8319980886033,12.));
#248905=CARTESIAN_POINT('Ctrl Pts',(11.0075792647477,21.8167823571168,12.));
#248906=CARTESIAN_POINT('Ctrl Pts',(10.9898769120913,21.8015809157302,12.));
#248907=CARTESIAN_POINT('Ctrl Pts',(10.9722807946157,21.7863944097143,12.));
#248908=CARTESIAN_POINT('Ctrl Pts',(10.9547911664457,21.7712234908468,12.));
#248909=CARTESIAN_POINT('Ctrl Pts',(10.9374082827446,21.7560688175252,12.));
#248910=CARTESIAN_POINT('Ctrl Pts',(10.9201323997386,21.74093105488,12.));
#248911=CARTESIAN_POINT('Ctrl Pts',(10.9029637747341,21.7258108748874,12.));
#248912=CARTESIAN_POINT('Ctrl Pts',(10.8859026661292,21.7107089564822,12.));
#248913=CARTESIAN_POINT('Ctrl Pts',(10.8689493334093,21.6956259856667,12.));
#248914=CARTESIAN_POINT('Ctrl Pts',(10.8521040371832,21.6805626556461,12.));
#248915=CARTESIAN_POINT('Ctrl Pts',(10.835367039227,21.6655196669727,12.));
#248916=CARTESIAN_POINT('Ctrl Pts',(10.8187386025135,21.6504977276864,12.));
#248917=CARTESIAN_POINT('Ctrl Pts',(10.8022189912369,21.6354975534558,12.));
#248918=CARTESIAN_POINT('Ctrl Pts',(10.7858084708262,21.6205198677176,12.));
#248919=CARTESIAN_POINT('Ctrl Pts',(10.7695073079554,21.6055654018179,12.));
#248920=CARTESIAN_POINT('Ctrl Pts',(10.7533157705943,21.5906348951745,12.));
#248921=CARTESIAN_POINT('Ctrl Pts',(10.7372341280468,21.5757290954372,12.));
#248922=CARTESIAN_POINT('Ctrl Pts',(10.7212626509816,21.5608487586467,12.));
#248923=CARTESIAN_POINT('Ctrl Pts',(10.7054016114571,21.5459946493955,12.));
#248924=CARTESIAN_POINT('Ctrl Pts',(10.689651282929,21.531167540981,12.));
#248925=CARTESIAN_POINT('Ctrl Pts',(10.6740119402835,21.5163682155805,12.));
#248926=CARTESIAN_POINT('Ctrl Pts',(10.658483859894,21.5015974644454,12.));
#248927=CARTESIAN_POINT('Ctrl Pts',(10.6430673196609,21.4868560880893,12.));
#248928=CARTESIAN_POINT('Ctrl Pts',(10.6277625990456,21.4721448964766,12.));
#248929=CARTESIAN_POINT('Ctrl Pts',(10.612569979096,21.4574647092093,12.));
#248930=CARTESIAN_POINT('Ctrl Pts',(10.597489742462,21.4428163557137,12.));
#248931=CARTESIAN_POINT('Ctrl Pts',(10.582522173457,21.4282006754624,12.));
#248932=CARTESIAN_POINT('Ctrl Pts',(10.5676675581106,21.4136185181974,12.));
#248933=CARTESIAN_POINT('Ctrl Pts',(10.5529261842107,21.3990707441495,12.));
#248934=CARTESIAN_POINT('Ctrl Pts',(10.5382983413422,21.3845582242604,12.));
#248935=CARTESIAN_POINT('Ctrl Pts',(10.523784320906,21.3700818403942,12.));
#248936=CARTESIAN_POINT('Ctrl Pts',(10.5093844161689,21.3556424855822,12.));
#248937=CARTESIAN_POINT('Ctrl Pts',(10.4950989223341,21.3412410642912,12.));
#248938=CARTESIAN_POINT('Ctrl Pts',(10.4809281365933,21.3268784926823,12.));
#248939=CARTESIAN_POINT('Ctrl Pts',(10.4668723581768,21.312555698873,12.));
#248940=CARTESIAN_POINT('Ctrl Pts',(10.452931888387,21.2982736231924,12.));
#248941=CARTESIAN_POINT('Ctrl Pts',(10.4391070306385,21.2840332184471,12.));
#248942=CARTESIAN_POINT('Ctrl Pts',(10.4253980905394,21.2698354502391,12.));
#248943=CARTESIAN_POINT('Ctrl Pts',(10.4118053759584,21.2556812972741,12.));
#248944=CARTESIAN_POINT('Ctrl Pts',(10.3983291970846,21.2415717516713,12.));
#248945=CARTESIAN_POINT('Ctrl Pts',(10.384969866479,21.2275078192708,12.));
#248946=CARTESIAN_POINT('Ctrl Pts',(10.3717276991137,21.2134905199359,12.));
#248947=CARTESIAN_POINT('Ctrl Pts',(10.3586030124595,21.1995208879205,12.));
#248948=CARTESIAN_POINT('Ctrl Pts',(10.3455961265706,21.1855999722427,12.));
#248949=CARTESIAN_POINT('Ctrl Pts',(10.3327073641574,21.1717288370512,12.));
#248950=CARTESIAN_POINT('Ctrl Pts',(10.3199370506541,21.1579085619959,12.));
#248951=CARTESIAN_POINT('Ctrl Pts',(10.307285514268,21.1441402425831,12.));
#248952=CARTESIAN_POINT('Ctrl Pts',(10.2947530860714,21.130424990599,12.));
#248953=CARTESIAN_POINT('Ctrl Pts',(10.2823401001067,21.1167639345623,12.));
#248954=CARTESIAN_POINT('Ctrl Pts',(10.2700468934743,21.1031582201625,12.));
#248955=CARTESIAN_POINT('Ctrl Pts',(10.2578738064183,21.0896090107066,12.));
#248956=CARTESIAN_POINT('Ctrl Pts',(10.2458211823915,21.0761174875448,12.));
#248957=CARTESIAN_POINT('Ctrl Pts',(10.233889368157,21.0626848505665,12.));
#248958=CARTESIAN_POINT('Ctrl Pts',(10.2220787139157,21.0493123187484,12.));
#248959=CARTESIAN_POINT('Ctrl Pts',(10.2103895734123,21.0360011306814,12.));
#248960=CARTESIAN_POINT('Ctrl Pts',(10.1988223040425,21.0227525451107,12.));
#248961=CARTESIAN_POINT('Ctrl Pts',(10.1873772669358,21.0095678414486,12.));
#248962=CARTESIAN_POINT('Ctrl Pts',(10.1760548270765,20.9964483203685,12.));
#248963=CARTESIAN_POINT('Ctrl Pts',(10.1648553534567,20.9833953044737,12.));
#248964=CARTESIAN_POINT('Ctrl Pts',(10.1537792192065,20.970410138937,12.));
#248965=CARTESIAN_POINT('Ctrl Pts',(10.1428268017257,20.9574941921591,12.));
#248966=CARTESIAN_POINT('Ctrl Pts',(10.1319984827909,20.944648856393,12.));
#248967=CARTESIAN_POINT('Ctrl Pts',(10.1212946487057,20.931875548473,12.));
#248968=CARTESIAN_POINT('Ctrl Pts',(10.1107156904836,20.9191757106266,12.));
#248969=CARTESIAN_POINT('Ctrl Pts',(10.1002620040076,20.9065508112556,12.));
#248970=CARTESIAN_POINT('Ctrl Pts',(10.0899339901916,20.8940023457371,12.));
#248971=CARTESIAN_POINT('Ctrl Pts',(10.0797320551154,20.8815318371844,12.));
#248972=CARTESIAN_POINT('Ctrl Pts',(10.0696566102219,20.8691408373705,12.));
#248973=CARTESIAN_POINT('Ctrl Pts',(10.0597080725375,20.856830927732,12.));
#248974=CARTESIAN_POINT('Ctrl Pts',(10.0498868648733,20.8446037203402,12.));
#248975=CARTESIAN_POINT('Ctrl Pts',(10.0401934160234,20.8324608588906,12.));
#248976=CARTESIAN_POINT('Ctrl Pts',(10.0306281609435,20.8204040196599,12.));
#248977=CARTESIAN_POINT('Ctrl Pts',(10.0211915410095,20.8084349126885,12.));
#248978=CARTESIAN_POINT('Ctrl Pts',(10.0118840042786,20.7965552829907,12.));
#248979=CARTESIAN_POINT('Ctrl Pts',(10.0027060057389,20.7847669117568,12.));
#248980=CARTESIAN_POINT('Ctrl Pts',(9.99365800754637,20.7730716175417,12.));
#248981=CARTESIAN_POINT('Ctrl Pts',(9.98474047926846,20.7614712574989,12.));
#248982=CARTESIAN_POINT('Ctrl Pts',(9.97595389823461,20.7499677289626,12.));
#248983=CARTESIAN_POINT('Ctrl Pts',(9.96729874986198,20.7385629709795,12.));
#248984=CARTESIAN_POINT('Ctrl Pts',(9.95877552798403,20.7272589658752,12.));
#248985=CARTESIAN_POINT('Ctrl Pts',(9.95038473514962,20.7160577407581,12.));
#248986=CARTESIAN_POINT('Ctrl Pts',(9.9421268829825,20.7049613692237,12.));
#248987=CARTESIAN_POINT('Ctrl Pts',(9.93400249259736,20.6939719732485,12.));
#248988=CARTESIAN_POINT('Ctrl Pts',(9.9260120949875,20.6830917250255,12.));
#248989=CARTESIAN_POINT('Ctrl Pts',(9.91815623141284,20.6723228488262,12.));
#248990=CARTESIAN_POINT('Ctrl Pts',(9.91043545377004,20.6616676228315,12.));
#248991=CARTESIAN_POINT('Ctrl Pts',(9.90285032516695,20.6511283817415,12.));
#248992=CARTESIAN_POINT('Ctrl Pts',(9.89540142049123,20.6407075193977,12.));
#248993=CARTESIAN_POINT('Ctrl Pts',(9.88808932697304,20.6304074914086,12.));
#248994=CARTESIAN_POINT('Ctrl Pts',(9.88091464472669,20.6202308177472,12.));
#248995=CARTESIAN_POINT('Ctrl Pts',(9.87387798732943,20.6101800854491,12.));
#248996=CARTESIAN_POINT('Ctrl Pts',(9.86697998242612,20.6002579513696,12.));
#248997=CARTESIAN_POINT('Ctrl Pts',(9.86022127232749,20.5904671449755,12.));
#248998=CARTESIAN_POINT('Ctrl Pts',(9.85360251457004,20.580810471002,12.));
#248999=CARTESIAN_POINT('Ctrl Pts',(9.84712438256308,20.5712908125145,12.));
#249000=CARTESIAN_POINT('Ctrl Pts',(9.84078756677589,20.5619111362406,12.));
#249001=CARTESIAN_POINT('Ctrl Pts',(9.8345927758532,20.5526744976461,12.));
#249002=CARTESIAN_POINT('Ctrl Pts',(9.82854073773857,20.5435840460717,12.));
#249003=CARTESIAN_POINT('Ctrl Pts',(9.82263220080327,20.534643029951,12.));
#249004=CARTESIAN_POINT('Ctrl Pts',(9.81686793455918,20.5258548000625,12.));
#249005=CARTESIAN_POINT('Ctrl Pts',(9.81124873025278,20.5172228122839,12.));
#249006=CARTESIAN_POINT('Ctrl Pts',(9.80577540161102,20.5087506310507,12.));
#249007=CARTESIAN_POINT('Ctrl Pts',(9.80044878520967,20.500441931211,12.));
#249008=CARTESIAN_POINT('Ctrl Pts',(9.79526974288343,20.4923005087945,12.));
#249009=CARTESIAN_POINT('Ctrl Pts',(9.79023916498659,20.4843302955329,12.));
#249010=CARTESIAN_POINT('Ctrl Pts',(9.78535797314162,20.4765353711585,12.));
#249011=CARTESIAN_POINT('Ctrl Pts',(9.78062712373313,20.4689199790668,12.));
#249012=CARTESIAN_POINT('Ctrl Pts',(9.77604760815522,20.4614885274973,12.));
#249013=CARTESIAN_POINT('Ctrl Pts',(9.77162045104069,20.4542455817527,12.));
#249014=CARTESIAN_POINT('Ctrl Pts',(9.76734670980896,20.447195862298,12.));
#249015=CARTESIAN_POINT('Ctrl Pts',(9.76322747195502,20.4403442329401,12.));
#249016=CARTESIAN_POINT('Ctrl Pts',(9.75926386289929,20.4336957355474,12.));
#249017=CARTESIAN_POINT('Ctrl Pts',(9.75545705902416,20.4272556476629,12.));
#249018=CARTESIAN_POINT('Ctrl Pts',(9.75180829786433,20.4210295275818,12.));
#249019=CARTESIAN_POINT('Ctrl Pts',(9.74831889242174,20.4150232777393,12.));
#249020=CARTESIAN_POINT('Ctrl Pts',(9.74499021838536,20.4092430879861,12.));
#249021=CARTESIAN_POINT('Ctrl Pts',(9.74182369656272,20.4036953576549,12.));
#249022=CARTESIAN_POINT('Ctrl Pts',(9.73882077613206,20.3983866213331,12.));
#249023=CARTESIAN_POINT('Ctrl Pts',(9.73598292014249,20.3933234845646,12.));
#249024=CARTESIAN_POINT('Ctrl Pts',(9.73331167102812,20.3885129129912,12.));
#249025=CARTESIAN_POINT('Ctrl Pts',(9.73080870123726,20.3839624556742,12.));
#249026=CARTESIAN_POINT('Ctrl Pts',(9.72847589116532,20.3796805893304,12.));
#249027=CARTESIAN_POINT('Ctrl Pts',(9.7263153173287,20.3756766651952,12.));
#249028=CARTESIAN_POINT('Ctrl Pts',(9.72432910043192,20.371960235676,12.));
#249029=CARTESIAN_POINT('Ctrl Pts',(9.72251930722503,20.3685406190576,12.));
#249030=CARTESIAN_POINT('Ctrl Pts',(9.72088778381101,20.3654261611055,12.));
#249031=CARTESIAN_POINT('Ctrl Pts',(9.71943648548114,20.362625691398,12.));
#249032=CARTESIAN_POINT('Ctrl Pts',(9.71816778327998,20.3601498764344,12.));
#249033=CARTESIAN_POINT('Ctrl Pts',(9.71708493723061,20.3580133103357,12.));
#249034=CARTESIAN_POINT('Ctrl Pts',(9.71619192554146,20.3562337557875,12.));
#249035=CARTESIAN_POINT('Ctrl Pts',(9.71549257088174,20.3548282742361,12.));
#249036=CARTESIAN_POINT('Ctrl Pts',(9.714989780521,20.3538098605706,12.));
#249037=CARTESIAN_POINT('Ctrl Pts',(9.71474590350791,20.3533097561886,12.));
#249038=CARTESIAN_POINT('Ctrl Pts',(9.71465227853122,20.3531126095522,12.));
#249039=CARTESIAN_POINT('Ctrl Pts',(9.71462954053074,20.353060251684,12.));
#249040=CARTESIAN_POINT('Ctrl Pts',(9.71462809124917,20.353053841303,12.));
#249041=CARTESIAN_POINT('',(12.4230808101438,22.8400320311648,0.));
#249042=CARTESIAN_POINT('Origin',(13.9675290154577,16.3449727195352,0.));
#249043=CARTESIAN_POINT('',(14.6513681262571,17.1452095830633,12.));
#249044=CARTESIAN_POINT('',(6.98376450772883,8.17248635976757,12.));
#249045=CARTESIAN_POINT('',(14.6513681262571,17.1452095830633,0.));
#249046=CARTESIAN_POINT('',(14.6513681262571,17.1452095830633,0.));
#249047=CARTESIAN_POINT('',(6.98376450772883,8.17248635976757,0.));
#249048=CARTESIAN_POINT('Ctrl Pts',(13.5685075571671,22.1787195904339,0.));
#249049=CARTESIAN_POINT('Ctrl Pts',(13.5685075571671,22.1787195904339,12.));
#249050=CARTESIAN_POINT('Ctrl Pts',(13.5683460612913,22.1730081264583,0.));
#249051=CARTESIAN_POINT('Ctrl Pts',(13.5683460612913,22.1730081264583,12.));
#249052=CARTESIAN_POINT('Ctrl Pts',(13.5680170531724,22.1615922804939,0.));
#249053=CARTESIAN_POINT('Ctrl Pts',(13.5680170531724,22.1615922804939,12.));
#249054=CARTESIAN_POINT('Ctrl Pts',(13.5675054918922,22.1444897575076,0.));
#249055=CARTESIAN_POINT('Ctrl Pts',(13.5675054918922,22.1444897575076,12.));
#249056=CARTESIAN_POINT('Ctrl Pts',(13.5667873105179,22.1217288871823,0.));
#249057=CARTESIAN_POINT('Ctrl Pts',(13.5667873105179,22.1217288871823,12.));
#249058=CARTESIAN_POINT('Ctrl Pts',(13.5658294169106,22.0933486464442,0.));
#249059=CARTESIAN_POINT('Ctrl Pts',(13.5658294169106,22.0933486464442,12.));
#249060=CARTESIAN_POINT('Ctrl Pts',(13.5648113688894,22.0650393089492,0.));
#249061=CARTESIAN_POINT('Ctrl Pts',(13.5648113688894,22.0650393089492,12.));
#249062=CARTESIAN_POINT('Ctrl Pts',(13.5637332022393,22.0368009736227,0.));
#249063=CARTESIAN_POINT('Ctrl Pts',(13.5637332022393,22.0368009736227,12.));
#249064=CARTESIAN_POINT('Ctrl Pts',(13.5625949868313,22.0086337943431,0.));
#249065=CARTESIAN_POINT('Ctrl Pts',(13.5625949868313,22.0086337943431,12.));
#249066=CARTESIAN_POINT('Ctrl Pts',(13.5613968357589,21.9805379899192,0.));
#249067=CARTESIAN_POINT('Ctrl Pts',(13.5613968357589,21.9805379899192,12.));
#249068=CARTESIAN_POINT('Ctrl Pts',(13.5601389185315,21.9525138592862,0.));
#249069=CARTESIAN_POINT('Ctrl Pts',(13.5601389185315,21.9525138592862,12.));
#249070=CARTESIAN_POINT('Ctrl Pts',(13.5588214586672,21.9245617765827,0.));
#249071=CARTESIAN_POINT('Ctrl Pts',(13.5588214586672,21.9245617765827,12.));
#249072=CARTESIAN_POINT('Ctrl Pts',(13.5574447178484,21.8966821688876,0.));
#249073=CARTESIAN_POINT('Ctrl Pts',(13.5574447178484,21.8966821688876,12.));
#249074=CARTESIAN_POINT('Ctrl Pts',(13.5560089839426,21.8688754989401,0.));
#249075=CARTESIAN_POINT('Ctrl Pts',(13.5560089839426,21.8688754989401,12.));
#249076=CARTESIAN_POINT('Ctrl Pts',(13.5545145573048,21.841142245609,0.));
#249077=CARTESIAN_POINT('Ctrl Pts',(13.5545145573048,21.841142245609,12.));
#249078=CARTESIAN_POINT('Ctrl Pts',(13.5529617381569,21.8134828857963,0.));
#249079=CARTESIAN_POINT('Ctrl Pts',(13.5529617381569,21.8134828857963,12.));
#249080=CARTESIAN_POINT('Ctrl Pts',(13.5513508127232,21.7858978745848,0.));
#249081=CARTESIAN_POINT('Ctrl Pts',(13.5513508127232,21.7858978745848,12.));
#249082=CARTESIAN_POINT('Ctrl Pts',(13.5496820422186,21.7583876294532,0.));
#249083=CARTESIAN_POINT('Ctrl Pts',(13.5496820422186,21.7583876294532,12.));
#249084=CARTESIAN_POINT('Ctrl Pts',(13.5479556704457,21.730952541226,0.));
#249085=CARTESIAN_POINT('Ctrl Pts',(13.5479556704457,21.730952541226,12.));
#249086=CARTESIAN_POINT('Ctrl Pts',(13.546171929503,21.7035929822939,0.));
#249087=CARTESIAN_POINT('Ctrl Pts',(13.546171929503,21.7035929822939,12.));
#249088=CARTESIAN_POINT('Ctrl Pts',(13.5443310461516,21.676309315769,0.));
#249089=CARTESIAN_POINT('Ctrl Pts',(13.5443310461516,21.676309315769,12.));
#249090=CARTESIAN_POINT('Ctrl Pts',(13.5424332480698,21.6491019044647,0.));
#249091=CARTESIAN_POINT('Ctrl Pts',(13.5424332480698,21.6491019044647,12.));
#249092=CARTESIAN_POINT('Ctrl Pts',(13.5404787697798,21.6219711193951,0.));
#249093=CARTESIAN_POINT('Ctrl Pts',(13.5404787697798,21.6219711193951,12.));
#249094=CARTESIAN_POINT('Ctrl Pts',(13.5384678597206,21.5949173499022,0.));
#249095=CARTESIAN_POINT('Ctrl Pts',(13.5384678597206,21.5949173499022,12.));
#249096=CARTESIAN_POINT('Ctrl Pts',(13.5364007790292,21.5679410019011,0.));
#249097=CARTESIAN_POINT('Ctrl Pts',(13.5364007790292,21.5679410019011,12.));
#249098=CARTESIAN_POINT('Ctrl Pts',(13.5342777983225,21.5410424932511,0.));
#249099=CARTESIAN_POINT('Ctrl Pts',(13.5342777983225,21.5410424932511,12.));
#249100=CARTESIAN_POINT('Ctrl Pts',(13.5320991952145,21.5142222501671,0.));
#249101=CARTESIAN_POINT('Ctrl Pts',(13.5320991952145,21.5142222501671,12.));
#249102=CARTESIAN_POINT('Ctrl Pts',(13.5298652514357,21.487480703047,0.));
#249103=CARTESIAN_POINT('Ctrl Pts',(13.5298652514357,21.487480703047,12.));
#249104=CARTESIAN_POINT('Ctrl Pts',(13.5275762503553,21.4608182828695,0.));
#249105=CARTESIAN_POINT('Ctrl Pts',(13.5275762503553,21.4608182828695,12.));
#249106=CARTESIAN_POINT('Ctrl Pts',(13.5252324737795,21.4342354165254,0.));
#249107=CARTESIAN_POINT('Ctrl Pts',(13.5252324737795,21.4342354165254,12.));
#249108=CARTESIAN_POINT('Ctrl Pts',(13.5228342013508,21.4077325259318,0.));
#249109=CARTESIAN_POINT('Ctrl Pts',(13.5228342013508,21.4077325259318,12.));
#249110=CARTESIAN_POINT('Ctrl Pts',(13.5203817122496,21.3813100304967,0.));
#249111=CARTESIAN_POINT('Ctrl Pts',(13.5203817122496,21.3813100304967,12.));
#249112=CARTESIAN_POINT('Ctrl Pts',(13.5178752862461,21.3549683486219,0.));
#249113=CARTESIAN_POINT('Ctrl Pts',(13.5178752862461,21.3549683486219,12.));
#249114=CARTESIAN_POINT('Ctrl Pts',(13.5153152050554,21.328707899634,0.));
#249115=CARTESIAN_POINT('Ctrl Pts',(13.5153152050554,21.328707899634,12.));
#249116=CARTESIAN_POINT('Ctrl Pts',(13.5127017534972,21.3025291054236,0.));
#249117=CARTESIAN_POINT('Ctrl Pts',(13.5127017534972,21.3025291054236,12.));
#249118=CARTESIAN_POINT('Ctrl Pts',(13.5100352209207,21.2764323924442,0.));
#249119=CARTESIAN_POINT('Ctrl Pts',(13.5100352209207,21.2764323924442,12.));
#249120=CARTESIAN_POINT('Ctrl Pts',(13.5073159019454,21.2504181927429,0.));
#249121=CARTESIAN_POINT('Ctrl Pts',(13.5073159019454,21.2504181927429,12.));
#249122=CARTESIAN_POINT('Ctrl Pts',(13.5045440957404,21.224486942933,0.));
#249123=CARTESIAN_POINT('Ctrl Pts',(13.5045440957404,21.224486942933,12.));
#249124=CARTESIAN_POINT('Ctrl Pts',(13.5017201056088,21.1986390835825,0.));
#249125=CARTESIAN_POINT('Ctrl Pts',(13.5017201056088,21.1986390835825,12.));
#249126=CARTESIAN_POINT('Ctrl Pts',(13.4988442384491,21.1728750584173,0.));
#249127=CARTESIAN_POINT('Ctrl Pts',(13.4988442384491,21.1728750584173,12.));
#249128=CARTESIAN_POINT('Ctrl Pts',(13.4959168042934,21.1471953136209,0.));
#249129=CARTESIAN_POINT('Ctrl Pts',(13.4959168042934,21.1471953136209,12.));
#249130=CARTESIAN_POINT('Ctrl Pts',(13.4929381157778,21.1216002970209,0.));
#249131=CARTESIAN_POINT('Ctrl Pts',(13.4929381157778,21.1216002970209,12.));
#249132=CARTESIAN_POINT('Ctrl Pts',(13.4899084877718,21.0960904575048,0.));
#249133=CARTESIAN_POINT('Ctrl Pts',(13.4899084877718,21.0960904575048,12.));
#249134=CARTESIAN_POINT('Ctrl Pts',(13.4868282377191,21.0706662455202,0.));
#249135=CARTESIAN_POINT('Ctrl Pts',(13.4868282377191,21.0706662455202,12.));
#249136=CARTESIAN_POINT('Ctrl Pts',(13.4836976858912,21.0453281134247,0.));
#249137=CARTESIAN_POINT('Ctrl Pts',(13.4836976858912,21.0453281134247,12.));
#249138=CARTESIAN_POINT('Ctrl Pts',(13.4805171556822,21.0200765158885,0.));
#249139=CARTESIAN_POINT('Ctrl Pts',(13.4805171556822,21.0200765158885,12.));
#249140=CARTESIAN_POINT('Ctrl Pts',(13.4772869738879,20.9949119102592,0.));
#249141=CARTESIAN_POINT('Ctrl Pts',(13.4772869738879,20.9949119102592,12.));
#249142=CARTESIAN_POINT('Ctrl Pts',(13.4740074710087,20.9698347569476,0.));
#249143=CARTESIAN_POINT('Ctrl Pts',(13.4740074710087,20.9698347569476,12.));
#249144=CARTESIAN_POINT('Ctrl Pts',(13.4706789815166,20.9448455197557,0.));
#249145=CARTESIAN_POINT('Ctrl Pts',(13.4706789815166,20.9448455197557,12.));
#249146=CARTESIAN_POINT('Ctrl Pts',(13.4673018437718,20.9199446657584,0.));
#249147=CARTESIAN_POINT('Ctrl Pts',(13.4673018437718,20.9199446657584,12.));
#249148=CARTESIAN_POINT('Ctrl Pts',(13.4638763999725,20.8951326652158,0.));
#249149=CARTESIAN_POINT('Ctrl Pts',(13.4638763999725,20.8951326652158,12.));
#249150=CARTESIAN_POINT('Ctrl Pts',(13.4604029960983,20.8704099914641,0.));
#249151=CARTESIAN_POINT('Ctrl Pts',(13.4604029960983,20.8704099914641,12.));
#249152=CARTESIAN_POINT('Ctrl Pts',(13.4568819818631,20.8457771208082,0.));
#249153=CARTESIAN_POINT('Ctrl Pts',(13.4568819818631,20.8457771208082,12.));
#249154=CARTESIAN_POINT('Ctrl Pts',(13.4533137106667,20.821234532398,0.));
#249155=CARTESIAN_POINT('Ctrl Pts',(13.4533137106667,20.821234532398,12.));
#249156=CARTESIAN_POINT('Ctrl Pts',(13.4496985395637,20.7967827081227,0.));
#249157=CARTESIAN_POINT('Ctrl Pts',(13.4496985395637,20.7967827081227,12.));
#249158=CARTESIAN_POINT('Ctrl Pts',(13.4460368293688,20.7724221327608,0.));
#249159=CARTESIAN_POINT('Ctrl Pts',(13.4460368293688,20.7724221327608,12.));
#249160=CARTESIAN_POINT('Ctrl Pts',(13.4423289447561,20.7481532941013,0.));
#249161=CARTESIAN_POINT('Ctrl Pts',(13.4423289447561,20.7481532941013,12.));
#249162=CARTESIAN_POINT('Ctrl Pts',(13.4385752543663,20.7239766830675,0.));
#249163=CARTESIAN_POINT('Ctrl Pts',(13.4385752543663,20.7239766830675,12.));
#249164=CARTESIAN_POINT('Ctrl Pts',(13.4347761309154,20.6998927938288,0.));
#249165=CARTESIAN_POINT('Ctrl Pts',(13.4347761309154,20.6998927938288,12.));
#249166=CARTESIAN_POINT('Ctrl Pts',(13.4309319513119,20.6759021239103,0.));
#249167=CARTESIAN_POINT('Ctrl Pts',(13.4309319513119,20.6759021239103,12.));
#249168=CARTESIAN_POINT('Ctrl Pts',(13.4270430967651,20.6520051742869,0.));
#249169=CARTESIAN_POINT('Ctrl Pts',(13.4270430967651,20.6520051742869,12.));
#249170=CARTESIAN_POINT('Ctrl Pts',(13.4231099528179,20.6282024494237,0.));
#249171=CARTESIAN_POINT('Ctrl Pts',(13.4231099528179,20.6282024494237,12.));
#249172=CARTESIAN_POINT('Ctrl Pts',(13.4191329093932,20.6044944573153,0.));
#249173=CARTESIAN_POINT('Ctrl Pts',(13.4191329093932,20.6044944573153,12.));
#249174=CARTESIAN_POINT('Ctrl Pts',(13.4151123608411,20.5808817095155,0.));
#249175=CARTESIAN_POINT('Ctrl Pts',(13.4151123608411,20.5808817095155,12.));
#249176=CARTESIAN_POINT('Ctrl Pts',(13.4110487059912,20.5573647211639,0.));
#249177=CARTESIAN_POINT('Ctrl Pts',(13.4110487059912,20.5573647211639,12.));
#249178=CARTESIAN_POINT('Ctrl Pts',(13.4069423482076,20.5339440109956,0.));
#249179=CARTESIAN_POINT('Ctrl Pts',(13.4069423482076,20.5339440109956,12.));
#249180=CARTESIAN_POINT('Ctrl Pts',(13.4027936954529,20.5106201013753,0.));
#249181=CARTESIAN_POINT('Ctrl Pts',(13.4027936954529,20.5106201013753,12.));
#249182=CARTESIAN_POINT('Ctrl Pts',(13.3986031603716,20.487393518404,0.));
#249183=CARTESIAN_POINT('Ctrl Pts',(13.3986031603716,20.487393518404,12.));
#249184=CARTESIAN_POINT('Ctrl Pts',(13.3943711603739,20.4642647920038,0.));
#249185=CARTESIAN_POINT('Ctrl Pts',(13.3943711603739,20.4642647920038,12.));
#249186=CARTESIAN_POINT('Ctrl Pts',(13.3900981177255,20.4412344560008,0.));
#249187=CARTESIAN_POINT('Ctrl Pts',(13.3900981177255,20.4412344560008,12.));
#249188=CARTESIAN_POINT('Ctrl Pts',(13.3857844596387,20.4183030482002,0.));
#249189=CARTESIAN_POINT('Ctrl Pts',(13.3857844596387,20.4183030482002,12.));
#249190=CARTESIAN_POINT('Ctrl Pts',(13.3814306183719,20.3954711104502,0.));
#249191=CARTESIAN_POINT('Ctrl Pts',(13.3814306183719,20.3954711104502,12.));
#249192=CARTESIAN_POINT('Ctrl Pts',(13.3770370313188,20.3727391887184,0.));
#249193=CARTESIAN_POINT('Ctrl Pts',(13.3770370313188,20.3727391887184,12.));
#249194=CARTESIAN_POINT('Ctrl Pts',(13.3726041410867,20.3501078331814,0.));
#249195=CARTESIAN_POINT('Ctrl Pts',(13.3726041410867,20.3501078331814,12.));
#249196=CARTESIAN_POINT('Ctrl Pts',(13.3681323955826,20.3275775983029,0.));
#249197=CARTESIAN_POINT('Ctrl Pts',(13.3681323955826,20.3275775983029,12.));
#249198=CARTESIAN_POINT('Ctrl Pts',(13.3636222481016,20.3051490429048,0.));
#249199=CARTESIAN_POINT('Ctrl Pts',(13.3636222481016,20.3051490429048,12.));
#249200=CARTESIAN_POINT('Ctrl Pts',(13.3590741574195,20.2828227302339,0.));
#249201=CARTESIAN_POINT('Ctrl Pts',(13.3590741574195,20.2828227302339,12.));
#249202=CARTESIAN_POINT('Ctrl Pts',(13.3544885878889,20.2605992280122,0.));
#249203=CARTESIAN_POINT('Ctrl Pts',(13.3544885878889,20.2605992280122,12.));
#249204=CARTESIAN_POINT('Ctrl Pts',(13.3498660095386,20.2384791085359,0.));
#249205=CARTESIAN_POINT('Ctrl Pts',(13.3498660095386,20.2384791085359,12.));
#249206=CARTESIAN_POINT('Ctrl Pts',(13.3452068981766,20.216462948786,0.));
#249207=CARTESIAN_POINT('Ctrl Pts',(13.3452068981766,20.216462948786,12.));
#249208=CARTESIAN_POINT('Ctrl Pts',(13.3405117354971,20.1945513305235,0.));
#249209=CARTESIAN_POINT('Ctrl Pts',(13.3405117354971,20.1945513305235,12.));
#249210=CARTESIAN_POINT('Ctrl Pts',(13.3357810091903,20.1727448403817,0.));
#249211=CARTESIAN_POINT('Ctrl Pts',(13.3357810091903,20.1727448403817,12.));
#249212=CARTESIAN_POINT('Ctrl Pts',(13.3310152130564,20.1510440699474,0.));
#249213=CARTESIAN_POINT('Ctrl Pts',(13.3310152130564,20.1510440699474,12.));
#249214=CARTESIAN_POINT('Ctrl Pts',(13.3262148471226,20.1294496158402,0.));
#249215=CARTESIAN_POINT('Ctrl Pts',(13.3262148471226,20.1294496158402,12.));
#249216=CARTESIAN_POINT('Ctrl Pts',(13.3213804177587,20.1079620798375,0.));
#249217=CARTESIAN_POINT('Ctrl Pts',(13.3213804177587,20.1079620798375,12.));
#249218=CARTESIAN_POINT('Ctrl Pts',(13.3165124377962,20.0865820689883,0.));
#249219=CARTESIAN_POINT('Ctrl Pts',(13.3165124377962,20.0865820689883,12.));
#249220=CARTESIAN_POINT('Ctrl Pts',(13.3116114266515,20.0653101957188,0.));
#249221=CARTESIAN_POINT('Ctrl Pts',(13.3116114266515,20.0653101957188,12.));
#249222=CARTESIAN_POINT('Ctrl Pts',(13.3066779104515,20.0441470779345,0.));
#249223=CARTESIAN_POINT('Ctrl Pts',(13.3066779104515,20.0441470779345,12.));
#249224=CARTESIAN_POINT('Ctrl Pts',(13.3017124221637,20.0230933391038,0.));
#249225=CARTESIAN_POINT('Ctrl Pts',(13.3017124221637,20.0230933391038,12.));
#249226=CARTESIAN_POINT('Ctrl Pts',(13.2967155017306,20.0021496083738,0.));
#249227=CARTESIAN_POINT('Ctrl Pts',(13.2967155017306,20.0021496083738,12.));
#249228=CARTESIAN_POINT('Ctrl Pts',(13.2916876962094,19.981316520717,0.));
#249229=CARTESIAN_POINT('Ctrl Pts',(13.2916876962094,19.981316520717,12.));
#249230=CARTESIAN_POINT('Ctrl Pts',(13.286629559915,19.9605947170586,0.));
#249231=CARTESIAN_POINT('Ctrl Pts',(13.286629559915,19.9605947170586,12.));
#249232=CARTESIAN_POINT('Ctrl Pts',(13.2815416545663,19.9399848444019,0.));
#249233=CARTESIAN_POINT('Ctrl Pts',(13.2815416545663,19.9399848444019,12.));
#249234=CARTESIAN_POINT('Ctrl Pts',(13.2764245494357,19.9194875559422,0.));
#249235=CARTESIAN_POINT('Ctrl Pts',(13.2764245494357,19.9194875559422,12.));
#249236=CARTESIAN_POINT('Ctrl Pts',(13.271278821502,19.8991035111745,0.));
#249237=CARTESIAN_POINT('Ctrl Pts',(13.271278821502,19.8991035111745,12.));
#249238=CARTESIAN_POINT('Ctrl Pts',(13.2661050556132,19.8788333760577,0.));
#249239=CARTESIAN_POINT('Ctrl Pts',(13.2661050556132,19.8788333760577,12.));
#249240=CARTESIAN_POINT('Ctrl Pts',(13.2609038446529,19.8586778231715,0.));
#249241=CARTESIAN_POINT('Ctrl Pts',(13.2609038446529,19.8586778231715,12.));
#249242=CARTESIAN_POINT('Ctrl Pts',(13.2556757897086,19.8386375318634,0.));
#249243=CARTESIAN_POINT('Ctrl Pts',(13.2556757897086,19.8386375318634,12.));
#249244=CARTESIAN_POINT('Ctrl Pts',(13.2504215002457,19.8187131883917,0.));
#249245=CARTESIAN_POINT('Ctrl Pts',(13.2504215002457,19.8187131883917,12.));
#249246=CARTESIAN_POINT('Ctrl Pts',(13.2451415942805,19.7989054860495,0.));
#249247=CARTESIAN_POINT('Ctrl Pts',(13.2451415942805,19.7989054860495,12.));
#249248=CARTESIAN_POINT('Ctrl Pts',(13.2398366985675,19.7792151253289,0.));
#249249=CARTESIAN_POINT('Ctrl Pts',(13.2398366985675,19.7792151253289,12.));
#249250=CARTESIAN_POINT('Ctrl Pts',(13.2345074487963,19.7596428141168,0.));
#249251=CARTESIAN_POINT('Ctrl Pts',(13.2345074487963,19.7596428141168,12.));
#249252=CARTESIAN_POINT('Ctrl Pts',(13.2291544897899,19.7401892678697,0.));
#249253=CARTESIAN_POINT('Ctrl Pts',(13.2291544897899,19.7401892678697,12.));
#249254=CARTESIAN_POINT('Ctrl Pts',(13.2237784757065,19.7208552097868,0.));
#249255=CARTESIAN_POINT('Ctrl Pts',(13.2237784757065,19.7208552097868,12.));
#249256=CARTESIAN_POINT('Ctrl Pts',(13.2183800702436,19.7016413709685,0.));
#249257=CARTESIAN_POINT('Ctrl Pts',(13.2183800702436,19.7016413709685,12.));
#249258=CARTESIAN_POINT('Ctrl Pts',(13.2129599468485,19.6825484905823,0.));
#249259=CARTESIAN_POINT('Ctrl Pts',(13.2129599468485,19.6825484905823,12.));
#249260=CARTESIAN_POINT('Ctrl Pts',(13.2075187889529,19.6635773160936,0.));
#249261=CARTESIAN_POINT('Ctrl Pts',(13.2075187889529,19.6635773160936,12.));
#249262=CARTESIAN_POINT('Ctrl Pts',(13.2020572902065,19.6447286034772,0.));
#249263=CARTESIAN_POINT('Ctrl Pts',(13.2020572902065,19.6447286034772,12.));
#249264=CARTESIAN_POINT('Ctrl Pts',(13.1965761547151,19.6260031174244,0.));
#249265=CARTESIAN_POINT('Ctrl Pts',(13.1965761547151,19.6260031174244,12.));
#249266=CARTESIAN_POINT('Ctrl Pts',(13.1910760972814,19.6074016315414,0.));
#249267=CARTESIAN_POINT('Ctrl Pts',(13.1910760972814,19.6074016315414,12.));
#249268=CARTESIAN_POINT('Ctrl Pts',(13.1855578436471,19.5889249285338,0.));
#249269=CARTESIAN_POINT('Ctrl Pts',(13.1855578436471,19.5889249285338,12.));
#249270=CARTESIAN_POINT('Ctrl Pts',(13.1800221307673,19.5705738004667,0.));
#249271=CARTESIAN_POINT('Ctrl Pts',(13.1800221307673,19.5705738004667,12.));
#249272=CARTESIAN_POINT('Ctrl Pts',(13.1744697070911,19.5523490490244,0.));
#249273=CARTESIAN_POINT('Ctrl Pts',(13.1744697070911,19.5523490490244,12.));
#249274=CARTESIAN_POINT('Ctrl Pts',(13.168901332843,19.5342514857562,0.));
#249275=CARTESIAN_POINT('Ctrl Pts',(13.168901332843,19.5342514857562,12.));
#249276=CARTESIAN_POINT('Ctrl Pts',(13.1633177803101,19.5162819323213,0.));
#249277=CARTESIAN_POINT('Ctrl Pts',(13.1633177803101,19.5162819323213,12.));
#249278=CARTESIAN_POINT('Ctrl Pts',(13.1577198341245,19.4984412207082,0.));
#249279=CARTESIAN_POINT('Ctrl Pts',(13.1577198341245,19.4984412207082,12.));
#249280=CARTESIAN_POINT('Ctrl Pts',(13.1521082915853,19.4807301935268,0.));
#249281=CARTESIAN_POINT('Ctrl Pts',(13.1521082915853,19.4807301935268,12.));
#249282=CARTESIAN_POINT('Ctrl Pts',(13.1464839629971,19.4631497043258,0.));
#249283=CARTESIAN_POINT('Ctrl Pts',(13.1464839629971,19.4631497043258,12.));
#249284=CARTESIAN_POINT('Ctrl Pts',(13.1408476720061,19.4457006178876,0.));
#249285=CARTESIAN_POINT('Ctrl Pts',(13.1408476720061,19.4457006178876,12.));
#249286=CARTESIAN_POINT('Ctrl Pts',(13.1352002559438,19.4283838105262,0.));
#249287=CARTESIAN_POINT('Ctrl Pts',(13.1352002559438,19.4283838105262,12.));
#249288=CARTESIAN_POINT('Ctrl Pts',(13.1295425661634,19.4112001703557,0.));
#249289=CARTESIAN_POINT('Ctrl Pts',(13.1295425661634,19.4112001703557,12.));
#249290=CARTESIAN_POINT('Ctrl Pts',(13.1238754684177,19.3941505976263,0.));
#249291=CARTESIAN_POINT('Ctrl Pts',(13.1238754684177,19.3941505976263,12.));
#249292=CARTESIAN_POINT('Ctrl Pts',(13.118199843271,19.3772360051091,0.));
#249293=CARTESIAN_POINT('Ctrl Pts',(13.118199843271,19.3772360051091,12.));
#249294=CARTESIAN_POINT('Ctrl Pts',(13.1125165865022,19.3604573184515,0.));
#249295=CARTESIAN_POINT('Ctrl Pts',(13.1125165865022,19.3604573184515,12.));
#249296=CARTESIAN_POINT('Ctrl Pts',(13.1068266095186,19.3438154765395,0.));
#249297=CARTESIAN_POINT('Ctrl Pts',(13.1068266095186,19.3438154765395,12.));
#249298=CARTESIAN_POINT('Ctrl Pts',(13.1011308397591,19.3273114318269,0.));
#249299=CARTESIAN_POINT('Ctrl Pts',(13.1011308397591,19.3273114318269,12.));
#249300=CARTESIAN_POINT('Ctrl Pts',(13.0954302211479,19.310946150736,0.));
#249301=CARTESIAN_POINT('Ctrl Pts',(13.0954302211479,19.310946150736,12.));
#249302=CARTESIAN_POINT('Ctrl Pts',(13.0897257145968,19.2947206141247,0.));
#249303=CARTESIAN_POINT('Ctrl Pts',(13.0897257145968,19.2947206141247,12.));
#249304=CARTESIAN_POINT('Ctrl Pts',(13.0840182984949,19.2786358177198,0.));
#249305=CARTESIAN_POINT('Ctrl Pts',(13.0840182984949,19.2786358177198,12.));
#249306=CARTESIAN_POINT('Ctrl Pts',(13.0783089692118,19.2626927725596,0.));
#249307=CARTESIAN_POINT('Ctrl Pts',(13.0783089692118,19.2626927725596,12.));
#249308=CARTESIAN_POINT('Ctrl Pts',(13.0725987415859,19.2468925053989,0.));
#249309=CARTESIAN_POINT('Ctrl Pts',(13.0725987415859,19.2468925053989,12.));
#249310=CARTESIAN_POINT('Ctrl Pts',(13.0668886494795,19.2312360592033,0.));
#249311=CARTESIAN_POINT('Ctrl Pts',(13.0668886494795,19.2312360592033,12.));
#249312=CARTESIAN_POINT('Ctrl Pts',(13.0611797463915,19.2157244937142,0.));
#249313=CARTESIAN_POINT('Ctrl Pts',(13.0611797463915,19.2157244937142,12.));
#249314=CARTESIAN_POINT('Ctrl Pts',(13.0554731060538,19.2003588859772,0.));
#249315=CARTESIAN_POINT('Ctrl Pts',(13.0554731060538,19.2003588859772,12.));
#249316=CARTESIAN_POINT('Ctrl Pts',(13.0497698230441,19.1851403308825,0.));
#249317=CARTESIAN_POINT('Ctrl Pts',(13.0497698230441,19.1851403308825,12.));
#249318=CARTESIAN_POINT('Ctrl Pts',(13.0440710133772,19.1700699416622,0.));
#249319=CARTESIAN_POINT('Ctrl Pts',(13.0440710133772,19.1700699416622,12.));
#249320=CARTESIAN_POINT('Ctrl Pts',(13.0383778152068,19.155148850523,0.));
#249321=CARTESIAN_POINT('Ctrl Pts',(13.0383778152068,19.155148850523,12.));
#249322=CARTESIAN_POINT('Ctrl Pts',(13.0326913895838,19.1403782093386,0.));
#249323=CARTESIAN_POINT('Ctrl Pts',(13.0326913895838,19.1403782093386,12.));
#249324=CARTESIAN_POINT('Ctrl Pts',(13.0270129211976,19.1257591903099,0.));
#249325=CARTESIAN_POINT('Ctrl Pts',(13.0270129211976,19.1257591903099,12.));
#249326=CARTESIAN_POINT('Ctrl Pts',(13.0213436191328,19.111292986631,0.));
#249327=CARTESIAN_POINT('Ctrl Pts',(13.0213436191328,19.111292986631,12.));
#249328=CARTESIAN_POINT('Ctrl Pts',(13.0156847176096,19.0969808131228,0.));
#249329=CARTESIAN_POINT('Ctrl Pts',(13.0156847176096,19.0969808131228,12.));
#249330=CARTESIAN_POINT('Ctrl Pts',(13.0100374768788,19.0828239070484,0.));
#249331=CARTESIAN_POINT('Ctrl Pts',(13.0100374768788,19.0828239070484,12.));
#249332=CARTESIAN_POINT('Ctrl Pts',(13.0044031841382,19.0688235289437,0.));
#249333=CARTESIAN_POINT('Ctrl Pts',(13.0044031841382,19.0688235289437,12.));
#249334=CARTESIAN_POINT('Ctrl Pts',(12.9987831544502,19.0549809634354,0.));
#249335=CARTESIAN_POINT('Ctrl Pts',(12.9987831544502,19.0549809634354,12.));
#249336=CARTESIAN_POINT('Ctrl Pts',(12.9931787316514,19.0412975200398,0.));
#249337=CARTESIAN_POINT('Ctrl Pts',(12.9931787316514,19.0412975200398,12.));
#249338=CARTESIAN_POINT('Ctrl Pts',(12.9875912893003,19.0277745339909,0.));
#249339=CARTESIAN_POINT('Ctrl Pts',(12.9875912893003,19.0277745339909,12.));
#249340=CARTESIAN_POINT('Ctrl Pts',(12.9820222318716,19.014413367335,0.));
#249341=CARTESIAN_POINT('Ctrl Pts',(12.9820222318716,19.014413367335,12.));
#249342=CARTESIAN_POINT('Ctrl Pts',(12.9764729959206,19.0012154099792,0.));
#249343=CARTESIAN_POINT('Ctrl Pts',(12.9764729959206,19.0012154099792,12.));
#249344=CARTESIAN_POINT('Ctrl Pts',(12.9709450512747,18.9881820807585,0.));
#249345=CARTESIAN_POINT('Ctrl Pts',(12.9709450512747,18.9881820807585,12.));
#249346=CARTESIAN_POINT('Ctrl Pts',(12.9654399021868,18.9753148284473,0.));
#249347=CARTESIAN_POINT('Ctrl Pts',(12.9654399021868,18.9753148284473,12.));
#249348=CARTESIAN_POINT('Ctrl Pts',(12.9599590886317,18.9626151329226,0.));
#249349=CARTESIAN_POINT('Ctrl Pts',(12.9599590886317,18.9626151329226,12.));
#249350=CARTESIAN_POINT('Ctrl Pts',(12.9545041877377,18.9500845064714,0.));
#249351=CARTESIAN_POINT('Ctrl Pts',(12.9545041877377,18.9500845064714,12.));
#249352=CARTESIAN_POINT('Ctrl Pts',(12.9490768151821,18.9377244950435,0.));
#249353=CARTESIAN_POINT('Ctrl Pts',(12.9490768151821,18.9377244950435,12.));
#249354=CARTESIAN_POINT('Ctrl Pts',(12.9436786266106,18.9255366795196,0.));
#249355=CARTESIAN_POINT('Ctrl Pts',(12.9436786266106,18.9255366795196,12.));
#249356=CARTESIAN_POINT('Ctrl Pts',(12.9383113190375,18.9135226769466,0.));
#249357=CARTESIAN_POINT('Ctrl Pts',(12.9383113190375,18.9135226769466,12.));
#249358=CARTESIAN_POINT('Ctrl Pts',(12.9329766328184,18.9016841423402,0.));
#249359=CARTESIAN_POINT('Ctrl Pts',(12.9329766328184,18.9016841423402,12.));
#249360=CARTESIAN_POINT('Ctrl Pts',(12.9276763536372,18.8900227704888,0.));
#249361=CARTESIAN_POINT('Ctrl Pts',(12.9276763536372,18.8900227704888,12.));
#249362=CARTESIAN_POINT('Ctrl Pts',(12.9224123144982,18.8785402977528,0.));
#249363=CARTESIAN_POINT('Ctrl Pts',(12.9224123144982,18.8785402977528,12.));
#249364=CARTESIAN_POINT('Ctrl Pts',(12.9171863977047,18.8672385038328,0.));
#249365=CARTESIAN_POINT('Ctrl Pts',(12.9171863977047,18.8672385038328,12.));
#249366=CARTESIAN_POINT('Ctrl Pts',(12.9120005369066,18.8561192136201,0.));
#249367=CARTESIAN_POINT('Ctrl Pts',(12.9120005369066,18.8561192136201,12.));
#249368=CARTESIAN_POINT('Ctrl Pts',(12.9068567191856,18.8451842990986,0.));
#249369=CARTESIAN_POINT('Ctrl Pts',(12.9068567191856,18.8451842990986,12.));
#249370=CARTESIAN_POINT('Ctrl Pts',(12.9017569871738,18.834435681259,0.));
#249371=CARTESIAN_POINT('Ctrl Pts',(12.9017569871738,18.834435681259,12.));
#249372=CARTESIAN_POINT('Ctrl Pts',(12.8967034410752,18.8238753319124,0.));
#249373=CARTESIAN_POINT('Ctrl Pts',(12.8967034410752,18.8238753319124,12.));
#249374=CARTESIAN_POINT('Ctrl Pts',(12.8916982409931,18.8135052757815,0.));
#249375=CARTESIAN_POINT('Ctrl Pts',(12.8916982409931,18.8135052757815,12.));
#249376=CARTESIAN_POINT('Ctrl Pts',(12.8867436109543,18.8033275941939,0.));
#249377=CARTESIAN_POINT('Ctrl Pts',(12.8867436109543,18.8033275941939,12.));
#249378=CARTESIAN_POINT('Ctrl Pts',(12.8818418427474,18.7933444285867,0.));
#249379=CARTESIAN_POINT('Ctrl Pts',(12.8818418427474,18.7933444285867,12.));
#249380=CARTESIAN_POINT('Ctrl Pts',(12.8769952998097,18.7835579840481,0.));
#249381=CARTESIAN_POINT('Ctrl Pts',(12.8769952998097,18.7835579840481,12.));
#249382=CARTESIAN_POINT('Ctrl Pts',(12.8722064211814,18.7739705329029,0.));
#249383=CARTESIAN_POINT('Ctrl Pts',(12.8722064211814,18.7739705329029,12.));
#249384=CARTESIAN_POINT('Ctrl Pts',(12.8674777239656,18.7645844169568,0.));
#249385=CARTESIAN_POINT('Ctrl Pts',(12.8674777239656,18.7645844169568,12.));
#249386=CARTESIAN_POINT('Ctrl Pts',(12.8628118054172,18.7554020493888,0.));
#249387=CARTESIAN_POINT('Ctrl Pts',(12.8628118054172,18.7554020493888,12.));
#249388=CARTESIAN_POINT('Ctrl Pts',(12.8582113455644,18.7464259171248,0.));
#249389=CARTESIAN_POINT('Ctrl Pts',(12.8582113455644,18.7464259171248,12.));
#249390=CARTESIAN_POINT('Ctrl Pts',(12.8536791086315,18.7376585820851,0.));
#249391=CARTESIAN_POINT('Ctrl Pts',(12.8536791086315,18.7376585820851,12.));
#249392=CARTESIAN_POINT('Ctrl Pts',(12.849217951159,18.7291026886552,0.));
#249393=CARTESIAN_POINT('Ctrl Pts',(12.849217951159,18.7291026886552,12.));
#249394=CARTESIAN_POINT('Ctrl Pts',(12.8448308329494,18.7207609737701,0.));
#249395=CARTESIAN_POINT('Ctrl Pts',(12.8448308329494,18.7207609737701,12.));
#249396=CARTESIAN_POINT('Ctrl Pts',(12.8405208263432,18.7126362754446,0.));
#249397=CARTESIAN_POINT('Ctrl Pts',(12.8405208263432,18.7126362754446,12.));
#249398=CARTESIAN_POINT('Ctrl Pts',(12.8362911280362,18.7047315436296,0.));
#249399=CARTESIAN_POINT('Ctrl Pts',(12.8362911280362,18.7047315436296,12.));
#249400=CARTESIAN_POINT('Ctrl Pts',(12.832145059979,18.6970498410173,0.));
#249401=CARTESIAN_POINT('Ctrl Pts',(12.832145059979,18.6970498410173,12.));
#249402=CARTESIAN_POINT('Ctrl Pts',(12.8280860635231,18.6895943376172,0.));
#249403=CARTESIAN_POINT('Ctrl Pts',(12.8280860635231,18.6895943376172,12.));
#249404=CARTESIAN_POINT('Ctrl Pts',(12.8241176980016,18.6823683094139,0.));
#249405=CARTESIAN_POINT('Ctrl Pts',(12.8241176980016,18.6823683094139,12.));
#249406=CARTESIAN_POINT('Ctrl Pts',(12.8202436318473,18.6753751301091,0.));
#249407=CARTESIAN_POINT('Ctrl Pts',(12.8202436318473,18.6753751301091,12.));
#249408=CARTESIAN_POINT('Ctrl Pts',(12.8164676687361,18.6686182952798,0.));
#249409=CARTESIAN_POINT('Ctrl Pts',(12.8164676687361,18.6686182952798,12.));
#249410=CARTESIAN_POINT('Ctrl Pts',(12.8127937909632,18.6621014624746,0.));
#249411=CARTESIAN_POINT('Ctrl Pts',(12.8127937909632,18.6621014624746,12.));
#249412=CARTESIAN_POINT('Ctrl Pts',(12.8092261933858,18.6558284825772,0.));
#249413=CARTESIAN_POINT('Ctrl Pts',(12.8092261933858,18.6558284825772,12.));
#249414=CARTESIAN_POINT('Ctrl Pts',(12.805769331162,18.6498034438986,0.));
#249415=CARTESIAN_POINT('Ctrl Pts',(12.805769331162,18.6498034438986,12.));
#249416=CARTESIAN_POINT('Ctrl Pts',(12.8024278770153,18.6440306327457,0.));
#249417=CARTESIAN_POINT('Ctrl Pts',(12.8024278770153,18.6440306327457,12.));
#249418=CARTESIAN_POINT('Ctrl Pts',(12.7992066625264,18.63851447924,0.));
#249419=CARTESIAN_POINT('Ctrl Pts',(12.7992066625264,18.63851447924,12.));
#249420=CARTESIAN_POINT('Ctrl Pts',(12.7961106222251,18.6332595057005,0.));
#249421=CARTESIAN_POINT('Ctrl Pts',(12.7961106222251,18.6332595057005,12.));
#249422=CARTESIAN_POINT('Ctrl Pts',(12.7931447451556,18.6282702819371,0.));
#249423=CARTESIAN_POINT('Ctrl Pts',(12.7931447451556,18.6282702819371,12.));
#249424=CARTESIAN_POINT('Ctrl Pts',(12.7903142925234,18.6235516265575,0.));
#249425=CARTESIAN_POINT('Ctrl Pts',(12.7903142925234,18.6235516265575,12.));
#249426=CARTESIAN_POINT('Ctrl Pts',(12.7876249657834,18.6191087624752,0.));
#249427=CARTESIAN_POINT('Ctrl Pts',(12.7876249657834,18.6191087624752,12.));
#249428=CARTESIAN_POINT('Ctrl Pts',(12.78508316579,18.6149475565189,0.));
#249429=CARTESIAN_POINT('Ctrl Pts',(12.78508316579,18.6149475565189,12.));
#249430=CARTESIAN_POINT('Ctrl Pts',(12.7826959526924,18.611074482622,0.));
#249431=CARTESIAN_POINT('Ctrl Pts',(12.7826959526924,18.611074482622,12.));
#249432=CARTESIAN_POINT('Ctrl Pts',(12.7804705387658,18.6074961535723,0.));
#249433=CARTESIAN_POINT('Ctrl Pts',(12.7804705387658,18.6074961535723,12.));
#249434=CARTESIAN_POINT('Ctrl Pts',(12.7784139605067,18.6042190183703,0.));
#249435=CARTESIAN_POINT('Ctrl Pts',(12.7784139605067,18.6042190183703,12.));
#249436=CARTESIAN_POINT('Ctrl Pts',(12.7765325225082,18.6012488486708,0.));
#249437=CARTESIAN_POINT('Ctrl Pts',(12.7765325225082,18.6012488486708,12.));
#249438=CARTESIAN_POINT('Ctrl Pts',(12.7748328937639,18.5985917525949,0.));
#249439=CARTESIAN_POINT('Ctrl Pts',(12.7748328937639,18.5985917525949,12.));
#249440=CARTESIAN_POINT('Ctrl Pts',(12.7733231262107,18.5962551167772,0.));
#249441=CARTESIAN_POINT('Ctrl Pts',(12.7733231262107,18.5962551167772,12.));
#249442=CARTESIAN_POINT('Ctrl Pts',(12.7720142287169,18.5942490615409,0.));
#249443=CARTESIAN_POINT('Ctrl Pts',(12.7720142287169,18.5942490615409,12.));
#249444=CARTESIAN_POINT('Ctrl Pts',(12.7709195951153,18.5925859134582,0.));
#249445=CARTESIAN_POINT('Ctrl Pts',(12.7709195951153,18.5925859134582,12.));
#249446=CARTESIAN_POINT('Ctrl Pts',(12.7700520897174,18.5912775137806,0.));
#249447=CARTESIAN_POINT('Ctrl Pts',(12.7700520897174,18.5912775137806,12.));
#249448=CARTESIAN_POINT('Ctrl Pts',(12.7694215127923,18.590332877722,0.));
#249449=CARTESIAN_POINT('Ctrl Pts',(12.7694215127923,18.590332877722,12.));
#249450=CARTESIAN_POINT('Ctrl Pts',(12.7691103481996,18.589871621842,0.));
#249451=CARTESIAN_POINT('Ctrl Pts',(12.7691103481996,18.589871621842,12.));
#249452=CARTESIAN_POINT('Ctrl Pts',(12.7689864266924,18.5896919669158,0.));
#249453=CARTESIAN_POINT('Ctrl Pts',(12.7689864266924,18.5896919669158,12.));
#249454=CARTESIAN_POINT('Ctrl Pts',(12.7689524524484,18.5896460962961,0.));
#249455=CARTESIAN_POINT('Ctrl Pts',(12.7689524524484,18.5896460962961,12.));
#249456=CARTESIAN_POINT('Ctrl Pts',(12.7689476255363,18.5896416359912,0.));
#249457=CARTESIAN_POINT('Ctrl Pts',(12.7689476255363,18.5896416359912,12.));
#249458=CARTESIAN_POINT('',(13.5685075571671,22.1787195904339,0.));
#249459=CARTESIAN_POINT('Ctrl Pts',(13.5685075571671,22.1787195904339,0.));
#249460=CARTESIAN_POINT('Ctrl Pts',(13.5683460612913,22.1730081264583,0.));
#249461=CARTESIAN_POINT('Ctrl Pts',(13.5680170531724,22.1615922804939,0.));
#249462=CARTESIAN_POINT('Ctrl Pts',(13.5675054918922,22.1444897575076,0.));
#249463=CARTESIAN_POINT('Ctrl Pts',(13.5667873105179,22.1217288871823,0.));
#249464=CARTESIAN_POINT('Ctrl Pts',(13.5658294169106,22.0933486464442,0.));
#249465=CARTESIAN_POINT('Ctrl Pts',(13.5648113688894,22.0650393089492,0.));
#249466=CARTESIAN_POINT('Ctrl Pts',(13.5637332022393,22.0368009736227,0.));
#249467=CARTESIAN_POINT('Ctrl Pts',(13.5625949868313,22.0086337943431,0.));
#249468=CARTESIAN_POINT('Ctrl Pts',(13.5613968357589,21.9805379899192,0.));
#249469=CARTESIAN_POINT('Ctrl Pts',(13.5601389185315,21.9525138592862,0.));
#249470=CARTESIAN_POINT('Ctrl Pts',(13.5588214586672,21.9245617765827,0.));
#249471=CARTESIAN_POINT('Ctrl Pts',(13.5574447178484,21.8966821688876,0.));
#249472=CARTESIAN_POINT('Ctrl Pts',(13.5560089839426,21.8688754989401,0.));
#249473=CARTESIAN_POINT('Ctrl Pts',(13.5545145573048,21.841142245609,0.));
#249474=CARTESIAN_POINT('Ctrl Pts',(13.5529617381569,21.8134828857963,0.));
#249475=CARTESIAN_POINT('Ctrl Pts',(13.5513508127232,21.7858978745848,0.));
#249476=CARTESIAN_POINT('Ctrl Pts',(13.5496820422186,21.7583876294532,0.));
#249477=CARTESIAN_POINT('Ctrl Pts',(13.5479556704457,21.730952541226,0.));
#249478=CARTESIAN_POINT('Ctrl Pts',(13.546171929503,21.7035929822939,0.));
#249479=CARTESIAN_POINT('Ctrl Pts',(13.5443310461516,21.676309315769,0.));
#249480=CARTESIAN_POINT('Ctrl Pts',(13.5424332480698,21.6491019044647,0.));
#249481=CARTESIAN_POINT('Ctrl Pts',(13.5404787697798,21.6219711193951,0.));
#249482=CARTESIAN_POINT('Ctrl Pts',(13.5384678597206,21.5949173499022,0.));
#249483=CARTESIAN_POINT('Ctrl Pts',(13.5364007790292,21.5679410019011,0.));
#249484=CARTESIAN_POINT('Ctrl Pts',(13.5342777983225,21.5410424932511,0.));
#249485=CARTESIAN_POINT('Ctrl Pts',(13.5320991952145,21.5142222501671,0.));
#249486=CARTESIAN_POINT('Ctrl Pts',(13.5298652514357,21.487480703047,0.));
#249487=CARTESIAN_POINT('Ctrl Pts',(13.5275762503553,21.4608182828695,0.));
#249488=CARTESIAN_POINT('Ctrl Pts',(13.5252324737795,21.4342354165254,0.));
#249489=CARTESIAN_POINT('Ctrl Pts',(13.5228342013508,21.4077325259318,0.));
#249490=CARTESIAN_POINT('Ctrl Pts',(13.5203817122496,21.3813100304967,0.));
#249491=CARTESIAN_POINT('Ctrl Pts',(13.5178752862461,21.3549683486219,0.));
#249492=CARTESIAN_POINT('Ctrl Pts',(13.5153152050554,21.328707899634,0.));
#249493=CARTESIAN_POINT('Ctrl Pts',(13.5127017534972,21.3025291054236,0.));
#249494=CARTESIAN_POINT('Ctrl Pts',(13.5100352209207,21.2764323924442,0.));
#249495=CARTESIAN_POINT('Ctrl Pts',(13.5073159019454,21.2504181927429,0.));
#249496=CARTESIAN_POINT('Ctrl Pts',(13.5045440957404,21.224486942933,0.));
#249497=CARTESIAN_POINT('Ctrl Pts',(13.5017201056088,21.1986390835825,0.));
#249498=CARTESIAN_POINT('Ctrl Pts',(13.4988442384491,21.1728750584173,0.));
#249499=CARTESIAN_POINT('Ctrl Pts',(13.4959168042934,21.1471953136209,0.));
#249500=CARTESIAN_POINT('Ctrl Pts',(13.4929381157778,21.1216002970209,0.));
#249501=CARTESIAN_POINT('Ctrl Pts',(13.4899084877718,21.0960904575048,0.));
#249502=CARTESIAN_POINT('Ctrl Pts',(13.4868282377191,21.0706662455202,0.));
#249503=CARTESIAN_POINT('Ctrl Pts',(13.4836976858912,21.0453281134247,0.));
#249504=CARTESIAN_POINT('Ctrl Pts',(13.4805171556822,21.0200765158885,0.));
#249505=CARTESIAN_POINT('Ctrl Pts',(13.4772869738879,20.9949119102592,0.));
#249506=CARTESIAN_POINT('Ctrl Pts',(13.4740074710087,20.9698347569476,0.));
#249507=CARTESIAN_POINT('Ctrl Pts',(13.4706789815166,20.9448455197557,0.));
#249508=CARTESIAN_POINT('Ctrl Pts',(13.4673018437718,20.9199446657584,0.));
#249509=CARTESIAN_POINT('Ctrl Pts',(13.4638763999725,20.8951326652158,0.));
#249510=CARTESIAN_POINT('Ctrl Pts',(13.4604029960983,20.8704099914641,0.));
#249511=CARTESIAN_POINT('Ctrl Pts',(13.4568819818631,20.8457771208082,0.));
#249512=CARTESIAN_POINT('Ctrl Pts',(13.4533137106667,20.821234532398,0.));
#249513=CARTESIAN_POINT('Ctrl Pts',(13.4496985395637,20.7967827081227,0.));
#249514=CARTESIAN_POINT('Ctrl Pts',(13.4460368293688,20.7724221327608,0.));
#249515=CARTESIAN_POINT('Ctrl Pts',(13.4423289447561,20.7481532941013,0.));
#249516=CARTESIAN_POINT('Ctrl Pts',(13.4385752543663,20.7239766830675,0.));
#249517=CARTESIAN_POINT('Ctrl Pts',(13.4347761309154,20.6998927938288,0.));
#249518=CARTESIAN_POINT('Ctrl Pts',(13.4309319513119,20.6759021239103,0.));
#249519=CARTESIAN_POINT('Ctrl Pts',(13.4270430967651,20.6520051742869,0.));
#249520=CARTESIAN_POINT('Ctrl Pts',(13.4231099528179,20.6282024494237,0.));
#249521=CARTESIAN_POINT('Ctrl Pts',(13.4191329093932,20.6044944573153,0.));
#249522=CARTESIAN_POINT('Ctrl Pts',(13.4151123608411,20.5808817095155,0.));
#249523=CARTESIAN_POINT('Ctrl Pts',(13.4110487059912,20.5573647211639,0.));
#249524=CARTESIAN_POINT('Ctrl Pts',(13.4069423482076,20.5339440109956,0.));
#249525=CARTESIAN_POINT('Ctrl Pts',(13.4027936954529,20.5106201013753,0.));
#249526=CARTESIAN_POINT('Ctrl Pts',(13.3986031603716,20.487393518404,0.));
#249527=CARTESIAN_POINT('Ctrl Pts',(13.3943711603739,20.4642647920038,0.));
#249528=CARTESIAN_POINT('Ctrl Pts',(13.3900981177255,20.4412344560008,0.));
#249529=CARTESIAN_POINT('Ctrl Pts',(13.3857844596387,20.4183030482002,0.));
#249530=CARTESIAN_POINT('Ctrl Pts',(13.3814306183719,20.3954711104502,0.));
#249531=CARTESIAN_POINT('Ctrl Pts',(13.3770370313188,20.3727391887184,0.));
#249532=CARTESIAN_POINT('Ctrl Pts',(13.3726041410867,20.3501078331814,0.));
#249533=CARTESIAN_POINT('Ctrl Pts',(13.3681323955826,20.3275775983029,0.));
#249534=CARTESIAN_POINT('Ctrl Pts',(13.3636222481016,20.3051490429048,0.));
#249535=CARTESIAN_POINT('Ctrl Pts',(13.3590741574195,20.2828227302339,0.));
#249536=CARTESIAN_POINT('Ctrl Pts',(13.3544885878889,20.2605992280122,0.));
#249537=CARTESIAN_POINT('Ctrl Pts',(13.3498660095386,20.2384791085359,0.));
#249538=CARTESIAN_POINT('Ctrl Pts',(13.3452068981766,20.216462948786,0.));
#249539=CARTESIAN_POINT('Ctrl Pts',(13.3405117354971,20.1945513305235,0.));
#249540=CARTESIAN_POINT('Ctrl Pts',(13.3357810091903,20.1727448403817,0.));
#249541=CARTESIAN_POINT('Ctrl Pts',(13.3310152130564,20.1510440699474,0.));
#249542=CARTESIAN_POINT('Ctrl Pts',(13.3262148471226,20.1294496158402,0.));
#249543=CARTESIAN_POINT('Ctrl Pts',(13.3213804177587,20.1079620798375,0.));
#249544=CARTESIAN_POINT('Ctrl Pts',(13.3165124377962,20.0865820689883,0.));
#249545=CARTESIAN_POINT('Ctrl Pts',(13.3116114266515,20.0653101957188,0.));
#249546=CARTESIAN_POINT('Ctrl Pts',(13.3066779104515,20.0441470779345,0.));
#249547=CARTESIAN_POINT('Ctrl Pts',(13.3017124221637,20.0230933391038,0.));
#249548=CARTESIAN_POINT('Ctrl Pts',(13.2967155017306,20.0021496083738,0.));
#249549=CARTESIAN_POINT('Ctrl Pts',(13.2916876962094,19.981316520717,0.));
#249550=CARTESIAN_POINT('Ctrl Pts',(13.286629559915,19.9605947170586,0.));
#249551=CARTESIAN_POINT('Ctrl Pts',(13.2815416545663,19.9399848444019,0.));
#249552=CARTESIAN_POINT('Ctrl Pts',(13.2764245494357,19.9194875559422,0.));
#249553=CARTESIAN_POINT('Ctrl Pts',(13.271278821502,19.8991035111745,0.));
#249554=CARTESIAN_POINT('Ctrl Pts',(13.2661050556132,19.8788333760577,0.));
#249555=CARTESIAN_POINT('Ctrl Pts',(13.2609038446529,19.8586778231715,0.));
#249556=CARTESIAN_POINT('Ctrl Pts',(13.2556757897086,19.8386375318634,0.));
#249557=CARTESIAN_POINT('Ctrl Pts',(13.2504215002457,19.8187131883917,0.));
#249558=CARTESIAN_POINT('Ctrl Pts',(13.2451415942805,19.7989054860495,0.));
#249559=CARTESIAN_POINT('Ctrl Pts',(13.2398366985675,19.7792151253289,0.));
#249560=CARTESIAN_POINT('Ctrl Pts',(13.2345074487963,19.7596428141168,0.));
#249561=CARTESIAN_POINT('Ctrl Pts',(13.2291544897899,19.7401892678697,0.));
#249562=CARTESIAN_POINT('Ctrl Pts',(13.2237784757065,19.7208552097868,0.));
#249563=CARTESIAN_POINT('Ctrl Pts',(13.2183800702436,19.7016413709685,0.));
#249564=CARTESIAN_POINT('Ctrl Pts',(13.2129599468485,19.6825484905823,0.));
#249565=CARTESIAN_POINT('Ctrl Pts',(13.2075187889529,19.6635773160936,0.));
#249566=CARTESIAN_POINT('Ctrl Pts',(13.2020572902065,19.6447286034772,0.));
#249567=CARTESIAN_POINT('Ctrl Pts',(13.1965761547151,19.6260031174244,0.));
#249568=CARTESIAN_POINT('Ctrl Pts',(13.1910760972814,19.6074016315414,0.));
#249569=CARTESIAN_POINT('Ctrl Pts',(13.1855578436471,19.5889249285338,0.));
#249570=CARTESIAN_POINT('Ctrl Pts',(13.1800221307673,19.5705738004667,0.));
#249571=CARTESIAN_POINT('Ctrl Pts',(13.1744697070911,19.5523490490244,0.));
#249572=CARTESIAN_POINT('Ctrl Pts',(13.168901332843,19.5342514857562,0.));
#249573=CARTESIAN_POINT('Ctrl Pts',(13.1633177803101,19.5162819323213,0.));
#249574=CARTESIAN_POINT('Ctrl Pts',(13.1577198341245,19.4984412207082,0.));
#249575=CARTESIAN_POINT('Ctrl Pts',(13.1521082915853,19.4807301935268,0.));
#249576=CARTESIAN_POINT('Ctrl Pts',(13.1464839629971,19.4631497043258,0.));
#249577=CARTESIAN_POINT('Ctrl Pts',(13.1408476720061,19.4457006178876,0.));
#249578=CARTESIAN_POINT('Ctrl Pts',(13.1352002559438,19.4283838105262,0.));
#249579=CARTESIAN_POINT('Ctrl Pts',(13.1295425661634,19.4112001703557,0.));
#249580=CARTESIAN_POINT('Ctrl Pts',(13.1238754684177,19.3941505976263,0.));
#249581=CARTESIAN_POINT('Ctrl Pts',(13.118199843271,19.3772360051091,0.));
#249582=CARTESIAN_POINT('Ctrl Pts',(13.1125165865022,19.3604573184515,0.));
#249583=CARTESIAN_POINT('Ctrl Pts',(13.1068266095186,19.3438154765395,0.));
#249584=CARTESIAN_POINT('Ctrl Pts',(13.1011308397591,19.3273114318269,0.));
#249585=CARTESIAN_POINT('Ctrl Pts',(13.0954302211479,19.310946150736,0.));
#249586=CARTESIAN_POINT('Ctrl Pts',(13.0897257145968,19.2947206141247,0.));
#249587=CARTESIAN_POINT('Ctrl Pts',(13.0840182984949,19.2786358177198,0.));
#249588=CARTESIAN_POINT('Ctrl Pts',(13.0783089692118,19.2626927725596,0.));
#249589=CARTESIAN_POINT('Ctrl Pts',(13.0725987415859,19.2468925053989,0.));
#249590=CARTESIAN_POINT('Ctrl Pts',(13.0668886494795,19.2312360592033,0.));
#249591=CARTESIAN_POINT('Ctrl Pts',(13.0611797463915,19.2157244937142,0.));
#249592=CARTESIAN_POINT('Ctrl Pts',(13.0554731060538,19.2003588859772,0.));
#249593=CARTESIAN_POINT('Ctrl Pts',(13.0497698230441,19.1851403308825,0.));
#249594=CARTESIAN_POINT('Ctrl Pts',(13.0440710133772,19.1700699416622,0.));
#249595=CARTESIAN_POINT('Ctrl Pts',(13.0383778152068,19.155148850523,0.));
#249596=CARTESIAN_POINT('Ctrl Pts',(13.0326913895838,19.1403782093386,0.));
#249597=CARTESIAN_POINT('Ctrl Pts',(13.0270129211976,19.1257591903099,0.));
#249598=CARTESIAN_POINT('Ctrl Pts',(13.0213436191328,19.111292986631,0.));
#249599=CARTESIAN_POINT('Ctrl Pts',(13.0156847176096,19.0969808131228,0.));
#249600=CARTESIAN_POINT('Ctrl Pts',(13.0100374768788,19.0828239070484,0.));
#249601=CARTESIAN_POINT('Ctrl Pts',(13.0044031841382,19.0688235289437,0.));
#249602=CARTESIAN_POINT('Ctrl Pts',(12.9987831544502,19.0549809634354,0.));
#249603=CARTESIAN_POINT('Ctrl Pts',(12.9931787316514,19.0412975200398,0.));
#249604=CARTESIAN_POINT('Ctrl Pts',(12.9875912893003,19.0277745339909,0.));
#249605=CARTESIAN_POINT('Ctrl Pts',(12.9820222318716,19.014413367335,0.));
#249606=CARTESIAN_POINT('Ctrl Pts',(12.9764729959206,19.0012154099792,0.));
#249607=CARTESIAN_POINT('Ctrl Pts',(12.9709450512747,18.9881820807585,0.));
#249608=CARTESIAN_POINT('Ctrl Pts',(12.9654399021868,18.9753148284473,0.));
#249609=CARTESIAN_POINT('Ctrl Pts',(12.9599590886317,18.9626151329226,0.));
#249610=CARTESIAN_POINT('Ctrl Pts',(12.9545041877377,18.9500845064714,0.));
#249611=CARTESIAN_POINT('Ctrl Pts',(12.9490768151821,18.9377244950435,0.));
#249612=CARTESIAN_POINT('Ctrl Pts',(12.9436786266106,18.9255366795196,0.));
#249613=CARTESIAN_POINT('Ctrl Pts',(12.9383113190375,18.9135226769466,0.));
#249614=CARTESIAN_POINT('Ctrl Pts',(12.9329766328184,18.9016841423402,0.));
#249615=CARTESIAN_POINT('Ctrl Pts',(12.9276763536372,18.8900227704888,0.));
#249616=CARTESIAN_POINT('Ctrl Pts',(12.9224123144982,18.8785402977528,0.));
#249617=CARTESIAN_POINT('Ctrl Pts',(12.9171863977047,18.8672385038328,0.));
#249618=CARTESIAN_POINT('Ctrl Pts',(12.9120005369066,18.8561192136201,0.));
#249619=CARTESIAN_POINT('Ctrl Pts',(12.9068567191856,18.8451842990986,0.));
#249620=CARTESIAN_POINT('Ctrl Pts',(12.9017569871738,18.834435681259,0.));
#249621=CARTESIAN_POINT('Ctrl Pts',(12.8967034410752,18.8238753319124,0.));
#249622=CARTESIAN_POINT('Ctrl Pts',(12.8916982409931,18.8135052757815,0.));
#249623=CARTESIAN_POINT('Ctrl Pts',(12.8867436109543,18.8033275941939,0.));
#249624=CARTESIAN_POINT('Ctrl Pts',(12.8818418427474,18.7933444285867,0.));
#249625=CARTESIAN_POINT('Ctrl Pts',(12.8769952998097,18.7835579840481,0.));
#249626=CARTESIAN_POINT('Ctrl Pts',(12.8722064211814,18.7739705329029,0.));
#249627=CARTESIAN_POINT('Ctrl Pts',(12.8674777239656,18.7645844169568,0.));
#249628=CARTESIAN_POINT('Ctrl Pts',(12.8628118054172,18.7554020493888,0.));
#249629=CARTESIAN_POINT('Ctrl Pts',(12.8582113455644,18.7464259171248,0.));
#249630=CARTESIAN_POINT('Ctrl Pts',(12.8536791086315,18.7376585820851,0.));
#249631=CARTESIAN_POINT('Ctrl Pts',(12.849217951159,18.7291026886552,0.));
#249632=CARTESIAN_POINT('Ctrl Pts',(12.8448308329494,18.7207609737701,0.));
#249633=CARTESIAN_POINT('Ctrl Pts',(12.8405208263432,18.7126362754446,0.));
#249634=CARTESIAN_POINT('Ctrl Pts',(12.8362911280362,18.7047315436296,0.));
#249635=CARTESIAN_POINT('Ctrl Pts',(12.832145059979,18.6970498410173,0.));
#249636=CARTESIAN_POINT('Ctrl Pts',(12.8280860635231,18.6895943376172,0.));
#249637=CARTESIAN_POINT('Ctrl Pts',(12.8241176980016,18.6823683094139,0.));
#249638=CARTESIAN_POINT('Ctrl Pts',(12.8202436318473,18.6753751301091,0.));
#249639=CARTESIAN_POINT('Ctrl Pts',(12.8164676687361,18.6686182952798,0.));
#249640=CARTESIAN_POINT('Ctrl Pts',(12.8127937909632,18.6621014624746,0.));
#249641=CARTESIAN_POINT('Ctrl Pts',(12.8092261933858,18.6558284825772,0.));
#249642=CARTESIAN_POINT('Ctrl Pts',(12.805769331162,18.6498034438986,0.));
#249643=CARTESIAN_POINT('Ctrl Pts',(12.8024278770153,18.6440306327457,0.));
#249644=CARTESIAN_POINT('Ctrl Pts',(12.7992066625264,18.63851447924,0.));
#249645=CARTESIAN_POINT('Ctrl Pts',(12.7961106222251,18.6332595057005,0.));
#249646=CARTESIAN_POINT('Ctrl Pts',(12.7931447451556,18.6282702819371,0.));
#249647=CARTESIAN_POINT('Ctrl Pts',(12.7903142925234,18.6235516265575,0.));
#249648=CARTESIAN_POINT('Ctrl Pts',(12.7876249657834,18.6191087624752,0.));
#249649=CARTESIAN_POINT('Ctrl Pts',(12.78508316579,18.6149475565189,0.));
#249650=CARTESIAN_POINT('Ctrl Pts',(12.7826959526924,18.611074482622,0.));
#249651=CARTESIAN_POINT('Ctrl Pts',(12.7804705387658,18.6074961535723,0.));
#249652=CARTESIAN_POINT('Ctrl Pts',(12.7784139605067,18.6042190183703,0.));
#249653=CARTESIAN_POINT('Ctrl Pts',(12.7765325225082,18.6012488486708,0.));
#249654=CARTESIAN_POINT('Ctrl Pts',(12.7748328937639,18.5985917525949,0.));
#249655=CARTESIAN_POINT('Ctrl Pts',(12.7733231262107,18.5962551167772,0.));
#249656=CARTESIAN_POINT('Ctrl Pts',(12.7720142287169,18.5942490615409,0.));
#249657=CARTESIAN_POINT('Ctrl Pts',(12.7709195951153,18.5925859134582,0.));
#249658=CARTESIAN_POINT('Ctrl Pts',(12.7700520897174,18.5912775137806,0.));
#249659=CARTESIAN_POINT('Ctrl Pts',(12.7694215127923,18.590332877722,0.));
#249660=CARTESIAN_POINT('Ctrl Pts',(12.7691103481996,18.589871621842,0.));
#249661=CARTESIAN_POINT('Ctrl Pts',(12.7689864266924,18.5896919669158,0.));
#249662=CARTESIAN_POINT('Ctrl Pts',(12.7689524524484,18.5896460962961,0.));
#249663=CARTESIAN_POINT('Ctrl Pts',(12.7689476255363,18.5896416359912,0.));
#249664=CARTESIAN_POINT('',(13.5685075571671,22.1787195904339,12.));
#249665=CARTESIAN_POINT('',(13.5685075571671,22.1787195904339,0.));
#249666=CARTESIAN_POINT('Ctrl Pts',(12.7689476255363,18.5896416359912,12.));
#249667=CARTESIAN_POINT('Ctrl Pts',(12.7689524524484,18.5896460962961,12.));
#249668=CARTESIAN_POINT('Ctrl Pts',(12.7689864266924,18.5896919669158,12.));
#249669=CARTESIAN_POINT('Ctrl Pts',(12.7691103481996,18.589871621842,12.));
#249670=CARTESIAN_POINT('Ctrl Pts',(12.7694215127923,18.590332877722,12.));
#249671=CARTESIAN_POINT('Ctrl Pts',(12.7700520897174,18.5912775137806,12.));
#249672=CARTESIAN_POINT('Ctrl Pts',(12.7709195951153,18.5925859134582,12.));
#249673=CARTESIAN_POINT('Ctrl Pts',(12.7720142287169,18.5942490615409,12.));
#249674=CARTESIAN_POINT('Ctrl Pts',(12.7733231262107,18.5962551167772,12.));
#249675=CARTESIAN_POINT('Ctrl Pts',(12.7748328937639,18.5985917525949,12.));
#249676=CARTESIAN_POINT('Ctrl Pts',(12.7765325225082,18.6012488486708,12.));
#249677=CARTESIAN_POINT('Ctrl Pts',(12.7784139605067,18.6042190183703,12.));
#249678=CARTESIAN_POINT('Ctrl Pts',(12.7804705387658,18.6074961535723,12.));
#249679=CARTESIAN_POINT('Ctrl Pts',(12.7826959526924,18.611074482622,12.));
#249680=CARTESIAN_POINT('Ctrl Pts',(12.78508316579,18.6149475565189,12.));
#249681=CARTESIAN_POINT('Ctrl Pts',(12.7876249657834,18.6191087624752,12.));
#249682=CARTESIAN_POINT('Ctrl Pts',(12.7903142925234,18.6235516265575,12.));
#249683=CARTESIAN_POINT('Ctrl Pts',(12.7931447451556,18.6282702819371,12.));
#249684=CARTESIAN_POINT('Ctrl Pts',(12.7961106222251,18.6332595057005,12.));
#249685=CARTESIAN_POINT('Ctrl Pts',(12.7992066625264,18.63851447924,12.));
#249686=CARTESIAN_POINT('Ctrl Pts',(12.8024278770153,18.6440306327457,12.));
#249687=CARTESIAN_POINT('Ctrl Pts',(12.805769331162,18.6498034438986,12.));
#249688=CARTESIAN_POINT('Ctrl Pts',(12.8092261933858,18.6558284825772,12.));
#249689=CARTESIAN_POINT('Ctrl Pts',(12.8127937909632,18.6621014624746,12.));
#249690=CARTESIAN_POINT('Ctrl Pts',(12.8164676687361,18.6686182952798,12.));
#249691=CARTESIAN_POINT('Ctrl Pts',(12.8202436318473,18.6753751301091,12.));
#249692=CARTESIAN_POINT('Ctrl Pts',(12.8241176980016,18.6823683094139,12.));
#249693=CARTESIAN_POINT('Ctrl Pts',(12.8280860635231,18.6895943376172,12.));
#249694=CARTESIAN_POINT('Ctrl Pts',(12.832145059979,18.6970498410173,12.));
#249695=CARTESIAN_POINT('Ctrl Pts',(12.8362911280362,18.7047315436296,12.));
#249696=CARTESIAN_POINT('Ctrl Pts',(12.8405208263432,18.7126362754446,12.));
#249697=CARTESIAN_POINT('Ctrl Pts',(12.8448308329494,18.7207609737701,12.));
#249698=CARTESIAN_POINT('Ctrl Pts',(12.849217951159,18.7291026886552,12.));
#249699=CARTESIAN_POINT('Ctrl Pts',(12.8536791086315,18.7376585820851,12.));
#249700=CARTESIAN_POINT('Ctrl Pts',(12.8582113455644,18.7464259171248,12.));
#249701=CARTESIAN_POINT('Ctrl Pts',(12.8628118054172,18.7554020493888,12.));
#249702=CARTESIAN_POINT('Ctrl Pts',(12.8674777239656,18.7645844169568,12.));
#249703=CARTESIAN_POINT('Ctrl Pts',(12.8722064211814,18.7739705329029,12.));
#249704=CARTESIAN_POINT('Ctrl Pts',(12.8769952998097,18.7835579840481,12.));
#249705=CARTESIAN_POINT('Ctrl Pts',(12.8818418427474,18.7933444285867,12.));
#249706=CARTESIAN_POINT('Ctrl Pts',(12.8867436109543,18.8033275941939,12.));
#249707=CARTESIAN_POINT('Ctrl Pts',(12.8916982409931,18.8135052757815,12.));
#249708=CARTESIAN_POINT('Ctrl Pts',(12.8967034410752,18.8238753319124,12.));
#249709=CARTESIAN_POINT('Ctrl Pts',(12.9017569871738,18.834435681259,12.));
#249710=CARTESIAN_POINT('Ctrl Pts',(12.9068567191856,18.8451842990986,12.));
#249711=CARTESIAN_POINT('Ctrl Pts',(12.9120005369066,18.8561192136201,12.));
#249712=CARTESIAN_POINT('Ctrl Pts',(12.9171863977047,18.8672385038328,12.));
#249713=CARTESIAN_POINT('Ctrl Pts',(12.9224123144982,18.8785402977528,12.));
#249714=CARTESIAN_POINT('Ctrl Pts',(12.9276763536372,18.8900227704888,12.));
#249715=CARTESIAN_POINT('Ctrl Pts',(12.9329766328184,18.9016841423402,12.));
#249716=CARTESIAN_POINT('Ctrl Pts',(12.9383113190375,18.9135226769466,12.));
#249717=CARTESIAN_POINT('Ctrl Pts',(12.9436786266106,18.9255366795196,12.));
#249718=CARTESIAN_POINT('Ctrl Pts',(12.9490768151821,18.9377244950435,12.));
#249719=CARTESIAN_POINT('Ctrl Pts',(12.9545041877377,18.9500845064714,12.));
#249720=CARTESIAN_POINT('Ctrl Pts',(12.9599590886317,18.9626151329226,12.));
#249721=CARTESIAN_POINT('Ctrl Pts',(12.9654399021868,18.9753148284473,12.));
#249722=CARTESIAN_POINT('Ctrl Pts',(12.9709450512747,18.9881820807585,12.));
#249723=CARTESIAN_POINT('Ctrl Pts',(12.9764729959206,19.0012154099792,12.));
#249724=CARTESIAN_POINT('Ctrl Pts',(12.9820222318716,19.014413367335,12.));
#249725=CARTESIAN_POINT('Ctrl Pts',(12.9875912893003,19.0277745339909,12.));
#249726=CARTESIAN_POINT('Ctrl Pts',(12.9931787316514,19.0412975200398,12.));
#249727=CARTESIAN_POINT('Ctrl Pts',(12.9987831544502,19.0549809634354,12.));
#249728=CARTESIAN_POINT('Ctrl Pts',(13.0044031841382,19.0688235289437,12.));
#249729=CARTESIAN_POINT('Ctrl Pts',(13.0100374768788,19.0828239070484,12.));
#249730=CARTESIAN_POINT('Ctrl Pts',(13.0156847176096,19.0969808131228,12.));
#249731=CARTESIAN_POINT('Ctrl Pts',(13.0213436191328,19.111292986631,12.));
#249732=CARTESIAN_POINT('Ctrl Pts',(13.0270129211976,19.1257591903099,12.));
#249733=CARTESIAN_POINT('Ctrl Pts',(13.0326913895838,19.1403782093386,12.));
#249734=CARTESIAN_POINT('Ctrl Pts',(13.0383778152068,19.155148850523,12.));
#249735=CARTESIAN_POINT('Ctrl Pts',(13.0440710133772,19.1700699416622,12.));
#249736=CARTESIAN_POINT('Ctrl Pts',(13.0497698230441,19.1851403308825,12.));
#249737=CARTESIAN_POINT('Ctrl Pts',(13.0554731060538,19.2003588859772,12.));
#249738=CARTESIAN_POINT('Ctrl Pts',(13.0611797463915,19.2157244937142,12.));
#249739=CARTESIAN_POINT('Ctrl Pts',(13.0668886494795,19.2312360592033,12.));
#249740=CARTESIAN_POINT('Ctrl Pts',(13.0725987415859,19.2468925053989,12.));
#249741=CARTESIAN_POINT('Ctrl Pts',(13.0783089692118,19.2626927725596,12.));
#249742=CARTESIAN_POINT('Ctrl Pts',(13.0840182984949,19.2786358177198,12.));
#249743=CARTESIAN_POINT('Ctrl Pts',(13.0897257145968,19.2947206141247,12.));
#249744=CARTESIAN_POINT('Ctrl Pts',(13.0954302211479,19.310946150736,12.));
#249745=CARTESIAN_POINT('Ctrl Pts',(13.1011308397591,19.3273114318269,12.));
#249746=CARTESIAN_POINT('Ctrl Pts',(13.1068266095186,19.3438154765395,12.));
#249747=CARTESIAN_POINT('Ctrl Pts',(13.1125165865022,19.3604573184515,12.));
#249748=CARTESIAN_POINT('Ctrl Pts',(13.118199843271,19.3772360051091,12.));
#249749=CARTESIAN_POINT('Ctrl Pts',(13.1238754684177,19.3941505976263,12.));
#249750=CARTESIAN_POINT('Ctrl Pts',(13.1295425661634,19.4112001703557,12.));
#249751=CARTESIAN_POINT('Ctrl Pts',(13.1352002559438,19.4283838105262,12.));
#249752=CARTESIAN_POINT('Ctrl Pts',(13.1408476720061,19.4457006178876,12.));
#249753=CARTESIAN_POINT('Ctrl Pts',(13.1464839629971,19.4631497043258,12.));
#249754=CARTESIAN_POINT('Ctrl Pts',(13.1521082915853,19.4807301935268,12.));
#249755=CARTESIAN_POINT('Ctrl Pts',(13.1577198341245,19.4984412207082,12.));
#249756=CARTESIAN_POINT('Ctrl Pts',(13.1633177803101,19.5162819323213,12.));
#249757=CARTESIAN_POINT('Ctrl Pts',(13.168901332843,19.5342514857562,12.));
#249758=CARTESIAN_POINT('Ctrl Pts',(13.1744697070911,19.5523490490244,12.));
#249759=CARTESIAN_POINT('Ctrl Pts',(13.1800221307673,19.5705738004667,12.));
#249760=CARTESIAN_POINT('Ctrl Pts',(13.1855578436471,19.5889249285338,12.));
#249761=CARTESIAN_POINT('Ctrl Pts',(13.1910760972814,19.6074016315414,12.));
#249762=CARTESIAN_POINT('Ctrl Pts',(13.1965761547151,19.6260031174244,12.));
#249763=CARTESIAN_POINT('Ctrl Pts',(13.2020572902065,19.6447286034772,12.));
#249764=CARTESIAN_POINT('Ctrl Pts',(13.2075187889529,19.6635773160936,12.));
#249765=CARTESIAN_POINT('Ctrl Pts',(13.2129599468485,19.6825484905823,12.));
#249766=CARTESIAN_POINT('Ctrl Pts',(13.2183800702436,19.7016413709685,12.));
#249767=CARTESIAN_POINT('Ctrl Pts',(13.2237784757065,19.7208552097868,12.));
#249768=CARTESIAN_POINT('Ctrl Pts',(13.2291544897899,19.7401892678697,12.));
#249769=CARTESIAN_POINT('Ctrl Pts',(13.2345074487963,19.7596428141168,12.));
#249770=CARTESIAN_POINT('Ctrl Pts',(13.2398366985675,19.7792151253289,12.));
#249771=CARTESIAN_POINT('Ctrl Pts',(13.2451415942805,19.7989054860495,12.));
#249772=CARTESIAN_POINT('Ctrl Pts',(13.2504215002457,19.8187131883917,12.));
#249773=CARTESIAN_POINT('Ctrl Pts',(13.2556757897086,19.8386375318634,12.));
#249774=CARTESIAN_POINT('Ctrl Pts',(13.2609038446529,19.8586778231715,12.));
#249775=CARTESIAN_POINT('Ctrl Pts',(13.2661050556132,19.8788333760577,12.));
#249776=CARTESIAN_POINT('Ctrl Pts',(13.271278821502,19.8991035111745,12.));
#249777=CARTESIAN_POINT('Ctrl Pts',(13.2764245494357,19.9194875559422,12.));
#249778=CARTESIAN_POINT('Ctrl Pts',(13.2815416545663,19.9399848444019,12.));
#249779=CARTESIAN_POINT('Ctrl Pts',(13.286629559915,19.9605947170586,12.));
#249780=CARTESIAN_POINT('Ctrl Pts',(13.2916876962094,19.981316520717,12.));
#249781=CARTESIAN_POINT('Ctrl Pts',(13.2967155017306,20.0021496083738,12.));
#249782=CARTESIAN_POINT('Ctrl Pts',(13.3017124221637,20.0230933391038,12.));
#249783=CARTESIAN_POINT('Ctrl Pts',(13.3066779104515,20.0441470779345,12.));
#249784=CARTESIAN_POINT('Ctrl Pts',(13.3116114266515,20.0653101957188,12.));
#249785=CARTESIAN_POINT('Ctrl Pts',(13.3165124377962,20.0865820689883,12.));
#249786=CARTESIAN_POINT('Ctrl Pts',(13.3213804177587,20.1079620798375,12.));
#249787=CARTESIAN_POINT('Ctrl Pts',(13.3262148471226,20.1294496158402,12.));
#249788=CARTESIAN_POINT('Ctrl Pts',(13.3310152130564,20.1510440699474,12.));
#249789=CARTESIAN_POINT('Ctrl Pts',(13.3357810091903,20.1727448403817,12.));
#249790=CARTESIAN_POINT('Ctrl Pts',(13.3405117354971,20.1945513305235,12.));
#249791=CARTESIAN_POINT('Ctrl Pts',(13.3452068981766,20.216462948786,12.));
#249792=CARTESIAN_POINT('Ctrl Pts',(13.3498660095386,20.2384791085359,12.));
#249793=CARTESIAN_POINT('Ctrl Pts',(13.3544885878889,20.2605992280122,12.));
#249794=CARTESIAN_POINT('Ctrl Pts',(13.3590741574195,20.2828227302339,12.));
#249795=CARTESIAN_POINT('Ctrl Pts',(13.3636222481016,20.3051490429048,12.));
#249796=CARTESIAN_POINT('Ctrl Pts',(13.3681323955826,20.3275775983029,12.));
#249797=CARTESIAN_POINT('Ctrl Pts',(13.3726041410867,20.3501078331814,12.));
#249798=CARTESIAN_POINT('Ctrl Pts',(13.3770370313188,20.3727391887184,12.));
#249799=CARTESIAN_POINT('Ctrl Pts',(13.3814306183719,20.3954711104502,12.));
#249800=CARTESIAN_POINT('Ctrl Pts',(13.3857844596387,20.4183030482002,12.));
#249801=CARTESIAN_POINT('Ctrl Pts',(13.3900981177255,20.4412344560008,12.));
#249802=CARTESIAN_POINT('Ctrl Pts',(13.3943711603739,20.4642647920038,12.));
#249803=CARTESIAN_POINT('Ctrl Pts',(13.3986031603716,20.487393518404,12.));
#249804=CARTESIAN_POINT('Ctrl Pts',(13.4027936954529,20.5106201013753,12.));
#249805=CARTESIAN_POINT('Ctrl Pts',(13.4069423482076,20.5339440109956,12.));
#249806=CARTESIAN_POINT('Ctrl Pts',(13.4110487059912,20.5573647211639,12.));
#249807=CARTESIAN_POINT('Ctrl Pts',(13.4151123608411,20.5808817095155,12.));
#249808=CARTESIAN_POINT('Ctrl Pts',(13.4191329093932,20.6044944573153,12.));
#249809=CARTESIAN_POINT('Ctrl Pts',(13.4231099528179,20.6282024494237,12.));
#249810=CARTESIAN_POINT('Ctrl Pts',(13.4270430967651,20.6520051742869,12.));
#249811=CARTESIAN_POINT('Ctrl Pts',(13.4309319513119,20.6759021239103,12.));
#249812=CARTESIAN_POINT('Ctrl Pts',(13.4347761309154,20.6998927938288,12.));
#249813=CARTESIAN_POINT('Ctrl Pts',(13.4385752543663,20.7239766830675,12.));
#249814=CARTESIAN_POINT('Ctrl Pts',(13.4423289447561,20.7481532941013,12.));
#249815=CARTESIAN_POINT('Ctrl Pts',(13.4460368293688,20.7724221327608,12.));
#249816=CARTESIAN_POINT('Ctrl Pts',(13.4496985395637,20.7967827081227,12.));
#249817=CARTESIAN_POINT('Ctrl Pts',(13.4533137106667,20.821234532398,12.));
#249818=CARTESIAN_POINT('Ctrl Pts',(13.4568819818631,20.8457771208082,12.));
#249819=CARTESIAN_POINT('Ctrl Pts',(13.4604029960983,20.8704099914641,12.));
#249820=CARTESIAN_POINT('Ctrl Pts',(13.4638763999725,20.8951326652158,12.));
#249821=CARTESIAN_POINT('Ctrl Pts',(13.4673018437718,20.9199446657584,12.));
#249822=CARTESIAN_POINT('Ctrl Pts',(13.4706789815166,20.9448455197557,12.));
#249823=CARTESIAN_POINT('Ctrl Pts',(13.4740074710087,20.9698347569476,12.));
#249824=CARTESIAN_POINT('Ctrl Pts',(13.4772869738879,20.9949119102592,12.));
#249825=CARTESIAN_POINT('Ctrl Pts',(13.4805171556822,21.0200765158885,12.));
#249826=CARTESIAN_POINT('Ctrl Pts',(13.4836976858912,21.0453281134247,12.));
#249827=CARTESIAN_POINT('Ctrl Pts',(13.4868282377191,21.0706662455202,12.));
#249828=CARTESIAN_POINT('Ctrl Pts',(13.4899084877718,21.0960904575048,12.));
#249829=CARTESIAN_POINT('Ctrl Pts',(13.4929381157778,21.1216002970209,12.));
#249830=CARTESIAN_POINT('Ctrl Pts',(13.4959168042934,21.1471953136209,12.));
#249831=CARTESIAN_POINT('Ctrl Pts',(13.4988442384491,21.1728750584173,12.));
#249832=CARTESIAN_POINT('Ctrl Pts',(13.5017201056088,21.1986390835825,12.));
#249833=CARTESIAN_POINT('Ctrl Pts',(13.5045440957404,21.224486942933,12.));
#249834=CARTESIAN_POINT('Ctrl Pts',(13.5073159019454,21.2504181927429,12.));
#249835=CARTESIAN_POINT('Ctrl Pts',(13.5100352209207,21.2764323924442,12.));
#249836=CARTESIAN_POINT('Ctrl Pts',(13.5127017534972,21.3025291054236,12.));
#249837=CARTESIAN_POINT('Ctrl Pts',(13.5153152050554,21.328707899634,12.));
#249838=CARTESIAN_POINT('Ctrl Pts',(13.5178752862461,21.3549683486219,12.));
#249839=CARTESIAN_POINT('Ctrl Pts',(13.5203817122496,21.3813100304967,12.));
#249840=CARTESIAN_POINT('Ctrl Pts',(13.5228342013508,21.4077325259318,12.));
#249841=CARTESIAN_POINT('Ctrl Pts',(13.5252324737795,21.4342354165254,12.));
#249842=CARTESIAN_POINT('Ctrl Pts',(13.5275762503553,21.4608182828695,12.));
#249843=CARTESIAN_POINT('Ctrl Pts',(13.5298652514357,21.487480703047,12.));
#249844=CARTESIAN_POINT('Ctrl Pts',(13.5320991952145,21.5142222501671,12.));
#249845=CARTESIAN_POINT('Ctrl Pts',(13.5342777983225,21.5410424932511,12.));
#249846=CARTESIAN_POINT('Ctrl Pts',(13.5364007790292,21.5679410019011,12.));
#249847=CARTESIAN_POINT('Ctrl Pts',(13.5384678597206,21.5949173499022,12.));
#249848=CARTESIAN_POINT('Ctrl Pts',(13.5404787697798,21.6219711193951,12.));
#249849=CARTESIAN_POINT('Ctrl Pts',(13.5424332480698,21.6491019044647,12.));
#249850=CARTESIAN_POINT('Ctrl Pts',(13.5443310461516,21.676309315769,12.));
#249851=CARTESIAN_POINT('Ctrl Pts',(13.546171929503,21.7035929822939,12.));
#249852=CARTESIAN_POINT('Ctrl Pts',(13.5479556704457,21.730952541226,12.));
#249853=CARTESIAN_POINT('Ctrl Pts',(13.5496820422186,21.7583876294532,12.));
#249854=CARTESIAN_POINT('Ctrl Pts',(13.5513508127232,21.7858978745848,12.));
#249855=CARTESIAN_POINT('Ctrl Pts',(13.5529617381569,21.8134828857963,12.));
#249856=CARTESIAN_POINT('Ctrl Pts',(13.5545145573048,21.841142245609,12.));
#249857=CARTESIAN_POINT('Ctrl Pts',(13.5560089839426,21.8688754989401,12.));
#249858=CARTESIAN_POINT('Ctrl Pts',(13.5574447178484,21.8966821688876,12.));
#249859=CARTESIAN_POINT('Ctrl Pts',(13.5588214586672,21.9245617765827,12.));
#249860=CARTESIAN_POINT('Ctrl Pts',(13.5601389185315,21.9525138592862,12.));
#249861=CARTESIAN_POINT('Ctrl Pts',(13.5613968357589,21.9805379899192,12.));
#249862=CARTESIAN_POINT('Ctrl Pts',(13.5625949868313,22.0086337943431,12.));
#249863=CARTESIAN_POINT('Ctrl Pts',(13.5637332022393,22.0368009736227,12.));
#249864=CARTESIAN_POINT('Ctrl Pts',(13.5648113688894,22.0650393089492,12.));
#249865=CARTESIAN_POINT('Ctrl Pts',(13.5658294169106,22.0933486464442,12.));
#249866=CARTESIAN_POINT('Ctrl Pts',(13.5667873105179,22.1217288871823,12.));
#249867=CARTESIAN_POINT('Ctrl Pts',(13.5675054918922,22.1444897575076,12.));
#249868=CARTESIAN_POINT('Ctrl Pts',(13.5680170531724,22.1615922804939,12.));
#249869=CARTESIAN_POINT('Ctrl Pts',(13.5683460612913,22.1730081264583,12.));
#249870=CARTESIAN_POINT('Ctrl Pts',(13.5685075571671,22.1787195904339,12.));
#249871=CARTESIAN_POINT('Ctrl Pts',(14.6513681262571,17.1452095830633,0.));
#249872=CARTESIAN_POINT('Ctrl Pts',(14.6513681262571,17.1452095830633,12.));
#249873=CARTESIAN_POINT('Ctrl Pts',(14.6513711852843,17.1452153999142,0.));
#249874=CARTESIAN_POINT('Ctrl Pts',(14.6513711852843,17.1452153999142,12.));
#249875=CARTESIAN_POINT('Ctrl Pts',(14.6514066997196,17.1452600887037,0.));
#249876=CARTESIAN_POINT('Ctrl Pts',(14.6514066997196,17.1452600887037,12.));
#249877=CARTESIAN_POINT('Ctrl Pts',(14.6515481598068,17.1454262858043,0.));
#249878=CARTESIAN_POINT('Ctrl Pts',(14.6515481598068,17.1454262858043,12.));
#249879=CARTESIAN_POINT('Ctrl Pts',(14.6519131634508,17.1458462295271,0.));
#249880=CARTESIAN_POINT('Ctrl Pts',(14.6519131634508,17.1458462295271,12.));
#249881=CARTESIAN_POINT('Ctrl Pts',(14.6526624064978,17.1466998098673,0.));
#249882=CARTESIAN_POINT('Ctrl Pts',(14.6526624064978,17.1466998098673,12.));
#249883=CARTESIAN_POINT('Ctrl Pts',(14.6537016966184,17.147876394491,0.));
#249884=CARTESIAN_POINT('Ctrl Pts',(14.6537016966184,17.147876394491,12.));
#249885=CARTESIAN_POINT('Ctrl Pts',(14.655024862281,17.1493641837558,0.));
#249886=CARTESIAN_POINT('Ctrl Pts',(14.655024862281,17.1493641837558,12.));
#249887=CARTESIAN_POINT('Ctrl Pts',(14.6566237952435,17.1511476869496,0.));
#249888=CARTESIAN_POINT('Ctrl Pts',(14.6566237952435,17.1511476869496,12.));
#249889=CARTESIAN_POINT('Ctrl Pts',(14.6584900555302,17.1532107762718,0.));
#249890=CARTESIAN_POINT('Ctrl Pts',(14.6584900555302,17.1532107762718,12.));
#249891=CARTESIAN_POINT('Ctrl Pts',(14.6606167169642,17.1555401986401,0.));
#249892=CARTESIAN_POINT('Ctrl Pts',(14.6606167169642,17.1555401986401,12.));
#249893=CARTESIAN_POINT('Ctrl Pts',(14.6629987285992,17.1581262646789,0.));
#249894=CARTESIAN_POINT('Ctrl Pts',(14.6629987285992,17.1581262646789,12.));
#249895=CARTESIAN_POINT('Ctrl Pts',(14.6656319165057,17.1609609517369,0.));
#249896=CARTESIAN_POINT('Ctrl Pts',(14.6656319165057,17.1609609517369,12.));
#249897=CARTESIAN_POINT('Ctrl Pts',(14.6685123374423,17.1640366762305,0.));
#249898=CARTESIAN_POINT('Ctrl Pts',(14.6685123374423,17.1640366762305,12.));
#249899=CARTESIAN_POINT('Ctrl Pts',(14.671635583332,17.167344972302,0.));
#249900=CARTESIAN_POINT('Ctrl Pts',(14.671635583332,17.167344972302,12.));
#249901=CARTESIAN_POINT('Ctrl Pts',(14.6749971333867,17.1708771619129,0.));
#249902=CARTESIAN_POINT('Ctrl Pts',(14.6749971333867,17.1708771619129,12.));
#249903=CARTESIAN_POINT('Ctrl Pts',(14.6785925615677,17.1746247499057,0.));
#249904=CARTESIAN_POINT('Ctrl Pts',(14.6785925615677,17.1746247499057,12.));
#249905=CARTESIAN_POINT('Ctrl Pts',(14.6824178576167,17.1785800350826,0.));
#249906=CARTESIAN_POINT('Ctrl Pts',(14.6824178576167,17.1785800350826,12.));
#249907=CARTESIAN_POINT('Ctrl Pts',(14.686469452232,17.182736158472,0.));
#249908=CARTESIAN_POINT('Ctrl Pts',(14.686469452232,17.182736158472,12.));
#249909=CARTESIAN_POINT('Ctrl Pts',(14.6907440526958,17.1870867909918,0.));
#249910=CARTESIAN_POINT('Ctrl Pts',(14.6907440526958,17.1870867909918,12.));
#249911=CARTESIAN_POINT('Ctrl Pts',(14.6952385361705,17.1916259308415,0.));
#249912=CARTESIAN_POINT('Ctrl Pts',(14.6952385361705,17.1916259308415,12.));
#249913=CARTESIAN_POINT('Ctrl Pts',(14.699949811582,17.1963476411694,0.));
#249914=CARTESIAN_POINT('Ctrl Pts',(14.699949811582,17.1963476411694,12.));
#249915=CARTESIAN_POINT('Ctrl Pts',(14.7048748502663,17.2012461084268,0.));
#249916=CARTESIAN_POINT('Ctrl Pts',(14.7048748502663,17.2012461084268,12.));
#249917=CARTESIAN_POINT('Ctrl Pts',(14.7100107213586,17.2063157097315,0.));
#249918=CARTESIAN_POINT('Ctrl Pts',(14.7100107213586,17.2063157097315,12.));
#249919=CARTESIAN_POINT('Ctrl Pts',(14.7153546289339,17.2115510835989,0.));
#249920=CARTESIAN_POINT('Ctrl Pts',(14.7153546289339,17.2115510835989,12.));
#249921=CARTESIAN_POINT('Ctrl Pts',(14.7209039390327,17.2169471814256,0.));
#249922=CARTESIAN_POINT('Ctrl Pts',(14.7209039390327,17.2169471814256,12.));
#249923=CARTESIAN_POINT('Ctrl Pts',(14.7266561494282,17.2224992099667,0.));
#249924=CARTESIAN_POINT('Ctrl Pts',(14.7266561494282,17.2224992099667,12.));
#249925=CARTESIAN_POINT('Ctrl Pts',(14.7326088681163,17.2282025904314,0.));
#249926=CARTESIAN_POINT('Ctrl Pts',(14.7326088681163,17.2282025904314,12.));
#249927=CARTESIAN_POINT('Ctrl Pts',(14.7387597858116,17.2340529062076,0.));
#249928=CARTESIAN_POINT('Ctrl Pts',(14.7387597858116,17.2340529062076,12.));
#249929=CARTESIAN_POINT('Ctrl Pts',(14.7451066593792,17.2400458713565,0.));
#249930=CARTESIAN_POINT('Ctrl Pts',(14.7451066593792,17.2400458713565,12.));
#249931=CARTESIAN_POINT('Ctrl Pts',(14.7516473175124,17.2461773413288,0.));
#249932=CARTESIAN_POINT('Ctrl Pts',(14.7516473175124,17.2461773413288,12.));
#249933=CARTESIAN_POINT('Ctrl Pts',(14.7583796616617,17.2524433146837,0.));
#249934=CARTESIAN_POINT('Ctrl Pts',(14.7583796616617,17.2524433146837,12.));
#249935=CARTESIAN_POINT('Ctrl Pts',(14.7653016697591,17.2588399401465,0.));
#249936=CARTESIAN_POINT('Ctrl Pts',(14.7653016697591,17.2588399401465,12.));
#249937=CARTESIAN_POINT('Ctrl Pts',(14.7724113956731,17.2653635155319,0.));
#249938=CARTESIAN_POINT('Ctrl Pts',(14.7724113956731,17.2653635155319,12.));
#249939=CARTESIAN_POINT('Ctrl Pts',(14.7797069617804,17.2720104735194,0.));
#249940=CARTESIAN_POINT('Ctrl Pts',(14.7797069617804,17.2720104735194,12.));
#249941=CARTESIAN_POINT('Ctrl Pts',(14.787186553128,17.2787773704849,0.));
#249942=CARTESIAN_POINT('Ctrl Pts',(14.787186553128,17.2787773704849,12.));
#249943=CARTESIAN_POINT('Ctrl Pts',(14.7948484105249,17.2856608733196,0.));
#249944=CARTESIAN_POINT('Ctrl Pts',(14.7948484105249,17.2856608733196,12.));
#249945=CARTESIAN_POINT('Ctrl Pts',(14.8026908254276,17.2926577496513,0.));
#249946=CARTESIAN_POINT('Ctrl Pts',(14.8026908254276,17.2926577496513,12.));
#249947=CARTESIAN_POINT('Ctrl Pts',(14.8107121391035,17.299764866148,0.));
#249948=CARTESIAN_POINT('Ctrl Pts',(14.8107121391035,17.299764866148,12.));
#249949=CARTESIAN_POINT('Ctrl Pts',(14.8189107410162,17.3069791853706,0.));
#249950=CARTESIAN_POINT('Ctrl Pts',(14.8189107410162,17.3069791853706,12.));
#249951=CARTESIAN_POINT('Ctrl Pts',(14.8272850675379,17.3142977632659,0.));
#249952=CARTESIAN_POINT('Ctrl Pts',(14.8272850675379,17.3142977632659,12.));
#249953=CARTESIAN_POINT('Ctrl Pts',(14.8358336004197,17.3217177462101,0.));
#249954=CARTESIAN_POINT('Ctrl Pts',(14.8358336004197,17.3217177462101,12.));
#249955=CARTESIAN_POINT('Ctrl Pts',(14.8445548643508,17.3292363662605,0.));
#249956=CARTESIAN_POINT('Ctrl Pts',(14.8445548643508,17.3292363662605,12.));
#249957=CARTESIAN_POINT('Ctrl Pts',(14.8534474245433,17.336850936485,0.));
#249958=CARTESIAN_POINT('Ctrl Pts',(14.8534474245433,17.336850936485,12.));
#249959=CARTESIAN_POINT('Ctrl Pts',(14.8625098843417,17.3445588463475,0.));
#249960=CARTESIAN_POINT('Ctrl Pts',(14.8625098843417,17.3445588463475,12.));
#249961=CARTESIAN_POINT('Ctrl Pts',(14.8717408826955,17.3523575568645,0.));
#249962=CARTESIAN_POINT('Ctrl Pts',(14.8717408826955,17.3523575568645,12.));
#249963=CARTESIAN_POINT('Ctrl Pts',(14.8811390927423,17.3602445978161,0.));
#249964=CARTESIAN_POINT('Ctrl Pts',(14.8811390927423,17.3602445978161,12.));
#249965=CARTESIAN_POINT('Ctrl Pts',(14.8907032205788,17.3682175653235,0.));
#249966=CARTESIAN_POINT('Ctrl Pts',(14.8907032205788,17.3682175653235,12.));
#249967=CARTESIAN_POINT('Ctrl Pts',(14.900432003961,17.3762741193076,0.));
#249968=CARTESIAN_POINT('Ctrl Pts',(14.900432003961,17.3762741193076,12.));
#249969=CARTESIAN_POINT('Ctrl Pts',(14.9103242110057,17.3844119809824,0.));
#249970=CARTESIAN_POINT('Ctrl Pts',(14.9103242110057,17.3844119809824,12.));
#249971=CARTESIAN_POINT('Ctrl Pts',(14.9203786389342,17.3926289303986,0.));
#249972=CARTESIAN_POINT('Ctrl Pts',(14.9203786389342,17.3926289303986,12.));
#249973=CARTESIAN_POINT('Ctrl Pts',(14.9305941128757,17.4009228040749,0.));
#249974=CARTESIAN_POINT('Ctrl Pts',(14.9305941128757,17.4009228040749,12.));
#249975=CARTESIAN_POINT('Ctrl Pts',(14.940969484645,17.4092914926071,0.));
#249976=CARTESIAN_POINT('Ctrl Pts',(14.940969484645,17.4092914926071,12.));
#249977=CARTESIAN_POINT('Ctrl Pts',(14.9515036315143,17.4177329382828,0.));
#249978=CARTESIAN_POINT('Ctrl Pts',(14.9515036315143,17.4177329382828,12.));
#249979=CARTESIAN_POINT('Ctrl Pts',(14.9621954549827,17.426245132709,0.));
#249980=CARTESIAN_POINT('Ctrl Pts',(14.9621954549827,17.426245132709,12.));
#249981=CARTESIAN_POINT('Ctrl Pts',(14.9730438799452,17.4348261151396,0.));
#249982=CARTESIAN_POINT('Ctrl Pts',(14.9730438799452,17.4348261151396,12.));
#249983=CARTESIAN_POINT('Ctrl Pts',(14.9840478538358,17.4434739707773,0.));
#249984=CARTESIAN_POINT('Ctrl Pts',(14.9840478538358,17.4434739707773,12.));
#249985=CARTESIAN_POINT('Ctrl Pts',(14.9952063457778,17.4521868291004,0.));
#249986=CARTESIAN_POINT('Ctrl Pts',(14.9952063457778,17.4521868291004,12.));
#249987=CARTESIAN_POINT('Ctrl Pts',(15.0065183456921,17.4609628621418,0.));
#249988=CARTESIAN_POINT('Ctrl Pts',(15.0065183456921,17.4609628621418,12.));
#249989=CARTESIAN_POINT('Ctrl Pts',(15.0179828635086,17.4698002829357,0.));
#249990=CARTESIAN_POINT('Ctrl Pts',(15.0179828635086,17.4698002829357,12.));
#249991=CARTESIAN_POINT('Ctrl Pts',(15.029598928488,17.4786973441417,0.));
#249992=CARTESIAN_POINT('Ctrl Pts',(15.029598928488,17.4786973441417,12.));
#249993=CARTESIAN_POINT('Ctrl Pts',(15.0413655884993,17.4876523366178,0.));
#249994=CARTESIAN_POINT('Ctrl Pts',(15.0413655884993,17.4876523366178,12.));
#249995=CARTESIAN_POINT('Ctrl Pts',(15.0532819093085,17.4966635880245,0.));
#249996=CARTESIAN_POINT('Ctrl Pts',(15.0532819093085,17.4966635880245,12.));
#249997=CARTESIAN_POINT('Ctrl Pts',(15.0653469738306,17.5057294613874,0.));
#249998=CARTESIAN_POINT('Ctrl Pts',(15.0653469738306,17.5057294613874,12.));
#249999=CARTESIAN_POINT('Ctrl Pts',(15.0775598815748,17.5148483539684,0.));
#250000=CARTESIAN_POINT('Ctrl Pts',(15.0775598815748,17.5148483539684,12.));
#250001=CARTESIAN_POINT('Ctrl Pts',(15.0899197481082,17.5240186961788,0.));
#250002=CARTESIAN_POINT('Ctrl Pts',(15.0899197481082,17.5240186961788,12.));
#250003=CARTESIAN_POINT('Ctrl Pts',(15.1024257045033,17.5332389504829,0.));
#250004=CARTESIAN_POINT('Ctrl Pts',(15.1024257045033,17.5332389504829,12.));
#250005=CARTESIAN_POINT('Ctrl Pts',(15.1150768967729,17.5425076102966,0.));
#250006=CARTESIAN_POINT('Ctrl Pts',(15.1150768967729,17.5425076102966,12.));
#250007=CARTESIAN_POINT('Ctrl Pts',(15.127872485314,17.5518231989122,0.));
#250008=CARTESIAN_POINT('Ctrl Pts',(15.127872485314,17.5518231989122,12.));
#250009=CARTESIAN_POINT('Ctrl Pts',(15.1408116444877,17.5611842686196,0.));
#250010=CARTESIAN_POINT('Ctrl Pts',(15.1408116444877,17.5611842686196,12.));
#250011=CARTESIAN_POINT('Ctrl Pts',(15.1538935621714,17.570589399803,0.));
#250012=CARTESIAN_POINT('Ctrl Pts',(15.1538935621714,17.570589399803,12.));
#250013=CARTESIAN_POINT('Ctrl Pts',(15.1671174393136,17.5800372000539,0.));
#250014=CARTESIAN_POINT('Ctrl Pts',(15.1671174393136,17.5800372000539,12.));
#250015=CARTESIAN_POINT('Ctrl Pts',(15.1804824894605,17.5895263032592,0.));
#250016=CARTESIAN_POINT('Ctrl Pts',(15.1804824894605,17.5895263032592,12.));
#250017=CARTESIAN_POINT('Ctrl Pts',(15.1939879383268,17.5990553687595,0.));
#250018=CARTESIAN_POINT('Ctrl Pts',(15.1939879383268,17.5990553687595,12.));
#250019=CARTESIAN_POINT('Ctrl Pts',(15.2076330234686,17.6086230806497,0.));
#250020=CARTESIAN_POINT('Ctrl Pts',(15.2076330234686,17.6086230806497,12.));
#250021=CARTESIAN_POINT('Ctrl Pts',(15.22141699392,17.6182281470467,0.));
#250022=CARTESIAN_POINT('Ctrl Pts',(15.22141699392,17.6182281470467,12.));
#250023=CARTESIAN_POINT('Ctrl Pts',(15.2353391098367,17.6278692993765,0.));
#250024=CARTESIAN_POINT('Ctrl Pts',(15.2353391098367,17.6278692993765,12.));
#250025=CARTESIAN_POINT('Ctrl Pts',(15.2493986421091,17.637545291637,0.));
#250026=CARTESIAN_POINT('Ctrl Pts',(15.2493986421091,17.637545291637,12.));
#250027=CARTESIAN_POINT('Ctrl Pts',(15.263594872029,17.6472548997329,0.));
#250028=CARTESIAN_POINT('Ctrl Pts',(15.263594872029,17.6472548997329,12.));
#250029=CARTESIAN_POINT('Ctrl Pts',(15.2779270910238,17.6569969209,0.));
#250030=CARTESIAN_POINT('Ctrl Pts',(15.2779270910238,17.6569969209,12.));
#250031=CARTESIAN_POINT('Ctrl Pts',(15.2923946003598,17.6667701731041,0.));
#250032=CARTESIAN_POINT('Ctrl Pts',(15.2923946003598,17.6667701731041,12.));
#250033=CARTESIAN_POINT('Ctrl Pts',(15.3069967108501,17.6765734944559,0.));
#250034=CARTESIAN_POINT('Ctrl Pts',(15.3069967108501,17.6765734944559,12.));
#250035=CARTESIAN_POINT('Ctrl Pts',(15.3217327425341,17.6864057426052,0.));
#250036=CARTESIAN_POINT('Ctrl Pts',(15.3217327425341,17.6864057426052,12.));
#250037=CARTESIAN_POINT('Ctrl Pts',(15.3366020244069,17.6962657941984,0.));
#250038=CARTESIAN_POINT('Ctrl Pts',(15.3366020244069,17.6962657941984,12.));
#250039=CARTESIAN_POINT('Ctrl Pts',(15.3516038942064,17.7061525444044,0.));
#250040=CARTESIAN_POINT('Ctrl Pts',(15.3516038942064,17.7061525444044,12.));
#250041=CARTESIAN_POINT('Ctrl Pts',(15.3667376981702,17.7160649064208,0.));
#250042=CARTESIAN_POINT('Ctrl Pts',(15.3667376981702,17.7160649064208,12.));
#250043=CARTESIAN_POINT('Ctrl Pts',(15.3820027907965,17.7260018109923,0.));
#250044=CARTESIAN_POINT('Ctrl Pts',(15.3820027907965,17.7260018109923,12.));
#250045=CARTESIAN_POINT('Ctrl Pts',(15.3973985345796,17.7359622059143,0.));
#250046=CARTESIAN_POINT('Ctrl Pts',(15.3973985345796,17.7359622059143,12.));
#250047=CARTESIAN_POINT('Ctrl Pts',(15.4129242997828,17.7459450555803,0.));
#250048=CARTESIAN_POINT('Ctrl Pts',(15.4129242997828,17.7459450555803,12.));
#250049=CARTESIAN_POINT('Ctrl Pts',(15.4285794642658,17.7559493405871,0.));
#250050=CARTESIAN_POINT('Ctrl Pts',(15.4285794642658,17.7559493405871,12.));
#250051=CARTESIAN_POINT('Ctrl Pts',(15.4443634132865,17.765974057326,0.));
#250052=CARTESIAN_POINT('Ctrl Pts',(15.4443634132865,17.765974057326,12.));
#250053=CARTESIAN_POINT('Ctrl Pts',(15.4602755393019,17.7760182175817,0.));
#250054=CARTESIAN_POINT('Ctrl Pts',(15.4602755393019,17.7760182175817,12.));
#250055=CARTESIAN_POINT('Ctrl Pts',(15.4763152417506,17.7860808481229,0.));
#250056=CARTESIAN_POINT('Ctrl Pts',(15.4763152417506,17.7860808481229,12.));
#250057=CARTESIAN_POINT('Ctrl Pts',(15.4924819268529,17.7961609903161,0.));
#250058=CARTESIAN_POINT('Ctrl Pts',(15.4924819268529,17.7961609903161,12.));
#250059=CARTESIAN_POINT('Ctrl Pts',(15.5087750074728,17.8062576997964,0.));
#250060=CARTESIAN_POINT('Ctrl Pts',(15.5087750074728,17.8062576997964,12.));
#250061=CARTESIAN_POINT('Ctrl Pts',(15.5251939029558,17.8163700461263,0.));
#250062=CARTESIAN_POINT('Ctrl Pts',(15.5251939029558,17.8163700461263,12.));
#250063=CARTESIAN_POINT('Ctrl Pts',(15.5417380389639,17.8264971124606,0.));
#250064=CARTESIAN_POINT('Ctrl Pts',(15.5417380389639,17.8264971124606,12.));
#250065=CARTESIAN_POINT('Ctrl Pts',(15.5584068472976,17.8366379952078,0.));
#250066=CARTESIAN_POINT('Ctrl Pts',(15.5584068472976,17.8366379952078,12.));
#250067=CARTESIAN_POINT('Ctrl Pts',(15.5751997657153,17.8467918036977,0.));
#250068=CARTESIAN_POINT('Ctrl Pts',(15.5751997657153,17.8467918036977,12.));
#250069=CARTESIAN_POINT('Ctrl Pts',(15.5921162378183,17.8569576598996,0.));
#250070=CARTESIAN_POINT('Ctrl Pts',(15.5921162378183,17.8569576598996,12.));
#250071=CARTESIAN_POINT('Ctrl Pts',(15.6091557129205,17.8671346981388,0.));
#250072=CARTESIAN_POINT('Ctrl Pts',(15.6091557129205,17.8671346981388,12.));
#250073=CARTESIAN_POINT('Ctrl Pts',(15.6263176459107,17.8773220648125,0.));
#250074=CARTESIAN_POINT('Ctrl Pts',(15.6263176459107,17.8773220648125,12.));
#250075=CARTESIAN_POINT('Ctrl Pts',(15.6436014971088,17.8875189181095,0.));
#250076=CARTESIAN_POINT('Ctrl Pts',(15.6436014971088,17.8875189181095,12.));
#250077=CARTESIAN_POINT('Ctrl Pts',(15.6610067321036,17.8977244277247,0.));
#250078=CARTESIAN_POINT('Ctrl Pts',(15.6610067321036,17.8977244277247,12.));
#250079=CARTESIAN_POINT('Ctrl Pts',(15.6785328216467,17.9079377746118,0.));
#250080=CARTESIAN_POINT('Ctrl Pts',(15.6785328216467,17.9079377746118,12.));
#250081=CARTESIAN_POINT('Ctrl Pts',(15.6961792415526,17.918158150746,0.));
#250082=CARTESIAN_POINT('Ctrl Pts',(15.6961792415526,17.918158150746,12.));
#250083=CARTESIAN_POINT('Ctrl Pts',(15.713945472584,17.9283847588837,0.));
#250084=CARTESIAN_POINT('Ctrl Pts',(15.713945472584,17.9283847588837,12.));
#250085=CARTESIAN_POINT('Ctrl Pts',(15.7318310003334,17.9386168123261,0.));
#250086=CARTESIAN_POINT('Ctrl Pts',(15.7318310003334,17.9386168123261,12.));
#250087=CARTESIAN_POINT('Ctrl Pts',(15.7498353150856,17.9488535346776,0.));
#250088=CARTESIAN_POINT('Ctrl Pts',(15.7498353150856,17.9488535346776,12.));
#250089=CARTESIAN_POINT('Ctrl Pts',(15.7679579117072,17.9590941596236,0.));
#250090=CARTESIAN_POINT('Ctrl Pts',(15.7679579117072,17.9590941596236,12.));
#250091=CARTESIAN_POINT('Ctrl Pts',(15.786198289572,17.9693379307297,0.));
#250092=CARTESIAN_POINT('Ctrl Pts',(15.786198289572,17.9693379307297,12.));
#250093=CARTESIAN_POINT('Ctrl Pts',(15.8045559524674,17.9795841012383,0.));
#250094=CARTESIAN_POINT('Ctrl Pts',(15.8045559524674,17.9795841012383,12.));
#250095=CARTESIAN_POINT('Ctrl Pts',(15.8230304084963,17.9898319338664,0.));
#250096=CARTESIAN_POINT('Ctrl Pts',(15.8230304084963,17.9898319338664,12.));
#250097=CARTESIAN_POINT('Ctrl Pts',(15.8416211699681,18.0000807006055,0.));
#250098=CARTESIAN_POINT('Ctrl Pts',(15.8416211699681,18.0000807006055,12.));
#250099=CARTESIAN_POINT('Ctrl Pts',(15.8603277532834,18.010329682521,0.));
#250100=CARTESIAN_POINT('Ctrl Pts',(15.8603277532834,18.010329682521,12.));
#250101=CARTESIAN_POINT('Ctrl Pts',(15.8791496788685,18.0205781695773,0.));
#250102=CARTESIAN_POINT('Ctrl Pts',(15.8791496788685,18.0205781695773,12.));
#250103=CARTESIAN_POINT('Ctrl Pts',(15.8980864711043,18.0308254604638,0.));
#250104=CARTESIAN_POINT('Ctrl Pts',(15.8980864711043,18.0308254604638,12.));
#250105=CARTESIAN_POINT('Ctrl Pts',(15.9171376582436,18.0410708624208,0.));
#250106=CARTESIAN_POINT('Ctrl Pts',(15.9171376582436,18.0410708624208,12.));
#250107=CARTESIAN_POINT('Ctrl Pts',(15.9363027723244,18.0513136910691,0.));
#250108=CARTESIAN_POINT('Ctrl Pts',(15.9363027723244,18.0513136910691,12.));
#250109=CARTESIAN_POINT('Ctrl Pts',(15.9555813490645,18.061553270236,0.));
#250110=CARTESIAN_POINT('Ctrl Pts',(15.9555813490645,18.061553270236,12.));
#250111=CARTESIAN_POINT('Ctrl Pts',(15.9749729277848,18.071788931796,0.));
#250112=CARTESIAN_POINT('Ctrl Pts',(15.9749729277848,18.071788931796,12.));
#250113=CARTESIAN_POINT('Ctrl Pts',(15.9944770513616,18.0820200155239,0.));
#250114=CARTESIAN_POINT('Ctrl Pts',(15.9944770513616,18.0820200155239,12.));
#250115=CARTESIAN_POINT('Ctrl Pts',(16.0140932661612,18.0922458689464,0.));
#250116=CARTESIAN_POINT('Ctrl Pts',(16.0140932661612,18.0922458689464,12.));
#250117=CARTESIAN_POINT('Ctrl Pts',(16.0338211219693,18.1024658471966,0.));
#250118=CARTESIAN_POINT('Ctrl Pts',(16.0338211219693,18.1024658471966,12.));
#250119=CARTESIAN_POINT('Ctrl Pts',(16.0536601719124,18.1126793128688,0.));
#250120=CARTESIAN_POINT('Ctrl Pts',(16.0536601719124,18.1126793128688,12.));
#250121=CARTESIAN_POINT('Ctrl Pts',(16.0736099723664,18.1228856358746,0.));
#250122=CARTESIAN_POINT('Ctrl Pts',(16.0736099723664,18.1228856358746,12.));
#250123=CARTESIAN_POINT('Ctrl Pts',(16.0936700829108,18.1330841933099,0.));
#250124=CARTESIAN_POINT('Ctrl Pts',(16.0936700829108,18.1330841933099,12.));
#250125=CARTESIAN_POINT('Ctrl Pts',(16.113840066279,18.1432743693231,0.));
#250126=CARTESIAN_POINT('Ctrl Pts',(16.113840066279,18.1432743693231,12.));
#250127=CARTESIAN_POINT('Ctrl Pts',(16.1341194882987,18.1534555549851,0.));
#250128=CARTESIAN_POINT('Ctrl Pts',(16.1341194882987,18.1534555549851,12.));
#250129=CARTESIAN_POINT('Ctrl Pts',(16.1545079178261,18.1636271481616,0.));
#250130=CARTESIAN_POINT('Ctrl Pts',(16.1545079178261,18.1636271481616,12.));
#250131=CARTESIAN_POINT('Ctrl Pts',(16.1750049266673,18.1737885533852,0.));
#250132=CARTESIAN_POINT('Ctrl Pts',(16.1750049266673,18.1737885533852,12.));
#250133=CARTESIAN_POINT('Ctrl Pts',(16.1956100895076,18.1839391817335,0.));
#250134=CARTESIAN_POINT('Ctrl Pts',(16.1956100895076,18.1839391817335,12.));
#250135=CARTESIAN_POINT('Ctrl Pts',(16.2163229838878,18.1940784507232,0.));
#250136=CARTESIAN_POINT('Ctrl Pts',(16.2163229838878,18.1940784507232,12.));
#250137=CARTESIAN_POINT('Ctrl Pts',(16.237143190164,18.2042057842037,0.));
#250138=CARTESIAN_POINT('Ctrl Pts',(16.237143190164,18.2042057842037,12.));
#250139=CARTESIAN_POINT('Ctrl Pts',(16.2580702914615,18.214320612253,0.));
#250140=CARTESIAN_POINT('Ctrl Pts',(16.2580702914615,18.214320612253,12.));
#250141=CARTESIAN_POINT('Ctrl Pts',(16.2791038736223,18.2244223710745,0.));
#250142=CARTESIAN_POINT('Ctrl Pts',(16.2791038736223,18.2244223710745,12.));
#250143=CARTESIAN_POINT('Ctrl Pts',(16.3002435251378,18.2345105028981,0.));
#250144=CARTESIAN_POINT('Ctrl Pts',(16.3002435251378,18.2345105028981,12.));
#250145=CARTESIAN_POINT('Ctrl Pts',(16.3214888370988,18.2445844558742,0.));
#250146=CARTESIAN_POINT('Ctrl Pts',(16.3214888370988,18.2445844558742,12.));
#250147=CARTESIAN_POINT('Ctrl Pts',(16.342839403159,18.2546436839609,0.));
#250148=CARTESIAN_POINT('Ctrl Pts',(16.342839403159,18.2546436839609,12.));
#250149=CARTESIAN_POINT('Ctrl Pts',(16.3642948194869,18.2646876468169,0.));
#250150=CARTESIAN_POINT('Ctrl Pts',(16.3642948194869,18.2646876468169,12.));
#250151=CARTESIAN_POINT('Ctrl Pts',(16.385854684708,18.2747158096934,0.));
#250152=CARTESIAN_POINT('Ctrl Pts',(16.385854684708,18.2747158096934,12.));
#250153=CARTESIAN_POINT('Ctrl Pts',(16.4075185998454,18.2847276433308,0.));
#250154=CARTESIAN_POINT('Ctrl Pts',(16.4075185998454,18.2847276433308,12.));
#250155=CARTESIAN_POINT('Ctrl Pts',(16.4292861682377,18.2947226238509,0.));
#250156=CARTESIAN_POINT('Ctrl Pts',(16.4292861682377,18.2947226238509,12.));
#250157=CARTESIAN_POINT('Ctrl Pts',(16.4511569955231,18.3047002326858,0.));
#250158=CARTESIAN_POINT('Ctrl Pts',(16.4511569955231,18.3047002326858,12.));
#250159=CARTESIAN_POINT('Ctrl Pts',(16.4731306896439,18.3146599565229,0.));
#250160=CARTESIAN_POINT('Ctrl Pts',(16.4731306896439,18.3146599565229,12.));
#250161=CARTESIAN_POINT('Ctrl Pts',(16.4952068608344,18.3246012872468,0.));
#250162=CARTESIAN_POINT('Ctrl Pts',(16.4952068608344,18.3246012872468,12.));
#250163=CARTESIAN_POINT('Ctrl Pts',(16.5173851216045,18.3345237218864,0.));
#250164=CARTESIAN_POINT('Ctrl Pts',(16.5173851216045,18.3345237218864,12.));
#250165=CARTESIAN_POINT('Ctrl Pts',(16.5396650867139,18.3444267625601,0.));
#250166=CARTESIAN_POINT('Ctrl Pts',(16.5396650867139,18.3444267625601,12.));
#250167=CARTESIAN_POINT('Ctrl Pts',(16.5620463731414,18.3543099164331,0.));
#250168=CARTESIAN_POINT('Ctrl Pts',(16.5620463731414,18.3543099164331,12.));
#250169=CARTESIAN_POINT('Ctrl Pts',(16.5845286000218,18.364172695589,0.));
#250170=CARTESIAN_POINT('Ctrl Pts',(16.5845286000218,18.364172695589,12.));
#250171=CARTESIAN_POINT('Ctrl Pts',(16.6071113885711,18.3740146168879,0.));
#250172=CARTESIAN_POINT('Ctrl Pts',(16.6071113885711,18.3740146168879,12.));
#250173=CARTESIAN_POINT('Ctrl Pts',(16.6297943620056,18.3838352018327,0.));
#250174=CARTESIAN_POINT('Ctrl Pts',(16.6297943620056,18.3838352018327,12.));
#250175=CARTESIAN_POINT('Ctrl Pts',(16.6525771454513,18.3936339764332,0.));
#250176=CARTESIAN_POINT('Ctrl Pts',(16.6525771454513,18.3936339764332,12.));
#250177=CARTESIAN_POINT('Ctrl Pts',(16.6754593658513,18.4034104710789,0.));
#250178=CARTESIAN_POINT('Ctrl Pts',(16.6754593658513,18.4034104710789,12.));
#250179=CARTESIAN_POINT('Ctrl Pts',(16.698440651849,18.413164220399,0.));
#250180=CARTESIAN_POINT('Ctrl Pts',(16.698440651849,18.413164220399,12.));
#250181=CARTESIAN_POINT('Ctrl Pts',(16.7215206338818,18.4228947633186,0.));
#250182=CARTESIAN_POINT('Ctrl Pts',(16.7215206338818,18.4228947633186,12.));
#250183=CARTESIAN_POINT('Ctrl Pts',(16.7446989442882,18.4326016431392,0.));
#250184=CARTESIAN_POINT('Ctrl Pts',(16.7446989442882,18.4326016431392,12.));
#250185=CARTESIAN_POINT('Ctrl Pts',(16.7679752173992,18.4422844076099,0.));
#250186=CARTESIAN_POINT('Ctrl Pts',(16.7679752173992,18.4422844076099,12.));
#250187=CARTESIAN_POINT('Ctrl Pts',(16.791349089629,18.4519426090124,0.));
#250188=CARTESIAN_POINT('Ctrl Pts',(16.791349089629,18.4519426090124,12.));
#250189=CARTESIAN_POINT('Ctrl Pts',(16.8148201995472,18.4615758042305,0.));
#250190=CARTESIAN_POINT('Ctrl Pts',(16.8148201995472,18.4615758042305,12.));
#250191=CARTESIAN_POINT('Ctrl Pts',(16.8383881879707,18.4711835548622,0.));
#250192=CARTESIAN_POINT('Ctrl Pts',(16.8383881879707,18.4711835548622,12.));
#250193=CARTESIAN_POINT('Ctrl Pts',(16.8620526977169,18.4807654268769,0.));
#250194=CARTESIAN_POINT('Ctrl Pts',(16.8620526977169,18.4807654268769,12.));
#250195=CARTESIAN_POINT('Ctrl Pts',(16.8858133733086,18.4903209902226,0.));
#250196=CARTESIAN_POINT('Ctrl Pts',(16.8858133733086,18.4903209902226,12.));
#250197=CARTESIAN_POINT('Ctrl Pts',(16.9096698606942,18.4998498184619,0.));
#250198=CARTESIAN_POINT('Ctrl Pts',(16.9096698606942,18.4998498184619,12.));
#250199=CARTESIAN_POINT('Ctrl Pts',(16.9336218069353,18.5093514883835,0.));
#250200=CARTESIAN_POINT('Ctrl Pts',(16.9336218069353,18.5093514883835,12.));
#250201=CARTESIAN_POINT('Ctrl Pts',(16.957668859934,18.518825579666,0.));
#250202=CARTESIAN_POINT('Ctrl Pts',(16.957668859934,18.518825579666,12.));
#250203=CARTESIAN_POINT('Ctrl Pts',(16.9818106680382,18.5282716744198,0.));
#250204=CARTESIAN_POINT('Ctrl Pts',(16.9818106680382,18.5282716744198,12.));
#250205=CARTESIAN_POINT('Ctrl Pts',(17.0060468805099,18.5376893576961,0.));
#250206=CARTESIAN_POINT('Ctrl Pts',(17.0060468805099,18.5376893576961,12.));
#250207=CARTESIAN_POINT('Ctrl Pts',(17.030377148174,18.5470782182089,0.));
#250208=CARTESIAN_POINT('Ctrl Pts',(17.030377148174,18.5470782182089,12.));
#250209=CARTESIAN_POINT('Ctrl Pts',(17.0548011239751,18.5564378489628,0.));
#250210=CARTESIAN_POINT('Ctrl Pts',(17.0548011239751,18.5564378489628,12.));
#250211=CARTESIAN_POINT('Ctrl Pts',(17.0793184636079,18.5657678479788,0.));
#250212=CARTESIAN_POINT('Ctrl Pts',(17.0793184636079,18.5657678479788,12.));
#250213=CARTESIAN_POINT('Ctrl Pts',(17.1039288260001,18.5750678188543,0.));
#250214=CARTESIAN_POINT('Ctrl Pts',(17.1039288260001,18.5750678188543,12.));
#250215=CARTESIAN_POINT('Ctrl Pts',(17.1286318741185,18.5843373717253,0.));
#250216=CARTESIAN_POINT('Ctrl Pts',(17.1286318741185,18.5843373717253,12.));
#250217=CARTESIAN_POINT('Ctrl Pts',(17.1534272741646,18.5935761222833,0.));
#250218=CARTESIAN_POINT('Ctrl Pts',(17.1534272741646,18.5935761222833,12.));
#250219=CARTESIAN_POINT('Ctrl Pts',(17.1783146940131,18.6027836898826,0.));
#250220=CARTESIAN_POINT('Ctrl Pts',(17.1783146940131,18.6027836898826,12.));
#250221=CARTESIAN_POINT('Ctrl Pts',(17.2032938019288,18.6119596959957,0.));
#250222=CARTESIAN_POINT('Ctrl Pts',(17.2032938019288,18.6119596959957,12.));
#250223=CARTESIAN_POINT('Ctrl Pts',(17.2283642650519,18.6211037624041,0.));
#250224=CARTESIAN_POINT('Ctrl Pts',(17.2283642650519,18.6211037624041,12.));
#250225=CARTESIAN_POINT('Ctrl Pts',(17.2535257482186,18.630215509794,0.));
#250226=CARTESIAN_POINT('Ctrl Pts',(17.2535257482186,18.630215509794,12.));
#250227=CARTESIAN_POINT('Ctrl Pts',(17.278777912021,18.639294555474,0.));
#250228=CARTESIAN_POINT('Ctrl Pts',(17.278777912021,18.639294555474,12.));
#250229=CARTESIAN_POINT('Ctrl Pts',(17.3041204135069,18.6483405141853,0.));
#250230=CARTESIAN_POINT('Ctrl Pts',(17.3041204135069,18.6483405141853,12.));
#250231=CARTESIAN_POINT('Ctrl Pts',(17.3295529098612,18.6573530024019,0.));
#250232=CARTESIAN_POINT('Ctrl Pts',(17.3295529098612,18.6573530024019,12.));
#250233=CARTESIAN_POINT('Ctrl Pts',(17.3550750612438,18.6663316416569,0.));
#250234=CARTESIAN_POINT('Ctrl Pts',(17.3550750612438,18.6663316416569,12.));
#250235=CARTESIAN_POINT('Ctrl Pts',(17.3806865340744,18.6752760624045,0.));
#250236=CARTESIAN_POINT('Ctrl Pts',(17.3806865340744,18.6752760624045,12.));
#250237=CARTESIAN_POINT('Ctrl Pts',(17.4063870038563,18.6841859073472,0.));
#250238=CARTESIAN_POINT('Ctrl Pts',(17.4063870038563,18.6841859073472,12.));
#250239=CARTESIAN_POINT('Ctrl Pts',(17.4321761588148,18.6930608357421,0.));
#250240=CARTESIAN_POINT('Ctrl Pts',(17.4321761588148,18.6930608357421,12.));
#250241=CARTESIAN_POINT('Ctrl Pts',(17.4580537012764,18.7019005250322,0.));
#250242=CARTESIAN_POINT('Ctrl Pts',(17.4580537012764,18.7019005250322,12.));
#250243=CARTESIAN_POINT('Ctrl Pts',(17.4840193397176,18.7107046613941,0.));
#250244=CARTESIAN_POINT('Ctrl Pts',(17.4840193397176,18.7107046613941,12.));
#250245=CARTESIAN_POINT('Ctrl Pts',(17.5100727820891,18.7194729318128,0.));
#250246=CARTESIAN_POINT('Ctrl Pts',(17.5100727820891,18.7194729318128,12.));
#250247=CARTESIAN_POINT('Ctrl Pts',(17.5362137287604,18.728205015716,0.));
#250248=CARTESIAN_POINT('Ctrl Pts',(17.5362137287604,18.728205015716,12.));
#250249=CARTESIAN_POINT('Ctrl Pts',(17.5624418653248,18.7369005764558,0.));
#250250=CARTESIAN_POINT('Ctrl Pts',(17.5624418653248,18.7369005764558,12.));
#250251=CARTESIAN_POINT('Ctrl Pts',(17.5887568561361,18.7455592536667,0.));
#250252=CARTESIAN_POINT('Ctrl Pts',(17.5887568561361,18.7455592536667,12.));
#250253=CARTESIAN_POINT('Ctrl Pts',(17.6151583356988,18.7541806530935,0.));
#250254=CARTESIAN_POINT('Ctrl Pts',(17.6151583356988,18.7541806530935,12.));
#250255=CARTESIAN_POINT('Ctrl Pts',(17.6416459210646,18.7627643613139,0.));
#250256=CARTESIAN_POINT('Ctrl Pts',(17.6416459210646,18.7627643613139,12.));
#250257=CARTESIAN_POINT('Ctrl Pts',(17.6682192274197,18.7713099642673,0.));
#250258=CARTESIAN_POINT('Ctrl Pts',(17.6682192274197,18.7713099642673,12.));
#250259=CARTESIAN_POINT('Ctrl Pts',(17.6948778822981,18.7798170641305,0.));
#250260=CARTESIAN_POINT('Ctrl Pts',(17.6948778822981,18.7798170641305,12.));
#250261=CARTESIAN_POINT('Ctrl Pts',(17.7216215409019,18.7882852976016,0.));
#250262=CARTESIAN_POINT('Ctrl Pts',(17.7216215409019,18.7882852976016,12.));
#250263=CARTESIAN_POINT('Ctrl Pts',(17.7484498996916,18.7967143519444,0.));
#250264=CARTESIAN_POINT('Ctrl Pts',(17.7484498996916,18.7967143519444,12.));
#250265=CARTESIAN_POINT('Ctrl Pts',(17.7753627137898,18.8051039860543,0.));
#250266=CARTESIAN_POINT('Ctrl Pts',(17.7753627137898,18.8051039860543,12.));
#250267=CARTESIAN_POINT('Ctrl Pts',(17.8023598011135,18.8134540340581,0.));
#250268=CARTESIAN_POINT('Ctrl Pts',(17.8023598011135,18.8134540340581,12.));
#250269=CARTESIAN_POINT('Ctrl Pts',(17.8294410311105,18.8217643886368,0.));
#250270=CARTESIAN_POINT('Ctrl Pts',(17.8294410311105,18.8217643886368,12.));
#250271=CARTESIAN_POINT('Ctrl Pts',(17.8566063174871,18.8300349896187,0.));
#250272=CARTESIAN_POINT('Ctrl Pts',(17.8566063174871,18.8300349896187,12.));
#250273=CARTESIAN_POINT('Ctrl Pts',(17.8784057509434,18.8366196462746,0.));
#250274=CARTESIAN_POINT('Ctrl Pts',(17.8784057509434,18.8366196462746,12.));
#250275=CARTESIAN_POINT('Ctrl Pts',(17.8947931177853,18.8415402351882,0.));
#250276=CARTESIAN_POINT('Ctrl Pts',(17.8947931177853,18.8415402351882,12.));
#250277=CARTESIAN_POINT('Ctrl Pts',(17.9057348246611,18.8448126709726,0.));
#250278=CARTESIAN_POINT('Ctrl Pts',(17.9057348246611,18.8448126709726,12.));
#250279=CARTESIAN_POINT('Ctrl Pts',(17.9112098770111,18.8464468996588,0.));
#250280=CARTESIAN_POINT('Ctrl Pts',(17.9112098770111,18.8464468996588,12.));
#250281=CARTESIAN_POINT('',(17.9112098770111,18.8464468996588,0.));
#250282=CARTESIAN_POINT('Ctrl Pts',(14.6513681262571,17.1452095830633,0.));
#250283=CARTESIAN_POINT('Ctrl Pts',(14.6513711852843,17.1452153999142,0.));
#250284=CARTESIAN_POINT('Ctrl Pts',(14.6514066997196,17.1452600887037,0.));
#250285=CARTESIAN_POINT('Ctrl Pts',(14.6515481598068,17.1454262858043,0.));
#250286=CARTESIAN_POINT('Ctrl Pts',(14.6519131634508,17.1458462295271,0.));
#250287=CARTESIAN_POINT('Ctrl Pts',(14.6526624064978,17.1466998098673,0.));
#250288=CARTESIAN_POINT('Ctrl Pts',(14.6537016966184,17.147876394491,0.));
#250289=CARTESIAN_POINT('Ctrl Pts',(14.655024862281,17.1493641837558,0.));
#250290=CARTESIAN_POINT('Ctrl Pts',(14.6566237952435,17.1511476869496,0.));
#250291=CARTESIAN_POINT('Ctrl Pts',(14.6584900555302,17.1532107762718,0.));
#250292=CARTESIAN_POINT('Ctrl Pts',(14.6606167169642,17.1555401986401,0.));
#250293=CARTESIAN_POINT('Ctrl Pts',(14.6629987285992,17.1581262646789,0.));
#250294=CARTESIAN_POINT('Ctrl Pts',(14.6656319165057,17.1609609517369,0.));
#250295=CARTESIAN_POINT('Ctrl Pts',(14.6685123374423,17.1640366762305,0.));
#250296=CARTESIAN_POINT('Ctrl Pts',(14.671635583332,17.167344972302,0.));
#250297=CARTESIAN_POINT('Ctrl Pts',(14.6749971333867,17.1708771619129,0.));
#250298=CARTESIAN_POINT('Ctrl Pts',(14.6785925615677,17.1746247499057,0.));
#250299=CARTESIAN_POINT('Ctrl Pts',(14.6824178576167,17.1785800350826,0.));
#250300=CARTESIAN_POINT('Ctrl Pts',(14.686469452232,17.182736158472,0.));
#250301=CARTESIAN_POINT('Ctrl Pts',(14.6907440526958,17.1870867909918,0.));
#250302=CARTESIAN_POINT('Ctrl Pts',(14.6952385361705,17.1916259308415,0.));
#250303=CARTESIAN_POINT('Ctrl Pts',(14.699949811582,17.1963476411694,0.));
#250304=CARTESIAN_POINT('Ctrl Pts',(14.7048748502663,17.2012461084268,0.));
#250305=CARTESIAN_POINT('Ctrl Pts',(14.7100107213586,17.2063157097315,0.));
#250306=CARTESIAN_POINT('Ctrl Pts',(14.7153546289339,17.2115510835989,0.));
#250307=CARTESIAN_POINT('Ctrl Pts',(14.7209039390327,17.2169471814256,0.));
#250308=CARTESIAN_POINT('Ctrl Pts',(14.7266561494282,17.2224992099667,0.));
#250309=CARTESIAN_POINT('Ctrl Pts',(14.7326088681163,17.2282025904314,0.));
#250310=CARTESIAN_POINT('Ctrl Pts',(14.7387597858116,17.2340529062076,0.));
#250311=CARTESIAN_POINT('Ctrl Pts',(14.7451066593792,17.2400458713565,0.));
#250312=CARTESIAN_POINT('Ctrl Pts',(14.7516473175124,17.2461773413288,0.));
#250313=CARTESIAN_POINT('Ctrl Pts',(14.7583796616617,17.2524433146837,0.));
#250314=CARTESIAN_POINT('Ctrl Pts',(14.7653016697591,17.2588399401465,0.));
#250315=CARTESIAN_POINT('Ctrl Pts',(14.7724113956731,17.2653635155319,0.));
#250316=CARTESIAN_POINT('Ctrl Pts',(14.7797069617804,17.2720104735194,0.));
#250317=CARTESIAN_POINT('Ctrl Pts',(14.787186553128,17.2787773704849,0.));
#250318=CARTESIAN_POINT('Ctrl Pts',(14.7948484105249,17.2856608733196,0.));
#250319=CARTESIAN_POINT('Ctrl Pts',(14.8026908254276,17.2926577496513,0.));
#250320=CARTESIAN_POINT('Ctrl Pts',(14.8107121391035,17.299764866148,0.));
#250321=CARTESIAN_POINT('Ctrl Pts',(14.8189107410162,17.3069791853706,0.));
#250322=CARTESIAN_POINT('Ctrl Pts',(14.8272850675379,17.3142977632659,0.));
#250323=CARTESIAN_POINT('Ctrl Pts',(14.8358336004197,17.3217177462101,0.));
#250324=CARTESIAN_POINT('Ctrl Pts',(14.8445548643508,17.3292363662605,0.));
#250325=CARTESIAN_POINT('Ctrl Pts',(14.8534474245433,17.336850936485,0.));
#250326=CARTESIAN_POINT('Ctrl Pts',(14.8625098843417,17.3445588463475,0.));
#250327=CARTESIAN_POINT('Ctrl Pts',(14.8717408826955,17.3523575568645,0.));
#250328=CARTESIAN_POINT('Ctrl Pts',(14.8811390927423,17.3602445978161,0.));
#250329=CARTESIAN_POINT('Ctrl Pts',(14.8907032205788,17.3682175653235,0.));
#250330=CARTESIAN_POINT('Ctrl Pts',(14.900432003961,17.3762741193076,0.));
#250331=CARTESIAN_POINT('Ctrl Pts',(14.9103242110057,17.3844119809824,0.));
#250332=CARTESIAN_POINT('Ctrl Pts',(14.9203786389342,17.3926289303986,0.));
#250333=CARTESIAN_POINT('Ctrl Pts',(14.9305941128757,17.4009228040749,0.));
#250334=CARTESIAN_POINT('Ctrl Pts',(14.940969484645,17.4092914926071,0.));
#250335=CARTESIAN_POINT('Ctrl Pts',(14.9515036315143,17.4177329382828,0.));
#250336=CARTESIAN_POINT('Ctrl Pts',(14.9621954549827,17.426245132709,0.));
#250337=CARTESIAN_POINT('Ctrl Pts',(14.9730438799452,17.4348261151396,0.));
#250338=CARTESIAN_POINT('Ctrl Pts',(14.9840478538358,17.4434739707773,0.));
#250339=CARTESIAN_POINT('Ctrl Pts',(14.9952063457778,17.4521868291004,0.));
#250340=CARTESIAN_POINT('Ctrl Pts',(15.0065183456921,17.4609628621418,0.));
#250341=CARTESIAN_POINT('Ctrl Pts',(15.0179828635086,17.4698002829357,0.));
#250342=CARTESIAN_POINT('Ctrl Pts',(15.029598928488,17.4786973441417,0.));
#250343=CARTESIAN_POINT('Ctrl Pts',(15.0413655884993,17.4876523366178,0.));
#250344=CARTESIAN_POINT('Ctrl Pts',(15.0532819093085,17.4966635880245,0.));
#250345=CARTESIAN_POINT('Ctrl Pts',(15.0653469738306,17.5057294613874,0.));
#250346=CARTESIAN_POINT('Ctrl Pts',(15.0775598815748,17.5148483539684,0.));
#250347=CARTESIAN_POINT('Ctrl Pts',(15.0899197481082,17.5240186961788,0.));
#250348=CARTESIAN_POINT('Ctrl Pts',(15.1024257045033,17.5332389504829,0.));
#250349=CARTESIAN_POINT('Ctrl Pts',(15.1150768967729,17.5425076102966,0.));
#250350=CARTESIAN_POINT('Ctrl Pts',(15.127872485314,17.5518231989122,0.));
#250351=CARTESIAN_POINT('Ctrl Pts',(15.1408116444877,17.5611842686196,0.));
#250352=CARTESIAN_POINT('Ctrl Pts',(15.1538935621714,17.570589399803,0.));
#250353=CARTESIAN_POINT('Ctrl Pts',(15.1671174393136,17.5800372000539,0.));
#250354=CARTESIAN_POINT('Ctrl Pts',(15.1804824894605,17.5895263032592,0.));
#250355=CARTESIAN_POINT('Ctrl Pts',(15.1939879383268,17.5990553687595,0.));
#250356=CARTESIAN_POINT('Ctrl Pts',(15.2076330234686,17.6086230806497,0.));
#250357=CARTESIAN_POINT('Ctrl Pts',(15.22141699392,17.6182281470467,0.));
#250358=CARTESIAN_POINT('Ctrl Pts',(15.2353391098367,17.6278692993765,0.));
#250359=CARTESIAN_POINT('Ctrl Pts',(15.2493986421091,17.637545291637,0.));
#250360=CARTESIAN_POINT('Ctrl Pts',(15.263594872029,17.6472548997329,0.));
#250361=CARTESIAN_POINT('Ctrl Pts',(15.2779270910238,17.6569969209,0.));
#250362=CARTESIAN_POINT('Ctrl Pts',(15.2923946003598,17.6667701731041,0.));
#250363=CARTESIAN_POINT('Ctrl Pts',(15.3069967108501,17.6765734944559,0.));
#250364=CARTESIAN_POINT('Ctrl Pts',(15.3217327425341,17.6864057426052,0.));
#250365=CARTESIAN_POINT('Ctrl Pts',(15.3366020244069,17.6962657941984,0.));
#250366=CARTESIAN_POINT('Ctrl Pts',(15.3516038942064,17.7061525444044,0.));
#250367=CARTESIAN_POINT('Ctrl Pts',(15.3667376981702,17.7160649064208,0.));
#250368=CARTESIAN_POINT('Ctrl Pts',(15.3820027907965,17.7260018109923,0.));
#250369=CARTESIAN_POINT('Ctrl Pts',(15.3973985345796,17.7359622059143,0.));
#250370=CARTESIAN_POINT('Ctrl Pts',(15.4129242997828,17.7459450555803,0.));
#250371=CARTESIAN_POINT('Ctrl Pts',(15.4285794642658,17.7559493405871,0.));
#250372=CARTESIAN_POINT('Ctrl Pts',(15.4443634132865,17.765974057326,0.));
#250373=CARTESIAN_POINT('Ctrl Pts',(15.4602755393019,17.7760182175817,0.));
#250374=CARTESIAN_POINT('Ctrl Pts',(15.4763152417506,17.7860808481229,0.));
#250375=CARTESIAN_POINT('Ctrl Pts',(15.4924819268529,17.7961609903161,0.));
#250376=CARTESIAN_POINT('Ctrl Pts',(15.5087750074728,17.8062576997964,0.));
#250377=CARTESIAN_POINT('Ctrl Pts',(15.5251939029558,17.8163700461263,0.));
#250378=CARTESIAN_POINT('Ctrl Pts',(15.5417380389639,17.8264971124606,0.));
#250379=CARTESIAN_POINT('Ctrl Pts',(15.5584068472976,17.8366379952078,0.));
#250380=CARTESIAN_POINT('Ctrl Pts',(15.5751997657153,17.8467918036977,0.));
#250381=CARTESIAN_POINT('Ctrl Pts',(15.5921162378183,17.8569576598996,0.));
#250382=CARTESIAN_POINT('Ctrl Pts',(15.6091557129205,17.8671346981388,0.));
#250383=CARTESIAN_POINT('Ctrl Pts',(15.6263176459107,17.8773220648125,0.));
#250384=CARTESIAN_POINT('Ctrl Pts',(15.6436014971088,17.8875189181095,0.));
#250385=CARTESIAN_POINT('Ctrl Pts',(15.6610067321036,17.8977244277247,0.));
#250386=CARTESIAN_POINT('Ctrl Pts',(15.6785328216467,17.9079377746118,0.));
#250387=CARTESIAN_POINT('Ctrl Pts',(15.6961792415526,17.918158150746,0.));
#250388=CARTESIAN_POINT('Ctrl Pts',(15.713945472584,17.9283847588837,0.));
#250389=CARTESIAN_POINT('Ctrl Pts',(15.7318310003334,17.9386168123261,0.));
#250390=CARTESIAN_POINT('Ctrl Pts',(15.7498353150856,17.9488535346776,0.));
#250391=CARTESIAN_POINT('Ctrl Pts',(15.7679579117072,17.9590941596236,0.));
#250392=CARTESIAN_POINT('Ctrl Pts',(15.786198289572,17.9693379307297,0.));
#250393=CARTESIAN_POINT('Ctrl Pts',(15.8045559524674,17.9795841012383,0.));
#250394=CARTESIAN_POINT('Ctrl Pts',(15.8230304084963,17.9898319338664,0.));
#250395=CARTESIAN_POINT('Ctrl Pts',(15.8416211699681,18.0000807006055,0.));
#250396=CARTESIAN_POINT('Ctrl Pts',(15.8603277532834,18.010329682521,0.));
#250397=CARTESIAN_POINT('Ctrl Pts',(15.8791496788685,18.0205781695773,0.));
#250398=CARTESIAN_POINT('Ctrl Pts',(15.8980864711043,18.0308254604638,0.));
#250399=CARTESIAN_POINT('Ctrl Pts',(15.9171376582436,18.0410708624208,0.));
#250400=CARTESIAN_POINT('Ctrl Pts',(15.9363027723244,18.0513136910691,0.));
#250401=CARTESIAN_POINT('Ctrl Pts',(15.9555813490645,18.061553270236,0.));
#250402=CARTESIAN_POINT('Ctrl Pts',(15.9749729277848,18.071788931796,0.));
#250403=CARTESIAN_POINT('Ctrl Pts',(15.9944770513616,18.0820200155239,0.));
#250404=CARTESIAN_POINT('Ctrl Pts',(16.0140932661612,18.0922458689464,0.));
#250405=CARTESIAN_POINT('Ctrl Pts',(16.0338211219693,18.1024658471966,0.));
#250406=CARTESIAN_POINT('Ctrl Pts',(16.0536601719124,18.1126793128688,0.));
#250407=CARTESIAN_POINT('Ctrl Pts',(16.0736099723664,18.1228856358746,0.));
#250408=CARTESIAN_POINT('Ctrl Pts',(16.0936700829108,18.1330841933099,0.));
#250409=CARTESIAN_POINT('Ctrl Pts',(16.113840066279,18.1432743693231,0.));
#250410=CARTESIAN_POINT('Ctrl Pts',(16.1341194882987,18.1534555549851,0.));
#250411=CARTESIAN_POINT('Ctrl Pts',(16.1545079178261,18.1636271481616,0.));
#250412=CARTESIAN_POINT('Ctrl Pts',(16.1750049266673,18.1737885533852,0.));
#250413=CARTESIAN_POINT('Ctrl Pts',(16.1956100895076,18.1839391817335,0.));
#250414=CARTESIAN_POINT('Ctrl Pts',(16.2163229838878,18.1940784507232,0.));
#250415=CARTESIAN_POINT('Ctrl Pts',(16.237143190164,18.2042057842037,0.));
#250416=CARTESIAN_POINT('Ctrl Pts',(16.2580702914615,18.214320612253,0.));
#250417=CARTESIAN_POINT('Ctrl Pts',(16.2791038736223,18.2244223710745,0.));
#250418=CARTESIAN_POINT('Ctrl Pts',(16.3002435251378,18.2345105028981,0.));
#250419=CARTESIAN_POINT('Ctrl Pts',(16.3214888370988,18.2445844558742,0.));
#250420=CARTESIAN_POINT('Ctrl Pts',(16.342839403159,18.2546436839609,0.));
#250421=CARTESIAN_POINT('Ctrl Pts',(16.3642948194869,18.2646876468169,0.));
#250422=CARTESIAN_POINT('Ctrl Pts',(16.385854684708,18.2747158096934,0.));
#250423=CARTESIAN_POINT('Ctrl Pts',(16.4075185998454,18.2847276433308,0.));
#250424=CARTESIAN_POINT('Ctrl Pts',(16.4292861682377,18.2947226238509,0.));
#250425=CARTESIAN_POINT('Ctrl Pts',(16.4511569955231,18.3047002326858,0.));
#250426=CARTESIAN_POINT('Ctrl Pts',(16.4731306896439,18.3146599565229,0.));
#250427=CARTESIAN_POINT('Ctrl Pts',(16.4952068608344,18.3246012872468,0.));
#250428=CARTESIAN_POINT('Ctrl Pts',(16.5173851216045,18.3345237218864,0.));
#250429=CARTESIAN_POINT('Ctrl Pts',(16.5396650867139,18.3444267625601,0.));
#250430=CARTESIAN_POINT('Ctrl Pts',(16.5620463731414,18.3543099164331,0.));
#250431=CARTESIAN_POINT('Ctrl Pts',(16.5845286000218,18.364172695589,0.));
#250432=CARTESIAN_POINT('Ctrl Pts',(16.6071113885711,18.3740146168879,0.));
#250433=CARTESIAN_POINT('Ctrl Pts',(16.6297943620056,18.3838352018327,0.));
#250434=CARTESIAN_POINT('Ctrl Pts',(16.6525771454513,18.3936339764332,0.));
#250435=CARTESIAN_POINT('Ctrl Pts',(16.6754593658513,18.4034104710789,0.));
#250436=CARTESIAN_POINT('Ctrl Pts',(16.698440651849,18.413164220399,0.));
#250437=CARTESIAN_POINT('Ctrl Pts',(16.7215206338818,18.4228947633186,0.));
#250438=CARTESIAN_POINT('Ctrl Pts',(16.7446989442882,18.4326016431392,0.));
#250439=CARTESIAN_POINT('Ctrl Pts',(16.7679752173992,18.4422844076099,0.));
#250440=CARTESIAN_POINT('Ctrl Pts',(16.791349089629,18.4519426090124,0.));
#250441=CARTESIAN_POINT('Ctrl Pts',(16.8148201995472,18.4615758042305,0.));
#250442=CARTESIAN_POINT('Ctrl Pts',(16.8383881879707,18.4711835548622,0.));
#250443=CARTESIAN_POINT('Ctrl Pts',(16.8620526977169,18.4807654268769,0.));
#250444=CARTESIAN_POINT('Ctrl Pts',(16.8858133733086,18.4903209902226,0.));
#250445=CARTESIAN_POINT('Ctrl Pts',(16.9096698606942,18.4998498184619,0.));
#250446=CARTESIAN_POINT('Ctrl Pts',(16.9336218069353,18.5093514883835,0.));
#250447=CARTESIAN_POINT('Ctrl Pts',(16.957668859934,18.518825579666,0.));
#250448=CARTESIAN_POINT('Ctrl Pts',(16.9818106680382,18.5282716744198,0.));
#250449=CARTESIAN_POINT('Ctrl Pts',(17.0060468805099,18.5376893576961,0.));
#250450=CARTESIAN_POINT('Ctrl Pts',(17.030377148174,18.5470782182089,0.));
#250451=CARTESIAN_POINT('Ctrl Pts',(17.0548011239751,18.5564378489628,0.));
#250452=CARTESIAN_POINT('Ctrl Pts',(17.0793184636079,18.5657678479788,0.));
#250453=CARTESIAN_POINT('Ctrl Pts',(17.1039288260001,18.5750678188543,0.));
#250454=CARTESIAN_POINT('Ctrl Pts',(17.1286318741185,18.5843373717253,0.));
#250455=CARTESIAN_POINT('Ctrl Pts',(17.1534272741646,18.5935761222833,0.));
#250456=CARTESIAN_POINT('Ctrl Pts',(17.1783146940131,18.6027836898826,0.));
#250457=CARTESIAN_POINT('Ctrl Pts',(17.2032938019288,18.6119596959957,0.));
#250458=CARTESIAN_POINT('Ctrl Pts',(17.2283642650519,18.6211037624041,0.));
#250459=CARTESIAN_POINT('Ctrl Pts',(17.2535257482186,18.630215509794,0.));
#250460=CARTESIAN_POINT('Ctrl Pts',(17.278777912021,18.639294555474,0.));
#250461=CARTESIAN_POINT('Ctrl Pts',(17.3041204135069,18.6483405141853,0.));
#250462=CARTESIAN_POINT('Ctrl Pts',(17.3295529098612,18.6573530024019,0.));
#250463=CARTESIAN_POINT('Ctrl Pts',(17.3550750612438,18.6663316416569,0.));
#250464=CARTESIAN_POINT('Ctrl Pts',(17.3806865340744,18.6752760624045,0.));
#250465=CARTESIAN_POINT('Ctrl Pts',(17.4063870038563,18.6841859073472,0.));
#250466=CARTESIAN_POINT('Ctrl Pts',(17.4321761588148,18.6930608357421,0.));
#250467=CARTESIAN_POINT('Ctrl Pts',(17.4580537012764,18.7019005250322,0.));
#250468=CARTESIAN_POINT('Ctrl Pts',(17.4840193397176,18.7107046613941,0.));
#250469=CARTESIAN_POINT('Ctrl Pts',(17.5100727820891,18.7194729318128,0.));
#250470=CARTESIAN_POINT('Ctrl Pts',(17.5362137287604,18.728205015716,0.));
#250471=CARTESIAN_POINT('Ctrl Pts',(17.5624418653248,18.7369005764558,0.));
#250472=CARTESIAN_POINT('Ctrl Pts',(17.5887568561361,18.7455592536667,0.));
#250473=CARTESIAN_POINT('Ctrl Pts',(17.6151583356988,18.7541806530935,0.));
#250474=CARTESIAN_POINT('Ctrl Pts',(17.6416459210646,18.7627643613139,0.));
#250475=CARTESIAN_POINT('Ctrl Pts',(17.6682192274197,18.7713099642673,0.));
#250476=CARTESIAN_POINT('Ctrl Pts',(17.6948778822981,18.7798170641305,0.));
#250477=CARTESIAN_POINT('Ctrl Pts',(17.7216215409019,18.7882852976016,0.));
#250478=CARTESIAN_POINT('Ctrl Pts',(17.7484498996916,18.7967143519444,0.));
#250479=CARTESIAN_POINT('Ctrl Pts',(17.7753627137898,18.8051039860543,0.));
#250480=CARTESIAN_POINT('Ctrl Pts',(17.8023598011135,18.8134540340581,0.));
#250481=CARTESIAN_POINT('Ctrl Pts',(17.8294410311105,18.8217643886368,0.));
#250482=CARTESIAN_POINT('Ctrl Pts',(17.8566063174871,18.8300349896187,0.));
#250483=CARTESIAN_POINT('Ctrl Pts',(17.8784057509434,18.8366196462746,0.));
#250484=CARTESIAN_POINT('Ctrl Pts',(17.8947931177853,18.8415402351882,0.));
#250485=CARTESIAN_POINT('Ctrl Pts',(17.9057348246611,18.8448126709726,0.));
#250486=CARTESIAN_POINT('Ctrl Pts',(17.9112098770111,18.8464468996588,0.));
#250487=CARTESIAN_POINT('',(17.9112098770111,18.8464468996588,12.));
#250488=CARTESIAN_POINT('Ctrl Pts',(17.9112098770111,18.8464468996588,12.));
#250489=CARTESIAN_POINT('Ctrl Pts',(17.9057348246611,18.8448126709726,12.));
#250490=CARTESIAN_POINT('Ctrl Pts',(17.8947931177853,18.8415402351882,12.));
#250491=CARTESIAN_POINT('Ctrl Pts',(17.8784057509434,18.8366196462746,12.));
#250492=CARTESIAN_POINT('Ctrl Pts',(17.8566063174871,18.8300349896187,12.));
#250493=CARTESIAN_POINT('Ctrl Pts',(17.8294410311105,18.8217643886368,12.));
#250494=CARTESIAN_POINT('Ctrl Pts',(17.8023598011135,18.8134540340581,12.));
#250495=CARTESIAN_POINT('Ctrl Pts',(17.7753627137898,18.8051039860543,12.));
#250496=CARTESIAN_POINT('Ctrl Pts',(17.7484498996916,18.7967143519444,12.));
#250497=CARTESIAN_POINT('Ctrl Pts',(17.7216215409019,18.7882852976016,12.));
#250498=CARTESIAN_POINT('Ctrl Pts',(17.6948778822981,18.7798170641305,12.));
#250499=CARTESIAN_POINT('Ctrl Pts',(17.6682192274197,18.7713099642673,12.));
#250500=CARTESIAN_POINT('Ctrl Pts',(17.6416459210646,18.7627643613139,12.));
#250501=CARTESIAN_POINT('Ctrl Pts',(17.6151583356988,18.7541806530935,12.));
#250502=CARTESIAN_POINT('Ctrl Pts',(17.5887568561361,18.7455592536667,12.));
#250503=CARTESIAN_POINT('Ctrl Pts',(17.5624418653248,18.7369005764558,12.));
#250504=CARTESIAN_POINT('Ctrl Pts',(17.5362137287604,18.728205015716,12.));
#250505=CARTESIAN_POINT('Ctrl Pts',(17.5100727820891,18.7194729318128,12.));
#250506=CARTESIAN_POINT('Ctrl Pts',(17.4840193397176,18.7107046613941,12.));
#250507=CARTESIAN_POINT('Ctrl Pts',(17.4580537012764,18.7019005250322,12.));
#250508=CARTESIAN_POINT('Ctrl Pts',(17.4321761588148,18.6930608357421,12.));
#250509=CARTESIAN_POINT('Ctrl Pts',(17.4063870038563,18.6841859073472,12.));
#250510=CARTESIAN_POINT('Ctrl Pts',(17.3806865340744,18.6752760624045,12.));
#250511=CARTESIAN_POINT('Ctrl Pts',(17.3550750612438,18.6663316416569,12.));
#250512=CARTESIAN_POINT('Ctrl Pts',(17.3295529098612,18.6573530024019,12.));
#250513=CARTESIAN_POINT('Ctrl Pts',(17.3041204135069,18.6483405141853,12.));
#250514=CARTESIAN_POINT('Ctrl Pts',(17.278777912021,18.639294555474,12.));
#250515=CARTESIAN_POINT('Ctrl Pts',(17.2535257482186,18.630215509794,12.));
#250516=CARTESIAN_POINT('Ctrl Pts',(17.2283642650519,18.6211037624041,12.));
#250517=CARTESIAN_POINT('Ctrl Pts',(17.2032938019288,18.6119596959957,12.));
#250518=CARTESIAN_POINT('Ctrl Pts',(17.1783146940131,18.6027836898826,12.));
#250519=CARTESIAN_POINT('Ctrl Pts',(17.1534272741646,18.5935761222833,12.));
#250520=CARTESIAN_POINT('Ctrl Pts',(17.1286318741185,18.5843373717253,12.));
#250521=CARTESIAN_POINT('Ctrl Pts',(17.1039288260001,18.5750678188543,12.));
#250522=CARTESIAN_POINT('Ctrl Pts',(17.0793184636079,18.5657678479788,12.));
#250523=CARTESIAN_POINT('Ctrl Pts',(17.0548011239751,18.5564378489628,12.));
#250524=CARTESIAN_POINT('Ctrl Pts',(17.030377148174,18.5470782182089,12.));
#250525=CARTESIAN_POINT('Ctrl Pts',(17.0060468805099,18.5376893576961,12.));
#250526=CARTESIAN_POINT('Ctrl Pts',(16.9818106680382,18.5282716744198,12.));
#250527=CARTESIAN_POINT('Ctrl Pts',(16.957668859934,18.518825579666,12.));
#250528=CARTESIAN_POINT('Ctrl Pts',(16.9336218069353,18.5093514883835,12.));
#250529=CARTESIAN_POINT('Ctrl Pts',(16.9096698606942,18.4998498184619,12.));
#250530=CARTESIAN_POINT('Ctrl Pts',(16.8858133733086,18.4903209902226,12.));
#250531=CARTESIAN_POINT('Ctrl Pts',(16.8620526977169,18.4807654268769,12.));
#250532=CARTESIAN_POINT('Ctrl Pts',(16.8383881879707,18.4711835548622,12.));
#250533=CARTESIAN_POINT('Ctrl Pts',(16.8148201995472,18.4615758042305,12.));
#250534=CARTESIAN_POINT('Ctrl Pts',(16.791349089629,18.4519426090124,12.));
#250535=CARTESIAN_POINT('Ctrl Pts',(16.7679752173992,18.4422844076099,12.));
#250536=CARTESIAN_POINT('Ctrl Pts',(16.7446989442882,18.4326016431392,12.));
#250537=CARTESIAN_POINT('Ctrl Pts',(16.7215206338818,18.4228947633186,12.));
#250538=CARTESIAN_POINT('Ctrl Pts',(16.698440651849,18.413164220399,12.));
#250539=CARTESIAN_POINT('Ctrl Pts',(16.6754593658513,18.4034104710789,12.));
#250540=CARTESIAN_POINT('Ctrl Pts',(16.6525771454513,18.3936339764332,12.));
#250541=CARTESIAN_POINT('Ctrl Pts',(16.6297943620056,18.3838352018327,12.));
#250542=CARTESIAN_POINT('Ctrl Pts',(16.6071113885711,18.3740146168879,12.));
#250543=CARTESIAN_POINT('Ctrl Pts',(16.5845286000218,18.364172695589,12.));
#250544=CARTESIAN_POINT('Ctrl Pts',(16.5620463731414,18.3543099164331,12.));
#250545=CARTESIAN_POINT('Ctrl Pts',(16.5396650867139,18.3444267625601,12.));
#250546=CARTESIAN_POINT('Ctrl Pts',(16.5173851216045,18.3345237218864,12.));
#250547=CARTESIAN_POINT('Ctrl Pts',(16.4952068608344,18.3246012872468,12.));
#250548=CARTESIAN_POINT('Ctrl Pts',(16.4731306896439,18.3146599565229,12.));
#250549=CARTESIAN_POINT('Ctrl Pts',(16.4511569955231,18.3047002326858,12.));
#250550=CARTESIAN_POINT('Ctrl Pts',(16.4292861682377,18.2947226238509,12.));
#250551=CARTESIAN_POINT('Ctrl Pts',(16.4075185998454,18.2847276433308,12.));
#250552=CARTESIAN_POINT('Ctrl Pts',(16.385854684708,18.2747158096934,12.));
#250553=CARTESIAN_POINT('Ctrl Pts',(16.3642948194869,18.2646876468169,12.));
#250554=CARTESIAN_POINT('Ctrl Pts',(16.342839403159,18.2546436839609,12.));
#250555=CARTESIAN_POINT('Ctrl Pts',(16.3214888370988,18.2445844558742,12.));
#250556=CARTESIAN_POINT('Ctrl Pts',(16.3002435251378,18.2345105028981,12.));
#250557=CARTESIAN_POINT('Ctrl Pts',(16.2791038736223,18.2244223710745,12.));
#250558=CARTESIAN_POINT('Ctrl Pts',(16.2580702914615,18.214320612253,12.));
#250559=CARTESIAN_POINT('Ctrl Pts',(16.237143190164,18.2042057842037,12.));
#250560=CARTESIAN_POINT('Ctrl Pts',(16.2163229838878,18.1940784507232,12.));
#250561=CARTESIAN_POINT('Ctrl Pts',(16.1956100895076,18.1839391817335,12.));
#250562=CARTESIAN_POINT('Ctrl Pts',(16.1750049266673,18.1737885533852,12.));
#250563=CARTESIAN_POINT('Ctrl Pts',(16.1545079178261,18.1636271481616,12.));
#250564=CARTESIAN_POINT('Ctrl Pts',(16.1341194882987,18.1534555549851,12.));
#250565=CARTESIAN_POINT('Ctrl Pts',(16.113840066279,18.1432743693231,12.));
#250566=CARTESIAN_POINT('Ctrl Pts',(16.0936700829108,18.1330841933099,12.));
#250567=CARTESIAN_POINT('Ctrl Pts',(16.0736099723664,18.1228856358746,12.));
#250568=CARTESIAN_POINT('Ctrl Pts',(16.0536601719124,18.1126793128688,12.));
#250569=CARTESIAN_POINT('Ctrl Pts',(16.0338211219693,18.1024658471966,12.));
#250570=CARTESIAN_POINT('Ctrl Pts',(16.0140932661612,18.0922458689464,12.));
#250571=CARTESIAN_POINT('Ctrl Pts',(15.9944770513616,18.0820200155239,12.));
#250572=CARTESIAN_POINT('Ctrl Pts',(15.9749729277848,18.071788931796,12.));
#250573=CARTESIAN_POINT('Ctrl Pts',(15.9555813490645,18.061553270236,12.));
#250574=CARTESIAN_POINT('Ctrl Pts',(15.9363027723244,18.0513136910691,12.));
#250575=CARTESIAN_POINT('Ctrl Pts',(15.9171376582436,18.0410708624208,12.));
#250576=CARTESIAN_POINT('Ctrl Pts',(15.8980864711043,18.0308254604638,12.));
#250577=CARTESIAN_POINT('Ctrl Pts',(15.8791496788685,18.0205781695773,12.));
#250578=CARTESIAN_POINT('Ctrl Pts',(15.8603277532834,18.010329682521,12.));
#250579=CARTESIAN_POINT('Ctrl Pts',(15.8416211699681,18.0000807006055,12.));
#250580=CARTESIAN_POINT('Ctrl Pts',(15.8230304084963,17.9898319338664,12.));
#250581=CARTESIAN_POINT('Ctrl Pts',(15.8045559524674,17.9795841012383,12.));
#250582=CARTESIAN_POINT('Ctrl Pts',(15.786198289572,17.9693379307297,12.));
#250583=CARTESIAN_POINT('Ctrl Pts',(15.7679579117072,17.9590941596236,12.));
#250584=CARTESIAN_POINT('Ctrl Pts',(15.7498353150856,17.9488535346776,12.));
#250585=CARTESIAN_POINT('Ctrl Pts',(15.7318310003334,17.9386168123261,12.));
#250586=CARTESIAN_POINT('Ctrl Pts',(15.713945472584,17.9283847588837,12.));
#250587=CARTESIAN_POINT('Ctrl Pts',(15.6961792415526,17.918158150746,12.));
#250588=CARTESIAN_POINT('Ctrl Pts',(15.6785328216467,17.9079377746118,12.));
#250589=CARTESIAN_POINT('Ctrl Pts',(15.6610067321036,17.8977244277247,12.));
#250590=CARTESIAN_POINT('Ctrl Pts',(15.6436014971088,17.8875189181095,12.));
#250591=CARTESIAN_POINT('Ctrl Pts',(15.6263176459107,17.8773220648125,12.));
#250592=CARTESIAN_POINT('Ctrl Pts',(15.6091557129205,17.8671346981388,12.));
#250593=CARTESIAN_POINT('Ctrl Pts',(15.5921162378183,17.8569576598996,12.));
#250594=CARTESIAN_POINT('Ctrl Pts',(15.5751997657153,17.8467918036977,12.));
#250595=CARTESIAN_POINT('Ctrl Pts',(15.5584068472976,17.8366379952078,12.));
#250596=CARTESIAN_POINT('Ctrl Pts',(15.5417380389639,17.8264971124606,12.));
#250597=CARTESIAN_POINT('Ctrl Pts',(15.5251939029558,17.8163700461263,12.));
#250598=CARTESIAN_POINT('Ctrl Pts',(15.5087750074728,17.8062576997964,12.));
#250599=CARTESIAN_POINT('Ctrl Pts',(15.4924819268529,17.7961609903161,12.));
#250600=CARTESIAN_POINT('Ctrl Pts',(15.4763152417506,17.7860808481229,12.));
#250601=CARTESIAN_POINT('Ctrl Pts',(15.4602755393019,17.7760182175817,12.));
#250602=CARTESIAN_POINT('Ctrl Pts',(15.4443634132865,17.765974057326,12.));
#250603=CARTESIAN_POINT('Ctrl Pts',(15.4285794642658,17.7559493405871,12.));
#250604=CARTESIAN_POINT('Ctrl Pts',(15.4129242997828,17.7459450555803,12.));
#250605=CARTESIAN_POINT('Ctrl Pts',(15.3973985345796,17.7359622059143,12.));
#250606=CARTESIAN_POINT('Ctrl Pts',(15.3820027907965,17.7260018109923,12.));
#250607=CARTESIAN_POINT('Ctrl Pts',(15.3667376981702,17.7160649064208,12.));
#250608=CARTESIAN_POINT('Ctrl Pts',(15.3516038942064,17.7061525444044,12.));
#250609=CARTESIAN_POINT('Ctrl Pts',(15.3366020244069,17.6962657941984,12.));
#250610=CARTESIAN_POINT('Ctrl Pts',(15.3217327425341,17.6864057426052,12.));
#250611=CARTESIAN_POINT('Ctrl Pts',(15.3069967108501,17.6765734944559,12.));
#250612=CARTESIAN_POINT('Ctrl Pts',(15.2923946003598,17.6667701731041,12.));
#250613=CARTESIAN_POINT('Ctrl Pts',(15.2779270910238,17.6569969209,12.));
#250614=CARTESIAN_POINT('Ctrl Pts',(15.263594872029,17.6472548997329,12.));
#250615=CARTESIAN_POINT('Ctrl Pts',(15.2493986421091,17.637545291637,12.));
#250616=CARTESIAN_POINT('Ctrl Pts',(15.2353391098367,17.6278692993765,12.));
#250617=CARTESIAN_POINT('Ctrl Pts',(15.22141699392,17.6182281470467,12.));
#250618=CARTESIAN_POINT('Ctrl Pts',(15.2076330234686,17.6086230806497,12.));
#250619=CARTESIAN_POINT('Ctrl Pts',(15.1939879383268,17.5990553687595,12.));
#250620=CARTESIAN_POINT('Ctrl Pts',(15.1804824894605,17.5895263032592,12.));
#250621=CARTESIAN_POINT('Ctrl Pts',(15.1671174393136,17.5800372000539,12.));
#250622=CARTESIAN_POINT('Ctrl Pts',(15.1538935621714,17.570589399803,12.));
#250623=CARTESIAN_POINT('Ctrl Pts',(15.1408116444877,17.5611842686196,12.));
#250624=CARTESIAN_POINT('Ctrl Pts',(15.127872485314,17.5518231989122,12.));
#250625=CARTESIAN_POINT('Ctrl Pts',(15.1150768967729,17.5425076102966,12.));
#250626=CARTESIAN_POINT('Ctrl Pts',(15.1024257045033,17.5332389504829,12.));
#250627=CARTESIAN_POINT('Ctrl Pts',(15.0899197481082,17.5240186961788,12.));
#250628=CARTESIAN_POINT('Ctrl Pts',(15.0775598815748,17.5148483539684,12.));
#250629=CARTESIAN_POINT('Ctrl Pts',(15.0653469738306,17.5057294613874,12.));
#250630=CARTESIAN_POINT('Ctrl Pts',(15.0532819093085,17.4966635880245,12.));
#250631=CARTESIAN_POINT('Ctrl Pts',(15.0413655884993,17.4876523366178,12.));
#250632=CARTESIAN_POINT('Ctrl Pts',(15.029598928488,17.4786973441417,12.));
#250633=CARTESIAN_POINT('Ctrl Pts',(15.0179828635086,17.4698002829357,12.));
#250634=CARTESIAN_POINT('Ctrl Pts',(15.0065183456921,17.4609628621418,12.));
#250635=CARTESIAN_POINT('Ctrl Pts',(14.9952063457778,17.4521868291004,12.));
#250636=CARTESIAN_POINT('Ctrl Pts',(14.9840478538358,17.4434739707773,12.));
#250637=CARTESIAN_POINT('Ctrl Pts',(14.9730438799452,17.4348261151396,12.));
#250638=CARTESIAN_POINT('Ctrl Pts',(14.9621954549827,17.426245132709,12.));
#250639=CARTESIAN_POINT('Ctrl Pts',(14.9515036315143,17.4177329382828,12.));
#250640=CARTESIAN_POINT('Ctrl Pts',(14.940969484645,17.4092914926071,12.));
#250641=CARTESIAN_POINT('Ctrl Pts',(14.9305941128757,17.4009228040749,12.));
#250642=CARTESIAN_POINT('Ctrl Pts',(14.9203786389342,17.3926289303986,12.));
#250643=CARTESIAN_POINT('Ctrl Pts',(14.9103242110057,17.3844119809824,12.));
#250644=CARTESIAN_POINT('Ctrl Pts',(14.900432003961,17.3762741193076,12.));
#250645=CARTESIAN_POINT('Ctrl Pts',(14.8907032205788,17.3682175653235,12.));
#250646=CARTESIAN_POINT('Ctrl Pts',(14.8811390927423,17.3602445978161,12.));
#250647=CARTESIAN_POINT('Ctrl Pts',(14.8717408826955,17.3523575568645,12.));
#250648=CARTESIAN_POINT('Ctrl Pts',(14.8625098843417,17.3445588463475,12.));
#250649=CARTESIAN_POINT('Ctrl Pts',(14.8534474245433,17.336850936485,12.));
#250650=CARTESIAN_POINT('Ctrl Pts',(14.8445548643508,17.3292363662605,12.));
#250651=CARTESIAN_POINT('Ctrl Pts',(14.8358336004197,17.3217177462101,12.));
#250652=CARTESIAN_POINT('Ctrl Pts',(14.8272850675379,17.3142977632659,12.));
#250653=CARTESIAN_POINT('Ctrl Pts',(14.8189107410162,17.3069791853706,12.));
#250654=CARTESIAN_POINT('Ctrl Pts',(14.8107121391035,17.299764866148,12.));
#250655=CARTESIAN_POINT('Ctrl Pts',(14.8026908254276,17.2926577496513,12.));
#250656=CARTESIAN_POINT('Ctrl Pts',(14.7948484105249,17.2856608733196,12.));
#250657=CARTESIAN_POINT('Ctrl Pts',(14.787186553128,17.2787773704849,12.));
#250658=CARTESIAN_POINT('Ctrl Pts',(14.7797069617804,17.2720104735194,12.));
#250659=CARTESIAN_POINT('Ctrl Pts',(14.7724113956731,17.2653635155319,12.));
#250660=CARTESIAN_POINT('Ctrl Pts',(14.7653016697591,17.2588399401465,12.));
#250661=CARTESIAN_POINT('Ctrl Pts',(14.7583796616617,17.2524433146837,12.));
#250662=CARTESIAN_POINT('Ctrl Pts',(14.7516473175124,17.2461773413288,12.));
#250663=CARTESIAN_POINT('Ctrl Pts',(14.7451066593792,17.2400458713565,12.));
#250664=CARTESIAN_POINT('Ctrl Pts',(14.7387597858116,17.2340529062076,12.));
#250665=CARTESIAN_POINT('Ctrl Pts',(14.7326088681163,17.2282025904314,12.));
#250666=CARTESIAN_POINT('Ctrl Pts',(14.7266561494282,17.2224992099667,12.));
#250667=CARTESIAN_POINT('Ctrl Pts',(14.7209039390327,17.2169471814256,12.));
#250668=CARTESIAN_POINT('Ctrl Pts',(14.7153546289339,17.2115510835989,12.));
#250669=CARTESIAN_POINT('Ctrl Pts',(14.7100107213586,17.2063157097315,12.));
#250670=CARTESIAN_POINT('Ctrl Pts',(14.7048748502663,17.2012461084268,12.));
#250671=CARTESIAN_POINT('Ctrl Pts',(14.699949811582,17.1963476411694,12.));
#250672=CARTESIAN_POINT('Ctrl Pts',(14.6952385361705,17.1916259308415,12.));
#250673=CARTESIAN_POINT('Ctrl Pts',(14.6907440526958,17.1870867909918,12.));
#250674=CARTESIAN_POINT('Ctrl Pts',(14.686469452232,17.182736158472,12.));
#250675=CARTESIAN_POINT('Ctrl Pts',(14.6824178576167,17.1785800350826,12.));
#250676=CARTESIAN_POINT('Ctrl Pts',(14.6785925615677,17.1746247499057,12.));
#250677=CARTESIAN_POINT('Ctrl Pts',(14.6749971333867,17.1708771619129,12.));
#250678=CARTESIAN_POINT('Ctrl Pts',(14.671635583332,17.167344972302,12.));
#250679=CARTESIAN_POINT('Ctrl Pts',(14.6685123374423,17.1640366762305,12.));
#250680=CARTESIAN_POINT('Ctrl Pts',(14.6656319165057,17.1609609517369,12.));
#250681=CARTESIAN_POINT('Ctrl Pts',(14.6629987285992,17.1581262646789,12.));
#250682=CARTESIAN_POINT('Ctrl Pts',(14.6606167169642,17.1555401986401,12.));
#250683=CARTESIAN_POINT('Ctrl Pts',(14.6584900555302,17.1532107762718,12.));
#250684=CARTESIAN_POINT('Ctrl Pts',(14.6566237952435,17.1511476869496,12.));
#250685=CARTESIAN_POINT('Ctrl Pts',(14.655024862281,17.1493641837558,12.));
#250686=CARTESIAN_POINT('Ctrl Pts',(14.6537016966184,17.147876394491,12.));
#250687=CARTESIAN_POINT('Ctrl Pts',(14.6526624064978,17.1466998098673,12.));
#250688=CARTESIAN_POINT('Ctrl Pts',(14.6519131634508,17.1458462295271,12.));
#250689=CARTESIAN_POINT('Ctrl Pts',(14.6515481598068,17.1454262858043,12.));
#250690=CARTESIAN_POINT('Ctrl Pts',(14.6514066997196,17.1452600887037,12.));
#250691=CARTESIAN_POINT('Ctrl Pts',(14.6513711852843,17.1452153999142,12.));
#250692=CARTESIAN_POINT('Ctrl Pts',(14.6513681262571,17.1452095830633,12.));
#250693=CARTESIAN_POINT('',(17.9112098770111,18.8464468996588,0.));
#250694=CARTESIAN_POINT('Origin',(17.7219872369693,12.1729687575668,0.));
#250695=CARTESIAN_POINT('',(18.5896416359912,12.7689476255363,12.));
#250696=CARTESIAN_POINT('',(8.86099361848466,6.08648437878338,12.));
#250697=CARTESIAN_POINT('',(18.5896416359912,12.7689476255363,0.));
#250698=CARTESIAN_POINT('',(18.5896416359912,12.7689476255363,0.));
#250699=CARTESIAN_POINT('',(8.86099361848466,6.08648437878338,0.));
#250700=CARTESIAN_POINT('Ctrl Pts',(18.8464468996588,17.9112098770111,0.));
#250701=CARTESIAN_POINT('Ctrl Pts',(18.8464468996588,17.9112098770111,12.));
#250702=CARTESIAN_POINT('Ctrl Pts',(18.8448126709691,17.9057348246595,0.));
#250703=CARTESIAN_POINT('Ctrl Pts',(18.8448126709691,17.9057348246595,12.));
#250704=CARTESIAN_POINT('Ctrl Pts',(18.8415402351786,17.8947931177807,0.));
#250705=CARTESIAN_POINT('Ctrl Pts',(18.8415402351786,17.8947931177807,12.));
#250706=CARTESIAN_POINT('Ctrl Pts',(18.8366196462581,17.8784057509356,0.));
#250707=CARTESIAN_POINT('Ctrl Pts',(18.8366196462581,17.8784057509356,12.));
#250708=CARTESIAN_POINT('Ctrl Pts',(18.8300349895974,17.8566063174771,0.));
#250709=CARTESIAN_POINT('Ctrl Pts',(18.8300349895974,17.8566063174771,12.));
#250710=CARTESIAN_POINT('Ctrl Pts',(18.8217643886157,17.8294410311006,0.));
#250711=CARTESIAN_POINT('Ctrl Pts',(18.8217643886157,17.8294410311006,12.));
#250712=CARTESIAN_POINT('Ctrl Pts',(18.8134540340417,17.8023598011057,0.));
#250713=CARTESIAN_POINT('Ctrl Pts',(18.8134540340417,17.8023598011057,12.));
#250714=CARTESIAN_POINT('Ctrl Pts',(18.8051039860448,17.7753627137853,0.));
#250715=CARTESIAN_POINT('Ctrl Pts',(18.8051039860448,17.7753627137853,12.));
#250716=CARTESIAN_POINT('Ctrl Pts',(18.7967143519419,17.7484498996905,0.));
#250717=CARTESIAN_POINT('Ctrl Pts',(18.7967143519419,17.7484498996905,12.));
#250718=CARTESIAN_POINT('Ctrl Pts',(18.7882852976049,17.7216215409035,0.));
#250719=CARTESIAN_POINT('Ctrl Pts',(18.7882852976049,17.7216215409035,12.));
#250720=CARTESIAN_POINT('Ctrl Pts',(18.7798170641374,17.6948778823014,0.));
#250721=CARTESIAN_POINT('Ctrl Pts',(18.7798170641374,17.6948778823014,12.));
#250722=CARTESIAN_POINT('Ctrl Pts',(18.7713099642754,17.6682192274236,0.));
#250723=CARTESIAN_POINT('Ctrl Pts',(18.7713099642754,17.6682192274236,12.));
#250724=CARTESIAN_POINT('Ctrl Pts',(18.762764361321,17.6416459210681,0.));
#250725=CARTESIAN_POINT('Ctrl Pts',(18.762764361321,17.6416459210681,12.));
#250726=CARTESIAN_POINT('Ctrl Pts',(18.7541806530984,17.6151583357012,0.));
#250727=CARTESIAN_POINT('Ctrl Pts',(18.7541806530984,17.6151583357012,12.));
#250728=CARTESIAN_POINT('Ctrl Pts',(18.7455592536687,17.5887568561371,0.));
#250729=CARTESIAN_POINT('Ctrl Pts',(18.7455592536687,17.5887568561371,12.));
#250730=CARTESIAN_POINT('Ctrl Pts',(18.7369005764553,17.5624418653245,0.));
#250731=CARTESIAN_POINT('Ctrl Pts',(18.7369005764553,17.5624418653245,12.));
#250732=CARTESIAN_POINT('Ctrl Pts',(18.7282050157138,17.5362137287593,0.));
#250733=CARTESIAN_POINT('Ctrl Pts',(18.7282050157138,17.5362137287593,12.));
#250734=CARTESIAN_POINT('Ctrl Pts',(18.7194729318098,17.5100727820876,0.));
#250735=CARTESIAN_POINT('Ctrl Pts',(18.7194729318098,17.5100727820876,12.));
#250736=CARTESIAN_POINT('Ctrl Pts',(18.7107046613912,17.4840193397162,0.));
#250737=CARTESIAN_POINT('Ctrl Pts',(18.7107046613912,17.4840193397162,12.));
#250738=CARTESIAN_POINT('Ctrl Pts',(18.70190052503,17.4580537012753,0.));
#250739=CARTESIAN_POINT('Ctrl Pts',(18.70190052503,17.4580537012753,12.));
#250740=CARTESIAN_POINT('Ctrl Pts',(18.6930608357409,17.4321761588142,0.));
#250741=CARTESIAN_POINT('Ctrl Pts',(18.6930608357409,17.4321761588142,12.));
#250742=CARTESIAN_POINT('Ctrl Pts',(18.6841859073471,17.4063870038562,0.));
#250743=CARTESIAN_POINT('Ctrl Pts',(18.6841859073471,17.4063870038562,12.));
#250744=CARTESIAN_POINT('Ctrl Pts',(18.6752760624052,17.3806865340747,0.));
#250745=CARTESIAN_POINT('Ctrl Pts',(18.6752760624052,17.3806865340747,12.));
#250746=CARTESIAN_POINT('Ctrl Pts',(18.6663316416582,17.3550750612443,0.));
#250747=CARTESIAN_POINT('Ctrl Pts',(18.6663316416582,17.3550750612443,12.));
#250748=CARTESIAN_POINT('Ctrl Pts',(18.6573530024033,17.3295529098618,0.));
#250749=CARTESIAN_POINT('Ctrl Pts',(18.6573530024033,17.3295529098618,12.));
#250750=CARTESIAN_POINT('Ctrl Pts',(18.6483405141865,17.3041204135074,0.));
#250751=CARTESIAN_POINT('Ctrl Pts',(18.6483405141865,17.3041204135074,12.));
#250752=CARTESIAN_POINT('Ctrl Pts',(18.6392945554748,17.2787779120213,0.));
#250753=CARTESIAN_POINT('Ctrl Pts',(18.6392945554748,17.2787779120213,12.));
#250754=CARTESIAN_POINT('Ctrl Pts',(18.6302155097943,17.2535257482187,0.));
#250755=CARTESIAN_POINT('Ctrl Pts',(18.6302155097943,17.2535257482187,12.));
#250756=CARTESIAN_POINT('Ctrl Pts',(18.6211037624038,17.2283642650518,0.));
#250757=CARTESIAN_POINT('Ctrl Pts',(18.6211037624038,17.2283642650518,12.));
#250758=CARTESIAN_POINT('Ctrl Pts',(18.6119596959949,17.2032938019284,0.));
#250759=CARTESIAN_POINT('Ctrl Pts',(18.6119596959949,17.2032938019284,12.));
#250760=CARTESIAN_POINT('Ctrl Pts',(18.6027836898817,17.1783146940127,0.));
#250761=CARTESIAN_POINT('Ctrl Pts',(18.6027836898817,17.1783146940127,12.));
#250762=CARTESIAN_POINT('Ctrl Pts',(18.5935761222825,17.1534272741643,0.));
#250763=CARTESIAN_POINT('Ctrl Pts',(18.5935761222825,17.1534272741643,12.));
#250764=CARTESIAN_POINT('Ctrl Pts',(18.5843373717247,17.1286318741183,0.));
#250765=CARTESIAN_POINT('Ctrl Pts',(18.5843373717247,17.1286318741183,12.));
#250766=CARTESIAN_POINT('Ctrl Pts',(18.5750678188542,17.1039288260001,0.));
#250767=CARTESIAN_POINT('Ctrl Pts',(18.5750678188542,17.1039288260001,12.));
#250768=CARTESIAN_POINT('Ctrl Pts',(18.5657678479789,17.0793184636079,0.));
#250769=CARTESIAN_POINT('Ctrl Pts',(18.5657678479789,17.0793184636079,12.));
#250770=CARTESIAN_POINT('Ctrl Pts',(18.556437848963,17.0548011239751,0.));
#250771=CARTESIAN_POINT('Ctrl Pts',(18.556437848963,17.0548011239751,12.));
#250772=CARTESIAN_POINT('Ctrl Pts',(18.547078218209,17.0303771481738,0.));
#250773=CARTESIAN_POINT('Ctrl Pts',(18.547078218209,17.0303771481738,12.));
#250774=CARTESIAN_POINT('Ctrl Pts',(18.5376893576961,17.0060468805097,0.));
#250775=CARTESIAN_POINT('Ctrl Pts',(18.5376893576961,17.0060468805097,12.));
#250776=CARTESIAN_POINT('Ctrl Pts',(18.5282716744197,16.981810668038,0.));
#250777=CARTESIAN_POINT('Ctrl Pts',(18.5282716744197,16.981810668038,12.));
#250778=CARTESIAN_POINT('Ctrl Pts',(18.5188255796659,16.9576688599339,0.));
#250779=CARTESIAN_POINT('Ctrl Pts',(18.5188255796659,16.9576688599339,12.));
#250780=CARTESIAN_POINT('Ctrl Pts',(18.5093514883835,16.9336218069353,0.));
#250781=CARTESIAN_POINT('Ctrl Pts',(18.5093514883835,16.9336218069353,12.));
#250782=CARTESIAN_POINT('Ctrl Pts',(18.499849818462,16.9096698606943,0.));
#250783=CARTESIAN_POINT('Ctrl Pts',(18.499849818462,16.9096698606943,12.));
#250784=CARTESIAN_POINT('Ctrl Pts',(18.4903209902227,16.8858133733088,0.));
#250785=CARTESIAN_POINT('Ctrl Pts',(18.4903209902227,16.8858133733088,12.));
#250786=CARTESIAN_POINT('Ctrl Pts',(18.4807654268771,16.8620526977171,0.));
#250787=CARTESIAN_POINT('Ctrl Pts',(18.4807654268771,16.8620526977171,12.));
#250788=CARTESIAN_POINT('Ctrl Pts',(18.4711835548623,16.8383881879709,0.));
#250789=CARTESIAN_POINT('Ctrl Pts',(18.4711835548623,16.8383881879709,12.));
#250790=CARTESIAN_POINT('Ctrl Pts',(18.4615758042305,16.8148201995472,0.));
#250791=CARTESIAN_POINT('Ctrl Pts',(18.4615758042305,16.8148201995472,12.));
#250792=CARTESIAN_POINT('Ctrl Pts',(18.4519426090123,16.791349089629,0.));
#250793=CARTESIAN_POINT('Ctrl Pts',(18.4519426090123,16.791349089629,12.));
#250794=CARTESIAN_POINT('Ctrl Pts',(18.44228440761,16.7679752173992,0.));
#250795=CARTESIAN_POINT('Ctrl Pts',(18.44228440761,16.7679752173992,12.));
#250796=CARTESIAN_POINT('Ctrl Pts',(18.4326016431392,16.7446989442882,0.));
#250797=CARTESIAN_POINT('Ctrl Pts',(18.4326016431392,16.7446989442882,12.));
#250798=CARTESIAN_POINT('Ctrl Pts',(18.4228947633187,16.7215206338818,0.));
#250799=CARTESIAN_POINT('Ctrl Pts',(18.4228947633187,16.7215206338818,12.));
#250800=CARTESIAN_POINT('Ctrl Pts',(18.413164220399,16.6984406518491,0.));
#250801=CARTESIAN_POINT('Ctrl Pts',(18.413164220399,16.6984406518491,12.));
#250802=CARTESIAN_POINT('Ctrl Pts',(18.403410471079,16.6754593658513,0.));
#250803=CARTESIAN_POINT('Ctrl Pts',(18.403410471079,16.6754593658513,12.));
#250804=CARTESIAN_POINT('Ctrl Pts',(18.3936339764332,16.6525771454513,0.));
#250805=CARTESIAN_POINT('Ctrl Pts',(18.3936339764332,16.6525771454513,12.));
#250806=CARTESIAN_POINT('Ctrl Pts',(18.3838352018327,16.6297943620056,0.));
#250807=CARTESIAN_POINT('Ctrl Pts',(18.3838352018327,16.6297943620056,12.));
#250808=CARTESIAN_POINT('Ctrl Pts',(18.3740146168879,16.607111388571,0.));
#250809=CARTESIAN_POINT('Ctrl Pts',(18.3740146168879,16.607111388571,12.));
#250810=CARTESIAN_POINT('Ctrl Pts',(18.3641726955889,16.5845286000217,0.));
#250811=CARTESIAN_POINT('Ctrl Pts',(18.3641726955889,16.5845286000217,12.));
#250812=CARTESIAN_POINT('Ctrl Pts',(18.354309916433,16.5620463731413,0.));
#250813=CARTESIAN_POINT('Ctrl Pts',(18.354309916433,16.5620463731413,12.));
#250814=CARTESIAN_POINT('Ctrl Pts',(18.34442676256,16.5396650867139,0.));
#250815=CARTESIAN_POINT('Ctrl Pts',(18.34442676256,16.5396650867139,12.));
#250816=CARTESIAN_POINT('Ctrl Pts',(18.3345237218864,16.5173851216045,0.));
#250817=CARTESIAN_POINT('Ctrl Pts',(18.3345237218864,16.5173851216045,12.));
#250818=CARTESIAN_POINT('Ctrl Pts',(18.3246012872469,16.4952068608345,0.));
#250819=CARTESIAN_POINT('Ctrl Pts',(18.3246012872469,16.4952068608345,12.));
#250820=CARTESIAN_POINT('Ctrl Pts',(18.3146599565231,16.4731306896441,0.));
#250821=CARTESIAN_POINT('Ctrl Pts',(18.3146599565231,16.4731306896441,12.));
#250822=CARTESIAN_POINT('Ctrl Pts',(18.304700232686,16.4511569955233,0.));
#250823=CARTESIAN_POINT('Ctrl Pts',(18.304700232686,16.4511569955233,12.));
#250824=CARTESIAN_POINT('Ctrl Pts',(18.294722623851,16.4292861682379,0.));
#250825=CARTESIAN_POINT('Ctrl Pts',(18.294722623851,16.4292861682379,12.));
#250826=CARTESIAN_POINT('Ctrl Pts',(18.2847276433309,16.4075185998455,0.));
#250827=CARTESIAN_POINT('Ctrl Pts',(18.2847276433309,16.4075185998455,12.));
#250828=CARTESIAN_POINT('Ctrl Pts',(18.2747158096934,16.385854684708,0.));
#250829=CARTESIAN_POINT('Ctrl Pts',(18.2747158096934,16.385854684708,12.));
#250830=CARTESIAN_POINT('Ctrl Pts',(18.2646876468169,16.3642948194868,0.));
#250831=CARTESIAN_POINT('Ctrl Pts',(18.2646876468169,16.3642948194868,12.));
#250832=CARTESIAN_POINT('Ctrl Pts',(18.2546436839608,16.3428394031589,0.));
#250833=CARTESIAN_POINT('Ctrl Pts',(18.2546436839608,16.3428394031589,12.));
#250834=CARTESIAN_POINT('Ctrl Pts',(18.2445844558742,16.3214888370987,0.));
#250835=CARTESIAN_POINT('Ctrl Pts',(18.2445844558742,16.3214888370987,12.));
#250836=CARTESIAN_POINT('Ctrl Pts',(18.2345105028982,16.3002435251378,0.));
#250837=CARTESIAN_POINT('Ctrl Pts',(18.2345105028982,16.3002435251378,12.));
#250838=CARTESIAN_POINT('Ctrl Pts',(18.2244223710745,16.2791038736223,0.));
#250839=CARTESIAN_POINT('Ctrl Pts',(18.2244223710745,16.2791038736223,12.));
#250840=CARTESIAN_POINT('Ctrl Pts',(18.2143206122529,16.2580702914615,0.));
#250841=CARTESIAN_POINT('Ctrl Pts',(18.2143206122529,16.2580702914615,12.));
#250842=CARTESIAN_POINT('Ctrl Pts',(18.2042057842035,16.2371431901638,0.));
#250843=CARTESIAN_POINT('Ctrl Pts',(18.2042057842035,16.2371431901638,12.));
#250844=CARTESIAN_POINT('Ctrl Pts',(18.1940784507229,16.2163229838875,0.));
#250845=CARTESIAN_POINT('Ctrl Pts',(18.1940784507229,16.2163229838875,12.));
#250846=CARTESIAN_POINT('Ctrl Pts',(18.1839391817331,16.1956100895073,0.));
#250847=CARTESIAN_POINT('Ctrl Pts',(18.1839391817331,16.1956100895073,12.));
#250848=CARTESIAN_POINT('Ctrl Pts',(18.1737885533849,16.1750049266671,0.));
#250849=CARTESIAN_POINT('Ctrl Pts',(18.1737885533849,16.1750049266671,12.));
#250850=CARTESIAN_POINT('Ctrl Pts',(18.1636271481615,16.154507917826,0.));
#250851=CARTESIAN_POINT('Ctrl Pts',(18.1636271481615,16.154507917826,12.));
#250852=CARTESIAN_POINT('Ctrl Pts',(18.1534555549852,16.1341194882988,0.));
#250853=CARTESIAN_POINT('Ctrl Pts',(18.1534555549852,16.1341194882988,12.));
#250854=CARTESIAN_POINT('Ctrl Pts',(18.1432743693235,16.1138400662794,0.));
#250855=CARTESIAN_POINT('Ctrl Pts',(18.1432743693235,16.1138400662794,12.));
#250856=CARTESIAN_POINT('Ctrl Pts',(18.1330841933105,16.0936700829112,0.));
#250857=CARTESIAN_POINT('Ctrl Pts',(18.1330841933105,16.0936700829112,12.));
#250858=CARTESIAN_POINT('Ctrl Pts',(18.1228856358751,16.0736099723668,0.));
#250859=CARTESIAN_POINT('Ctrl Pts',(18.1228856358751,16.0736099723668,12.));
#250860=CARTESIAN_POINT('Ctrl Pts',(18.112679312869,16.0536601719126,0.));
#250861=CARTESIAN_POINT('Ctrl Pts',(18.112679312869,16.0536601719126,12.));
#250862=CARTESIAN_POINT('Ctrl Pts',(18.1024658471966,16.0338211219693,0.));
#250863=CARTESIAN_POINT('Ctrl Pts',(18.1024658471966,16.0338211219693,12.));
#250864=CARTESIAN_POINT('Ctrl Pts',(18.0922458689462,16.014093266161,0.));
#250865=CARTESIAN_POINT('Ctrl Pts',(18.0922458689462,16.014093266161,12.));
#250866=CARTESIAN_POINT('Ctrl Pts',(18.0820200155236,15.9944770513613,0.));
#250867=CARTESIAN_POINT('Ctrl Pts',(18.0820200155236,15.9944770513613,12.));
#250868=CARTESIAN_POINT('Ctrl Pts',(18.0717889317958,15.9749729277846,0.));
#250869=CARTESIAN_POINT('Ctrl Pts',(18.0717889317958,15.9749729277846,12.));
#250870=CARTESIAN_POINT('Ctrl Pts',(18.061553270236,15.9555813490644,0.));
#250871=CARTESIAN_POINT('Ctrl Pts',(18.061553270236,15.9555813490644,12.));
#250872=CARTESIAN_POINT('Ctrl Pts',(18.0513136910691,15.9363027723244,0.));
#250873=CARTESIAN_POINT('Ctrl Pts',(18.0513136910691,15.9363027723244,12.));
#250874=CARTESIAN_POINT('Ctrl Pts',(18.0410708624208,15.9171376582436,0.));
#250875=CARTESIAN_POINT('Ctrl Pts',(18.0410708624208,15.9171376582436,12.));
#250876=CARTESIAN_POINT('Ctrl Pts',(18.0308254604636,15.8980864711042,0.));
#250877=CARTESIAN_POINT('Ctrl Pts',(18.0308254604636,15.8980864711042,12.));
#250878=CARTESIAN_POINT('Ctrl Pts',(18.0205781695769,15.8791496788683,0.));
#250879=CARTESIAN_POINT('Ctrl Pts',(18.0205781695769,15.8791496788683,12.));
#250880=CARTESIAN_POINT('Ctrl Pts',(18.0103296825205,15.8603277532831,0.));
#250881=CARTESIAN_POINT('Ctrl Pts',(18.0103296825205,15.8603277532831,12.));
#250882=CARTESIAN_POINT('Ctrl Pts',(18.0000807006052,15.8416211699679,0.));
#250883=CARTESIAN_POINT('Ctrl Pts',(18.0000807006052,15.8416211699679,12.));
#250884=CARTESIAN_POINT('Ctrl Pts',(17.9898319338664,15.8230304084962,0.));
#250885=CARTESIAN_POINT('Ctrl Pts',(17.9898319338664,15.8230304084962,12.));
#250886=CARTESIAN_POINT('Ctrl Pts',(17.9795841012386,15.8045559524677,0.));
#250887=CARTESIAN_POINT('Ctrl Pts',(17.9795841012386,15.8045559524677,12.));
#250888=CARTESIAN_POINT('Ctrl Pts',(17.9693379307303,15.7861982895724,0.));
#250889=CARTESIAN_POINT('Ctrl Pts',(17.9693379307303,15.7861982895724,12.));
#250890=CARTESIAN_POINT('Ctrl Pts',(17.9590941596242,15.7679579117077,0.));
#250891=CARTESIAN_POINT('Ctrl Pts',(17.9590941596242,15.7679579117077,12.));
#250892=CARTESIAN_POINT('Ctrl Pts',(17.9488535346781,15.749835315086,0.));
#250893=CARTESIAN_POINT('Ctrl Pts',(17.9488535346781,15.749835315086,12.));
#250894=CARTESIAN_POINT('Ctrl Pts',(17.9386168123262,15.7318310003335,0.));
#250895=CARTESIAN_POINT('Ctrl Pts',(17.9386168123262,15.7318310003335,12.));
#250896=CARTESIAN_POINT('Ctrl Pts',(17.9283847588836,15.7139454725839,0.));
#250897=CARTESIAN_POINT('Ctrl Pts',(17.9283847588836,15.7139454725839,12.));
#250898=CARTESIAN_POINT('Ctrl Pts',(17.9181581507455,15.6961792415522,0.));
#250899=CARTESIAN_POINT('Ctrl Pts',(17.9181581507455,15.6961792415522,12.));
#250900=CARTESIAN_POINT('Ctrl Pts',(17.9079377746111,15.6785328216461,0.));
#250901=CARTESIAN_POINT('Ctrl Pts',(17.9079377746111,15.6785328216461,12.));
#250902=CARTESIAN_POINT('Ctrl Pts',(17.897724427724,15.661006732103,0.));
#250903=CARTESIAN_POINT('Ctrl Pts',(17.897724427724,15.661006732103,12.));
#250904=CARTESIAN_POINT('Ctrl Pts',(17.8875189181091,15.6436014971085,0.));
#250905=CARTESIAN_POINT('Ctrl Pts',(17.8875189181091,15.6436014971085,12.));
#250906=CARTESIAN_POINT('Ctrl Pts',(17.8773220648125,15.6263176459108,0.));
#250907=CARTESIAN_POINT('Ctrl Pts',(17.8773220648125,15.6263176459108,12.));
#250908=CARTESIAN_POINT('Ctrl Pts',(17.8671346981394,15.609155712921,0.));
#250909=CARTESIAN_POINT('Ctrl Pts',(17.8671346981394,15.609155712921,12.));
#250910=CARTESIAN_POINT('Ctrl Pts',(17.8569576599006,15.5921162378192,0.));
#250911=CARTESIAN_POINT('Ctrl Pts',(17.8569576599006,15.5921162378192,12.));
#250912=CARTESIAN_POINT('Ctrl Pts',(17.8467918036987,15.5751997657163,0.));
#250913=CARTESIAN_POINT('Ctrl Pts',(17.8467918036987,15.5751997657163,12.));
#250914=CARTESIAN_POINT('Ctrl Pts',(17.8366379952085,15.5584068472982,0.));
#250915=CARTESIAN_POINT('Ctrl Pts',(17.8366379952085,15.5584068472982,12.));
#250916=CARTESIAN_POINT('Ctrl Pts',(17.8264971124606,15.541738038964,0.));
#250917=CARTESIAN_POINT('Ctrl Pts',(17.8264971124606,15.541738038964,12.));
#250918=CARTESIAN_POINT('Ctrl Pts',(17.8163700461256,15.5251939029552,0.));
#250919=CARTESIAN_POINT('Ctrl Pts',(17.8163700461256,15.5251939029552,12.));
#250920=CARTESIAN_POINT('Ctrl Pts',(17.8062576997952,15.5087750074718,0.));
#250921=CARTESIAN_POINT('Ctrl Pts',(17.8062576997952,15.5087750074718,12.));
#250922=CARTESIAN_POINT('Ctrl Pts',(17.7961609903148,15.4924819268517,0.));
#250923=CARTESIAN_POINT('Ctrl Pts',(17.7961609903148,15.4924819268517,12.));
#250924=CARTESIAN_POINT('Ctrl Pts',(17.7860808481219,15.4763152417497,0.));
#250925=CARTESIAN_POINT('Ctrl Pts',(17.7860808481219,15.4763152417497,12.));
#250926=CARTESIAN_POINT('Ctrl Pts',(17.7760182175815,15.4602755393018,0.));
#250927=CARTESIAN_POINT('Ctrl Pts',(17.7760182175815,15.4602755393018,12.));
#250928=CARTESIAN_POINT('Ctrl Pts',(17.7659740573265,15.4443634132869,0.));
#250929=CARTESIAN_POINT('Ctrl Pts',(17.7659740573265,15.4443634132869,12.));
#250930=CARTESIAN_POINT('Ctrl Pts',(17.7559493405881,15.4285794642668,0.));
#250931=CARTESIAN_POINT('Ctrl Pts',(17.7559493405881,15.4285794642668,12.));
#250932=CARTESIAN_POINT('Ctrl Pts',(17.7459450555812,15.4129242997837,0.));
#250933=CARTESIAN_POINT('Ctrl Pts',(17.7459450555812,15.4129242997837,12.));
#250934=CARTESIAN_POINT('Ctrl Pts',(17.7359622059149,15.3973985345802,0.));
#250935=CARTESIAN_POINT('Ctrl Pts',(17.7359622059149,15.3973985345802,12.));
#250936=CARTESIAN_POINT('Ctrl Pts',(17.7260018109924,15.3820027907967,0.));
#250937=CARTESIAN_POINT('Ctrl Pts',(17.7260018109924,15.3820027907967,12.));
#250938=CARTESIAN_POINT('Ctrl Pts',(17.7160649064206,15.3667376981699,0.));
#250939=CARTESIAN_POINT('Ctrl Pts',(17.7160649064206,15.3667376981699,12.));
#250940=CARTESIAN_POINT('Ctrl Pts',(17.7061525444042,15.351603894206,0.));
#250941=CARTESIAN_POINT('Ctrl Pts',(17.7061525444042,15.351603894206,12.));
#250942=CARTESIAN_POINT('Ctrl Pts',(17.6962657941983,15.3366020244066,0.));
#250943=CARTESIAN_POINT('Ctrl Pts',(17.6962657941983,15.3366020244066,12.));
#250944=CARTESIAN_POINT('Ctrl Pts',(17.6864057426052,15.3217327425338,0.));
#250945=CARTESIAN_POINT('Ctrl Pts',(17.6864057426052,15.3217327425338,12.));
#250946=CARTESIAN_POINT('Ctrl Pts',(17.676573494456,15.3069967108501,0.));
#250947=CARTESIAN_POINT('Ctrl Pts',(17.676573494456,15.3069967108501,12.));
#250948=CARTESIAN_POINT('Ctrl Pts',(17.6667701731041,15.2923946003598,0.));
#250949=CARTESIAN_POINT('Ctrl Pts',(17.6667701731041,15.2923946003598,12.));
#250950=CARTESIAN_POINT('Ctrl Pts',(17.6569969209,15.2779270910239,0.));
#250951=CARTESIAN_POINT('Ctrl Pts',(17.6569969209,15.2779270910239,12.));
#250952=CARTESIAN_POINT('Ctrl Pts',(17.6472548997328,15.2635948720292,0.));
#250953=CARTESIAN_POINT('Ctrl Pts',(17.6472548997328,15.2635948720292,12.));
#250954=CARTESIAN_POINT('Ctrl Pts',(17.6375452916369,15.2493986421092,0.));
#250955=CARTESIAN_POINT('Ctrl Pts',(17.6375452916369,15.2493986421092,12.));
#250956=CARTESIAN_POINT('Ctrl Pts',(17.6278692993764,15.2353391098367,0.));
#250957=CARTESIAN_POINT('Ctrl Pts',(17.6278692993764,15.2353391098367,12.));
#250958=CARTESIAN_POINT('Ctrl Pts',(17.6182281470468,15.22141699392,0.));
#250959=CARTESIAN_POINT('Ctrl Pts',(17.6182281470468,15.22141699392,12.));
#250960=CARTESIAN_POINT('Ctrl Pts',(17.60862308065,15.2076330234686,0.));
#250961=CARTESIAN_POINT('Ctrl Pts',(17.60862308065,15.2076330234686,12.));
#250962=CARTESIAN_POINT('Ctrl Pts',(17.5990553687599,15.1939879383268,0.));
#250963=CARTESIAN_POINT('Ctrl Pts',(17.5990553687599,15.1939879383268,12.));
#250964=CARTESIAN_POINT('Ctrl Pts',(17.5895263032595,15.1804824894605,0.));
#250965=CARTESIAN_POINT('Ctrl Pts',(17.5895263032595,15.1804824894605,12.));
#250966=CARTESIAN_POINT('Ctrl Pts',(17.580037200054,15.1671174393137,0.));
#250967=CARTESIAN_POINT('Ctrl Pts',(17.580037200054,15.1671174393137,12.));
#250968=CARTESIAN_POINT('Ctrl Pts',(17.5705893998029,15.1538935621714,0.));
#250969=CARTESIAN_POINT('Ctrl Pts',(17.5705893998029,15.1538935621714,12.));
#250970=CARTESIAN_POINT('Ctrl Pts',(17.5611842686192,15.1408116444876,0.));
#250971=CARTESIAN_POINT('Ctrl Pts',(17.5611842686192,15.1408116444876,12.));
#250972=CARTESIAN_POINT('Ctrl Pts',(17.5518231989117,15.1278724853138,0.));
#250973=CARTESIAN_POINT('Ctrl Pts',(17.5518231989117,15.1278724853138,12.));
#250974=CARTESIAN_POINT('Ctrl Pts',(17.5425076102963,15.1150768967728,0.));
#250975=CARTESIAN_POINT('Ctrl Pts',(17.5425076102963,15.1150768967728,12.));
#250976=CARTESIAN_POINT('Ctrl Pts',(17.5332389504829,15.1024257045033,0.));
#250977=CARTESIAN_POINT('Ctrl Pts',(17.5332389504829,15.1024257045033,12.));
#250978=CARTESIAN_POINT('Ctrl Pts',(17.524018696179,15.0899197481082,0.));
#250979=CARTESIAN_POINT('Ctrl Pts',(17.524018696179,15.0899197481082,12.));
#250980=CARTESIAN_POINT('Ctrl Pts',(17.5148483539687,15.0775598815749,0.));
#250981=CARTESIAN_POINT('Ctrl Pts',(17.5148483539687,15.0775598815749,12.));
#250982=CARTESIAN_POINT('Ctrl Pts',(17.5057294613877,15.0653469738307,0.));
#250983=CARTESIAN_POINT('Ctrl Pts',(17.5057294613877,15.0653469738307,12.));
#250984=CARTESIAN_POINT('Ctrl Pts',(17.4966635880246,15.0532819093085,0.));
#250985=CARTESIAN_POINT('Ctrl Pts',(17.4966635880246,15.0532819093085,12.));
#250986=CARTESIAN_POINT('Ctrl Pts',(17.4876523366178,15.0413655884993,0.));
#250987=CARTESIAN_POINT('Ctrl Pts',(17.4876523366178,15.0413655884993,12.));
#250988=CARTESIAN_POINT('Ctrl Pts',(17.4786973441417,15.029598928488,0.));
#250989=CARTESIAN_POINT('Ctrl Pts',(17.4786973441417,15.029598928488,12.));
#250990=CARTESIAN_POINT('Ctrl Pts',(17.4698002829357,15.0179828635087,0.));
#250991=CARTESIAN_POINT('Ctrl Pts',(17.4698002829357,15.0179828635087,12.));
#250992=CARTESIAN_POINT('Ctrl Pts',(17.4609628621419,15.0065183456923,0.));
#250993=CARTESIAN_POINT('Ctrl Pts',(17.4609628621419,15.0065183456923,12.));
#250994=CARTESIAN_POINT('Ctrl Pts',(17.4521868291005,14.9952063457779,0.));
#250995=CARTESIAN_POINT('Ctrl Pts',(17.4521868291005,14.9952063457779,12.));
#250996=CARTESIAN_POINT('Ctrl Pts',(17.4434739707773,14.9840478538357,0.));
#250997=CARTESIAN_POINT('Ctrl Pts',(17.4434739707773,14.9840478538357,12.));
#250998=CARTESIAN_POINT('Ctrl Pts',(17.4348261151395,14.973043879945,0.));
#250999=CARTESIAN_POINT('Ctrl Pts',(17.4348261151395,14.973043879945,12.));
#251000=CARTESIAN_POINT('Ctrl Pts',(17.4262451327088,14.9621954549825,0.));
#251001=CARTESIAN_POINT('Ctrl Pts',(17.4262451327088,14.9621954549825,12.));
#251002=CARTESIAN_POINT('Ctrl Pts',(17.4177329382827,14.9515036315142,0.));
#251003=CARTESIAN_POINT('Ctrl Pts',(17.4177329382827,14.9515036315142,12.));
#251004=CARTESIAN_POINT('Ctrl Pts',(17.4092914926071,14.940969484645,0.));
#251005=CARTESIAN_POINT('Ctrl Pts',(17.4092914926071,14.940969484645,12.));
#251006=CARTESIAN_POINT('Ctrl Pts',(17.400922804075,14.9305941128758,0.));
#251007=CARTESIAN_POINT('Ctrl Pts',(17.400922804075,14.9305941128758,12.));
#251008=CARTESIAN_POINT('Ctrl Pts',(17.3926289303987,14.9203786389343,0.));
#251009=CARTESIAN_POINT('Ctrl Pts',(17.3926289303987,14.9203786389343,12.));
#251010=CARTESIAN_POINT('Ctrl Pts',(17.3844119809823,14.9103242110057,0.));
#251011=CARTESIAN_POINT('Ctrl Pts',(17.3844119809823,14.9103242110057,12.));
#251012=CARTESIAN_POINT('Ctrl Pts',(17.3762741193075,14.9004320039609,0.));
#251013=CARTESIAN_POINT('Ctrl Pts',(17.3762741193075,14.9004320039609,12.));
#251014=CARTESIAN_POINT('Ctrl Pts',(17.3682175653236,14.8907032205789,0.));
#251015=CARTESIAN_POINT('Ctrl Pts',(17.3682175653236,14.8907032205789,12.));
#251016=CARTESIAN_POINT('Ctrl Pts',(17.3602445978163,14.8811390927424,0.));
#251017=CARTESIAN_POINT('Ctrl Pts',(17.3602445978163,14.8811390927424,12.));
#251018=CARTESIAN_POINT('Ctrl Pts',(17.3523575568648,14.8717408826958,0.));
#251019=CARTESIAN_POINT('Ctrl Pts',(17.3523575568648,14.8717408826958,12.));
#251020=CARTESIAN_POINT('Ctrl Pts',(17.3445588463477,14.8625098843419,0.));
#251021=CARTESIAN_POINT('Ctrl Pts',(17.3445588463477,14.8625098843419,12.));
#251022=CARTESIAN_POINT('Ctrl Pts',(17.336850936485,14.8534474245433,0.));
#251023=CARTESIAN_POINT('Ctrl Pts',(17.336850936485,14.8534474245433,12.));
#251024=CARTESIAN_POINT('Ctrl Pts',(17.3292363662601,14.8445548643505,0.));
#251025=CARTESIAN_POINT('Ctrl Pts',(17.3292363662601,14.8445548643505,12.));
#251026=CARTESIAN_POINT('Ctrl Pts',(17.3217177462096,14.8358336004193,0.));
#251027=CARTESIAN_POINT('Ctrl Pts',(17.3217177462096,14.8358336004193,12.));
#251028=CARTESIAN_POINT('Ctrl Pts',(17.3142977632656,14.8272850675375,0.));
#251029=CARTESIAN_POINT('Ctrl Pts',(17.3142977632656,14.8272850675375,12.));
#251030=CARTESIAN_POINT('Ctrl Pts',(17.3069791853705,14.8189107410161,0.));
#251031=CARTESIAN_POINT('Ctrl Pts',(17.3069791853705,14.8189107410161,12.));
#251032=CARTESIAN_POINT('Ctrl Pts',(17.2997648661483,14.8107121391038,0.));
#251033=CARTESIAN_POINT('Ctrl Pts',(17.2997648661483,14.8107121391038,12.));
#251034=CARTESIAN_POINT('Ctrl Pts',(17.2926577496519,14.8026908254281,0.));
#251035=CARTESIAN_POINT('Ctrl Pts',(17.2926577496519,14.8026908254281,12.));
#251036=CARTESIAN_POINT('Ctrl Pts',(17.28566087332,14.7948484105253,0.));
#251037=CARTESIAN_POINT('Ctrl Pts',(17.28566087332,14.7948484105253,12.));
#251038=CARTESIAN_POINT('Ctrl Pts',(17.278777370485,14.787186553128,0.));
#251039=CARTESIAN_POINT('Ctrl Pts',(17.278777370485,14.787186553128,12.));
#251040=CARTESIAN_POINT('Ctrl Pts',(17.2720104735192,14.7797069617802,0.));
#251041=CARTESIAN_POINT('Ctrl Pts',(17.2720104735192,14.7797069617802,12.));
#251042=CARTESIAN_POINT('Ctrl Pts',(17.2653635155317,14.7724113956728,0.));
#251043=CARTESIAN_POINT('Ctrl Pts',(17.2653635155317,14.7724113956728,12.));
#251044=CARTESIAN_POINT('Ctrl Pts',(17.2588399401464,14.7653016697589,0.));
#251045=CARTESIAN_POINT('Ctrl Pts',(17.2588399401464,14.7653016697589,12.));
#251046=CARTESIAN_POINT('Ctrl Pts',(17.2524433146837,14.7583796616617,0.));
#251047=CARTESIAN_POINT('Ctrl Pts',(17.2524433146837,14.7583796616617,12.));
#251048=CARTESIAN_POINT('Ctrl Pts',(17.2461773413289,14.7516473175125,0.));
#251049=CARTESIAN_POINT('Ctrl Pts',(17.2461773413289,14.7516473175125,12.));
#251050=CARTESIAN_POINT('Ctrl Pts',(17.2400458713566,14.7451066593793,0.));
#251051=CARTESIAN_POINT('Ctrl Pts',(17.2400458713566,14.7451066593793,12.));
#251052=CARTESIAN_POINT('Ctrl Pts',(17.2340529062077,14.7387597858117,0.));
#251053=CARTESIAN_POINT('Ctrl Pts',(17.2340529062077,14.7387597858117,12.));
#251054=CARTESIAN_POINT('Ctrl Pts',(17.2282025904314,14.7326088681163,0.));
#251055=CARTESIAN_POINT('Ctrl Pts',(17.2282025904314,14.7326088681163,12.));
#251056=CARTESIAN_POINT('Ctrl Pts',(17.2224992099666,14.7266561494282,0.));
#251057=CARTESIAN_POINT('Ctrl Pts',(17.2224992099666,14.7266561494282,12.));
#251058=CARTESIAN_POINT('Ctrl Pts',(17.2169471814255,14.7209039390326,0.));
#251059=CARTESIAN_POINT('Ctrl Pts',(17.2169471814255,14.7209039390326,12.));
#251060=CARTESIAN_POINT('Ctrl Pts',(17.2115510835988,14.7153546289338,0.));
#251061=CARTESIAN_POINT('Ctrl Pts',(17.2115510835988,14.7153546289338,12.));
#251062=CARTESIAN_POINT('Ctrl Pts',(17.2063157097316,14.7100107213587,0.));
#251063=CARTESIAN_POINT('Ctrl Pts',(17.2063157097316,14.7100107213587,12.));
#251064=CARTESIAN_POINT('Ctrl Pts',(17.2012461084268,14.7048748502663,0.));
#251065=CARTESIAN_POINT('Ctrl Pts',(17.2012461084268,14.7048748502663,12.));
#251066=CARTESIAN_POINT('Ctrl Pts',(17.1963476411694,14.699949811582,0.));
#251067=CARTESIAN_POINT('Ctrl Pts',(17.1963476411694,14.699949811582,12.));
#251068=CARTESIAN_POINT('Ctrl Pts',(17.1916259308415,14.6952385361706,0.));
#251069=CARTESIAN_POINT('Ctrl Pts',(17.1916259308415,14.6952385361706,12.));
#251070=CARTESIAN_POINT('Ctrl Pts',(17.1870867909918,14.6907440526958,0.));
#251071=CARTESIAN_POINT('Ctrl Pts',(17.1870867909918,14.6907440526958,12.));
#251072=CARTESIAN_POINT('Ctrl Pts',(17.182736158472,14.6864694522319,0.));
#251073=CARTESIAN_POINT('Ctrl Pts',(17.182736158472,14.6864694522319,12.));
#251074=CARTESIAN_POINT('Ctrl Pts',(17.1785800350827,14.6824178576167,0.));
#251075=CARTESIAN_POINT('Ctrl Pts',(17.1785800350827,14.6824178576167,12.));
#251076=CARTESIAN_POINT('Ctrl Pts',(17.1746247499057,14.6785925615676,0.));
#251077=CARTESIAN_POINT('Ctrl Pts',(17.1746247499057,14.6785925615676,12.));
#251078=CARTESIAN_POINT('Ctrl Pts',(17.1708771619129,14.6749971333867,0.));
#251079=CARTESIAN_POINT('Ctrl Pts',(17.1708771619129,14.6749971333867,12.));
#251080=CARTESIAN_POINT('Ctrl Pts',(17.1673449723019,14.6716355833321,0.));
#251081=CARTESIAN_POINT('Ctrl Pts',(17.1673449723019,14.6716355833321,12.));
#251082=CARTESIAN_POINT('Ctrl Pts',(17.1640366762304,14.6685123374424,0.));
#251083=CARTESIAN_POINT('Ctrl Pts',(17.1640366762304,14.6685123374424,12.));
#251084=CARTESIAN_POINT('Ctrl Pts',(17.1609609517369,14.6656319165057,0.));
#251085=CARTESIAN_POINT('Ctrl Pts',(17.1609609517369,14.6656319165057,12.));
#251086=CARTESIAN_POINT('Ctrl Pts',(17.1581262646789,14.662998728599,0.));
#251087=CARTESIAN_POINT('Ctrl Pts',(17.1581262646789,14.662998728599,12.));
#251088=CARTESIAN_POINT('Ctrl Pts',(17.1555401986403,14.660616716964,0.));
#251089=CARTESIAN_POINT('Ctrl Pts',(17.1555401986403,14.660616716964,12.));
#251090=CARTESIAN_POINT('Ctrl Pts',(17.1532107762719,14.6584900555301,0.));
#251091=CARTESIAN_POINT('Ctrl Pts',(17.1532107762719,14.6584900555301,12.));
#251092=CARTESIAN_POINT('Ctrl Pts',(17.1511476869495,14.6566237952435,0.));
#251093=CARTESIAN_POINT('Ctrl Pts',(17.1511476869495,14.6566237952435,12.));
#251094=CARTESIAN_POINT('Ctrl Pts',(17.1493641837556,14.6550248622813,0.));
#251095=CARTESIAN_POINT('Ctrl Pts',(17.1493641837556,14.6550248622813,12.));
#251096=CARTESIAN_POINT('Ctrl Pts',(17.1478763944909,14.6537016966188,0.));
#251097=CARTESIAN_POINT('Ctrl Pts',(17.1478763944909,14.6537016966188,12.));
#251098=CARTESIAN_POINT('Ctrl Pts',(17.1466998098673,14.6526624064978,0.));
#251099=CARTESIAN_POINT('Ctrl Pts',(17.1466998098673,14.6526624064978,12.));
#251100=CARTESIAN_POINT('Ctrl Pts',(17.1458462295273,14.65191316345,0.));
#251101=CARTESIAN_POINT('Ctrl Pts',(17.1458462295273,14.65191316345,12.));
#251102=CARTESIAN_POINT('Ctrl Pts',(17.1454262858045,14.6515481598057,0.));
#251103=CARTESIAN_POINT('Ctrl Pts',(17.1454262858045,14.6515481598057,12.));
#251104=CARTESIAN_POINT('Ctrl Pts',(17.1452600887039,14.6514066997188,0.));
#251105=CARTESIAN_POINT('Ctrl Pts',(17.1452600887039,14.6514066997188,12.));
#251106=CARTESIAN_POINT('Ctrl Pts',(17.1452153999142,14.651371185284,0.));
#251107=CARTESIAN_POINT('Ctrl Pts',(17.1452153999142,14.651371185284,12.));
#251108=CARTESIAN_POINT('Ctrl Pts',(17.1452095830633,14.6513681262571,0.));
#251109=CARTESIAN_POINT('Ctrl Pts',(17.1452095830633,14.6513681262571,12.));
#251110=CARTESIAN_POINT('',(18.8464468996588,17.9112098770111,0.));
#251111=CARTESIAN_POINT('Ctrl Pts',(18.8464468996588,17.9112098770111,0.));
#251112=CARTESIAN_POINT('Ctrl Pts',(18.8448126709691,17.9057348246595,0.));
#251113=CARTESIAN_POINT('Ctrl Pts',(18.8415402351786,17.8947931177807,0.));
#251114=CARTESIAN_POINT('Ctrl Pts',(18.8366196462581,17.8784057509356,0.));
#251115=CARTESIAN_POINT('Ctrl Pts',(18.8300349895974,17.8566063174771,0.));
#251116=CARTESIAN_POINT('Ctrl Pts',(18.8217643886157,17.8294410311006,0.));
#251117=CARTESIAN_POINT('Ctrl Pts',(18.8134540340417,17.8023598011057,0.));
#251118=CARTESIAN_POINT('Ctrl Pts',(18.8051039860448,17.7753627137853,0.));
#251119=CARTESIAN_POINT('Ctrl Pts',(18.7967143519419,17.7484498996905,0.));
#251120=CARTESIAN_POINT('Ctrl Pts',(18.7882852976049,17.7216215409035,0.));
#251121=CARTESIAN_POINT('Ctrl Pts',(18.7798170641374,17.6948778823014,0.));
#251122=CARTESIAN_POINT('Ctrl Pts',(18.7713099642754,17.6682192274236,0.));
#251123=CARTESIAN_POINT('Ctrl Pts',(18.762764361321,17.6416459210681,0.));
#251124=CARTESIAN_POINT('Ctrl Pts',(18.7541806530984,17.6151583357012,0.));
#251125=CARTESIAN_POINT('Ctrl Pts',(18.7455592536687,17.5887568561371,0.));
#251126=CARTESIAN_POINT('Ctrl Pts',(18.7369005764553,17.5624418653245,0.));
#251127=CARTESIAN_POINT('Ctrl Pts',(18.7282050157138,17.5362137287593,0.));
#251128=CARTESIAN_POINT('Ctrl Pts',(18.7194729318098,17.5100727820876,0.));
#251129=CARTESIAN_POINT('Ctrl Pts',(18.7107046613912,17.4840193397162,0.));
#251130=CARTESIAN_POINT('Ctrl Pts',(18.70190052503,17.4580537012753,0.));
#251131=CARTESIAN_POINT('Ctrl Pts',(18.6930608357409,17.4321761588142,0.));
#251132=CARTESIAN_POINT('Ctrl Pts',(18.6841859073471,17.4063870038562,0.));
#251133=CARTESIAN_POINT('Ctrl Pts',(18.6752760624052,17.3806865340747,0.));
#251134=CARTESIAN_POINT('Ctrl Pts',(18.6663316416582,17.3550750612443,0.));
#251135=CARTESIAN_POINT('Ctrl Pts',(18.6573530024033,17.3295529098618,0.));
#251136=CARTESIAN_POINT('Ctrl Pts',(18.6483405141865,17.3041204135074,0.));
#251137=CARTESIAN_POINT('Ctrl Pts',(18.6392945554748,17.2787779120213,0.));
#251138=CARTESIAN_POINT('Ctrl Pts',(18.6302155097943,17.2535257482187,0.));
#251139=CARTESIAN_POINT('Ctrl Pts',(18.6211037624038,17.2283642650518,0.));
#251140=CARTESIAN_POINT('Ctrl Pts',(18.6119596959949,17.2032938019284,0.));
#251141=CARTESIAN_POINT('Ctrl Pts',(18.6027836898817,17.1783146940127,0.));
#251142=CARTESIAN_POINT('Ctrl Pts',(18.5935761222825,17.1534272741643,0.));
#251143=CARTESIAN_POINT('Ctrl Pts',(18.5843373717247,17.1286318741183,0.));
#251144=CARTESIAN_POINT('Ctrl Pts',(18.5750678188542,17.1039288260001,0.));
#251145=CARTESIAN_POINT('Ctrl Pts',(18.5657678479789,17.0793184636079,0.));
#251146=CARTESIAN_POINT('Ctrl Pts',(18.556437848963,17.0548011239751,0.));
#251147=CARTESIAN_POINT('Ctrl Pts',(18.547078218209,17.0303771481738,0.));
#251148=CARTESIAN_POINT('Ctrl Pts',(18.5376893576961,17.0060468805097,0.));
#251149=CARTESIAN_POINT('Ctrl Pts',(18.5282716744197,16.981810668038,0.));
#251150=CARTESIAN_POINT('Ctrl Pts',(18.5188255796659,16.9576688599339,0.));
#251151=CARTESIAN_POINT('Ctrl Pts',(18.5093514883835,16.9336218069353,0.));
#251152=CARTESIAN_POINT('Ctrl Pts',(18.499849818462,16.9096698606943,0.));
#251153=CARTESIAN_POINT('Ctrl Pts',(18.4903209902227,16.8858133733088,0.));
#251154=CARTESIAN_POINT('Ctrl Pts',(18.4807654268771,16.8620526977171,0.));
#251155=CARTESIAN_POINT('Ctrl Pts',(18.4711835548623,16.8383881879709,0.));
#251156=CARTESIAN_POINT('Ctrl Pts',(18.4615758042305,16.8148201995472,0.));
#251157=CARTESIAN_POINT('Ctrl Pts',(18.4519426090123,16.791349089629,0.));
#251158=CARTESIAN_POINT('Ctrl Pts',(18.44228440761,16.7679752173992,0.));
#251159=CARTESIAN_POINT('Ctrl Pts',(18.4326016431392,16.7446989442882,0.));
#251160=CARTESIAN_POINT('Ctrl Pts',(18.4228947633187,16.7215206338818,0.));
#251161=CARTESIAN_POINT('Ctrl Pts',(18.413164220399,16.6984406518491,0.));
#251162=CARTESIAN_POINT('Ctrl Pts',(18.403410471079,16.6754593658513,0.));
#251163=CARTESIAN_POINT('Ctrl Pts',(18.3936339764332,16.6525771454513,0.));
#251164=CARTESIAN_POINT('Ctrl Pts',(18.3838352018327,16.6297943620056,0.));
#251165=CARTESIAN_POINT('Ctrl Pts',(18.3740146168879,16.607111388571,0.));
#251166=CARTESIAN_POINT('Ctrl Pts',(18.3641726955889,16.5845286000217,0.));
#251167=CARTESIAN_POINT('Ctrl Pts',(18.354309916433,16.5620463731413,0.));
#251168=CARTESIAN_POINT('Ctrl Pts',(18.34442676256,16.5396650867139,0.));
#251169=CARTESIAN_POINT('Ctrl Pts',(18.3345237218864,16.5173851216045,0.));
#251170=CARTESIAN_POINT('Ctrl Pts',(18.3246012872469,16.4952068608345,0.));
#251171=CARTESIAN_POINT('Ctrl Pts',(18.3146599565231,16.4731306896441,0.));
#251172=CARTESIAN_POINT('Ctrl Pts',(18.304700232686,16.4511569955233,0.));
#251173=CARTESIAN_POINT('Ctrl Pts',(18.294722623851,16.4292861682379,0.));
#251174=CARTESIAN_POINT('Ctrl Pts',(18.2847276433309,16.4075185998455,0.));
#251175=CARTESIAN_POINT('Ctrl Pts',(18.2747158096934,16.385854684708,0.));
#251176=CARTESIAN_POINT('Ctrl Pts',(18.2646876468169,16.3642948194868,0.));
#251177=CARTESIAN_POINT('Ctrl Pts',(18.2546436839608,16.3428394031589,0.));
#251178=CARTESIAN_POINT('Ctrl Pts',(18.2445844558742,16.3214888370987,0.));
#251179=CARTESIAN_POINT('Ctrl Pts',(18.2345105028982,16.3002435251378,0.));
#251180=CARTESIAN_POINT('Ctrl Pts',(18.2244223710745,16.2791038736223,0.));
#251181=CARTESIAN_POINT('Ctrl Pts',(18.2143206122529,16.2580702914615,0.));
#251182=CARTESIAN_POINT('Ctrl Pts',(18.2042057842035,16.2371431901638,0.));
#251183=CARTESIAN_POINT('Ctrl Pts',(18.1940784507229,16.2163229838875,0.));
#251184=CARTESIAN_POINT('Ctrl Pts',(18.1839391817331,16.1956100895073,0.));
#251185=CARTESIAN_POINT('Ctrl Pts',(18.1737885533849,16.1750049266671,0.));
#251186=CARTESIAN_POINT('Ctrl Pts',(18.1636271481615,16.154507917826,0.));
#251187=CARTESIAN_POINT('Ctrl Pts',(18.1534555549852,16.1341194882988,0.));
#251188=CARTESIAN_POINT('Ctrl Pts',(18.1432743693235,16.1138400662794,0.));
#251189=CARTESIAN_POINT('Ctrl Pts',(18.1330841933105,16.0936700829112,0.));
#251190=CARTESIAN_POINT('Ctrl Pts',(18.1228856358751,16.0736099723668,0.));
#251191=CARTESIAN_POINT('Ctrl Pts',(18.112679312869,16.0536601719126,0.));
#251192=CARTESIAN_POINT('Ctrl Pts',(18.1024658471966,16.0338211219693,0.));
#251193=CARTESIAN_POINT('Ctrl Pts',(18.0922458689462,16.014093266161,0.));
#251194=CARTESIAN_POINT('Ctrl Pts',(18.0820200155236,15.9944770513613,0.));
#251195=CARTESIAN_POINT('Ctrl Pts',(18.0717889317958,15.9749729277846,0.));
#251196=CARTESIAN_POINT('Ctrl Pts',(18.061553270236,15.9555813490644,0.));
#251197=CARTESIAN_POINT('Ctrl Pts',(18.0513136910691,15.9363027723244,0.));
#251198=CARTESIAN_POINT('Ctrl Pts',(18.0410708624208,15.9171376582436,0.));
#251199=CARTESIAN_POINT('Ctrl Pts',(18.0308254604636,15.8980864711042,0.));
#251200=CARTESIAN_POINT('Ctrl Pts',(18.0205781695769,15.8791496788683,0.));
#251201=CARTESIAN_POINT('Ctrl Pts',(18.0103296825205,15.8603277532831,0.));
#251202=CARTESIAN_POINT('Ctrl Pts',(18.0000807006052,15.8416211699679,0.));
#251203=CARTESIAN_POINT('Ctrl Pts',(17.9898319338664,15.8230304084962,0.));
#251204=CARTESIAN_POINT('Ctrl Pts',(17.9795841012386,15.8045559524677,0.));
#251205=CARTESIAN_POINT('Ctrl Pts',(17.9693379307303,15.7861982895724,0.));
#251206=CARTESIAN_POINT('Ctrl Pts',(17.9590941596242,15.7679579117077,0.));
#251207=CARTESIAN_POINT('Ctrl Pts',(17.9488535346781,15.749835315086,0.));
#251208=CARTESIAN_POINT('Ctrl Pts',(17.9386168123262,15.7318310003335,0.));
#251209=CARTESIAN_POINT('Ctrl Pts',(17.9283847588836,15.7139454725839,0.));
#251210=CARTESIAN_POINT('Ctrl Pts',(17.9181581507455,15.6961792415522,0.));
#251211=CARTESIAN_POINT('Ctrl Pts',(17.9079377746111,15.6785328216461,0.));
#251212=CARTESIAN_POINT('Ctrl Pts',(17.897724427724,15.661006732103,0.));
#251213=CARTESIAN_POINT('Ctrl Pts',(17.8875189181091,15.6436014971085,0.));
#251214=CARTESIAN_POINT('Ctrl Pts',(17.8773220648125,15.6263176459108,0.));
#251215=CARTESIAN_POINT('Ctrl Pts',(17.8671346981394,15.609155712921,0.));
#251216=CARTESIAN_POINT('Ctrl Pts',(17.8569576599006,15.5921162378192,0.));
#251217=CARTESIAN_POINT('Ctrl Pts',(17.8467918036987,15.5751997657163,0.));
#251218=CARTESIAN_POINT('Ctrl Pts',(17.8366379952085,15.5584068472982,0.));
#251219=CARTESIAN_POINT('Ctrl Pts',(17.8264971124606,15.541738038964,0.));
#251220=CARTESIAN_POINT('Ctrl Pts',(17.8163700461256,15.5251939029552,0.));
#251221=CARTESIAN_POINT('Ctrl Pts',(17.8062576997952,15.5087750074718,0.));
#251222=CARTESIAN_POINT('Ctrl Pts',(17.7961609903148,15.4924819268517,0.));
#251223=CARTESIAN_POINT('Ctrl Pts',(17.7860808481219,15.4763152417497,0.));
#251224=CARTESIAN_POINT('Ctrl Pts',(17.7760182175815,15.4602755393018,0.));
#251225=CARTESIAN_POINT('Ctrl Pts',(17.7659740573265,15.4443634132869,0.));
#251226=CARTESIAN_POINT('Ctrl Pts',(17.7559493405881,15.4285794642668,0.));
#251227=CARTESIAN_POINT('Ctrl Pts',(17.7459450555812,15.4129242997837,0.));
#251228=CARTESIAN_POINT('Ctrl Pts',(17.7359622059149,15.3973985345802,0.));
#251229=CARTESIAN_POINT('Ctrl Pts',(17.7260018109924,15.3820027907967,0.));
#251230=CARTESIAN_POINT('Ctrl Pts',(17.7160649064206,15.3667376981699,0.));
#251231=CARTESIAN_POINT('Ctrl Pts',(17.7061525444042,15.351603894206,0.));
#251232=CARTESIAN_POINT('Ctrl Pts',(17.6962657941983,15.3366020244066,0.));
#251233=CARTESIAN_POINT('Ctrl Pts',(17.6864057426052,15.3217327425338,0.));
#251234=CARTESIAN_POINT('Ctrl Pts',(17.676573494456,15.3069967108501,0.));
#251235=CARTESIAN_POINT('Ctrl Pts',(17.6667701731041,15.2923946003598,0.));
#251236=CARTESIAN_POINT('Ctrl Pts',(17.6569969209,15.2779270910239,0.));
#251237=CARTESIAN_POINT('Ctrl Pts',(17.6472548997328,15.2635948720292,0.));
#251238=CARTESIAN_POINT('Ctrl Pts',(17.6375452916369,15.2493986421092,0.));
#251239=CARTESIAN_POINT('Ctrl Pts',(17.6278692993764,15.2353391098367,0.));
#251240=CARTESIAN_POINT('Ctrl Pts',(17.6182281470468,15.22141699392,0.));
#251241=CARTESIAN_POINT('Ctrl Pts',(17.60862308065,15.2076330234686,0.));
#251242=CARTESIAN_POINT('Ctrl Pts',(17.5990553687599,15.1939879383268,0.));
#251243=CARTESIAN_POINT('Ctrl Pts',(17.5895263032595,15.1804824894605,0.));
#251244=CARTESIAN_POINT('Ctrl Pts',(17.580037200054,15.1671174393137,0.));
#251245=CARTESIAN_POINT('Ctrl Pts',(17.5705893998029,15.1538935621714,0.));
#251246=CARTESIAN_POINT('Ctrl Pts',(17.5611842686192,15.1408116444876,0.));
#251247=CARTESIAN_POINT('Ctrl Pts',(17.5518231989117,15.1278724853138,0.));
#251248=CARTESIAN_POINT('Ctrl Pts',(17.5425076102963,15.1150768967728,0.));
#251249=CARTESIAN_POINT('Ctrl Pts',(17.5332389504829,15.1024257045033,0.));
#251250=CARTESIAN_POINT('Ctrl Pts',(17.524018696179,15.0899197481082,0.));
#251251=CARTESIAN_POINT('Ctrl Pts',(17.5148483539687,15.0775598815749,0.));
#251252=CARTESIAN_POINT('Ctrl Pts',(17.5057294613877,15.0653469738307,0.));
#251253=CARTESIAN_POINT('Ctrl Pts',(17.4966635880246,15.0532819093085,0.));
#251254=CARTESIAN_POINT('Ctrl Pts',(17.4876523366178,15.0413655884993,0.));
#251255=CARTESIAN_POINT('Ctrl Pts',(17.4786973441417,15.029598928488,0.));
#251256=CARTESIAN_POINT('Ctrl Pts',(17.4698002829357,15.0179828635087,0.));
#251257=CARTESIAN_POINT('Ctrl Pts',(17.4609628621419,15.0065183456923,0.));
#251258=CARTESIAN_POINT('Ctrl Pts',(17.4521868291005,14.9952063457779,0.));
#251259=CARTESIAN_POINT('Ctrl Pts',(17.4434739707773,14.9840478538357,0.));
#251260=CARTESIAN_POINT('Ctrl Pts',(17.4348261151395,14.973043879945,0.));
#251261=CARTESIAN_POINT('Ctrl Pts',(17.4262451327088,14.9621954549825,0.));
#251262=CARTESIAN_POINT('Ctrl Pts',(17.4177329382827,14.9515036315142,0.));
#251263=CARTESIAN_POINT('Ctrl Pts',(17.4092914926071,14.940969484645,0.));
#251264=CARTESIAN_POINT('Ctrl Pts',(17.400922804075,14.9305941128758,0.));
#251265=CARTESIAN_POINT('Ctrl Pts',(17.3926289303987,14.9203786389343,0.));
#251266=CARTESIAN_POINT('Ctrl Pts',(17.3844119809823,14.9103242110057,0.));
#251267=CARTESIAN_POINT('Ctrl Pts',(17.3762741193075,14.9004320039609,0.));
#251268=CARTESIAN_POINT('Ctrl Pts',(17.3682175653236,14.8907032205789,0.));
#251269=CARTESIAN_POINT('Ctrl Pts',(17.3602445978163,14.8811390927424,0.));
#251270=CARTESIAN_POINT('Ctrl Pts',(17.3523575568648,14.8717408826958,0.));
#251271=CARTESIAN_POINT('Ctrl Pts',(17.3445588463477,14.8625098843419,0.));
#251272=CARTESIAN_POINT('Ctrl Pts',(17.336850936485,14.8534474245433,0.));
#251273=CARTESIAN_POINT('Ctrl Pts',(17.3292363662601,14.8445548643505,0.));
#251274=CARTESIAN_POINT('Ctrl Pts',(17.3217177462096,14.8358336004193,0.));
#251275=CARTESIAN_POINT('Ctrl Pts',(17.3142977632656,14.8272850675375,0.));
#251276=CARTESIAN_POINT('Ctrl Pts',(17.3069791853705,14.8189107410161,0.));
#251277=CARTESIAN_POINT('Ctrl Pts',(17.2997648661483,14.8107121391038,0.));
#251278=CARTESIAN_POINT('Ctrl Pts',(17.2926577496519,14.8026908254281,0.));
#251279=CARTESIAN_POINT('Ctrl Pts',(17.28566087332,14.7948484105253,0.));
#251280=CARTESIAN_POINT('Ctrl Pts',(17.278777370485,14.787186553128,0.));
#251281=CARTESIAN_POINT('Ctrl Pts',(17.2720104735192,14.7797069617802,0.));
#251282=CARTESIAN_POINT('Ctrl Pts',(17.2653635155317,14.7724113956728,0.));
#251283=CARTESIAN_POINT('Ctrl Pts',(17.2588399401464,14.7653016697589,0.));
#251284=CARTESIAN_POINT('Ctrl Pts',(17.2524433146837,14.7583796616617,0.));
#251285=CARTESIAN_POINT('Ctrl Pts',(17.2461773413289,14.7516473175125,0.));
#251286=CARTESIAN_POINT('Ctrl Pts',(17.2400458713566,14.7451066593793,0.));
#251287=CARTESIAN_POINT('Ctrl Pts',(17.2340529062077,14.7387597858117,0.));
#251288=CARTESIAN_POINT('Ctrl Pts',(17.2282025904314,14.7326088681163,0.));
#251289=CARTESIAN_POINT('Ctrl Pts',(17.2224992099666,14.7266561494282,0.));
#251290=CARTESIAN_POINT('Ctrl Pts',(17.2169471814255,14.7209039390326,0.));
#251291=CARTESIAN_POINT('Ctrl Pts',(17.2115510835988,14.7153546289338,0.));
#251292=CARTESIAN_POINT('Ctrl Pts',(17.2063157097316,14.7100107213587,0.));
#251293=CARTESIAN_POINT('Ctrl Pts',(17.2012461084268,14.7048748502663,0.));
#251294=CARTESIAN_POINT('Ctrl Pts',(17.1963476411694,14.699949811582,0.));
#251295=CARTESIAN_POINT('Ctrl Pts',(17.1916259308415,14.6952385361706,0.));
#251296=CARTESIAN_POINT('Ctrl Pts',(17.1870867909918,14.6907440526958,0.));
#251297=CARTESIAN_POINT('Ctrl Pts',(17.182736158472,14.6864694522319,0.));
#251298=CARTESIAN_POINT('Ctrl Pts',(17.1785800350827,14.6824178576167,0.));
#251299=CARTESIAN_POINT('Ctrl Pts',(17.1746247499057,14.6785925615676,0.));
#251300=CARTESIAN_POINT('Ctrl Pts',(17.1708771619129,14.6749971333867,0.));
#251301=CARTESIAN_POINT('Ctrl Pts',(17.1673449723019,14.6716355833321,0.));
#251302=CARTESIAN_POINT('Ctrl Pts',(17.1640366762304,14.6685123374424,0.));
#251303=CARTESIAN_POINT('Ctrl Pts',(17.1609609517369,14.6656319165057,0.));
#251304=CARTESIAN_POINT('Ctrl Pts',(17.1581262646789,14.662998728599,0.));
#251305=CARTESIAN_POINT('Ctrl Pts',(17.1555401986403,14.660616716964,0.));
#251306=CARTESIAN_POINT('Ctrl Pts',(17.1532107762719,14.6584900555301,0.));
#251307=CARTESIAN_POINT('Ctrl Pts',(17.1511476869495,14.6566237952435,0.));
#251308=CARTESIAN_POINT('Ctrl Pts',(17.1493641837556,14.6550248622813,0.));
#251309=CARTESIAN_POINT('Ctrl Pts',(17.1478763944909,14.6537016966188,0.));
#251310=CARTESIAN_POINT('Ctrl Pts',(17.1466998098673,14.6526624064978,0.));
#251311=CARTESIAN_POINT('Ctrl Pts',(17.1458462295273,14.65191316345,0.));
#251312=CARTESIAN_POINT('Ctrl Pts',(17.1454262858045,14.6515481598057,0.));
#251313=CARTESIAN_POINT('Ctrl Pts',(17.1452600887039,14.6514066997188,0.));
#251314=CARTESIAN_POINT('Ctrl Pts',(17.1452153999142,14.651371185284,0.));
#251315=CARTESIAN_POINT('Ctrl Pts',(17.1452095830633,14.6513681262571,0.));
#251316=CARTESIAN_POINT('',(18.8464468996588,17.9112098770111,12.));
#251317=CARTESIAN_POINT('',(18.8464468996588,17.9112098770111,0.));
#251318=CARTESIAN_POINT('Ctrl Pts',(17.1452095830633,14.6513681262571,12.));
#251319=CARTESIAN_POINT('Ctrl Pts',(17.1452153999142,14.651371185284,12.));
#251320=CARTESIAN_POINT('Ctrl Pts',(17.1452600887039,14.6514066997188,12.));
#251321=CARTESIAN_POINT('Ctrl Pts',(17.1454262858045,14.6515481598057,12.));
#251322=CARTESIAN_POINT('Ctrl Pts',(17.1458462295273,14.65191316345,12.));
#251323=CARTESIAN_POINT('Ctrl Pts',(17.1466998098673,14.6526624064978,12.));
#251324=CARTESIAN_POINT('Ctrl Pts',(17.1478763944909,14.6537016966188,12.));
#251325=CARTESIAN_POINT('Ctrl Pts',(17.1493641837556,14.6550248622813,12.));
#251326=CARTESIAN_POINT('Ctrl Pts',(17.1511476869495,14.6566237952435,12.));
#251327=CARTESIAN_POINT('Ctrl Pts',(17.1532107762719,14.6584900555301,12.));
#251328=CARTESIAN_POINT('Ctrl Pts',(17.1555401986403,14.660616716964,12.));
#251329=CARTESIAN_POINT('Ctrl Pts',(17.1581262646789,14.662998728599,12.));
#251330=CARTESIAN_POINT('Ctrl Pts',(17.1609609517369,14.6656319165057,12.));
#251331=CARTESIAN_POINT('Ctrl Pts',(17.1640366762304,14.6685123374424,12.));
#251332=CARTESIAN_POINT('Ctrl Pts',(17.1673449723019,14.6716355833321,12.));
#251333=CARTESIAN_POINT('Ctrl Pts',(17.1708771619129,14.6749971333867,12.));
#251334=CARTESIAN_POINT('Ctrl Pts',(17.1746247499057,14.6785925615676,12.));
#251335=CARTESIAN_POINT('Ctrl Pts',(17.1785800350827,14.6824178576167,12.));
#251336=CARTESIAN_POINT('Ctrl Pts',(17.182736158472,14.6864694522319,12.));
#251337=CARTESIAN_POINT('Ctrl Pts',(17.1870867909918,14.6907440526958,12.));
#251338=CARTESIAN_POINT('Ctrl Pts',(17.1916259308415,14.6952385361706,12.));
#251339=CARTESIAN_POINT('Ctrl Pts',(17.1963476411694,14.699949811582,12.));
#251340=CARTESIAN_POINT('Ctrl Pts',(17.2012461084268,14.7048748502663,12.));
#251341=CARTESIAN_POINT('Ctrl Pts',(17.2063157097316,14.7100107213587,12.));
#251342=CARTESIAN_POINT('Ctrl Pts',(17.2115510835988,14.7153546289338,12.));
#251343=CARTESIAN_POINT('Ctrl Pts',(17.2169471814255,14.7209039390326,12.));
#251344=CARTESIAN_POINT('Ctrl Pts',(17.2224992099666,14.7266561494282,12.));
#251345=CARTESIAN_POINT('Ctrl Pts',(17.2282025904314,14.7326088681163,12.));
#251346=CARTESIAN_POINT('Ctrl Pts',(17.2340529062077,14.7387597858117,12.));
#251347=CARTESIAN_POINT('Ctrl Pts',(17.2400458713566,14.7451066593793,12.));
#251348=CARTESIAN_POINT('Ctrl Pts',(17.2461773413289,14.7516473175125,12.));
#251349=CARTESIAN_POINT('Ctrl Pts',(17.2524433146837,14.7583796616617,12.));
#251350=CARTESIAN_POINT('Ctrl Pts',(17.2588399401464,14.7653016697589,12.));
#251351=CARTESIAN_POINT('Ctrl Pts',(17.2653635155317,14.7724113956728,12.));
#251352=CARTESIAN_POINT('Ctrl Pts',(17.2720104735192,14.7797069617802,12.));
#251353=CARTESIAN_POINT('Ctrl Pts',(17.278777370485,14.787186553128,12.));
#251354=CARTESIAN_POINT('Ctrl Pts',(17.28566087332,14.7948484105253,12.));
#251355=CARTESIAN_POINT('Ctrl Pts',(17.2926577496519,14.8026908254281,12.));
#251356=CARTESIAN_POINT('Ctrl Pts',(17.2997648661483,14.8107121391038,12.));
#251357=CARTESIAN_POINT('Ctrl Pts',(17.3069791853705,14.8189107410161,12.));
#251358=CARTESIAN_POINT('Ctrl Pts',(17.3142977632656,14.8272850675375,12.));
#251359=CARTESIAN_POINT('Ctrl Pts',(17.3217177462096,14.8358336004193,12.));
#251360=CARTESIAN_POINT('Ctrl Pts',(17.3292363662601,14.8445548643505,12.));
#251361=CARTESIAN_POINT('Ctrl Pts',(17.336850936485,14.8534474245433,12.));
#251362=CARTESIAN_POINT('Ctrl Pts',(17.3445588463477,14.8625098843419,12.));
#251363=CARTESIAN_POINT('Ctrl Pts',(17.3523575568648,14.8717408826958,12.));
#251364=CARTESIAN_POINT('Ctrl Pts',(17.3602445978163,14.8811390927424,12.));
#251365=CARTESIAN_POINT('Ctrl Pts',(17.3682175653236,14.8907032205789,12.));
#251366=CARTESIAN_POINT('Ctrl Pts',(17.3762741193075,14.9004320039609,12.));
#251367=CARTESIAN_POINT('Ctrl Pts',(17.3844119809823,14.9103242110057,12.));
#251368=CARTESIAN_POINT('Ctrl Pts',(17.3926289303987,14.9203786389343,12.));
#251369=CARTESIAN_POINT('Ctrl Pts',(17.400922804075,14.9305941128758,12.));
#251370=CARTESIAN_POINT('Ctrl Pts',(17.4092914926071,14.940969484645,12.));
#251371=CARTESIAN_POINT('Ctrl Pts',(17.4177329382827,14.9515036315142,12.));
#251372=CARTESIAN_POINT('Ctrl Pts',(17.4262451327088,14.9621954549825,12.));
#251373=CARTESIAN_POINT('Ctrl Pts',(17.4348261151395,14.973043879945,12.));
#251374=CARTESIAN_POINT('Ctrl Pts',(17.4434739707773,14.9840478538357,12.));
#251375=CARTESIAN_POINT('Ctrl Pts',(17.4521868291005,14.9952063457779,12.));
#251376=CARTESIAN_POINT('Ctrl Pts',(17.4609628621419,15.0065183456923,12.));
#251377=CARTESIAN_POINT('Ctrl Pts',(17.4698002829357,15.0179828635087,12.));
#251378=CARTESIAN_POINT('Ctrl Pts',(17.4786973441417,15.029598928488,12.));
#251379=CARTESIAN_POINT('Ctrl Pts',(17.4876523366178,15.0413655884993,12.));
#251380=CARTESIAN_POINT('Ctrl Pts',(17.4966635880246,15.0532819093085,12.));
#251381=CARTESIAN_POINT('Ctrl Pts',(17.5057294613877,15.0653469738307,12.));
#251382=CARTESIAN_POINT('Ctrl Pts',(17.5148483539687,15.0775598815749,12.));
#251383=CARTESIAN_POINT('Ctrl Pts',(17.524018696179,15.0899197481082,12.));
#251384=CARTESIAN_POINT('Ctrl Pts',(17.5332389504829,15.1024257045033,12.));
#251385=CARTESIAN_POINT('Ctrl Pts',(17.5425076102963,15.1150768967728,12.));
#251386=CARTESIAN_POINT('Ctrl Pts',(17.5518231989117,15.1278724853138,12.));
#251387=CARTESIAN_POINT('Ctrl Pts',(17.5611842686192,15.1408116444876,12.));
#251388=CARTESIAN_POINT('Ctrl Pts',(17.5705893998029,15.1538935621714,12.));
#251389=CARTESIAN_POINT('Ctrl Pts',(17.580037200054,15.1671174393137,12.));
#251390=CARTESIAN_POINT('Ctrl Pts',(17.5895263032595,15.1804824894605,12.));
#251391=CARTESIAN_POINT('Ctrl Pts',(17.5990553687599,15.1939879383268,12.));
#251392=CARTESIAN_POINT('Ctrl Pts',(17.60862308065,15.2076330234686,12.));
#251393=CARTESIAN_POINT('Ctrl Pts',(17.6182281470468,15.22141699392,12.));
#251394=CARTESIAN_POINT('Ctrl Pts',(17.6278692993764,15.2353391098367,12.));
#251395=CARTESIAN_POINT('Ctrl Pts',(17.6375452916369,15.2493986421092,12.));
#251396=CARTESIAN_POINT('Ctrl Pts',(17.6472548997328,15.2635948720292,12.));
#251397=CARTESIAN_POINT('Ctrl Pts',(17.6569969209,15.2779270910239,12.));
#251398=CARTESIAN_POINT('Ctrl Pts',(17.6667701731041,15.2923946003598,12.));
#251399=CARTESIAN_POINT('Ctrl Pts',(17.676573494456,15.3069967108501,12.));
#251400=CARTESIAN_POINT('Ctrl Pts',(17.6864057426052,15.3217327425338,12.));
#251401=CARTESIAN_POINT('Ctrl Pts',(17.6962657941983,15.3366020244066,12.));
#251402=CARTESIAN_POINT('Ctrl Pts',(17.7061525444042,15.351603894206,12.));
#251403=CARTESIAN_POINT('Ctrl Pts',(17.7160649064206,15.3667376981699,12.));
#251404=CARTESIAN_POINT('Ctrl Pts',(17.7260018109924,15.3820027907967,12.));
#251405=CARTESIAN_POINT('Ctrl Pts',(17.7359622059149,15.3973985345802,12.));
#251406=CARTESIAN_POINT('Ctrl Pts',(17.7459450555812,15.4129242997837,12.));
#251407=CARTESIAN_POINT('Ctrl Pts',(17.7559493405881,15.4285794642668,12.));
#251408=CARTESIAN_POINT('Ctrl Pts',(17.7659740573265,15.4443634132869,12.));
#251409=CARTESIAN_POINT('Ctrl Pts',(17.7760182175815,15.4602755393018,12.));
#251410=CARTESIAN_POINT('Ctrl Pts',(17.7860808481219,15.4763152417497,12.));
#251411=CARTESIAN_POINT('Ctrl Pts',(17.7961609903148,15.4924819268517,12.));
#251412=CARTESIAN_POINT('Ctrl Pts',(17.8062576997952,15.5087750074718,12.));
#251413=CARTESIAN_POINT('Ctrl Pts',(17.8163700461256,15.5251939029552,12.));
#251414=CARTESIAN_POINT('Ctrl Pts',(17.8264971124606,15.541738038964,12.));
#251415=CARTESIAN_POINT('Ctrl Pts',(17.8366379952085,15.5584068472982,12.));
#251416=CARTESIAN_POINT('Ctrl Pts',(17.8467918036987,15.5751997657163,12.));
#251417=CARTESIAN_POINT('Ctrl Pts',(17.8569576599006,15.5921162378192,12.));
#251418=CARTESIAN_POINT('Ctrl Pts',(17.8671346981394,15.609155712921,12.));
#251419=CARTESIAN_POINT('Ctrl Pts',(17.8773220648125,15.6263176459108,12.));
#251420=CARTESIAN_POINT('Ctrl Pts',(17.8875189181091,15.6436014971085,12.));
#251421=CARTESIAN_POINT('Ctrl Pts',(17.897724427724,15.661006732103,12.));
#251422=CARTESIAN_POINT('Ctrl Pts',(17.9079377746111,15.6785328216461,12.));
#251423=CARTESIAN_POINT('Ctrl Pts',(17.9181581507455,15.6961792415522,12.));
#251424=CARTESIAN_POINT('Ctrl Pts',(17.9283847588836,15.7139454725839,12.));
#251425=CARTESIAN_POINT('Ctrl Pts',(17.9386168123262,15.7318310003335,12.));
#251426=CARTESIAN_POINT('Ctrl Pts',(17.9488535346781,15.749835315086,12.));
#251427=CARTESIAN_POINT('Ctrl Pts',(17.9590941596242,15.7679579117077,12.));
#251428=CARTESIAN_POINT('Ctrl Pts',(17.9693379307303,15.7861982895724,12.));
#251429=CARTESIAN_POINT('Ctrl Pts',(17.9795841012386,15.8045559524677,12.));
#251430=CARTESIAN_POINT('Ctrl Pts',(17.9898319338664,15.8230304084962,12.));
#251431=CARTESIAN_POINT('Ctrl Pts',(18.0000807006052,15.8416211699679,12.));
#251432=CARTESIAN_POINT('Ctrl Pts',(18.0103296825205,15.8603277532831,12.));
#251433=CARTESIAN_POINT('Ctrl Pts',(18.0205781695769,15.8791496788683,12.));
#251434=CARTESIAN_POINT('Ctrl Pts',(18.0308254604636,15.8980864711042,12.));
#251435=CARTESIAN_POINT('Ctrl Pts',(18.0410708624208,15.9171376582436,12.));
#251436=CARTESIAN_POINT('Ctrl Pts',(18.0513136910691,15.9363027723244,12.));
#251437=CARTESIAN_POINT('Ctrl Pts',(18.061553270236,15.9555813490644,12.));
#251438=CARTESIAN_POINT('Ctrl Pts',(18.0717889317958,15.9749729277846,12.));
#251439=CARTESIAN_POINT('Ctrl Pts',(18.0820200155236,15.9944770513613,12.));
#251440=CARTESIAN_POINT('Ctrl Pts',(18.0922458689462,16.014093266161,12.));
#251441=CARTESIAN_POINT('Ctrl Pts',(18.1024658471966,16.0338211219693,12.));
#251442=CARTESIAN_POINT('Ctrl Pts',(18.112679312869,16.0536601719126,12.));
#251443=CARTESIAN_POINT('Ctrl Pts',(18.1228856358751,16.0736099723668,12.));
#251444=CARTESIAN_POINT('Ctrl Pts',(18.1330841933105,16.0936700829112,12.));
#251445=CARTESIAN_POINT('Ctrl Pts',(18.1432743693235,16.1138400662794,12.));
#251446=CARTESIAN_POINT('Ctrl Pts',(18.1534555549852,16.1341194882988,12.));
#251447=CARTESIAN_POINT('Ctrl Pts',(18.1636271481615,16.154507917826,12.));
#251448=CARTESIAN_POINT('Ctrl Pts',(18.1737885533849,16.1750049266671,12.));
#251449=CARTESIAN_POINT('Ctrl Pts',(18.1839391817331,16.1956100895073,12.));
#251450=CARTESIAN_POINT('Ctrl Pts',(18.1940784507229,16.2163229838875,12.));
#251451=CARTESIAN_POINT('Ctrl Pts',(18.2042057842035,16.2371431901638,12.));
#251452=CARTESIAN_POINT('Ctrl Pts',(18.2143206122529,16.2580702914615,12.));
#251453=CARTESIAN_POINT('Ctrl Pts',(18.2244223710745,16.2791038736223,12.));
#251454=CARTESIAN_POINT('Ctrl Pts',(18.2345105028982,16.3002435251378,12.));
#251455=CARTESIAN_POINT('Ctrl Pts',(18.2445844558742,16.3214888370987,12.));
#251456=CARTESIAN_POINT('Ctrl Pts',(18.2546436839608,16.3428394031589,12.));
#251457=CARTESIAN_POINT('Ctrl Pts',(18.2646876468169,16.3642948194868,12.));
#251458=CARTESIAN_POINT('Ctrl Pts',(18.2747158096934,16.385854684708,12.));
#251459=CARTESIAN_POINT('Ctrl Pts',(18.2847276433309,16.4075185998455,12.));
#251460=CARTESIAN_POINT('Ctrl Pts',(18.294722623851,16.4292861682379,12.));
#251461=CARTESIAN_POINT('Ctrl Pts',(18.304700232686,16.4511569955233,12.));
#251462=CARTESIAN_POINT('Ctrl Pts',(18.3146599565231,16.4731306896441,12.));
#251463=CARTESIAN_POINT('Ctrl Pts',(18.3246012872469,16.4952068608345,12.));
#251464=CARTESIAN_POINT('Ctrl Pts',(18.3345237218864,16.5173851216045,12.));
#251465=CARTESIAN_POINT('Ctrl Pts',(18.34442676256,16.5396650867139,12.));
#251466=CARTESIAN_POINT('Ctrl Pts',(18.354309916433,16.5620463731413,12.));
#251467=CARTESIAN_POINT('Ctrl Pts',(18.3641726955889,16.5845286000217,12.));
#251468=CARTESIAN_POINT('Ctrl Pts',(18.3740146168879,16.607111388571,12.));
#251469=CARTESIAN_POINT('Ctrl Pts',(18.3838352018327,16.6297943620056,12.));
#251470=CARTESIAN_POINT('Ctrl Pts',(18.3936339764332,16.6525771454513,12.));
#251471=CARTESIAN_POINT('Ctrl Pts',(18.403410471079,16.6754593658513,12.));
#251472=CARTESIAN_POINT('Ctrl Pts',(18.413164220399,16.6984406518491,12.));
#251473=CARTESIAN_POINT('Ctrl Pts',(18.4228947633187,16.7215206338818,12.));
#251474=CARTESIAN_POINT('Ctrl Pts',(18.4326016431392,16.7446989442882,12.));
#251475=CARTESIAN_POINT('Ctrl Pts',(18.44228440761,16.7679752173992,12.));
#251476=CARTESIAN_POINT('Ctrl Pts',(18.4519426090123,16.791349089629,12.));
#251477=CARTESIAN_POINT('Ctrl Pts',(18.4615758042305,16.8148201995472,12.));
#251478=CARTESIAN_POINT('Ctrl Pts',(18.4711835548623,16.8383881879709,12.));
#251479=CARTESIAN_POINT('Ctrl Pts',(18.4807654268771,16.8620526977171,12.));
#251480=CARTESIAN_POINT('Ctrl Pts',(18.4903209902227,16.8858133733088,12.));
#251481=CARTESIAN_POINT('Ctrl Pts',(18.499849818462,16.9096698606943,12.));
#251482=CARTESIAN_POINT('Ctrl Pts',(18.5093514883835,16.9336218069353,12.));
#251483=CARTESIAN_POINT('Ctrl Pts',(18.5188255796659,16.9576688599339,12.));
#251484=CARTESIAN_POINT('Ctrl Pts',(18.5282716744197,16.981810668038,12.));
#251485=CARTESIAN_POINT('Ctrl Pts',(18.5376893576961,17.0060468805097,12.));
#251486=CARTESIAN_POINT('Ctrl Pts',(18.547078218209,17.0303771481738,12.));
#251487=CARTESIAN_POINT('Ctrl Pts',(18.556437848963,17.0548011239751,12.));
#251488=CARTESIAN_POINT('Ctrl Pts',(18.5657678479789,17.0793184636079,12.));
#251489=CARTESIAN_POINT('Ctrl Pts',(18.5750678188542,17.1039288260001,12.));
#251490=CARTESIAN_POINT('Ctrl Pts',(18.5843373717247,17.1286318741183,12.));
#251491=CARTESIAN_POINT('Ctrl Pts',(18.5935761222825,17.1534272741643,12.));
#251492=CARTESIAN_POINT('Ctrl Pts',(18.6027836898817,17.1783146940127,12.));
#251493=CARTESIAN_POINT('Ctrl Pts',(18.6119596959949,17.2032938019284,12.));
#251494=CARTESIAN_POINT('Ctrl Pts',(18.6211037624038,17.2283642650518,12.));
#251495=CARTESIAN_POINT('Ctrl Pts',(18.6302155097943,17.2535257482187,12.));
#251496=CARTESIAN_POINT('Ctrl Pts',(18.6392945554748,17.2787779120213,12.));
#251497=CARTESIAN_POINT('Ctrl Pts',(18.6483405141865,17.3041204135074,12.));
#251498=CARTESIAN_POINT('Ctrl Pts',(18.6573530024033,17.3295529098618,12.));
#251499=CARTESIAN_POINT('Ctrl Pts',(18.6663316416582,17.3550750612443,12.));
#251500=CARTESIAN_POINT('Ctrl Pts',(18.6752760624052,17.3806865340747,12.));
#251501=CARTESIAN_POINT('Ctrl Pts',(18.6841859073471,17.4063870038562,12.));
#251502=CARTESIAN_POINT('Ctrl Pts',(18.6930608357409,17.4321761588142,12.));
#251503=CARTESIAN_POINT('Ctrl Pts',(18.70190052503,17.4580537012753,12.));
#251504=CARTESIAN_POINT('Ctrl Pts',(18.7107046613912,17.4840193397162,12.));
#251505=CARTESIAN_POINT('Ctrl Pts',(18.7194729318098,17.5100727820876,12.));
#251506=CARTESIAN_POINT('Ctrl Pts',(18.7282050157138,17.5362137287593,12.));
#251507=CARTESIAN_POINT('Ctrl Pts',(18.7369005764553,17.5624418653245,12.));
#251508=CARTESIAN_POINT('Ctrl Pts',(18.7455592536687,17.5887568561371,12.));
#251509=CARTESIAN_POINT('Ctrl Pts',(18.7541806530984,17.6151583357012,12.));
#251510=CARTESIAN_POINT('Ctrl Pts',(18.762764361321,17.6416459210681,12.));
#251511=CARTESIAN_POINT('Ctrl Pts',(18.7713099642754,17.6682192274236,12.));
#251512=CARTESIAN_POINT('Ctrl Pts',(18.7798170641374,17.6948778823014,12.));
#251513=CARTESIAN_POINT('Ctrl Pts',(18.7882852976049,17.7216215409035,12.));
#251514=CARTESIAN_POINT('Ctrl Pts',(18.7967143519419,17.7484498996905,12.));
#251515=CARTESIAN_POINT('Ctrl Pts',(18.8051039860448,17.7753627137853,12.));
#251516=CARTESIAN_POINT('Ctrl Pts',(18.8134540340417,17.8023598011057,12.));
#251517=CARTESIAN_POINT('Ctrl Pts',(18.8217643886157,17.8294410311006,12.));
#251518=CARTESIAN_POINT('Ctrl Pts',(18.8300349895974,17.8566063174771,12.));
#251519=CARTESIAN_POINT('Ctrl Pts',(18.8366196462581,17.8784057509356,12.));
#251520=CARTESIAN_POINT('Ctrl Pts',(18.8415402351786,17.8947931177807,12.));
#251521=CARTESIAN_POINT('Ctrl Pts',(18.8448126709691,17.9057348246595,12.));
#251522=CARTESIAN_POINT('Ctrl Pts',(18.8464468996588,17.9112098770111,12.));
#251523=CARTESIAN_POINT('Ctrl Pts',(18.5896416359912,12.7689476255363,0.));
#251524=CARTESIAN_POINT('Ctrl Pts',(18.5896416359912,12.7689476255363,12.));
#251525=CARTESIAN_POINT('Ctrl Pts',(18.5896460962964,12.7689524524483,0.));
#251526=CARTESIAN_POINT('Ctrl Pts',(18.5896460962964,12.7689524524483,12.));
#251527=CARTESIAN_POINT('Ctrl Pts',(18.5896919669165,12.768986426692,0.));
#251528=CARTESIAN_POINT('Ctrl Pts',(18.5896919669165,12.768986426692,12.));
#251529=CARTESIAN_POINT('Ctrl Pts',(18.589871621843,12.769110348199,0.));
#251530=CARTESIAN_POINT('Ctrl Pts',(18.589871621843,12.769110348199,12.));
#251531=CARTESIAN_POINT('Ctrl Pts',(18.5903328777227,12.7694215127919,0.));
#251532=CARTESIAN_POINT('Ctrl Pts',(18.5903328777227,12.7694215127919,12.));
#251533=CARTESIAN_POINT('Ctrl Pts',(18.5912775137806,12.7700520897173,0.));
#251534=CARTESIAN_POINT('Ctrl Pts',(18.5912775137806,12.7700520897173,12.));
#251535=CARTESIAN_POINT('Ctrl Pts',(18.5925859134579,12.7709195951156,0.));
#251536=CARTESIAN_POINT('Ctrl Pts',(18.5925859134579,12.7709195951156,12.));
#251537=CARTESIAN_POINT('Ctrl Pts',(18.5942490615407,12.7720142287172,0.));
#251538=CARTESIAN_POINT('Ctrl Pts',(18.5942490615407,12.7720142287172,12.));
#251539=CARTESIAN_POINT('Ctrl Pts',(18.5962551167772,12.7733231262108,0.));
#251540=CARTESIAN_POINT('Ctrl Pts',(18.5962551167772,12.7733231262108,12.));
#251541=CARTESIAN_POINT('Ctrl Pts',(18.598591752595,12.7748328937638,0.));
#251542=CARTESIAN_POINT('Ctrl Pts',(18.598591752595,12.7748328937638,12.));
#251543=CARTESIAN_POINT('Ctrl Pts',(18.6012488486709,12.7765325225081,0.));
#251544=CARTESIAN_POINT('Ctrl Pts',(18.6012488486709,12.7765325225081,12.));
#251545=CARTESIAN_POINT('Ctrl Pts',(18.6042190183704,12.7784139605066,0.));
#251546=CARTESIAN_POINT('Ctrl Pts',(18.6042190183704,12.7784139605066,12.));
#251547=CARTESIAN_POINT('Ctrl Pts',(18.6074961535723,12.7804705387658,0.));
#251548=CARTESIAN_POINT('Ctrl Pts',(18.6074961535723,12.7804705387658,12.));
#251549=CARTESIAN_POINT('Ctrl Pts',(18.6110744826219,12.7826959526925,0.));
#251550=CARTESIAN_POINT('Ctrl Pts',(18.6110744826219,12.7826959526925,12.));
#251551=CARTESIAN_POINT('Ctrl Pts',(18.6149475565188,12.7850831657901,0.));
#251552=CARTESIAN_POINT('Ctrl Pts',(18.6149475565188,12.7850831657901,12.));
#251553=CARTESIAN_POINT('Ctrl Pts',(18.6191087624752,12.7876249657834,0.));
#251554=CARTESIAN_POINT('Ctrl Pts',(18.6191087624752,12.7876249657834,12.));
#251555=CARTESIAN_POINT('Ctrl Pts',(18.6235516265575,12.7903142925234,0.));
#251556=CARTESIAN_POINT('Ctrl Pts',(18.6235516265575,12.7903142925234,12.));
#251557=CARTESIAN_POINT('Ctrl Pts',(18.6282702819371,12.7931447451555,0.));
#251558=CARTESIAN_POINT('Ctrl Pts',(18.6282702819371,12.7931447451555,12.));
#251559=CARTESIAN_POINT('Ctrl Pts',(18.6332595057006,12.7961106222251,0.));
#251560=CARTESIAN_POINT('Ctrl Pts',(18.6332595057006,12.7961106222251,12.));
#251561=CARTESIAN_POINT('Ctrl Pts',(18.63851447924,12.7992066625264,0.));
#251562=CARTESIAN_POINT('Ctrl Pts',(18.63851447924,12.7992066625264,12.));
#251563=CARTESIAN_POINT('Ctrl Pts',(18.6440306327456,12.8024278770153,0.));
#251564=CARTESIAN_POINT('Ctrl Pts',(18.6440306327456,12.8024278770153,12.));
#251565=CARTESIAN_POINT('Ctrl Pts',(18.6498034438987,12.805769331162,0.));
#251566=CARTESIAN_POINT('Ctrl Pts',(18.6498034438987,12.805769331162,12.));
#251567=CARTESIAN_POINT('Ctrl Pts',(18.6558284825773,12.8092261933858,0.));
#251568=CARTESIAN_POINT('Ctrl Pts',(18.6558284825773,12.8092261933858,12.));
#251569=CARTESIAN_POINT('Ctrl Pts',(18.6621014624746,12.8127937909631,0.));
#251570=CARTESIAN_POINT('Ctrl Pts',(18.6621014624746,12.8127937909631,12.));
#251571=CARTESIAN_POINT('Ctrl Pts',(18.6686182952799,12.8164676687362,0.));
#251572=CARTESIAN_POINT('Ctrl Pts',(18.6686182952799,12.8164676687362,12.));
#251573=CARTESIAN_POINT('Ctrl Pts',(18.6753751301092,12.8202436318474,0.));
#251574=CARTESIAN_POINT('Ctrl Pts',(18.6753751301092,12.8202436318474,12.));
#251575=CARTESIAN_POINT('Ctrl Pts',(18.6823683094139,12.8241176980017,0.));
#251576=CARTESIAN_POINT('Ctrl Pts',(18.6823683094139,12.8241176980017,12.));
#251577=CARTESIAN_POINT('Ctrl Pts',(18.6895943376171,12.8280860635231,0.));
#251578=CARTESIAN_POINT('Ctrl Pts',(18.6895943376171,12.8280860635231,12.));
#251579=CARTESIAN_POINT('Ctrl Pts',(18.6970498410172,12.8321450599789,0.));
#251580=CARTESIAN_POINT('Ctrl Pts',(18.6970498410172,12.8321450599789,12.));
#251581=CARTESIAN_POINT('Ctrl Pts',(18.7047315436294,12.8362911280361,0.));
#251582=CARTESIAN_POINT('Ctrl Pts',(18.7047315436294,12.8362911280361,12.));
#251583=CARTESIAN_POINT('Ctrl Pts',(18.7126362754445,12.8405208263431,0.));
#251584=CARTESIAN_POINT('Ctrl Pts',(18.7126362754445,12.8405208263431,12.));
#251585=CARTESIAN_POINT('Ctrl Pts',(18.7207609737702,12.8448308329494,0.));
#251586=CARTESIAN_POINT('Ctrl Pts',(18.7207609737702,12.8448308329494,12.));
#251587=CARTESIAN_POINT('Ctrl Pts',(18.7291026886554,12.8492179511591,0.));
#251588=CARTESIAN_POINT('Ctrl Pts',(18.7291026886554,12.8492179511591,12.));
#251589=CARTESIAN_POINT('Ctrl Pts',(18.7376585820854,12.8536791086316,0.));
#251590=CARTESIAN_POINT('Ctrl Pts',(18.7376585820854,12.8536791086316,12.));
#251591=CARTESIAN_POINT('Ctrl Pts',(18.7464259171251,12.8582113455646,0.));
#251592=CARTESIAN_POINT('Ctrl Pts',(18.7464259171251,12.8582113455646,12.));
#251593=CARTESIAN_POINT('Ctrl Pts',(18.7554020493887,12.8628118054171,0.));
#251594=CARTESIAN_POINT('Ctrl Pts',(18.7554020493887,12.8628118054171,12.));
#251595=CARTESIAN_POINT('Ctrl Pts',(18.7645844169564,12.8674777239653,0.));
#251596=CARTESIAN_POINT('Ctrl Pts',(18.7645844169564,12.8674777239653,12.));
#251597=CARTESIAN_POINT('Ctrl Pts',(18.7739705329022,12.872206421181,0.));
#251598=CARTESIAN_POINT('Ctrl Pts',(18.7739705329022,12.872206421181,12.));
#251599=CARTESIAN_POINT('Ctrl Pts',(18.7835579840477,12.8769952998095,0.));
#251600=CARTESIAN_POINT('Ctrl Pts',(18.7835579840477,12.8769952998095,12.));
#251601=CARTESIAN_POINT('Ctrl Pts',(18.7933444285868,12.8818418427475,0.));
#251602=CARTESIAN_POINT('Ctrl Pts',(18.7933444285868,12.8818418427475,12.));
#251603=CARTESIAN_POINT('Ctrl Pts',(18.8033275941943,12.8867436109546,0.));
#251604=CARTESIAN_POINT('Ctrl Pts',(18.8033275941943,12.8867436109546,12.));
#251605=CARTESIAN_POINT('Ctrl Pts',(18.813505275782,12.8916982409935,0.));
#251606=CARTESIAN_POINT('Ctrl Pts',(18.813505275782,12.8916982409935,12.));
#251607=CARTESIAN_POINT('Ctrl Pts',(18.8238753319129,12.8967034410755,0.));
#251608=CARTESIAN_POINT('Ctrl Pts',(18.8238753319129,12.8967034410755,12.));
#251609=CARTESIAN_POINT('Ctrl Pts',(18.834435681259,12.9017569871738,0.));
#251610=CARTESIAN_POINT('Ctrl Pts',(18.834435681259,12.9017569871738,12.));
#251611=CARTESIAN_POINT('Ctrl Pts',(18.8451842990984,12.9068567191854,0.));
#251612=CARTESIAN_POINT('Ctrl Pts',(18.8451842990984,12.9068567191854,12.));
#251613=CARTESIAN_POINT('Ctrl Pts',(18.8561192136198,12.9120005369063,0.));
#251614=CARTESIAN_POINT('Ctrl Pts',(18.8561192136198,12.9120005369063,12.));
#251615=CARTESIAN_POINT('Ctrl Pts',(18.8672385038326,12.9171863977045,0.));
#251616=CARTESIAN_POINT('Ctrl Pts',(18.8672385038326,12.9171863977045,12.));
#251617=CARTESIAN_POINT('Ctrl Pts',(18.8785402977527,12.9224123144982,0.));
#251618=CARTESIAN_POINT('Ctrl Pts',(18.8785402977527,12.9224123144982,12.));
#251619=CARTESIAN_POINT('Ctrl Pts',(18.8900227704889,12.9276763536373,0.));
#251620=CARTESIAN_POINT('Ctrl Pts',(18.8900227704889,12.9276763536373,12.));
#251621=CARTESIAN_POINT('Ctrl Pts',(18.9016841423403,12.9329766328185,0.));
#251622=CARTESIAN_POINT('Ctrl Pts',(18.9016841423403,12.9329766328185,12.));
#251623=CARTESIAN_POINT('Ctrl Pts',(18.9135226769465,12.9383113190375,0.));
#251624=CARTESIAN_POINT('Ctrl Pts',(18.9135226769465,12.9383113190375,12.));
#251625=CARTESIAN_POINT('Ctrl Pts',(18.9255366795195,12.9436786266105,0.));
#251626=CARTESIAN_POINT('Ctrl Pts',(18.9255366795195,12.9436786266105,12.));
#251627=CARTESIAN_POINT('Ctrl Pts',(18.9377244950435,12.9490768151821,0.));
#251628=CARTESIAN_POINT('Ctrl Pts',(18.9377244950435,12.9490768151821,12.));
#251629=CARTESIAN_POINT('Ctrl Pts',(18.9500845064715,12.9545041877377,0.));
#251630=CARTESIAN_POINT('Ctrl Pts',(18.9500845064715,12.9545041877377,12.));
#251631=CARTESIAN_POINT('Ctrl Pts',(18.9626151329229,12.9599590886319,0.));
#251632=CARTESIAN_POINT('Ctrl Pts',(18.9626151329229,12.9599590886319,12.));
#251633=CARTESIAN_POINT('Ctrl Pts',(18.9753148284475,12.9654399021869,0.));
#251634=CARTESIAN_POINT('Ctrl Pts',(18.9753148284475,12.9654399021869,12.));
#251635=CARTESIAN_POINT('Ctrl Pts',(18.9881820807585,12.9709450512747,0.));
#251636=CARTESIAN_POINT('Ctrl Pts',(18.9881820807585,12.9709450512747,12.));
#251637=CARTESIAN_POINT('Ctrl Pts',(19.0012154099791,12.9764729959205,0.));
#251638=CARTESIAN_POINT('Ctrl Pts',(19.0012154099791,12.9764729959205,12.));
#251639=CARTESIAN_POINT('Ctrl Pts',(19.0144133673348,12.9820222318716,0.));
#251640=CARTESIAN_POINT('Ctrl Pts',(19.0144133673348,12.9820222318716,12.));
#251641=CARTESIAN_POINT('Ctrl Pts',(19.0277745339908,12.9875912893003,0.));
#251642=CARTESIAN_POINT('Ctrl Pts',(19.0277745339908,12.9875912893003,12.));
#251643=CARTESIAN_POINT('Ctrl Pts',(19.0412975200398,12.9931787316515,0.));
#251644=CARTESIAN_POINT('Ctrl Pts',(19.0412975200398,12.9931787316515,12.));
#251645=CARTESIAN_POINT('Ctrl Pts',(19.0549809634355,12.9987831544502,0.));
#251646=CARTESIAN_POINT('Ctrl Pts',(19.0549809634355,12.9987831544502,12.));
#251647=CARTESIAN_POINT('Ctrl Pts',(19.0688235289437,13.0044031841381,0.));
#251648=CARTESIAN_POINT('Ctrl Pts',(19.0688235289437,13.0044031841381,12.));
#251649=CARTESIAN_POINT('Ctrl Pts',(19.0828239070482,13.0100374768786,0.));
#251650=CARTESIAN_POINT('Ctrl Pts',(19.0828239070482,13.0100374768786,12.));
#251651=CARTESIAN_POINT('Ctrl Pts',(19.0969808131226,13.0156847176094,0.));
#251652=CARTESIAN_POINT('Ctrl Pts',(19.0969808131226,13.0156847176094,12.));
#251653=CARTESIAN_POINT('Ctrl Pts',(19.1112929866308,13.0213436191326,0.));
#251654=CARTESIAN_POINT('Ctrl Pts',(19.1112929866308,13.0213436191326,12.));
#251655=CARTESIAN_POINT('Ctrl Pts',(19.1257591903099,13.0270129211976,0.));
#251656=CARTESIAN_POINT('Ctrl Pts',(19.1257591903099,13.0270129211976,12.));
#251657=CARTESIAN_POINT('Ctrl Pts',(19.1403782093389,13.0326913895841,0.));
#251658=CARTESIAN_POINT('Ctrl Pts',(19.1403782093389,13.0326913895841,12.));
#251659=CARTESIAN_POINT('Ctrl Pts',(19.1551488505233,13.0383778152072,0.));
#251660=CARTESIAN_POINT('Ctrl Pts',(19.1551488505233,13.0383778152072,12.));
#251661=CARTESIAN_POINT('Ctrl Pts',(19.1700699416625,13.0440710133775,0.));
#251662=CARTESIAN_POINT('Ctrl Pts',(19.1700699416625,13.0440710133775,12.));
#251663=CARTESIAN_POINT('Ctrl Pts',(19.1851403308825,13.0497698230442,0.));
#251664=CARTESIAN_POINT('Ctrl Pts',(19.1851403308825,13.0497698230442,12.));
#251665=CARTESIAN_POINT('Ctrl Pts',(19.2003588859771,13.0554731060537,0.));
#251666=CARTESIAN_POINT('Ctrl Pts',(19.2003588859771,13.0554731060537,12.));
#251667=CARTESIAN_POINT('Ctrl Pts',(19.2157244937141,13.0611797463913,0.));
#251668=CARTESIAN_POINT('Ctrl Pts',(19.2157244937141,13.0611797463913,12.));
#251669=CARTESIAN_POINT('Ctrl Pts',(19.2312360592031,13.0668886494791,0.));
#251670=CARTESIAN_POINT('Ctrl Pts',(19.2312360592031,13.0668886494791,12.));
#251671=CARTESIAN_POINT('Ctrl Pts',(19.2468925053988,13.0725987415856,0.));
#251672=CARTESIAN_POINT('Ctrl Pts',(19.2468925053988,13.0725987415856,12.));
#251673=CARTESIAN_POINT('Ctrl Pts',(19.2626927725596,13.0783089692118,0.));
#251674=CARTESIAN_POINT('Ctrl Pts',(19.2626927725596,13.0783089692118,12.));
#251675=CARTESIAN_POINT('Ctrl Pts',(19.2786358177198,13.0840182984949,0.));
#251676=CARTESIAN_POINT('Ctrl Pts',(19.2786358177198,13.0840182984949,12.));
#251677=CARTESIAN_POINT('Ctrl Pts',(19.2947206141246,13.089725714597,0.));
#251678=CARTESIAN_POINT('Ctrl Pts',(19.2947206141246,13.089725714597,12.));
#251679=CARTESIAN_POINT('Ctrl Pts',(19.3109461507358,13.095430221148,0.));
#251680=CARTESIAN_POINT('Ctrl Pts',(19.3109461507358,13.095430221148,12.));
#251681=CARTESIAN_POINT('Ctrl Pts',(19.3273114318268,13.1011308397592,0.));
#251682=CARTESIAN_POINT('Ctrl Pts',(19.3273114318268,13.1011308397592,12.));
#251683=CARTESIAN_POINT('Ctrl Pts',(19.3438154765395,13.1068266095186,0.));
#251684=CARTESIAN_POINT('Ctrl Pts',(19.3438154765395,13.1068266095186,12.));
#251685=CARTESIAN_POINT('Ctrl Pts',(19.3604573184516,13.1125165865021,0.));
#251686=CARTESIAN_POINT('Ctrl Pts',(19.3604573184516,13.1125165865021,12.));
#251687=CARTESIAN_POINT('Ctrl Pts',(19.3772360051093,13.118199843271,0.));
#251688=CARTESIAN_POINT('Ctrl Pts',(19.3772360051093,13.118199843271,12.));
#251689=CARTESIAN_POINT('Ctrl Pts',(19.3941505976267,13.1238754684177,0.));
#251690=CARTESIAN_POINT('Ctrl Pts',(19.3941505976267,13.1238754684177,12.));
#251691=CARTESIAN_POINT('Ctrl Pts',(19.4112001703561,13.1295425661635,0.));
#251692=CARTESIAN_POINT('Ctrl Pts',(19.4112001703561,13.1295425661635,12.));
#251693=CARTESIAN_POINT('Ctrl Pts',(19.4283838105265,13.135200255944,0.));
#251694=CARTESIAN_POINT('Ctrl Pts',(19.4283838105265,13.135200255944,12.));
#251695=CARTESIAN_POINT('Ctrl Pts',(19.4457006178875,13.140847672006,0.));
#251696=CARTESIAN_POINT('Ctrl Pts',(19.4457006178875,13.140847672006,12.));
#251697=CARTESIAN_POINT('Ctrl Pts',(19.463149704325,13.1464839629966,0.));
#251698=CARTESIAN_POINT('Ctrl Pts',(19.463149704325,13.1464839629966,12.));
#251699=CARTESIAN_POINT('Ctrl Pts',(19.4807301935256,13.1521082915846,0.));
#251700=CARTESIAN_POINT('Ctrl Pts',(19.4807301935256,13.1521082915846,12.));
#251701=CARTESIAN_POINT('Ctrl Pts',(19.498441220707,13.1577198341238,0.));
#251702=CARTESIAN_POINT('Ctrl Pts',(19.498441220707,13.1577198341238,12.));
#251703=CARTESIAN_POINT('Ctrl Pts',(19.5162819323207,13.1633177803097,0.));
#251704=CARTESIAN_POINT('Ctrl Pts',(19.5162819323207,13.1633177803097,12.));
#251705=CARTESIAN_POINT('Ctrl Pts',(19.5342514857564,13.1689013328432,0.));
#251706=CARTESIAN_POINT('Ctrl Pts',(19.5342514857564,13.1689013328432,12.));
#251707=CARTESIAN_POINT('Ctrl Pts',(19.5523490490254,13.1744697070918,0.));
#251708=CARTESIAN_POINT('Ctrl Pts',(19.5523490490254,13.1744697070918,12.));
#251709=CARTESIAN_POINT('Ctrl Pts',(19.5705738004682,13.1800221307683,0.));
#251710=CARTESIAN_POINT('Ctrl Pts',(19.5705738004682,13.1800221307683,12.));
#251711=CARTESIAN_POINT('Ctrl Pts',(19.5889249285352,13.185557843648,0.));
#251712=CARTESIAN_POINT('Ctrl Pts',(19.5889249285352,13.185557843648,12.));
#251713=CARTESIAN_POINT('Ctrl Pts',(19.6074016315421,13.1910760972818,0.));
#251714=CARTESIAN_POINT('Ctrl Pts',(19.6074016315421,13.1910760972818,12.));
#251715=CARTESIAN_POINT('Ctrl Pts',(19.6260031174244,13.196576154715,0.));
#251716=CARTESIAN_POINT('Ctrl Pts',(19.6260031174244,13.196576154715,12.));
#251717=CARTESIAN_POINT('Ctrl Pts',(19.6447286034764,13.202057290206,0.));
#251718=CARTESIAN_POINT('Ctrl Pts',(19.6447286034764,13.202057290206,12.));
#251719=CARTESIAN_POINT('Ctrl Pts',(19.6635773160924,13.2075187889522,0.));
#251720=CARTESIAN_POINT('Ctrl Pts',(19.6635773160924,13.2075187889522,12.));
#251721=CARTESIAN_POINT('Ctrl Pts',(19.6825484905812,13.2129599468478,0.));
#251722=CARTESIAN_POINT('Ctrl Pts',(19.6825484905812,13.2129599468478,12.));
#251723=CARTESIAN_POINT('Ctrl Pts',(19.7016413709678,13.2183800702431,0.));
#251724=CARTESIAN_POINT('Ctrl Pts',(19.7016413709678,13.2183800702431,12.));
#251725=CARTESIAN_POINT('Ctrl Pts',(19.7208552097867,13.2237784757065,0.));
#251726=CARTESIAN_POINT('Ctrl Pts',(19.7208552097867,13.2237784757065,12.));
#251727=CARTESIAN_POINT('Ctrl Pts',(19.7401892678701,13.2291544897902,0.));
#251728=CARTESIAN_POINT('Ctrl Pts',(19.7401892678701,13.2291544897902,12.));
#251729=CARTESIAN_POINT('Ctrl Pts',(19.7596428141176,13.2345074487968,0.));
#251730=CARTESIAN_POINT('Ctrl Pts',(19.7596428141176,13.2345074487968,12.));
#251731=CARTESIAN_POINT('Ctrl Pts',(19.7792151253297,13.239836698568,0.));
#251732=CARTESIAN_POINT('Ctrl Pts',(19.7792151253297,13.239836698568,12.));
#251733=CARTESIAN_POINT('Ctrl Pts',(19.7989054860501,13.2451415942809,0.));
#251734=CARTESIAN_POINT('Ctrl Pts',(19.7989054860501,13.2451415942809,12.));
#251735=CARTESIAN_POINT('Ctrl Pts',(19.8187131883919,13.2504215002458,0.));
#251736=CARTESIAN_POINT('Ctrl Pts',(19.8187131883919,13.2504215002458,12.));
#251737=CARTESIAN_POINT('Ctrl Pts',(19.8386375318632,13.2556757897085,0.));
#251738=CARTESIAN_POINT('Ctrl Pts',(19.8386375318632,13.2556757897085,12.));
#251739=CARTESIAN_POINT('Ctrl Pts',(19.8586778231711,13.2609038446525,0.));
#251740=CARTESIAN_POINT('Ctrl Pts',(19.8586778231711,13.2609038446525,12.));
#251741=CARTESIAN_POINT('Ctrl Pts',(19.8788333760571,13.2661050556128,0.));
#251742=CARTESIAN_POINT('Ctrl Pts',(19.8788333760571,13.2661050556128,12.));
#251743=CARTESIAN_POINT('Ctrl Pts',(19.8991035111739,13.2712788215015,0.));
#251744=CARTESIAN_POINT('Ctrl Pts',(19.8991035111739,13.2712788215015,12.));
#251745=CARTESIAN_POINT('Ctrl Pts',(19.9194875559419,13.2764245494354,0.));
#251746=CARTESIAN_POINT('Ctrl Pts',(19.9194875559419,13.2764245494354,12.));
#251747=CARTESIAN_POINT('Ctrl Pts',(19.9399848444019,13.2815416545663,0.));
#251748=CARTESIAN_POINT('Ctrl Pts',(19.9399848444019,13.2815416545663,12.));
#251749=CARTESIAN_POINT('Ctrl Pts',(19.9605947170589,13.2866295599152,0.));
#251750=CARTESIAN_POINT('Ctrl Pts',(19.9605947170589,13.2866295599152,12.));
#251751=CARTESIAN_POINT('Ctrl Pts',(19.9813165207174,13.2916876962098,0.));
#251752=CARTESIAN_POINT('Ctrl Pts',(19.9813165207174,13.2916876962098,12.));
#251753=CARTESIAN_POINT('Ctrl Pts',(20.0021496083742,13.296715501731,0.));
#251754=CARTESIAN_POINT('Ctrl Pts',(20.0021496083742,13.296715501731,12.));
#251755=CARTESIAN_POINT('Ctrl Pts',(20.0230933391039,13.3017124221639,0.));
#251756=CARTESIAN_POINT('Ctrl Pts',(20.0230933391039,13.3017124221639,12.));
#251757=CARTESIAN_POINT('Ctrl Pts',(20.0441470779345,13.3066779104515,0.));
#251758=CARTESIAN_POINT('Ctrl Pts',(20.0441470779345,13.3066779104515,12.));
#251759=CARTESIAN_POINT('Ctrl Pts',(20.0653101957188,13.3116114266514,0.));
#251760=CARTESIAN_POINT('Ctrl Pts',(20.0653101957188,13.3116114266514,12.));
#251761=CARTESIAN_POINT('Ctrl Pts',(20.0865820689883,13.3165124377963,0.));
#251762=CARTESIAN_POINT('Ctrl Pts',(20.0865820689883,13.3165124377963,12.));
#251763=CARTESIAN_POINT('Ctrl Pts',(20.1079620798377,13.3213804177588,0.));
#251764=CARTESIAN_POINT('Ctrl Pts',(20.1079620798377,13.3213804177588,12.));
#251765=CARTESIAN_POINT('Ctrl Pts',(20.1294496158405,13.3262148471228,0.));
#251766=CARTESIAN_POINT('Ctrl Pts',(20.1294496158405,13.3262148471228,12.));
#251767=CARTESIAN_POINT('Ctrl Pts',(20.1510440699477,13.3310152130565,0.));
#251768=CARTESIAN_POINT('Ctrl Pts',(20.1510440699477,13.3310152130565,12.));
#251769=CARTESIAN_POINT('Ctrl Pts',(20.1727448403818,13.3357810091903,0.));
#251770=CARTESIAN_POINT('Ctrl Pts',(20.1727448403818,13.3357810091903,12.));
#251771=CARTESIAN_POINT('Ctrl Pts',(20.1945513305233,13.3405117354969,0.));
#251772=CARTESIAN_POINT('Ctrl Pts',(20.1945513305233,13.3405117354969,12.));
#251773=CARTESIAN_POINT('Ctrl Pts',(20.2164629487855,13.3452068981763,0.));
#251774=CARTESIAN_POINT('Ctrl Pts',(20.2164629487855,13.3452068981763,12.));
#251775=CARTESIAN_POINT('Ctrl Pts',(20.2384791085354,13.3498660095382,0.));
#251776=CARTESIAN_POINT('Ctrl Pts',(20.2384791085354,13.3498660095382,12.));
#251777=CARTESIAN_POINT('Ctrl Pts',(20.2605992280117,13.3544885878886,0.));
#251778=CARTESIAN_POINT('Ctrl Pts',(20.2605992280117,13.3544885878886,12.));
#251779=CARTESIAN_POINT('Ctrl Pts',(20.2828227302337,13.3590741574194,0.));
#251780=CARTESIAN_POINT('Ctrl Pts',(20.2828227302337,13.3590741574194,12.));
#251781=CARTESIAN_POINT('Ctrl Pts',(20.3051490429049,13.3636222481017,0.));
#251782=CARTESIAN_POINT('Ctrl Pts',(20.3051490429049,13.3636222481017,12.));
#251783=CARTESIAN_POINT('Ctrl Pts',(20.3275775983032,13.3681323955828,0.));
#251784=CARTESIAN_POINT('Ctrl Pts',(20.3275775983032,13.3681323955828,12.));
#251785=CARTESIAN_POINT('Ctrl Pts',(20.3501078331818,13.372604141087,0.));
#251786=CARTESIAN_POINT('Ctrl Pts',(20.3501078331818,13.372604141087,12.));
#251787=CARTESIAN_POINT('Ctrl Pts',(20.3727391887187,13.377037031319,0.));
#251788=CARTESIAN_POINT('Ctrl Pts',(20.3727391887187,13.377037031319,12.));
#251789=CARTESIAN_POINT('Ctrl Pts',(20.3954711104504,13.3814306183721,0.));
#251790=CARTESIAN_POINT('Ctrl Pts',(20.3954711104504,13.3814306183721,12.));
#251791=CARTESIAN_POINT('Ctrl Pts',(20.4183030482002,13.3857844596387,0.));
#251792=CARTESIAN_POINT('Ctrl Pts',(20.4183030482002,13.3857844596387,12.));
#251793=CARTESIAN_POINT('Ctrl Pts',(20.4412344560007,13.3900981177254,0.));
#251794=CARTESIAN_POINT('Ctrl Pts',(20.4412344560007,13.3900981177254,12.));
#251795=CARTESIAN_POINT('Ctrl Pts',(20.4642647920038,13.3943711603739,0.));
#251796=CARTESIAN_POINT('Ctrl Pts',(20.4642647920038,13.3943711603739,12.));
#251797=CARTESIAN_POINT('Ctrl Pts',(20.4873935184041,13.3986031603716,0.));
#251798=CARTESIAN_POINT('Ctrl Pts',(20.4873935184041,13.3986031603716,12.));
#251799=CARTESIAN_POINT('Ctrl Pts',(20.5106201013755,13.4027936954529,0.));
#251800=CARTESIAN_POINT('Ctrl Pts',(20.5106201013755,13.4027936954529,12.));
#251801=CARTESIAN_POINT('Ctrl Pts',(20.5339440109957,13.4069423482077,0.));
#251802=CARTESIAN_POINT('Ctrl Pts',(20.5339440109957,13.4069423482077,12.));
#251803=CARTESIAN_POINT('Ctrl Pts',(20.557364721164,13.4110487059912,0.));
#251804=CARTESIAN_POINT('Ctrl Pts',(20.557364721164,13.4110487059912,12.));
#251805=CARTESIAN_POINT('Ctrl Pts',(20.5808817095155,13.4151123608411,0.));
#251806=CARTESIAN_POINT('Ctrl Pts',(20.5808817095155,13.4151123608411,12.));
#251807=CARTESIAN_POINT('Ctrl Pts',(20.6044944573151,13.4191329093932,0.));
#251808=CARTESIAN_POINT('Ctrl Pts',(20.6044944573151,13.4191329093932,12.));
#251809=CARTESIAN_POINT('Ctrl Pts',(20.6282024494234,13.4231099528178,0.));
#251810=CARTESIAN_POINT('Ctrl Pts',(20.6282024494234,13.4231099528178,12.));
#251811=CARTESIAN_POINT('Ctrl Pts',(20.6520051742867,13.4270430967651,0.));
#251812=CARTESIAN_POINT('Ctrl Pts',(20.6520051742867,13.4270430967651,12.));
#251813=CARTESIAN_POINT('Ctrl Pts',(20.6759021239102,13.4309319513119,0.));
#251814=CARTESIAN_POINT('Ctrl Pts',(20.6759021239102,13.4309319513119,12.));
#251815=CARTESIAN_POINT('Ctrl Pts',(20.6998927938288,13.4347761309154,0.));
#251816=CARTESIAN_POINT('Ctrl Pts',(20.6998927938288,13.4347761309154,12.));
#251817=CARTESIAN_POINT('Ctrl Pts',(20.7239766830675,13.4385752543663,0.));
#251818=CARTESIAN_POINT('Ctrl Pts',(20.7239766830675,13.4385752543663,12.));
#251819=CARTESIAN_POINT('Ctrl Pts',(20.7481532941014,13.4423289447561,0.));
#251820=CARTESIAN_POINT('Ctrl Pts',(20.7481532941014,13.4423289447561,12.));
#251821=CARTESIAN_POINT('Ctrl Pts',(20.7724221327609,13.4460368293689,0.));
#251822=CARTESIAN_POINT('Ctrl Pts',(20.7724221327609,13.4460368293689,12.));
#251823=CARTESIAN_POINT('Ctrl Pts',(20.7967827081228,13.4496985395637,0.));
#251824=CARTESIAN_POINT('Ctrl Pts',(20.7967827081228,13.4496985395637,12.));
#251825=CARTESIAN_POINT('Ctrl Pts',(20.821234532398,13.4533137106667,0.));
#251826=CARTESIAN_POINT('Ctrl Pts',(20.821234532398,13.4533137106667,12.));
#251827=CARTESIAN_POINT('Ctrl Pts',(20.8457771208083,13.4568819818631,0.));
#251828=CARTESIAN_POINT('Ctrl Pts',(20.8457771208083,13.4568819818631,12.));
#251829=CARTESIAN_POINT('Ctrl Pts',(20.8704099914641,13.4604029960983,0.));
#251830=CARTESIAN_POINT('Ctrl Pts',(20.8704099914641,13.4604029960983,12.));
#251831=CARTESIAN_POINT('Ctrl Pts',(20.8951326652158,13.4638763999725,0.));
#251832=CARTESIAN_POINT('Ctrl Pts',(20.8951326652158,13.4638763999725,12.));
#251833=CARTESIAN_POINT('Ctrl Pts',(20.9199446657583,13.4673018437717,0.));
#251834=CARTESIAN_POINT('Ctrl Pts',(20.9199446657583,13.4673018437717,12.));
#251835=CARTESIAN_POINT('Ctrl Pts',(20.9448455197557,13.4706789815166,0.));
#251836=CARTESIAN_POINT('Ctrl Pts',(20.9448455197557,13.4706789815166,12.));
#251837=CARTESIAN_POINT('Ctrl Pts',(20.9698347569477,13.4740074710086,0.));
#251838=CARTESIAN_POINT('Ctrl Pts',(20.9698347569477,13.4740074710086,12.));
#251839=CARTESIAN_POINT('Ctrl Pts',(20.9949119102592,13.4772869738879,0.));
#251840=CARTESIAN_POINT('Ctrl Pts',(20.9949119102592,13.4772869738879,12.));
#251841=CARTESIAN_POINT('Ctrl Pts',(21.0200765158884,13.4805171556822,0.));
#251842=CARTESIAN_POINT('Ctrl Pts',(21.0200765158884,13.4805171556822,12.));
#251843=CARTESIAN_POINT('Ctrl Pts',(21.0453281134245,13.4836976858912,0.));
#251844=CARTESIAN_POINT('Ctrl Pts',(21.0453281134245,13.4836976858912,12.));
#251845=CARTESIAN_POINT('Ctrl Pts',(21.0706662455199,13.4868282377191,0.));
#251846=CARTESIAN_POINT('Ctrl Pts',(21.0706662455199,13.4868282377191,12.));
#251847=CARTESIAN_POINT('Ctrl Pts',(21.0960904575046,13.4899084877717,0.));
#251848=CARTESIAN_POINT('Ctrl Pts',(21.0960904575046,13.4899084877717,12.));
#251849=CARTESIAN_POINT('Ctrl Pts',(21.1216002970207,13.4929381157778,0.));
#251850=CARTESIAN_POINT('Ctrl Pts',(21.1216002970207,13.4929381157778,12.));
#251851=CARTESIAN_POINT('Ctrl Pts',(21.1471953136209,13.4959168042934,0.));
#251852=CARTESIAN_POINT('Ctrl Pts',(21.1471953136209,13.4959168042934,12.));
#251853=CARTESIAN_POINT('Ctrl Pts',(21.1728750584175,13.4988442384491,0.));
#251854=CARTESIAN_POINT('Ctrl Pts',(21.1728750584175,13.4988442384491,12.));
#251855=CARTESIAN_POINT('Ctrl Pts',(21.1986390835828,13.5017201056088,0.));
#251856=CARTESIAN_POINT('Ctrl Pts',(21.1986390835828,13.5017201056088,12.));
#251857=CARTESIAN_POINT('Ctrl Pts',(21.2244869429332,13.5045440957404,0.));
#251858=CARTESIAN_POINT('Ctrl Pts',(21.2244869429332,13.5045440957404,12.));
#251859=CARTESIAN_POINT('Ctrl Pts',(21.250418192743,13.5073159019452,0.));
#251860=CARTESIAN_POINT('Ctrl Pts',(21.250418192743,13.5073159019452,12.));
#251861=CARTESIAN_POINT('Ctrl Pts',(21.2764323924442,13.5100352209205,0.));
#251862=CARTESIAN_POINT('Ctrl Pts',(21.2764323924442,13.5100352209205,12.));
#251863=CARTESIAN_POINT('Ctrl Pts',(21.3025291054235,13.5127017534971,0.));
#251864=CARTESIAN_POINT('Ctrl Pts',(21.3025291054235,13.5127017534971,12.));
#251865=CARTESIAN_POINT('Ctrl Pts',(21.3287078996341,13.5153152050555,0.));
#251866=CARTESIAN_POINT('Ctrl Pts',(21.3287078996341,13.5153152050555,12.));
#251867=CARTESIAN_POINT('Ctrl Pts',(21.3549683486222,13.5178752862466,0.));
#251868=CARTESIAN_POINT('Ctrl Pts',(21.3549683486222,13.5178752862466,12.));
#251869=CARTESIAN_POINT('Ctrl Pts',(21.3813100304973,13.5203817122504,0.));
#251870=CARTESIAN_POINT('Ctrl Pts',(21.3813100304973,13.5203817122504,12.));
#251871=CARTESIAN_POINT('Ctrl Pts',(21.4077325259324,13.5228342013516,0.));
#251872=CARTESIAN_POINT('Ctrl Pts',(21.4077325259324,13.5228342013516,12.));
#251873=CARTESIAN_POINT('Ctrl Pts',(21.4342354165259,13.5252324737802,0.));
#251874=CARTESIAN_POINT('Ctrl Pts',(21.4342354165259,13.5252324737802,12.));
#251875=CARTESIAN_POINT('Ctrl Pts',(21.4608182828697,13.5275762503555,0.));
#251876=CARTESIAN_POINT('Ctrl Pts',(21.4608182828697,13.5275762503555,12.));
#251877=CARTESIAN_POINT('Ctrl Pts',(21.4874807030468,13.5298652514355,0.));
#251878=CARTESIAN_POINT('Ctrl Pts',(21.4874807030468,13.5298652514355,12.));
#251879=CARTESIAN_POINT('Ctrl Pts',(21.5142222501666,13.5320991952138,0.));
#251880=CARTESIAN_POINT('Ctrl Pts',(21.5142222501666,13.5320991952138,12.));
#251881=CARTESIAN_POINT('Ctrl Pts',(21.5410424932503,13.5342777983215,0.));
#251882=CARTESIAN_POINT('Ctrl Pts',(21.5410424932503,13.5342777983215,12.));
#251883=CARTESIAN_POINT('Ctrl Pts',(21.5679410019001,13.536400779028,0.));
#251884=CARTESIAN_POINT('Ctrl Pts',(21.5679410019001,13.536400779028,12.));
#251885=CARTESIAN_POINT('Ctrl Pts',(21.5949173499013,13.5384678597195,0.));
#251886=CARTESIAN_POINT('Ctrl Pts',(21.5949173499013,13.5384678597195,12.));
#251887=CARTESIAN_POINT('Ctrl Pts',(21.6219711193946,13.5404787697792,0.));
#251888=CARTESIAN_POINT('Ctrl Pts',(21.6219711193946,13.5404787697792,12.));
#251889=CARTESIAN_POINT('Ctrl Pts',(21.6491019044648,13.5424332480699,0.));
#251890=CARTESIAN_POINT('Ctrl Pts',(21.6491019044648,13.5424332480699,12.));
#251891=CARTESIAN_POINT('Ctrl Pts',(21.6763093157699,13.5443310461526,0.));
#251892=CARTESIAN_POINT('Ctrl Pts',(21.6763093157699,13.5443310461526,12.));
#251893=CARTESIAN_POINT('Ctrl Pts',(21.7035929822955,13.5461719295048,0.));
#251894=CARTESIAN_POINT('Ctrl Pts',(21.7035929822955,13.5461719295048,12.));
#251895=CARTESIAN_POINT('Ctrl Pts',(21.7309525412281,13.5479556704481,0.));
#251896=CARTESIAN_POINT('Ctrl Pts',(21.7309525412281,13.5479556704481,12.));
#251897=CARTESIAN_POINT('Ctrl Pts',(21.7583876294554,13.5496820422211,0.));
#251898=CARTESIAN_POINT('Ctrl Pts',(21.7583876294554,13.5496820422211,12.));
#251899=CARTESIAN_POINT('Ctrl Pts',(21.7858978745865,13.551350812725,0.));
#251900=CARTESIAN_POINT('Ctrl Pts',(21.7858978745865,13.551350812725,12.));
#251901=CARTESIAN_POINT('Ctrl Pts',(21.8134828857967,13.5529617381573,0.));
#251902=CARTESIAN_POINT('Ctrl Pts',(21.8134828857967,13.5529617381573,12.));
#251903=CARTESIAN_POINT('Ctrl Pts',(21.8411422456075,13.5545145573031,0.));
#251904=CARTESIAN_POINT('Ctrl Pts',(21.8411422456075,13.5545145573031,12.));
#251905=CARTESIAN_POINT('Ctrl Pts',(21.8688754989365,13.5560089839385,0.));
#251906=CARTESIAN_POINT('Ctrl Pts',(21.8688754989365,13.5560089839385,12.));
#251907=CARTESIAN_POINT('Ctrl Pts',(21.8966821688824,13.5574447178425,0.));
#251908=CARTESIAN_POINT('Ctrl Pts',(21.8966821688824,13.5574447178425,12.));
#251909=CARTESIAN_POINT('Ctrl Pts',(21.9245617765769,13.5588214586604,0.));
#251910=CARTESIAN_POINT('Ctrl Pts',(21.9245617765769,13.5588214586604,12.));
#251911=CARTESIAN_POINT('Ctrl Pts',(21.9525138592813,13.5601389185257,0.));
#251912=CARTESIAN_POINT('Ctrl Pts',(21.9525138592813,13.5601389185257,12.));
#251913=CARTESIAN_POINT('Ctrl Pts',(21.9805379899168,13.5613968357561,0.));
#251914=CARTESIAN_POINT('Ctrl Pts',(21.9805379899168,13.5613968357561,12.));
#251915=CARTESIAN_POINT('Ctrl Pts',(22.0086337943449,13.5625949868333,0.));
#251916=CARTESIAN_POINT('Ctrl Pts',(22.0086337943449,13.5625949868333,12.));
#251917=CARTESIAN_POINT('Ctrl Pts',(22.0368009736295,13.5637332022473,0.));
#251918=CARTESIAN_POINT('Ctrl Pts',(22.0368009736295,13.5637332022473,12.));
#251919=CARTESIAN_POINT('Ctrl Pts',(22.0650393089609,13.5648113689033,0.));
#251920=CARTESIAN_POINT('Ctrl Pts',(22.0650393089609,13.5648113689033,12.));
#251921=CARTESIAN_POINT('Ctrl Pts',(22.0933486464593,13.5658294169284,0.));
#251922=CARTESIAN_POINT('Ctrl Pts',(22.0933486464593,13.5658294169284,12.));
#251923=CARTESIAN_POINT('Ctrl Pts',(22.1217288871975,13.5667873105359,0.));
#251924=CARTESIAN_POINT('Ctrl Pts',(22.1217288871975,13.5667873105359,12.));
#251925=CARTESIAN_POINT('Ctrl Pts',(22.1444897575194,13.5675054919061,0.));
#251926=CARTESIAN_POINT('Ctrl Pts',(22.1444897575194,13.5675054919061,12.));
#251927=CARTESIAN_POINT('Ctrl Pts',(22.1615922805008,13.5680170531805,0.));
#251928=CARTESIAN_POINT('Ctrl Pts',(22.1615922805008,13.5680170531805,12.));
#251929=CARTESIAN_POINT('Ctrl Pts',(22.1730081264608,13.5683460612942,0.));
#251930=CARTESIAN_POINT('Ctrl Pts',(22.1730081264608,13.5683460612942,12.));
#251931=CARTESIAN_POINT('Ctrl Pts',(22.1787195904339,13.5685075571671,0.));
#251932=CARTESIAN_POINT('Ctrl Pts',(22.1787195904339,13.5685075571671,12.));
#251933=CARTESIAN_POINT('',(22.1787195904339,13.5685075571671,0.));
#251934=CARTESIAN_POINT('Ctrl Pts',(18.5896416359912,12.7689476255363,0.));
#251935=CARTESIAN_POINT('Ctrl Pts',(18.5896460962964,12.7689524524483,0.));
#251936=CARTESIAN_POINT('Ctrl Pts',(18.5896919669165,12.768986426692,0.));
#251937=CARTESIAN_POINT('Ctrl Pts',(18.589871621843,12.769110348199,0.));
#251938=CARTESIAN_POINT('Ctrl Pts',(18.5903328777227,12.7694215127919,0.));
#251939=CARTESIAN_POINT('Ctrl Pts',(18.5912775137806,12.7700520897173,0.));
#251940=CARTESIAN_POINT('Ctrl Pts',(18.5925859134579,12.7709195951156,0.));
#251941=CARTESIAN_POINT('Ctrl Pts',(18.5942490615407,12.7720142287172,0.));
#251942=CARTESIAN_POINT('Ctrl Pts',(18.5962551167772,12.7733231262108,0.));
#251943=CARTESIAN_POINT('Ctrl Pts',(18.598591752595,12.7748328937638,0.));
#251944=CARTESIAN_POINT('Ctrl Pts',(18.6012488486709,12.7765325225081,0.));
#251945=CARTESIAN_POINT('Ctrl Pts',(18.6042190183704,12.7784139605066,0.));
#251946=CARTESIAN_POINT('Ctrl Pts',(18.6074961535723,12.7804705387658,0.));
#251947=CARTESIAN_POINT('Ctrl Pts',(18.6110744826219,12.7826959526925,0.));
#251948=CARTESIAN_POINT('Ctrl Pts',(18.6149475565188,12.7850831657901,0.));
#251949=CARTESIAN_POINT('Ctrl Pts',(18.6191087624752,12.7876249657834,0.));
#251950=CARTESIAN_POINT('Ctrl Pts',(18.6235516265575,12.7903142925234,0.));
#251951=CARTESIAN_POINT('Ctrl Pts',(18.6282702819371,12.7931447451555,0.));
#251952=CARTESIAN_POINT('Ctrl Pts',(18.6332595057006,12.7961106222251,0.));
#251953=CARTESIAN_POINT('Ctrl Pts',(18.63851447924,12.7992066625264,0.));
#251954=CARTESIAN_POINT('Ctrl Pts',(18.6440306327456,12.8024278770153,0.));
#251955=CARTESIAN_POINT('Ctrl Pts',(18.6498034438987,12.805769331162,0.));
#251956=CARTESIAN_POINT('Ctrl Pts',(18.6558284825773,12.8092261933858,0.));
#251957=CARTESIAN_POINT('Ctrl Pts',(18.6621014624746,12.8127937909631,0.));
#251958=CARTESIAN_POINT('Ctrl Pts',(18.6686182952799,12.8164676687362,0.));
#251959=CARTESIAN_POINT('Ctrl Pts',(18.6753751301092,12.8202436318474,0.));
#251960=CARTESIAN_POINT('Ctrl Pts',(18.6823683094139,12.8241176980017,0.));
#251961=CARTESIAN_POINT('Ctrl Pts',(18.6895943376171,12.8280860635231,0.));
#251962=CARTESIAN_POINT('Ctrl Pts',(18.6970498410172,12.8321450599789,0.));
#251963=CARTESIAN_POINT('Ctrl Pts',(18.7047315436294,12.8362911280361,0.));
#251964=CARTESIAN_POINT('Ctrl Pts',(18.7126362754445,12.8405208263431,0.));
#251965=CARTESIAN_POINT('Ctrl Pts',(18.7207609737702,12.8448308329494,0.));
#251966=CARTESIAN_POINT('Ctrl Pts',(18.7291026886554,12.8492179511591,0.));
#251967=CARTESIAN_POINT('Ctrl Pts',(18.7376585820854,12.8536791086316,0.));
#251968=CARTESIAN_POINT('Ctrl Pts',(18.7464259171251,12.8582113455646,0.));
#251969=CARTESIAN_POINT('Ctrl Pts',(18.7554020493887,12.8628118054171,0.));
#251970=CARTESIAN_POINT('Ctrl Pts',(18.7645844169564,12.8674777239653,0.));
#251971=CARTESIAN_POINT('Ctrl Pts',(18.7739705329022,12.872206421181,0.));
#251972=CARTESIAN_POINT('Ctrl Pts',(18.7835579840477,12.8769952998095,0.));
#251973=CARTESIAN_POINT('Ctrl Pts',(18.7933444285868,12.8818418427475,0.));
#251974=CARTESIAN_POINT('Ctrl Pts',(18.8033275941943,12.8867436109546,0.));
#251975=CARTESIAN_POINT('Ctrl Pts',(18.813505275782,12.8916982409935,0.));
#251976=CARTESIAN_POINT('Ctrl Pts',(18.8238753319129,12.8967034410755,0.));
#251977=CARTESIAN_POINT('Ctrl Pts',(18.834435681259,12.9017569871738,0.));
#251978=CARTESIAN_POINT('Ctrl Pts',(18.8451842990984,12.9068567191854,0.));
#251979=CARTESIAN_POINT('Ctrl Pts',(18.8561192136198,12.9120005369063,0.));
#251980=CARTESIAN_POINT('Ctrl Pts',(18.8672385038326,12.9171863977045,0.));
#251981=CARTESIAN_POINT('Ctrl Pts',(18.8785402977527,12.9224123144982,0.));
#251982=CARTESIAN_POINT('Ctrl Pts',(18.8900227704889,12.9276763536373,0.));
#251983=CARTESIAN_POINT('Ctrl Pts',(18.9016841423403,12.9329766328185,0.));
#251984=CARTESIAN_POINT('Ctrl Pts',(18.9135226769465,12.9383113190375,0.));
#251985=CARTESIAN_POINT('Ctrl Pts',(18.9255366795195,12.9436786266105,0.));
#251986=CARTESIAN_POINT('Ctrl Pts',(18.9377244950435,12.9490768151821,0.));
#251987=CARTESIAN_POINT('Ctrl Pts',(18.9500845064715,12.9545041877377,0.));
#251988=CARTESIAN_POINT('Ctrl Pts',(18.9626151329229,12.9599590886319,0.));
#251989=CARTESIAN_POINT('Ctrl Pts',(18.9753148284475,12.9654399021869,0.));
#251990=CARTESIAN_POINT('Ctrl Pts',(18.9881820807585,12.9709450512747,0.));
#251991=CARTESIAN_POINT('Ctrl Pts',(19.0012154099791,12.9764729959205,0.));
#251992=CARTESIAN_POINT('Ctrl Pts',(19.0144133673348,12.9820222318716,0.));
#251993=CARTESIAN_POINT('Ctrl Pts',(19.0277745339908,12.9875912893003,0.));
#251994=CARTESIAN_POINT('Ctrl Pts',(19.0412975200398,12.9931787316515,0.));
#251995=CARTESIAN_POINT('Ctrl Pts',(19.0549809634355,12.9987831544502,0.));
#251996=CARTESIAN_POINT('Ctrl Pts',(19.0688235289437,13.0044031841381,0.));
#251997=CARTESIAN_POINT('Ctrl Pts',(19.0828239070482,13.0100374768786,0.));
#251998=CARTESIAN_POINT('Ctrl Pts',(19.0969808131226,13.0156847176094,0.));
#251999=CARTESIAN_POINT('Ctrl Pts',(19.1112929866308,13.0213436191326,0.));
#252000=CARTESIAN_POINT('Ctrl Pts',(19.1257591903099,13.0270129211976,0.));
#252001=CARTESIAN_POINT('Ctrl Pts',(19.1403782093389,13.0326913895841,0.));
#252002=CARTESIAN_POINT('Ctrl Pts',(19.1551488505233,13.0383778152072,0.));
#252003=CARTESIAN_POINT('Ctrl Pts',(19.1700699416625,13.0440710133775,0.));
#252004=CARTESIAN_POINT('Ctrl Pts',(19.1851403308825,13.0497698230442,0.));
#252005=CARTESIAN_POINT('Ctrl Pts',(19.2003588859771,13.0554731060537,0.));
#252006=CARTESIAN_POINT('Ctrl Pts',(19.2157244937141,13.0611797463913,0.));
#252007=CARTESIAN_POINT('Ctrl Pts',(19.2312360592031,13.0668886494791,0.));
#252008=CARTESIAN_POINT('Ctrl Pts',(19.2468925053988,13.0725987415856,0.));
#252009=CARTESIAN_POINT('Ctrl Pts',(19.2626927725596,13.0783089692118,0.));
#252010=CARTESIAN_POINT('Ctrl Pts',(19.2786358177198,13.0840182984949,0.));
#252011=CARTESIAN_POINT('Ctrl Pts',(19.2947206141246,13.089725714597,0.));
#252012=CARTESIAN_POINT('Ctrl Pts',(19.3109461507358,13.095430221148,0.));
#252013=CARTESIAN_POINT('Ctrl Pts',(19.3273114318268,13.1011308397592,0.));
#252014=CARTESIAN_POINT('Ctrl Pts',(19.3438154765395,13.1068266095186,0.));
#252015=CARTESIAN_POINT('Ctrl Pts',(19.3604573184516,13.1125165865021,0.));
#252016=CARTESIAN_POINT('Ctrl Pts',(19.3772360051093,13.118199843271,0.));
#252017=CARTESIAN_POINT('Ctrl Pts',(19.3941505976267,13.1238754684177,0.));
#252018=CARTESIAN_POINT('Ctrl Pts',(19.4112001703561,13.1295425661635,0.));
#252019=CARTESIAN_POINT('Ctrl Pts',(19.4283838105265,13.135200255944,0.));
#252020=CARTESIAN_POINT('Ctrl Pts',(19.4457006178875,13.140847672006,0.));
#252021=CARTESIAN_POINT('Ctrl Pts',(19.463149704325,13.1464839629966,0.));
#252022=CARTESIAN_POINT('Ctrl Pts',(19.4807301935256,13.1521082915846,0.));
#252023=CARTESIAN_POINT('Ctrl Pts',(19.498441220707,13.1577198341238,0.));
#252024=CARTESIAN_POINT('Ctrl Pts',(19.5162819323207,13.1633177803097,0.));
#252025=CARTESIAN_POINT('Ctrl Pts',(19.5342514857564,13.1689013328432,0.));
#252026=CARTESIAN_POINT('Ctrl Pts',(19.5523490490254,13.1744697070918,0.));
#252027=CARTESIAN_POINT('Ctrl Pts',(19.5705738004682,13.1800221307683,0.));
#252028=CARTESIAN_POINT('Ctrl Pts',(19.5889249285352,13.185557843648,0.));
#252029=CARTESIAN_POINT('Ctrl Pts',(19.6074016315421,13.1910760972818,0.));
#252030=CARTESIAN_POINT('Ctrl Pts',(19.6260031174244,13.196576154715,0.));
#252031=CARTESIAN_POINT('Ctrl Pts',(19.6447286034764,13.202057290206,0.));
#252032=CARTESIAN_POINT('Ctrl Pts',(19.6635773160924,13.2075187889522,0.));
#252033=CARTESIAN_POINT('Ctrl Pts',(19.6825484905812,13.2129599468478,0.));
#252034=CARTESIAN_POINT('Ctrl Pts',(19.7016413709678,13.2183800702431,0.));
#252035=CARTESIAN_POINT('Ctrl Pts',(19.7208552097867,13.2237784757065,0.));
#252036=CARTESIAN_POINT('Ctrl Pts',(19.7401892678701,13.2291544897902,0.));
#252037=CARTESIAN_POINT('Ctrl Pts',(19.7596428141176,13.2345074487968,0.));
#252038=CARTESIAN_POINT('Ctrl Pts',(19.7792151253297,13.239836698568,0.));
#252039=CARTESIAN_POINT('Ctrl Pts',(19.7989054860501,13.2451415942809,0.));
#252040=CARTESIAN_POINT('Ctrl Pts',(19.8187131883919,13.2504215002458,0.));
#252041=CARTESIAN_POINT('Ctrl Pts',(19.8386375318632,13.2556757897085,0.));
#252042=CARTESIAN_POINT('Ctrl Pts',(19.8586778231711,13.2609038446525,0.));
#252043=CARTESIAN_POINT('Ctrl Pts',(19.8788333760571,13.2661050556128,0.));
#252044=CARTESIAN_POINT('Ctrl Pts',(19.8991035111739,13.2712788215015,0.));
#252045=CARTESIAN_POINT('Ctrl Pts',(19.9194875559419,13.2764245494354,0.));
#252046=CARTESIAN_POINT('Ctrl Pts',(19.9399848444019,13.2815416545663,0.));
#252047=CARTESIAN_POINT('Ctrl Pts',(19.9605947170589,13.2866295599152,0.));
#252048=CARTESIAN_POINT('Ctrl Pts',(19.9813165207174,13.2916876962098,0.));
#252049=CARTESIAN_POINT('Ctrl Pts',(20.0021496083742,13.296715501731,0.));
#252050=CARTESIAN_POINT('Ctrl Pts',(20.0230933391039,13.3017124221639,0.));
#252051=CARTESIAN_POINT('Ctrl Pts',(20.0441470779345,13.3066779104515,0.));
#252052=CARTESIAN_POINT('Ctrl Pts',(20.0653101957188,13.3116114266514,0.));
#252053=CARTESIAN_POINT('Ctrl Pts',(20.0865820689883,13.3165124377963,0.));
#252054=CARTESIAN_POINT('Ctrl Pts',(20.1079620798377,13.3213804177588,0.));
#252055=CARTESIAN_POINT('Ctrl Pts',(20.1294496158405,13.3262148471228,0.));
#252056=CARTESIAN_POINT('Ctrl Pts',(20.1510440699477,13.3310152130565,0.));
#252057=CARTESIAN_POINT('Ctrl Pts',(20.1727448403818,13.3357810091903,0.));
#252058=CARTESIAN_POINT('Ctrl Pts',(20.1945513305233,13.3405117354969,0.));
#252059=CARTESIAN_POINT('Ctrl Pts',(20.2164629487855,13.3452068981763,0.));
#252060=CARTESIAN_POINT('Ctrl Pts',(20.2384791085354,13.3498660095382,0.));
#252061=CARTESIAN_POINT('Ctrl Pts',(20.2605992280117,13.3544885878886,0.));
#252062=CARTESIAN_POINT('Ctrl Pts',(20.2828227302337,13.3590741574194,0.));
#252063=CARTESIAN_POINT('Ctrl Pts',(20.3051490429049,13.3636222481017,0.));
#252064=CARTESIAN_POINT('Ctrl Pts',(20.3275775983032,13.3681323955828,0.));
#252065=CARTESIAN_POINT('Ctrl Pts',(20.3501078331818,13.372604141087,0.));
#252066=CARTESIAN_POINT('Ctrl Pts',(20.3727391887187,13.377037031319,0.));
#252067=CARTESIAN_POINT('Ctrl Pts',(20.3954711104504,13.3814306183721,0.));
#252068=CARTESIAN_POINT('Ctrl Pts',(20.4183030482002,13.3857844596387,0.));
#252069=CARTESIAN_POINT('Ctrl Pts',(20.4412344560007,13.3900981177254,0.));
#252070=CARTESIAN_POINT('Ctrl Pts',(20.4642647920038,13.3943711603739,0.));
#252071=CARTESIAN_POINT('Ctrl Pts',(20.4873935184041,13.3986031603716,0.));
#252072=CARTESIAN_POINT('Ctrl Pts',(20.5106201013755,13.4027936954529,0.));
#252073=CARTESIAN_POINT('Ctrl Pts',(20.5339440109957,13.4069423482077,0.));
#252074=CARTESIAN_POINT('Ctrl Pts',(20.557364721164,13.4110487059912,0.));
#252075=CARTESIAN_POINT('Ctrl Pts',(20.5808817095155,13.4151123608411,0.));
#252076=CARTESIAN_POINT('Ctrl Pts',(20.6044944573151,13.4191329093932,0.));
#252077=CARTESIAN_POINT('Ctrl Pts',(20.6282024494234,13.4231099528178,0.));
#252078=CARTESIAN_POINT('Ctrl Pts',(20.6520051742867,13.4270430967651,0.));
#252079=CARTESIAN_POINT('Ctrl Pts',(20.6759021239102,13.4309319513119,0.));
#252080=CARTESIAN_POINT('Ctrl Pts',(20.6998927938288,13.4347761309154,0.));
#252081=CARTESIAN_POINT('Ctrl Pts',(20.7239766830675,13.4385752543663,0.));
#252082=CARTESIAN_POINT('Ctrl Pts',(20.7481532941014,13.4423289447561,0.));
#252083=CARTESIAN_POINT('Ctrl Pts',(20.7724221327609,13.4460368293689,0.));
#252084=CARTESIAN_POINT('Ctrl Pts',(20.7967827081228,13.4496985395637,0.));
#252085=CARTESIAN_POINT('Ctrl Pts',(20.821234532398,13.4533137106667,0.));
#252086=CARTESIAN_POINT('Ctrl Pts',(20.8457771208083,13.4568819818631,0.));
#252087=CARTESIAN_POINT('Ctrl Pts',(20.8704099914641,13.4604029960983,0.));
#252088=CARTESIAN_POINT('Ctrl Pts',(20.8951326652158,13.4638763999725,0.));
#252089=CARTESIAN_POINT('Ctrl Pts',(20.9199446657583,13.4673018437717,0.));
#252090=CARTESIAN_POINT('Ctrl Pts',(20.9448455197557,13.4706789815166,0.));
#252091=CARTESIAN_POINT('Ctrl Pts',(20.9698347569477,13.4740074710086,0.));
#252092=CARTESIAN_POINT('Ctrl Pts',(20.9949119102592,13.4772869738879,0.));
#252093=CARTESIAN_POINT('Ctrl Pts',(21.0200765158884,13.4805171556822,0.));
#252094=CARTESIAN_POINT('Ctrl Pts',(21.0453281134245,13.4836976858912,0.));
#252095=CARTESIAN_POINT('Ctrl Pts',(21.0706662455199,13.4868282377191,0.));
#252096=CARTESIAN_POINT('Ctrl Pts',(21.0960904575046,13.4899084877717,0.));
#252097=CARTESIAN_POINT('Ctrl Pts',(21.1216002970207,13.4929381157778,0.));
#252098=CARTESIAN_POINT('Ctrl Pts',(21.1471953136209,13.4959168042934,0.));
#252099=CARTESIAN_POINT('Ctrl Pts',(21.1728750584175,13.4988442384491,0.));
#252100=CARTESIAN_POINT('Ctrl Pts',(21.1986390835828,13.5017201056088,0.));
#252101=CARTESIAN_POINT('Ctrl Pts',(21.2244869429332,13.5045440957404,0.));
#252102=CARTESIAN_POINT('Ctrl Pts',(21.250418192743,13.5073159019452,0.));
#252103=CARTESIAN_POINT('Ctrl Pts',(21.2764323924442,13.5100352209205,0.));
#252104=CARTESIAN_POINT('Ctrl Pts',(21.3025291054235,13.5127017534971,0.));
#252105=CARTESIAN_POINT('Ctrl Pts',(21.3287078996341,13.5153152050555,0.));
#252106=CARTESIAN_POINT('Ctrl Pts',(21.3549683486222,13.5178752862466,0.));
#252107=CARTESIAN_POINT('Ctrl Pts',(21.3813100304973,13.5203817122504,0.));
#252108=CARTESIAN_POINT('Ctrl Pts',(21.4077325259324,13.5228342013516,0.));
#252109=CARTESIAN_POINT('Ctrl Pts',(21.4342354165259,13.5252324737802,0.));
#252110=CARTESIAN_POINT('Ctrl Pts',(21.4608182828697,13.5275762503555,0.));
#252111=CARTESIAN_POINT('Ctrl Pts',(21.4874807030468,13.5298652514355,0.));
#252112=CARTESIAN_POINT('Ctrl Pts',(21.5142222501666,13.5320991952138,0.));
#252113=CARTESIAN_POINT('Ctrl Pts',(21.5410424932503,13.5342777983215,0.));
#252114=CARTESIAN_POINT('Ctrl Pts',(21.5679410019001,13.536400779028,0.));
#252115=CARTESIAN_POINT('Ctrl Pts',(21.5949173499013,13.5384678597195,0.));
#252116=CARTESIAN_POINT('Ctrl Pts',(21.6219711193946,13.5404787697792,0.));
#252117=CARTESIAN_POINT('Ctrl Pts',(21.6491019044648,13.5424332480699,0.));
#252118=CARTESIAN_POINT('Ctrl Pts',(21.6763093157699,13.5443310461526,0.));
#252119=CARTESIAN_POINT('Ctrl Pts',(21.7035929822955,13.5461719295048,0.));
#252120=CARTESIAN_POINT('Ctrl Pts',(21.7309525412281,13.5479556704481,0.));
#252121=CARTESIAN_POINT('Ctrl Pts',(21.7583876294554,13.5496820422211,0.));
#252122=CARTESIAN_POINT('Ctrl Pts',(21.7858978745865,13.551350812725,0.));
#252123=CARTESIAN_POINT('Ctrl Pts',(21.8134828857967,13.5529617381573,0.));
#252124=CARTESIAN_POINT('Ctrl Pts',(21.8411422456075,13.5545145573031,0.));
#252125=CARTESIAN_POINT('Ctrl Pts',(21.8688754989365,13.5560089839385,0.));
#252126=CARTESIAN_POINT('Ctrl Pts',(21.8966821688824,13.5574447178425,0.));
#252127=CARTESIAN_POINT('Ctrl Pts',(21.9245617765769,13.5588214586604,0.));
#252128=CARTESIAN_POINT('Ctrl Pts',(21.9525138592813,13.5601389185257,0.));
#252129=CARTESIAN_POINT('Ctrl Pts',(21.9805379899168,13.5613968357561,0.));
#252130=CARTESIAN_POINT('Ctrl Pts',(22.0086337943449,13.5625949868333,0.));
#252131=CARTESIAN_POINT('Ctrl Pts',(22.0368009736295,13.5637332022473,0.));
#252132=CARTESIAN_POINT('Ctrl Pts',(22.0650393089609,13.5648113689033,0.));
#252133=CARTESIAN_POINT('Ctrl Pts',(22.0933486464593,13.5658294169284,0.));
#252134=CARTESIAN_POINT('Ctrl Pts',(22.1217288871975,13.5667873105359,0.));
#252135=CARTESIAN_POINT('Ctrl Pts',(22.1444897575194,13.5675054919061,0.));
#252136=CARTESIAN_POINT('Ctrl Pts',(22.1615922805008,13.5680170531805,0.));
#252137=CARTESIAN_POINT('Ctrl Pts',(22.1730081264608,13.5683460612942,0.));
#252138=CARTESIAN_POINT('Ctrl Pts',(22.1787195904339,13.5685075571671,0.));
#252139=CARTESIAN_POINT('',(22.1787195904339,13.5685075571671,12.));
#252140=CARTESIAN_POINT('Ctrl Pts',(22.1787195904339,13.5685075571671,12.));
#252141=CARTESIAN_POINT('Ctrl Pts',(22.1730081264608,13.5683460612942,12.));
#252142=CARTESIAN_POINT('Ctrl Pts',(22.1615922805008,13.5680170531805,12.));
#252143=CARTESIAN_POINT('Ctrl Pts',(22.1444897575194,13.5675054919061,12.));
#252144=CARTESIAN_POINT('Ctrl Pts',(22.1217288871975,13.5667873105359,12.));
#252145=CARTESIAN_POINT('Ctrl Pts',(22.0933486464593,13.5658294169284,12.));
#252146=CARTESIAN_POINT('Ctrl Pts',(22.0650393089609,13.5648113689033,12.));
#252147=CARTESIAN_POINT('Ctrl Pts',(22.0368009736295,13.5637332022473,12.));
#252148=CARTESIAN_POINT('Ctrl Pts',(22.0086337943449,13.5625949868333,12.));
#252149=CARTESIAN_POINT('Ctrl Pts',(21.9805379899168,13.5613968357561,12.));
#252150=CARTESIAN_POINT('Ctrl Pts',(21.9525138592813,13.5601389185257,12.));
#252151=CARTESIAN_POINT('Ctrl Pts',(21.9245617765769,13.5588214586604,12.));
#252152=CARTESIAN_POINT('Ctrl Pts',(21.8966821688824,13.5574447178425,12.));
#252153=CARTESIAN_POINT('Ctrl Pts',(21.8688754989365,13.5560089839385,12.));
#252154=CARTESIAN_POINT('Ctrl Pts',(21.8411422456075,13.5545145573031,12.));
#252155=CARTESIAN_POINT('Ctrl Pts',(21.8134828857967,13.5529617381573,12.));
#252156=CARTESIAN_POINT('Ctrl Pts',(21.7858978745865,13.551350812725,12.));
#252157=CARTESIAN_POINT('Ctrl Pts',(21.7583876294554,13.5496820422211,12.));
#252158=CARTESIAN_POINT('Ctrl Pts',(21.7309525412281,13.5479556704481,12.));
#252159=CARTESIAN_POINT('Ctrl Pts',(21.7035929822955,13.5461719295048,12.));
#252160=CARTESIAN_POINT('Ctrl Pts',(21.6763093157699,13.5443310461526,12.));
#252161=CARTESIAN_POINT('Ctrl Pts',(21.6491019044648,13.5424332480699,12.));
#252162=CARTESIAN_POINT('Ctrl Pts',(21.6219711193946,13.5404787697792,12.));
#252163=CARTESIAN_POINT('Ctrl Pts',(21.5949173499013,13.5384678597195,12.));
#252164=CARTESIAN_POINT('Ctrl Pts',(21.5679410019001,13.536400779028,12.));
#252165=CARTESIAN_POINT('Ctrl Pts',(21.5410424932503,13.5342777983215,12.));
#252166=CARTESIAN_POINT('Ctrl Pts',(21.5142222501666,13.5320991952138,12.));
#252167=CARTESIAN_POINT('Ctrl Pts',(21.4874807030468,13.5298652514355,12.));
#252168=CARTESIAN_POINT('Ctrl Pts',(21.4608182828697,13.5275762503555,12.));
#252169=CARTESIAN_POINT('Ctrl Pts',(21.4342354165259,13.5252324737802,12.));
#252170=CARTESIAN_POINT('Ctrl Pts',(21.4077325259324,13.5228342013516,12.));
#252171=CARTESIAN_POINT('Ctrl Pts',(21.3813100304973,13.5203817122504,12.));
#252172=CARTESIAN_POINT('Ctrl Pts',(21.3549683486222,13.5178752862466,12.));
#252173=CARTESIAN_POINT('Ctrl Pts',(21.3287078996341,13.5153152050555,12.));
#252174=CARTESIAN_POINT('Ctrl Pts',(21.3025291054235,13.5127017534971,12.));
#252175=CARTESIAN_POINT('Ctrl Pts',(21.2764323924442,13.5100352209205,12.));
#252176=CARTESIAN_POINT('Ctrl Pts',(21.250418192743,13.5073159019452,12.));
#252177=CARTESIAN_POINT('Ctrl Pts',(21.2244869429332,13.5045440957404,12.));
#252178=CARTESIAN_POINT('Ctrl Pts',(21.1986390835828,13.5017201056088,12.));
#252179=CARTESIAN_POINT('Ctrl Pts',(21.1728750584175,13.4988442384491,12.));
#252180=CARTESIAN_POINT('Ctrl Pts',(21.1471953136209,13.4959168042934,12.));
#252181=CARTESIAN_POINT('Ctrl Pts',(21.1216002970207,13.4929381157778,12.));
#252182=CARTESIAN_POINT('Ctrl Pts',(21.0960904575046,13.4899084877717,12.));
#252183=CARTESIAN_POINT('Ctrl Pts',(21.0706662455199,13.4868282377191,12.));
#252184=CARTESIAN_POINT('Ctrl Pts',(21.0453281134245,13.4836976858912,12.));
#252185=CARTESIAN_POINT('Ctrl Pts',(21.0200765158884,13.4805171556822,12.));
#252186=CARTESIAN_POINT('Ctrl Pts',(20.9949119102592,13.4772869738879,12.));
#252187=CARTESIAN_POINT('Ctrl Pts',(20.9698347569477,13.4740074710086,12.));
#252188=CARTESIAN_POINT('Ctrl Pts',(20.9448455197557,13.4706789815166,12.));
#252189=CARTESIAN_POINT('Ctrl Pts',(20.9199446657583,13.4673018437717,12.));
#252190=CARTESIAN_POINT('Ctrl Pts',(20.8951326652158,13.4638763999725,12.));
#252191=CARTESIAN_POINT('Ctrl Pts',(20.8704099914641,13.4604029960983,12.));
#252192=CARTESIAN_POINT('Ctrl Pts',(20.8457771208083,13.4568819818631,12.));
#252193=CARTESIAN_POINT('Ctrl Pts',(20.821234532398,13.4533137106667,12.));
#252194=CARTESIAN_POINT('Ctrl Pts',(20.7967827081228,13.4496985395637,12.));
#252195=CARTESIAN_POINT('Ctrl Pts',(20.7724221327609,13.4460368293689,12.));
#252196=CARTESIAN_POINT('Ctrl Pts',(20.7481532941014,13.4423289447561,12.));
#252197=CARTESIAN_POINT('Ctrl Pts',(20.7239766830675,13.4385752543663,12.));
#252198=CARTESIAN_POINT('Ctrl Pts',(20.6998927938288,13.4347761309154,12.));
#252199=CARTESIAN_POINT('Ctrl Pts',(20.6759021239102,13.4309319513119,12.));
#252200=CARTESIAN_POINT('Ctrl Pts',(20.6520051742867,13.4270430967651,12.));
#252201=CARTESIAN_POINT('Ctrl Pts',(20.6282024494234,13.4231099528178,12.));
#252202=CARTESIAN_POINT('Ctrl Pts',(20.6044944573151,13.4191329093932,12.));
#252203=CARTESIAN_POINT('Ctrl Pts',(20.5808817095155,13.4151123608411,12.));
#252204=CARTESIAN_POINT('Ctrl Pts',(20.557364721164,13.4110487059912,12.));
#252205=CARTESIAN_POINT('Ctrl Pts',(20.5339440109957,13.4069423482077,12.));
#252206=CARTESIAN_POINT('Ctrl Pts',(20.5106201013755,13.4027936954529,12.));
#252207=CARTESIAN_POINT('Ctrl Pts',(20.4873935184041,13.3986031603716,12.));
#252208=CARTESIAN_POINT('Ctrl Pts',(20.4642647920038,13.3943711603739,12.));
#252209=CARTESIAN_POINT('Ctrl Pts',(20.4412344560007,13.3900981177254,12.));
#252210=CARTESIAN_POINT('Ctrl Pts',(20.4183030482002,13.3857844596387,12.));
#252211=CARTESIAN_POINT('Ctrl Pts',(20.3954711104504,13.3814306183721,12.));
#252212=CARTESIAN_POINT('Ctrl Pts',(20.3727391887187,13.377037031319,12.));
#252213=CARTESIAN_POINT('Ctrl Pts',(20.3501078331818,13.372604141087,12.));
#252214=CARTESIAN_POINT('Ctrl Pts',(20.3275775983032,13.3681323955828,12.));
#252215=CARTESIAN_POINT('Ctrl Pts',(20.3051490429049,13.3636222481017,12.));
#252216=CARTESIAN_POINT('Ctrl Pts',(20.2828227302337,13.3590741574194,12.));
#252217=CARTESIAN_POINT('Ctrl Pts',(20.2605992280117,13.3544885878886,12.));
#252218=CARTESIAN_POINT('Ctrl Pts',(20.2384791085354,13.3498660095382,12.));
#252219=CARTESIAN_POINT('Ctrl Pts',(20.2164629487855,13.3452068981763,12.));
#252220=CARTESIAN_POINT('Ctrl Pts',(20.1945513305233,13.3405117354969,12.));
#252221=CARTESIAN_POINT('Ctrl Pts',(20.1727448403818,13.3357810091903,12.));
#252222=CARTESIAN_POINT('Ctrl Pts',(20.1510440699477,13.3310152130565,12.));
#252223=CARTESIAN_POINT('Ctrl Pts',(20.1294496158405,13.3262148471228,12.));
#252224=CARTESIAN_POINT('Ctrl Pts',(20.1079620798377,13.3213804177588,12.));
#252225=CARTESIAN_POINT('Ctrl Pts',(20.0865820689883,13.3165124377963,12.));
#252226=CARTESIAN_POINT('Ctrl Pts',(20.0653101957188,13.3116114266514,12.));
#252227=CARTESIAN_POINT('Ctrl Pts',(20.0441470779345,13.3066779104515,12.));
#252228=CARTESIAN_POINT('Ctrl Pts',(20.0230933391039,13.3017124221639,12.));
#252229=CARTESIAN_POINT('Ctrl Pts',(20.0021496083742,13.296715501731,12.));
#252230=CARTESIAN_POINT('Ctrl Pts',(19.9813165207174,13.2916876962098,12.));
#252231=CARTESIAN_POINT('Ctrl Pts',(19.9605947170589,13.2866295599152,12.));
#252232=CARTESIAN_POINT('Ctrl Pts',(19.9399848444019,13.2815416545663,12.));
#252233=CARTESIAN_POINT('Ctrl Pts',(19.9194875559419,13.2764245494354,12.));
#252234=CARTESIAN_POINT('Ctrl Pts',(19.8991035111739,13.2712788215015,12.));
#252235=CARTESIAN_POINT('Ctrl Pts',(19.8788333760571,13.2661050556128,12.));
#252236=CARTESIAN_POINT('Ctrl Pts',(19.8586778231711,13.2609038446525,12.));
#252237=CARTESIAN_POINT('Ctrl Pts',(19.8386375318632,13.2556757897085,12.));
#252238=CARTESIAN_POINT('Ctrl Pts',(19.8187131883919,13.2504215002458,12.));
#252239=CARTESIAN_POINT('Ctrl Pts',(19.7989054860501,13.2451415942809,12.));
#252240=CARTESIAN_POINT('Ctrl Pts',(19.7792151253297,13.239836698568,12.));
#252241=CARTESIAN_POINT('Ctrl Pts',(19.7596428141176,13.2345074487968,12.));
#252242=CARTESIAN_POINT('Ctrl Pts',(19.7401892678701,13.2291544897902,12.));
#252243=CARTESIAN_POINT('Ctrl Pts',(19.7208552097867,13.2237784757065,12.));
#252244=CARTESIAN_POINT('Ctrl Pts',(19.7016413709678,13.2183800702431,12.));
#252245=CARTESIAN_POINT('Ctrl Pts',(19.6825484905812,13.2129599468478,12.));
#252246=CARTESIAN_POINT('Ctrl Pts',(19.6635773160924,13.2075187889522,12.));
#252247=CARTESIAN_POINT('Ctrl Pts',(19.6447286034764,13.202057290206,12.));
#252248=CARTESIAN_POINT('Ctrl Pts',(19.6260031174244,13.196576154715,12.));
#252249=CARTESIAN_POINT('Ctrl Pts',(19.6074016315421,13.1910760972818,12.));
#252250=CARTESIAN_POINT('Ctrl Pts',(19.5889249285352,13.185557843648,12.));
#252251=CARTESIAN_POINT('Ctrl Pts',(19.5705738004682,13.1800221307683,12.));
#252252=CARTESIAN_POINT('Ctrl Pts',(19.5523490490254,13.1744697070918,12.));
#252253=CARTESIAN_POINT('Ctrl Pts',(19.5342514857564,13.1689013328432,12.));
#252254=CARTESIAN_POINT('Ctrl Pts',(19.5162819323207,13.1633177803097,12.));
#252255=CARTESIAN_POINT('Ctrl Pts',(19.498441220707,13.1577198341238,12.));
#252256=CARTESIAN_POINT('Ctrl Pts',(19.4807301935256,13.1521082915846,12.));
#252257=CARTESIAN_POINT('Ctrl Pts',(19.463149704325,13.1464839629966,12.));
#252258=CARTESIAN_POINT('Ctrl Pts',(19.4457006178875,13.140847672006,12.));
#252259=CARTESIAN_POINT('Ctrl Pts',(19.4283838105265,13.135200255944,12.));
#252260=CARTESIAN_POINT('Ctrl Pts',(19.4112001703561,13.1295425661635,12.));
#252261=CARTESIAN_POINT('Ctrl Pts',(19.3941505976267,13.1238754684177,12.));
#252262=CARTESIAN_POINT('Ctrl Pts',(19.3772360051093,13.118199843271,12.));
#252263=CARTESIAN_POINT('Ctrl Pts',(19.3604573184516,13.1125165865021,12.));
#252264=CARTESIAN_POINT('Ctrl Pts',(19.3438154765395,13.1068266095186,12.));
#252265=CARTESIAN_POINT('Ctrl Pts',(19.3273114318268,13.1011308397592,12.));
#252266=CARTESIAN_POINT('Ctrl Pts',(19.3109461507358,13.095430221148,12.));
#252267=CARTESIAN_POINT('Ctrl Pts',(19.2947206141246,13.089725714597,12.));
#252268=CARTESIAN_POINT('Ctrl Pts',(19.2786358177198,13.0840182984949,12.));
#252269=CARTESIAN_POINT('Ctrl Pts',(19.2626927725596,13.0783089692118,12.));
#252270=CARTESIAN_POINT('Ctrl Pts',(19.2468925053988,13.0725987415856,12.));
#252271=CARTESIAN_POINT('Ctrl Pts',(19.2312360592031,13.0668886494791,12.));
#252272=CARTESIAN_POINT('Ctrl Pts',(19.2157244937141,13.0611797463913,12.));
#252273=CARTESIAN_POINT('Ctrl Pts',(19.2003588859771,13.0554731060537,12.));
#252274=CARTESIAN_POINT('Ctrl Pts',(19.1851403308825,13.0497698230442,12.));
#252275=CARTESIAN_POINT('Ctrl Pts',(19.1700699416625,13.0440710133775,12.));
#252276=CARTESIAN_POINT('Ctrl Pts',(19.1551488505233,13.0383778152072,12.));
#252277=CARTESIAN_POINT('Ctrl Pts',(19.1403782093389,13.0326913895841,12.));
#252278=CARTESIAN_POINT('Ctrl Pts',(19.1257591903099,13.0270129211976,12.));
#252279=CARTESIAN_POINT('Ctrl Pts',(19.1112929866308,13.0213436191326,12.));
#252280=CARTESIAN_POINT('Ctrl Pts',(19.0969808131226,13.0156847176094,12.));
#252281=CARTESIAN_POINT('Ctrl Pts',(19.0828239070482,13.0100374768786,12.));
#252282=CARTESIAN_POINT('Ctrl Pts',(19.0688235289437,13.0044031841381,12.));
#252283=CARTESIAN_POINT('Ctrl Pts',(19.0549809634355,12.9987831544502,12.));
#252284=CARTESIAN_POINT('Ctrl Pts',(19.0412975200398,12.9931787316515,12.));
#252285=CARTESIAN_POINT('Ctrl Pts',(19.0277745339908,12.9875912893003,12.));
#252286=CARTESIAN_POINT('Ctrl Pts',(19.0144133673348,12.9820222318716,12.));
#252287=CARTESIAN_POINT('Ctrl Pts',(19.0012154099791,12.9764729959205,12.));
#252288=CARTESIAN_POINT('Ctrl Pts',(18.9881820807585,12.9709450512747,12.));
#252289=CARTESIAN_POINT('Ctrl Pts',(18.9753148284475,12.9654399021869,12.));
#252290=CARTESIAN_POINT('Ctrl Pts',(18.9626151329229,12.9599590886319,12.));
#252291=CARTESIAN_POINT('Ctrl Pts',(18.9500845064715,12.9545041877377,12.));
#252292=CARTESIAN_POINT('Ctrl Pts',(18.9377244950435,12.9490768151821,12.));
#252293=CARTESIAN_POINT('Ctrl Pts',(18.9255366795195,12.9436786266105,12.));
#252294=CARTESIAN_POINT('Ctrl Pts',(18.9135226769465,12.9383113190375,12.));
#252295=CARTESIAN_POINT('Ctrl Pts',(18.9016841423403,12.9329766328185,12.));
#252296=CARTESIAN_POINT('Ctrl Pts',(18.8900227704889,12.9276763536373,12.));
#252297=CARTESIAN_POINT('Ctrl Pts',(18.8785402977527,12.9224123144982,12.));
#252298=CARTESIAN_POINT('Ctrl Pts',(18.8672385038326,12.9171863977045,12.));
#252299=CARTESIAN_POINT('Ctrl Pts',(18.8561192136198,12.9120005369063,12.));
#252300=CARTESIAN_POINT('Ctrl Pts',(18.8451842990984,12.9068567191854,12.));
#252301=CARTESIAN_POINT('Ctrl Pts',(18.834435681259,12.9017569871738,12.));
#252302=CARTESIAN_POINT('Ctrl Pts',(18.8238753319129,12.8967034410755,12.));
#252303=CARTESIAN_POINT('Ctrl Pts',(18.813505275782,12.8916982409935,12.));
#252304=CARTESIAN_POINT('Ctrl Pts',(18.8033275941943,12.8867436109546,12.));
#252305=CARTESIAN_POINT('Ctrl Pts',(18.7933444285868,12.8818418427475,12.));
#252306=CARTESIAN_POINT('Ctrl Pts',(18.7835579840477,12.8769952998095,12.));
#252307=CARTESIAN_POINT('Ctrl Pts',(18.7739705329022,12.872206421181,12.));
#252308=CARTESIAN_POINT('Ctrl Pts',(18.7645844169564,12.8674777239653,12.));
#252309=CARTESIAN_POINT('Ctrl Pts',(18.7554020493887,12.8628118054171,12.));
#252310=CARTESIAN_POINT('Ctrl Pts',(18.7464259171251,12.8582113455646,12.));
#252311=CARTESIAN_POINT('Ctrl Pts',(18.7376585820854,12.8536791086316,12.));
#252312=CARTESIAN_POINT('Ctrl Pts',(18.7291026886554,12.8492179511591,12.));
#252313=CARTESIAN_POINT('Ctrl Pts',(18.7207609737702,12.8448308329494,12.));
#252314=CARTESIAN_POINT('Ctrl Pts',(18.7126362754445,12.8405208263431,12.));
#252315=CARTESIAN_POINT('Ctrl Pts',(18.7047315436294,12.8362911280361,12.));
#252316=CARTESIAN_POINT('Ctrl Pts',(18.6970498410172,12.8321450599789,12.));
#252317=CARTESIAN_POINT('Ctrl Pts',(18.6895943376171,12.8280860635231,12.));
#252318=CARTESIAN_POINT('Ctrl Pts',(18.6823683094139,12.8241176980017,12.));
#252319=CARTESIAN_POINT('Ctrl Pts',(18.6753751301092,12.8202436318474,12.));
#252320=CARTESIAN_POINT('Ctrl Pts',(18.6686182952799,12.8164676687362,12.));
#252321=CARTESIAN_POINT('Ctrl Pts',(18.6621014624746,12.8127937909631,12.));
#252322=CARTESIAN_POINT('Ctrl Pts',(18.6558284825773,12.8092261933858,12.));
#252323=CARTESIAN_POINT('Ctrl Pts',(18.6498034438987,12.805769331162,12.));
#252324=CARTESIAN_POINT('Ctrl Pts',(18.6440306327456,12.8024278770153,12.));
#252325=CARTESIAN_POINT('Ctrl Pts',(18.63851447924,12.7992066625264,12.));
#252326=CARTESIAN_POINT('Ctrl Pts',(18.6332595057006,12.7961106222251,12.));
#252327=CARTESIAN_POINT('Ctrl Pts',(18.6282702819371,12.7931447451555,12.));
#252328=CARTESIAN_POINT('Ctrl Pts',(18.6235516265575,12.7903142925234,12.));
#252329=CARTESIAN_POINT('Ctrl Pts',(18.6191087624752,12.7876249657834,12.));
#252330=CARTESIAN_POINT('Ctrl Pts',(18.6149475565188,12.7850831657901,12.));
#252331=CARTESIAN_POINT('Ctrl Pts',(18.6110744826219,12.7826959526925,12.));
#252332=CARTESIAN_POINT('Ctrl Pts',(18.6074961535723,12.7804705387658,12.));
#252333=CARTESIAN_POINT('Ctrl Pts',(18.6042190183704,12.7784139605066,12.));
#252334=CARTESIAN_POINT('Ctrl Pts',(18.6012488486709,12.7765325225081,12.));
#252335=CARTESIAN_POINT('Ctrl Pts',(18.598591752595,12.7748328937638,12.));
#252336=CARTESIAN_POINT('Ctrl Pts',(18.5962551167772,12.7733231262108,12.));
#252337=CARTESIAN_POINT('Ctrl Pts',(18.5942490615407,12.7720142287172,12.));
#252338=CARTESIAN_POINT('Ctrl Pts',(18.5925859134579,12.7709195951156,12.));
#252339=CARTESIAN_POINT('Ctrl Pts',(18.5912775137806,12.7700520897173,12.));
#252340=CARTESIAN_POINT('Ctrl Pts',(18.5903328777227,12.7694215127919,12.));
#252341=CARTESIAN_POINT('Ctrl Pts',(18.589871621843,12.769110348199,12.));
#252342=CARTESIAN_POINT('Ctrl Pts',(18.5896919669165,12.768986426692,12.));
#252343=CARTESIAN_POINT('Ctrl Pts',(18.5896460962964,12.7689524524483,12.));
#252344=CARTESIAN_POINT('Ctrl Pts',(18.5896416359912,12.7689476255363,12.));
#252345=CARTESIAN_POINT('',(22.1787195904339,13.5685075571671,0.));
#252346=CARTESIAN_POINT('Origin',(20.2687213152502,7.17139709155223,0.));
#252347=CARTESIAN_POINT('',(21.2610617890679,7.52250298901264,12.));
#252348=CARTESIAN_POINT('',(10.1343606576251,3.58569854577611,12.));
#252349=CARTESIAN_POINT('',(21.2610617890679,7.52250298901264,0.));
#252350=CARTESIAN_POINT('',(21.2610617890679,7.52250298901264,0.));
#252351=CARTESIAN_POINT('',(10.1343606576251,3.58569854577611,0.));
#252352=CARTESIAN_POINT('Ctrl Pts',(22.8400320311648,12.4230808101438,0.));
#252353=CARTESIAN_POINT('Ctrl Pts',(22.8400320311648,12.4230808101438,12.));
#252354=CARTESIAN_POINT('Ctrl Pts',(22.8370364396459,12.418215285186,0.));
#252355=CARTESIAN_POINT('Ctrl Pts',(22.8370364396459,12.418215285186,12.));
#252356=CARTESIAN_POINT('Ctrl Pts',(22.8310435872747,12.4084933766347,0.));
#252357=CARTESIAN_POINT('Ctrl Pts',(22.8310435872747,12.4084933766347,12.));
#252358=CARTESIAN_POINT('Ctrl Pts',(22.8220493007173,12.3939379378998,0.));
#252359=CARTESIAN_POINT('Ctrl Pts',(22.8220493007173,12.3939379378998,12.));
#252360=CARTESIAN_POINT('Ctrl Pts',(22.81004690224,12.374585536673,0.));
#252361=CARTESIAN_POINT('Ctrl Pts',(22.81004690224,12.374585536673,12.));
#252362=CARTESIAN_POINT('Ctrl Pts',(22.795027221673,12.3504864740319,0.));
#252363=CARTESIAN_POINT('Ctrl Pts',(22.795027221673,12.3504864740319,12.));
#252364=CARTESIAN_POINT('Ctrl Pts',(22.7799908974768,12.3264788926075,0.));
#252365=CARTESIAN_POINT('Ctrl Pts',(22.7799908974768,12.3264788926075,12.));
#252366=CARTESIAN_POINT('Ctrl Pts',(22.764938010105,12.3025628601792,0.));
#252367=CARTESIAN_POINT('Ctrl Pts',(22.764938010105,12.3025628601792,12.));
#252368=CARTESIAN_POINT('Ctrl Pts',(22.7498686970069,12.2787384750742,0.));
#252369=CARTESIAN_POINT('Ctrl Pts',(22.7498686970069,12.2787384750742,12.));
#252370=CARTESIAN_POINT('Ctrl Pts',(22.7347831655287,12.2550058702395,0.));
#252371=CARTESIAN_POINT('Ctrl Pts',(22.7347831655287,12.2550058702395,12.));
#252372=CARTESIAN_POINT('Ctrl Pts',(22.7196817119374,12.2313652198061,0.));
#252373=CARTESIAN_POINT('Ctrl Pts',(22.7196817119374,12.2313652198061,12.));
#252374=CARTESIAN_POINT('Ctrl Pts',(22.7045647168747,12.2078167360284,0.));
#252375=CARTESIAN_POINT('Ctrl Pts',(22.7045647168747,12.2078167360284,12.));
#252376=CARTESIAN_POINT('Ctrl Pts',(22.6894326205037,12.1843606579262,0.));
#252377=CARTESIAN_POINT('Ctrl Pts',(22.6894326205037,12.1843606579262,12.));
#252378=CARTESIAN_POINT('Ctrl Pts',(22.6742859034944,12.1609972423099,0.));
#252379=CARTESIAN_POINT('Ctrl Pts',(22.6742859034944,12.1609972423099,12.));
#252380=CARTESIAN_POINT('Ctrl Pts',(22.6591250653965,12.1377267537145,0.));
#252381=CARTESIAN_POINT('Ctrl Pts',(22.6591250653965,12.1377267537145,12.));
#252382=CARTESIAN_POINT('Ctrl Pts',(22.6439506046605,12.1145494550383,0.));
#252383=CARTESIAN_POINT('Ctrl Pts',(22.6439506046605,12.1145494550383,12.));
#252384=CARTESIAN_POINT('Ctrl Pts',(22.6287629967056,12.0914655972823,0.));
#252385=CARTESIAN_POINT('Ctrl Pts',(22.6287629967056,12.0914655972823,12.));
#252386=CARTESIAN_POINT('Ctrl Pts',(22.6135626764898,12.0684754113862,0.));
#252387=CARTESIAN_POINT('Ctrl Pts',(22.6135626764898,12.0684754113862,12.));
#252388=CARTESIAN_POINT('Ctrl Pts',(22.5983500505644,12.0455791139128,0.));
#252389=CARTESIAN_POINT('Ctrl Pts',(22.5983500505644,12.0455791139128,12.));
#252390=CARTESIAN_POINT('Ctrl Pts',(22.5831255061282,12.0227769113127,0.));
#252391=CARTESIAN_POINT('Ctrl Pts',(22.5831255061282,12.0227769113127,12.));
#252392=CARTESIAN_POINT('Ctrl Pts',(22.5678894211181,12.0000690046695,0.));
#252393=CARTESIAN_POINT('Ctrl Pts',(22.5678894211181,12.0000690046695,12.));
#252394=CARTESIAN_POINT('Ctrl Pts',(22.5526421741158,11.9774555943496,0.));
#252395=CARTESIAN_POINT('Ctrl Pts',(22.5526421741158,11.9774555943496,12.));
#252396=CARTESIAN_POINT('Ctrl Pts',(22.5373841537307,11.9549368843997,0.));
#252397=CARTESIAN_POINT('Ctrl Pts',(22.5373841537307,11.9549368843997,12.));
#252398=CARTESIAN_POINT('Ctrl Pts',(22.5221157697883,11.9325130877803,0.));
#252399=CARTESIAN_POINT('Ctrl Pts',(22.5221157697883,11.9325130877803,12.));
#252400=CARTESIAN_POINT('Ctrl Pts',(22.5068374513973,11.9101844254557,0.));
#252401=CARTESIAN_POINT('Ctrl Pts',(22.5068374513973,11.9101844254557,12.));
#252402=CARTESIAN_POINT('Ctrl Pts',(22.4915496418485,11.8879511239943,0.));
#252403=CARTESIAN_POINT('Ctrl Pts',(22.4915496418485,11.8879511239943,12.));
#252404=CARTESIAN_POINT('Ctrl Pts',(22.4762527946702,11.8658134137019,0.));
#252405=CARTESIAN_POINT('Ctrl Pts',(22.4762527946702,11.8658134137019,12.));
#252406=CARTESIAN_POINT('Ctrl Pts',(22.4609473690471,11.8437715264487,0.));
#252407=CARTESIAN_POINT('Ctrl Pts',(22.4609473690471,11.8437715264487,12.));
#252408=CARTESIAN_POINT('Ctrl Pts',(22.4456338258735,11.8218256937889,0.));
#252409=CARTESIAN_POINT('Ctrl Pts',(22.4456338258735,11.8218256937889,12.));
#252410=CARTESIAN_POINT('Ctrl Pts',(22.430312622646,11.7999761445173,0.));
#252411=CARTESIAN_POINT('Ctrl Pts',(22.430312622646,11.7999761445173,12.));
#252412=CARTESIAN_POINT('Ctrl Pts',(22.4149842125008,11.7782231042039,0.));
#252413=CARTESIAN_POINT('Ctrl Pts',(22.4149842125008,11.7782231042039,12.));
#252414=CARTESIAN_POINT('Ctrl Pts',(22.3996490469191,11.7565667964764,0.));
#252415=CARTESIAN_POINT('Ctrl Pts',(22.3996490469191,11.7565667964764,12.));
#252416=CARTESIAN_POINT('Ctrl Pts',(22.3843075773899,11.7350074437961,0.));
#252417=CARTESIAN_POINT('Ctrl Pts',(22.3843075773899,11.7350074437961,12.));
#252418=CARTESIAN_POINT('Ctrl Pts',(22.3689602575491,11.7135452684532,0.));
#252419=CARTESIAN_POINT('Ctrl Pts',(22.3689602575491,11.7135452684532,12.));
#252420=CARTESIAN_POINT('Ctrl Pts',(22.3536075450029,11.6921804934056,0.));
#252421=CARTESIAN_POINT('Ctrl Pts',(22.3536075450029,11.6921804934056,12.));
#252422=CARTESIAN_POINT('Ctrl Pts',(22.3382499035619,11.6709133432985,0.));
#252423=CARTESIAN_POINT('Ctrl Pts',(22.3382499035619,11.6709133432985,12.));
#252424=CARTESIAN_POINT('Ctrl Pts',(22.3228878043976,11.6497440449857,0.));
#252425=CARTESIAN_POINT('Ctrl Pts',(22.3228878043976,11.6497440449857,12.));
#252426=CARTESIAN_POINT('Ctrl Pts',(22.3075217249049,11.6286728270009,0.));
#252427=CARTESIAN_POINT('Ctrl Pts',(22.3075217249049,11.6286728270009,12.));
#252428=CARTESIAN_POINT('Ctrl Pts',(22.2921521480356,11.6076999192357,0.));
#252429=CARTESIAN_POINT('Ctrl Pts',(22.2921521480356,11.6076999192357,12.));
#252430=CARTESIAN_POINT('Ctrl Pts',(22.2767795614348,11.5868255525188,0.));
#252431=CARTESIAN_POINT('Ctrl Pts',(22.2767795614348,11.5868255525188,12.));
#252432=CARTESIAN_POINT('Ctrl Pts',(22.2614044566898,11.5660499582403,0.));
#252433=CARTESIAN_POINT('Ctrl Pts',(22.2614044566898,11.5660499582403,12.));
#252434=CARTESIAN_POINT('Ctrl Pts',(22.2460273284654,11.5453733679121,0.));
#252435=CARTESIAN_POINT('Ctrl Pts',(22.2460273284654,11.5453733679121,12.));
#252436=CARTESIAN_POINT('Ctrl Pts',(22.2306486738901,11.5247960128477,0.));
#252437=CARTESIAN_POINT('Ctrl Pts',(22.2306486738901,11.5247960128477,12.));
#252438=CARTESIAN_POINT('Ctrl Pts',(22.2152689931022,11.5043181244242,0.));
#252439=CARTESIAN_POINT('Ctrl Pts',(22.2152689931022,11.5043181244242,12.));
#252440=CARTESIAN_POINT('Ctrl Pts',(22.1998887896436,11.483939934259,0.));
#252441=CARTESIAN_POINT('Ctrl Pts',(22.1998887896436,11.483939934259,12.));
#252442=CARTESIAN_POINT('Ctrl Pts',(22.184508570917,11.463661674411,0.));
#252443=CARTESIAN_POINT('Ctrl Pts',(22.184508570917,11.463661674411,12.));
#252444=CARTESIAN_POINT('Ctrl Pts',(22.1691288486096,11.443483577557,0.));
#252445=CARTESIAN_POINT('Ctrl Pts',(22.1691288486096,11.443483577557,12.));
#252446=CARTESIAN_POINT('Ctrl Pts',(22.1537501391487,11.4234058771742,0.));
#252447=CARTESIAN_POINT('Ctrl Pts',(22.1537501391487,11.4234058771742,12.));
#252448=CARTESIAN_POINT('Ctrl Pts',(22.1383729640964,11.4034288076908,0.));
#252449=CARTESIAN_POINT('Ctrl Pts',(22.1383729640964,11.4034288076908,12.));
#252450=CARTESIAN_POINT('Ctrl Pts',(22.1229978500186,11.3835526044256,0.));
#252451=CARTESIAN_POINT('Ctrl Pts',(22.1229978500186,11.3835526044256,12.));
#252452=CARTESIAN_POINT('Ctrl Pts',(22.1076253283979,11.3637775035367,0.));
#252453=CARTESIAN_POINT('Ctrl Pts',(22.1076253283979,11.3637775035367,12.));
#252454=CARTESIAN_POINT('Ctrl Pts',(22.0922559355294,11.3441037419553,0.));
#252455=CARTESIAN_POINT('Ctrl Pts',(22.0922559355294,11.3441037419553,12.));
#252456=CARTESIAN_POINT('Ctrl Pts',(22.0768902124267,11.3245315573168,0.));
#252457=CARTESIAN_POINT('Ctrl Pts',(22.0768902124267,11.3245315573168,12.));
#252458=CARTESIAN_POINT('Ctrl Pts',(22.0615287047179,11.3050611878771,0.));
#252459=CARTESIAN_POINT('Ctrl Pts',(22.0615287047179,11.3050611878771,12.));
#252460=CARTESIAN_POINT('Ctrl Pts',(22.046171962566,11.2856928724374,0.));
#252461=CARTESIAN_POINT('Ctrl Pts',(22.046171962566,11.2856928724374,12.));
#252462=CARTESIAN_POINT('Ctrl Pts',(22.030820540835,11.2664268504206,0.));
#252463=CARTESIAN_POINT('Ctrl Pts',(22.030820540835,11.2664268504206,12.));
#252464=CARTESIAN_POINT('Ctrl Pts',(22.0154749992363,11.2472633619275,0.));
#252465=CARTESIAN_POINT('Ctrl Pts',(22.0154749992363,11.2472633619275,12.));
#252466=CARTESIAN_POINT('Ctrl Pts',(22.0001359024839,11.2282026477896,0.));
#252467=CARTESIAN_POINT('Ctrl Pts',(22.0001359024839,11.2282026477896,12.));
#252468=CARTESIAN_POINT('Ctrl Pts',(21.9848038204439,11.2092449496125,0.));
#252469=CARTESIAN_POINT('Ctrl Pts',(21.9848038204439,11.2092449496125,12.));
#252470=CARTESIAN_POINT('Ctrl Pts',(21.9694793282914,11.190390509811,0.));
#252471=CARTESIAN_POINT('Ctrl Pts',(21.9694793282914,11.190390509811,12.));
#252472=CARTESIAN_POINT('Ctrl Pts',(21.9541630066506,11.1716395716376,0.));
#252473=CARTESIAN_POINT('Ctrl Pts',(21.9541630066506,11.1716395716376,12.));
#252474=CARTESIAN_POINT('Ctrl Pts',(21.9388554416439,11.1529923792003,0.));
#252475=CARTESIAN_POINT('Ctrl Pts',(21.9388554416439,11.1529923792003,12.));
#252476=CARTESIAN_POINT('Ctrl Pts',(21.923557224952,11.1344491774741,0.));
#252477=CARTESIAN_POINT('Ctrl Pts',(21.923557224952,11.1344491774741,12.));
#252478=CARTESIAN_POINT('Ctrl Pts',(21.9082689538688,11.1160102123024,0.));
#252479=CARTESIAN_POINT('Ctrl Pts',(21.9082689538688,11.1160102123024,12.));
#252480=CARTESIAN_POINT('Ctrl Pts',(21.8929912313608,11.0976757303944,0.));
#252481=CARTESIAN_POINT('Ctrl Pts',(21.8929912313608,11.0976757303944,12.));
#252482=CARTESIAN_POINT('Ctrl Pts',(21.877724666119,11.0794459793057,0.));
#252483=CARTESIAN_POINT('Ctrl Pts',(21.877724666119,11.0794459793057,12.));
#252484=CARTESIAN_POINT('Ctrl Pts',(21.8624698726318,11.0613212074363,0.));
#252485=CARTESIAN_POINT('Ctrl Pts',(21.8624698726318,11.0613212074363,12.));
#252486=CARTESIAN_POINT('Ctrl Pts',(21.8472274713103,11.0433016640807,0.));
#252487=CARTESIAN_POINT('Ctrl Pts',(21.8472274713103,11.0433016640807,12.));
#252488=CARTESIAN_POINT('Ctrl Pts',(21.8319980886033,11.0253875994598,0.));
#252489=CARTESIAN_POINT('Ctrl Pts',(21.8319980886033,11.0253875994598,12.));
#252490=CARTESIAN_POINT('Ctrl Pts',(21.8167823571168,11.0075792647477,0.));
#252491=CARTESIAN_POINT('Ctrl Pts',(21.8167823571168,11.0075792647477,12.));
#252492=CARTESIAN_POINT('Ctrl Pts',(21.8015809157301,10.9898769120912,0.));
#252493=CARTESIAN_POINT('Ctrl Pts',(21.8015809157301,10.9898769120912,12.));
#252494=CARTESIAN_POINT('Ctrl Pts',(21.7863944097141,10.9722807946156,0.));
#252495=CARTESIAN_POINT('Ctrl Pts',(21.7863944097141,10.9722807946156,12.));
#252496=CARTESIAN_POINT('Ctrl Pts',(21.7712234908464,10.9547911664455,0.));
#252497=CARTESIAN_POINT('Ctrl Pts',(21.7712234908464,10.9547911664455,12.));
#252498=CARTESIAN_POINT('Ctrl Pts',(21.7560688175247,10.9374082827444,0.));
#252499=CARTESIAN_POINT('Ctrl Pts',(21.7560688175247,10.9374082827444,12.));
#252500=CARTESIAN_POINT('Ctrl Pts',(21.7409310548797,10.9201323997384,0.));
#252501=CARTESIAN_POINT('Ctrl Pts',(21.7409310548797,10.9201323997384,12.));
#252502=CARTESIAN_POINT('Ctrl Pts',(21.7258108748873,10.902963774734,0.));
#252503=CARTESIAN_POINT('Ctrl Pts',(21.7258108748873,10.902963774734,12.));
#252504=CARTESIAN_POINT('Ctrl Pts',(21.7107089564825,10.8859026661293,0.));
#252505=CARTESIAN_POINT('Ctrl Pts',(21.7107089564825,10.8859026661293,12.));
#252506=CARTESIAN_POINT('Ctrl Pts',(21.6956259856672,10.8689493334095,0.));
#252507=CARTESIAN_POINT('Ctrl Pts',(21.6956259856672,10.8689493334095,12.));
#252508=CARTESIAN_POINT('Ctrl Pts',(21.6805626556467,10.8521040371835,0.));
#252509=CARTESIAN_POINT('Ctrl Pts',(21.6805626556467,10.8521040371835,12.));
#252510=CARTESIAN_POINT('Ctrl Pts',(21.6655196669732,10.8353670392272,0.));
#252511=CARTESIAN_POINT('Ctrl Pts',(21.6655196669732,10.8353670392272,12.));
#252512=CARTESIAN_POINT('Ctrl Pts',(21.6504977276866,10.8187386025136,0.));
#252513=CARTESIAN_POINT('Ctrl Pts',(21.6504977276866,10.8187386025136,12.));
#252514=CARTESIAN_POINT('Ctrl Pts',(21.6354975534557,10.8022189912369,0.));
#252515=CARTESIAN_POINT('Ctrl Pts',(21.6354975534557,10.8022189912369,12.));
#252516=CARTESIAN_POINT('Ctrl Pts',(21.6205198677173,10.7858084708261,0.));
#252517=CARTESIAN_POINT('Ctrl Pts',(21.6205198677173,10.7858084708261,12.));
#252518=CARTESIAN_POINT('Ctrl Pts',(21.6055654018176,10.7695073079552,0.));
#252519=CARTESIAN_POINT('Ctrl Pts',(21.6055654018176,10.7695073079552,12.));
#252520=CARTESIAN_POINT('Ctrl Pts',(21.5906348951743,10.7533157705941,0.));
#252521=CARTESIAN_POINT('Ctrl Pts',(21.5906348951743,10.7533157705941,12.));
#252522=CARTESIAN_POINT('Ctrl Pts',(21.5757290954371,10.7372341280467,0.));
#252523=CARTESIAN_POINT('Ctrl Pts',(21.5757290954371,10.7372341280467,12.));
#252524=CARTESIAN_POINT('Ctrl Pts',(21.5608487586468,10.7212626509816,0.));
#252525=CARTESIAN_POINT('Ctrl Pts',(21.5608487586468,10.7212626509816,12.));
#252526=CARTESIAN_POINT('Ctrl Pts',(21.5459946493955,10.7054016114571,0.));
#252527=CARTESIAN_POINT('Ctrl Pts',(21.5459946493955,10.7054016114571,12.));
#252528=CARTESIAN_POINT('Ctrl Pts',(21.5311675409807,10.689651282929,0.));
#252529=CARTESIAN_POINT('Ctrl Pts',(21.5311675409807,10.689651282929,12.));
#252530=CARTESIAN_POINT('Ctrl Pts',(21.51636821558,10.6740119402834,0.));
#252531=CARTESIAN_POINT('Ctrl Pts',(21.51636821558,10.6740119402834,12.));
#252532=CARTESIAN_POINT('Ctrl Pts',(21.5015974644449,10.6584838598939,0.));
#252533=CARTESIAN_POINT('Ctrl Pts',(21.5015974644449,10.6584838598939,12.));
#252534=CARTESIAN_POINT('Ctrl Pts',(21.4868560880889,10.6430673196607,0.));
#252535=CARTESIAN_POINT('Ctrl Pts',(21.4868560880889,10.6430673196607,12.));
#252536=CARTESIAN_POINT('Ctrl Pts',(21.4721448964766,10.6277625990456,0.));
#252537=CARTESIAN_POINT('Ctrl Pts',(21.4721448964766,10.6277625990456,12.));
#252538=CARTESIAN_POINT('Ctrl Pts',(21.4574647092097,10.6125699790961,0.));
#252539=CARTESIAN_POINT('Ctrl Pts',(21.4574647092097,10.6125699790961,12.));
#252540=CARTESIAN_POINT('Ctrl Pts',(21.4428163557144,10.5974897424622,0.));
#252541=CARTESIAN_POINT('Ctrl Pts',(21.4428163557144,10.5974897424622,12.));
#252542=CARTESIAN_POINT('Ctrl Pts',(21.4282006754631,10.5825221734573,0.));
#252543=CARTESIAN_POINT('Ctrl Pts',(21.4282006754631,10.5825221734573,12.));
#252544=CARTESIAN_POINT('Ctrl Pts',(21.4136185181979,10.5676675581108,0.));
#252545=CARTESIAN_POINT('Ctrl Pts',(21.4136185181979,10.5676675581108,12.));
#252546=CARTESIAN_POINT('Ctrl Pts',(21.3990707441497,10.5529261842108,0.));
#252547=CARTESIAN_POINT('Ctrl Pts',(21.3990707441497,10.5529261842108,12.));
#252548=CARTESIAN_POINT('Ctrl Pts',(21.3845582242602,10.5382983413421,0.));
#252549=CARTESIAN_POINT('Ctrl Pts',(21.3845582242602,10.5382983413421,12.));
#252550=CARTESIAN_POINT('Ctrl Pts',(21.3700818403936,10.5237843209057,0.));
#252551=CARTESIAN_POINT('Ctrl Pts',(21.3700818403936,10.5237843209057,12.));
#252552=CARTESIAN_POINT('Ctrl Pts',(21.3556424855814,10.5093844161685,0.));
#252553=CARTESIAN_POINT('Ctrl Pts',(21.3556424855814,10.5093844161685,12.));
#252554=CARTESIAN_POINT('Ctrl Pts',(21.3412410642904,10.4950989223337,0.));
#252555=CARTESIAN_POINT('Ctrl Pts',(21.3412410642904,10.4950989223337,12.));
#252556=CARTESIAN_POINT('Ctrl Pts',(21.3268784926819,10.4809281365931,0.));
#252557=CARTESIAN_POINT('Ctrl Pts',(21.3268784926819,10.4809281365931,12.));
#252558=CARTESIAN_POINT('Ctrl Pts',(21.3125556988731,10.4668723581768,0.));
#252559=CARTESIAN_POINT('Ctrl Pts',(21.3125556988731,10.4668723581768,12.));
#252560=CARTESIAN_POINT('Ctrl Pts',(21.2982736231931,10.4529318883874,0.));
#252561=CARTESIAN_POINT('Ctrl Pts',(21.2982736231931,10.4529318883874,12.));
#252562=CARTESIAN_POINT('Ctrl Pts',(21.2840332184483,10.4391070306391,0.));
#252563=CARTESIAN_POINT('Ctrl Pts',(21.2840332184483,10.4391070306391,12.));
#252564=CARTESIAN_POINT('Ctrl Pts',(21.2698354502403,10.42539809054,0.));
#252565=CARTESIAN_POINT('Ctrl Pts',(21.2698354502403,10.42539809054,12.));
#252566=CARTESIAN_POINT('Ctrl Pts',(21.255681297275,10.4118053759588,0.));
#252567=CARTESIAN_POINT('Ctrl Pts',(21.255681297275,10.4118053759588,12.));
#252568=CARTESIAN_POINT('Ctrl Pts',(21.2415717516714,10.3983291970846,0.));
#252569=CARTESIAN_POINT('Ctrl Pts',(21.2415717516714,10.3983291970846,12.));
#252570=CARTESIAN_POINT('Ctrl Pts',(21.22750781927,10.3849698664786,0.));
#252571=CARTESIAN_POINT('Ctrl Pts',(21.22750781927,10.3849698664786,12.));
#252572=CARTESIAN_POINT('Ctrl Pts',(21.2134905199345,10.371727699113,0.));
#252573=CARTESIAN_POINT('Ctrl Pts',(21.2134905199345,10.371727699113,12.));
#252574=CARTESIAN_POINT('Ctrl Pts',(21.199520887919,10.3586030124587,0.));
#252575=CARTESIAN_POINT('Ctrl Pts',(21.199520887919,10.3586030124587,12.));
#252576=CARTESIAN_POINT('Ctrl Pts',(21.1855999722416,10.3455961265701,0.));
#252577=CARTESIAN_POINT('Ctrl Pts',(21.1855999722416,10.3455961265701,12.));
#252578=CARTESIAN_POINT('Ctrl Pts',(21.1717288370509,10.3327073641572,0.));
#252579=CARTESIAN_POINT('Ctrl Pts',(21.1717288370509,10.3327073641572,12.));
#252580=CARTESIAN_POINT('Ctrl Pts',(21.1579085619965,10.3199370506544,0.));
#252581=CARTESIAN_POINT('Ctrl Pts',(21.1579085619965,10.3199370506544,12.));
#252582=CARTESIAN_POINT('Ctrl Pts',(21.1441402425843,10.3072855142687,0.));
#252583=CARTESIAN_POINT('Ctrl Pts',(21.1441402425843,10.3072855142687,12.));
#252584=CARTESIAN_POINT('Ctrl Pts',(21.1304249906002,10.2947530860721,0.));
#252585=CARTESIAN_POINT('Ctrl Pts',(21.1304249906002,10.2947530860721,12.));
#252586=CARTESIAN_POINT('Ctrl Pts',(21.1167639345631,10.2823401001072,0.));
#252587=CARTESIAN_POINT('Ctrl Pts',(21.1167639345631,10.2823401001072,12.));
#252588=CARTESIAN_POINT('Ctrl Pts',(21.1031582201627,10.2700468934744,0.));
#252589=CARTESIAN_POINT('Ctrl Pts',(21.1031582201627,10.2700468934744,12.));
#252590=CARTESIAN_POINT('Ctrl Pts',(21.0896090107063,10.2578738064181,0.));
#252591=CARTESIAN_POINT('Ctrl Pts',(21.0896090107063,10.2578738064181,12.));
#252592=CARTESIAN_POINT('Ctrl Pts',(21.0761174875444,10.2458211823912,0.));
#252593=CARTESIAN_POINT('Ctrl Pts',(21.0761174875444,10.2458211823912,12.));
#252594=CARTESIAN_POINT('Ctrl Pts',(21.0626848505663,10.2338893681567,0.));
#252595=CARTESIAN_POINT('Ctrl Pts',(21.0626848505663,10.2338893681567,12.));
#252596=CARTESIAN_POINT('Ctrl Pts',(21.0493123187483,10.2220787139155,0.));
#252597=CARTESIAN_POINT('Ctrl Pts',(21.0493123187483,10.2220787139155,12.));
#252598=CARTESIAN_POINT('Ctrl Pts',(21.0360011306815,10.2103895734123,0.));
#252599=CARTESIAN_POINT('Ctrl Pts',(21.0360011306815,10.2103895734123,12.));
#252600=CARTESIAN_POINT('Ctrl Pts',(21.0227525451107,10.1988223040425,0.));
#252601=CARTESIAN_POINT('Ctrl Pts',(21.0227525451107,10.1988223040425,12.));
#252602=CARTESIAN_POINT('Ctrl Pts',(21.0095678414486,10.187377266936,0.));
#252603=CARTESIAN_POINT('Ctrl Pts',(21.0095678414486,10.187377266936,12.));
#252604=CARTESIAN_POINT('Ctrl Pts',(20.9964483203686,10.1760548270767,0.));
#252605=CARTESIAN_POINT('Ctrl Pts',(20.9964483203686,10.1760548270767,12.));
#252606=CARTESIAN_POINT('Ctrl Pts',(20.9833953044736,10.1648553534568,0.));
#252607=CARTESIAN_POINT('Ctrl Pts',(20.9833953044736,10.1648553534568,12.));
#252608=CARTESIAN_POINT('Ctrl Pts',(20.9704101389369,10.1537792192065,0.));
#252609=CARTESIAN_POINT('Ctrl Pts',(20.9704101389369,10.1537792192065,12.));
#252610=CARTESIAN_POINT('Ctrl Pts',(20.9574941921591,10.1428268017256,0.));
#252611=CARTESIAN_POINT('Ctrl Pts',(20.9574941921591,10.1428268017256,12.));
#252612=CARTESIAN_POINT('Ctrl Pts',(20.9446488563933,10.1319984827908,0.));
#252613=CARTESIAN_POINT('Ctrl Pts',(20.9446488563933,10.1319984827908,12.));
#252614=CARTESIAN_POINT('Ctrl Pts',(20.9318755484734,10.1212946487057,0.));
#252615=CARTESIAN_POINT('Ctrl Pts',(20.9318755484734,10.1212946487057,12.));
#252616=CARTESIAN_POINT('Ctrl Pts',(20.919175710627,10.1107156904836,0.));
#252617=CARTESIAN_POINT('Ctrl Pts',(20.919175710627,10.1107156904836,12.));
#252618=CARTESIAN_POINT('Ctrl Pts',(20.9065508112557,10.1002620040076,0.));
#252619=CARTESIAN_POINT('Ctrl Pts',(20.9065508112557,10.1002620040076,12.));
#252620=CARTESIAN_POINT('Ctrl Pts',(20.894002345737,10.0899339901916,0.));
#252621=CARTESIAN_POINT('Ctrl Pts',(20.894002345737,10.0899339901916,12.));
#252622=CARTESIAN_POINT('Ctrl Pts',(20.881531837184,10.0797320551154,0.));
#252623=CARTESIAN_POINT('Ctrl Pts',(20.881531837184,10.0797320551154,12.));
#252624=CARTESIAN_POINT('Ctrl Pts',(20.86914083737,10.0696566102218,0.));
#252625=CARTESIAN_POINT('Ctrl Pts',(20.86914083737,10.0696566102218,12.));
#252626=CARTESIAN_POINT('Ctrl Pts',(20.8568309277316,10.0597080725375,0.));
#252627=CARTESIAN_POINT('Ctrl Pts',(20.8568309277316,10.0597080725375,12.));
#252628=CARTESIAN_POINT('Ctrl Pts',(20.8446037203402,10.0498868648733,0.));
#252629=CARTESIAN_POINT('Ctrl Pts',(20.8446037203402,10.0498868648733,12.));
#252630=CARTESIAN_POINT('Ctrl Pts',(20.8324608588909,10.0401934160234,0.));
#252631=CARTESIAN_POINT('Ctrl Pts',(20.8324608588909,10.0401934160234,12.));
#252632=CARTESIAN_POINT('Ctrl Pts',(20.8204040196602,10.0306281609435,0.));
#252633=CARTESIAN_POINT('Ctrl Pts',(20.8204040196602,10.0306281609435,12.));
#252634=CARTESIAN_POINT('Ctrl Pts',(20.8084349126888,10.0211915410095,0.));
#252635=CARTESIAN_POINT('Ctrl Pts',(20.8084349126888,10.0211915410095,12.));
#252636=CARTESIAN_POINT('Ctrl Pts',(20.7965552829908,10.0118840042786,0.));
#252637=CARTESIAN_POINT('Ctrl Pts',(20.7965552829908,10.0118840042786,12.));
#252638=CARTESIAN_POINT('Ctrl Pts',(20.7847669117568,10.0027060057389,0.));
#252639=CARTESIAN_POINT('Ctrl Pts',(20.7847669117568,10.0027060057389,12.));
#252640=CARTESIAN_POINT('Ctrl Pts',(20.7730716175417,9.9936580075464,0.));
#252641=CARTESIAN_POINT('Ctrl Pts',(20.7730716175417,9.9936580075464,12.));
#252642=CARTESIAN_POINT('Ctrl Pts',(20.761471257499,9.98474047926853,0.));
#252643=CARTESIAN_POINT('Ctrl Pts',(20.761471257499,9.98474047926853,12.));
#252644=CARTESIAN_POINT('Ctrl Pts',(20.7499677289627,9.9759538982347,0.));
#252645=CARTESIAN_POINT('Ctrl Pts',(20.7499677289627,9.9759538982347,12.));
#252646=CARTESIAN_POINT('Ctrl Pts',(20.7385629709795,9.96729874986202,0.));
#252647=CARTESIAN_POINT('Ctrl Pts',(20.7385629709795,9.96729874986202,12.));
#252648=CARTESIAN_POINT('Ctrl Pts',(20.7272589658751,9.95877552798398,0.));
#252649=CARTESIAN_POINT('Ctrl Pts',(20.7272589658751,9.95877552798398,12.));
#252650=CARTESIAN_POINT('Ctrl Pts',(20.7160577407579,9.95038473514949,0.));
#252651=CARTESIAN_POINT('Ctrl Pts',(20.7160577407579,9.95038473514949,12.));
#252652=CARTESIAN_POINT('Ctrl Pts',(20.7049613692234,9.94212688298236,0.));
#252653=CARTESIAN_POINT('Ctrl Pts',(20.7049613692234,9.94212688298236,12.));
#252654=CARTESIAN_POINT('Ctrl Pts',(20.6939719732484,9.9340024925973,0.));
#252655=CARTESIAN_POINT('Ctrl Pts',(20.6939719732484,9.9340024925973,12.));
#252656=CARTESIAN_POINT('Ctrl Pts',(20.6830917250255,9.92601209498749,0.));
#252657=CARTESIAN_POINT('Ctrl Pts',(20.6830917250255,9.92601209498749,12.));
#252658=CARTESIAN_POINT('Ctrl Pts',(20.6723228488263,9.91815623141289,0.));
#252659=CARTESIAN_POINT('Ctrl Pts',(20.6723228488263,9.91815623141289,12.));
#252660=CARTESIAN_POINT('Ctrl Pts',(20.6616676228315,9.91043545377008,0.));
#252661=CARTESIAN_POINT('Ctrl Pts',(20.6616676228315,9.91043545377008,12.));
#252662=CARTESIAN_POINT('Ctrl Pts',(20.6511283817414,9.90285032516693,0.));
#252663=CARTESIAN_POINT('Ctrl Pts',(20.6511283817414,9.90285032516693,12.));
#252664=CARTESIAN_POINT('Ctrl Pts',(20.6407075193976,9.8954014204912,0.));
#252665=CARTESIAN_POINT('Ctrl Pts',(20.6407075193976,9.8954014204912,12.));
#252666=CARTESIAN_POINT('Ctrl Pts',(20.6304074914087,9.88808932697306,0.));
#252667=CARTESIAN_POINT('Ctrl Pts',(20.6304074914087,9.88808932697306,12.));
#252668=CARTESIAN_POINT('Ctrl Pts',(20.6202308177474,9.88091464472676,0.));
#252669=CARTESIAN_POINT('Ctrl Pts',(20.6202308177474,9.88091464472676,12.));
#252670=CARTESIAN_POINT('Ctrl Pts',(20.6101800854494,9.87387798732956,0.));
#252671=CARTESIAN_POINT('Ctrl Pts',(20.6101800854494,9.87387798732956,12.));
#252672=CARTESIAN_POINT('Ctrl Pts',(20.6002579513699,9.86697998242623,0.));
#252673=CARTESIAN_POINT('Ctrl Pts',(20.6002579513699,9.86697998242623,12.));
#252674=CARTESIAN_POINT('Ctrl Pts',(20.5904671449754,9.86022127232748,0.));
#252675=CARTESIAN_POINT('Ctrl Pts',(20.5904671449754,9.86022127232748,12.));
#252676=CARTESIAN_POINT('Ctrl Pts',(20.5808104710015,9.85360251456981,0.));
#252677=CARTESIAN_POINT('Ctrl Pts',(20.5808104710015,9.85360251456981,12.));
#252678=CARTESIAN_POINT('Ctrl Pts',(20.5712908125139,9.84712438256278,0.));
#252679=CARTESIAN_POINT('Ctrl Pts',(20.5712908125139,9.84712438256278,12.));
#252680=CARTESIAN_POINT('Ctrl Pts',(20.5619111362402,9.84078756677565,0.));
#252681=CARTESIAN_POINT('Ctrl Pts',(20.5619111362402,9.84078756677565,12.));
#252682=CARTESIAN_POINT('Ctrl Pts',(20.552674497646,9.83459277585315,0.));
#252683=CARTESIAN_POINT('Ctrl Pts',(20.552674497646,9.83459277585315,12.));
#252684=CARTESIAN_POINT('Ctrl Pts',(20.5435840460721,9.82854073773878,0.));
#252685=CARTESIAN_POINT('Ctrl Pts',(20.5435840460721,9.82854073773878,12.));
#252686=CARTESIAN_POINT('Ctrl Pts',(20.5346430299517,9.82263220080363,0.));
#252687=CARTESIAN_POINT('Ctrl Pts',(20.5346430299517,9.82263220080363,12.));
#252688=CARTESIAN_POINT('Ctrl Pts',(20.5258548000629,9.81686793455943,0.));
#252689=CARTESIAN_POINT('Ctrl Pts',(20.5258548000629,9.81686793455943,12.));
#252690=CARTESIAN_POINT('Ctrl Pts',(20.517222812284,9.81124873025282,0.));
#252691=CARTESIAN_POINT('Ctrl Pts',(20.517222812284,9.81124873025282,12.));
#252692=CARTESIAN_POINT('Ctrl Pts',(20.5087506310505,9.80577540161088,0.));
#252693=CARTESIAN_POINT('Ctrl Pts',(20.5087506310505,9.80577540161088,12.));
#252694=CARTESIAN_POINT('Ctrl Pts',(20.5004419312107,9.80044878520949,0.));
#252695=CARTESIAN_POINT('Ctrl Pts',(20.5004419312107,9.80044878520949,12.));
#252696=CARTESIAN_POINT('Ctrl Pts',(20.4923005087943,9.79526974288331,0.));
#252697=CARTESIAN_POINT('Ctrl Pts',(20.4923005087943,9.79526974288331,12.));
#252698=CARTESIAN_POINT('Ctrl Pts',(20.4843302955329,9.79023916498656,0.));
#252699=CARTESIAN_POINT('Ctrl Pts',(20.4843302955329,9.79023916498656,12.));
#252700=CARTESIAN_POINT('Ctrl Pts',(20.4765353711586,9.78535797314167,0.));
#252701=CARTESIAN_POINT('Ctrl Pts',(20.4765353711586,9.78535797314167,12.));
#252702=CARTESIAN_POINT('Ctrl Pts',(20.4689199790669,9.78062712373321,0.));
#252703=CARTESIAN_POINT('Ctrl Pts',(20.4689199790669,9.78062712373321,12.));
#252704=CARTESIAN_POINT('Ctrl Pts',(20.4614885274975,9.77604760815529,0.));
#252705=CARTESIAN_POINT('Ctrl Pts',(20.4614885274975,9.77604760815529,12.));
#252706=CARTESIAN_POINT('Ctrl Pts',(20.4542455817527,9.7716204510407,0.));
#252707=CARTESIAN_POINT('Ctrl Pts',(20.4542455817527,9.7716204510407,12.));
#252708=CARTESIAN_POINT('Ctrl Pts',(20.447195862298,9.76734670980892,0.));
#252709=CARTESIAN_POINT('Ctrl Pts',(20.447195862298,9.76734670980892,12.));
#252710=CARTESIAN_POINT('Ctrl Pts',(20.44034423294,9.76322747195495,0.));
#252711=CARTESIAN_POINT('Ctrl Pts',(20.44034423294,9.76322747195495,12.));
#252712=CARTESIAN_POINT('Ctrl Pts',(20.4336957355473,9.75926386289923,0.));
#252713=CARTESIAN_POINT('Ctrl Pts',(20.4336957355473,9.75926386289923,12.));
#252714=CARTESIAN_POINT('Ctrl Pts',(20.4272556476629,9.75545705902418,0.));
#252715=CARTESIAN_POINT('Ctrl Pts',(20.4272556476629,9.75545705902418,12.));
#252716=CARTESIAN_POINT('Ctrl Pts',(20.4210295275817,9.7518082978643,0.));
#252717=CARTESIAN_POINT('Ctrl Pts',(20.4210295275817,9.7518082978643,12.));
#252718=CARTESIAN_POINT('Ctrl Pts',(20.4150232777393,9.74831889242174,0.));
#252719=CARTESIAN_POINT('Ctrl Pts',(20.4150232777393,9.74831889242174,12.));
#252720=CARTESIAN_POINT('Ctrl Pts',(20.4092430879861,9.74499021838538,0.));
#252721=CARTESIAN_POINT('Ctrl Pts',(20.4092430879861,9.74499021838538,12.));
#252722=CARTESIAN_POINT('Ctrl Pts',(20.4036953576549,9.74182369656272,0.));
#252723=CARTESIAN_POINT('Ctrl Pts',(20.4036953576549,9.74182369656272,12.));
#252724=CARTESIAN_POINT('Ctrl Pts',(20.3983866213331,9.73882077613201,0.));
#252725=CARTESIAN_POINT('Ctrl Pts',(20.3983866213331,9.73882077613201,12.));
#252726=CARTESIAN_POINT('Ctrl Pts',(20.3933234845647,9.73598292014243,0.));
#252727=CARTESIAN_POINT('Ctrl Pts',(20.3933234845647,9.73598292014243,12.));
#252728=CARTESIAN_POINT('Ctrl Pts',(20.3885129129912,9.73331167102808,0.));
#252729=CARTESIAN_POINT('Ctrl Pts',(20.3885129129912,9.73331167102808,12.));
#252730=CARTESIAN_POINT('Ctrl Pts',(20.3839624556742,9.73080870123727,0.));
#252731=CARTESIAN_POINT('Ctrl Pts',(20.3839624556742,9.73080870123727,12.));
#252732=CARTESIAN_POINT('Ctrl Pts',(20.3796805893304,9.72847589116542,0.));
#252733=CARTESIAN_POINT('Ctrl Pts',(20.3796805893304,9.72847589116542,12.));
#252734=CARTESIAN_POINT('Ctrl Pts',(20.3756766651951,9.72631531732881,0.));
#252735=CARTESIAN_POINT('Ctrl Pts',(20.3756766651951,9.72631531732881,12.));
#252736=CARTESIAN_POINT('Ctrl Pts',(20.371960235676,9.72432910043194,0.));
#252737=CARTESIAN_POINT('Ctrl Pts',(20.371960235676,9.72432910043194,12.));
#252738=CARTESIAN_POINT('Ctrl Pts',(20.3685406190576,9.7225193072249,0.));
#252739=CARTESIAN_POINT('Ctrl Pts',(20.3685406190576,9.7225193072249,12.));
#252740=CARTESIAN_POINT('Ctrl Pts',(20.3654261611056,9.72088778381081,0.));
#252741=CARTESIAN_POINT('Ctrl Pts',(20.3654261611056,9.72088778381081,12.));
#252742=CARTESIAN_POINT('Ctrl Pts',(20.3626256913981,9.71943648548099,0.));
#252743=CARTESIAN_POINT('Ctrl Pts',(20.3626256913981,9.71943648548099,12.));
#252744=CARTESIAN_POINT('Ctrl Pts',(20.3601498764344,9.71816778328007,0.));
#252745=CARTESIAN_POINT('Ctrl Pts',(20.3601498764344,9.71816778328007,12.));
#252746=CARTESIAN_POINT('Ctrl Pts',(20.3580133103356,9.71708493723096,0.));
#252747=CARTESIAN_POINT('Ctrl Pts',(20.3580133103356,9.71708493723096,12.));
#252748=CARTESIAN_POINT('Ctrl Pts',(20.3562337557875,9.71619192554186,0.));
#252749=CARTESIAN_POINT('Ctrl Pts',(20.3562337557875,9.71619192554186,12.));
#252750=CARTESIAN_POINT('Ctrl Pts',(20.3548282742361,9.71549257088173,0.));
#252751=CARTESIAN_POINT('Ctrl Pts',(20.3548282742361,9.71549257088173,12.));
#252752=CARTESIAN_POINT('Ctrl Pts',(20.3538098605706,9.71498978052021,0.));
#252753=CARTESIAN_POINT('Ctrl Pts',(20.3538098605706,9.71498978052021,12.));
#252754=CARTESIAN_POINT('Ctrl Pts',(20.3533097561886,9.71474590350681,0.));
#252755=CARTESIAN_POINT('Ctrl Pts',(20.3533097561886,9.71474590350681,12.));
#252756=CARTESIAN_POINT('Ctrl Pts',(20.3531126095522,9.71465227853042,0.));
#252757=CARTESIAN_POINT('Ctrl Pts',(20.3531126095522,9.71465227853042,12.));
#252758=CARTESIAN_POINT('Ctrl Pts',(20.353060251684,9.71462954053042,0.));
#252759=CARTESIAN_POINT('Ctrl Pts',(20.353060251684,9.71462954053042,12.));
#252760=CARTESIAN_POINT('Ctrl Pts',(20.353053841303,9.71462809124916,0.));
#252761=CARTESIAN_POINT('Ctrl Pts',(20.353053841303,9.71462809124916,12.));
#252762=CARTESIAN_POINT('',(22.8400320311648,12.4230808101438,0.));
#252763=CARTESIAN_POINT('Ctrl Pts',(22.8400320311648,12.4230808101438,0.));
#252764=CARTESIAN_POINT('Ctrl Pts',(22.8370364396459,12.418215285186,0.));
#252765=CARTESIAN_POINT('Ctrl Pts',(22.8310435872747,12.4084933766347,0.));
#252766=CARTESIAN_POINT('Ctrl Pts',(22.8220493007173,12.3939379378998,0.));
#252767=CARTESIAN_POINT('Ctrl Pts',(22.81004690224,12.374585536673,0.));
#252768=CARTESIAN_POINT('Ctrl Pts',(22.795027221673,12.3504864740319,0.));
#252769=CARTESIAN_POINT('Ctrl Pts',(22.7799908974768,12.3264788926075,0.));
#252770=CARTESIAN_POINT('Ctrl Pts',(22.764938010105,12.3025628601792,0.));
#252771=CARTESIAN_POINT('Ctrl Pts',(22.7498686970069,12.2787384750742,0.));
#252772=CARTESIAN_POINT('Ctrl Pts',(22.7347831655287,12.2550058702395,0.));
#252773=CARTESIAN_POINT('Ctrl Pts',(22.7196817119374,12.2313652198061,0.));
#252774=CARTESIAN_POINT('Ctrl Pts',(22.7045647168747,12.2078167360284,0.));
#252775=CARTESIAN_POINT('Ctrl Pts',(22.6894326205037,12.1843606579262,0.));
#252776=CARTESIAN_POINT('Ctrl Pts',(22.6742859034944,12.1609972423099,0.));
#252777=CARTESIAN_POINT('Ctrl Pts',(22.6591250653965,12.1377267537145,0.));
#252778=CARTESIAN_POINT('Ctrl Pts',(22.6439506046605,12.1145494550383,0.));
#252779=CARTESIAN_POINT('Ctrl Pts',(22.6287629967056,12.0914655972823,0.));
#252780=CARTESIAN_POINT('Ctrl Pts',(22.6135626764898,12.0684754113862,0.));
#252781=CARTESIAN_POINT('Ctrl Pts',(22.5983500505644,12.0455791139128,0.));
#252782=CARTESIAN_POINT('Ctrl Pts',(22.5831255061282,12.0227769113127,0.));
#252783=CARTESIAN_POINT('Ctrl Pts',(22.5678894211181,12.0000690046695,0.));
#252784=CARTESIAN_POINT('Ctrl Pts',(22.5526421741158,11.9774555943496,0.));
#252785=CARTESIAN_POINT('Ctrl Pts',(22.5373841537307,11.9549368843997,0.));
#252786=CARTESIAN_POINT('Ctrl Pts',(22.5221157697883,11.9325130877803,0.));
#252787=CARTESIAN_POINT('Ctrl Pts',(22.5068374513973,11.9101844254557,0.));
#252788=CARTESIAN_POINT('Ctrl Pts',(22.4915496418485,11.8879511239943,0.));
#252789=CARTESIAN_POINT('Ctrl Pts',(22.4762527946702,11.8658134137019,0.));
#252790=CARTESIAN_POINT('Ctrl Pts',(22.4609473690471,11.8437715264487,0.));
#252791=CARTESIAN_POINT('Ctrl Pts',(22.4456338258735,11.8218256937889,0.));
#252792=CARTESIAN_POINT('Ctrl Pts',(22.430312622646,11.7999761445173,0.));
#252793=CARTESIAN_POINT('Ctrl Pts',(22.4149842125008,11.7782231042039,0.));
#252794=CARTESIAN_POINT('Ctrl Pts',(22.3996490469191,11.7565667964764,0.));
#252795=CARTESIAN_POINT('Ctrl Pts',(22.3843075773899,11.7350074437961,0.));
#252796=CARTESIAN_POINT('Ctrl Pts',(22.3689602575491,11.7135452684532,0.));
#252797=CARTESIAN_POINT('Ctrl Pts',(22.3536075450029,11.6921804934056,0.));
#252798=CARTESIAN_POINT('Ctrl Pts',(22.3382499035619,11.6709133432985,0.));
#252799=CARTESIAN_POINT('Ctrl Pts',(22.3228878043976,11.6497440449857,0.));
#252800=CARTESIAN_POINT('Ctrl Pts',(22.3075217249049,11.6286728270009,0.));
#252801=CARTESIAN_POINT('Ctrl Pts',(22.2921521480356,11.6076999192357,0.));
#252802=CARTESIAN_POINT('Ctrl Pts',(22.2767795614348,11.5868255525188,0.));
#252803=CARTESIAN_POINT('Ctrl Pts',(22.2614044566898,11.5660499582403,0.));
#252804=CARTESIAN_POINT('Ctrl Pts',(22.2460273284654,11.5453733679121,0.));
#252805=CARTESIAN_POINT('Ctrl Pts',(22.2306486738901,11.5247960128477,0.));
#252806=CARTESIAN_POINT('Ctrl Pts',(22.2152689931022,11.5043181244242,0.));
#252807=CARTESIAN_POINT('Ctrl Pts',(22.1998887896436,11.483939934259,0.));
#252808=CARTESIAN_POINT('Ctrl Pts',(22.184508570917,11.463661674411,0.));
#252809=CARTESIAN_POINT('Ctrl Pts',(22.1691288486096,11.443483577557,0.));
#252810=CARTESIAN_POINT('Ctrl Pts',(22.1537501391487,11.4234058771742,0.));
#252811=CARTESIAN_POINT('Ctrl Pts',(22.1383729640964,11.4034288076908,0.));
#252812=CARTESIAN_POINT('Ctrl Pts',(22.1229978500186,11.3835526044256,0.));
#252813=CARTESIAN_POINT('Ctrl Pts',(22.1076253283979,11.3637775035367,0.));
#252814=CARTESIAN_POINT('Ctrl Pts',(22.0922559355294,11.3441037419553,0.));
#252815=CARTESIAN_POINT('Ctrl Pts',(22.0768902124267,11.3245315573168,0.));
#252816=CARTESIAN_POINT('Ctrl Pts',(22.0615287047179,11.3050611878771,0.));
#252817=CARTESIAN_POINT('Ctrl Pts',(22.046171962566,11.2856928724374,0.));
#252818=CARTESIAN_POINT('Ctrl Pts',(22.030820540835,11.2664268504206,0.));
#252819=CARTESIAN_POINT('Ctrl Pts',(22.0154749992363,11.2472633619275,0.));
#252820=CARTESIAN_POINT('Ctrl Pts',(22.0001359024839,11.2282026477896,0.));
#252821=CARTESIAN_POINT('Ctrl Pts',(21.9848038204439,11.2092449496125,0.));
#252822=CARTESIAN_POINT('Ctrl Pts',(21.9694793282914,11.190390509811,0.));
#252823=CARTESIAN_POINT('Ctrl Pts',(21.9541630066506,11.1716395716376,0.));
#252824=CARTESIAN_POINT('Ctrl Pts',(21.9388554416439,11.1529923792003,0.));
#252825=CARTESIAN_POINT('Ctrl Pts',(21.923557224952,11.1344491774741,0.));
#252826=CARTESIAN_POINT('Ctrl Pts',(21.9082689538688,11.1160102123024,0.));
#252827=CARTESIAN_POINT('Ctrl Pts',(21.8929912313608,11.0976757303944,0.));
#252828=CARTESIAN_POINT('Ctrl Pts',(21.877724666119,11.0794459793057,0.));
#252829=CARTESIAN_POINT('Ctrl Pts',(21.8624698726318,11.0613212074363,0.));
#252830=CARTESIAN_POINT('Ctrl Pts',(21.8472274713103,11.0433016640807,0.));
#252831=CARTESIAN_POINT('Ctrl Pts',(21.8319980886033,11.0253875994598,0.));
#252832=CARTESIAN_POINT('Ctrl Pts',(21.8167823571168,11.0075792647477,0.));
#252833=CARTESIAN_POINT('Ctrl Pts',(21.8015809157301,10.9898769120912,0.));
#252834=CARTESIAN_POINT('Ctrl Pts',(21.7863944097141,10.9722807946156,0.));
#252835=CARTESIAN_POINT('Ctrl Pts',(21.7712234908464,10.9547911664455,0.));
#252836=CARTESIAN_POINT('Ctrl Pts',(21.7560688175247,10.9374082827444,0.));
#252837=CARTESIAN_POINT('Ctrl Pts',(21.7409310548797,10.9201323997384,0.));
#252838=CARTESIAN_POINT('Ctrl Pts',(21.7258108748873,10.902963774734,0.));
#252839=CARTESIAN_POINT('Ctrl Pts',(21.7107089564825,10.8859026661293,0.));
#252840=CARTESIAN_POINT('Ctrl Pts',(21.6956259856672,10.8689493334095,0.));
#252841=CARTESIAN_POINT('Ctrl Pts',(21.6805626556467,10.8521040371835,0.));
#252842=CARTESIAN_POINT('Ctrl Pts',(21.6655196669732,10.8353670392272,0.));
#252843=CARTESIAN_POINT('Ctrl Pts',(21.6504977276866,10.8187386025136,0.));
#252844=CARTESIAN_POINT('Ctrl Pts',(21.6354975534557,10.8022189912369,0.));
#252845=CARTESIAN_POINT('Ctrl Pts',(21.6205198677173,10.7858084708261,0.));
#252846=CARTESIAN_POINT('Ctrl Pts',(21.6055654018176,10.7695073079552,0.));
#252847=CARTESIAN_POINT('Ctrl Pts',(21.5906348951743,10.7533157705941,0.));
#252848=CARTESIAN_POINT('Ctrl Pts',(21.5757290954371,10.7372341280467,0.));
#252849=CARTESIAN_POINT('Ctrl Pts',(21.5608487586468,10.7212626509816,0.));
#252850=CARTESIAN_POINT('Ctrl Pts',(21.5459946493955,10.7054016114571,0.));
#252851=CARTESIAN_POINT('Ctrl Pts',(21.5311675409807,10.689651282929,0.));
#252852=CARTESIAN_POINT('Ctrl Pts',(21.51636821558,10.6740119402834,0.));
#252853=CARTESIAN_POINT('Ctrl Pts',(21.5015974644449,10.6584838598939,0.));
#252854=CARTESIAN_POINT('Ctrl Pts',(21.4868560880889,10.6430673196607,0.));
#252855=CARTESIAN_POINT('Ctrl Pts',(21.4721448964766,10.6277625990456,0.));
#252856=CARTESIAN_POINT('Ctrl Pts',(21.4574647092097,10.6125699790961,0.));
#252857=CARTESIAN_POINT('Ctrl Pts',(21.4428163557144,10.5974897424622,0.));
#252858=CARTESIAN_POINT('Ctrl Pts',(21.4282006754631,10.5825221734573,0.));
#252859=CARTESIAN_POINT('Ctrl Pts',(21.4136185181979,10.5676675581108,0.));
#252860=CARTESIAN_POINT('Ctrl Pts',(21.3990707441497,10.5529261842108,0.));
#252861=CARTESIAN_POINT('Ctrl Pts',(21.3845582242602,10.5382983413421,0.));
#252862=CARTESIAN_POINT('Ctrl Pts',(21.3700818403936,10.5237843209057,0.));
#252863=CARTESIAN_POINT('Ctrl Pts',(21.3556424855814,10.5093844161685,0.));
#252864=CARTESIAN_POINT('Ctrl Pts',(21.3412410642904,10.4950989223337,0.));
#252865=CARTESIAN_POINT('Ctrl Pts',(21.3268784926819,10.4809281365931,0.));
#252866=CARTESIAN_POINT('Ctrl Pts',(21.3125556988731,10.4668723581768,0.));
#252867=CARTESIAN_POINT('Ctrl Pts',(21.2982736231931,10.4529318883874,0.));
#252868=CARTESIAN_POINT('Ctrl Pts',(21.2840332184483,10.4391070306391,0.));
#252869=CARTESIAN_POINT('Ctrl Pts',(21.2698354502403,10.42539809054,0.));
#252870=CARTESIAN_POINT('Ctrl Pts',(21.255681297275,10.4118053759588,0.));
#252871=CARTESIAN_POINT('Ctrl Pts',(21.2415717516714,10.3983291970846,0.));
#252872=CARTESIAN_POINT('Ctrl Pts',(21.22750781927,10.3849698664786,0.));
#252873=CARTESIAN_POINT('Ctrl Pts',(21.2134905199345,10.371727699113,0.));
#252874=CARTESIAN_POINT('Ctrl Pts',(21.199520887919,10.3586030124587,0.));
#252875=CARTESIAN_POINT('Ctrl Pts',(21.1855999722416,10.3455961265701,0.));
#252876=CARTESIAN_POINT('Ctrl Pts',(21.1717288370509,10.3327073641572,0.));
#252877=CARTESIAN_POINT('Ctrl Pts',(21.1579085619965,10.3199370506544,0.));
#252878=CARTESIAN_POINT('Ctrl Pts',(21.1441402425843,10.3072855142687,0.));
#252879=CARTESIAN_POINT('Ctrl Pts',(21.1304249906002,10.2947530860721,0.));
#252880=CARTESIAN_POINT('Ctrl Pts',(21.1167639345631,10.2823401001072,0.));
#252881=CARTESIAN_POINT('Ctrl Pts',(21.1031582201627,10.2700468934744,0.));
#252882=CARTESIAN_POINT('Ctrl Pts',(21.0896090107063,10.2578738064181,0.));
#252883=CARTESIAN_POINT('Ctrl Pts',(21.0761174875444,10.2458211823912,0.));
#252884=CARTESIAN_POINT('Ctrl Pts',(21.0626848505663,10.2338893681567,0.));
#252885=CARTESIAN_POINT('Ctrl Pts',(21.0493123187483,10.2220787139155,0.));
#252886=CARTESIAN_POINT('Ctrl Pts',(21.0360011306815,10.2103895734123,0.));
#252887=CARTESIAN_POINT('Ctrl Pts',(21.0227525451107,10.1988223040425,0.));
#252888=CARTESIAN_POINT('Ctrl Pts',(21.0095678414486,10.187377266936,0.));
#252889=CARTESIAN_POINT('Ctrl Pts',(20.9964483203686,10.1760548270767,0.));
#252890=CARTESIAN_POINT('Ctrl Pts',(20.9833953044736,10.1648553534568,0.));
#252891=CARTESIAN_POINT('Ctrl Pts',(20.9704101389369,10.1537792192065,0.));
#252892=CARTESIAN_POINT('Ctrl Pts',(20.9574941921591,10.1428268017256,0.));
#252893=CARTESIAN_POINT('Ctrl Pts',(20.9446488563933,10.1319984827908,0.));
#252894=CARTESIAN_POINT('Ctrl Pts',(20.9318755484734,10.1212946487057,0.));
#252895=CARTESIAN_POINT('Ctrl Pts',(20.919175710627,10.1107156904836,0.));
#252896=CARTESIAN_POINT('Ctrl Pts',(20.9065508112557,10.1002620040076,0.));
#252897=CARTESIAN_POINT('Ctrl Pts',(20.894002345737,10.0899339901916,0.));
#252898=CARTESIAN_POINT('Ctrl Pts',(20.881531837184,10.0797320551154,0.));
#252899=CARTESIAN_POINT('Ctrl Pts',(20.86914083737,10.0696566102218,0.));
#252900=CARTESIAN_POINT('Ctrl Pts',(20.8568309277316,10.0597080725375,0.));
#252901=CARTESIAN_POINT('Ctrl Pts',(20.8446037203402,10.0498868648733,0.));
#252902=CARTESIAN_POINT('Ctrl Pts',(20.8324608588909,10.0401934160234,0.));
#252903=CARTESIAN_POINT('Ctrl Pts',(20.8204040196602,10.0306281609435,0.));
#252904=CARTESIAN_POINT('Ctrl Pts',(20.8084349126888,10.0211915410095,0.));
#252905=CARTESIAN_POINT('Ctrl Pts',(20.7965552829908,10.0118840042786,0.));
#252906=CARTESIAN_POINT('Ctrl Pts',(20.7847669117568,10.0027060057389,0.));
#252907=CARTESIAN_POINT('Ctrl Pts',(20.7730716175417,9.9936580075464,0.));
#252908=CARTESIAN_POINT('Ctrl Pts',(20.761471257499,9.98474047926853,0.));
#252909=CARTESIAN_POINT('Ctrl Pts',(20.7499677289627,9.9759538982347,0.));
#252910=CARTESIAN_POINT('Ctrl Pts',(20.7385629709795,9.96729874986202,0.));
#252911=CARTESIAN_POINT('Ctrl Pts',(20.7272589658751,9.95877552798398,0.));
#252912=CARTESIAN_POINT('Ctrl Pts',(20.7160577407579,9.95038473514949,0.));
#252913=CARTESIAN_POINT('Ctrl Pts',(20.7049613692234,9.94212688298236,0.));
#252914=CARTESIAN_POINT('Ctrl Pts',(20.6939719732484,9.9340024925973,0.));
#252915=CARTESIAN_POINT('Ctrl Pts',(20.6830917250255,9.92601209498749,0.));
#252916=CARTESIAN_POINT('Ctrl Pts',(20.6723228488263,9.91815623141289,0.));
#252917=CARTESIAN_POINT('Ctrl Pts',(20.6616676228315,9.91043545377008,0.));
#252918=CARTESIAN_POINT('Ctrl Pts',(20.6511283817414,9.90285032516693,0.));
#252919=CARTESIAN_POINT('Ctrl Pts',(20.6407075193976,9.8954014204912,0.));
#252920=CARTESIAN_POINT('Ctrl Pts',(20.6304074914087,9.88808932697306,0.));
#252921=CARTESIAN_POINT('Ctrl Pts',(20.6202308177474,9.88091464472676,0.));
#252922=CARTESIAN_POINT('Ctrl Pts',(20.6101800854494,9.87387798732956,0.));
#252923=CARTESIAN_POINT('Ctrl Pts',(20.6002579513699,9.86697998242623,0.));
#252924=CARTESIAN_POINT('Ctrl Pts',(20.5904671449754,9.86022127232748,0.));
#252925=CARTESIAN_POINT('Ctrl Pts',(20.5808104710015,9.85360251456981,0.));
#252926=CARTESIAN_POINT('Ctrl Pts',(20.5712908125139,9.84712438256278,0.));
#252927=CARTESIAN_POINT('Ctrl Pts',(20.5619111362402,9.84078756677565,0.));
#252928=CARTESIAN_POINT('Ctrl Pts',(20.552674497646,9.83459277585315,0.));
#252929=CARTESIAN_POINT('Ctrl Pts',(20.5435840460721,9.82854073773878,0.));
#252930=CARTESIAN_POINT('Ctrl Pts',(20.5346430299517,9.82263220080363,0.));
#252931=CARTESIAN_POINT('Ctrl Pts',(20.5258548000629,9.81686793455943,0.));
#252932=CARTESIAN_POINT('Ctrl Pts',(20.517222812284,9.81124873025282,0.));
#252933=CARTESIAN_POINT('Ctrl Pts',(20.5087506310505,9.80577540161088,0.));
#252934=CARTESIAN_POINT('Ctrl Pts',(20.5004419312107,9.80044878520949,0.));
#252935=CARTESIAN_POINT('Ctrl Pts',(20.4923005087943,9.79526974288331,0.));
#252936=CARTESIAN_POINT('Ctrl Pts',(20.4843302955329,9.79023916498656,0.));
#252937=CARTESIAN_POINT('Ctrl Pts',(20.4765353711586,9.78535797314167,0.));
#252938=CARTESIAN_POINT('Ctrl Pts',(20.4689199790669,9.78062712373321,0.));
#252939=CARTESIAN_POINT('Ctrl Pts',(20.4614885274975,9.77604760815529,0.));
#252940=CARTESIAN_POINT('Ctrl Pts',(20.4542455817527,9.7716204510407,0.));
#252941=CARTESIAN_POINT('Ctrl Pts',(20.447195862298,9.76734670980892,0.));
#252942=CARTESIAN_POINT('Ctrl Pts',(20.44034423294,9.76322747195495,0.));
#252943=CARTESIAN_POINT('Ctrl Pts',(20.4336957355473,9.75926386289923,0.));
#252944=CARTESIAN_POINT('Ctrl Pts',(20.4272556476629,9.75545705902418,0.));
#252945=CARTESIAN_POINT('Ctrl Pts',(20.4210295275817,9.7518082978643,0.));
#252946=CARTESIAN_POINT('Ctrl Pts',(20.4150232777393,9.74831889242174,0.));
#252947=CARTESIAN_POINT('Ctrl Pts',(20.4092430879861,9.74499021838538,0.));
#252948=CARTESIAN_POINT('Ctrl Pts',(20.4036953576549,9.74182369656272,0.));
#252949=CARTESIAN_POINT('Ctrl Pts',(20.3983866213331,9.73882077613201,0.));
#252950=CARTESIAN_POINT('Ctrl Pts',(20.3933234845647,9.73598292014243,0.));
#252951=CARTESIAN_POINT('Ctrl Pts',(20.3885129129912,9.73331167102808,0.));
#252952=CARTESIAN_POINT('Ctrl Pts',(20.3839624556742,9.73080870123727,0.));
#252953=CARTESIAN_POINT('Ctrl Pts',(20.3796805893304,9.72847589116542,0.));
#252954=CARTESIAN_POINT('Ctrl Pts',(20.3756766651951,9.72631531732881,0.));
#252955=CARTESIAN_POINT('Ctrl Pts',(20.371960235676,9.72432910043194,0.));
#252956=CARTESIAN_POINT('Ctrl Pts',(20.3685406190576,9.7225193072249,0.));
#252957=CARTESIAN_POINT('Ctrl Pts',(20.3654261611056,9.72088778381081,0.));
#252958=CARTESIAN_POINT('Ctrl Pts',(20.3626256913981,9.71943648548099,0.));
#252959=CARTESIAN_POINT('Ctrl Pts',(20.3601498764344,9.71816778328007,0.));
#252960=CARTESIAN_POINT('Ctrl Pts',(20.3580133103356,9.71708493723096,0.));
#252961=CARTESIAN_POINT('Ctrl Pts',(20.3562337557875,9.71619192554186,0.));
#252962=CARTESIAN_POINT('Ctrl Pts',(20.3548282742361,9.71549257088173,0.));
#252963=CARTESIAN_POINT('Ctrl Pts',(20.3538098605706,9.71498978052021,0.));
#252964=CARTESIAN_POINT('Ctrl Pts',(20.3533097561886,9.71474590350681,0.));
#252965=CARTESIAN_POINT('Ctrl Pts',(20.3531126095522,9.71465227853042,0.));
#252966=CARTESIAN_POINT('Ctrl Pts',(20.353060251684,9.71462954053042,0.));
#252967=CARTESIAN_POINT('Ctrl Pts',(20.353053841303,9.71462809124916,0.));
#252968=CARTESIAN_POINT('',(22.8400320311648,12.4230808101438,12.));
#252969=CARTESIAN_POINT('',(22.8400320311648,12.4230808101438,0.));
#252970=CARTESIAN_POINT('Ctrl Pts',(20.353053841303,9.71462809124916,12.));
#252971=CARTESIAN_POINT('Ctrl Pts',(20.353060251684,9.71462954053042,12.));
#252972=CARTESIAN_POINT('Ctrl Pts',(20.3531126095522,9.71465227853042,12.));
#252973=CARTESIAN_POINT('Ctrl Pts',(20.3533097561886,9.71474590350681,12.));
#252974=CARTESIAN_POINT('Ctrl Pts',(20.3538098605706,9.71498978052021,12.));
#252975=CARTESIAN_POINT('Ctrl Pts',(20.3548282742361,9.71549257088173,12.));
#252976=CARTESIAN_POINT('Ctrl Pts',(20.3562337557875,9.71619192554186,12.));
#252977=CARTESIAN_POINT('Ctrl Pts',(20.3580133103356,9.71708493723096,12.));
#252978=CARTESIAN_POINT('Ctrl Pts',(20.3601498764344,9.71816778328007,12.));
#252979=CARTESIAN_POINT('Ctrl Pts',(20.3626256913981,9.71943648548099,12.));
#252980=CARTESIAN_POINT('Ctrl Pts',(20.3654261611056,9.72088778381081,12.));
#252981=CARTESIAN_POINT('Ctrl Pts',(20.3685406190576,9.7225193072249,12.));
#252982=CARTESIAN_POINT('Ctrl Pts',(20.371960235676,9.72432910043194,12.));
#252983=CARTESIAN_POINT('Ctrl Pts',(20.3756766651951,9.72631531732881,12.));
#252984=CARTESIAN_POINT('Ctrl Pts',(20.3796805893304,9.72847589116542,12.));
#252985=CARTESIAN_POINT('Ctrl Pts',(20.3839624556742,9.73080870123727,12.));
#252986=CARTESIAN_POINT('Ctrl Pts',(20.3885129129912,9.73331167102808,12.));
#252987=CARTESIAN_POINT('Ctrl Pts',(20.3933234845647,9.73598292014243,12.));
#252988=CARTESIAN_POINT('Ctrl Pts',(20.3983866213331,9.73882077613201,12.));
#252989=CARTESIAN_POINT('Ctrl Pts',(20.4036953576549,9.74182369656272,12.));
#252990=CARTESIAN_POINT('Ctrl Pts',(20.4092430879861,9.74499021838538,12.));
#252991=CARTESIAN_POINT('Ctrl Pts',(20.4150232777393,9.74831889242174,12.));
#252992=CARTESIAN_POINT('Ctrl Pts',(20.4210295275817,9.7518082978643,12.));
#252993=CARTESIAN_POINT('Ctrl Pts',(20.4272556476629,9.75545705902418,12.));
#252994=CARTESIAN_POINT('Ctrl Pts',(20.4336957355473,9.75926386289923,12.));
#252995=CARTESIAN_POINT('Ctrl Pts',(20.44034423294,9.76322747195495,12.));
#252996=CARTESIAN_POINT('Ctrl Pts',(20.447195862298,9.76734670980892,12.));
#252997=CARTESIAN_POINT('Ctrl Pts',(20.4542455817527,9.7716204510407,12.));
#252998=CARTESIAN_POINT('Ctrl Pts',(20.4614885274975,9.77604760815529,12.));
#252999=CARTESIAN_POINT('Ctrl Pts',(20.4689199790669,9.78062712373321,12.));
#253000=CARTESIAN_POINT('Ctrl Pts',(20.4765353711586,9.78535797314167,12.));
#253001=CARTESIAN_POINT('Ctrl Pts',(20.4843302955329,9.79023916498656,12.));
#253002=CARTESIAN_POINT('Ctrl Pts',(20.4923005087943,9.79526974288331,12.));
#253003=CARTESIAN_POINT('Ctrl Pts',(20.5004419312107,9.80044878520949,12.));
#253004=CARTESIAN_POINT('Ctrl Pts',(20.5087506310505,9.80577540161088,12.));
#253005=CARTESIAN_POINT('Ctrl Pts',(20.517222812284,9.81124873025282,12.));
#253006=CARTESIAN_POINT('Ctrl Pts',(20.5258548000629,9.81686793455943,12.));
#253007=CARTESIAN_POINT('Ctrl Pts',(20.5346430299517,9.82263220080363,12.));
#253008=CARTESIAN_POINT('Ctrl Pts',(20.5435840460721,9.82854073773878,12.));
#253009=CARTESIAN_POINT('Ctrl Pts',(20.552674497646,9.83459277585315,12.));
#253010=CARTESIAN_POINT('Ctrl Pts',(20.5619111362402,9.84078756677565,12.));
#253011=CARTESIAN_POINT('Ctrl Pts',(20.5712908125139,9.84712438256278,12.));
#253012=CARTESIAN_POINT('Ctrl Pts',(20.5808104710015,9.85360251456981,12.));
#253013=CARTESIAN_POINT('Ctrl Pts',(20.5904671449754,9.86022127232748,12.));
#253014=CARTESIAN_POINT('Ctrl Pts',(20.6002579513699,9.86697998242623,12.));
#253015=CARTESIAN_POINT('Ctrl Pts',(20.6101800854494,9.87387798732956,12.));
#253016=CARTESIAN_POINT('Ctrl Pts',(20.6202308177474,9.88091464472676,12.));
#253017=CARTESIAN_POINT('Ctrl Pts',(20.6304074914087,9.88808932697306,12.));
#253018=CARTESIAN_POINT('Ctrl Pts',(20.6407075193976,9.8954014204912,12.));
#253019=CARTESIAN_POINT('Ctrl Pts',(20.6511283817414,9.90285032516693,12.));
#253020=CARTESIAN_POINT('Ctrl Pts',(20.6616676228315,9.91043545377008,12.));
#253021=CARTESIAN_POINT('Ctrl Pts',(20.6723228488263,9.91815623141289,12.));
#253022=CARTESIAN_POINT('Ctrl Pts',(20.6830917250255,9.92601209498749,12.));
#253023=CARTESIAN_POINT('Ctrl Pts',(20.6939719732484,9.9340024925973,12.));
#253024=CARTESIAN_POINT('Ctrl Pts',(20.7049613692234,9.94212688298236,12.));
#253025=CARTESIAN_POINT('Ctrl Pts',(20.7160577407579,9.95038473514949,12.));
#253026=CARTESIAN_POINT('Ctrl Pts',(20.7272589658751,9.95877552798398,12.));
#253027=CARTESIAN_POINT('Ctrl Pts',(20.7385629709795,9.96729874986202,12.));
#253028=CARTESIAN_POINT('Ctrl Pts',(20.7499677289627,9.9759538982347,12.));
#253029=CARTESIAN_POINT('Ctrl Pts',(20.761471257499,9.98474047926853,12.));
#253030=CARTESIAN_POINT('Ctrl Pts',(20.7730716175417,9.9936580075464,12.));
#253031=CARTESIAN_POINT('Ctrl Pts',(20.7847669117568,10.0027060057389,12.));
#253032=CARTESIAN_POINT('Ctrl Pts',(20.7965552829908,10.0118840042786,12.));
#253033=CARTESIAN_POINT('Ctrl Pts',(20.8084349126888,10.0211915410095,12.));
#253034=CARTESIAN_POINT('Ctrl Pts',(20.8204040196602,10.0306281609435,12.));
#253035=CARTESIAN_POINT('Ctrl Pts',(20.8324608588909,10.0401934160234,12.));
#253036=CARTESIAN_POINT('Ctrl Pts',(20.8446037203402,10.0498868648733,12.));
#253037=CARTESIAN_POINT('Ctrl Pts',(20.8568309277316,10.0597080725375,12.));
#253038=CARTESIAN_POINT('Ctrl Pts',(20.86914083737,10.0696566102218,12.));
#253039=CARTESIAN_POINT('Ctrl Pts',(20.881531837184,10.0797320551154,12.));
#253040=CARTESIAN_POINT('Ctrl Pts',(20.894002345737,10.0899339901916,12.));
#253041=CARTESIAN_POINT('Ctrl Pts',(20.9065508112557,10.1002620040076,12.));
#253042=CARTESIAN_POINT('Ctrl Pts',(20.919175710627,10.1107156904836,12.));
#253043=CARTESIAN_POINT('Ctrl Pts',(20.9318755484734,10.1212946487057,12.));
#253044=CARTESIAN_POINT('Ctrl Pts',(20.9446488563933,10.1319984827908,12.));
#253045=CARTESIAN_POINT('Ctrl Pts',(20.9574941921591,10.1428268017256,12.));
#253046=CARTESIAN_POINT('Ctrl Pts',(20.9704101389369,10.1537792192065,12.));
#253047=CARTESIAN_POINT('Ctrl Pts',(20.9833953044736,10.1648553534568,12.));
#253048=CARTESIAN_POINT('Ctrl Pts',(20.9964483203686,10.1760548270767,12.));
#253049=CARTESIAN_POINT('Ctrl Pts',(21.0095678414486,10.187377266936,12.));
#253050=CARTESIAN_POINT('Ctrl Pts',(21.0227525451107,10.1988223040425,12.));
#253051=CARTESIAN_POINT('Ctrl Pts',(21.0360011306815,10.2103895734123,12.));
#253052=CARTESIAN_POINT('Ctrl Pts',(21.0493123187483,10.2220787139155,12.));
#253053=CARTESIAN_POINT('Ctrl Pts',(21.0626848505663,10.2338893681567,12.));
#253054=CARTESIAN_POINT('Ctrl Pts',(21.0761174875444,10.2458211823912,12.));
#253055=CARTESIAN_POINT('Ctrl Pts',(21.0896090107063,10.2578738064181,12.));
#253056=CARTESIAN_POINT('Ctrl Pts',(21.1031582201627,10.2700468934744,12.));
#253057=CARTESIAN_POINT('Ctrl Pts',(21.1167639345631,10.2823401001072,12.));
#253058=CARTESIAN_POINT('Ctrl Pts',(21.1304249906002,10.2947530860721,12.));
#253059=CARTESIAN_POINT('Ctrl Pts',(21.1441402425843,10.3072855142687,12.));
#253060=CARTESIAN_POINT('Ctrl Pts',(21.1579085619965,10.3199370506544,12.));
#253061=CARTESIAN_POINT('Ctrl Pts',(21.1717288370509,10.3327073641572,12.));
#253062=CARTESIAN_POINT('Ctrl Pts',(21.1855999722416,10.3455961265701,12.));
#253063=CARTESIAN_POINT('Ctrl Pts',(21.199520887919,10.3586030124587,12.));
#253064=CARTESIAN_POINT('Ctrl Pts',(21.2134905199345,10.371727699113,12.));
#253065=CARTESIAN_POINT('Ctrl Pts',(21.22750781927,10.3849698664786,12.));
#253066=CARTESIAN_POINT('Ctrl Pts',(21.2415717516714,10.3983291970846,12.));
#253067=CARTESIAN_POINT('Ctrl Pts',(21.255681297275,10.4118053759588,12.));
#253068=CARTESIAN_POINT('Ctrl Pts',(21.2698354502403,10.42539809054,12.));
#253069=CARTESIAN_POINT('Ctrl Pts',(21.2840332184483,10.4391070306391,12.));
#253070=CARTESIAN_POINT('Ctrl Pts',(21.2982736231931,10.4529318883874,12.));
#253071=CARTESIAN_POINT('Ctrl Pts',(21.3125556988731,10.4668723581768,12.));
#253072=CARTESIAN_POINT('Ctrl Pts',(21.3268784926819,10.4809281365931,12.));
#253073=CARTESIAN_POINT('Ctrl Pts',(21.3412410642904,10.4950989223337,12.));
#253074=CARTESIAN_POINT('Ctrl Pts',(21.3556424855814,10.5093844161685,12.));
#253075=CARTESIAN_POINT('Ctrl Pts',(21.3700818403936,10.5237843209057,12.));
#253076=CARTESIAN_POINT('Ctrl Pts',(21.3845582242602,10.5382983413421,12.));
#253077=CARTESIAN_POINT('Ctrl Pts',(21.3990707441497,10.5529261842108,12.));
#253078=CARTESIAN_POINT('Ctrl Pts',(21.4136185181979,10.5676675581108,12.));
#253079=CARTESIAN_POINT('Ctrl Pts',(21.4282006754631,10.5825221734573,12.));
#253080=CARTESIAN_POINT('Ctrl Pts',(21.4428163557144,10.5974897424622,12.));
#253081=CARTESIAN_POINT('Ctrl Pts',(21.4574647092097,10.6125699790961,12.));
#253082=CARTESIAN_POINT('Ctrl Pts',(21.4721448964766,10.6277625990456,12.));
#253083=CARTESIAN_POINT('Ctrl Pts',(21.4868560880889,10.6430673196607,12.));
#253084=CARTESIAN_POINT('Ctrl Pts',(21.5015974644449,10.6584838598939,12.));
#253085=CARTESIAN_POINT('Ctrl Pts',(21.51636821558,10.6740119402834,12.));
#253086=CARTESIAN_POINT('Ctrl Pts',(21.5311675409807,10.689651282929,12.));
#253087=CARTESIAN_POINT('Ctrl Pts',(21.5459946493955,10.7054016114571,12.));
#253088=CARTESIAN_POINT('Ctrl Pts',(21.5608487586468,10.7212626509816,12.));
#253089=CARTESIAN_POINT('Ctrl Pts',(21.5757290954371,10.7372341280467,12.));
#253090=CARTESIAN_POINT('Ctrl Pts',(21.5906348951743,10.7533157705941,12.));
#253091=CARTESIAN_POINT('Ctrl Pts',(21.6055654018176,10.7695073079552,12.));
#253092=CARTESIAN_POINT('Ctrl Pts',(21.6205198677173,10.7858084708261,12.));
#253093=CARTESIAN_POINT('Ctrl Pts',(21.6354975534557,10.8022189912369,12.));
#253094=CARTESIAN_POINT('Ctrl Pts',(21.6504977276866,10.8187386025136,12.));
#253095=CARTESIAN_POINT('Ctrl Pts',(21.6655196669732,10.8353670392272,12.));
#253096=CARTESIAN_POINT('Ctrl Pts',(21.6805626556467,10.8521040371835,12.));
#253097=CARTESIAN_POINT('Ctrl Pts',(21.6956259856672,10.8689493334095,12.));
#253098=CARTESIAN_POINT('Ctrl Pts',(21.7107089564825,10.8859026661293,12.));
#253099=CARTESIAN_POINT('Ctrl Pts',(21.7258108748873,10.902963774734,12.));
#253100=CARTESIAN_POINT('Ctrl Pts',(21.7409310548797,10.9201323997384,12.));
#253101=CARTESIAN_POINT('Ctrl Pts',(21.7560688175247,10.9374082827444,12.));
#253102=CARTESIAN_POINT('Ctrl Pts',(21.7712234908464,10.9547911664455,12.));
#253103=CARTESIAN_POINT('Ctrl Pts',(21.7863944097141,10.9722807946156,12.));
#253104=CARTESIAN_POINT('Ctrl Pts',(21.8015809157301,10.9898769120912,12.));
#253105=CARTESIAN_POINT('Ctrl Pts',(21.8167823571168,11.0075792647477,12.));
#253106=CARTESIAN_POINT('Ctrl Pts',(21.8319980886033,11.0253875994598,12.));
#253107=CARTESIAN_POINT('Ctrl Pts',(21.8472274713103,11.0433016640807,12.));
#253108=CARTESIAN_POINT('Ctrl Pts',(21.8624698726318,11.0613212074363,12.));
#253109=CARTESIAN_POINT('Ctrl Pts',(21.877724666119,11.0794459793057,12.));
#253110=CARTESIAN_POINT('Ctrl Pts',(21.8929912313608,11.0976757303944,12.));
#253111=CARTESIAN_POINT('Ctrl Pts',(21.9082689538688,11.1160102123024,12.));
#253112=CARTESIAN_POINT('Ctrl Pts',(21.923557224952,11.1344491774741,12.));
#253113=CARTESIAN_POINT('Ctrl Pts',(21.9388554416439,11.1529923792003,12.));
#253114=CARTESIAN_POINT('Ctrl Pts',(21.9541630066506,11.1716395716376,12.));
#253115=CARTESIAN_POINT('Ctrl Pts',(21.9694793282914,11.190390509811,12.));
#253116=CARTESIAN_POINT('Ctrl Pts',(21.9848038204439,11.2092449496125,12.));
#253117=CARTESIAN_POINT('Ctrl Pts',(22.0001359024839,11.2282026477896,12.));
#253118=CARTESIAN_POINT('Ctrl Pts',(22.0154749992363,11.2472633619275,12.));
#253119=CARTESIAN_POINT('Ctrl Pts',(22.030820540835,11.2664268504206,12.));
#253120=CARTESIAN_POINT('Ctrl Pts',(22.046171962566,11.2856928724374,12.));
#253121=CARTESIAN_POINT('Ctrl Pts',(22.0615287047179,11.3050611878771,12.));
#253122=CARTESIAN_POINT('Ctrl Pts',(22.0768902124267,11.3245315573168,12.));
#253123=CARTESIAN_POINT('Ctrl Pts',(22.0922559355294,11.3441037419553,12.));
#253124=CARTESIAN_POINT('Ctrl Pts',(22.1076253283979,11.3637775035367,12.));
#253125=CARTESIAN_POINT('Ctrl Pts',(22.1229978500186,11.3835526044256,12.));
#253126=CARTESIAN_POINT('Ctrl Pts',(22.1383729640964,11.4034288076908,12.));
#253127=CARTESIAN_POINT('Ctrl Pts',(22.1537501391487,11.4234058771742,12.));
#253128=CARTESIAN_POINT('Ctrl Pts',(22.1691288486096,11.443483577557,12.));
#253129=CARTESIAN_POINT('Ctrl Pts',(22.184508570917,11.463661674411,12.));
#253130=CARTESIAN_POINT('Ctrl Pts',(22.1998887896436,11.483939934259,12.));
#253131=CARTESIAN_POINT('Ctrl Pts',(22.2152689931022,11.5043181244242,12.));
#253132=CARTESIAN_POINT('Ctrl Pts',(22.2306486738901,11.5247960128477,12.));
#253133=CARTESIAN_POINT('Ctrl Pts',(22.2460273284654,11.5453733679121,12.));
#253134=CARTESIAN_POINT('Ctrl Pts',(22.2614044566898,11.5660499582403,12.));
#253135=CARTESIAN_POINT('Ctrl Pts',(22.2767795614348,11.5868255525188,12.));
#253136=CARTESIAN_POINT('Ctrl Pts',(22.2921521480356,11.6076999192357,12.));
#253137=CARTESIAN_POINT('Ctrl Pts',(22.3075217249049,11.6286728270009,12.));
#253138=CARTESIAN_POINT('Ctrl Pts',(22.3228878043976,11.6497440449857,12.));
#253139=CARTESIAN_POINT('Ctrl Pts',(22.3382499035619,11.6709133432985,12.));
#253140=CARTESIAN_POINT('Ctrl Pts',(22.3536075450029,11.6921804934056,12.));
#253141=CARTESIAN_POINT('Ctrl Pts',(22.3689602575491,11.7135452684532,12.));
#253142=CARTESIAN_POINT('Ctrl Pts',(22.3843075773899,11.7350074437961,12.));
#253143=CARTESIAN_POINT('Ctrl Pts',(22.3996490469191,11.7565667964764,12.));
#253144=CARTESIAN_POINT('Ctrl Pts',(22.4149842125008,11.7782231042039,12.));
#253145=CARTESIAN_POINT('Ctrl Pts',(22.430312622646,11.7999761445173,12.));
#253146=CARTESIAN_POINT('Ctrl Pts',(22.4456338258735,11.8218256937889,12.));
#253147=CARTESIAN_POINT('Ctrl Pts',(22.4609473690471,11.8437715264487,12.));
#253148=CARTESIAN_POINT('Ctrl Pts',(22.4762527946702,11.8658134137019,12.));
#253149=CARTESIAN_POINT('Ctrl Pts',(22.4915496418485,11.8879511239943,12.));
#253150=CARTESIAN_POINT('Ctrl Pts',(22.5068374513973,11.9101844254557,12.));
#253151=CARTESIAN_POINT('Ctrl Pts',(22.5221157697883,11.9325130877803,12.));
#253152=CARTESIAN_POINT('Ctrl Pts',(22.5373841537307,11.9549368843997,12.));
#253153=CARTESIAN_POINT('Ctrl Pts',(22.5526421741158,11.9774555943496,12.));
#253154=CARTESIAN_POINT('Ctrl Pts',(22.5678894211181,12.0000690046695,12.));
#253155=CARTESIAN_POINT('Ctrl Pts',(22.5831255061282,12.0227769113127,12.));
#253156=CARTESIAN_POINT('Ctrl Pts',(22.5983500505644,12.0455791139128,12.));
#253157=CARTESIAN_POINT('Ctrl Pts',(22.6135626764898,12.0684754113862,12.));
#253158=CARTESIAN_POINT('Ctrl Pts',(22.6287629967056,12.0914655972823,12.));
#253159=CARTESIAN_POINT('Ctrl Pts',(22.6439506046605,12.1145494550383,12.));
#253160=CARTESIAN_POINT('Ctrl Pts',(22.6591250653965,12.1377267537145,12.));
#253161=CARTESIAN_POINT('Ctrl Pts',(22.6742859034944,12.1609972423099,12.));
#253162=CARTESIAN_POINT('Ctrl Pts',(22.6894326205037,12.1843606579262,12.));
#253163=CARTESIAN_POINT('Ctrl Pts',(22.7045647168747,12.2078167360284,12.));
#253164=CARTESIAN_POINT('Ctrl Pts',(22.7196817119374,12.2313652198061,12.));
#253165=CARTESIAN_POINT('Ctrl Pts',(22.7347831655287,12.2550058702395,12.));
#253166=CARTESIAN_POINT('Ctrl Pts',(22.7498686970069,12.2787384750742,12.));
#253167=CARTESIAN_POINT('Ctrl Pts',(22.764938010105,12.3025628601792,12.));
#253168=CARTESIAN_POINT('Ctrl Pts',(22.7799908974768,12.3264788926075,12.));
#253169=CARTESIAN_POINT('Ctrl Pts',(22.795027221673,12.3504864740319,12.));
#253170=CARTESIAN_POINT('Ctrl Pts',(22.81004690224,12.374585536673,12.));
#253171=CARTESIAN_POINT('Ctrl Pts',(22.8220493007173,12.3939379378998,12.));
#253172=CARTESIAN_POINT('Ctrl Pts',(22.8310435872747,12.4084933766347,12.));
#253173=CARTESIAN_POINT('Ctrl Pts',(22.8370364396459,12.418215285186,12.));
#253174=CARTESIAN_POINT('Ctrl Pts',(22.8400320311648,12.4230808101438,12.));
#253175=CARTESIAN_POINT('Ctrl Pts',(21.2610617890679,7.52250298901264,0.));
#253176=CARTESIAN_POINT('Ctrl Pts',(21.2610617890679,7.52250298901264,12.));
#253177=CARTESIAN_POINT('Ctrl Pts',(21.2610673466886,7.5225064970397,0.));
#253178=CARTESIAN_POINT('Ctrl Pts',(21.2610673466886,7.5225064970397,12.));
#253179=CARTESIAN_POINT('Ctrl Pts',(21.2611204474866,7.52252744144904,0.));
#253180=CARTESIAN_POINT('Ctrl Pts',(21.2611204474866,7.52252744144904,12.));
#253181=CARTESIAN_POINT('Ctrl Pts',(21.261326054066,7.52260064231661,0.));
#253182=CARTESIAN_POINT('Ctrl Pts',(21.261326054066,7.52260064231661,12.));
#253183=CARTESIAN_POINT('Ctrl Pts',(21.2618521283555,7.5227818224267,0.));
#253184=CARTESIAN_POINT('Ctrl Pts',(21.2618521283555,7.5227818224267,12.));
#253185=CARTESIAN_POINT('Ctrl Pts',(21.262927782038,7.52314642316199,0.));
#253186=CARTESIAN_POINT('Ctrl Pts',(21.262927782038,7.52314642316199,12.));
#253187=CARTESIAN_POINT('Ctrl Pts',(21.2644161259962,7.52364573027553,0.));
#253188=CARTESIAN_POINT('Ctrl Pts',(21.2644161259962,7.52364573027553,12.));
#253189=CARTESIAN_POINT('Ctrl Pts',(21.2663059157058,7.52427261074298,0.));
#253190=CARTESIAN_POINT('Ctrl Pts',(21.2663059157058,7.52427261074298,12.));
#253191=CARTESIAN_POINT('Ctrl Pts',(21.2685823838671,7.52501770333531,0.));
#253192=CARTESIAN_POINT('Ctrl Pts',(21.2685823838671,7.52501770333531,12.));
#253193=CARTESIAN_POINT('Ctrl Pts',(21.2712301573466,7.5258712609553,0.));
#253194=CARTESIAN_POINT('Ctrl Pts',(21.2712301573466,7.5258712609553,12.));
#253195=CARTESIAN_POINT('Ctrl Pts',(21.2742366113579,7.52682526918541,0.));
#253196=CARTESIAN_POINT('Ctrl Pts',(21.2742366113579,7.52682526918541,12.));
#253197=CARTESIAN_POINT('Ctrl Pts',(21.2775925269652,7.52787386225333,0.));
#253198=CARTESIAN_POINT('Ctrl Pts',(21.2775925269652,7.52787386225333,12.));
#253199=CARTESIAN_POINT('Ctrl Pts',(21.2812902781143,7.52901217930408,0.));
#253200=CARTESIAN_POINT('Ctrl Pts',(21.2812902781143,7.52901217930408,12.));
#253201=CARTESIAN_POINT('Ctrl Pts',(21.2853226580657,7.5302356243823,0.));
#253202=CARTESIAN_POINT('Ctrl Pts',(21.2853226580657,7.5302356243823,12.));
#253203=CARTESIAN_POINT('Ctrl Pts',(21.2896816163842,7.53153906987856,0.));
#253204=CARTESIAN_POINT('Ctrl Pts',(21.2896816163842,7.53153906987856,12.));
#253205=CARTESIAN_POINT('Ctrl Pts',(21.2943588989331,7.53291726078527,0.));
#253206=CARTESIAN_POINT('Ctrl Pts',(21.2943588989331,7.53291726078527,12.));
#253207=CARTESIAN_POINT('Ctrl Pts',(21.2993464250717,7.53436505309943,0.));
#253208=CARTESIAN_POINT('Ctrl Pts',(21.2993464250717,7.53436505309943,12.));
#253209=CARTESIAN_POINT('Ctrl Pts',(21.3046368712157,7.53587778251736,0.));
#253210=CARTESIAN_POINT('Ctrl Pts',(21.3046368712157,7.53587778251736,12.));
#253211=CARTESIAN_POINT('Ctrl Pts',(21.310223716773,7.53745129364616,0.));
#253212=CARTESIAN_POINT('Ctrl Pts',(21.310223716773,7.53745129364616,12.));
#253213=CARTESIAN_POINT('Ctrl Pts',(21.3161009456256,7.53908175169899,0.));
#253214=CARTESIAN_POINT('Ctrl Pts',(21.3161009456256,7.53908175169899,12.));
#253215=CARTESIAN_POINT('Ctrl Pts',(21.3222628524165,7.54076552038279,0.));
#253216=CARTESIAN_POINT('Ctrl Pts',(21.3222628524165,7.54076552038279,12.));
#253217=CARTESIAN_POINT('Ctrl Pts',(21.328703791771,7.54249900377031,0.));
#253218=CARTESIAN_POINT('Ctrl Pts',(21.328703791771,7.54249900377031,12.));
#253219=CARTESIAN_POINT('Ctrl Pts',(21.3354182340149,7.54427868151268,0.));
#253220=CARTESIAN_POINT('Ctrl Pts',(21.3354182340149,7.54427868151268,12.));
#253221=CARTESIAN_POINT('Ctrl Pts',(21.3424008295038,7.54610114948347,0.));
#253222=CARTESIAN_POINT('Ctrl Pts',(21.3424008295038,7.54610114948347,12.));
#253223=CARTESIAN_POINT('Ctrl Pts',(21.3496464761531,7.54796316246331,0.));
#253224=CARTESIAN_POINT('Ctrl Pts',(21.3496464761531,7.54796316246331,12.));
#253225=CARTESIAN_POINT('Ctrl Pts',(21.3571503685855,7.5498616652131,0.));
#253226=CARTESIAN_POINT('Ctrl Pts',(21.3571503685855,7.5498616652131,12.));
#253227=CARTESIAN_POINT('Ctrl Pts',(21.3649079431865,7.55179375777444,0.));
#253228=CARTESIAN_POINT('Ctrl Pts',(21.3649079431865,7.55179375777444,12.));
#253229=CARTESIAN_POINT('Ctrl Pts',(21.3729148390243,7.55375667080029,0.));
#253230=CARTESIAN_POINT('Ctrl Pts',(21.3729148390243,7.55375667080029,12.));
#253231=CARTESIAN_POINT('Ctrl Pts',(21.3811668478932,7.55574773403503,0.));
#253232=CARTESIAN_POINT('Ctrl Pts',(21.3811668478932,7.55574773403503,12.));
#253233=CARTESIAN_POINT('Ctrl Pts',(21.3896598842117,7.55776435731417,0.));
#253234=CARTESIAN_POINT('Ctrl Pts',(21.3896598842117,7.55776435731417,12.));
#253235=CARTESIAN_POINT('Ctrl Pts',(21.3983899952987,7.55980403700611,0.));
#253236=CARTESIAN_POINT('Ctrl Pts',(21.3983899952987,7.55980403700611,12.));
#253237=CARTESIAN_POINT('Ctrl Pts',(21.4073533630365,7.56186435703622,0.));
#253238=CARTESIAN_POINT('Ctrl Pts',(21.4073533630365,7.56186435703622,12.));
#253239=CARTESIAN_POINT('Ctrl Pts',(21.4165463106254,7.56394299313685,0.));
#253240=CARTESIAN_POINT('Ctrl Pts',(21.4165463106254,7.56394299313685,12.));
#253241=CARTESIAN_POINT('Ctrl Pts',(21.4259653015736,7.56603771218712,0.));
#253242=CARTESIAN_POINT('Ctrl Pts',(21.4259653015736,7.56603771218712,12.));
#253243=CARTESIAN_POINT('Ctrl Pts',(21.4356069261513,7.56814636360848,0.));
#253244=CARTESIAN_POINT('Ctrl Pts',(21.4356069261513,7.56814636360848,12.));
#253245=CARTESIAN_POINT('Ctrl Pts',(21.4454678907509,7.57026687261166,0.));
#253246=CARTESIAN_POINT('Ctrl Pts',(21.4454678907509,7.57026687261166,12.));
#253247=CARTESIAN_POINT('Ctrl Pts',(21.4555450053142,7.57239723223506,0.));
#253248=CARTESIAN_POINT('Ctrl Pts',(21.4555450053142,7.57239723223506,12.));
#253249=CARTESIAN_POINT('Ctrl Pts',(21.4658351740128,7.57453549743412,0.));
#253250=CARTESIAN_POINT('Ctrl Pts',(21.4658351740128,7.57453549743412,12.));
#253251=CARTESIAN_POINT('Ctrl Pts',(21.4763353936762,7.57667978402987,0.));
#253252=CARTESIAN_POINT('Ctrl Pts',(21.4763353936762,7.57667978402987,12.));
#253253=CARTESIAN_POINT('Ctrl Pts',(21.4870427508194,7.57882826679132,0.));
#253254=CARTESIAN_POINT('Ctrl Pts',(21.4870427508194,7.57882826679132,12.));
#253255=CARTESIAN_POINT('Ctrl Pts',(21.4979544192744,7.58097917790744,0.));
#253256=CARTESIAN_POINT('Ctrl Pts',(21.4979544192744,7.58097917790744,12.));
#253257=CARTESIAN_POINT('Ctrl Pts',(21.5090676573873,7.5831308051918,0.));
#253258=CARTESIAN_POINT('Ctrl Pts',(21.5090676573873,7.5831308051918,12.));
#253259=CARTESIAN_POINT('Ctrl Pts',(21.5203798035299,7.5852814891913,0.));
#253260=CARTESIAN_POINT('Ctrl Pts',(21.5203798035299,7.5852814891913,12.));
#253261=CARTESIAN_POINT('Ctrl Pts',(21.5318882716736,7.58742962034834,0.));
#253262=CARTESIAN_POINT('Ctrl Pts',(21.5318882716736,7.58742962034834,12.));
#253263=CARTESIAN_POINT('Ctrl Pts',(21.543590547011,7.58957363620014,0.));
#253264=CARTESIAN_POINT('Ctrl Pts',(21.543590547011,7.58957363620014,12.));
#253265=CARTESIAN_POINT('Ctrl Pts',(21.5554841813462,7.59171201844777,0.));
#253266=CARTESIAN_POINT('Ctrl Pts',(21.5554841813462,7.59171201844777,12.));
#253267=CARTESIAN_POINT('Ctrl Pts',(21.5675667904726,7.59384329124918,0.));
#253268=CARTESIAN_POINT('Ctrl Pts',(21.5675667904726,7.59384329124918,12.));
#253269=CARTESIAN_POINT('Ctrl Pts',(21.5798360518978,7.59596601973584,0.));
#253270=CARTESIAN_POINT('Ctrl Pts',(21.5798360518978,7.59596601973584,12.));
#253271=CARTESIAN_POINT('Ctrl Pts',(21.5922897024466,7.59807880846195,0.));
#253272=CARTESIAN_POINT('Ctrl Pts',(21.5922897024466,7.59807880846195,12.));
#253273=CARTESIAN_POINT('Ctrl Pts',(21.6049255358843,7.60018029988241,0.));
#253274=CARTESIAN_POINT('Ctrl Pts',(21.6049255358843,7.60018029988241,12.));
#253275=CARTESIAN_POINT('Ctrl Pts',(21.617741400599,7.60226917285429,0.));
#253276=CARTESIAN_POINT('Ctrl Pts',(21.617741400599,7.60226917285429,12.));
#253277=CARTESIAN_POINT('Ctrl Pts',(21.6307351973822,7.60434414118296,0.));
#253278=CARTESIAN_POINT('Ctrl Pts',(21.6307351973822,7.60434414118296,12.));
#253279=CARTESIAN_POINT('Ctrl Pts',(21.6439048771743,7.60640395216357,0.));
#253280=CARTESIAN_POINT('Ctrl Pts',(21.6439048771743,7.60640395216357,12.));
#253281=CARTESIAN_POINT('Ctrl Pts',(21.6572484388081,7.60844738512874,0.));
#253282=CARTESIAN_POINT('Ctrl Pts',(21.6572484388081,7.60844738512874,12.));
#253283=CARTESIAN_POINT('Ctrl Pts',(21.6707639267576,7.61047325000956,0.));
#253284=CARTESIAN_POINT('Ctrl Pts',(21.6707639267576,7.61047325000956,12.));
#253285=CARTESIAN_POINT('Ctrl Pts',(21.6844494295815,7.61248038630269,0.));
#253286=CARTESIAN_POINT('Ctrl Pts',(21.6844494295815,7.61248038630269,12.));
#253287=CARTESIAN_POINT('Ctrl Pts',(21.6983030783322,7.61446766202787,0.));
#253288=CARTESIAN_POINT('Ctrl Pts',(21.6983030783322,7.61446766202787,12.));
#253289=CARTESIAN_POINT('Ctrl Pts',(21.7123230449834,7.61643397270421,0.));
#253290=CARTESIAN_POINT('Ctrl Pts',(21.7123230449834,7.61643397270421,12.));
#253291=CARTESIAN_POINT('Ctrl Pts',(21.7265075407975,7.61837824030538,0.));
#253292=CARTESIAN_POINT('Ctrl Pts',(21.7265075407975,7.61837824030538,12.));
#253293=CARTESIAN_POINT('Ctrl Pts',(21.7408548148656,7.62029941230855,0.));
#253294=CARTESIAN_POINT('Ctrl Pts',(21.7408548148656,7.62029941230855,12.));
#253295=CARTESIAN_POINT('Ctrl Pts',(21.7553631528328,7.62219646084229,0.));
#253296=CARTESIAN_POINT('Ctrl Pts',(21.7553631528328,7.62219646084229,12.));
#253297=CARTESIAN_POINT('Ctrl Pts',(21.7700308755584,7.62406838181166,0.));
#253298=CARTESIAN_POINT('Ctrl Pts',(21.7700308755584,7.62406838181166,12.));
#253299=CARTESIAN_POINT('Ctrl Pts',(21.7848563378021,7.62591419404513,0.));
#253300=CARTESIAN_POINT('Ctrl Pts',(21.7848563378021,7.62591419404513,12.));
#253301=CARTESIAN_POINT('Ctrl Pts',(21.799837926858,7.62773293842389,0.));
#253302=CARTESIAN_POINT('Ctrl Pts',(21.799837926858,7.62773293842389,12.));
#253303=CARTESIAN_POINT('Ctrl Pts',(21.814974061509,7.62952367718127,0.));
#253304=CARTESIAN_POINT('Ctrl Pts',(21.814974061509,7.62952367718127,12.));
#253305=CARTESIAN_POINT('Ctrl Pts',(21.8302631910195,7.63128549323023,0.));
#253306=CARTESIAN_POINT('Ctrl Pts',(21.8302631910195,7.63128549323023,12.));
#253307=CARTESIAN_POINT('Ctrl Pts',(21.8457037941084,7.63301748948936,0.));
#253308=CARTESIAN_POINT('Ctrl Pts',(21.8457037941084,7.63301748948936,12.));
#253309=CARTESIAN_POINT('Ctrl Pts',(21.8612943779089,7.63471878821226,0.));
#253310=CARTESIAN_POINT('Ctrl Pts',(21.8612943779089,7.63471878821226,12.));
#253311=CARTESIAN_POINT('Ctrl Pts',(21.8770334769496,7.636388530334,0.));
#253312=CARTESIAN_POINT('Ctrl Pts',(21.8770334769496,7.636388530334,12.));
#253313=CARTESIAN_POINT('Ctrl Pts',(21.8929196523514,7.63802587492035,0.));
#253314=CARTESIAN_POINT('Ctrl Pts',(21.8929196523514,7.63802587492035,12.));
#253315=CARTESIAN_POINT('Ctrl Pts',(21.9089514909874,7.63962999860927,0.));
#253316=CARTESIAN_POINT('Ctrl Pts',(21.9089514909874,7.63962999860927,12.));
#253317=CARTESIAN_POINT('Ctrl Pts',(21.9251276046545,7.64120009506532,0.));
#253318=CARTESIAN_POINT('Ctrl Pts',(21.9251276046545,7.64120009506532,12.));
#253319=CARTESIAN_POINT('Ctrl Pts',(21.9414466292072,7.64273537442682,0.));
#253320=CARTESIAN_POINT('Ctrl Pts',(21.9414466292072,7.64273537442682,12.));
#253321=CARTESIAN_POINT('Ctrl Pts',(21.9579072237651,7.64423506279123,0.));
#253322=CARTESIAN_POINT('Ctrl Pts',(21.9579072237651,7.64423506279123,12.));
#253323=CARTESIAN_POINT('Ctrl Pts',(21.9745080700798,7.64569840177336,0.));
#253324=CARTESIAN_POINT('Ctrl Pts',(21.9745080700798,7.64569840177336,12.));
#253325=CARTESIAN_POINT('Ctrl Pts',(21.9912478718542,7.6471246480525,0.));
#253326=CARTESIAN_POINT('Ctrl Pts',(21.9912478718542,7.6471246480525,12.));
#253327=CARTESIAN_POINT('Ctrl Pts',(22.0081253540774,7.64851307293352,0.));
#253328=CARTESIAN_POINT('Ctrl Pts',(22.0081253540774,7.64851307293352,12.));
#253329=CARTESIAN_POINT('Ctrl Pts',(22.0251392623209,7.64986296190169,0.));
#253330=CARTESIAN_POINT('Ctrl Pts',(22.0251392623209,7.64986296190169,12.));
#253331=CARTESIAN_POINT('Ctrl Pts',(22.0422883621174,7.65117361421359,0.));
#253332=CARTESIAN_POINT('Ctrl Pts',(22.0422883621174,7.65117361421359,12.));
#253333=CARTESIAN_POINT('Ctrl Pts',(22.0595714384431,7.65244434253113,0.));
#253334=CARTESIAN_POINT('Ctrl Pts',(22.0595714384431,7.65244434253113,12.));
#253335=CARTESIAN_POINT('Ctrl Pts',(22.0769872951596,7.65367447254949,0.));
#253336=CARTESIAN_POINT('Ctrl Pts',(22.0769872951596,7.65367447254949,12.));
#253337=CARTESIAN_POINT('Ctrl Pts',(22.094534754469,7.65486334263644,0.));
#253338=CARTESIAN_POINT('Ctrl Pts',(22.094534754469,7.65486334263644,12.));
#253339=CARTESIAN_POINT('Ctrl Pts',(22.1122126563329,7.65601030346807,0.));
#253340=CARTESIAN_POINT('Ctrl Pts',(22.1122126563329,7.65601030346807,12.));
#253341=CARTESIAN_POINT('Ctrl Pts',(22.1300198579675,7.65711471769397,0.));
#253342=CARTESIAN_POINT('Ctrl Pts',(22.1300198579675,7.65711471769397,12.));
#253343=CARTESIAN_POINT('Ctrl Pts',(22.1479552334211,7.65817595963349,0.));
#253344=CARTESIAN_POINT('Ctrl Pts',(22.1479552334211,7.65817595963349,12.));
#253345=CARTESIAN_POINT('Ctrl Pts',(22.1660176731178,7.65919341496931,0.));
#253346=CARTESIAN_POINT('Ctrl Pts',(22.1660176731178,7.65919341496931,12.));
#253347=CARTESIAN_POINT('Ctrl Pts',(22.1842060834091,7.66016648045005,0.));
#253348=CARTESIAN_POINT('Ctrl Pts',(22.1842060834091,7.66016648045005,12.));
#253349=CARTESIAN_POINT('Ctrl Pts',(22.2025193860964,7.66109456359271,0.));
#253350=CARTESIAN_POINT('Ctrl Pts',(22.2025193860964,7.66109456359271,12.));
#253351=CARTESIAN_POINT('Ctrl Pts',(22.2209565180085,7.661977082404,0.));
#253352=CARTESIAN_POINT('Ctrl Pts',(22.2209565180085,7.661977082404,12.));
#253353=CARTESIAN_POINT('Ctrl Pts',(22.2395164306547,7.66281346512509,0.));
#253354=CARTESIAN_POINT('Ctrl Pts',(22.2395164306547,7.66281346512509,12.));
#253355=CARTESIAN_POINT('Ctrl Pts',(22.258198089848,7.66360314997641,0.));
#253356=CARTESIAN_POINT('Ctrl Pts',(22.258198089848,7.66360314997641,12.));
#253357=CARTESIAN_POINT('Ctrl Pts',(22.2770004753335,7.66434558490979,0.));
#253358=CARTESIAN_POINT('Ctrl Pts',(22.2770004753335,7.66434558490979,12.));
#253359=CARTESIAN_POINT('Ctrl Pts',(22.2959225803937,7.66504022736299,0.));
#253360=CARTESIAN_POINT('Ctrl Pts',(22.2959225803937,7.66504022736299,12.));
#253361=CARTESIAN_POINT('Ctrl Pts',(22.314963411484,7.66568654402494,0.));
#253362=CARTESIAN_POINT('Ctrl Pts',(22.314963411484,7.66568654402494,12.));
#253363=CARTESIAN_POINT('Ctrl Pts',(22.3341219879469,7.66628401061952,0.));
#253364=CARTESIAN_POINT('Ctrl Pts',(22.3341219879469,7.66628401061952,12.));
#253365=CARTESIAN_POINT('Ctrl Pts',(22.3533973417021,7.66683211169159,0.));
#253366=CARTESIAN_POINT('Ctrl Pts',(22.3533973417021,7.66683211169159,12.));
#253367=CARTESIAN_POINT('Ctrl Pts',(22.372788516936,7.66733034039883,0.));
#253368=CARTESIAN_POINT('Ctrl Pts',(22.372788516936,7.66733034039883,12.));
#253369=CARTESIAN_POINT('Ctrl Pts',(22.3922945697773,7.6677781983079,0.));
#253370=CARTESIAN_POINT('Ctrl Pts',(22.3922945697773,7.6677781983079,12.));
#253371=CARTESIAN_POINT('Ctrl Pts',(22.4119145679758,7.6681751951964,0.));
#253372=CARTESIAN_POINT('Ctrl Pts',(22.4119145679758,7.6681751951964,12.));
#253373=CARTESIAN_POINT('Ctrl Pts',(22.4316475906603,7.66852084886704,0.));
#253374=CARTESIAN_POINT('Ctrl Pts',(22.4316475906603,7.66852084886704,12.));
#253375=CARTESIAN_POINT('Ctrl Pts',(22.4514927280855,7.66881468496635,0.));
#253376=CARTESIAN_POINT('Ctrl Pts',(22.4514927280855,7.66881468496635,12.));
#253377=CARTESIAN_POINT('Ctrl Pts',(22.4714490813699,7.66905623680831,0.));
#253378=CARTESIAN_POINT('Ctrl Pts',(22.4714490813699,7.66905623680831,12.));
#253379=CARTESIAN_POINT('Ctrl Pts',(22.4915157622312,7.66924504520315,0.));
#253380=CARTESIAN_POINT('Ctrl Pts',(22.4915157622312,7.66924504520315,12.));
#253381=CARTESIAN_POINT('Ctrl Pts',(22.5116918927031,7.66938065829108,0.));
#253382=CARTESIAN_POINT('Ctrl Pts',(22.5116918927031,7.66938065829108,12.));
#253383=CARTESIAN_POINT('Ctrl Pts',(22.53197660492,7.66946263138144,0.));
#253384=CARTESIAN_POINT('Ctrl Pts',(22.53197660492,7.66946263138144,12.));
#253385=CARTESIAN_POINT('Ctrl Pts',(22.5523690409116,7.66949052679693,0.));
#253386=CARTESIAN_POINT('Ctrl Pts',(22.5523690409116,7.66949052679693,12.));
#253387=CARTESIAN_POINT('Ctrl Pts',(22.5728683523831,7.66946391372306,0.));
#253388=CARTESIAN_POINT('Ctrl Pts',(22.5728683523831,7.66946391372306,12.));
#253389=CARTESIAN_POINT('Ctrl Pts',(22.5934737004953,7.66938236806233,0.));
#253390=CARTESIAN_POINT('Ctrl Pts',(22.5934737004953,7.66938236806233,12.));
#253391=CARTESIAN_POINT('Ctrl Pts',(22.6141842556243,7.66924547229414,0.));
#253392=CARTESIAN_POINT('Ctrl Pts',(22.6141842556243,7.66924547229414,12.));
#253393=CARTESIAN_POINT('Ctrl Pts',(22.6349991971541,7.66905281533715,0.));
#253394=CARTESIAN_POINT('Ctrl Pts',(22.6349991971541,7.66905281533715,12.));
#253395=CARTESIAN_POINT('Ctrl Pts',(22.6559177133127,7.66880399241323,0.));
#253396=CARTESIAN_POINT('Ctrl Pts',(22.6559177133127,7.66880399241323,12.));
#253397=CARTESIAN_POINT('Ctrl Pts',(22.6769390009885,7.66849860491743,0.));
#253398=CARTESIAN_POINT('Ctrl Pts',(22.6769390009885,7.66849860491743,12.));
#253399=CARTESIAN_POINT('Ctrl Pts',(22.6980622655446,7.66813626029275,0.));
#253400=CARTESIAN_POINT('Ctrl Pts',(22.6980622655446,7.66813626029275,12.));
#253401=CARTESIAN_POINT('Ctrl Pts',(22.7192867206245,7.66771657191028,0.));
#253402=CARTESIAN_POINT('Ctrl Pts',(22.7192867206245,7.66771657191028,12.));
#253403=CARTESIAN_POINT('Ctrl Pts',(22.7406115879513,7.6672391589544,0.));
#253404=CARTESIAN_POINT('Ctrl Pts',(22.7406115879513,7.6672391589544,12.));
#253405=CARTESIAN_POINT('Ctrl Pts',(22.7620360971843,7.66670364630299,0.));
#253406=CARTESIAN_POINT('Ctrl Pts',(22.7620360971843,7.66670364630299,12.));
#253407=CARTESIAN_POINT('Ctrl Pts',(22.7835594857699,7.66610966441273,0.));
#253408=CARTESIAN_POINT('Ctrl Pts',(22.7835594857699,7.66610966441273,12.));
#253409=CARTESIAN_POINT('Ctrl Pts',(22.8051809987833,7.66545684920987,0.));
#253410=CARTESIAN_POINT('Ctrl Pts',(22.8051809987833,7.66545684920987,12.));
#253411=CARTESIAN_POINT('Ctrl Pts',(22.8268998887678,7.66474484198549,0.));
#253412=CARTESIAN_POINT('Ctrl Pts',(22.8268998887678,7.66474484198549,12.));
#253413=CARTESIAN_POINT('Ctrl Pts',(22.848715415557,7.66397328929803,0.));
#253414=CARTESIAN_POINT('Ctrl Pts',(22.848715415557,7.66397328929803,12.));
#253415=CARTESIAN_POINT('Ctrl Pts',(22.8706268461283,7.66314184287337,0.));
#253416=CARTESIAN_POINT('Ctrl Pts',(22.8706268461283,7.66314184287337,12.));
#253417=CARTESIAN_POINT('Ctrl Pts',(22.8926334544883,7.66225015950156,0.));
#253418=CARTESIAN_POINT('Ctrl Pts',(22.8926334544883,7.66225015950156,12.));
#253419=CARTESIAN_POINT('Ctrl Pts',(22.9147345215421,7.66129790094108,0.));
#253420=CARTESIAN_POINT('Ctrl Pts',(22.9147345215421,7.66129790094108,12.));
#253421=CARTESIAN_POINT('Ctrl Pts',(22.9369293349593,7.66028473382778,0.));
#253422=CARTESIAN_POINT('Ctrl Pts',(22.9369293349593,7.66028473382778,12.));
#253423=CARTESIAN_POINT('Ctrl Pts',(22.959217189033,7.65921032958902,0.));
#253424=CARTESIAN_POINT('Ctrl Pts',(22.959217189033,7.65921032958902,12.));
#253425=CARTESIAN_POINT('Ctrl Pts',(22.9815973845296,7.65807436436432,0.));
#253426=CARTESIAN_POINT('Ctrl Pts',(22.9815973845296,7.65807436436432,12.));
#253427=CARTESIAN_POINT('Ctrl Pts',(23.0040692285814,7.65687651891305,0.));
#253428=CARTESIAN_POINT('Ctrl Pts',(23.0040692285814,7.65687651891305,12.));
#253429=CARTESIAN_POINT('Ctrl Pts',(23.0266320345787,7.65561647852534,0.));
#253430=CARTESIAN_POINT('Ctrl Pts',(23.0266320345787,7.65561647852534,12.));
#253431=CARTESIAN_POINT('Ctrl Pts',(23.0492851220528,7.65429393293946,0.));
#253432=CARTESIAN_POINT('Ctrl Pts',(23.0492851220528,7.65429393293946,12.));
#253433=CARTESIAN_POINT('Ctrl Pts',(23.072027816555,7.65290857626358,0.));
#253434=CARTESIAN_POINT('Ctrl Pts',(23.072027816555,7.65290857626358,12.));
#253435=CARTESIAN_POINT('Ctrl Pts',(23.094859449525,7.65146010690476,0.));
#253436=CARTESIAN_POINT('Ctrl Pts',(23.094859449525,7.65146010690476,12.));
#253437=CARTESIAN_POINT('Ctrl Pts',(23.1177793581679,7.6499482274986,0.));
#253438=CARTESIAN_POINT('Ctrl Pts',(23.1177793581679,7.6499482274986,12.));
#253439=CARTESIAN_POINT('Ctrl Pts',(23.1407868853819,7.64837264482943,0.));
#253440=CARTESIAN_POINT('Ctrl Pts',(23.1407868853819,7.64837264482943,12.));
#253441=CARTESIAN_POINT('Ctrl Pts',(23.1638813796694,7.64673306975805,0.));
#253442=CARTESIAN_POINT('Ctrl Pts',(23.1638813796694,7.64673306975805,12.));
#253443=CARTESIAN_POINT('Ctrl Pts',(23.1870621950452,7.64502921715483,0.));
#253444=CARTESIAN_POINT('Ctrl Pts',(23.1870621950452,7.64502921715483,12.));
#253445=CARTESIAN_POINT('Ctrl Pts',(23.2103286909398,7.6432608058368,0.));
#253446=CARTESIAN_POINT('Ctrl Pts',(23.2103286909398,7.6432608058368,12.));
#253447=CARTESIAN_POINT('Ctrl Pts',(23.2336802320912,7.64142755851505,0.));
#253448=CARTESIAN_POINT('Ctrl Pts',(23.2336802320912,7.64142755851505,12.));
#253449=CARTESIAN_POINT('Ctrl Pts',(23.2571161884488,7.63952920172835,0.));
#253450=CARTESIAN_POINT('Ctrl Pts',(23.2571161884488,7.63952920172835,12.));
#253451=CARTESIAN_POINT('Ctrl Pts',(23.2806359350855,7.63756546576374,0.));
#253452=CARTESIAN_POINT('Ctrl Pts',(23.2806359350855,7.63756546576374,12.));
#253453=CARTESIAN_POINT('Ctrl Pts',(23.3042388521022,7.63553608458783,0.));
#253454=CARTESIAN_POINT('Ctrl Pts',(23.3042388521022,7.63553608458783,12.));
#253455=CARTESIAN_POINT('Ctrl Pts',(23.3279243245241,7.63344079578162,0.));
#253456=CARTESIAN_POINT('Ctrl Pts',(23.3279243245241,7.63344079578162,12.));
#253457=CARTESIAN_POINT('Ctrl Pts',(23.3516917421972,7.63127934048137,0.));
#253458=CARTESIAN_POINT('Ctrl Pts',(23.3516917421972,7.63127934048137,12.));
#253459=CARTESIAN_POINT('Ctrl Pts',(23.3755404996636,7.62905146332593,0.));
#253460=CARTESIAN_POINT('Ctrl Pts',(23.3755404996636,7.62905146332593,12.));
#253461=CARTESIAN_POINT('Ctrl Pts',(23.399469996112,7.62675691240329,0.));
#253462=CARTESIAN_POINT('Ctrl Pts',(23.399469996112,7.62675691240329,12.));
#253463=CARTESIAN_POINT('Ctrl Pts',(23.4234796353542,7.6243954392005,0.));
#253464=CARTESIAN_POINT('Ctrl Pts',(23.4234796353542,7.6243954392005,12.));
#253465=CARTESIAN_POINT('Ctrl Pts',(23.4475688257854,7.62196679855955,0.));
#253466=CARTESIAN_POINT('Ctrl Pts',(23.4475688257854,7.62196679855955,12.));
#253467=CARTESIAN_POINT('Ctrl Pts',(23.4717369803438,7.61947074863977,0.));
#253468=CARTESIAN_POINT('Ctrl Pts',(23.4717369803438,7.61947074863977,12.));
#253469=CARTESIAN_POINT('Ctrl Pts',(23.4959835164609,7.61690705088319,0.));
#253470=CARTESIAN_POINT('Ctrl Pts',(23.4959835164609,7.61690705088319,12.));
#253471=CARTESIAN_POINT('Ctrl Pts',(23.5203078560129,7.61427546999298,0.));
#253472=CARTESIAN_POINT('Ctrl Pts',(23.5203078560129,7.61427546999298,12.));
#253473=CARTESIAN_POINT('Ctrl Pts',(23.544709425203,7.61157577385372,0.));
#253474=CARTESIAN_POINT('Ctrl Pts',(23.544709425203,7.61157577385372,12.));
#253475=CARTESIAN_POINT('Ctrl Pts',(23.5691876544244,7.608807733446,0.));
#253476=CARTESIAN_POINT('Ctrl Pts',(23.5691876544244,7.608807733446,12.));
#253477=CARTESIAN_POINT('Ctrl Pts',(23.5937419781245,7.60597112277094,0.));
#253478=CARTESIAN_POINT('Ctrl Pts',(23.5937419781245,7.60597112277094,12.));
#253479=CARTESIAN_POINT('Ctrl Pts',(23.6183718346576,7.60306571877806,0.));
#253480=CARTESIAN_POINT('Ctrl Pts',(23.6183718346576,7.60306571877806,12.));
#253481=CARTESIAN_POINT('Ctrl Pts',(23.6430766661418,7.60009130130126,0.));
#253482=CARTESIAN_POINT('Ctrl Pts',(23.6430766661418,7.60009130130126,12.));
#253483=CARTESIAN_POINT('Ctrl Pts',(23.6678559182875,7.59704765299567,0.));
#253484=CARTESIAN_POINT('Ctrl Pts',(23.6678559182875,7.59704765299567,12.));
#253485=CARTESIAN_POINT('Ctrl Pts',(23.6927090405066,7.59393455934035,0.));
#253486=CARTESIAN_POINT('Ctrl Pts',(23.6927090405066,7.59393455934035,12.));
#253487=CARTESIAN_POINT('Ctrl Pts',(23.7176354860456,7.59075180865321,0.));
#253488=CARTESIAN_POINT('Ctrl Pts',(23.7176354860456,7.59075180865321,12.));
#253489=CARTESIAN_POINT('Ctrl Pts',(23.7426347121006,7.58749919210826,0.));
#253490=CARTESIAN_POINT('Ctrl Pts',(23.7426347121006,7.58749919210826,12.));
#253491=CARTESIAN_POINT('Ctrl Pts',(23.7677061799376,7.58417650376271,0.));
#253492=CARTESIAN_POINT('Ctrl Pts',(23.7677061799376,7.58417650376271,12.));
#253493=CARTESIAN_POINT('Ctrl Pts',(23.7928493549908,7.58078354058213,0.));
#253494=CARTESIAN_POINT('Ctrl Pts',(23.7928493549908,7.58078354058213,12.));
#253495=CARTESIAN_POINT('Ctrl Pts',(23.8180637069976,7.57732010249066,0.));
#253496=CARTESIAN_POINT('Ctrl Pts',(23.8180637069976,7.57732010249066,12.));
#253497=CARTESIAN_POINT('Ctrl Pts',(23.8433487096132,7.57378599219814,0.));
#253498=CARTESIAN_POINT('Ctrl Pts',(23.8433487096132,7.57378599219814,12.));
#253499=CARTESIAN_POINT('Ctrl Pts',(23.8687038399595,7.57018101500709,0.));
#253500=CARTESIAN_POINT('Ctrl Pts',(23.8687038399595,7.57018101500709,12.));
#253501=CARTESIAN_POINT('Ctrl Pts',(23.8941285782002,7.56650497863791,0.));
#253502=CARTESIAN_POINT('Ctrl Pts',(23.8941285782002,7.56650497863791,12.));
#253503=CARTESIAN_POINT('Ctrl Pts',(23.9196224070759,7.56275769304773,0.));
#253504=CARTESIAN_POINT('Ctrl Pts',(23.9196224070759,7.56275769304773,12.));
#253505=CARTESIAN_POINT('Ctrl Pts',(23.9451848115002,7.5589389702768,0.));
#253506=CARTESIAN_POINT('Ctrl Pts',(23.9451848115002,7.5589389702768,12.));
#253507=CARTESIAN_POINT('Ctrl Pts',(23.9708152779886,7.55504862424808,0.));
#253508=CARTESIAN_POINT('Ctrl Pts',(23.9708152779886,7.55504862424808,12.));
#253509=CARTESIAN_POINT('Ctrl Pts',(23.9965132953187,7.55108647097432,0.));
#253510=CARTESIAN_POINT('Ctrl Pts',(23.9965132953187,7.55108647097432,12.));
#253511=CARTESIAN_POINT('Ctrl Pts',(24.0222783554531,7.54705232885895,0.));
#253512=CARTESIAN_POINT('Ctrl Pts',(24.0222783554531,7.54705232885895,12.));
#253513=CARTESIAN_POINT('Ctrl Pts',(24.0481099543353,7.54294601896128,0.));
#253514=CARTESIAN_POINT('Ctrl Pts',(24.0481099543353,7.54294601896128,12.));
#253515=CARTESIAN_POINT('Ctrl Pts',(24.0740075927984,7.53876736531005,0.));
#253516=CARTESIAN_POINT('Ctrl Pts',(24.0740075927984,7.53876736531005,12.));
#253517=CARTESIAN_POINT('Ctrl Pts',(24.0999707772642,7.53451619514659,0.));
#253518=CARTESIAN_POINT('Ctrl Pts',(24.0999707772642,7.53451619514659,12.));
#253519=CARTESIAN_POINT('Ctrl Pts',(24.1259990209211,7.53019233935537,0.));
#253520=CARTESIAN_POINT('Ctrl Pts',(24.1259990209211,7.53019233935537,12.));
#253521=CARTESIAN_POINT('Ctrl Pts',(24.152091842537,7.52579563201479,0.));
#253522=CARTESIAN_POINT('Ctrl Pts',(24.152091842537,7.52579563201479,12.));
#253523=CARTESIAN_POINT('Ctrl Pts',(24.1782487641602,7.52132590953863,0.));
#253524=CARTESIAN_POINT('Ctrl Pts',(24.1782487641602,7.52132590953863,12.));
#253525=CARTESIAN_POINT('Ctrl Pts',(24.2044693092356,7.51678300997998,0.));
#253526=CARTESIAN_POINT('Ctrl Pts',(24.2044693092356,7.51678300997998,12.));
#253527=CARTESIAN_POINT('Ctrl Pts',(24.230753000389,7.51216677222199,0.));
#253528=CARTESIAN_POINT('Ctrl Pts',(24.230753000389,7.51216677222199,12.));
#253529=CARTESIAN_POINT('Ctrl Pts',(24.2570993577032,7.50747703535115,0.));
#253530=CARTESIAN_POINT('Ctrl Pts',(24.2570993577032,7.50747703535115,12.));
#253531=CARTESIAN_POINT('Ctrl Pts',(24.2835078958966,7.50271363765099,0.));
#253532=CARTESIAN_POINT('Ctrl Pts',(24.2835078958966,7.50271363765099,12.));
#253533=CARTESIAN_POINT('Ctrl Pts',(24.3099781253345,7.49787641695359,0.));
#253534=CARTESIAN_POINT('Ctrl Pts',(24.3099781253345,7.49787641695359,12.));
#253535=CARTESIAN_POINT('Ctrl Pts',(24.3365095573673,7.4929652125233,0.));
#253536=CARTESIAN_POINT('Ctrl Pts',(24.3365095573673,7.4929652125233,12.));
#253537=CARTESIAN_POINT('Ctrl Pts',(24.3631017084513,7.48797986651828,0.));
#253538=CARTESIAN_POINT('Ctrl Pts',(24.3631017084513,7.48797986651828,12.));
#253539=CARTESIAN_POINT('Ctrl Pts',(24.3897541049248,7.48292022569254,0.));
#253540=CARTESIAN_POINT('Ctrl Pts',(24.3897541049248,7.48292022569254,12.));
#253541=CARTESIAN_POINT('Ctrl Pts',(24.4164662871165,7.47778614286574,0.));
#253542=CARTESIAN_POINT('Ctrl Pts',(24.4164662871165,7.47778614286574,12.));
#253543=CARTESIAN_POINT('Ctrl Pts',(24.4432378146501,7.47257747883319,0.));
#253544=CARTESIAN_POINT('Ctrl Pts',(24.4432378146501,7.47257747883319,12.));
#253545=CARTESIAN_POINT('Ctrl Pts',(24.4700682684544,7.46729410308923,0.));
#253546=CARTESIAN_POINT('Ctrl Pts',(24.4700682684544,7.46729410308923,12.));
#253547=CARTESIAN_POINT('Ctrl Pts',(24.4969572391509,7.46193588961642,0.));
#253548=CARTESIAN_POINT('Ctrl Pts',(24.4969572391509,7.46193588961642,12.));
#253549=CARTESIAN_POINT('Ctrl Pts',(24.52390431731,7.45650271336046,0.));
#253550=CARTESIAN_POINT('Ctrl Pts',(24.52390431731,7.45650271336046,12.));
#253551=CARTESIAN_POINT('Ctrl Pts',(24.5509090831579,7.45099444651296,0.));
#253552=CARTESIAN_POINT('Ctrl Pts',(24.5509090831579,7.45099444651296,12.));
#253553=CARTESIAN_POINT('Ctrl Pts',(24.5779710960865,7.44541095473163,0.));
#253554=CARTESIAN_POINT('Ctrl Pts',(24.5779710960865,7.44541095473163,12.));
#253555=CARTESIAN_POINT('Ctrl Pts',(24.6050898852349,7.43975209375375,0.));
#253556=CARTESIAN_POINT('Ctrl Pts',(24.6050898852349,7.43975209375375,12.));
#253557=CARTESIAN_POINT('Ctrl Pts',(24.6322649369472,7.43401770489221,0.));
#253558=CARTESIAN_POINT('Ctrl Pts',(24.6322649369472,7.43401770489221,12.));
#253559=CARTESIAN_POINT('Ctrl Pts',(24.659495712869,7.42820762158681,0.));
#253560=CARTESIAN_POINT('Ctrl Pts',(24.659495712869,7.42820762158681,12.));
#253561=CARTESIAN_POINT('Ctrl Pts',(24.6867816727118,7.42232167765763,0.));
#253562=CARTESIAN_POINT('Ctrl Pts',(24.6867816727118,7.42232167765763,12.));
#253563=CARTESIAN_POINT('Ctrl Pts',(24.7141222949988,7.41635971481243,0.));
#253564=CARTESIAN_POINT('Ctrl Pts',(24.7141222949988,7.41635971481243,12.));
#253565=CARTESIAN_POINT('Ctrl Pts',(24.7415170994754,7.41032159082173,0.));
#253566=CARTESIAN_POINT('Ctrl Pts',(24.7415170994754,7.41032159082173,12.));
#253567=CARTESIAN_POINT('Ctrl Pts',(24.7689656669005,7.40420718661755,0.));
#253568=CARTESIAN_POINT('Ctrl Pts',(24.7689656669005,7.40420718661755,12.));
#253569=CARTESIAN_POINT('Ctrl Pts',(24.7964676646518,7.39801641583613,0.));
#253570=CARTESIAN_POINT('Ctrl Pts',(24.7964676646518,7.39801641583613,12.));
#253571=CARTESIAN_POINT('Ctrl Pts',(24.8240228521042,7.39174922586841,0.));
#253572=CARTESIAN_POINT('Ctrl Pts',(24.8240228521042,7.39174922586841,12.));
#253573=CARTESIAN_POINT('Ctrl Pts',(24.8516310625367,7.38540558904946,0.));
#253574=CARTESIAN_POINT('Ctrl Pts',(24.8516310625367,7.38540558904946,12.));
#253575=CARTESIAN_POINT('Ctrl Pts',(24.8792921911309,7.3789854964161,0.));
#253576=CARTESIAN_POINT('Ctrl Pts',(24.8792921911309,7.3789854964161,12.));
#253577=CARTESIAN_POINT('Ctrl Pts',(24.9014633826201,7.37378825962718,0.));
#253578=CARTESIAN_POINT('Ctrl Pts',(24.9014633826201,7.37378825962718,12.));
#253579=CARTESIAN_POINT('Ctrl Pts',(24.9181155530631,7.36985593120697,0.));
#253580=CARTESIAN_POINT('Ctrl Pts',(24.9181155530631,7.36985593120697,12.));
#253581=CARTESIAN_POINT('Ctrl Pts',(24.9292275670705,7.3672190902906,0.));
#253582=CARTESIAN_POINT('Ctrl Pts',(24.9292275670705,7.3672190902906,12.));
#253583=CARTESIAN_POINT('Ctrl Pts',(24.9347862158358,7.36589684767344,0.));
#253584=CARTESIAN_POINT('Ctrl Pts',(24.9347862158358,7.36589684767344,12.));
#253585=CARTESIAN_POINT('',(24.9347862158358,7.36589684767344,0.));
#253586=CARTESIAN_POINT('Ctrl Pts',(21.2610617890679,7.52250298901264,0.));
#253587=CARTESIAN_POINT('Ctrl Pts',(21.2610673466886,7.5225064970397,0.));
#253588=CARTESIAN_POINT('Ctrl Pts',(21.2611204474866,7.52252744144904,0.));
#253589=CARTESIAN_POINT('Ctrl Pts',(21.261326054066,7.52260064231661,0.));
#253590=CARTESIAN_POINT('Ctrl Pts',(21.2618521283555,7.5227818224267,0.));
#253591=CARTESIAN_POINT('Ctrl Pts',(21.262927782038,7.52314642316199,0.));
#253592=CARTESIAN_POINT('Ctrl Pts',(21.2644161259962,7.52364573027553,0.));
#253593=CARTESIAN_POINT('Ctrl Pts',(21.2663059157058,7.52427261074298,0.));
#253594=CARTESIAN_POINT('Ctrl Pts',(21.2685823838671,7.52501770333531,0.));
#253595=CARTESIAN_POINT('Ctrl Pts',(21.2712301573466,7.5258712609553,0.));
#253596=CARTESIAN_POINT('Ctrl Pts',(21.2742366113579,7.52682526918541,0.));
#253597=CARTESIAN_POINT('Ctrl Pts',(21.2775925269652,7.52787386225333,0.));
#253598=CARTESIAN_POINT('Ctrl Pts',(21.2812902781143,7.52901217930408,0.));
#253599=CARTESIAN_POINT('Ctrl Pts',(21.2853226580657,7.5302356243823,0.));
#253600=CARTESIAN_POINT('Ctrl Pts',(21.2896816163842,7.53153906987856,0.));
#253601=CARTESIAN_POINT('Ctrl Pts',(21.2943588989331,7.53291726078527,0.));
#253602=CARTESIAN_POINT('Ctrl Pts',(21.2993464250717,7.53436505309943,0.));
#253603=CARTESIAN_POINT('Ctrl Pts',(21.3046368712157,7.53587778251736,0.));
#253604=CARTESIAN_POINT('Ctrl Pts',(21.310223716773,7.53745129364616,0.));
#253605=CARTESIAN_POINT('Ctrl Pts',(21.3161009456256,7.53908175169899,0.));
#253606=CARTESIAN_POINT('Ctrl Pts',(21.3222628524165,7.54076552038279,0.));
#253607=CARTESIAN_POINT('Ctrl Pts',(21.328703791771,7.54249900377031,0.));
#253608=CARTESIAN_POINT('Ctrl Pts',(21.3354182340149,7.54427868151268,0.));
#253609=CARTESIAN_POINT('Ctrl Pts',(21.3424008295038,7.54610114948347,0.));
#253610=CARTESIAN_POINT('Ctrl Pts',(21.3496464761531,7.54796316246331,0.));
#253611=CARTESIAN_POINT('Ctrl Pts',(21.3571503685855,7.5498616652131,0.));
#253612=CARTESIAN_POINT('Ctrl Pts',(21.3649079431865,7.55179375777444,0.));
#253613=CARTESIAN_POINT('Ctrl Pts',(21.3729148390243,7.55375667080029,0.));
#253614=CARTESIAN_POINT('Ctrl Pts',(21.3811668478932,7.55574773403503,0.));
#253615=CARTESIAN_POINT('Ctrl Pts',(21.3896598842117,7.55776435731417,0.));
#253616=CARTESIAN_POINT('Ctrl Pts',(21.3983899952987,7.55980403700611,0.));
#253617=CARTESIAN_POINT('Ctrl Pts',(21.4073533630365,7.56186435703622,0.));
#253618=CARTESIAN_POINT('Ctrl Pts',(21.4165463106254,7.56394299313685,0.));
#253619=CARTESIAN_POINT('Ctrl Pts',(21.4259653015736,7.56603771218712,0.));
#253620=CARTESIAN_POINT('Ctrl Pts',(21.4356069261513,7.56814636360848,0.));
#253621=CARTESIAN_POINT('Ctrl Pts',(21.4454678907509,7.57026687261166,0.));
#253622=CARTESIAN_POINT('Ctrl Pts',(21.4555450053142,7.57239723223506,0.));
#253623=CARTESIAN_POINT('Ctrl Pts',(21.4658351740128,7.57453549743412,0.));
#253624=CARTESIAN_POINT('Ctrl Pts',(21.4763353936762,7.57667978402987,0.));
#253625=CARTESIAN_POINT('Ctrl Pts',(21.4870427508194,7.57882826679132,0.));
#253626=CARTESIAN_POINT('Ctrl Pts',(21.4979544192744,7.58097917790744,0.));
#253627=CARTESIAN_POINT('Ctrl Pts',(21.5090676573873,7.5831308051918,0.));
#253628=CARTESIAN_POINT('Ctrl Pts',(21.5203798035299,7.5852814891913,0.));
#253629=CARTESIAN_POINT('Ctrl Pts',(21.5318882716736,7.58742962034834,0.));
#253630=CARTESIAN_POINT('Ctrl Pts',(21.543590547011,7.58957363620014,0.));
#253631=CARTESIAN_POINT('Ctrl Pts',(21.5554841813462,7.59171201844777,0.));
#253632=CARTESIAN_POINT('Ctrl Pts',(21.5675667904726,7.59384329124918,0.));
#253633=CARTESIAN_POINT('Ctrl Pts',(21.5798360518978,7.59596601973584,0.));
#253634=CARTESIAN_POINT('Ctrl Pts',(21.5922897024466,7.59807880846195,0.));
#253635=CARTESIAN_POINT('Ctrl Pts',(21.6049255358843,7.60018029988241,0.));
#253636=CARTESIAN_POINT('Ctrl Pts',(21.617741400599,7.60226917285429,0.));
#253637=CARTESIAN_POINT('Ctrl Pts',(21.6307351973822,7.60434414118296,0.));
#253638=CARTESIAN_POINT('Ctrl Pts',(21.6439048771743,7.60640395216357,0.));
#253639=CARTESIAN_POINT('Ctrl Pts',(21.6572484388081,7.60844738512874,0.));
#253640=CARTESIAN_POINT('Ctrl Pts',(21.6707639267576,7.61047325000956,0.));
#253641=CARTESIAN_POINT('Ctrl Pts',(21.6844494295815,7.61248038630269,0.));
#253642=CARTESIAN_POINT('Ctrl Pts',(21.6983030783322,7.61446766202787,0.));
#253643=CARTESIAN_POINT('Ctrl Pts',(21.7123230449834,7.61643397270421,0.));
#253644=CARTESIAN_POINT('Ctrl Pts',(21.7265075407975,7.61837824030538,0.));
#253645=CARTESIAN_POINT('Ctrl Pts',(21.7408548148656,7.62029941230855,0.));
#253646=CARTESIAN_POINT('Ctrl Pts',(21.7553631528328,7.62219646084229,0.));
#253647=CARTESIAN_POINT('Ctrl Pts',(21.7700308755584,7.62406838181166,0.));
#253648=CARTESIAN_POINT('Ctrl Pts',(21.7848563378021,7.62591419404513,0.));
#253649=CARTESIAN_POINT('Ctrl Pts',(21.799837926858,7.62773293842389,0.));
#253650=CARTESIAN_POINT('Ctrl Pts',(21.814974061509,7.62952367718127,0.));
#253651=CARTESIAN_POINT('Ctrl Pts',(21.8302631910195,7.63128549323023,0.));
#253652=CARTESIAN_POINT('Ctrl Pts',(21.8457037941084,7.63301748948936,0.));
#253653=CARTESIAN_POINT('Ctrl Pts',(21.8612943779089,7.63471878821226,0.));
#253654=CARTESIAN_POINT('Ctrl Pts',(21.8770334769496,7.636388530334,0.));
#253655=CARTESIAN_POINT('Ctrl Pts',(21.8929196523514,7.63802587492035,0.));
#253656=CARTESIAN_POINT('Ctrl Pts',(21.9089514909874,7.63962999860927,0.));
#253657=CARTESIAN_POINT('Ctrl Pts',(21.9251276046545,7.64120009506532,0.));
#253658=CARTESIAN_POINT('Ctrl Pts',(21.9414466292072,7.64273537442682,0.));
#253659=CARTESIAN_POINT('Ctrl Pts',(21.9579072237651,7.64423506279123,0.));
#253660=CARTESIAN_POINT('Ctrl Pts',(21.9745080700798,7.64569840177336,0.));
#253661=CARTESIAN_POINT('Ctrl Pts',(21.9912478718542,7.6471246480525,0.));
#253662=CARTESIAN_POINT('Ctrl Pts',(22.0081253540774,7.64851307293352,0.));
#253663=CARTESIAN_POINT('Ctrl Pts',(22.0251392623209,7.64986296190169,0.));
#253664=CARTESIAN_POINT('Ctrl Pts',(22.0422883621174,7.65117361421359,0.));
#253665=CARTESIAN_POINT('Ctrl Pts',(22.0595714384431,7.65244434253113,0.));
#253666=CARTESIAN_POINT('Ctrl Pts',(22.0769872951596,7.65367447254949,0.));
#253667=CARTESIAN_POINT('Ctrl Pts',(22.094534754469,7.65486334263644,0.));
#253668=CARTESIAN_POINT('Ctrl Pts',(22.1122126563329,7.65601030346807,0.));
#253669=CARTESIAN_POINT('Ctrl Pts',(22.1300198579675,7.65711471769397,0.));
#253670=CARTESIAN_POINT('Ctrl Pts',(22.1479552334211,7.65817595963349,0.));
#253671=CARTESIAN_POINT('Ctrl Pts',(22.1660176731178,7.65919341496931,0.));
#253672=CARTESIAN_POINT('Ctrl Pts',(22.1842060834091,7.66016648045005,0.));
#253673=CARTESIAN_POINT('Ctrl Pts',(22.2025193860964,7.66109456359271,0.));
#253674=CARTESIAN_POINT('Ctrl Pts',(22.2209565180085,7.661977082404,0.));
#253675=CARTESIAN_POINT('Ctrl Pts',(22.2395164306547,7.66281346512509,0.));
#253676=CARTESIAN_POINT('Ctrl Pts',(22.258198089848,7.66360314997641,0.));
#253677=CARTESIAN_POINT('Ctrl Pts',(22.2770004753335,7.66434558490979,0.));
#253678=CARTESIAN_POINT('Ctrl Pts',(22.2959225803937,7.66504022736299,0.));
#253679=CARTESIAN_POINT('Ctrl Pts',(22.314963411484,7.66568654402494,0.));
#253680=CARTESIAN_POINT('Ctrl Pts',(22.3341219879469,7.66628401061952,0.));
#253681=CARTESIAN_POINT('Ctrl Pts',(22.3533973417021,7.66683211169159,0.));
#253682=CARTESIAN_POINT('Ctrl Pts',(22.372788516936,7.66733034039883,0.));
#253683=CARTESIAN_POINT('Ctrl Pts',(22.3922945697773,7.6677781983079,0.));
#253684=CARTESIAN_POINT('Ctrl Pts',(22.4119145679758,7.6681751951964,0.));
#253685=CARTESIAN_POINT('Ctrl Pts',(22.4316475906603,7.66852084886704,0.));
#253686=CARTESIAN_POINT('Ctrl Pts',(22.4514927280855,7.66881468496635,0.));
#253687=CARTESIAN_POINT('Ctrl Pts',(22.4714490813699,7.66905623680831,0.));
#253688=CARTESIAN_POINT('Ctrl Pts',(22.4915157622312,7.66924504520315,0.));
#253689=CARTESIAN_POINT('Ctrl Pts',(22.5116918927031,7.66938065829108,0.));
#253690=CARTESIAN_POINT('Ctrl Pts',(22.53197660492,7.66946263138144,0.));
#253691=CARTESIAN_POINT('Ctrl Pts',(22.5523690409116,7.66949052679693,0.));
#253692=CARTESIAN_POINT('Ctrl Pts',(22.5728683523831,7.66946391372306,0.));
#253693=CARTESIAN_POINT('Ctrl Pts',(22.5934737004953,7.66938236806233,0.));
#253694=CARTESIAN_POINT('Ctrl Pts',(22.6141842556243,7.66924547229414,0.));
#253695=CARTESIAN_POINT('Ctrl Pts',(22.6349991971541,7.66905281533715,0.));
#253696=CARTESIAN_POINT('Ctrl Pts',(22.6559177133127,7.66880399241323,0.));
#253697=CARTESIAN_POINT('Ctrl Pts',(22.6769390009885,7.66849860491743,0.));
#253698=CARTESIAN_POINT('Ctrl Pts',(22.6980622655446,7.66813626029275,0.));
#253699=CARTESIAN_POINT('Ctrl Pts',(22.7192867206245,7.66771657191028,0.));
#253700=CARTESIAN_POINT('Ctrl Pts',(22.7406115879513,7.6672391589544,0.));
#253701=CARTESIAN_POINT('Ctrl Pts',(22.7620360971843,7.66670364630299,0.));
#253702=CARTESIAN_POINT('Ctrl Pts',(22.7835594857699,7.66610966441273,0.));
#253703=CARTESIAN_POINT('Ctrl Pts',(22.8051809987833,7.66545684920987,0.));
#253704=CARTESIAN_POINT('Ctrl Pts',(22.8268998887678,7.66474484198549,0.));
#253705=CARTESIAN_POINT('Ctrl Pts',(22.848715415557,7.66397328929803,0.));
#253706=CARTESIAN_POINT('Ctrl Pts',(22.8706268461283,7.66314184287337,0.));
#253707=CARTESIAN_POINT('Ctrl Pts',(22.8926334544883,7.66225015950156,0.));
#253708=CARTESIAN_POINT('Ctrl Pts',(22.9147345215421,7.66129790094108,0.));
#253709=CARTESIAN_POINT('Ctrl Pts',(22.9369293349593,7.66028473382778,0.));
#253710=CARTESIAN_POINT('Ctrl Pts',(22.959217189033,7.65921032958902,0.));
#253711=CARTESIAN_POINT('Ctrl Pts',(22.9815973845296,7.65807436436432,0.));
#253712=CARTESIAN_POINT('Ctrl Pts',(23.0040692285814,7.65687651891305,0.));
#253713=CARTESIAN_POINT('Ctrl Pts',(23.0266320345787,7.65561647852534,0.));
#253714=CARTESIAN_POINT('Ctrl Pts',(23.0492851220528,7.65429393293946,0.));
#253715=CARTESIAN_POINT('Ctrl Pts',(23.072027816555,7.65290857626358,0.));
#253716=CARTESIAN_POINT('Ctrl Pts',(23.094859449525,7.65146010690476,0.));
#253717=CARTESIAN_POINT('Ctrl Pts',(23.1177793581679,7.6499482274986,0.));
#253718=CARTESIAN_POINT('Ctrl Pts',(23.1407868853819,7.64837264482943,0.));
#253719=CARTESIAN_POINT('Ctrl Pts',(23.1638813796694,7.64673306975805,0.));
#253720=CARTESIAN_POINT('Ctrl Pts',(23.1870621950452,7.64502921715483,0.));
#253721=CARTESIAN_POINT('Ctrl Pts',(23.2103286909398,7.6432608058368,0.));
#253722=CARTESIAN_POINT('Ctrl Pts',(23.2336802320912,7.64142755851505,0.));
#253723=CARTESIAN_POINT('Ctrl Pts',(23.2571161884488,7.63952920172835,0.));
#253724=CARTESIAN_POINT('Ctrl Pts',(23.2806359350855,7.63756546576374,0.));
#253725=CARTESIAN_POINT('Ctrl Pts',(23.3042388521022,7.63553608458783,0.));
#253726=CARTESIAN_POINT('Ctrl Pts',(23.3279243245241,7.63344079578162,0.));
#253727=CARTESIAN_POINT('Ctrl Pts',(23.3516917421972,7.63127934048137,0.));
#253728=CARTESIAN_POINT('Ctrl Pts',(23.3755404996636,7.62905146332593,0.));
#253729=CARTESIAN_POINT('Ctrl Pts',(23.399469996112,7.62675691240329,0.));
#253730=CARTESIAN_POINT('Ctrl Pts',(23.4234796353542,7.6243954392005,0.));
#253731=CARTESIAN_POINT('Ctrl Pts',(23.4475688257854,7.62196679855955,0.));
#253732=CARTESIAN_POINT('Ctrl Pts',(23.4717369803438,7.61947074863977,0.));
#253733=CARTESIAN_POINT('Ctrl Pts',(23.4959835164609,7.61690705088319,0.));
#253734=CARTESIAN_POINT('Ctrl Pts',(23.5203078560129,7.61427546999298,0.));
#253735=CARTESIAN_POINT('Ctrl Pts',(23.544709425203,7.61157577385372,0.));
#253736=CARTESIAN_POINT('Ctrl Pts',(23.5691876544244,7.608807733446,0.));
#253737=CARTESIAN_POINT('Ctrl Pts',(23.5937419781245,7.60597112277094,0.));
#253738=CARTESIAN_POINT('Ctrl Pts',(23.6183718346576,7.60306571877806,0.));
#253739=CARTESIAN_POINT('Ctrl Pts',(23.6430766661418,7.60009130130126,0.));
#253740=CARTESIAN_POINT('Ctrl Pts',(23.6678559182875,7.59704765299567,0.));
#253741=CARTESIAN_POINT('Ctrl Pts',(23.6927090405066,7.59393455934035,0.));
#253742=CARTESIAN_POINT('Ctrl Pts',(23.7176354860456,7.59075180865321,0.));
#253743=CARTESIAN_POINT('Ctrl Pts',(23.7426347121006,7.58749919210826,0.));
#253744=CARTESIAN_POINT('Ctrl Pts',(23.7677061799376,7.58417650376271,0.));
#253745=CARTESIAN_POINT('Ctrl Pts',(23.7928493549908,7.58078354058213,0.));
#253746=CARTESIAN_POINT('Ctrl Pts',(23.8180637069976,7.57732010249066,0.));
#253747=CARTESIAN_POINT('Ctrl Pts',(23.8433487096132,7.57378599219814,0.));
#253748=CARTESIAN_POINT('Ctrl Pts',(23.8687038399595,7.57018101500709,0.));
#253749=CARTESIAN_POINT('Ctrl Pts',(23.8941285782002,7.56650497863791,0.));
#253750=CARTESIAN_POINT('Ctrl Pts',(23.9196224070759,7.56275769304773,0.));
#253751=CARTESIAN_POINT('Ctrl Pts',(23.9451848115002,7.5589389702768,0.));
#253752=CARTESIAN_POINT('Ctrl Pts',(23.9708152779886,7.55504862424808,0.));
#253753=CARTESIAN_POINT('Ctrl Pts',(23.9965132953187,7.55108647097432,0.));
#253754=CARTESIAN_POINT('Ctrl Pts',(24.0222783554531,7.54705232885895,0.));
#253755=CARTESIAN_POINT('Ctrl Pts',(24.0481099543353,7.54294601896128,0.));
#253756=CARTESIAN_POINT('Ctrl Pts',(24.0740075927984,7.53876736531005,0.));
#253757=CARTESIAN_POINT('Ctrl Pts',(24.0999707772642,7.53451619514659,0.));
#253758=CARTESIAN_POINT('Ctrl Pts',(24.1259990209211,7.53019233935537,0.));
#253759=CARTESIAN_POINT('Ctrl Pts',(24.152091842537,7.52579563201479,0.));
#253760=CARTESIAN_POINT('Ctrl Pts',(24.1782487641602,7.52132590953863,0.));
#253761=CARTESIAN_POINT('Ctrl Pts',(24.2044693092356,7.51678300997998,0.));
#253762=CARTESIAN_POINT('Ctrl Pts',(24.230753000389,7.51216677222199,0.));
#253763=CARTESIAN_POINT('Ctrl Pts',(24.2570993577032,7.50747703535115,0.));
#253764=CARTESIAN_POINT('Ctrl Pts',(24.2835078958966,7.50271363765099,0.));
#253765=CARTESIAN_POINT('Ctrl Pts',(24.3099781253345,7.49787641695359,0.));
#253766=CARTESIAN_POINT('Ctrl Pts',(24.3365095573673,7.4929652125233,0.));
#253767=CARTESIAN_POINT('Ctrl Pts',(24.3631017084513,7.48797986651828,0.));
#253768=CARTESIAN_POINT('Ctrl Pts',(24.3897541049248,7.48292022569254,0.));
#253769=CARTESIAN_POINT('Ctrl Pts',(24.4164662871165,7.47778614286574,0.));
#253770=CARTESIAN_POINT('Ctrl Pts',(24.4432378146501,7.47257747883319,0.));
#253771=CARTESIAN_POINT('Ctrl Pts',(24.4700682684544,7.46729410308923,0.));
#253772=CARTESIAN_POINT('Ctrl Pts',(24.4969572391509,7.46193588961642,0.));
#253773=CARTESIAN_POINT('Ctrl Pts',(24.52390431731,7.45650271336046,0.));
#253774=CARTESIAN_POINT('Ctrl Pts',(24.5509090831579,7.45099444651296,0.));
#253775=CARTESIAN_POINT('Ctrl Pts',(24.5779710960865,7.44541095473163,0.));
#253776=CARTESIAN_POINT('Ctrl Pts',(24.6050898852349,7.43975209375375,0.));
#253777=CARTESIAN_POINT('Ctrl Pts',(24.6322649369472,7.43401770489221,0.));
#253778=CARTESIAN_POINT('Ctrl Pts',(24.659495712869,7.42820762158681,0.));
#253779=CARTESIAN_POINT('Ctrl Pts',(24.6867816727118,7.42232167765763,0.));
#253780=CARTESIAN_POINT('Ctrl Pts',(24.7141222949988,7.41635971481243,0.));
#253781=CARTESIAN_POINT('Ctrl Pts',(24.7415170994754,7.41032159082173,0.));
#253782=CARTESIAN_POINT('Ctrl Pts',(24.7689656669005,7.40420718661755,0.));
#253783=CARTESIAN_POINT('Ctrl Pts',(24.7964676646518,7.39801641583613,0.));
#253784=CARTESIAN_POINT('Ctrl Pts',(24.8240228521042,7.39174922586841,0.));
#253785=CARTESIAN_POINT('Ctrl Pts',(24.8516310625367,7.38540558904946,0.));
#253786=CARTESIAN_POINT('Ctrl Pts',(24.8792921911309,7.3789854964161,0.));
#253787=CARTESIAN_POINT('Ctrl Pts',(24.9014633826201,7.37378825962718,0.));
#253788=CARTESIAN_POINT('Ctrl Pts',(24.9181155530631,7.36985593120697,0.));
#253789=CARTESIAN_POINT('Ctrl Pts',(24.9292275670705,7.3672190902906,0.));
#253790=CARTESIAN_POINT('Ctrl Pts',(24.9347862158358,7.36589684767344,0.));
#253791=CARTESIAN_POINT('',(24.9347862158358,7.36589684767344,12.));
#253792=CARTESIAN_POINT('Ctrl Pts',(24.9347862158358,7.36589684767344,12.));
#253793=CARTESIAN_POINT('Ctrl Pts',(24.9292275670705,7.3672190902906,12.));
#253794=CARTESIAN_POINT('Ctrl Pts',(24.9181155530631,7.36985593120697,12.));
#253795=CARTESIAN_POINT('Ctrl Pts',(24.9014633826201,7.37378825962718,12.));
#253796=CARTESIAN_POINT('Ctrl Pts',(24.8792921911309,7.3789854964161,12.));
#253797=CARTESIAN_POINT('Ctrl Pts',(24.8516310625367,7.38540558904946,12.));
#253798=CARTESIAN_POINT('Ctrl Pts',(24.8240228521042,7.39174922586841,12.));
#253799=CARTESIAN_POINT('Ctrl Pts',(24.7964676646518,7.39801641583613,12.));
#253800=CARTESIAN_POINT('Ctrl Pts',(24.7689656669005,7.40420718661755,12.));
#253801=CARTESIAN_POINT('Ctrl Pts',(24.7415170994754,7.41032159082173,12.));
#253802=CARTESIAN_POINT('Ctrl Pts',(24.7141222949988,7.41635971481243,12.));
#253803=CARTESIAN_POINT('Ctrl Pts',(24.6867816727118,7.42232167765763,12.));
#253804=CARTESIAN_POINT('Ctrl Pts',(24.659495712869,7.42820762158681,12.));
#253805=CARTESIAN_POINT('Ctrl Pts',(24.6322649369472,7.43401770489221,12.));
#253806=CARTESIAN_POINT('Ctrl Pts',(24.6050898852349,7.43975209375375,12.));
#253807=CARTESIAN_POINT('Ctrl Pts',(24.5779710960865,7.44541095473163,12.));
#253808=CARTESIAN_POINT('Ctrl Pts',(24.5509090831579,7.45099444651296,12.));
#253809=CARTESIAN_POINT('Ctrl Pts',(24.52390431731,7.45650271336046,12.));
#253810=CARTESIAN_POINT('Ctrl Pts',(24.4969572391509,7.46193588961642,12.));
#253811=CARTESIAN_POINT('Ctrl Pts',(24.4700682684544,7.46729410308923,12.));
#253812=CARTESIAN_POINT('Ctrl Pts',(24.4432378146501,7.47257747883319,12.));
#253813=CARTESIAN_POINT('Ctrl Pts',(24.4164662871165,7.47778614286574,12.));
#253814=CARTESIAN_POINT('Ctrl Pts',(24.3897541049248,7.48292022569254,12.));
#253815=CARTESIAN_POINT('Ctrl Pts',(24.3631017084513,7.48797986651828,12.));
#253816=CARTESIAN_POINT('Ctrl Pts',(24.3365095573673,7.4929652125233,12.));
#253817=CARTESIAN_POINT('Ctrl Pts',(24.3099781253345,7.49787641695359,12.));
#253818=CARTESIAN_POINT('Ctrl Pts',(24.2835078958966,7.50271363765099,12.));
#253819=CARTESIAN_POINT('Ctrl Pts',(24.2570993577032,7.50747703535115,12.));
#253820=CARTESIAN_POINT('Ctrl Pts',(24.230753000389,7.51216677222199,12.));
#253821=CARTESIAN_POINT('Ctrl Pts',(24.2044693092356,7.51678300997998,12.));
#253822=CARTESIAN_POINT('Ctrl Pts',(24.1782487641602,7.52132590953863,12.));
#253823=CARTESIAN_POINT('Ctrl Pts',(24.152091842537,7.52579563201479,12.));
#253824=CARTESIAN_POINT('Ctrl Pts',(24.1259990209211,7.53019233935537,12.));
#253825=CARTESIAN_POINT('Ctrl Pts',(24.0999707772642,7.53451619514659,12.));
#253826=CARTESIAN_POINT('Ctrl Pts',(24.0740075927984,7.53876736531005,12.));
#253827=CARTESIAN_POINT('Ctrl Pts',(24.0481099543353,7.54294601896128,12.));
#253828=CARTESIAN_POINT('Ctrl Pts',(24.0222783554531,7.54705232885895,12.));
#253829=CARTESIAN_POINT('Ctrl Pts',(23.9965132953187,7.55108647097432,12.));
#253830=CARTESIAN_POINT('Ctrl Pts',(23.9708152779886,7.55504862424808,12.));
#253831=CARTESIAN_POINT('Ctrl Pts',(23.9451848115002,7.5589389702768,12.));
#253832=CARTESIAN_POINT('Ctrl Pts',(23.9196224070759,7.56275769304773,12.));
#253833=CARTESIAN_POINT('Ctrl Pts',(23.8941285782002,7.56650497863791,12.));
#253834=CARTESIAN_POINT('Ctrl Pts',(23.8687038399595,7.57018101500709,12.));
#253835=CARTESIAN_POINT('Ctrl Pts',(23.8433487096132,7.57378599219814,12.));
#253836=CARTESIAN_POINT('Ctrl Pts',(23.8180637069976,7.57732010249066,12.));
#253837=CARTESIAN_POINT('Ctrl Pts',(23.7928493549908,7.58078354058213,12.));
#253838=CARTESIAN_POINT('Ctrl Pts',(23.7677061799376,7.58417650376271,12.));
#253839=CARTESIAN_POINT('Ctrl Pts',(23.7426347121006,7.58749919210826,12.));
#253840=CARTESIAN_POINT('Ctrl Pts',(23.7176354860456,7.59075180865321,12.));
#253841=CARTESIAN_POINT('Ctrl Pts',(23.6927090405066,7.59393455934035,12.));
#253842=CARTESIAN_POINT('Ctrl Pts',(23.6678559182875,7.59704765299567,12.));
#253843=CARTESIAN_POINT('Ctrl Pts',(23.6430766661418,7.60009130130126,12.));
#253844=CARTESIAN_POINT('Ctrl Pts',(23.6183718346576,7.60306571877806,12.));
#253845=CARTESIAN_POINT('Ctrl Pts',(23.5937419781245,7.60597112277094,12.));
#253846=CARTESIAN_POINT('Ctrl Pts',(23.5691876544244,7.608807733446,12.));
#253847=CARTESIAN_POINT('Ctrl Pts',(23.544709425203,7.61157577385372,12.));
#253848=CARTESIAN_POINT('Ctrl Pts',(23.5203078560129,7.61427546999298,12.));
#253849=CARTESIAN_POINT('Ctrl Pts',(23.4959835164609,7.61690705088319,12.));
#253850=CARTESIAN_POINT('Ctrl Pts',(23.4717369803438,7.61947074863977,12.));
#253851=CARTESIAN_POINT('Ctrl Pts',(23.4475688257854,7.62196679855955,12.));
#253852=CARTESIAN_POINT('Ctrl Pts',(23.4234796353542,7.6243954392005,12.));
#253853=CARTESIAN_POINT('Ctrl Pts',(23.399469996112,7.62675691240329,12.));
#253854=CARTESIAN_POINT('Ctrl Pts',(23.3755404996636,7.62905146332593,12.));
#253855=CARTESIAN_POINT('Ctrl Pts',(23.3516917421972,7.63127934048137,12.));
#253856=CARTESIAN_POINT('Ctrl Pts',(23.3279243245241,7.63344079578162,12.));
#253857=CARTESIAN_POINT('Ctrl Pts',(23.3042388521022,7.63553608458783,12.));
#253858=CARTESIAN_POINT('Ctrl Pts',(23.2806359350855,7.63756546576374,12.));
#253859=CARTESIAN_POINT('Ctrl Pts',(23.2571161884488,7.63952920172835,12.));
#253860=CARTESIAN_POINT('Ctrl Pts',(23.2336802320912,7.64142755851505,12.));
#253861=CARTESIAN_POINT('Ctrl Pts',(23.2103286909398,7.6432608058368,12.));
#253862=CARTESIAN_POINT('Ctrl Pts',(23.1870621950452,7.64502921715483,12.));
#253863=CARTESIAN_POINT('Ctrl Pts',(23.1638813796694,7.64673306975805,12.));
#253864=CARTESIAN_POINT('Ctrl Pts',(23.1407868853819,7.64837264482943,12.));
#253865=CARTESIAN_POINT('Ctrl Pts',(23.1177793581679,7.6499482274986,12.));
#253866=CARTESIAN_POINT('Ctrl Pts',(23.094859449525,7.65146010690476,12.));
#253867=CARTESIAN_POINT('Ctrl Pts',(23.072027816555,7.65290857626358,12.));
#253868=CARTESIAN_POINT('Ctrl Pts',(23.0492851220528,7.65429393293946,12.));
#253869=CARTESIAN_POINT('Ctrl Pts',(23.0266320345787,7.65561647852534,12.));
#253870=CARTESIAN_POINT('Ctrl Pts',(23.0040692285814,7.65687651891305,12.));
#253871=CARTESIAN_POINT('Ctrl Pts',(22.9815973845296,7.65807436436432,12.));
#253872=CARTESIAN_POINT('Ctrl Pts',(22.959217189033,7.65921032958902,12.));
#253873=CARTESIAN_POINT('Ctrl Pts',(22.9369293349593,7.66028473382778,12.));
#253874=CARTESIAN_POINT('Ctrl Pts',(22.9147345215421,7.66129790094108,12.));
#253875=CARTESIAN_POINT('Ctrl Pts',(22.8926334544883,7.66225015950156,12.));
#253876=CARTESIAN_POINT('Ctrl Pts',(22.8706268461283,7.66314184287337,12.));
#253877=CARTESIAN_POINT('Ctrl Pts',(22.848715415557,7.66397328929803,12.));
#253878=CARTESIAN_POINT('Ctrl Pts',(22.8268998887678,7.66474484198549,12.));
#253879=CARTESIAN_POINT('Ctrl Pts',(22.8051809987833,7.66545684920987,12.));
#253880=CARTESIAN_POINT('Ctrl Pts',(22.7835594857699,7.66610966441273,12.));
#253881=CARTESIAN_POINT('Ctrl Pts',(22.7620360971843,7.66670364630299,12.));
#253882=CARTESIAN_POINT('Ctrl Pts',(22.7406115879513,7.6672391589544,12.));
#253883=CARTESIAN_POINT('Ctrl Pts',(22.7192867206245,7.66771657191028,12.));
#253884=CARTESIAN_POINT('Ctrl Pts',(22.6980622655446,7.66813626029275,12.));
#253885=CARTESIAN_POINT('Ctrl Pts',(22.6769390009885,7.66849860491743,12.));
#253886=CARTESIAN_POINT('Ctrl Pts',(22.6559177133127,7.66880399241323,12.));
#253887=CARTESIAN_POINT('Ctrl Pts',(22.6349991971541,7.66905281533715,12.));
#253888=CARTESIAN_POINT('Ctrl Pts',(22.6141842556243,7.66924547229414,12.));
#253889=CARTESIAN_POINT('Ctrl Pts',(22.5934737004953,7.66938236806233,12.));
#253890=CARTESIAN_POINT('Ctrl Pts',(22.5728683523831,7.66946391372306,12.));
#253891=CARTESIAN_POINT('Ctrl Pts',(22.5523690409116,7.66949052679693,12.));
#253892=CARTESIAN_POINT('Ctrl Pts',(22.53197660492,7.66946263138144,12.));
#253893=CARTESIAN_POINT('Ctrl Pts',(22.5116918927031,7.66938065829108,12.));
#253894=CARTESIAN_POINT('Ctrl Pts',(22.4915157622312,7.66924504520315,12.));
#253895=CARTESIAN_POINT('Ctrl Pts',(22.4714490813699,7.66905623680831,12.));
#253896=CARTESIAN_POINT('Ctrl Pts',(22.4514927280855,7.66881468496635,12.));
#253897=CARTESIAN_POINT('Ctrl Pts',(22.4316475906603,7.66852084886704,12.));
#253898=CARTESIAN_POINT('Ctrl Pts',(22.4119145679758,7.6681751951964,12.));
#253899=CARTESIAN_POINT('Ctrl Pts',(22.3922945697773,7.6677781983079,12.));
#253900=CARTESIAN_POINT('Ctrl Pts',(22.372788516936,7.66733034039883,12.));
#253901=CARTESIAN_POINT('Ctrl Pts',(22.3533973417021,7.66683211169159,12.));
#253902=CARTESIAN_POINT('Ctrl Pts',(22.3341219879469,7.66628401061952,12.));
#253903=CARTESIAN_POINT('Ctrl Pts',(22.314963411484,7.66568654402494,12.));
#253904=CARTESIAN_POINT('Ctrl Pts',(22.2959225803937,7.66504022736299,12.));
#253905=CARTESIAN_POINT('Ctrl Pts',(22.2770004753335,7.66434558490979,12.));
#253906=CARTESIAN_POINT('Ctrl Pts',(22.258198089848,7.66360314997641,12.));
#253907=CARTESIAN_POINT('Ctrl Pts',(22.2395164306547,7.66281346512509,12.));
#253908=CARTESIAN_POINT('Ctrl Pts',(22.2209565180085,7.661977082404,12.));
#253909=CARTESIAN_POINT('Ctrl Pts',(22.2025193860964,7.66109456359271,12.));
#253910=CARTESIAN_POINT('Ctrl Pts',(22.1842060834091,7.66016648045005,12.));
#253911=CARTESIAN_POINT('Ctrl Pts',(22.1660176731178,7.65919341496931,12.));
#253912=CARTESIAN_POINT('Ctrl Pts',(22.1479552334211,7.65817595963349,12.));
#253913=CARTESIAN_POINT('Ctrl Pts',(22.1300198579675,7.65711471769397,12.));
#253914=CARTESIAN_POINT('Ctrl Pts',(22.1122126563329,7.65601030346807,12.));
#253915=CARTESIAN_POINT('Ctrl Pts',(22.094534754469,7.65486334263644,12.));
#253916=CARTESIAN_POINT('Ctrl Pts',(22.0769872951596,7.65367447254949,12.));
#253917=CARTESIAN_POINT('Ctrl Pts',(22.0595714384431,7.65244434253113,12.));
#253918=CARTESIAN_POINT('Ctrl Pts',(22.0422883621174,7.65117361421359,12.));
#253919=CARTESIAN_POINT('Ctrl Pts',(22.0251392623209,7.64986296190169,12.));
#253920=CARTESIAN_POINT('Ctrl Pts',(22.0081253540774,7.64851307293352,12.));
#253921=CARTESIAN_POINT('Ctrl Pts',(21.9912478718542,7.6471246480525,12.));
#253922=CARTESIAN_POINT('Ctrl Pts',(21.9745080700798,7.64569840177336,12.));
#253923=CARTESIAN_POINT('Ctrl Pts',(21.9579072237651,7.64423506279123,12.));
#253924=CARTESIAN_POINT('Ctrl Pts',(21.9414466292072,7.64273537442682,12.));
#253925=CARTESIAN_POINT('Ctrl Pts',(21.9251276046545,7.64120009506532,12.));
#253926=CARTESIAN_POINT('Ctrl Pts',(21.9089514909874,7.63962999860927,12.));
#253927=CARTESIAN_POINT('Ctrl Pts',(21.8929196523514,7.63802587492035,12.));
#253928=CARTESIAN_POINT('Ctrl Pts',(21.8770334769496,7.636388530334,12.));
#253929=CARTESIAN_POINT('Ctrl Pts',(21.8612943779089,7.63471878821226,12.));
#253930=CARTESIAN_POINT('Ctrl Pts',(21.8457037941084,7.63301748948936,12.));
#253931=CARTESIAN_POINT('Ctrl Pts',(21.8302631910195,7.63128549323023,12.));
#253932=CARTESIAN_POINT('Ctrl Pts',(21.814974061509,7.62952367718127,12.));
#253933=CARTESIAN_POINT('Ctrl Pts',(21.799837926858,7.62773293842389,12.));
#253934=CARTESIAN_POINT('Ctrl Pts',(21.7848563378021,7.62591419404513,12.));
#253935=CARTESIAN_POINT('Ctrl Pts',(21.7700308755584,7.62406838181166,12.));
#253936=CARTESIAN_POINT('Ctrl Pts',(21.7553631528328,7.62219646084229,12.));
#253937=CARTESIAN_POINT('Ctrl Pts',(21.7408548148656,7.62029941230855,12.));
#253938=CARTESIAN_POINT('Ctrl Pts',(21.7265075407975,7.61837824030538,12.));
#253939=CARTESIAN_POINT('Ctrl Pts',(21.7123230449834,7.61643397270421,12.));
#253940=CARTESIAN_POINT('Ctrl Pts',(21.6983030783322,7.61446766202787,12.));
#253941=CARTESIAN_POINT('Ctrl Pts',(21.6844494295815,7.61248038630269,12.));
#253942=CARTESIAN_POINT('Ctrl Pts',(21.6707639267576,7.61047325000956,12.));
#253943=CARTESIAN_POINT('Ctrl Pts',(21.6572484388081,7.60844738512874,12.));
#253944=CARTESIAN_POINT('Ctrl Pts',(21.6439048771743,7.60640395216357,12.));
#253945=CARTESIAN_POINT('Ctrl Pts',(21.6307351973822,7.60434414118296,12.));
#253946=CARTESIAN_POINT('Ctrl Pts',(21.617741400599,7.60226917285429,12.));
#253947=CARTESIAN_POINT('Ctrl Pts',(21.6049255358843,7.60018029988241,12.));
#253948=CARTESIAN_POINT('Ctrl Pts',(21.5922897024466,7.59807880846195,12.));
#253949=CARTESIAN_POINT('Ctrl Pts',(21.5798360518978,7.59596601973584,12.));
#253950=CARTESIAN_POINT('Ctrl Pts',(21.5675667904726,7.59384329124918,12.));
#253951=CARTESIAN_POINT('Ctrl Pts',(21.5554841813462,7.59171201844777,12.));
#253952=CARTESIAN_POINT('Ctrl Pts',(21.543590547011,7.58957363620014,12.));
#253953=CARTESIAN_POINT('Ctrl Pts',(21.5318882716736,7.58742962034834,12.));
#253954=CARTESIAN_POINT('Ctrl Pts',(21.5203798035299,7.5852814891913,12.));
#253955=CARTESIAN_POINT('Ctrl Pts',(21.5090676573873,7.5831308051918,12.));
#253956=CARTESIAN_POINT('Ctrl Pts',(21.4979544192744,7.58097917790744,12.));
#253957=CARTESIAN_POINT('Ctrl Pts',(21.4870427508194,7.57882826679132,12.));
#253958=CARTESIAN_POINT('Ctrl Pts',(21.4763353936762,7.57667978402987,12.));
#253959=CARTESIAN_POINT('Ctrl Pts',(21.4658351740128,7.57453549743412,12.));
#253960=CARTESIAN_POINT('Ctrl Pts',(21.4555450053142,7.57239723223506,12.));
#253961=CARTESIAN_POINT('Ctrl Pts',(21.4454678907509,7.57026687261166,12.));
#253962=CARTESIAN_POINT('Ctrl Pts',(21.4356069261513,7.56814636360848,12.));
#253963=CARTESIAN_POINT('Ctrl Pts',(21.4259653015736,7.56603771218712,12.));
#253964=CARTESIAN_POINT('Ctrl Pts',(21.4165463106254,7.56394299313685,12.));
#253965=CARTESIAN_POINT('Ctrl Pts',(21.4073533630365,7.56186435703622,12.));
#253966=CARTESIAN_POINT('Ctrl Pts',(21.3983899952987,7.55980403700611,12.));
#253967=CARTESIAN_POINT('Ctrl Pts',(21.3896598842117,7.55776435731417,12.));
#253968=CARTESIAN_POINT('Ctrl Pts',(21.3811668478932,7.55574773403503,12.));
#253969=CARTESIAN_POINT('Ctrl Pts',(21.3729148390243,7.55375667080029,12.));
#253970=CARTESIAN_POINT('Ctrl Pts',(21.3649079431865,7.55179375777444,12.));
#253971=CARTESIAN_POINT('Ctrl Pts',(21.3571503685855,7.5498616652131,12.));
#253972=CARTESIAN_POINT('Ctrl Pts',(21.3496464761531,7.54796316246331,12.));
#253973=CARTESIAN_POINT('Ctrl Pts',(21.3424008295038,7.54610114948347,12.));
#253974=CARTESIAN_POINT('Ctrl Pts',(21.3354182340149,7.54427868151268,12.));
#253975=CARTESIAN_POINT('Ctrl Pts',(21.328703791771,7.54249900377031,12.));
#253976=CARTESIAN_POINT('Ctrl Pts',(21.3222628524165,7.54076552038279,12.));
#253977=CARTESIAN_POINT('Ctrl Pts',(21.3161009456256,7.53908175169899,12.));
#253978=CARTESIAN_POINT('Ctrl Pts',(21.310223716773,7.53745129364616,12.));
#253979=CARTESIAN_POINT('Ctrl Pts',(21.3046368712157,7.53587778251736,12.));
#253980=CARTESIAN_POINT('Ctrl Pts',(21.2993464250717,7.53436505309943,12.));
#253981=CARTESIAN_POINT('Ctrl Pts',(21.2943588989331,7.53291726078527,12.));
#253982=CARTESIAN_POINT('Ctrl Pts',(21.2896816163842,7.53153906987856,12.));
#253983=CARTESIAN_POINT('Ctrl Pts',(21.2853226580657,7.5302356243823,12.));
#253984=CARTESIAN_POINT('Ctrl Pts',(21.2812902781143,7.52901217930408,12.));
#253985=CARTESIAN_POINT('Ctrl Pts',(21.2775925269652,7.52787386225333,12.));
#253986=CARTESIAN_POINT('Ctrl Pts',(21.2742366113579,7.52682526918541,12.));
#253987=CARTESIAN_POINT('Ctrl Pts',(21.2712301573466,7.5258712609553,12.));
#253988=CARTESIAN_POINT('Ctrl Pts',(21.2685823838671,7.52501770333531,12.));
#253989=CARTESIAN_POINT('Ctrl Pts',(21.2663059157058,7.52427261074298,12.));
#253990=CARTESIAN_POINT('Ctrl Pts',(21.2644161259962,7.52364573027553,12.));
#253991=CARTESIAN_POINT('Ctrl Pts',(21.262927782038,7.52314642316199,12.));
#253992=CARTESIAN_POINT('Ctrl Pts',(21.2618521283555,7.5227818224267,12.));
#253993=CARTESIAN_POINT('Ctrl Pts',(21.261326054066,7.52260064231661,12.));
#253994=CARTESIAN_POINT('Ctrl Pts',(21.2611204474866,7.52252744144904,12.));
#253995=CARTESIAN_POINT('Ctrl Pts',(21.2610673466886,7.5225064970397,12.));
#253996=CARTESIAN_POINT('Ctrl Pts',(21.2610617890679,7.52250298901264,12.));
#253997=CARTESIAN_POINT('',(24.9347862158358,7.36589684767344,0.));
#253998=CARTESIAN_POINT('Origin',(0.,0.,0.));
#253999=CARTESIAN_POINT('Origin',(0.,0.,0.));
#254000=CARTESIAN_POINT('Origin',(0.,0.,0.));
#254001=CARTESIAN_POINT('Origin',(0.,0.,0.));
#254002=CARTESIAN_POINT('Origin',(0.,0.,0.));
#254003=CARTESIAN_POINT('Origin',(0.,0.,0.));
#254004=CARTESIAN_POINT('Origin',(0.,0.,0.));
#254005=CARTESIAN_POINT('Origin',(0.,0.,0.));
#254006=CARTESIAN_POINT('Origin',(0.,0.,0.));
#254007=CARTESIAN_POINT('Origin',(0.,0.,0.));
#254008=CARTESIAN_POINT('Origin',(0.,0.,0.));
#254009=CARTESIAN_POINT('Origin',(0.,0.,0.));
#254010=CARTESIAN_POINT('Origin',(0.,0.,0.));
#254011=CARTESIAN_POINT('Origin',(0.,0.,0.));
#254012=CARTESIAN_POINT('Origin',(0.,0.,0.));
#254013=CARTESIAN_POINT('Origin',(0.,0.,0.));
#254014=CARTESIAN_POINT('Origin',(0.,0.,0.));
#254015=CARTESIAN_POINT('Origin',(0.,0.,0.));
#254016=CARTESIAN_POINT('Origin',(0.,0.,0.));
#254017=CARTESIAN_POINT('Origin',(0.,0.,0.));
#254018=CARTESIAN_POINT('Origin',(0.,0.,0.));
#254019=CARTESIAN_POINT('Origin',(0.,0.,0.));
#254020=CARTESIAN_POINT('Origin',(0.,0.,0.));
#254021=CARTESIAN_POINT('',(25.2771067246846,6.08833931617698,0.));
#254022=CARTESIAN_POINT('Origin',(0.,0.,0.));
#254023=CARTESIAN_POINT('',(22.1738711152697,4.11585220600461,0.));
#254024=CARTESIAN_POINT('Ctrl Pts',(25.2771067246846,6.08833931617698,0.));
#254025=CARTESIAN_POINT('Ctrl Pts',(25.2729539149479,6.08441489609824,0.));
#254026=CARTESIAN_POINT('Ctrl Pts',(25.2646490489816,6.07657531787578,0.));
#254027=CARTESIAN_POINT('Ctrl Pts',(25.2521940105523,6.06484373634697,0.));
#254028=CARTESIAN_POINT('Ctrl Pts',(25.2355918138798,6.04925720151412,0.));
#254029=CARTESIAN_POINT('Ctrl Pts',(25.2148466201368,6.02986667390187,0.));
#254030=CARTESIAN_POINT('Ctrl Pts',(25.1941090269638,6.0105688180476,0.));
#254031=CARTESIAN_POINT('Ctrl Pts',(25.1733791296154,5.99136367859839,0.));
#254032=CARTESIAN_POINT('Ctrl Pts',(25.1526570863065,5.97225131495636,0.));
#254033=CARTESIAN_POINT('Ctrl Pts',(25.1319431317273,5.95323180187348,0.));
#254034=CARTESIAN_POINT('Ctrl Pts',(25.1112375971182,5.93430523086776,0.));
#254035=CARTESIAN_POINT('Ctrl Pts',(25.0905409050863,5.91547170844382,0.));
#254036=CARTESIAN_POINT('Ctrl Pts',(25.0698535426593,5.89673135155459,0.));
#254037=CARTESIAN_POINT('Ctrl Pts',(25.0491760405965,5.87808428385329,0.));
#254038=CARTESIAN_POINT('Ctrl Pts',(25.0285089498922,5.8595306315681,0.));
#254039=CARTESIAN_POINT('Ctrl Pts',(25.0078528200558,5.84107051963074,0.));
#254040=CARTESIAN_POINT('Ctrl Pts',(24.9872081752709,5.82270406744214,0.));
#254041=CARTESIAN_POINT('Ctrl Pts',(24.9665754954462,5.80443138549747,0.));
#254042=CARTESIAN_POINT('Ctrl Pts',(24.9459552293308,5.78625257775703,0.));
#254043=CARTESIAN_POINT('Ctrl Pts',(24.9253478043632,5.76816774342236,0.));
#254044=CARTESIAN_POINT('Ctrl Pts',(24.9047536376467,5.75017697890813,0.));
#254045=CARTESIAN_POINT('Ctrl Pts',(24.8841731467219,5.73228037976927,0.));
#254046=CARTESIAN_POINT('Ctrl Pts',(24.8636067597677,5.71447804252019,0.));
#254047=CARTESIAN_POINT('Ctrl Pts',(24.8430549277634,5.6967700667943,0.));
#254048=CARTESIAN_POINT('Ctrl Pts',(24.822518122386,5.67915655496524,0.));
#254049=CARTESIAN_POINT('Ctrl Pts',(24.8019968304618,5.66163761114903,0.));
#254050=CARTESIAN_POINT('Ctrl Pts',(24.7814915496728,5.64421334042248,0.));
#254051=CARTESIAN_POINT('Ctrl Pts',(24.76100278357,5.62688384790919,0.));
#254052=CARTESIAN_POINT('Ctrl Pts',(24.7405310372736,5.60964923798495,0.));
#254053=CARTESIAN_POINT('Ctrl Pts',(24.7200768119079,5.59250961323995,0.));
#254054=CARTESIAN_POINT('Ctrl Pts',(24.6996406035507,5.57546507427767,0.));
#254055=CARTESIAN_POINT('Ctrl Pts',(24.6792229061785,5.55851572025389,0.));
#254056=CARTESIAN_POINT('Ctrl Pts',(24.6588242134733,5.54166164919593,0.));
#254057=CARTESIAN_POINT('Ctrl Pts',(24.6384450211466,5.52490295840996,0.));
#254058=CARTESIAN_POINT('Ctrl Pts',(24.618085828918,5.50823974481959,0.));
#254059=CARTESIAN_POINT('Ctrl Pts',(24.5977471429365,5.49167210537235,0.));
#254060=CARTESIAN_POINT('Ctrl Pts',(24.5774294770329,5.47520013724403,0.));
#254061=CARTESIAN_POINT('Ctrl Pts',(24.5571333514841,5.45882393762244,0.));
#254062=CARTESIAN_POINT('Ctrl Pts',(24.5368592922861,5.44254360356866,0.));
#254063=CARTESIAN_POINT('Ctrl Pts',(24.5166078302107,5.42635923183411,0.));
#254064=CARTESIAN_POINT('Ctrl Pts',(24.4963794999831,5.41027091869242,0.));
#254065=CARTESIAN_POINT('Ctrl Pts',(24.4761748393322,5.39427875973831,0.));
#254066=CARTESIAN_POINT('Ctrl Pts',(24.4559943883159,5.37838284973706,0.));
#254067=CARTESIAN_POINT('Ctrl Pts',(24.4358386899152,5.36258328273639,0.));
#254068=CARTESIAN_POINT('Ctrl Pts',(24.4157082904615,5.34688015213546,0.));
#254069=CARTESIAN_POINT('Ctrl Pts',(24.3956037401293,5.33127355076037,0.));
#254070=CARTESIAN_POINT('Ctrl Pts',(24.3755255933917,5.31576357092525,0.));
#254071=CARTESIAN_POINT('Ctrl Pts',(24.3554744095075,5.30035030449059,0.));
#254072=CARTESIAN_POINT('Ctrl Pts',(24.3354507529415,5.28503384290644,0.));
#254073=CARTESIAN_POINT('Ctrl Pts',(24.3154551932222,5.26981427718796,0.));
#254074=CARTESIAN_POINT('Ctrl Pts',(24.2954883048448,5.25469169788856,0.));
#254075=CARTESIAN_POINT('Ctrl Pts',(24.2755506671526,5.23966619506289,0.));
#254076=CARTESIAN_POINT('Ctrl Pts',(24.2556428642294,5.22473785822441,0.));
#254077=CARTESIAN_POINT('Ctrl Pts',(24.2357654847765,5.20990677629173,0.));
#254078=CARTESIAN_POINT('Ctrl Pts',(24.215919122017,5.19517303753643,0.));
#254079=CARTESIAN_POINT('Ctrl Pts',(24.1961043738754,5.18053672961392,0.));
#254080=CARTESIAN_POINT('Ctrl Pts',(24.1763218431343,5.16599793957979,0.));
#254081=CARTESIAN_POINT('Ctrl Pts',(24.156572137597,5.15155675390075,0.));
#254082=CARTESIAN_POINT('Ctrl Pts',(24.1368558702443,5.13721325845745,0.));
#254083=CARTESIAN_POINT('Ctrl Pts',(24.117173659394,5.1229675385386,0.));
#254084=CARTESIAN_POINT('Ctrl Pts',(24.0975261288446,5.10881967883132,0.));
#254085=CARTESIAN_POINT('Ctrl Pts',(24.0779139079266,5.09476976342625,0.));
#254086=CARTESIAN_POINT('Ctrl Pts',(24.0583376315638,5.08081787581277,0.));
#254087=CARTESIAN_POINT('Ctrl Pts',(24.0387979403268,5.06696409886641,0.));
#254088=CARTESIAN_POINT('Ctrl Pts',(24.0192954804896,5.05320851483065,0.));
#254089=CARTESIAN_POINT('Ctrl Pts',(23.9998309040746,5.03955120528521,0.));
#254090=CARTESIAN_POINT('Ctrl Pts',(23.9804048689227,5.02599225112454,0.));
#254091=CARTESIAN_POINT('Ctrl Pts',(23.961018038827,5.01253173257453,0.));
#254092=CARTESIAN_POINT('Ctrl Pts',(23.9416710836529,4.99916972919307,0.));
#254093=CARTESIAN_POINT('Ctrl Pts',(23.9223646794592,4.98590631986533,0.));
#254094=CARTESIAN_POINT('Ctrl Pts',(23.9030995086163,4.97274158279227,0.));
#254095=CARTESIAN_POINT('Ctrl Pts',(23.8838762599218,4.95967559546561,0.));
#254096=CARTESIAN_POINT('Ctrl Pts',(23.8646956287168,4.9467084346586,0.));
#254097=CARTESIAN_POINT('Ctrl Pts',(23.8455583170057,4.93384017643432,0.));
#254098=CARTESIAN_POINT('Ctrl Pts',(23.8264650335717,4.92107089613969,0.));
#254099=CARTESIAN_POINT('Ctrl Pts',(23.8074164940896,4.90840066839344,0.));
#254100=CARTESIAN_POINT('Ctrl Pts',(23.7884134212384,4.89582956706775,0.));
#254101=CARTESIAN_POINT('Ctrl Pts',(23.7694565448049,4.88335766525573,0.));
#254102=CARTESIAN_POINT('Ctrl Pts',(23.7505466018245,4.87098503527152,0.));
#254103=CARTESIAN_POINT('Ctrl Pts',(23.7316843367313,4.85871174865499,0.));
#254104=CARTESIAN_POINT('Ctrl Pts',(23.7128705015017,4.84653787616426,0.));
#254105=CARTESIAN_POINT('Ctrl Pts',(23.6941058557971,4.83446348776266,0.));
#254106=CARTESIAN_POINT('Ctrl Pts',(23.675391167102,4.82248865259562,0.));
#254107=CARTESIAN_POINT('Ctrl Pts',(23.6567272108628,4.81061343896432,0.));
#254108=CARTESIAN_POINT('Ctrl Pts',(23.6381147706579,4.7988379143322,0.));
#254109=CARTESIAN_POINT('Ctrl Pts',(23.6195546383624,4.78716214532098,0.));
#254110=CARTESIAN_POINT('Ctrl Pts',(23.6010476143099,4.77558619769872,0.));
#254111=CARTESIAN_POINT('Ctrl Pts',(23.5825945074535,4.76411013636251,0.));
#254112=CARTESIAN_POINT('Ctrl Pts',(23.5641961355168,4.75273402530617,0.));
#254113=CARTESIAN_POINT('Ctrl Pts',(23.545853325171,4.74145792760699,0.));
#254114=CARTESIAN_POINT('Ctrl Pts',(23.5275669122372,4.7302819054303,0.));
#254115=CARTESIAN_POINT('Ctrl Pts',(23.509337741878,4.71920602001902,0.));
#254116=CARTESIAN_POINT('Ctrl Pts',(23.491166668789,4.70823033167819,0.));
#254117=CARTESIAN_POINT('Ctrl Pts',(23.4730545573853,4.69735489975024,0.));
#254118=CARTESIAN_POINT('Ctrl Pts',(23.455002281986,4.68657978258303,0.));
#254119=CARTESIAN_POINT('Ctrl Pts',(23.4370107270451,4.67590503753059,0.));
#254120=CARTESIAN_POINT('Ctrl Pts',(23.4190807873803,4.6653307209467,0.));
#254121=CARTESIAN_POINT('Ctrl Pts',(23.4012133683959,4.65485688816924,0.));
#254122=CARTESIAN_POINT('Ctrl Pts',(23.3834093863068,4.6444835934993,0.));
#254123=CARTESIAN_POINT('Ctrl Pts',(23.3656697683489,4.63421089016541,0.));
#254124=CARTESIAN_POINT('Ctrl Pts',(23.3479954530272,4.62403883030805,0.));
#254125=CARTESIAN_POINT('Ctrl Pts',(23.3303873903938,4.6139674649783,0.));
#254126=CARTESIAN_POINT('Ctrl Pts',(23.3128465423115,4.60399684412163,0.));
#254127=CARTESIAN_POINT('Ctrl Pts',(23.2953738827191,4.5941270165575,0.));
#254128=CARTESIAN_POINT('Ctrl Pts',(23.2779703978876,4.5843580299469,0.));
#254129=CARTESIAN_POINT('Ctrl Pts',(23.2606370866866,4.57468993076097,0.));
#254130=CARTESIAN_POINT('Ctrl Pts',(23.2433749609131,4.56512276427839,0.));
#254131=CARTESIAN_POINT('Ctrl Pts',(23.2261850456064,4.55565657456975,0.));
#254132=CARTESIAN_POINT('Ctrl Pts',(23.2090683793629,4.54629140447544,0.));
#254133=CARTESIAN_POINT('Ctrl Pts',(23.1920260146465,4.53702729557566,0.));
#254134=CARTESIAN_POINT('Ctrl Pts',(23.1750590180908,4.52786428815015,0.));
#254135=CARTESIAN_POINT('Ctrl Pts',(23.1581684708761,4.51880242116748,0.));
#254136=CARTESIAN_POINT('Ctrl Pts',(23.1413554691123,4.5098417322706,0.));
#254137=CARTESIAN_POINT('Ctrl Pts',(23.1246211242115,4.50098225775171,0.));
#254138=CARTESIAN_POINT('Ctrl Pts',(23.1079665632636,4.49222403252216,0.));
#254139=CARTESIAN_POINT('Ctrl Pts',(23.0913929293922,4.48356709006788,0.));
#254140=CARTESIAN_POINT('Ctrl Pts',(23.0749013821881,4.47501146242856,0.));
#254141=CARTESIAN_POINT('Ctrl Pts',(23.0584930981732,4.46655718018231,0.));
#254142=CARTESIAN_POINT('Ctrl Pts',(23.0421692712467,4.45820427241683,0.));
#254143=CARTESIAN_POINT('Ctrl Pts',(23.0259311131392,4.44995276669687,0.));
#254144=CARTESIAN_POINT('Ctrl Pts',(23.0097798538395,4.44180268901643,0.));
#254145=CARTESIAN_POINT('Ctrl Pts',(22.9937167421006,4.43375406376879,0.));
#254146=CARTESIAN_POINT('Ctrl Pts',(22.977743046002,4.42580691372752,0.));
#254147=CARTESIAN_POINT('Ctrl Pts',(22.9618600534866,4.41796126001302,0.));
#254148=CARTESIAN_POINT('Ctrl Pts',(22.9460690729093,4.41021712205554,0.));
#254149=CARTESIAN_POINT('Ctrl Pts',(22.930371433555,4.40257451754324,0.));
#254150=CARTESIAN_POINT('Ctrl Pts',(22.9147684862426,4.39503346238473,0.));
#254151=CARTESIAN_POINT('Ctrl Pts',(22.8992616040108,4.38759397068406,0.));
#254152=CARTESIAN_POINT('Ctrl Pts',(22.8838521827701,4.38025605470093,0.));
#254153=CARTESIAN_POINT('Ctrl Pts',(22.8685416419725,4.37301972480746,0.));
#254154=CARTESIAN_POINT('Ctrl Pts',(22.8533314252422,4.36588498942997,0.));
#254155=CARTESIAN_POINT('Ctrl Pts',(22.8382230011184,4.35885185500546,0.));
#254156=CARTESIAN_POINT('Ctrl Pts',(22.8232178638876,4.35192032594791,0.));
#254157=CARTESIAN_POINT('Ctrl Pts',(22.8083175343791,4.34509040460062,0.));
#254158=CARTESIAN_POINT('Ctrl Pts',(22.7935235607806,4.33836209118446,0.));
#254159=CARTESIAN_POINT('Ctrl Pts',(22.7788375194076,4.3317353837319,0.));
#254160=CARTESIAN_POINT('Ctrl Pts',(22.7642610156475,4.32521027803754,0.));
#254161=CARTESIAN_POINT('Ctrl Pts',(22.7497956849848,4.31878676761235,0.));
#254162=CARTESIAN_POINT('Ctrl Pts',(22.7354431939926,4.31246484362549,0.));
#254163=CARTESIAN_POINT('Ctrl Pts',(22.7212052413386,4.30624449484069,0.));
#254164=CARTESIAN_POINT('Ctrl Pts',(22.7070835587564,4.3001257075406,0.));
#254165=CARTESIAN_POINT('Ctrl Pts',(22.6930799122548,4.29410846547056,0.));
#254166=CARTESIAN_POINT('Ctrl Pts',(22.6791961033537,4.28819274977763,0.));
#254167=CARTESIAN_POINT('Ctrl Pts',(22.6654339703109,4.28237853894059,0.));
#254168=CARTESIAN_POINT('Ctrl Pts',(22.6517953893303,4.2766658086912,0.));
#254169=CARTESIAN_POINT('Ctrl Pts',(22.6382822758172,4.27105453193004,0.));
#254170=CARTESIAN_POINT('Ctrl Pts',(22.6248965859977,4.26554467865576,0.));
#254171=CARTESIAN_POINT('Ctrl Pts',(22.6116403184821,4.26013621588305,0.));
#254172=CARTESIAN_POINT('Ctrl Pts',(22.5985155158636,4.25482910755481,0.));
#254173=CARTESIAN_POINT('Ctrl Pts',(22.5855242662477,4.24962331444177,0.));
#254174=CARTESIAN_POINT('Ctrl Pts',(22.572668704992,4.24451879404851,0.));
#254175=CARTESIAN_POINT('Ctrl Pts',(22.5599510166429,4.23951550052523,0.));
#254176=CARTESIAN_POINT('Ctrl Pts',(22.5473734368086,4.23461338456712,0.));
#254177=CARTESIAN_POINT('Ctrl Pts',(22.5349382540588,4.22981239330733,0.));
#254178=CARTESIAN_POINT('Ctrl Pts',(22.5226478117886,4.22511247020041,0.));
#254179=CARTESIAN_POINT('Ctrl Pts',(22.5105045108881,4.22051355490196,0.));
#254180=CARTESIAN_POINT('Ctrl Pts',(22.4985108124228,4.21601558313906,0.));
#254181=CARTESIAN_POINT('Ctrl Pts',(22.4866692403147,4.21161848657428,0.));
#254182=CARTESIAN_POINT('Ctrl Pts',(22.4749823839917,4.20732219265649,0.));
#254183=CARTESIAN_POINT('Ctrl Pts',(22.4634529011437,4.20312662448174,0.));
#254184=CARTESIAN_POINT('Ctrl Pts',(22.4520835205422,4.19903170066358,0.));
#254185=CARTESIAN_POINT('Ctrl Pts',(22.4408770448917,4.1950373351886,0.));
#254186=CARTESIAN_POINT('Ctrl Pts',(22.4298363535416,4.19114343726932,0.));
#254187=CARTESIAN_POINT('Ctrl Pts',(22.4189644056109,4.18734991117707,0.));
#254188=CARTESIAN_POINT('Ctrl Pts',(22.4082642454448,4.18365665600839,0.));
#254189=CARTESIAN_POINT('Ctrl Pts',(22.3977390078074,4.18006356544879,0.));
#254190=CARTESIAN_POINT('Ctrl Pts',(22.3873919231339,4.17657052752834,0.));
#254191=CARTESIAN_POINT('Ctrl Pts',(22.3772263228624,4.17317742436162,0.));
#254192=CARTESIAN_POINT('Ctrl Pts',(22.3672456427605,4.1698841319947,0.));
#254193=CARTESIAN_POINT('Ctrl Pts',(22.3574534257397,4.16669052026602,0.));
#254194=CARTESIAN_POINT('Ctrl Pts',(22.3478533253886,4.1635964526318,0.));
#254195=CARTESIAN_POINT('Ctrl Pts',(22.3384491078599,4.16060178604154,0.));
#254196=CARTESIAN_POINT('Ctrl Pts',(22.3292446628957,4.15770637047882,0.));
#254197=CARTESIAN_POINT('Ctrl Pts',(22.3202440186979,4.15491004835278,0.));
#254198=CARTESIAN_POINT('Ctrl Pts',(22.3114513545186,4.15221265396993,0.));
#254199=CARTESIAN_POINT('Ctrl Pts',(22.3028710166935,4.14961401285526,0.));
#254200=CARTESIAN_POINT('Ctrl Pts',(22.2945075198468,4.14711394168559,0.));
#254201=CARTESIAN_POINT('Ctrl Pts',(22.2863655389167,4.14471224859295,0.));
#254202=CARTESIAN_POINT('Ctrl Pts',(22.2784499072026,4.14240873321982,0.));
#254203=CARTESIAN_POINT('Ctrl Pts',(22.2707656042456,4.14020318715988,0.));
#254204=CARTESIAN_POINT('Ctrl Pts',(22.263317791397,4.13809539255419,0.));
#254205=CARTESIAN_POINT('Ctrl Pts',(22.2561118708422,4.13608511977226,0.));
#254206=CARTESIAN_POINT('Ctrl Pts',(22.2491535317789,4.13417212558809,0.));
#254207=CARTESIAN_POINT('Ctrl Pts',(22.2424488153523,4.1323561506016,0.));
#254208=CARTESIAN_POINT('Ctrl Pts',(22.2360040565534,4.13063692157499,0.));
#254209=CARTESIAN_POINT('Ctrl Pts',(22.2298258043947,4.12901415463379,0.));
#254210=CARTESIAN_POINT('Ctrl Pts',(22.2239207458781,4.127487558301,0.));
#254211=CARTESIAN_POINT('Ctrl Pts',(22.2182956401341,4.126056836133,0.));
#254212=CARTESIAN_POINT('Ctrl Pts',(22.2129576146671,4.12472167516602,0.));
#254213=CARTESIAN_POINT('Ctrl Pts',(22.2079143941719,4.12348173702025,0.));
#254214=CARTESIAN_POINT('Ctrl Pts',(22.2031746532106,4.12233664408237,0.));
#254215=CARTESIAN_POINT('Ctrl Pts',(22.1987479618246,4.12128598183533,0.));
#254216=CARTESIAN_POINT('Ctrl Pts',(22.1946440958098,4.12032932637738,0.));
#254217=CARTESIAN_POINT('Ctrl Pts',(22.1908725908525,4.11946626228623,0.));
#254218=CARTESIAN_POINT('Ctrl Pts',(22.1874419861496,4.11869641271752,0.));
#254219=CARTESIAN_POINT('Ctrl Pts',(22.1843613164855,4.11801938107464,0.));
#254220=CARTESIAN_POINT('Ctrl Pts',(22.1816414985788,4.11743469691765,0.));
#254221=CARTESIAN_POINT('Ctrl Pts',(22.179297473024,4.11694173195041,0.));
#254222=CARTESIAN_POINT('Ctrl Pts',(22.177347426894,4.11653973150558,0.));
#254223=CARTESIAN_POINT('Ctrl Pts',(22.1758088296598,4.11622797217066,0.));
#254224=CARTESIAN_POINT('Ctrl Pts',(22.1746949858773,4.11600589882768,0.));
#254225=CARTESIAN_POINT('Ctrl Pts',(22.174148802123,4.11589976826061,0.));
#254226=CARTESIAN_POINT('Ctrl Pts',(22.1739341411684,4.1158603587821,0.));
#254227=CARTESIAN_POINT('Ctrl Pts',(22.1738776823239,4.11585194677412,0.));
#254228=CARTESIAN_POINT('Ctrl Pts',(22.1738711152697,4.11585220600461,0.));
#254229=CARTESIAN_POINT('',(21.624941921198,4.01396149767428,0.));
#254230=CARTESIAN_POINT('',(11.0869355576349,2.05792610300232,0.));
#254231=CARTESIAN_POINT('',(21.2226420728916,3.44230496120419,0.));
#254232=CARTESIAN_POINT('Origin',(21.7161918885402,3.52235856495312,0.));
#254233=CARTESIAN_POINT('',(21.3904321633055,2.16781269186828,0.));
#254234=CARTESIAN_POINT('Origin',(7.7715611723761E-13,7.16093850883226E-14,
0.));
#254235=CARTESIAN_POINT('',(21.9269795755927,1.71975774210841,0.));
#254236=CARTESIAN_POINT('Origin',(21.8878840740801,2.21822694051638,0.));
#254237=CARTESIAN_POINT('',(22.4835757167854,1.76341220531179,0.));
#254238=CARTESIAN_POINT('',(10.7170877657712,0.840553282521227,0.));
#254239=CARTESIAN_POINT('',(25.991588367311,0.661312440730894,0.));
#254240=CARTESIAN_POINT('Ctrl Pts',(22.4835757167854,1.76341220531179,0.));
#254241=CARTESIAN_POINT('Ctrl Pts',(22.483581992979,1.76341415538764,0.));
#254242=CARTESIAN_POINT('Ctrl Pts',(22.4836387052232,1.7634206426357,0.));
#254243=CARTESIAN_POINT('Ctrl Pts',(22.4838562517069,1.76343813434565,0.));
#254244=CARTESIAN_POINT('Ctrl Pts',(22.4844112933129,1.76347698284792,0.));
#254245=CARTESIAN_POINT('Ctrl Pts',(22.4855446605991,1.76355076045546,0.));
#254246=CARTESIAN_POINT('Ctrl Pts',(22.4871115206571,1.76364784232963,0.));
#254247=CARTESIAN_POINT('Ctrl Pts',(22.4890991659478,1.76376424879505,0.));
#254248=CARTESIAN_POINT('Ctrl Pts',(22.4914909094908,1.76389475965724,0.));
#254249=CARTESIAN_POINT('Ctrl Pts',(22.4942693792449,1.76403393880301,0.));
#254250=CARTESIAN_POINT('Ctrl Pts',(22.4974203063191,1.76417731243462,0.));
#254251=CARTESIAN_POINT('Ctrl Pts',(22.5009332677316,1.76432160068726,0.));
#254252=CARTESIAN_POINT('Ctrl Pts',(22.5047996391978,1.76446408210366,0.));
#254253=CARTESIAN_POINT('Ctrl Pts',(22.5090112700212,1.76460218257323,0.));
#254254=CARTESIAN_POINT('Ctrl Pts',(22.5135590569554,1.76473303281159,0.));
#254255=CARTESIAN_POINT('Ctrl Pts',(22.5184336670207,1.76485369319896,0.));
#254256=CARTESIAN_POINT('Ctrl Pts',(22.5236259635515,1.76496128643369,0.));
#254257=CARTESIAN_POINT('Ctrl Pts',(22.529127665298,1.76505320262752,0.));
#254258=CARTESIAN_POINT('Ctrl Pts',(22.5349313983571,1.7651271156325,0.));
#254259=CARTESIAN_POINT('Ctrl Pts',(22.5410303590891,1.76518087841493,0.));
#254260=CARTESIAN_POINT('Ctrl Pts',(22.5474180954006,1.76521245524047,0.));
#254261=CARTESIAN_POINT('Ctrl Pts',(22.5540882235837,1.76521983384063,0.));
#254262=CARTESIAN_POINT('Ctrl Pts',(22.5610344912501,1.7652010450045,0.));
#254263=CARTESIAN_POINT('Ctrl Pts',(22.5682508499873,1.76515418518829,0.));
#254264=CARTESIAN_POINT('Ctrl Pts',(22.5757315316355,1.76507744026747,0.));
#254265=CARTESIAN_POINT('Ctrl Pts',(22.5834711038024,1.76496910283089,0.));
#254266=CARTESIAN_POINT('Ctrl Pts',(22.5914644078106,1.76482755288411,0.));
#254267=CARTESIAN_POINT('Ctrl Pts',(22.5997065145638,1.76465124413556,0.));
#254268=CARTESIAN_POINT('Ctrl Pts',(22.6081926681342,1.76443868648015,0.));
#254269=CARTESIAN_POINT('Ctrl Pts',(22.6169182517693,1.76418843543739,0.));
#254270=CARTESIAN_POINT('Ctrl Pts',(22.6258787994847,1.76389909571402,0.));
#254271=CARTESIAN_POINT('Ctrl Pts',(22.635069997936,1.76356932176272,0.));
#254272=CARTESIAN_POINT('Ctrl Pts',(22.6444876940425,1.76319782013914,0.));
#254273=CARTESIAN_POINT('Ctrl Pts',(22.6541278938413,1.76278334912559,0.));
#254274=CARTESIAN_POINT('Ctrl Pts',(22.6639867471756,1.76232471392568,0.));
#254275=CARTESIAN_POINT('Ctrl Pts',(22.6740605356699,1.76182076289525,0.));
#254276=CARTESIAN_POINT('Ctrl Pts',(22.6843456585245,1.76127038310613,0.));
#254277=CARTESIAN_POINT('Ctrl Pts',(22.6948386219843,1.76067249704884,0.));
#254278=CARTESIAN_POINT('Ctrl Pts',(22.7055360375481,1.76002606202399,0.));
#254279=CARTESIAN_POINT('Ctrl Pts',(22.7164346186007,1.75933006905924,0.));
#254280=CARTESIAN_POINT('Ctrl Pts',(22.7275311777305,1.75858354204635,0.));
#254281=CARTESIAN_POINT('Ctrl Pts',(22.7388226235565,1.75778553673249,0.));
#254282=CARTESIAN_POINT('Ctrl Pts',(22.7503059556455,1.75693513908911,0.));
#254283=CARTESIAN_POINT('Ctrl Pts',(22.7619782595013,1.75603146371641,0.));
#254284=CARTESIAN_POINT('Ctrl Pts',(22.7738367016115,1.75507365227127,0.));
#254285=CARTESIAN_POINT('Ctrl Pts',(22.7858785242358,1.7540608718293,0.));
#254286=CARTESIAN_POINT('Ctrl Pts',(22.7981010424312,1.75299231391461,0.));
#254287=CARTESIAN_POINT('Ctrl Pts',(22.8105016414712,1.7518671936559,0.));
#254288=CARTESIAN_POINT('Ctrl Pts',(22.8230777741285,1.75068474890884,0.));
#254289=CARTESIAN_POINT('Ctrl Pts',(22.8358269579854,1.74944423940117,0.));
#254290=CARTESIAN_POINT('Ctrl Pts',(22.8487467728075,1.74814494588492,0.));
#254291=CARTESIAN_POINT('Ctrl Pts',(22.8618348580234,1.74678616930663,0.));
#254292=CARTESIAN_POINT('Ctrl Pts',(22.8750889101696,1.745367229982,0.));
#254293=CARTESIAN_POINT('Ctrl Pts',(22.8885066803351,1.74388746677702,0.));
#254294=CARTESIAN_POINT('Ctrl Pts',(22.9020859716144,1.74234623630079,0.));
#254295=CARTESIAN_POINT('Ctrl Pts',(22.9158246373365,1.74074291231057,0.));
#254296=CARTESIAN_POINT('Ctrl Pts',(22.9297205792587,1.73907688511665,0.));
#254297=CARTESIAN_POINT('Ctrl Pts',(22.9437717457825,1.73734756100038,0.));
#254298=CARTESIAN_POINT('Ctrl Pts',(22.9579761301062,1.73555436162771,0.));
#254299=CARTESIAN_POINT('Ctrl Pts',(22.9723317685688,1.73369672350818,0.));
#254300=CARTESIAN_POINT('Ctrl Pts',(22.9868367391978,1.73177409750194,0.));
#254301=CARTESIAN_POINT('Ctrl Pts',(23.0014891601891,1.72978594832137,0.));
#254302=CARTESIAN_POINT('Ctrl Pts',(23.0162871884167,1.72773175404703,0.));
#254303=CARTESIAN_POINT('Ctrl Pts',(23.031229017888,1.72561100564033,0.));
#254304=CARTESIAN_POINT('Ctrl Pts',(23.0463128785528,1.72342320653731,0.));
#254305=CARTESIAN_POINT('Ctrl Pts',(23.0615370351559,1.72116787225981,0.));
#254306=CARTESIAN_POINT('Ctrl Pts',(23.0768997860709,1.71884453003027,0.));
#254307=CARTESIAN_POINT('Ctrl Pts',(23.0923994621216,1.71645271839311,0.));
#254308=CARTESIAN_POINT('Ctrl Pts',(23.1080344254291,1.71399198684725,0.));
#254309=CARTESIAN_POINT('Ctrl Pts',(23.1238030684929,1.71146189552192,0.));
#254310=CARTESIAN_POINT('Ctrl Pts',(23.1397038132358,1.7088620148546,0.));
#254311=CARTESIAN_POINT('Ctrl Pts',(23.1557351100613,1.70619192527847,0.));
#254312=CARTESIAN_POINT('Ctrl Pts',(23.1718954368749,1.70345121691259,0.));
#254313=CARTESIAN_POINT('Ctrl Pts',(23.1881832981848,1.70063948926988,0.));
#254314=CARTESIAN_POINT('Ctrl Pts',(23.2045972243765,1.69775635099425,0.));
#254315=CARTESIAN_POINT('Ctrl Pts',(23.2211357709374,1.69480141959946,0.));
#254316=CARTESIAN_POINT('Ctrl Pts',(23.2377975177014,1.69177432121716,0.));
#254317=CARTESIAN_POINT('Ctrl Pts',(23.2545810680536,1.6886746903491,0.));
#254318=CARTESIAN_POINT('Ctrl Pts',(23.2714850482245,1.68550216963275,0.));
#254319=CARTESIAN_POINT('Ctrl Pts',(23.2885081066949,1.68225640962181,0.));
#254320=CARTESIAN_POINT('Ctrl Pts',(23.3056489135611,1.67893706857123,0.));
#254321=CARTESIAN_POINT('Ctrl Pts',(23.3229061599145,1.67554381222988,0.));
#254322=CARTESIAN_POINT('Ctrl Pts',(23.3402785571866,1.67207631363905,0.));
#254323=CARTESIAN_POINT('Ctrl Pts',(23.3577648365747,1.66853425293978,0.));
#254324=CARTESIAN_POINT('Ctrl Pts',(23.375363748555,1.66491731718864,0.));
#254325=CARTESIAN_POINT('Ctrl Pts',(23.3930740623622,1.66122520018008,0.));
#254326=CARTESIAN_POINT('Ctrl Pts',(23.4108945654803,1.65745760227507,0.));
#254327=CARTESIAN_POINT('Ctrl Pts',(23.4288240631034,1.6536142302373,0.));
#254328=CARTESIAN_POINT('Ctrl Pts',(23.446861377656,1.6496947970734,0.));
#254329=CARTESIAN_POINT('Ctrl Pts',(23.4650053483919,1.64569902187608,0.));
#254330=CARTESIAN_POINT('Ctrl Pts',(23.4832548309638,1.64162662967525,0.));
#254331=CARTESIAN_POINT('Ctrl Pts',(23.5016086970006,1.63747735129474,0.));
#254332=CARTESIAN_POINT('Ctrl Pts',(23.5200658336624,1.63325092321731,0.));
#254333=CARTESIAN_POINT('Ctrl Pts',(23.5386251432278,1.62894708745231,0.));
#254334=CARTESIAN_POINT('Ctrl Pts',(23.5572855427617,1.62456559140072,0.));
#254335=CARTESIAN_POINT('Ctrl Pts',(23.5760459637608,1.62010618772869,0.));
#254336=CARTESIAN_POINT('Ctrl Pts',(23.5949053517996,1.61556863424697,0.));
#254337=CARTESIAN_POINT('Ctrl Pts',(23.6138626661644,1.61095269379773,0.));
#254338=CARTESIAN_POINT('Ctrl Pts',(23.6329168794916,1.60625813414666,0.));
#254339=CARTESIAN_POINT('Ctrl Pts',(23.6520669774863,1.60148472786588,0.));
#254340=CARTESIAN_POINT('Ctrl Pts',(23.6713119586302,1.59663225222459,0.));
#254341=CARTESIAN_POINT('Ctrl Pts',(23.6906508338832,1.59170048908631,0.));
#254342=CARTESIAN_POINT('Ctrl Pts',(23.7100826263835,1.58668922481222,0.));
#254343=CARTESIAN_POINT('Ctrl Pts',(23.7296063711308,1.58159825017362,0.));
#254344=CARTESIAN_POINT('Ctrl Pts',(23.7492211147369,1.57642736025251,0.));
#254345=CARTESIAN_POINT('Ctrl Pts',(23.7689259151869,1.57117635434412,0.));
#254346=CARTESIAN_POINT('Ctrl Pts',(23.788719841588,1.56584503586844,0.));
#254347=CARTESIAN_POINT('Ctrl Pts',(23.8086019739192,1.56043321228631,0.));
#254348=CARTESIAN_POINT('Ctrl Pts',(23.8285714027631,1.55494069502628,0.));
#254349=CARTESIAN_POINT('Ctrl Pts',(23.8486272290698,1.5493672994053,0.));
#254350=CARTESIAN_POINT('Ctrl Pts',(23.8687685639635,1.54371284453978,0.));
#254351=CARTESIAN_POINT('Ctrl Pts',(23.8889945285313,1.53797715326748,0.));
#254352=CARTESIAN_POINT('Ctrl Pts',(23.9093042536119,1.53216005207462,0.));
#254353=CARTESIAN_POINT('Ctrl Pts',(23.9296968795761,1.5262613710304,0.));
#254354=CARTESIAN_POINT('Ctrl Pts',(23.9501715561038,1.52028094372806,0.));
#254355=CARTESIAN_POINT('Ctrl Pts',(23.9707274420145,1.51421860720628,0.));
#254356=CARTESIAN_POINT('Ctrl Pts',(23.991363705093,1.50807420187703,0.));
#254357=CARTESIAN_POINT('Ctrl Pts',(24.0120795219086,1.50184757146099,0.));
#254358=CARTESIAN_POINT('Ctrl Pts',(24.0328740776331,1.49553856292798,0.));
#254359=CARTESIAN_POINT('Ctrl Pts',(24.053746565843,1.48914702644883,0.));
#254360=CARTESIAN_POINT('Ctrl Pts',(24.074696188353,1.4826728153368,0.));
#254361=CARTESIAN_POINT('Ctrl Pts',(24.0957221550782,1.47611578597742,0.));
#254362=CARTESIAN_POINT('Ctrl Pts',(24.1168236838827,1.46947579776992,0.));
#254363=CARTESIAN_POINT('Ctrl Pts',(24.1380000004272,1.46275271307398,0.));
#254364=CARTESIAN_POINT('Ctrl Pts',(24.1592503380105,1.45594639716314,0.));
#254365=CARTESIAN_POINT('Ctrl Pts',(24.1805739374033,1.44905671818721,0.));
#254366=CARTESIAN_POINT('Ctrl Pts',(24.2019700467214,1.44208354711074,0.));
#254367=CARTESIAN_POINT('Ctrl Pts',(24.2234379212978,1.43502675765502,0.));
#254368=CARTESIAN_POINT('Ctrl Pts',(24.2449768235485,1.42788622624851,0.));
#254369=CARTESIAN_POINT('Ctrl Pts',(24.2665860228357,1.42066183198252,0.));
#254370=CARTESIAN_POINT('Ctrl Pts',(24.2882647953214,1.41335345657685,0.));
#254371=CARTESIAN_POINT('Ctrl Pts',(24.3100124238316,1.40596098434341,0.));
#254372=CARTESIAN_POINT('Ctrl Pts',(24.3318281977647,1.3984843021281,0.));
#254373=CARTESIAN_POINT('Ctrl Pts',(24.3537114129877,1.3909232992639,0.));
#254374=CARTESIAN_POINT('Ctrl Pts',(24.37566137173,1.38327786752998,0.));
#254375=CARTESIAN_POINT('Ctrl Pts',(24.3976773824731,1.37554790111608,0.));
#254376=CARTESIAN_POINT('Ctrl Pts',(24.4197587598337,1.36773329659954,0.));
#254377=CARTESIAN_POINT('Ctrl Pts',(24.4419048244524,1.35983395290624,0.));
#254378=CARTESIAN_POINT('Ctrl Pts',(24.4641149028894,1.35184977125645,0.));
#254379=CARTESIAN_POINT('Ctrl Pts',(24.4863883275135,1.34378065512335,0.));
#254380=CARTESIAN_POINT('Ctrl Pts',(24.5087244363856,1.33562651019684,0.));
#254381=CARTESIAN_POINT('Ctrl Pts',(24.5311225731434,1.32738724435326,0.));
#254382=CARTESIAN_POINT('Ctrl Pts',(24.5535820868671,1.31906276763669,0.));
#254383=CARTESIAN_POINT('Ctrl Pts',(24.576102332018,1.31065299222023,0.));
#254384=CARTESIAN_POINT('Ctrl Pts',(24.5986826684025,1.30215783236364,0.));
#254385=CARTESIAN_POINT('Ctrl Pts',(24.6213224611228,1.29357720438108,0.));
#254386=CARTESIAN_POINT('Ctrl Pts',(24.6440210805278,1.28491102661514,0.));
#254387=CARTESIAN_POINT('Ctrl Pts',(24.666777902156,1.2761592194164,0.));
#254388=CARTESIAN_POINT('Ctrl Pts',(24.6895923066837,1.26732170513497,0.));
#254389=CARTESIAN_POINT('Ctrl Pts',(24.7124636797895,1.25839840807415,0.));
#254390=CARTESIAN_POINT('Ctrl Pts',(24.7353914120012,1.24938925444324,0.));
#254391=CARTESIAN_POINT('Ctrl Pts',(24.7583748985439,1.24029417231988,0.));
#254392=CARTESIAN_POINT('Ctrl Pts',(24.78141353918,1.23111309161843,0.));
#254393=CARTESIAN_POINT('Ctrl Pts',(24.8045067380536,1.22184594406527,0.));
#254394=CARTESIAN_POINT('Ctrl Pts',(24.8276539035092,1.21249266318205,0.));
#254395=CARTESIAN_POINT('Ctrl Pts',(24.8508544481973,1.20305318426016,0.));
#254396=CARTESIAN_POINT('Ctrl Pts',(24.8741077892074,1.19352744434059,0.));
#254397=CARTESIAN_POINT('Ctrl Pts',(24.8974133481829,1.18391538220098,0.));
#254398=CARTESIAN_POINT('Ctrl Pts',(24.9207705514449,1.1742169383504,0.));
#254399=CARTESIAN_POINT('Ctrl Pts',(24.9441788300932,1.16443205502852,0.));
#254400=CARTESIAN_POINT('Ctrl Pts',(24.9676376201501,1.15456067621894,0.));
#254401=CARTESIAN_POINT('Ctrl Pts',(24.9911463621431,1.14460274758206,0.));
#254402=CARTESIAN_POINT('Ctrl Pts',(25.0147045006193,1.13455821638536,0.));
#254403=CARTESIAN_POINT('Ctrl Pts',(25.0383114836898,1.12442703144455,0.));
#254404=CARTESIAN_POINT('Ctrl Pts',(25.0619667625336,1.1142091430689,0.));
#254405=CARTESIAN_POINT('Ctrl Pts',(25.085669790968,1.10390450301741,0.));
#254406=CARTESIAN_POINT('Ctrl Pts',(25.1094200248448,1.09351306445299,0.));
#254407=CARTESIAN_POINT('Ctrl Pts',(25.1332169227415,1.08303478197174,0.));
#254408=CARTESIAN_POINT('Ctrl Pts',(25.1570599469311,1.0724696116546,0.));
#254409=CARTESIAN_POINT('Ctrl Pts',(25.1809485642191,1.06181751111754,0.));
#254410=CARTESIAN_POINT('Ctrl Pts',(25.2048822469027,1.05107843957926,0.));
#254411=CARTESIAN_POINT('Ctrl Pts',(25.2288604735087,1.04025235791515,0.));
#254412=CARTESIAN_POINT('Ctrl Pts',(25.2528827300427,1.0293392287683,0.));
#254413=CARTESIAN_POINT('Ctrl Pts',(25.2769485087268,1.01833901642273,0.));
#254414=CARTESIAN_POINT('Ctrl Pts',(25.3010573055557,1.00725168656934,0.));
#254415=CARTESIAN_POINT('Ctrl Pts',(25.3252086182976,0.996077206120921,
0.));
#254416=CARTESIAN_POINT('Ctrl Pts',(25.3494019441444,0.984815543004091,
0.));
#254417=CARTESIAN_POINT('Ctrl Pts',(25.3736367778842,0.97346666600005,0.));
#254418=CARTESIAN_POINT('Ctrl Pts',(25.3979126089155,0.962030544502806,
0.));
#254419=CARTESIAN_POINT('Ctrl Pts',(25.4222289223155,0.950507148596971,
0.));
#254420=CARTESIAN_POINT('Ctrl Pts',(25.4465852044835,0.938896449495636,
0.));
#254421=CARTESIAN_POINT('Ctrl Pts',(25.4709809474996,0.927198419885607,
0.));
#254422=CARTESIAN_POINT('Ctrl Pts',(25.4954156541787,0.915413034335334,
0.));
#254423=CARTESIAN_POINT('Ctrl Pts',(25.5198888424195,0.903540269651155,
0.));
#254424=CARTESIAN_POINT('Ctrl Pts',(25.5444000508223,0.891580105349469,
0.));
#254425=CARTESIAN_POINT('Ctrl Pts',(25.568948840818,0.879532523835094,0.));
#254426=CARTESIAN_POINT('Ctrl Pts',(25.5935347843616,0.867397509339473,
0.));
#254427=CARTESIAN_POINT('Ctrl Pts',(25.618157453608,0.855175047037618,0.));
#254428=CARTESIAN_POINT('Ctrl Pts',(25.6428164100078,0.842865122121547,
0.));
#254429=CARTESIAN_POINT('Ctrl Pts',(25.6675111931957,0.83046771886437,0.));
#254430=CARTESIAN_POINT('Ctrl Pts',(25.6922413110172,0.817982819786722,
0.));
#254431=CARTESIAN_POINT('Ctrl Pts',(25.7170062262474,0.805410404552597,
0.));
#254432=CARTESIAN_POINT('Ctrl Pts',(25.7418053757671,0.792750451613538,
0.));
#254433=CARTESIAN_POINT('Ctrl Pts',(25.7666381946871,0.780002940289028,
0.));
#254434=CARTESIAN_POINT('Ctrl Pts',(25.7915041383304,0.767167852648643,
0.));
#254435=CARTESIAN_POINT('Ctrl Pts',(25.816402705995,0.754245175608291,0.));
#254436=CARTESIAN_POINT('Ctrl Pts',(25.841333461908,0.741234902664698,0.));
#254437=CARTESIAN_POINT('Ctrl Pts',(25.8662960624285,0.728137036485881,
0.));
#254438=CARTESIAN_POINT('Ctrl Pts',(25.8912902615141,0.714951588533756,
0.));
#254439=CARTESIAN_POINT('Ctrl Pts',(25.9163158909645,0.701678575236605,
0.));
#254440=CARTESIAN_POINT('Ctrl Pts',(25.941372847213,0.68831801506568,0.));
#254441=CARTESIAN_POINT('Ctrl Pts',(25.9614434298092,0.677559543215907,
0.));
#254442=CARTESIAN_POINT('Ctrl Pts',(25.9765104298171,0.669451306784419,
0.));
#254443=CARTESIAN_POINT('Ctrl Pts',(25.9865613464809,0.664028313188916,
0.));
#254444=CARTESIAN_POINT('Ctrl Pts',(25.991588367311,0.661312440730894,0.));
#254445=CARTESIAN_POINT('Origin',(0.,0.,0.));
#254446=CARTESIAN_POINT('',(-7.,-8.57252759403147E-16,0.));
#254447=CARTESIAN_POINT('Origin',(0.,0.,0.));
#254448=CARTESIAN_POINT('Origin',(0.,0.,12.));
#254449=CARTESIAN_POINT('',(25.991588367311,0.661312440730894,12.));
#254450=CARTESIAN_POINT('Origin',(0.,0.,12.));
#254451=CARTESIAN_POINT('',(22.4835757167854,1.76341220531179,12.));
#254452=CARTESIAN_POINT('Ctrl Pts',(25.991588367311,0.661312440730894,12.));
#254453=CARTESIAN_POINT('Ctrl Pts',(25.9865613464809,0.664028313188916,
12.));
#254454=CARTESIAN_POINT('Ctrl Pts',(25.9765104298171,0.669451306784419,
12.));
#254455=CARTESIAN_POINT('Ctrl Pts',(25.9614434298092,0.677559543215907,
12.));
#254456=CARTESIAN_POINT('Ctrl Pts',(25.941372847213,0.68831801506568,12.));
#254457=CARTESIAN_POINT('Ctrl Pts',(25.9163158909645,0.701678575236605,
12.));
#254458=CARTESIAN_POINT('Ctrl Pts',(25.8912902615141,0.714951588533756,
12.));
#254459=CARTESIAN_POINT('Ctrl Pts',(25.8662960624285,0.728137036485881,
12.));
#254460=CARTESIAN_POINT('Ctrl Pts',(25.841333461908,0.741234902664698,12.));
#254461=CARTESIAN_POINT('Ctrl Pts',(25.816402705995,0.754245175608291,12.));
#254462=CARTESIAN_POINT('Ctrl Pts',(25.7915041383304,0.767167852648643,
12.));
#254463=CARTESIAN_POINT('Ctrl Pts',(25.7666381946871,0.780002940289028,
12.));
#254464=CARTESIAN_POINT('Ctrl Pts',(25.7418053757671,0.792750451613538,
12.));
#254465=CARTESIAN_POINT('Ctrl Pts',(25.7170062262474,0.805410404552597,
12.));
#254466=CARTESIAN_POINT('Ctrl Pts',(25.6922413110172,0.817982819786722,
12.));
#254467=CARTESIAN_POINT('Ctrl Pts',(25.6675111931957,0.83046771886437,12.));
#254468=CARTESIAN_POINT('Ctrl Pts',(25.6428164100078,0.842865122121547,
12.));
#254469=CARTESIAN_POINT('Ctrl Pts',(25.618157453608,0.855175047037618,12.));
#254470=CARTESIAN_POINT('Ctrl Pts',(25.5935347843616,0.867397509339473,
12.));
#254471=CARTESIAN_POINT('Ctrl Pts',(25.568948840818,0.879532523835094,12.));
#254472=CARTESIAN_POINT('Ctrl Pts',(25.5444000508223,0.891580105349469,
12.));
#254473=CARTESIAN_POINT('Ctrl Pts',(25.5198888424195,0.903540269651155,
12.));
#254474=CARTESIAN_POINT('Ctrl Pts',(25.4954156541787,0.915413034335334,
12.));
#254475=CARTESIAN_POINT('Ctrl Pts',(25.4709809474996,0.927198419885607,
12.));
#254476=CARTESIAN_POINT('Ctrl Pts',(25.4465852044835,0.938896449495636,
12.));
#254477=CARTESIAN_POINT('Ctrl Pts',(25.4222289223155,0.950507148596971,
12.));
#254478=CARTESIAN_POINT('Ctrl Pts',(25.3979126089155,0.962030544502806,
12.));
#254479=CARTESIAN_POINT('Ctrl Pts',(25.3736367778842,0.97346666600005,12.));
#254480=CARTESIAN_POINT('Ctrl Pts',(25.3494019441444,0.984815543004091,
12.));
#254481=CARTESIAN_POINT('Ctrl Pts',(25.3252086182976,0.996077206120921,
12.));
#254482=CARTESIAN_POINT('Ctrl Pts',(25.3010573055557,1.00725168656934,12.));
#254483=CARTESIAN_POINT('Ctrl Pts',(25.2769485087268,1.01833901642273,12.));
#254484=CARTESIAN_POINT('Ctrl Pts',(25.2528827300427,1.0293392287683,12.));
#254485=CARTESIAN_POINT('Ctrl Pts',(25.2288604735087,1.04025235791515,12.));
#254486=CARTESIAN_POINT('Ctrl Pts',(25.2048822469027,1.05107843957926,12.));
#254487=CARTESIAN_POINT('Ctrl Pts',(25.1809485642191,1.06181751111754,12.));
#254488=CARTESIAN_POINT('Ctrl Pts',(25.1570599469311,1.0724696116546,12.));
#254489=CARTESIAN_POINT('Ctrl Pts',(25.1332169227415,1.08303478197174,12.));
#254490=CARTESIAN_POINT('Ctrl Pts',(25.1094200248448,1.09351306445299,12.));
#254491=CARTESIAN_POINT('Ctrl Pts',(25.085669790968,1.10390450301741,12.));
#254492=CARTESIAN_POINT('Ctrl Pts',(25.0619667625336,1.1142091430689,12.));
#254493=CARTESIAN_POINT('Ctrl Pts',(25.0383114836898,1.12442703144455,12.));
#254494=CARTESIAN_POINT('Ctrl Pts',(25.0147045006193,1.13455821638536,12.));
#254495=CARTESIAN_POINT('Ctrl Pts',(24.9911463621431,1.14460274758206,12.));
#254496=CARTESIAN_POINT('Ctrl Pts',(24.9676376201501,1.15456067621894,12.));
#254497=CARTESIAN_POINT('Ctrl Pts',(24.9441788300932,1.16443205502852,12.));
#254498=CARTESIAN_POINT('Ctrl Pts',(24.9207705514449,1.1742169383504,12.));
#254499=CARTESIAN_POINT('Ctrl Pts',(24.8974133481829,1.18391538220098,12.));
#254500=CARTESIAN_POINT('Ctrl Pts',(24.8741077892074,1.19352744434059,12.));
#254501=CARTESIAN_POINT('Ctrl Pts',(24.8508544481973,1.20305318426016,12.));
#254502=CARTESIAN_POINT('Ctrl Pts',(24.8276539035092,1.21249266318205,12.));
#254503=CARTESIAN_POINT('Ctrl Pts',(24.8045067380536,1.22184594406527,12.));
#254504=CARTESIAN_POINT('Ctrl Pts',(24.78141353918,1.23111309161843,12.));
#254505=CARTESIAN_POINT('Ctrl Pts',(24.7583748985439,1.24029417231988,12.));
#254506=CARTESIAN_POINT('Ctrl Pts',(24.7353914120012,1.24938925444324,12.));
#254507=CARTESIAN_POINT('Ctrl Pts',(24.7124636797895,1.25839840807415,12.));
#254508=CARTESIAN_POINT('Ctrl Pts',(24.6895923066837,1.26732170513497,12.));
#254509=CARTESIAN_POINT('Ctrl Pts',(24.666777902156,1.2761592194164,12.));
#254510=CARTESIAN_POINT('Ctrl Pts',(24.6440210805278,1.28491102661514,12.));
#254511=CARTESIAN_POINT('Ctrl Pts',(24.6213224611228,1.29357720438108,12.));
#254512=CARTESIAN_POINT('Ctrl Pts',(24.5986826684025,1.30215783236364,12.));
#254513=CARTESIAN_POINT('Ctrl Pts',(24.576102332018,1.31065299222023,12.));
#254514=CARTESIAN_POINT('Ctrl Pts',(24.5535820868671,1.31906276763669,12.));
#254515=CARTESIAN_POINT('Ctrl Pts',(24.5311225731434,1.32738724435326,12.));
#254516=CARTESIAN_POINT('Ctrl Pts',(24.5087244363856,1.33562651019684,12.));
#254517=CARTESIAN_POINT('Ctrl Pts',(24.4863883275135,1.34378065512335,12.));
#254518=CARTESIAN_POINT('Ctrl Pts',(24.4641149028894,1.35184977125645,12.));
#254519=CARTESIAN_POINT('Ctrl Pts',(24.4419048244524,1.35983395290624,12.));
#254520=CARTESIAN_POINT('Ctrl Pts',(24.4197587598337,1.36773329659954,12.));
#254521=CARTESIAN_POINT('Ctrl Pts',(24.3976773824731,1.37554790111608,12.));
#254522=CARTESIAN_POINT('Ctrl Pts',(24.37566137173,1.38327786752998,12.));
#254523=CARTESIAN_POINT('Ctrl Pts',(24.3537114129877,1.3909232992639,12.));
#254524=CARTESIAN_POINT('Ctrl Pts',(24.3318281977647,1.3984843021281,12.));
#254525=CARTESIAN_POINT('Ctrl Pts',(24.3100124238316,1.40596098434341,12.));
#254526=CARTESIAN_POINT('Ctrl Pts',(24.2882647953214,1.41335345657685,12.));
#254527=CARTESIAN_POINT('Ctrl Pts',(24.2665860228357,1.42066183198252,12.));
#254528=CARTESIAN_POINT('Ctrl Pts',(24.2449768235485,1.42788622624851,12.));
#254529=CARTESIAN_POINT('Ctrl Pts',(24.2234379212978,1.43502675765502,12.));
#254530=CARTESIAN_POINT('Ctrl Pts',(24.2019700467214,1.44208354711074,12.));
#254531=CARTESIAN_POINT('Ctrl Pts',(24.1805739374033,1.44905671818721,12.));
#254532=CARTESIAN_POINT('Ctrl Pts',(24.1592503380105,1.45594639716314,12.));
#254533=CARTESIAN_POINT('Ctrl Pts',(24.1380000004272,1.46275271307398,12.));
#254534=CARTESIAN_POINT('Ctrl Pts',(24.1168236838827,1.46947579776992,12.));
#254535=CARTESIAN_POINT('Ctrl Pts',(24.0957221550782,1.47611578597742,12.));
#254536=CARTESIAN_POINT('Ctrl Pts',(24.074696188353,1.4826728153368,12.));
#254537=CARTESIAN_POINT('Ctrl Pts',(24.053746565843,1.48914702644883,12.));
#254538=CARTESIAN_POINT('Ctrl Pts',(24.0328740776331,1.49553856292798,12.));
#254539=CARTESIAN_POINT('Ctrl Pts',(24.0120795219086,1.50184757146099,12.));
#254540=CARTESIAN_POINT('Ctrl Pts',(23.991363705093,1.50807420187703,12.));
#254541=CARTESIAN_POINT('Ctrl Pts',(23.9707274420145,1.51421860720628,12.));
#254542=CARTESIAN_POINT('Ctrl Pts',(23.9501715561038,1.52028094372806,12.));
#254543=CARTESIAN_POINT('Ctrl Pts',(23.9296968795761,1.5262613710304,12.));
#254544=CARTESIAN_POINT('Ctrl Pts',(23.9093042536119,1.53216005207462,12.));
#254545=CARTESIAN_POINT('Ctrl Pts',(23.8889945285313,1.53797715326748,12.));
#254546=CARTESIAN_POINT('Ctrl Pts',(23.8687685639635,1.54371284453978,12.));
#254547=CARTESIAN_POINT('Ctrl Pts',(23.8486272290698,1.5493672994053,12.));
#254548=CARTESIAN_POINT('Ctrl Pts',(23.8285714027631,1.55494069502628,12.));
#254549=CARTESIAN_POINT('Ctrl Pts',(23.8086019739192,1.56043321228631,12.));
#254550=CARTESIAN_POINT('Ctrl Pts',(23.788719841588,1.56584503586844,12.));
#254551=CARTESIAN_POINT('Ctrl Pts',(23.7689259151869,1.57117635434412,12.));
#254552=CARTESIAN_POINT('Ctrl Pts',(23.7492211147369,1.57642736025251,12.));
#254553=CARTESIAN_POINT('Ctrl Pts',(23.7296063711308,1.58159825017362,12.));
#254554=CARTESIAN_POINT('Ctrl Pts',(23.7100826263835,1.58668922481222,12.));
#254555=CARTESIAN_POINT('Ctrl Pts',(23.6906508338832,1.59170048908631,12.));
#254556=CARTESIAN_POINT('Ctrl Pts',(23.6713119586302,1.59663225222459,12.));
#254557=CARTESIAN_POINT('Ctrl Pts',(23.6520669774863,1.60148472786588,12.));
#254558=CARTESIAN_POINT('Ctrl Pts',(23.6329168794916,1.60625813414666,12.));
#254559=CARTESIAN_POINT('Ctrl Pts',(23.6138626661644,1.61095269379773,12.));
#254560=CARTESIAN_POINT('Ctrl Pts',(23.5949053517996,1.61556863424697,12.));
#254561=CARTESIAN_POINT('Ctrl Pts',(23.5760459637608,1.62010618772869,12.));
#254562=CARTESIAN_POINT('Ctrl Pts',(23.5572855427617,1.62456559140072,12.));
#254563=CARTESIAN_POINT('Ctrl Pts',(23.5386251432278,1.62894708745231,12.));
#254564=CARTESIAN_POINT('Ctrl Pts',(23.5200658336624,1.63325092321731,12.));
#254565=CARTESIAN_POINT('Ctrl Pts',(23.5016086970006,1.63747735129474,12.));
#254566=CARTESIAN_POINT('Ctrl Pts',(23.4832548309638,1.64162662967525,12.));
#254567=CARTESIAN_POINT('Ctrl Pts',(23.4650053483919,1.64569902187608,12.));
#254568=CARTESIAN_POINT('Ctrl Pts',(23.446861377656,1.6496947970734,12.));
#254569=CARTESIAN_POINT('Ctrl Pts',(23.4288240631034,1.6536142302373,12.));
#254570=CARTESIAN_POINT('Ctrl Pts',(23.4108945654803,1.65745760227507,12.));
#254571=CARTESIAN_POINT('Ctrl Pts',(23.3930740623622,1.66122520018008,12.));
#254572=CARTESIAN_POINT('Ctrl Pts',(23.375363748555,1.66491731718864,12.));
#254573=CARTESIAN_POINT('Ctrl Pts',(23.3577648365747,1.66853425293978,12.));
#254574=CARTESIAN_POINT('Ctrl Pts',(23.3402785571866,1.67207631363905,12.));
#254575=CARTESIAN_POINT('Ctrl Pts',(23.3229061599145,1.67554381222988,12.));
#254576=CARTESIAN_POINT('Ctrl Pts',(23.3056489135611,1.67893706857123,12.));
#254577=CARTESIAN_POINT('Ctrl Pts',(23.2885081066949,1.68225640962181,12.));
#254578=CARTESIAN_POINT('Ctrl Pts',(23.2714850482245,1.68550216963275,12.));
#254579=CARTESIAN_POINT('Ctrl Pts',(23.2545810680536,1.6886746903491,12.));
#254580=CARTESIAN_POINT('Ctrl Pts',(23.2377975177014,1.69177432121716,12.));
#254581=CARTESIAN_POINT('Ctrl Pts',(23.2211357709374,1.69480141959946,12.));
#254582=CARTESIAN_POINT('Ctrl Pts',(23.2045972243765,1.69775635099425,12.));
#254583=CARTESIAN_POINT('Ctrl Pts',(23.1881832981848,1.70063948926988,12.));
#254584=CARTESIAN_POINT('Ctrl Pts',(23.1718954368749,1.70345121691259,12.));
#254585=CARTESIAN_POINT('Ctrl Pts',(23.1557351100613,1.70619192527847,12.));
#254586=CARTESIAN_POINT('Ctrl Pts',(23.1397038132358,1.7088620148546,12.));
#254587=CARTESIAN_POINT('Ctrl Pts',(23.1238030684929,1.71146189552192,12.));
#254588=CARTESIAN_POINT('Ctrl Pts',(23.1080344254291,1.71399198684725,12.));
#254589=CARTESIAN_POINT('Ctrl Pts',(23.0923994621216,1.71645271839311,12.));
#254590=CARTESIAN_POINT('Ctrl Pts',(23.0768997860709,1.71884453003027,12.));
#254591=CARTESIAN_POINT('Ctrl Pts',(23.0615370351559,1.72116787225981,12.));
#254592=CARTESIAN_POINT('Ctrl Pts',(23.0463128785528,1.72342320653731,12.));
#254593=CARTESIAN_POINT('Ctrl Pts',(23.031229017888,1.72561100564033,12.));
#254594=CARTESIAN_POINT('Ctrl Pts',(23.0162871884167,1.72773175404703,12.));
#254595=CARTESIAN_POINT('Ctrl Pts',(23.0014891601891,1.72978594832137,12.));
#254596=CARTESIAN_POINT('Ctrl Pts',(22.9868367391978,1.73177409750194,12.));
#254597=CARTESIAN_POINT('Ctrl Pts',(22.9723317685688,1.73369672350818,12.));
#254598=CARTESIAN_POINT('Ctrl Pts',(22.9579761301062,1.73555436162771,12.));
#254599=CARTESIAN_POINT('Ctrl Pts',(22.9437717457825,1.73734756100038,12.));
#254600=CARTESIAN_POINT('Ctrl Pts',(22.9297205792587,1.73907688511665,12.));
#254601=CARTESIAN_POINT('Ctrl Pts',(22.9158246373365,1.74074291231057,12.));
#254602=CARTESIAN_POINT('Ctrl Pts',(22.9020859716144,1.74234623630079,12.));
#254603=CARTESIAN_POINT('Ctrl Pts',(22.8885066803351,1.74388746677702,12.));
#254604=CARTESIAN_POINT('Ctrl Pts',(22.8750889101696,1.745367229982,12.));
#254605=CARTESIAN_POINT('Ctrl Pts',(22.8618348580234,1.74678616930663,12.));
#254606=CARTESIAN_POINT('Ctrl Pts',(22.8487467728075,1.74814494588492,12.));
#254607=CARTESIAN_POINT('Ctrl Pts',(22.8358269579854,1.74944423940117,12.));
#254608=CARTESIAN_POINT('Ctrl Pts',(22.8230777741285,1.75068474890884,12.));
#254609=CARTESIAN_POINT('Ctrl Pts',(22.8105016414712,1.7518671936559,12.));
#254610=CARTESIAN_POINT('Ctrl Pts',(22.7981010424312,1.75299231391461,12.));
#254611=CARTESIAN_POINT('Ctrl Pts',(22.7858785242358,1.7540608718293,12.));
#254612=CARTESIAN_POINT('Ctrl Pts',(22.7738367016115,1.75507365227127,12.));
#254613=CARTESIAN_POINT('Ctrl Pts',(22.7619782595013,1.75603146371641,12.));
#254614=CARTESIAN_POINT('Ctrl Pts',(22.7503059556455,1.75693513908911,12.));
#254615=CARTESIAN_POINT('Ctrl Pts',(22.7388226235565,1.75778553673249,12.));
#254616=CARTESIAN_POINT('Ctrl Pts',(22.7275311777305,1.75858354204635,12.));
#254617=CARTESIAN_POINT('Ctrl Pts',(22.7164346186007,1.75933006905924,12.));
#254618=CARTESIAN_POINT('Ctrl Pts',(22.7055360375481,1.76002606202399,12.));
#254619=CARTESIAN_POINT('Ctrl Pts',(22.6948386219843,1.76067249704884,12.));
#254620=CARTESIAN_POINT('Ctrl Pts',(22.6843456585245,1.76127038310613,12.));
#254621=CARTESIAN_POINT('Ctrl Pts',(22.6740605356699,1.76182076289525,12.));
#254622=CARTESIAN_POINT('Ctrl Pts',(22.6639867471756,1.76232471392568,12.));
#254623=CARTESIAN_POINT('Ctrl Pts',(22.6541278938413,1.76278334912559,12.));
#254624=CARTESIAN_POINT('Ctrl Pts',(22.6444876940425,1.76319782013914,12.));
#254625=CARTESIAN_POINT('Ctrl Pts',(22.635069997936,1.76356932176272,12.));
#254626=CARTESIAN_POINT('Ctrl Pts',(22.6258787994847,1.76389909571402,12.));
#254627=CARTESIAN_POINT('Ctrl Pts',(22.6169182517693,1.76418843543739,12.));
#254628=CARTESIAN_POINT('Ctrl Pts',(22.6081926681342,1.76443868648015,12.));
#254629=CARTESIAN_POINT('Ctrl Pts',(22.5997065145638,1.76465124413556,12.));
#254630=CARTESIAN_POINT('Ctrl Pts',(22.5914644078106,1.76482755288411,12.));
#254631=CARTESIAN_POINT('Ctrl Pts',(22.5834711038024,1.76496910283089,12.));
#254632=CARTESIAN_POINT('Ctrl Pts',(22.5757315316355,1.76507744026747,12.));
#254633=CARTESIAN_POINT('Ctrl Pts',(22.5682508499873,1.76515418518829,12.));
#254634=CARTESIAN_POINT('Ctrl Pts',(22.5610344912501,1.7652010450045,12.));
#254635=CARTESIAN_POINT('Ctrl Pts',(22.5540882235837,1.76521983384063,12.));
#254636=CARTESIAN_POINT('Ctrl Pts',(22.5474180954006,1.76521245524047,12.));
#254637=CARTESIAN_POINT('Ctrl Pts',(22.5410303590891,1.76518087841493,12.));
#254638=CARTESIAN_POINT('Ctrl Pts',(22.5349313983571,1.7651271156325,12.));
#254639=CARTESIAN_POINT('Ctrl Pts',(22.529127665298,1.76505320262752,12.));
#254640=CARTESIAN_POINT('Ctrl Pts',(22.5236259635515,1.76496128643369,12.));
#254641=CARTESIAN_POINT('Ctrl Pts',(22.5184336670207,1.76485369319896,12.));
#254642=CARTESIAN_POINT('Ctrl Pts',(22.5135590569554,1.76473303281159,12.));
#254643=CARTESIAN_POINT('Ctrl Pts',(22.5090112700212,1.76460218257323,12.));
#254644=CARTESIAN_POINT('Ctrl Pts',(22.5047996391978,1.76446408210366,12.));
#254645=CARTESIAN_POINT('Ctrl Pts',(22.5009332677316,1.76432160068726,12.));
#254646=CARTESIAN_POINT('Ctrl Pts',(22.4974203063191,1.76417731243462,12.));
#254647=CARTESIAN_POINT('Ctrl Pts',(22.4942693792449,1.76403393880301,12.));
#254648=CARTESIAN_POINT('Ctrl Pts',(22.4914909094908,1.76389475965724,12.));
#254649=CARTESIAN_POINT('Ctrl Pts',(22.4890991659478,1.76376424879505,12.));
#254650=CARTESIAN_POINT('Ctrl Pts',(22.4871115206571,1.76364784232963,12.));
#254651=CARTESIAN_POINT('Ctrl Pts',(22.4855446605991,1.76355076045546,12.));
#254652=CARTESIAN_POINT('Ctrl Pts',(22.4844112933129,1.76347698284792,12.));
#254653=CARTESIAN_POINT('Ctrl Pts',(22.4838562517069,1.76343813434565,12.));
#254654=CARTESIAN_POINT('Ctrl Pts',(22.4836387052232,1.7634206426357,12.));
#254655=CARTESIAN_POINT('Ctrl Pts',(22.483581992979,1.76341415538764,12.));
#254656=CARTESIAN_POINT('Ctrl Pts',(22.4835757167854,1.76341220531179,12.));
#254657=CARTESIAN_POINT('',(21.9269795755927,1.71975774210841,12.));
#254658=CARTESIAN_POINT('',(10.7170877657712,0.840553282521227,12.));
#254659=CARTESIAN_POINT('',(21.3904321633055,2.16781269186828,12.));
#254660=CARTESIAN_POINT('Origin',(21.8878840740801,2.21822694051638,12.));
#254661=CARTESIAN_POINT('',(21.2226420728916,3.44230496120419,12.));
#254662=CARTESIAN_POINT('Origin',(7.7715611723761E-13,7.16093850883226E-14,
12.));
#254663=CARTESIAN_POINT('',(21.624941921198,4.01396149767428,12.));
#254664=CARTESIAN_POINT('Origin',(21.7161918885402,3.52235856495312,12.));
#254665=CARTESIAN_POINT('',(22.1738711152697,4.11585220600461,12.));
#254666=CARTESIAN_POINT('',(11.0869355576349,2.05792610300232,12.));
#254667=CARTESIAN_POINT('',(25.2771067246846,6.08833931617698,12.));
#254668=CARTESIAN_POINT('Ctrl Pts',(22.1738711152697,4.11585220600461,12.));
#254669=CARTESIAN_POINT('Ctrl Pts',(22.1738776823239,4.11585194677412,12.));
#254670=CARTESIAN_POINT('Ctrl Pts',(22.1739341411684,4.1158603587821,12.));
#254671=CARTESIAN_POINT('Ctrl Pts',(22.174148802123,4.11589976826061,12.));
#254672=CARTESIAN_POINT('Ctrl Pts',(22.1746949858773,4.11600589882768,12.));
#254673=CARTESIAN_POINT('Ctrl Pts',(22.1758088296598,4.11622797217066,12.));
#254674=CARTESIAN_POINT('Ctrl Pts',(22.177347426894,4.11653973150558,12.));
#254675=CARTESIAN_POINT('Ctrl Pts',(22.179297473024,4.11694173195041,12.));
#254676=CARTESIAN_POINT('Ctrl Pts',(22.1816414985788,4.11743469691765,12.));
#254677=CARTESIAN_POINT('Ctrl Pts',(22.1843613164855,4.11801938107464,12.));
#254678=CARTESIAN_POINT('Ctrl Pts',(22.1874419861496,4.11869641271752,12.));
#254679=CARTESIAN_POINT('Ctrl Pts',(22.1908725908525,4.11946626228623,12.));
#254680=CARTESIAN_POINT('Ctrl Pts',(22.1946440958098,4.12032932637738,12.));
#254681=CARTESIAN_POINT('Ctrl Pts',(22.1987479618246,4.12128598183533,12.));
#254682=CARTESIAN_POINT('Ctrl Pts',(22.2031746532106,4.12233664408237,12.));
#254683=CARTESIAN_POINT('Ctrl Pts',(22.2079143941719,4.12348173702025,12.));
#254684=CARTESIAN_POINT('Ctrl Pts',(22.2129576146671,4.12472167516602,12.));
#254685=CARTESIAN_POINT('Ctrl Pts',(22.2182956401341,4.126056836133,12.));
#254686=CARTESIAN_POINT('Ctrl Pts',(22.2239207458781,4.127487558301,12.));
#254687=CARTESIAN_POINT('Ctrl Pts',(22.2298258043947,4.12901415463379,12.));
#254688=CARTESIAN_POINT('Ctrl Pts',(22.2360040565534,4.13063692157499,12.));
#254689=CARTESIAN_POINT('Ctrl Pts',(22.2424488153523,4.1323561506016,12.));
#254690=CARTESIAN_POINT('Ctrl Pts',(22.2491535317789,4.13417212558809,12.));
#254691=CARTESIAN_POINT('Ctrl Pts',(22.2561118708422,4.13608511977226,12.));
#254692=CARTESIAN_POINT('Ctrl Pts',(22.263317791397,4.13809539255419,12.));
#254693=CARTESIAN_POINT('Ctrl Pts',(22.2707656042456,4.14020318715988,12.));
#254694=CARTESIAN_POINT('Ctrl Pts',(22.2784499072026,4.14240873321982,12.));
#254695=CARTESIAN_POINT('Ctrl Pts',(22.2863655389167,4.14471224859295,12.));
#254696=CARTESIAN_POINT('Ctrl Pts',(22.2945075198468,4.14711394168559,12.));
#254697=CARTESIAN_POINT('Ctrl Pts',(22.3028710166935,4.14961401285526,12.));
#254698=CARTESIAN_POINT('Ctrl Pts',(22.3114513545186,4.15221265396993,12.));
#254699=CARTESIAN_POINT('Ctrl Pts',(22.3202440186979,4.15491004835278,12.));
#254700=CARTESIAN_POINT('Ctrl Pts',(22.3292446628957,4.15770637047882,12.));
#254701=CARTESIAN_POINT('Ctrl Pts',(22.3384491078599,4.16060178604154,12.));
#254702=CARTESIAN_POINT('Ctrl Pts',(22.3478533253886,4.1635964526318,12.));
#254703=CARTESIAN_POINT('Ctrl Pts',(22.3574534257397,4.16669052026602,12.));
#254704=CARTESIAN_POINT('Ctrl Pts',(22.3672456427605,4.1698841319947,12.));
#254705=CARTESIAN_POINT('Ctrl Pts',(22.3772263228624,4.17317742436162,12.));
#254706=CARTESIAN_POINT('Ctrl Pts',(22.3873919231339,4.17657052752834,12.));
#254707=CARTESIAN_POINT('Ctrl Pts',(22.3977390078074,4.18006356544879,12.));
#254708=CARTESIAN_POINT('Ctrl Pts',(22.4082642454448,4.18365665600839,12.));
#254709=CARTESIAN_POINT('Ctrl Pts',(22.4189644056109,4.18734991117707,12.));
#254710=CARTESIAN_POINT('Ctrl Pts',(22.4298363535416,4.19114343726932,12.));
#254711=CARTESIAN_POINT('Ctrl Pts',(22.4408770448917,4.1950373351886,12.));
#254712=CARTESIAN_POINT('Ctrl Pts',(22.4520835205422,4.19903170066358,12.));
#254713=CARTESIAN_POINT('Ctrl Pts',(22.4634529011437,4.20312662448174,12.));
#254714=CARTESIAN_POINT('Ctrl Pts',(22.4749823839917,4.20732219265649,12.));
#254715=CARTESIAN_POINT('Ctrl Pts',(22.4866692403147,4.21161848657428,12.));
#254716=CARTESIAN_POINT('Ctrl Pts',(22.4985108124228,4.21601558313906,12.));
#254717=CARTESIAN_POINT('Ctrl Pts',(22.5105045108881,4.22051355490196,12.));
#254718=CARTESIAN_POINT('Ctrl Pts',(22.5226478117886,4.22511247020041,12.));
#254719=CARTESIAN_POINT('Ctrl Pts',(22.5349382540588,4.22981239330733,12.));
#254720=CARTESIAN_POINT('Ctrl Pts',(22.5473734368086,4.23461338456712,12.));
#254721=CARTESIAN_POINT('Ctrl Pts',(22.5599510166429,4.23951550052523,12.));
#254722=CARTESIAN_POINT('Ctrl Pts',(22.572668704992,4.24451879404851,12.));
#254723=CARTESIAN_POINT('Ctrl Pts',(22.5855242662477,4.24962331444177,12.));
#254724=CARTESIAN_POINT('Ctrl Pts',(22.5985155158636,4.25482910755481,12.));
#254725=CARTESIAN_POINT('Ctrl Pts',(22.6116403184821,4.26013621588305,12.));
#254726=CARTESIAN_POINT('Ctrl Pts',(22.6248965859977,4.26554467865576,12.));
#254727=CARTESIAN_POINT('Ctrl Pts',(22.6382822758172,4.27105453193004,12.));
#254728=CARTESIAN_POINT('Ctrl Pts',(22.6517953893303,4.2766658086912,12.));
#254729=CARTESIAN_POINT('Ctrl Pts',(22.6654339703109,4.28237853894059,12.));
#254730=CARTESIAN_POINT('Ctrl Pts',(22.6791961033537,4.28819274977763,12.));
#254731=CARTESIAN_POINT('Ctrl Pts',(22.6930799122548,4.29410846547056,12.));
#254732=CARTESIAN_POINT('Ctrl Pts',(22.7070835587564,4.3001257075406,12.));
#254733=CARTESIAN_POINT('Ctrl Pts',(22.7212052413386,4.30624449484069,12.));
#254734=CARTESIAN_POINT('Ctrl Pts',(22.7354431939926,4.31246484362549,12.));
#254735=CARTESIAN_POINT('Ctrl Pts',(22.7497956849848,4.31878676761235,12.));
#254736=CARTESIAN_POINT('Ctrl Pts',(22.7642610156475,4.32521027803754,12.));
#254737=CARTESIAN_POINT('Ctrl Pts',(22.7788375194076,4.3317353837319,12.));
#254738=CARTESIAN_POINT('Ctrl Pts',(22.7935235607806,4.33836209118446,12.));
#254739=CARTESIAN_POINT('Ctrl Pts',(22.8083175343791,4.34509040460062,12.));
#254740=CARTESIAN_POINT('Ctrl Pts',(22.8232178638876,4.35192032594791,12.));
#254741=CARTESIAN_POINT('Ctrl Pts',(22.8382230011184,4.35885185500546,12.));
#254742=CARTESIAN_POINT('Ctrl Pts',(22.8533314252422,4.36588498942997,12.));
#254743=CARTESIAN_POINT('Ctrl Pts',(22.8685416419725,4.37301972480746,12.));
#254744=CARTESIAN_POINT('Ctrl Pts',(22.8838521827701,4.38025605470093,12.));
#254745=CARTESIAN_POINT('Ctrl Pts',(22.8992616040108,4.38759397068406,12.));
#254746=CARTESIAN_POINT('Ctrl Pts',(22.9147684862426,4.39503346238473,12.));
#254747=CARTESIAN_POINT('Ctrl Pts',(22.930371433555,4.40257451754324,12.));
#254748=CARTESIAN_POINT('Ctrl Pts',(22.9460690729093,4.41021712205554,12.));
#254749=CARTESIAN_POINT('Ctrl Pts',(22.9618600534866,4.41796126001302,12.));
#254750=CARTESIAN_POINT('Ctrl Pts',(22.977743046002,4.42580691372752,12.));
#254751=CARTESIAN_POINT('Ctrl Pts',(22.9937167421006,4.43375406376879,12.));
#254752=CARTESIAN_POINT('Ctrl Pts',(23.0097798538395,4.44180268901643,12.));
#254753=CARTESIAN_POINT('Ctrl Pts',(23.0259311131392,4.44995276669687,12.));
#254754=CARTESIAN_POINT('Ctrl Pts',(23.0421692712467,4.45820427241683,12.));
#254755=CARTESIAN_POINT('Ctrl Pts',(23.0584930981732,4.46655718018231,12.));
#254756=CARTESIAN_POINT('Ctrl Pts',(23.0749013821881,4.47501146242856,12.));
#254757=CARTESIAN_POINT('Ctrl Pts',(23.0913929293922,4.48356709006788,12.));
#254758=CARTESIAN_POINT('Ctrl Pts',(23.1079665632636,4.49222403252216,12.));
#254759=CARTESIAN_POINT('Ctrl Pts',(23.1246211242115,4.50098225775171,12.));
#254760=CARTESIAN_POINT('Ctrl Pts',(23.1413554691123,4.5098417322706,12.));
#254761=CARTESIAN_POINT('Ctrl Pts',(23.1581684708761,4.51880242116748,12.));
#254762=CARTESIAN_POINT('Ctrl Pts',(23.1750590180908,4.52786428815015,12.));
#254763=CARTESIAN_POINT('Ctrl Pts',(23.1920260146465,4.53702729557566,12.));
#254764=CARTESIAN_POINT('Ctrl Pts',(23.2090683793629,4.54629140447544,12.));
#254765=CARTESIAN_POINT('Ctrl Pts',(23.2261850456064,4.55565657456975,12.));
#254766=CARTESIAN_POINT('Ctrl Pts',(23.2433749609131,4.56512276427839,12.));
#254767=CARTESIAN_POINT('Ctrl Pts',(23.2606370866866,4.57468993076097,12.));
#254768=CARTESIAN_POINT('Ctrl Pts',(23.2779703978876,4.5843580299469,12.));
#254769=CARTESIAN_POINT('Ctrl Pts',(23.2953738827191,4.5941270165575,12.));
#254770=CARTESIAN_POINT('Ctrl Pts',(23.3128465423115,4.60399684412163,12.));
#254771=CARTESIAN_POINT('Ctrl Pts',(23.3303873903938,4.6139674649783,12.));
#254772=CARTESIAN_POINT('Ctrl Pts',(23.3479954530272,4.62403883030805,12.));
#254773=CARTESIAN_POINT('Ctrl Pts',(23.3656697683489,4.63421089016541,12.));
#254774=CARTESIAN_POINT('Ctrl Pts',(23.3834093863068,4.6444835934993,12.));
#254775=CARTESIAN_POINT('Ctrl Pts',(23.4012133683959,4.65485688816924,12.));
#254776=CARTESIAN_POINT('Ctrl Pts',(23.4190807873803,4.6653307209467,12.));
#254777=CARTESIAN_POINT('Ctrl Pts',(23.4370107270451,4.67590503753059,12.));
#254778=CARTESIAN_POINT('Ctrl Pts',(23.455002281986,4.68657978258303,12.));
#254779=CARTESIAN_POINT('Ctrl Pts',(23.4730545573853,4.69735489975024,12.));
#254780=CARTESIAN_POINT('Ctrl Pts',(23.491166668789,4.70823033167819,12.));
#254781=CARTESIAN_POINT('Ctrl Pts',(23.509337741878,4.71920602001902,12.));
#254782=CARTESIAN_POINT('Ctrl Pts',(23.5275669122372,4.7302819054303,12.));
#254783=CARTESIAN_POINT('Ctrl Pts',(23.545853325171,4.74145792760699,12.));
#254784=CARTESIAN_POINT('Ctrl Pts',(23.5641961355168,4.75273402530617,12.));
#254785=CARTESIAN_POINT('Ctrl Pts',(23.5825945074535,4.76411013636251,12.));
#254786=CARTESIAN_POINT('Ctrl Pts',(23.6010476143099,4.77558619769872,12.));
#254787=CARTESIAN_POINT('Ctrl Pts',(23.6195546383624,4.78716214532098,12.));
#254788=CARTESIAN_POINT('Ctrl Pts',(23.6381147706579,4.7988379143322,12.));
#254789=CARTESIAN_POINT('Ctrl Pts',(23.6567272108628,4.81061343896432,12.));
#254790=CARTESIAN_POINT('Ctrl Pts',(23.675391167102,4.82248865259562,12.));
#254791=CARTESIAN_POINT('Ctrl Pts',(23.6941058557971,4.83446348776266,12.));
#254792=CARTESIAN_POINT('Ctrl Pts',(23.7128705015017,4.84653787616426,12.));
#254793=CARTESIAN_POINT('Ctrl Pts',(23.7316843367313,4.85871174865499,12.));
#254794=CARTESIAN_POINT('Ctrl Pts',(23.7505466018245,4.87098503527152,12.));
#254795=CARTESIAN_POINT('Ctrl Pts',(23.7694565448049,4.88335766525573,12.));
#254796=CARTESIAN_POINT('Ctrl Pts',(23.7884134212384,4.89582956706775,12.));
#254797=CARTESIAN_POINT('Ctrl Pts',(23.8074164940896,4.90840066839344,12.));
#254798=CARTESIAN_POINT('Ctrl Pts',(23.8264650335717,4.92107089613969,12.));
#254799=CARTESIAN_POINT('Ctrl Pts',(23.8455583170057,4.93384017643432,12.));
#254800=CARTESIAN_POINT('Ctrl Pts',(23.8646956287168,4.9467084346586,12.));
#254801=CARTESIAN_POINT('Ctrl Pts',(23.8838762599218,4.95967559546561,12.));
#254802=CARTESIAN_POINT('Ctrl Pts',(23.9030995086163,4.97274158279227,12.));
#254803=CARTESIAN_POINT('Ctrl Pts',(23.9223646794592,4.98590631986533,12.));
#254804=CARTESIAN_POINT('Ctrl Pts',(23.9416710836529,4.99916972919307,12.));
#254805=CARTESIAN_POINT('Ctrl Pts',(23.961018038827,5.01253173257453,12.));
#254806=CARTESIAN_POINT('Ctrl Pts',(23.9804048689227,5.02599225112454,12.));
#254807=CARTESIAN_POINT('Ctrl Pts',(23.9998309040746,5.03955120528521,12.));
#254808=CARTESIAN_POINT('Ctrl Pts',(24.0192954804896,5.05320851483065,12.));
#254809=CARTESIAN_POINT('Ctrl Pts',(24.0387979403268,5.06696409886641,12.));
#254810=CARTESIAN_POINT('Ctrl Pts',(24.0583376315638,5.08081787581277,12.));
#254811=CARTESIAN_POINT('Ctrl Pts',(24.0779139079266,5.09476976342625,12.));
#254812=CARTESIAN_POINT('Ctrl Pts',(24.0975261288446,5.10881967883132,12.));
#254813=CARTESIAN_POINT('Ctrl Pts',(24.117173659394,5.1229675385386,12.));
#254814=CARTESIAN_POINT('Ctrl Pts',(24.1368558702443,5.13721325845745,12.));
#254815=CARTESIAN_POINT('Ctrl Pts',(24.156572137597,5.15155675390075,12.));
#254816=CARTESIAN_POINT('Ctrl Pts',(24.1763218431343,5.16599793957979,12.));
#254817=CARTESIAN_POINT('Ctrl Pts',(24.1961043738754,5.18053672961392,12.));
#254818=CARTESIAN_POINT('Ctrl Pts',(24.215919122017,5.19517303753643,12.));
#254819=CARTESIAN_POINT('Ctrl Pts',(24.2357654847765,5.20990677629173,12.));
#254820=CARTESIAN_POINT('Ctrl Pts',(24.2556428642294,5.22473785822441,12.));
#254821=CARTESIAN_POINT('Ctrl Pts',(24.2755506671526,5.23966619506289,12.));
#254822=CARTESIAN_POINT('Ctrl Pts',(24.2954883048448,5.25469169788856,12.));
#254823=CARTESIAN_POINT('Ctrl Pts',(24.3154551932222,5.26981427718796,12.));
#254824=CARTESIAN_POINT('Ctrl Pts',(24.3354507529415,5.28503384290644,12.));
#254825=CARTESIAN_POINT('Ctrl Pts',(24.3554744095075,5.30035030449059,12.));
#254826=CARTESIAN_POINT('Ctrl Pts',(24.3755255933917,5.31576357092525,12.));
#254827=CARTESIAN_POINT('Ctrl Pts',(24.3956037401293,5.33127355076037,12.));
#254828=CARTESIAN_POINT('Ctrl Pts',(24.4157082904615,5.34688015213546,12.));
#254829=CARTESIAN_POINT('Ctrl Pts',(24.4358386899152,5.36258328273639,12.));
#254830=CARTESIAN_POINT('Ctrl Pts',(24.4559943883159,5.37838284973706,12.));
#254831=CARTESIAN_POINT('Ctrl Pts',(24.4761748393322,5.39427875973831,12.));
#254832=CARTESIAN_POINT('Ctrl Pts',(24.4963794999831,5.41027091869242,12.));
#254833=CARTESIAN_POINT('Ctrl Pts',(24.5166078302107,5.42635923183411,12.));
#254834=CARTESIAN_POINT('Ctrl Pts',(24.5368592922861,5.44254360356866,12.));
#254835=CARTESIAN_POINT('Ctrl Pts',(24.5571333514841,5.45882393762244,12.));
#254836=CARTESIAN_POINT('Ctrl Pts',(24.5774294770329,5.47520013724403,12.));
#254837=CARTESIAN_POINT('Ctrl Pts',(24.5977471429365,5.49167210537235,12.));
#254838=CARTESIAN_POINT('Ctrl Pts',(24.618085828918,5.50823974481959,12.));
#254839=CARTESIAN_POINT('Ctrl Pts',(24.6384450211466,5.52490295840996,12.));
#254840=CARTESIAN_POINT('Ctrl Pts',(24.6588242134733,5.54166164919593,12.));
#254841=CARTESIAN_POINT('Ctrl Pts',(24.6792229061785,5.55851572025389,12.));
#254842=CARTESIAN_POINT('Ctrl Pts',(24.6996406035507,5.57546507427767,12.));
#254843=CARTESIAN_POINT('Ctrl Pts',(24.7200768119079,5.59250961323995,12.));
#254844=CARTESIAN_POINT('Ctrl Pts',(24.7405310372736,5.60964923798495,12.));
#254845=CARTESIAN_POINT('Ctrl Pts',(24.76100278357,5.62688384790919,12.));
#254846=CARTESIAN_POINT('Ctrl Pts',(24.7814915496728,5.64421334042248,12.));
#254847=CARTESIAN_POINT('Ctrl Pts',(24.8019968304618,5.66163761114903,12.));
#254848=CARTESIAN_POINT('Ctrl Pts',(24.822518122386,5.67915655496524,12.));
#254849=CARTESIAN_POINT('Ctrl Pts',(24.8430549277634,5.6967700667943,12.));
#254850=CARTESIAN_POINT('Ctrl Pts',(24.8636067597677,5.71447804252019,12.));
#254851=CARTESIAN_POINT('Ctrl Pts',(24.8841731467219,5.73228037976927,12.));
#254852=CARTESIAN_POINT('Ctrl Pts',(24.9047536376467,5.75017697890813,12.));
#254853=CARTESIAN_POINT('Ctrl Pts',(24.9253478043632,5.76816774342236,12.));
#254854=CARTESIAN_POINT('Ctrl Pts',(24.9459552293308,5.78625257775703,12.));
#254855=CARTESIAN_POINT('Ctrl Pts',(24.9665754954462,5.80443138549747,12.));
#254856=CARTESIAN_POINT('Ctrl Pts',(24.9872081752709,5.82270406744214,12.));
#254857=CARTESIAN_POINT('Ctrl Pts',(25.0078528200558,5.84107051963074,12.));
#254858=CARTESIAN_POINT('Ctrl Pts',(25.0285089498922,5.8595306315681,12.));
#254859=CARTESIAN_POINT('Ctrl Pts',(25.0491760405965,5.87808428385329,12.));
#254860=CARTESIAN_POINT('Ctrl Pts',(25.0698535426593,5.89673135155459,12.));
#254861=CARTESIAN_POINT('Ctrl Pts',(25.0905409050863,5.91547170844382,12.));
#254862=CARTESIAN_POINT('Ctrl Pts',(25.1112375971182,5.93430523086776,12.));
#254863=CARTESIAN_POINT('Ctrl Pts',(25.1319431317273,5.95323180187348,12.));
#254864=CARTESIAN_POINT('Ctrl Pts',(25.1526570863065,5.97225131495636,12.));
#254865=CARTESIAN_POINT('Ctrl Pts',(25.1733791296154,5.99136367859839,12.));
#254866=CARTESIAN_POINT('Ctrl Pts',(25.1941090269638,6.0105688180476,12.));
#254867=CARTESIAN_POINT('Ctrl Pts',(25.2148466201368,6.02986667390187,12.));
#254868=CARTESIAN_POINT('Ctrl Pts',(25.2355918138798,6.04925720151412,12.));
#254869=CARTESIAN_POINT('Ctrl Pts',(25.2521940105523,6.06484373634697,12.));
#254870=CARTESIAN_POINT('Ctrl Pts',(25.2646490489816,6.07657531787578,12.));
#254871=CARTESIAN_POINT('Ctrl Pts',(25.2729539149479,6.08441489609824,12.));
#254872=CARTESIAN_POINT('Ctrl Pts',(25.2771067246846,6.08833931617698,12.));
#254873=CARTESIAN_POINT('Origin',(0.,0.,12.));
#254874=CARTESIAN_POINT('Origin',(0.,0.,12.));
#254875=CARTESIAN_POINT('Origin',(0.,0.,12.));
#254876=CARTESIAN_POINT('Origin',(0.,0.,12.));
#254877=CARTESIAN_POINT('Origin',(0.,0.,12.));
#254878=CARTESIAN_POINT('Origin',(0.,0.,12.));
#254879=CARTESIAN_POINT('Origin',(0.,0.,12.));
#254880=CARTESIAN_POINT('Origin',(0.,0.,12.));
#254881=CARTESIAN_POINT('Origin',(0.,0.,12.));
#254882=CARTESIAN_POINT('Origin',(0.,0.,12.));
#254883=CARTESIAN_POINT('Origin',(0.,0.,12.));
#254884=CARTESIAN_POINT('Origin',(0.,0.,12.));
#254885=CARTESIAN_POINT('Origin',(0.,0.,12.));
#254886=CARTESIAN_POINT('Origin',(0.,0.,12.));
#254887=CARTESIAN_POINT('Origin',(0.,0.,12.));
#254888=CARTESIAN_POINT('Origin',(0.,0.,12.));
#254889=CARTESIAN_POINT('Origin',(0.,0.,12.));
#254890=CARTESIAN_POINT('Origin',(0.,0.,12.));
#254891=CARTESIAN_POINT('Origin',(0.,0.,12.));
#254892=CARTESIAN_POINT('Origin',(0.,0.,12.));
#254893=CARTESIAN_POINT('Origin',(0.,0.,12.));
#254894=CARTESIAN_POINT('Origin',(0.,0.,12.));
#254895=CARTESIAN_POINT('Origin',(0.,0.,12.));
#254896=CARTESIAN_POINT('',(-7.,-8.57252759403147E-16,12.));
#254897=CARTESIAN_POINT('Origin',(0.,0.,12.));
#254898=CARTESIAN_POINT('Origin',(0.,0.,0.));
#254899=CARTESIAN_POINT('',(25.2771067246846,6.08833931617698,0.));
#254900=CARTESIAN_POINT('Origin',(0.,0.,0.));
#254901=CARTESIAN_POINT('Origin',(0.,0.,0.));
#254902=CARTESIAN_POINT('Origin',(0.,0.,0.));
#254903=CARTESIAN_POINT('Origin',(0.,0.,0.));
#254904=CARTESIAN_POINT('Origin',(0.,0.,0.));
#254905=CARTESIAN_POINT('Origin',(0.,0.,0.));
#254906=CARTESIAN_POINT('Origin',(0.,0.,0.));
#254907=CARTESIAN_POINT('Origin',(0.,0.,0.));
#254908=CARTESIAN_POINT('Origin',(0.,0.,0.));
#254909=CARTESIAN_POINT('Origin',(0.,0.,0.));
#254910=CARTESIAN_POINT('Origin',(0.,0.,0.));
#254911=CARTESIAN_POINT('Origin',(0.,0.,0.));
#254912=CARTESIAN_POINT('Origin',(0.,0.,0.));
#254913=CARTESIAN_POINT('Origin',(0.,0.,0.));
#254914=CARTESIAN_POINT('Origin',(0.,0.,0.));
#254915=CARTESIAN_POINT('Origin',(0.,0.,0.));
#254916=CARTESIAN_POINT('Origin',(0.,0.,0.));
#254917=CARTESIAN_POINT('Origin',(0.,0.,0.));
#254918=CARTESIAN_POINT('Origin',(0.,0.,0.));
#254919=CARTESIAN_POINT('Origin',(0.,0.,0.));
#254920=CARTESIAN_POINT('Origin',(0.,0.,0.));
#254921=CARTESIAN_POINT('Origin',(0.,0.,0.));
#254922=CARTESIAN_POINT('Origin',(21.7161918885402,3.52235856495312,0.));
#254923=CARTESIAN_POINT('',(21.624941921198,4.01396149767428,0.));
#254924=CARTESIAN_POINT('',(21.2226420728916,3.44230496120418,0.));
#254925=CARTESIAN_POINT('Origin',(22.1738711152697,4.11585220600461,0.));
#254926=CARTESIAN_POINT('',(22.1738711152697,4.11585220600461,0.));
#254927=CARTESIAN_POINT('Origin',(21.8878840740801,2.21822694051638,0.));
#254928=CARTESIAN_POINT('',(21.3904321633055,2.16781269186828,0.));
#254929=CARTESIAN_POINT('',(21.9269795755927,1.71975774210841,0.));
#254930=CARTESIAN_POINT('Origin',(7.7715611723761E-13,7.16093850883226E-14,
0.));
#254931=CARTESIAN_POINT('Origin',(21.4341755315424,1.68110656504246,0.));
#254932=CARTESIAN_POINT('',(22.4835757167854,1.76341220531179,0.));
#254933=CARTESIAN_POINT('Ctrl Pts',(25.2771067246846,6.08833931617698,0.));
#254934=CARTESIAN_POINT('Ctrl Pts',(25.2771067246846,6.08833931617698,12.));
#254935=CARTESIAN_POINT('Ctrl Pts',(25.2729539149479,6.08441489609824,0.));
#254936=CARTESIAN_POINT('Ctrl Pts',(25.2729539149479,6.08441489609824,12.));
#254937=CARTESIAN_POINT('Ctrl Pts',(25.2646490489816,6.07657531787578,0.));
#254938=CARTESIAN_POINT('Ctrl Pts',(25.2646490489816,6.07657531787578,12.));
#254939=CARTESIAN_POINT('Ctrl Pts',(25.2521940105523,6.06484373634697,0.));
#254940=CARTESIAN_POINT('Ctrl Pts',(25.2521940105523,6.06484373634697,12.));
#254941=CARTESIAN_POINT('Ctrl Pts',(25.2355918138798,6.04925720151412,0.));
#254942=CARTESIAN_POINT('Ctrl Pts',(25.2355918138798,6.04925720151412,12.));
#254943=CARTESIAN_POINT('Ctrl Pts',(25.2148466201368,6.02986667390187,0.));
#254944=CARTESIAN_POINT('Ctrl Pts',(25.2148466201368,6.02986667390187,12.));
#254945=CARTESIAN_POINT('Ctrl Pts',(25.1941090269638,6.0105688180476,0.));
#254946=CARTESIAN_POINT('Ctrl Pts',(25.1941090269638,6.0105688180476,12.));
#254947=CARTESIAN_POINT('Ctrl Pts',(25.1733791296154,5.99136367859839,0.));
#254948=CARTESIAN_POINT('Ctrl Pts',(25.1733791296154,5.99136367859839,12.));
#254949=CARTESIAN_POINT('Ctrl Pts',(25.1526570863065,5.97225131495636,0.));
#254950=CARTESIAN_POINT('Ctrl Pts',(25.1526570863065,5.97225131495636,12.));
#254951=CARTESIAN_POINT('Ctrl Pts',(25.1319431317273,5.95323180187348,0.));
#254952=CARTESIAN_POINT('Ctrl Pts',(25.1319431317273,5.95323180187348,12.));
#254953=CARTESIAN_POINT('Ctrl Pts',(25.1112375971182,5.93430523086776,0.));
#254954=CARTESIAN_POINT('Ctrl Pts',(25.1112375971182,5.93430523086776,12.));
#254955=CARTESIAN_POINT('Ctrl Pts',(25.0905409050863,5.91547170844382,0.));
#254956=CARTESIAN_POINT('Ctrl Pts',(25.0905409050863,5.91547170844382,12.));
#254957=CARTESIAN_POINT('Ctrl Pts',(25.0698535426593,5.89673135155459,0.));
#254958=CARTESIAN_POINT('Ctrl Pts',(25.0698535426593,5.89673135155459,12.));
#254959=CARTESIAN_POINT('Ctrl Pts',(25.0491760405965,5.87808428385329,0.));
#254960=CARTESIAN_POINT('Ctrl Pts',(25.0491760405965,5.87808428385329,12.));
#254961=CARTESIAN_POINT('Ctrl Pts',(25.0285089498922,5.8595306315681,0.));
#254962=CARTESIAN_POINT('Ctrl Pts',(25.0285089498922,5.8595306315681,12.));
#254963=CARTESIAN_POINT('Ctrl Pts',(25.0078528200558,5.84107051963074,0.));
#254964=CARTESIAN_POINT('Ctrl Pts',(25.0078528200558,5.84107051963074,12.));
#254965=CARTESIAN_POINT('Ctrl Pts',(24.9872081752709,5.82270406744214,0.));
#254966=CARTESIAN_POINT('Ctrl Pts',(24.9872081752709,5.82270406744214,12.));
#254967=CARTESIAN_POINT('Ctrl Pts',(24.9665754954462,5.80443138549747,0.));
#254968=CARTESIAN_POINT('Ctrl Pts',(24.9665754954462,5.80443138549747,12.));
#254969=CARTESIAN_POINT('Ctrl Pts',(24.9459552293308,5.78625257775703,0.));
#254970=CARTESIAN_POINT('Ctrl Pts',(24.9459552293308,5.78625257775703,12.));
#254971=CARTESIAN_POINT('Ctrl Pts',(24.9253478043632,5.76816774342236,0.));
#254972=CARTESIAN_POINT('Ctrl Pts',(24.9253478043632,5.76816774342236,12.));
#254973=CARTESIAN_POINT('Ctrl Pts',(24.9047536376467,5.75017697890813,0.));
#254974=CARTESIAN_POINT('Ctrl Pts',(24.9047536376467,5.75017697890813,12.));
#254975=CARTESIAN_POINT('Ctrl Pts',(24.8841731467219,5.73228037976927,0.));
#254976=CARTESIAN_POINT('Ctrl Pts',(24.8841731467219,5.73228037976927,12.));
#254977=CARTESIAN_POINT('Ctrl Pts',(24.8636067597677,5.71447804252019,0.));
#254978=CARTESIAN_POINT('Ctrl Pts',(24.8636067597677,5.71447804252019,12.));
#254979=CARTESIAN_POINT('Ctrl Pts',(24.8430549277634,5.6967700667943,0.));
#254980=CARTESIAN_POINT('Ctrl Pts',(24.8430549277634,5.6967700667943,12.));
#254981=CARTESIAN_POINT('Ctrl Pts',(24.822518122386,5.67915655496524,0.));
#254982=CARTESIAN_POINT('Ctrl Pts',(24.822518122386,5.67915655496524,12.));
#254983=CARTESIAN_POINT('Ctrl Pts',(24.8019968304618,5.66163761114903,0.));
#254984=CARTESIAN_POINT('Ctrl Pts',(24.8019968304618,5.66163761114903,12.));
#254985=CARTESIAN_POINT('Ctrl Pts',(24.7814915496728,5.64421334042248,0.));
#254986=CARTESIAN_POINT('Ctrl Pts',(24.7814915496728,5.64421334042248,12.));
#254987=CARTESIAN_POINT('Ctrl Pts',(24.76100278357,5.62688384790919,0.));
#254988=CARTESIAN_POINT('Ctrl Pts',(24.76100278357,5.62688384790919,12.));
#254989=CARTESIAN_POINT('Ctrl Pts',(24.7405310372736,5.60964923798495,0.));
#254990=CARTESIAN_POINT('Ctrl Pts',(24.7405310372736,5.60964923798495,12.));
#254991=CARTESIAN_POINT('Ctrl Pts',(24.7200768119079,5.59250961323995,0.));
#254992=CARTESIAN_POINT('Ctrl Pts',(24.7200768119079,5.59250961323995,12.));
#254993=CARTESIAN_POINT('Ctrl Pts',(24.6996406035507,5.57546507427767,0.));
#254994=CARTESIAN_POINT('Ctrl Pts',(24.6996406035507,5.57546507427767,12.));
#254995=CARTESIAN_POINT('Ctrl Pts',(24.6792229061785,5.55851572025389,0.));
#254996=CARTESIAN_POINT('Ctrl Pts',(24.6792229061785,5.55851572025389,12.));
#254997=CARTESIAN_POINT('Ctrl Pts',(24.6588242134733,5.54166164919593,0.));
#254998=CARTESIAN_POINT('Ctrl Pts',(24.6588242134733,5.54166164919593,12.));
#254999=CARTESIAN_POINT('Ctrl Pts',(24.6384450211466,5.52490295840996,0.));
#255000=CARTESIAN_POINT('Ctrl Pts',(24.6384450211466,5.52490295840996,12.));
#255001=CARTESIAN_POINT('Ctrl Pts',(24.618085828918,5.50823974481959,0.));
#255002=CARTESIAN_POINT('Ctrl Pts',(24.618085828918,5.50823974481959,12.));
#255003=CARTESIAN_POINT('Ctrl Pts',(24.5977471429365,5.49167210537235,0.));
#255004=CARTESIAN_POINT('Ctrl Pts',(24.5977471429365,5.49167210537235,12.));
#255005=CARTESIAN_POINT('Ctrl Pts',(24.5774294770329,5.47520013724403,0.));
#255006=CARTESIAN_POINT('Ctrl Pts',(24.5774294770329,5.47520013724403,12.));
#255007=CARTESIAN_POINT('Ctrl Pts',(24.5571333514841,5.45882393762244,0.));
#255008=CARTESIAN_POINT('Ctrl Pts',(24.5571333514841,5.45882393762244,12.));
#255009=CARTESIAN_POINT('Ctrl Pts',(24.5368592922861,5.44254360356866,0.));
#255010=CARTESIAN_POINT('Ctrl Pts',(24.5368592922861,5.44254360356866,12.));
#255011=CARTESIAN_POINT('Ctrl Pts',(24.5166078302107,5.42635923183411,0.));
#255012=CARTESIAN_POINT('Ctrl Pts',(24.5166078302107,5.42635923183411,12.));
#255013=CARTESIAN_POINT('Ctrl Pts',(24.4963794999831,5.41027091869242,0.));
#255014=CARTESIAN_POINT('Ctrl Pts',(24.4963794999831,5.41027091869242,12.));
#255015=CARTESIAN_POINT('Ctrl Pts',(24.4761748393322,5.39427875973831,0.));
#255016=CARTESIAN_POINT('Ctrl Pts',(24.4761748393322,5.39427875973831,12.));
#255017=CARTESIAN_POINT('Ctrl Pts',(24.4559943883159,5.37838284973706,0.));
#255018=CARTESIAN_POINT('Ctrl Pts',(24.4559943883159,5.37838284973706,12.));
#255019=CARTESIAN_POINT('Ctrl Pts',(24.4358386899152,5.36258328273639,0.));
#255020=CARTESIAN_POINT('Ctrl Pts',(24.4358386899152,5.36258328273639,12.));
#255021=CARTESIAN_POINT('Ctrl Pts',(24.4157082904615,5.34688015213546,0.));
#255022=CARTESIAN_POINT('Ctrl Pts',(24.4157082904615,5.34688015213546,12.));
#255023=CARTESIAN_POINT('Ctrl Pts',(24.3956037401293,5.33127355076037,0.));
#255024=CARTESIAN_POINT('Ctrl Pts',(24.3956037401293,5.33127355076037,12.));
#255025=CARTESIAN_POINT('Ctrl Pts',(24.3755255933917,5.31576357092525,0.));
#255026=CARTESIAN_POINT('Ctrl Pts',(24.3755255933917,5.31576357092525,12.));
#255027=CARTESIAN_POINT('Ctrl Pts',(24.3554744095075,5.30035030449059,0.));
#255028=CARTESIAN_POINT('Ctrl Pts',(24.3554744095075,5.30035030449059,12.));
#255029=CARTESIAN_POINT('Ctrl Pts',(24.3354507529415,5.28503384290644,0.));
#255030=CARTESIAN_POINT('Ctrl Pts',(24.3354507529415,5.28503384290644,12.));
#255031=CARTESIAN_POINT('Ctrl Pts',(24.3154551932222,5.26981427718796,0.));
#255032=CARTESIAN_POINT('Ctrl Pts',(24.3154551932222,5.26981427718796,12.));
#255033=CARTESIAN_POINT('Ctrl Pts',(24.2954883048448,5.25469169788856,0.));
#255034=CARTESIAN_POINT('Ctrl Pts',(24.2954883048448,5.25469169788856,12.));
#255035=CARTESIAN_POINT('Ctrl Pts',(24.2755506671526,5.23966619506289,0.));
#255036=CARTESIAN_POINT('Ctrl Pts',(24.2755506671526,5.23966619506289,12.));
#255037=CARTESIAN_POINT('Ctrl Pts',(24.2556428642294,5.22473785822441,0.));
#255038=CARTESIAN_POINT('Ctrl Pts',(24.2556428642294,5.22473785822441,12.));
#255039=CARTESIAN_POINT('Ctrl Pts',(24.2357654847765,5.20990677629173,0.));
#255040=CARTESIAN_POINT('Ctrl Pts',(24.2357654847765,5.20990677629173,12.));
#255041=CARTESIAN_POINT('Ctrl Pts',(24.215919122017,5.19517303753643,0.));
#255042=CARTESIAN_POINT('Ctrl Pts',(24.215919122017,5.19517303753643,12.));
#255043=CARTESIAN_POINT('Ctrl Pts',(24.1961043738754,5.18053672961392,0.));
#255044=CARTESIAN_POINT('Ctrl Pts',(24.1961043738754,5.18053672961392,12.));
#255045=CARTESIAN_POINT('Ctrl Pts',(24.1763218431343,5.16599793957979,0.));
#255046=CARTESIAN_POINT('Ctrl Pts',(24.1763218431343,5.16599793957979,12.));
#255047=CARTESIAN_POINT('Ctrl Pts',(24.156572137597,5.15155675390075,0.));
#255048=CARTESIAN_POINT('Ctrl Pts',(24.156572137597,5.15155675390075,12.));
#255049=CARTESIAN_POINT('Ctrl Pts',(24.1368558702443,5.13721325845745,0.));
#255050=CARTESIAN_POINT('Ctrl Pts',(24.1368558702443,5.13721325845745,12.));
#255051=CARTESIAN_POINT('Ctrl Pts',(24.117173659394,5.1229675385386,0.));
#255052=CARTESIAN_POINT('Ctrl Pts',(24.117173659394,5.1229675385386,12.));
#255053=CARTESIAN_POINT('Ctrl Pts',(24.0975261288446,5.10881967883132,0.));
#255054=CARTESIAN_POINT('Ctrl Pts',(24.0975261288446,5.10881967883132,12.));
#255055=CARTESIAN_POINT('Ctrl Pts',(24.0779139079266,5.09476976342625,0.));
#255056=CARTESIAN_POINT('Ctrl Pts',(24.0779139079266,5.09476976342625,12.));
#255057=CARTESIAN_POINT('Ctrl Pts',(24.0583376315638,5.08081787581277,0.));
#255058=CARTESIAN_POINT('Ctrl Pts',(24.0583376315638,5.08081787581277,12.));
#255059=CARTESIAN_POINT('Ctrl Pts',(24.0387979403268,5.06696409886641,0.));
#255060=CARTESIAN_POINT('Ctrl Pts',(24.0387979403268,5.06696409886641,12.));
#255061=CARTESIAN_POINT('Ctrl Pts',(24.0192954804896,5.05320851483065,0.));
#255062=CARTESIAN_POINT('Ctrl Pts',(24.0192954804896,5.05320851483065,12.));
#255063=CARTESIAN_POINT('Ctrl Pts',(23.9998309040746,5.03955120528521,0.));
#255064=CARTESIAN_POINT('Ctrl Pts',(23.9998309040746,5.03955120528521,12.));
#255065=CARTESIAN_POINT('Ctrl Pts',(23.9804048689227,5.02599225112454,0.));
#255066=CARTESIAN_POINT('Ctrl Pts',(23.9804048689227,5.02599225112454,12.));
#255067=CARTESIAN_POINT('Ctrl Pts',(23.961018038827,5.01253173257453,0.));
#255068=CARTESIAN_POINT('Ctrl Pts',(23.961018038827,5.01253173257453,12.));
#255069=CARTESIAN_POINT('Ctrl Pts',(23.9416710836529,4.99916972919307,0.));
#255070=CARTESIAN_POINT('Ctrl Pts',(23.9416710836529,4.99916972919307,12.));
#255071=CARTESIAN_POINT('Ctrl Pts',(23.9223646794592,4.98590631986533,0.));
#255072=CARTESIAN_POINT('Ctrl Pts',(23.9223646794592,4.98590631986533,12.));
#255073=CARTESIAN_POINT('Ctrl Pts',(23.9030995086163,4.97274158279227,0.));
#255074=CARTESIAN_POINT('Ctrl Pts',(23.9030995086163,4.97274158279227,12.));
#255075=CARTESIAN_POINT('Ctrl Pts',(23.8838762599218,4.95967559546561,0.));
#255076=CARTESIAN_POINT('Ctrl Pts',(23.8838762599218,4.95967559546561,12.));
#255077=CARTESIAN_POINT('Ctrl Pts',(23.8646956287168,4.9467084346586,0.));
#255078=CARTESIAN_POINT('Ctrl Pts',(23.8646956287168,4.9467084346586,12.));
#255079=CARTESIAN_POINT('Ctrl Pts',(23.8455583170057,4.93384017643432,0.));
#255080=CARTESIAN_POINT('Ctrl Pts',(23.8455583170057,4.93384017643432,12.));
#255081=CARTESIAN_POINT('Ctrl Pts',(23.8264650335717,4.92107089613969,0.));
#255082=CARTESIAN_POINT('Ctrl Pts',(23.8264650335717,4.92107089613969,12.));
#255083=CARTESIAN_POINT('Ctrl Pts',(23.8074164940896,4.90840066839344,0.));
#255084=CARTESIAN_POINT('Ctrl Pts',(23.8074164940896,4.90840066839344,12.));
#255085=CARTESIAN_POINT('Ctrl Pts',(23.7884134212384,4.89582956706775,0.));
#255086=CARTESIAN_POINT('Ctrl Pts',(23.7884134212384,4.89582956706775,12.));
#255087=CARTESIAN_POINT('Ctrl Pts',(23.7694565448049,4.88335766525573,0.));
#255088=CARTESIAN_POINT('Ctrl Pts',(23.7694565448049,4.88335766525573,12.));
#255089=CARTESIAN_POINT('Ctrl Pts',(23.7505466018245,4.87098503527152,0.));
#255090=CARTESIAN_POINT('Ctrl Pts',(23.7505466018245,4.87098503527152,12.));
#255091=CARTESIAN_POINT('Ctrl Pts',(23.7316843367313,4.85871174865499,0.));
#255092=CARTESIAN_POINT('Ctrl Pts',(23.7316843367313,4.85871174865499,12.));
#255093=CARTESIAN_POINT('Ctrl Pts',(23.7128705015017,4.84653787616426,0.));
#255094=CARTESIAN_POINT('Ctrl Pts',(23.7128705015017,4.84653787616426,12.));
#255095=CARTESIAN_POINT('Ctrl Pts',(23.6941058557971,4.83446348776266,0.));
#255096=CARTESIAN_POINT('Ctrl Pts',(23.6941058557971,4.83446348776266,12.));
#255097=CARTESIAN_POINT('Ctrl Pts',(23.675391167102,4.82248865259562,0.));
#255098=CARTESIAN_POINT('Ctrl Pts',(23.675391167102,4.82248865259562,12.));
#255099=CARTESIAN_POINT('Ctrl Pts',(23.6567272108628,4.81061343896432,0.));
#255100=CARTESIAN_POINT('Ctrl Pts',(23.6567272108628,4.81061343896432,12.));
#255101=CARTESIAN_POINT('Ctrl Pts',(23.6381147706579,4.7988379143322,0.));
#255102=CARTESIAN_POINT('Ctrl Pts',(23.6381147706579,4.7988379143322,12.));
#255103=CARTESIAN_POINT('Ctrl Pts',(23.6195546383624,4.78716214532098,0.));
#255104=CARTESIAN_POINT('Ctrl Pts',(23.6195546383624,4.78716214532098,12.));
#255105=CARTESIAN_POINT('Ctrl Pts',(23.6010476143099,4.77558619769872,0.));
#255106=CARTESIAN_POINT('Ctrl Pts',(23.6010476143099,4.77558619769872,12.));
#255107=CARTESIAN_POINT('Ctrl Pts',(23.5825945074535,4.76411013636251,0.));
#255108=CARTESIAN_POINT('Ctrl Pts',(23.5825945074535,4.76411013636251,12.));
#255109=CARTESIAN_POINT('Ctrl Pts',(23.5641961355168,4.75273402530617,0.));
#255110=CARTESIAN_POINT('Ctrl Pts',(23.5641961355168,4.75273402530617,12.));
#255111=CARTESIAN_POINT('Ctrl Pts',(23.545853325171,4.74145792760699,0.));
#255112=CARTESIAN_POINT('Ctrl Pts',(23.545853325171,4.74145792760699,12.));
#255113=CARTESIAN_POINT('Ctrl Pts',(23.5275669122372,4.7302819054303,0.));
#255114=CARTESIAN_POINT('Ctrl Pts',(23.5275669122372,4.7302819054303,12.));
#255115=CARTESIAN_POINT('Ctrl Pts',(23.509337741878,4.71920602001902,0.));
#255116=CARTESIAN_POINT('Ctrl Pts',(23.509337741878,4.71920602001902,12.));
#255117=CARTESIAN_POINT('Ctrl Pts',(23.491166668789,4.70823033167819,0.));
#255118=CARTESIAN_POINT('Ctrl Pts',(23.491166668789,4.70823033167819,12.));
#255119=CARTESIAN_POINT('Ctrl Pts',(23.4730545573853,4.69735489975024,0.));
#255120=CARTESIAN_POINT('Ctrl Pts',(23.4730545573853,4.69735489975024,12.));
#255121=CARTESIAN_POINT('Ctrl Pts',(23.455002281986,4.68657978258303,0.));
#255122=CARTESIAN_POINT('Ctrl Pts',(23.455002281986,4.68657978258303,12.));
#255123=CARTESIAN_POINT('Ctrl Pts',(23.4370107270451,4.67590503753059,0.));
#255124=CARTESIAN_POINT('Ctrl Pts',(23.4370107270451,4.67590503753059,12.));
#255125=CARTESIAN_POINT('Ctrl Pts',(23.4190807873803,4.6653307209467,0.));
#255126=CARTESIAN_POINT('Ctrl Pts',(23.4190807873803,4.6653307209467,12.));
#255127=CARTESIAN_POINT('Ctrl Pts',(23.4012133683959,4.65485688816924,0.));
#255128=CARTESIAN_POINT('Ctrl Pts',(23.4012133683959,4.65485688816924,12.));
#255129=CARTESIAN_POINT('Ctrl Pts',(23.3834093863068,4.6444835934993,0.));
#255130=CARTESIAN_POINT('Ctrl Pts',(23.3834093863068,4.6444835934993,12.));
#255131=CARTESIAN_POINT('Ctrl Pts',(23.3656697683489,4.63421089016541,0.));
#255132=CARTESIAN_POINT('Ctrl Pts',(23.3656697683489,4.63421089016541,12.));
#255133=CARTESIAN_POINT('Ctrl Pts',(23.3479954530272,4.62403883030805,0.));
#255134=CARTESIAN_POINT('Ctrl Pts',(23.3479954530272,4.62403883030805,12.));
#255135=CARTESIAN_POINT('Ctrl Pts',(23.3303873903938,4.6139674649783,0.));
#255136=CARTESIAN_POINT('Ctrl Pts',(23.3303873903938,4.6139674649783,12.));
#255137=CARTESIAN_POINT('Ctrl Pts',(23.3128465423115,4.60399684412163,0.));
#255138=CARTESIAN_POINT('Ctrl Pts',(23.3128465423115,4.60399684412163,12.));
#255139=CARTESIAN_POINT('Ctrl Pts',(23.2953738827191,4.5941270165575,0.));
#255140=CARTESIAN_POINT('Ctrl Pts',(23.2953738827191,4.5941270165575,12.));
#255141=CARTESIAN_POINT('Ctrl Pts',(23.2779703978876,4.5843580299469,0.));
#255142=CARTESIAN_POINT('Ctrl Pts',(23.2779703978876,4.5843580299469,12.));
#255143=CARTESIAN_POINT('Ctrl Pts',(23.2606370866866,4.57468993076097,0.));
#255144=CARTESIAN_POINT('Ctrl Pts',(23.2606370866866,4.57468993076097,12.));
#255145=CARTESIAN_POINT('Ctrl Pts',(23.2433749609131,4.56512276427839,0.));
#255146=CARTESIAN_POINT('Ctrl Pts',(23.2433749609131,4.56512276427839,12.));
#255147=CARTESIAN_POINT('Ctrl Pts',(23.2261850456064,4.55565657456975,0.));
#255148=CARTESIAN_POINT('Ctrl Pts',(23.2261850456064,4.55565657456975,12.));
#255149=CARTESIAN_POINT('Ctrl Pts',(23.2090683793629,4.54629140447544,0.));
#255150=CARTESIAN_POINT('Ctrl Pts',(23.2090683793629,4.54629140447544,12.));
#255151=CARTESIAN_POINT('Ctrl Pts',(23.1920260146465,4.53702729557566,0.));
#255152=CARTESIAN_POINT('Ctrl Pts',(23.1920260146465,4.53702729557566,12.));
#255153=CARTESIAN_POINT('Ctrl Pts',(23.1750590180908,4.52786428815015,0.));
#255154=CARTESIAN_POINT('Ctrl Pts',(23.1750590180908,4.52786428815015,12.));
#255155=CARTESIAN_POINT('Ctrl Pts',(23.1581684708761,4.51880242116748,0.));
#255156=CARTESIAN_POINT('Ctrl Pts',(23.1581684708761,4.51880242116748,12.));
#255157=CARTESIAN_POINT('Ctrl Pts',(23.1413554691123,4.5098417322706,0.));
#255158=CARTESIAN_POINT('Ctrl Pts',(23.1413554691123,4.5098417322706,12.));
#255159=CARTESIAN_POINT('Ctrl Pts',(23.1246211242115,4.50098225775171,0.));
#255160=CARTESIAN_POINT('Ctrl Pts',(23.1246211242115,4.50098225775171,12.));
#255161=CARTESIAN_POINT('Ctrl Pts',(23.1079665632636,4.49222403252216,0.));
#255162=CARTESIAN_POINT('Ctrl Pts',(23.1079665632636,4.49222403252216,12.));
#255163=CARTESIAN_POINT('Ctrl Pts',(23.0913929293922,4.48356709006788,0.));
#255164=CARTESIAN_POINT('Ctrl Pts',(23.0913929293922,4.48356709006788,12.));
#255165=CARTESIAN_POINT('Ctrl Pts',(23.0749013821881,4.47501146242856,0.));
#255166=CARTESIAN_POINT('Ctrl Pts',(23.0749013821881,4.47501146242856,12.));
#255167=CARTESIAN_POINT('Ctrl Pts',(23.0584930981732,4.46655718018231,0.));
#255168=CARTESIAN_POINT('Ctrl Pts',(23.0584930981732,4.46655718018231,12.));
#255169=CARTESIAN_POINT('Ctrl Pts',(23.0421692712467,4.45820427241683,0.));
#255170=CARTESIAN_POINT('Ctrl Pts',(23.0421692712467,4.45820427241683,12.));
#255171=CARTESIAN_POINT('Ctrl Pts',(23.0259311131392,4.44995276669687,0.));
#255172=CARTESIAN_POINT('Ctrl Pts',(23.0259311131392,4.44995276669687,12.));
#255173=CARTESIAN_POINT('Ctrl Pts',(23.0097798538395,4.44180268901643,0.));
#255174=CARTESIAN_POINT('Ctrl Pts',(23.0097798538395,4.44180268901643,12.));
#255175=CARTESIAN_POINT('Ctrl Pts',(22.9937167421006,4.43375406376879,0.));
#255176=CARTESIAN_POINT('Ctrl Pts',(22.9937167421006,4.43375406376879,12.));
#255177=CARTESIAN_POINT('Ctrl Pts',(22.977743046002,4.42580691372752,0.));
#255178=CARTESIAN_POINT('Ctrl Pts',(22.977743046002,4.42580691372752,12.));
#255179=CARTESIAN_POINT('Ctrl Pts',(22.9618600534866,4.41796126001302,0.));
#255180=CARTESIAN_POINT('Ctrl Pts',(22.9618600534866,4.41796126001302,12.));
#255181=CARTESIAN_POINT('Ctrl Pts',(22.9460690729093,4.41021712205554,0.));
#255182=CARTESIAN_POINT('Ctrl Pts',(22.9460690729093,4.41021712205554,12.));
#255183=CARTESIAN_POINT('Ctrl Pts',(22.930371433555,4.40257451754324,0.));
#255184=CARTESIAN_POINT('Ctrl Pts',(22.930371433555,4.40257451754324,12.));
#255185=CARTESIAN_POINT('Ctrl Pts',(22.9147684862426,4.39503346238473,0.));
#255186=CARTESIAN_POINT('Ctrl Pts',(22.9147684862426,4.39503346238473,12.));
#255187=CARTESIAN_POINT('Ctrl Pts',(22.8992616040108,4.38759397068406,0.));
#255188=CARTESIAN_POINT('Ctrl Pts',(22.8992616040108,4.38759397068406,12.));
#255189=CARTESIAN_POINT('Ctrl Pts',(22.8838521827701,4.38025605470093,0.));
#255190=CARTESIAN_POINT('Ctrl Pts',(22.8838521827701,4.38025605470093,12.));
#255191=CARTESIAN_POINT('Ctrl Pts',(22.8685416419725,4.37301972480746,0.));
#255192=CARTESIAN_POINT('Ctrl Pts',(22.8685416419725,4.37301972480746,12.));
#255193=CARTESIAN_POINT('Ctrl Pts',(22.8533314252422,4.36588498942997,0.));
#255194=CARTESIAN_POINT('Ctrl Pts',(22.8533314252422,4.36588498942997,12.));
#255195=CARTESIAN_POINT('Ctrl Pts',(22.8382230011184,4.35885185500546,0.));
#255196=CARTESIAN_POINT('Ctrl Pts',(22.8382230011184,4.35885185500546,12.));
#255197=CARTESIAN_POINT('Ctrl Pts',(22.8232178638876,4.35192032594791,0.));
#255198=CARTESIAN_POINT('Ctrl Pts',(22.8232178638876,4.35192032594791,12.));
#255199=CARTESIAN_POINT('Ctrl Pts',(22.8083175343791,4.34509040460062,0.));
#255200=CARTESIAN_POINT('Ctrl Pts',(22.8083175343791,4.34509040460062,12.));
#255201=CARTESIAN_POINT('Ctrl Pts',(22.7935235607806,4.33836209118446,0.));
#255202=CARTESIAN_POINT('Ctrl Pts',(22.7935235607806,4.33836209118446,12.));
#255203=CARTESIAN_POINT('Ctrl Pts',(22.7788375194076,4.3317353837319,0.));
#255204=CARTESIAN_POINT('Ctrl Pts',(22.7788375194076,4.3317353837319,12.));
#255205=CARTESIAN_POINT('Ctrl Pts',(22.7642610156475,4.32521027803754,0.));
#255206=CARTESIAN_POINT('Ctrl Pts',(22.7642610156475,4.32521027803754,12.));
#255207=CARTESIAN_POINT('Ctrl Pts',(22.7497956849848,4.31878676761235,0.));
#255208=CARTESIAN_POINT('Ctrl Pts',(22.7497956849848,4.31878676761235,12.));
#255209=CARTESIAN_POINT('Ctrl Pts',(22.7354431939926,4.31246484362549,0.));
#255210=CARTESIAN_POINT('Ctrl Pts',(22.7354431939926,4.31246484362549,12.));
#255211=CARTESIAN_POINT('Ctrl Pts',(22.7212052413386,4.30624449484069,0.));
#255212=CARTESIAN_POINT('Ctrl Pts',(22.7212052413386,4.30624449484069,12.));
#255213=CARTESIAN_POINT('Ctrl Pts',(22.7070835587564,4.3001257075406,0.));
#255214=CARTESIAN_POINT('Ctrl Pts',(22.7070835587564,4.3001257075406,12.));
#255215=CARTESIAN_POINT('Ctrl Pts',(22.6930799122548,4.29410846547056,0.));
#255216=CARTESIAN_POINT('Ctrl Pts',(22.6930799122548,4.29410846547056,12.));
#255217=CARTESIAN_POINT('Ctrl Pts',(22.6791961033537,4.28819274977763,0.));
#255218=CARTESIAN_POINT('Ctrl Pts',(22.6791961033537,4.28819274977763,12.));
#255219=CARTESIAN_POINT('Ctrl Pts',(22.6654339703109,4.28237853894059,0.));
#255220=CARTESIAN_POINT('Ctrl Pts',(22.6654339703109,4.28237853894059,12.));
#255221=CARTESIAN_POINT('Ctrl Pts',(22.6517953893303,4.2766658086912,0.));
#255222=CARTESIAN_POINT('Ctrl Pts',(22.6517953893303,4.2766658086912,12.));
#255223=CARTESIAN_POINT('Ctrl Pts',(22.6382822758172,4.27105453193004,0.));
#255224=CARTESIAN_POINT('Ctrl Pts',(22.6382822758172,4.27105453193004,12.));
#255225=CARTESIAN_POINT('Ctrl Pts',(22.6248965859977,4.26554467865576,0.));
#255226=CARTESIAN_POINT('Ctrl Pts',(22.6248965859977,4.26554467865576,12.));
#255227=CARTESIAN_POINT('Ctrl Pts',(22.6116403184821,4.26013621588305,0.));
#255228=CARTESIAN_POINT('Ctrl Pts',(22.6116403184821,4.26013621588305,12.));
#255229=CARTESIAN_POINT('Ctrl Pts',(22.5985155158636,4.25482910755481,0.));
#255230=CARTESIAN_POINT('Ctrl Pts',(22.5985155158636,4.25482910755481,12.));
#255231=CARTESIAN_POINT('Ctrl Pts',(22.5855242662477,4.24962331444177,0.));
#255232=CARTESIAN_POINT('Ctrl Pts',(22.5855242662477,4.24962331444177,12.));
#255233=CARTESIAN_POINT('Ctrl Pts',(22.572668704992,4.24451879404851,0.));
#255234=CARTESIAN_POINT('Ctrl Pts',(22.572668704992,4.24451879404851,12.));
#255235=CARTESIAN_POINT('Ctrl Pts',(22.5599510166429,4.23951550052523,0.));
#255236=CARTESIAN_POINT('Ctrl Pts',(22.5599510166429,4.23951550052523,12.));
#255237=CARTESIAN_POINT('Ctrl Pts',(22.5473734368086,4.23461338456712,0.));
#255238=CARTESIAN_POINT('Ctrl Pts',(22.5473734368086,4.23461338456712,12.));
#255239=CARTESIAN_POINT('Ctrl Pts',(22.5349382540588,4.22981239330733,0.));
#255240=CARTESIAN_POINT('Ctrl Pts',(22.5349382540588,4.22981239330733,12.));
#255241=CARTESIAN_POINT('Ctrl Pts',(22.5226478117886,4.22511247020041,0.));
#255242=CARTESIAN_POINT('Ctrl Pts',(22.5226478117886,4.22511247020041,12.));
#255243=CARTESIAN_POINT('Ctrl Pts',(22.5105045108881,4.22051355490196,0.));
#255244=CARTESIAN_POINT('Ctrl Pts',(22.5105045108881,4.22051355490196,12.));
#255245=CARTESIAN_POINT('Ctrl Pts',(22.4985108124228,4.21601558313906,0.));
#255246=CARTESIAN_POINT('Ctrl Pts',(22.4985108124228,4.21601558313906,12.));
#255247=CARTESIAN_POINT('Ctrl Pts',(22.4866692403147,4.21161848657428,0.));
#255248=CARTESIAN_POINT('Ctrl Pts',(22.4866692403147,4.21161848657428,12.));
#255249=CARTESIAN_POINT('Ctrl Pts',(22.4749823839917,4.20732219265649,0.));
#255250=CARTESIAN_POINT('Ctrl Pts',(22.4749823839917,4.20732219265649,12.));
#255251=CARTESIAN_POINT('Ctrl Pts',(22.4634529011437,4.20312662448174,0.));
#255252=CARTESIAN_POINT('Ctrl Pts',(22.4634529011437,4.20312662448174,12.));
#255253=CARTESIAN_POINT('Ctrl Pts',(22.4520835205422,4.19903170066358,0.));
#255254=CARTESIAN_POINT('Ctrl Pts',(22.4520835205422,4.19903170066358,12.));
#255255=CARTESIAN_POINT('Ctrl Pts',(22.4408770448917,4.1950373351886,0.));
#255256=CARTESIAN_POINT('Ctrl Pts',(22.4408770448917,4.1950373351886,12.));
#255257=CARTESIAN_POINT('Ctrl Pts',(22.4298363535416,4.19114343726932,0.));
#255258=CARTESIAN_POINT('Ctrl Pts',(22.4298363535416,4.19114343726932,12.));
#255259=CARTESIAN_POINT('Ctrl Pts',(22.4189644056109,4.18734991117707,0.));
#255260=CARTESIAN_POINT('Ctrl Pts',(22.4189644056109,4.18734991117707,12.));
#255261=CARTESIAN_POINT('Ctrl Pts',(22.4082642454448,4.18365665600839,0.));
#255262=CARTESIAN_POINT('Ctrl Pts',(22.4082642454448,4.18365665600839,12.));
#255263=CARTESIAN_POINT('Ctrl Pts',(22.3977390078074,4.18006356544879,0.));
#255264=CARTESIAN_POINT('Ctrl Pts',(22.3977390078074,4.18006356544879,12.));
#255265=CARTESIAN_POINT('Ctrl Pts',(22.3873919231339,4.17657052752834,0.));
#255266=CARTESIAN_POINT('Ctrl Pts',(22.3873919231339,4.17657052752834,12.));
#255267=CARTESIAN_POINT('Ctrl Pts',(22.3772263228624,4.17317742436162,0.));
#255268=CARTESIAN_POINT('Ctrl Pts',(22.3772263228624,4.17317742436162,12.));
#255269=CARTESIAN_POINT('Ctrl Pts',(22.3672456427605,4.1698841319947,0.));
#255270=CARTESIAN_POINT('Ctrl Pts',(22.3672456427605,4.1698841319947,12.));
#255271=CARTESIAN_POINT('Ctrl Pts',(22.3574534257397,4.16669052026602,0.));
#255272=CARTESIAN_POINT('Ctrl Pts',(22.3574534257397,4.16669052026602,12.));
#255273=CARTESIAN_POINT('Ctrl Pts',(22.3478533253886,4.1635964526318,0.));
#255274=CARTESIAN_POINT('Ctrl Pts',(22.3478533253886,4.1635964526318,12.));
#255275=CARTESIAN_POINT('Ctrl Pts',(22.3384491078599,4.16060178604154,0.));
#255276=CARTESIAN_POINT('Ctrl Pts',(22.3384491078599,4.16060178604154,12.));
#255277=CARTESIAN_POINT('Ctrl Pts',(22.3292446628957,4.15770637047882,0.));
#255278=CARTESIAN_POINT('Ctrl Pts',(22.3292446628957,4.15770637047882,12.));
#255279=CARTESIAN_POINT('Ctrl Pts',(22.3202440186979,4.15491004835278,0.));
#255280=CARTESIAN_POINT('Ctrl Pts',(22.3202440186979,4.15491004835278,12.));
#255281=CARTESIAN_POINT('Ctrl Pts',(22.3114513545186,4.15221265396993,0.));
#255282=CARTESIAN_POINT('Ctrl Pts',(22.3114513545186,4.15221265396993,12.));
#255283=CARTESIAN_POINT('Ctrl Pts',(22.3028710166935,4.14961401285526,0.));
#255284=CARTESIAN_POINT('Ctrl Pts',(22.3028710166935,4.14961401285526,12.));
#255285=CARTESIAN_POINT('Ctrl Pts',(22.2945075198468,4.14711394168559,0.));
#255286=CARTESIAN_POINT('Ctrl Pts',(22.2945075198468,4.14711394168559,12.));
#255287=CARTESIAN_POINT('Ctrl Pts',(22.2863655389167,4.14471224859295,0.));
#255288=CARTESIAN_POINT('Ctrl Pts',(22.2863655389167,4.14471224859295,12.));
#255289=CARTESIAN_POINT('Ctrl Pts',(22.2784499072026,4.14240873321982,0.));
#255290=CARTESIAN_POINT('Ctrl Pts',(22.2784499072026,4.14240873321982,12.));
#255291=CARTESIAN_POINT('Ctrl Pts',(22.2707656042456,4.14020318715988,0.));
#255292=CARTESIAN_POINT('Ctrl Pts',(22.2707656042456,4.14020318715988,12.));
#255293=CARTESIAN_POINT('Ctrl Pts',(22.263317791397,4.13809539255419,0.));
#255294=CARTESIAN_POINT('Ctrl Pts',(22.263317791397,4.13809539255419,12.));
#255295=CARTESIAN_POINT('Ctrl Pts',(22.2561118708422,4.13608511977226,0.));
#255296=CARTESIAN_POINT('Ctrl Pts',(22.2561118708422,4.13608511977226,12.));
#255297=CARTESIAN_POINT('Ctrl Pts',(22.2491535317789,4.13417212558809,0.));
#255298=CARTESIAN_POINT('Ctrl Pts',(22.2491535317789,4.13417212558809,12.));
#255299=CARTESIAN_POINT('Ctrl Pts',(22.2424488153523,4.1323561506016,0.));
#255300=CARTESIAN_POINT('Ctrl Pts',(22.2424488153523,4.1323561506016,12.));
#255301=CARTESIAN_POINT('Ctrl Pts',(22.2360040565534,4.13063692157499,0.));
#255302=CARTESIAN_POINT('Ctrl Pts',(22.2360040565534,4.13063692157499,12.));
#255303=CARTESIAN_POINT('Ctrl Pts',(22.2298258043947,4.12901415463379,0.));
#255304=CARTESIAN_POINT('Ctrl Pts',(22.2298258043947,4.12901415463379,12.));
#255305=CARTESIAN_POINT('Ctrl Pts',(22.2239207458781,4.127487558301,0.));
#255306=CARTESIAN_POINT('Ctrl Pts',(22.2239207458781,4.127487558301,12.));
#255307=CARTESIAN_POINT('Ctrl Pts',(22.2182956401341,4.126056836133,0.));
#255308=CARTESIAN_POINT('Ctrl Pts',(22.2182956401341,4.126056836133,12.));
#255309=CARTESIAN_POINT('Ctrl Pts',(22.2129576146671,4.12472167516602,0.));
#255310=CARTESIAN_POINT('Ctrl Pts',(22.2129576146671,4.12472167516602,12.));
#255311=CARTESIAN_POINT('Ctrl Pts',(22.2079143941719,4.12348173702025,0.));
#255312=CARTESIAN_POINT('Ctrl Pts',(22.2079143941719,4.12348173702025,12.));
#255313=CARTESIAN_POINT('Ctrl Pts',(22.2031746532106,4.12233664408237,0.));
#255314=CARTESIAN_POINT('Ctrl Pts',(22.2031746532106,4.12233664408237,12.));
#255315=CARTESIAN_POINT('Ctrl Pts',(22.1987479618246,4.12128598183533,0.));
#255316=CARTESIAN_POINT('Ctrl Pts',(22.1987479618246,4.12128598183533,12.));
#255317=CARTESIAN_POINT('Ctrl Pts',(22.1946440958098,4.12032932637738,0.));
#255318=CARTESIAN_POINT('Ctrl Pts',(22.1946440958098,4.12032932637738,12.));
#255319=CARTESIAN_POINT('Ctrl Pts',(22.1908725908525,4.11946626228623,0.));
#255320=CARTESIAN_POINT('Ctrl Pts',(22.1908725908525,4.11946626228623,12.));
#255321=CARTESIAN_POINT('Ctrl Pts',(22.1874419861496,4.11869641271752,0.));
#255322=CARTESIAN_POINT('Ctrl Pts',(22.1874419861496,4.11869641271752,12.));
#255323=CARTESIAN_POINT('Ctrl Pts',(22.1843613164855,4.11801938107464,0.));
#255324=CARTESIAN_POINT('Ctrl Pts',(22.1843613164855,4.11801938107464,12.));
#255325=CARTESIAN_POINT('Ctrl Pts',(22.1816414985788,4.11743469691765,0.));
#255326=CARTESIAN_POINT('Ctrl Pts',(22.1816414985788,4.11743469691765,12.));
#255327=CARTESIAN_POINT('Ctrl Pts',(22.179297473024,4.11694173195041,0.));
#255328=CARTESIAN_POINT('Ctrl Pts',(22.179297473024,4.11694173195041,12.));
#255329=CARTESIAN_POINT('Ctrl Pts',(22.177347426894,4.11653973150558,0.));
#255330=CARTESIAN_POINT('Ctrl Pts',(22.177347426894,4.11653973150558,12.));
#255331=CARTESIAN_POINT('Ctrl Pts',(22.1758088296598,4.11622797217066,0.));
#255332=CARTESIAN_POINT('Ctrl Pts',(22.1758088296598,4.11622797217066,12.));
#255333=CARTESIAN_POINT('Ctrl Pts',(22.1746949858773,4.11600589882768,0.));
#255334=CARTESIAN_POINT('Ctrl Pts',(22.1746949858773,4.11600589882768,12.));
#255335=CARTESIAN_POINT('Ctrl Pts',(22.174148802123,4.11589976826061,0.));
#255336=CARTESIAN_POINT('Ctrl Pts',(22.174148802123,4.11589976826061,12.));
#255337=CARTESIAN_POINT('Ctrl Pts',(22.1739341411684,4.1158603587821,0.));
#255338=CARTESIAN_POINT('Ctrl Pts',(22.1739341411684,4.1158603587821,12.));
#255339=CARTESIAN_POINT('Ctrl Pts',(22.1738776823239,4.11585194677412,0.));
#255340=CARTESIAN_POINT('Ctrl Pts',(22.1738776823239,4.11585194677412,12.));
#255341=CARTESIAN_POINT('Ctrl Pts',(22.1738711152697,4.11585220600461,0.));
#255342=CARTESIAN_POINT('Ctrl Pts',(22.1738711152697,4.11585220600461,12.));
#255343=CARTESIAN_POINT('Ctrl Pts',(22.4835757167854,1.76341220531179,0.));
#255344=CARTESIAN_POINT('Ctrl Pts',(22.4835757167854,1.76341220531179,12.));
#255345=CARTESIAN_POINT('Ctrl Pts',(22.483581992979,1.76341415538764,0.));
#255346=CARTESIAN_POINT('Ctrl Pts',(22.483581992979,1.76341415538764,12.));
#255347=CARTESIAN_POINT('Ctrl Pts',(22.4836387052232,1.7634206426357,0.));
#255348=CARTESIAN_POINT('Ctrl Pts',(22.4836387052232,1.7634206426357,12.));
#255349=CARTESIAN_POINT('Ctrl Pts',(22.4838562517069,1.76343813434565,0.));
#255350=CARTESIAN_POINT('Ctrl Pts',(22.4838562517069,1.76343813434565,12.));
#255351=CARTESIAN_POINT('Ctrl Pts',(22.4844112933129,1.76347698284792,0.));
#255352=CARTESIAN_POINT('Ctrl Pts',(22.4844112933129,1.76347698284792,12.));
#255353=CARTESIAN_POINT('Ctrl Pts',(22.4855446605991,1.76355076045546,0.));
#255354=CARTESIAN_POINT('Ctrl Pts',(22.4855446605991,1.76355076045546,12.));
#255355=CARTESIAN_POINT('Ctrl Pts',(22.4871115206571,1.76364784232963,0.));
#255356=CARTESIAN_POINT('Ctrl Pts',(22.4871115206571,1.76364784232963,12.));
#255357=CARTESIAN_POINT('Ctrl Pts',(22.4890991659478,1.76376424879505,0.));
#255358=CARTESIAN_POINT('Ctrl Pts',(22.4890991659478,1.76376424879505,12.));
#255359=CARTESIAN_POINT('Ctrl Pts',(22.4914909094908,1.76389475965724,0.));
#255360=CARTESIAN_POINT('Ctrl Pts',(22.4914909094908,1.76389475965724,12.));
#255361=CARTESIAN_POINT('Ctrl Pts',(22.4942693792449,1.76403393880301,0.));
#255362=CARTESIAN_POINT('Ctrl Pts',(22.4942693792449,1.76403393880301,12.));
#255363=CARTESIAN_POINT('Ctrl Pts',(22.4974203063191,1.76417731243462,0.));
#255364=CARTESIAN_POINT('Ctrl Pts',(22.4974203063191,1.76417731243462,12.));
#255365=CARTESIAN_POINT('Ctrl Pts',(22.5009332677316,1.76432160068726,0.));
#255366=CARTESIAN_POINT('Ctrl Pts',(22.5009332677316,1.76432160068726,12.));
#255367=CARTESIAN_POINT('Ctrl Pts',(22.5047996391978,1.76446408210366,0.));
#255368=CARTESIAN_POINT('Ctrl Pts',(22.5047996391978,1.76446408210366,12.));
#255369=CARTESIAN_POINT('Ctrl Pts',(22.5090112700212,1.76460218257323,0.));
#255370=CARTESIAN_POINT('Ctrl Pts',(22.5090112700212,1.76460218257323,12.));
#255371=CARTESIAN_POINT('Ctrl Pts',(22.5135590569554,1.76473303281159,0.));
#255372=CARTESIAN_POINT('Ctrl Pts',(22.5135590569554,1.76473303281159,12.));
#255373=CARTESIAN_POINT('Ctrl Pts',(22.5184336670207,1.76485369319896,0.));
#255374=CARTESIAN_POINT('Ctrl Pts',(22.5184336670207,1.76485369319896,12.));
#255375=CARTESIAN_POINT('Ctrl Pts',(22.5236259635515,1.76496128643369,0.));
#255376=CARTESIAN_POINT('Ctrl Pts',(22.5236259635515,1.76496128643369,12.));
#255377=CARTESIAN_POINT('Ctrl Pts',(22.529127665298,1.76505320262752,0.));
#255378=CARTESIAN_POINT('Ctrl Pts',(22.529127665298,1.76505320262752,12.));
#255379=CARTESIAN_POINT('Ctrl Pts',(22.5349313983571,1.7651271156325,0.));
#255380=CARTESIAN_POINT('Ctrl Pts',(22.5349313983571,1.7651271156325,12.));
#255381=CARTESIAN_POINT('Ctrl Pts',(22.5410303590891,1.76518087841493,0.));
#255382=CARTESIAN_POINT('Ctrl Pts',(22.5410303590891,1.76518087841493,12.));
#255383=CARTESIAN_POINT('Ctrl Pts',(22.5474180954006,1.76521245524047,0.));
#255384=CARTESIAN_POINT('Ctrl Pts',(22.5474180954006,1.76521245524047,12.));
#255385=CARTESIAN_POINT('Ctrl Pts',(22.5540882235837,1.76521983384063,0.));
#255386=CARTESIAN_POINT('Ctrl Pts',(22.5540882235837,1.76521983384063,12.));
#255387=CARTESIAN_POINT('Ctrl Pts',(22.5610344912501,1.7652010450045,0.));
#255388=CARTESIAN_POINT('Ctrl Pts',(22.5610344912501,1.7652010450045,12.));
#255389=CARTESIAN_POINT('Ctrl Pts',(22.5682508499873,1.76515418518829,0.));
#255390=CARTESIAN_POINT('Ctrl Pts',(22.5682508499873,1.76515418518829,12.));
#255391=CARTESIAN_POINT('Ctrl Pts',(22.5757315316355,1.76507744026747,0.));
#255392=CARTESIAN_POINT('Ctrl Pts',(22.5757315316355,1.76507744026747,12.));
#255393=CARTESIAN_POINT('Ctrl Pts',(22.5834711038024,1.76496910283089,0.));
#255394=CARTESIAN_POINT('Ctrl Pts',(22.5834711038024,1.76496910283089,12.));
#255395=CARTESIAN_POINT('Ctrl Pts',(22.5914644078106,1.76482755288411,0.));
#255396=CARTESIAN_POINT('Ctrl Pts',(22.5914644078106,1.76482755288411,12.));
#255397=CARTESIAN_POINT('Ctrl Pts',(22.5997065145638,1.76465124413556,0.));
#255398=CARTESIAN_POINT('Ctrl Pts',(22.5997065145638,1.76465124413556,12.));
#255399=CARTESIAN_POINT('Ctrl Pts',(22.6081926681342,1.76443868648015,0.));
#255400=CARTESIAN_POINT('Ctrl Pts',(22.6081926681342,1.76443868648015,12.));
#255401=CARTESIAN_POINT('Ctrl Pts',(22.6169182517693,1.76418843543739,0.));
#255402=CARTESIAN_POINT('Ctrl Pts',(22.6169182517693,1.76418843543739,12.));
#255403=CARTESIAN_POINT('Ctrl Pts',(22.6258787994847,1.76389909571402,0.));
#255404=CARTESIAN_POINT('Ctrl Pts',(22.6258787994847,1.76389909571402,12.));
#255405=CARTESIAN_POINT('Ctrl Pts',(22.635069997936,1.76356932176272,0.));
#255406=CARTESIAN_POINT('Ctrl Pts',(22.635069997936,1.76356932176272,12.));
#255407=CARTESIAN_POINT('Ctrl Pts',(22.6444876940425,1.76319782013914,0.));
#255408=CARTESIAN_POINT('Ctrl Pts',(22.6444876940425,1.76319782013914,12.));
#255409=CARTESIAN_POINT('Ctrl Pts',(22.6541278938413,1.76278334912559,0.));
#255410=CARTESIAN_POINT('Ctrl Pts',(22.6541278938413,1.76278334912559,12.));
#255411=CARTESIAN_POINT('Ctrl Pts',(22.6639867471756,1.76232471392568,0.));
#255412=CARTESIAN_POINT('Ctrl Pts',(22.6639867471756,1.76232471392568,12.));
#255413=CARTESIAN_POINT('Ctrl Pts',(22.6740605356699,1.76182076289525,0.));
#255414=CARTESIAN_POINT('Ctrl Pts',(22.6740605356699,1.76182076289525,12.));
#255415=CARTESIAN_POINT('Ctrl Pts',(22.6843456585245,1.76127038310613,0.));
#255416=CARTESIAN_POINT('Ctrl Pts',(22.6843456585245,1.76127038310613,12.));
#255417=CARTESIAN_POINT('Ctrl Pts',(22.6948386219843,1.76067249704884,0.));
#255418=CARTESIAN_POINT('Ctrl Pts',(22.6948386219843,1.76067249704884,12.));
#255419=CARTESIAN_POINT('Ctrl Pts',(22.7055360375481,1.76002606202399,0.));
#255420=CARTESIAN_POINT('Ctrl Pts',(22.7055360375481,1.76002606202399,12.));
#255421=CARTESIAN_POINT('Ctrl Pts',(22.7164346186007,1.75933006905924,0.));
#255422=CARTESIAN_POINT('Ctrl Pts',(22.7164346186007,1.75933006905924,12.));
#255423=CARTESIAN_POINT('Ctrl Pts',(22.7275311777305,1.75858354204635,0.));
#255424=CARTESIAN_POINT('Ctrl Pts',(22.7275311777305,1.75858354204635,12.));
#255425=CARTESIAN_POINT('Ctrl Pts',(22.7388226235565,1.75778553673249,0.));
#255426=CARTESIAN_POINT('Ctrl Pts',(22.7388226235565,1.75778553673249,12.));
#255427=CARTESIAN_POINT('Ctrl Pts',(22.7503059556455,1.75693513908911,0.));
#255428=CARTESIAN_POINT('Ctrl Pts',(22.7503059556455,1.75693513908911,12.));
#255429=CARTESIAN_POINT('Ctrl Pts',(22.7619782595013,1.75603146371641,0.));
#255430=CARTESIAN_POINT('Ctrl Pts',(22.7619782595013,1.75603146371641,12.));
#255431=CARTESIAN_POINT('Ctrl Pts',(22.7738367016115,1.75507365227127,0.));
#255432=CARTESIAN_POINT('Ctrl Pts',(22.7738367016115,1.75507365227127,12.));
#255433=CARTESIAN_POINT('Ctrl Pts',(22.7858785242358,1.7540608718293,0.));
#255434=CARTESIAN_POINT('Ctrl Pts',(22.7858785242358,1.7540608718293,12.));
#255435=CARTESIAN_POINT('Ctrl Pts',(22.7981010424312,1.75299231391461,0.));
#255436=CARTESIAN_POINT('Ctrl Pts',(22.7981010424312,1.75299231391461,12.));
#255437=CARTESIAN_POINT('Ctrl Pts',(22.8105016414712,1.7518671936559,0.));
#255438=CARTESIAN_POINT('Ctrl Pts',(22.8105016414712,1.7518671936559,12.));
#255439=CARTESIAN_POINT('Ctrl Pts',(22.8230777741285,1.75068474890884,0.));
#255440=CARTESIAN_POINT('Ctrl Pts',(22.8230777741285,1.75068474890884,12.));
#255441=CARTESIAN_POINT('Ctrl Pts',(22.8358269579854,1.74944423940117,0.));
#255442=CARTESIAN_POINT('Ctrl Pts',(22.8358269579854,1.74944423940117,12.));
#255443=CARTESIAN_POINT('Ctrl Pts',(22.8487467728075,1.74814494588492,0.));
#255444=CARTESIAN_POINT('Ctrl Pts',(22.8487467728075,1.74814494588492,12.));
#255445=CARTESIAN_POINT('Ctrl Pts',(22.8618348580234,1.74678616930663,0.));
#255446=CARTESIAN_POINT('Ctrl Pts',(22.8618348580234,1.74678616930663,12.));
#255447=CARTESIAN_POINT('Ctrl Pts',(22.8750889101696,1.745367229982,0.));
#255448=CARTESIAN_POINT('Ctrl Pts',(22.8750889101696,1.745367229982,12.));
#255449=CARTESIAN_POINT('Ctrl Pts',(22.8885066803351,1.74388746677702,0.));
#255450=CARTESIAN_POINT('Ctrl Pts',(22.8885066803351,1.74388746677702,12.));
#255451=CARTESIAN_POINT('Ctrl Pts',(22.9020859716144,1.74234623630079,0.));
#255452=CARTESIAN_POINT('Ctrl Pts',(22.9020859716144,1.74234623630079,12.));
#255453=CARTESIAN_POINT('Ctrl Pts',(22.9158246373365,1.74074291231057,0.));
#255454=CARTESIAN_POINT('Ctrl Pts',(22.9158246373365,1.74074291231057,12.));
#255455=CARTESIAN_POINT('Ctrl Pts',(22.9297205792587,1.73907688511665,0.));
#255456=CARTESIAN_POINT('Ctrl Pts',(22.9297205792587,1.73907688511665,12.));
#255457=CARTESIAN_POINT('Ctrl Pts',(22.9437717457825,1.73734756100038,0.));
#255458=CARTESIAN_POINT('Ctrl Pts',(22.9437717457825,1.73734756100038,12.));
#255459=CARTESIAN_POINT('Ctrl Pts',(22.9579761301062,1.73555436162771,0.));
#255460=CARTESIAN_POINT('Ctrl Pts',(22.9579761301062,1.73555436162771,12.));
#255461=CARTESIAN_POINT('Ctrl Pts',(22.9723317685688,1.73369672350818,0.));
#255462=CARTESIAN_POINT('Ctrl Pts',(22.9723317685688,1.73369672350818,12.));
#255463=CARTESIAN_POINT('Ctrl Pts',(22.9868367391978,1.73177409750194,0.));
#255464=CARTESIAN_POINT('Ctrl Pts',(22.9868367391978,1.73177409750194,12.));
#255465=CARTESIAN_POINT('Ctrl Pts',(23.0014891601891,1.72978594832137,0.));
#255466=CARTESIAN_POINT('Ctrl Pts',(23.0014891601891,1.72978594832137,12.));
#255467=CARTESIAN_POINT('Ctrl Pts',(23.0162871884167,1.72773175404703,0.));
#255468=CARTESIAN_POINT('Ctrl Pts',(23.0162871884167,1.72773175404703,12.));
#255469=CARTESIAN_POINT('Ctrl Pts',(23.031229017888,1.72561100564033,0.));
#255470=CARTESIAN_POINT('Ctrl Pts',(23.031229017888,1.72561100564033,12.));
#255471=CARTESIAN_POINT('Ctrl Pts',(23.0463128785528,1.72342320653731,0.));
#255472=CARTESIAN_POINT('Ctrl Pts',(23.0463128785528,1.72342320653731,12.));
#255473=CARTESIAN_POINT('Ctrl Pts',(23.0615370351559,1.72116787225981,0.));
#255474=CARTESIAN_POINT('Ctrl Pts',(23.0615370351559,1.72116787225981,12.));
#255475=CARTESIAN_POINT('Ctrl Pts',(23.0768997860709,1.71884453003027,0.));
#255476=CARTESIAN_POINT('Ctrl Pts',(23.0768997860709,1.71884453003027,12.));
#255477=CARTESIAN_POINT('Ctrl Pts',(23.0923994621216,1.71645271839311,0.));
#255478=CARTESIAN_POINT('Ctrl Pts',(23.0923994621216,1.71645271839311,12.));
#255479=CARTESIAN_POINT('Ctrl Pts',(23.1080344254291,1.71399198684725,0.));
#255480=CARTESIAN_POINT('Ctrl Pts',(23.1080344254291,1.71399198684725,12.));
#255481=CARTESIAN_POINT('Ctrl Pts',(23.1238030684929,1.71146189552192,0.));
#255482=CARTESIAN_POINT('Ctrl Pts',(23.1238030684929,1.71146189552192,12.));
#255483=CARTESIAN_POINT('Ctrl Pts',(23.1397038132358,1.7088620148546,0.));
#255484=CARTESIAN_POINT('Ctrl Pts',(23.1397038132358,1.7088620148546,12.));
#255485=CARTESIAN_POINT('Ctrl Pts',(23.1557351100613,1.70619192527847,0.));
#255486=CARTESIAN_POINT('Ctrl Pts',(23.1557351100613,1.70619192527847,12.));
#255487=CARTESIAN_POINT('Ctrl Pts',(23.1718954368749,1.70345121691259,0.));
#255488=CARTESIAN_POINT('Ctrl Pts',(23.1718954368749,1.70345121691259,12.));
#255489=CARTESIAN_POINT('Ctrl Pts',(23.1881832981848,1.70063948926988,0.));
#255490=CARTESIAN_POINT('Ctrl Pts',(23.1881832981848,1.70063948926988,12.));
#255491=CARTESIAN_POINT('Ctrl Pts',(23.2045972243765,1.69775635099425,0.));
#255492=CARTESIAN_POINT('Ctrl Pts',(23.2045972243765,1.69775635099425,12.));
#255493=CARTESIAN_POINT('Ctrl Pts',(23.2211357709374,1.69480141959946,0.));
#255494=CARTESIAN_POINT('Ctrl Pts',(23.2211357709374,1.69480141959946,12.));
#255495=CARTESIAN_POINT('Ctrl Pts',(23.2377975177014,1.69177432121716,0.));
#255496=CARTESIAN_POINT('Ctrl Pts',(23.2377975177014,1.69177432121716,12.));
#255497=CARTESIAN_POINT('Ctrl Pts',(23.2545810680536,1.6886746903491,0.));
#255498=CARTESIAN_POINT('Ctrl Pts',(23.2545810680536,1.6886746903491,12.));
#255499=CARTESIAN_POINT('Ctrl Pts',(23.2714850482245,1.68550216963275,0.));
#255500=CARTESIAN_POINT('Ctrl Pts',(23.2714850482245,1.68550216963275,12.));
#255501=CARTESIAN_POINT('Ctrl Pts',(23.2885081066949,1.68225640962181,0.));
#255502=CARTESIAN_POINT('Ctrl Pts',(23.2885081066949,1.68225640962181,12.));
#255503=CARTESIAN_POINT('Ctrl Pts',(23.3056489135611,1.67893706857123,0.));
#255504=CARTESIAN_POINT('Ctrl Pts',(23.3056489135611,1.67893706857123,12.));
#255505=CARTESIAN_POINT('Ctrl Pts',(23.3229061599145,1.67554381222988,0.));
#255506=CARTESIAN_POINT('Ctrl Pts',(23.3229061599145,1.67554381222988,12.));
#255507=CARTESIAN_POINT('Ctrl Pts',(23.3402785571866,1.67207631363905,0.));
#255508=CARTESIAN_POINT('Ctrl Pts',(23.3402785571866,1.67207631363905,12.));
#255509=CARTESIAN_POINT('Ctrl Pts',(23.3577648365747,1.66853425293978,0.));
#255510=CARTESIAN_POINT('Ctrl Pts',(23.3577648365747,1.66853425293978,12.));
#255511=CARTESIAN_POINT('Ctrl Pts',(23.375363748555,1.66491731718864,0.));
#255512=CARTESIAN_POINT('Ctrl Pts',(23.375363748555,1.66491731718864,12.));
#255513=CARTESIAN_POINT('Ctrl Pts',(23.3930740623622,1.66122520018008,0.));
#255514=CARTESIAN_POINT('Ctrl Pts',(23.3930740623622,1.66122520018008,12.));
#255515=CARTESIAN_POINT('Ctrl Pts',(23.4108945654803,1.65745760227507,0.));
#255516=CARTESIAN_POINT('Ctrl Pts',(23.4108945654803,1.65745760227507,12.));
#255517=CARTESIAN_POINT('Ctrl Pts',(23.4288240631034,1.6536142302373,0.));
#255518=CARTESIAN_POINT('Ctrl Pts',(23.4288240631034,1.6536142302373,12.));
#255519=CARTESIAN_POINT('Ctrl Pts',(23.446861377656,1.6496947970734,0.));
#255520=CARTESIAN_POINT('Ctrl Pts',(23.446861377656,1.6496947970734,12.));
#255521=CARTESIAN_POINT('Ctrl Pts',(23.4650053483919,1.64569902187608,0.));
#255522=CARTESIAN_POINT('Ctrl Pts',(23.4650053483919,1.64569902187608,12.));
#255523=CARTESIAN_POINT('Ctrl Pts',(23.4832548309638,1.64162662967525,0.));
#255524=CARTESIAN_POINT('Ctrl Pts',(23.4832548309638,1.64162662967525,12.));
#255525=CARTESIAN_POINT('Ctrl Pts',(23.5016086970006,1.63747735129474,0.));
#255526=CARTESIAN_POINT('Ctrl Pts',(23.5016086970006,1.63747735129474,12.));
#255527=CARTESIAN_POINT('Ctrl Pts',(23.5200658336624,1.63325092321731,0.));
#255528=CARTESIAN_POINT('Ctrl Pts',(23.5200658336624,1.63325092321731,12.));
#255529=CARTESIAN_POINT('Ctrl Pts',(23.5386251432278,1.62894708745231,0.));
#255530=CARTESIAN_POINT('Ctrl Pts',(23.5386251432278,1.62894708745231,12.));
#255531=CARTESIAN_POINT('Ctrl Pts',(23.5572855427617,1.62456559140072,0.));
#255532=CARTESIAN_POINT('Ctrl Pts',(23.5572855427617,1.62456559140072,12.));
#255533=CARTESIAN_POINT('Ctrl Pts',(23.5760459637608,1.62010618772869,0.));
#255534=CARTESIAN_POINT('Ctrl Pts',(23.5760459637608,1.62010618772869,12.));
#255535=CARTESIAN_POINT('Ctrl Pts',(23.5949053517996,1.61556863424697,0.));
#255536=CARTESIAN_POINT('Ctrl Pts',(23.5949053517996,1.61556863424697,12.));
#255537=CARTESIAN_POINT('Ctrl Pts',(23.6138626661644,1.61095269379773,0.));
#255538=CARTESIAN_POINT('Ctrl Pts',(23.6138626661644,1.61095269379773,12.));
#255539=CARTESIAN_POINT('Ctrl Pts',(23.6329168794916,1.60625813414666,0.));
#255540=CARTESIAN_POINT('Ctrl Pts',(23.6329168794916,1.60625813414666,12.));
#255541=CARTESIAN_POINT('Ctrl Pts',(23.6520669774863,1.60148472786588,0.));
#255542=CARTESIAN_POINT('Ctrl Pts',(23.6520669774863,1.60148472786588,12.));
#255543=CARTESIAN_POINT('Ctrl Pts',(23.6713119586302,1.59663225222459,0.));
#255544=CARTESIAN_POINT('Ctrl Pts',(23.6713119586302,1.59663225222459,12.));
#255545=CARTESIAN_POINT('Ctrl Pts',(23.6906508338832,1.59170048908631,0.));
#255546=CARTESIAN_POINT('Ctrl Pts',(23.6906508338832,1.59170048908631,12.));
#255547=CARTESIAN_POINT('Ctrl Pts',(23.7100826263835,1.58668922481222,0.));
#255548=CARTESIAN_POINT('Ctrl Pts',(23.7100826263835,1.58668922481222,12.));
#255549=CARTESIAN_POINT('Ctrl Pts',(23.7296063711308,1.58159825017362,0.));
#255550=CARTESIAN_POINT('Ctrl Pts',(23.7296063711308,1.58159825017362,12.));
#255551=CARTESIAN_POINT('Ctrl Pts',(23.7492211147369,1.57642736025251,0.));
#255552=CARTESIAN_POINT('Ctrl Pts',(23.7492211147369,1.57642736025251,12.));
#255553=CARTESIAN_POINT('Ctrl Pts',(23.7689259151869,1.57117635434412,0.));
#255554=CARTESIAN_POINT('Ctrl Pts',(23.7689259151869,1.57117635434412,12.));
#255555=CARTESIAN_POINT('Ctrl Pts',(23.788719841588,1.56584503586844,0.));
#255556=CARTESIAN_POINT('Ctrl Pts',(23.788719841588,1.56584503586844,12.));
#255557=CARTESIAN_POINT('Ctrl Pts',(23.8086019739192,1.56043321228631,0.));
#255558=CARTESIAN_POINT('Ctrl Pts',(23.8086019739192,1.56043321228631,12.));
#255559=CARTESIAN_POINT('Ctrl Pts',(23.8285714027631,1.55494069502628,0.));
#255560=CARTESIAN_POINT('Ctrl Pts',(23.8285714027631,1.55494069502628,12.));
#255561=CARTESIAN_POINT('Ctrl Pts',(23.8486272290698,1.5493672994053,0.));
#255562=CARTESIAN_POINT('Ctrl Pts',(23.8486272290698,1.5493672994053,12.));
#255563=CARTESIAN_POINT('Ctrl Pts',(23.8687685639635,1.54371284453978,0.));
#255564=CARTESIAN_POINT('Ctrl Pts',(23.8687685639635,1.54371284453978,12.));
#255565=CARTESIAN_POINT('Ctrl Pts',(23.8889945285313,1.53797715326748,0.));
#255566=CARTESIAN_POINT('Ctrl Pts',(23.8889945285313,1.53797715326748,12.));
#255567=CARTESIAN_POINT('Ctrl Pts',(23.9093042536119,1.53216005207462,0.));
#255568=CARTESIAN_POINT('Ctrl Pts',(23.9093042536119,1.53216005207462,12.));
#255569=CARTESIAN_POINT('Ctrl Pts',(23.9296968795761,1.5262613710304,0.));
#255570=CARTESIAN_POINT('Ctrl Pts',(23.9296968795761,1.5262613710304,12.));
#255571=CARTESIAN_POINT('Ctrl Pts',(23.9501715561038,1.52028094372806,0.));
#255572=CARTESIAN_POINT('Ctrl Pts',(23.9501715561038,1.52028094372806,12.));
#255573=CARTESIAN_POINT('Ctrl Pts',(23.9707274420145,1.51421860720628,0.));
#255574=CARTESIAN_POINT('Ctrl Pts',(23.9707274420145,1.51421860720628,12.));
#255575=CARTESIAN_POINT('Ctrl Pts',(23.991363705093,1.50807420187703,0.));
#255576=CARTESIAN_POINT('Ctrl Pts',(23.991363705093,1.50807420187703,12.));
#255577=CARTESIAN_POINT('Ctrl Pts',(24.0120795219086,1.50184757146099,0.));
#255578=CARTESIAN_POINT('Ctrl Pts',(24.0120795219086,1.50184757146099,12.));
#255579=CARTESIAN_POINT('Ctrl Pts',(24.0328740776331,1.49553856292798,0.));
#255580=CARTESIAN_POINT('Ctrl Pts',(24.0328740776331,1.49553856292798,12.));
#255581=CARTESIAN_POINT('Ctrl Pts',(24.053746565843,1.48914702644883,0.));
#255582=CARTESIAN_POINT('Ctrl Pts',(24.053746565843,1.48914702644883,12.));
#255583=CARTESIAN_POINT('Ctrl Pts',(24.074696188353,1.4826728153368,0.));
#255584=CARTESIAN_POINT('Ctrl Pts',(24.074696188353,1.4826728153368,12.));
#255585=CARTESIAN_POINT('Ctrl Pts',(24.0957221550782,1.47611578597742,0.));
#255586=CARTESIAN_POINT('Ctrl Pts',(24.0957221550782,1.47611578597742,12.));
#255587=CARTESIAN_POINT('Ctrl Pts',(24.1168236838827,1.46947579776992,0.));
#255588=CARTESIAN_POINT('Ctrl Pts',(24.1168236838827,1.46947579776992,12.));
#255589=CARTESIAN_POINT('Ctrl Pts',(24.1380000004272,1.46275271307398,0.));
#255590=CARTESIAN_POINT('Ctrl Pts',(24.1380000004272,1.46275271307398,12.));
#255591=CARTESIAN_POINT('Ctrl Pts',(24.1592503380105,1.45594639716314,0.));
#255592=CARTESIAN_POINT('Ctrl Pts',(24.1592503380105,1.45594639716314,12.));
#255593=CARTESIAN_POINT('Ctrl Pts',(24.1805739374033,1.44905671818721,0.));
#255594=CARTESIAN_POINT('Ctrl Pts',(24.1805739374033,1.44905671818721,12.));
#255595=CARTESIAN_POINT('Ctrl Pts',(24.2019700467214,1.44208354711074,0.));
#255596=CARTESIAN_POINT('Ctrl Pts',(24.2019700467214,1.44208354711074,12.));
#255597=CARTESIAN_POINT('Ctrl Pts',(24.2234379212978,1.43502675765502,0.));
#255598=CARTESIAN_POINT('Ctrl Pts',(24.2234379212978,1.43502675765502,12.));
#255599=CARTESIAN_POINT('Ctrl Pts',(24.2449768235485,1.42788622624851,0.));
#255600=CARTESIAN_POINT('Ctrl Pts',(24.2449768235485,1.42788622624851,12.));
#255601=CARTESIAN_POINT('Ctrl Pts',(24.2665860228357,1.42066183198252,0.));
#255602=CARTESIAN_POINT('Ctrl Pts',(24.2665860228357,1.42066183198252,12.));
#255603=CARTESIAN_POINT('Ctrl Pts',(24.2882647953214,1.41335345657685,0.));
#255604=CARTESIAN_POINT('Ctrl Pts',(24.2882647953214,1.41335345657685,12.));
#255605=CARTESIAN_POINT('Ctrl Pts',(24.3100124238316,1.40596098434341,0.));
#255606=CARTESIAN_POINT('Ctrl Pts',(24.3100124238316,1.40596098434341,12.));
#255607=CARTESIAN_POINT('Ctrl Pts',(24.3318281977647,1.3984843021281,0.));
#255608=CARTESIAN_POINT('Ctrl Pts',(24.3318281977647,1.3984843021281,12.));
#255609=CARTESIAN_POINT('Ctrl Pts',(24.3537114129877,1.3909232992639,0.));
#255610=CARTESIAN_POINT('Ctrl Pts',(24.3537114129877,1.3909232992639,12.));
#255611=CARTESIAN_POINT('Ctrl Pts',(24.37566137173,1.38327786752998,0.));
#255612=CARTESIAN_POINT('Ctrl Pts',(24.37566137173,1.38327786752998,12.));
#255613=CARTESIAN_POINT('Ctrl Pts',(24.3976773824731,1.37554790111608,0.));
#255614=CARTESIAN_POINT('Ctrl Pts',(24.3976773824731,1.37554790111608,12.));
#255615=CARTESIAN_POINT('Ctrl Pts',(24.4197587598337,1.36773329659954,0.));
#255616=CARTESIAN_POINT('Ctrl Pts',(24.4197587598337,1.36773329659954,12.));
#255617=CARTESIAN_POINT('Ctrl Pts',(24.4419048244524,1.35983395290624,0.));
#255618=CARTESIAN_POINT('Ctrl Pts',(24.4419048244524,1.35983395290624,12.));
#255619=CARTESIAN_POINT('Ctrl Pts',(24.4641149028894,1.35184977125645,0.));
#255620=CARTESIAN_POINT('Ctrl Pts',(24.4641149028894,1.35184977125645,12.));
#255621=CARTESIAN_POINT('Ctrl Pts',(24.4863883275135,1.34378065512335,0.));
#255622=CARTESIAN_POINT('Ctrl Pts',(24.4863883275135,1.34378065512335,12.));
#255623=CARTESIAN_POINT('Ctrl Pts',(24.5087244363856,1.33562651019684,0.));
#255624=CARTESIAN_POINT('Ctrl Pts',(24.5087244363856,1.33562651019684,12.));
#255625=CARTESIAN_POINT('Ctrl Pts',(24.5311225731434,1.32738724435326,0.));
#255626=CARTESIAN_POINT('Ctrl Pts',(24.5311225731434,1.32738724435326,12.));
#255627=CARTESIAN_POINT('Ctrl Pts',(24.5535820868671,1.31906276763669,0.));
#255628=CARTESIAN_POINT('Ctrl Pts',(24.5535820868671,1.31906276763669,12.));
#255629=CARTESIAN_POINT('Ctrl Pts',(24.576102332018,1.31065299222023,0.));
#255630=CARTESIAN_POINT('Ctrl Pts',(24.576102332018,1.31065299222023,12.));
#255631=CARTESIAN_POINT('Ctrl Pts',(24.5986826684025,1.30215783236364,0.));
#255632=CARTESIAN_POINT('Ctrl Pts',(24.5986826684025,1.30215783236364,12.));
#255633=CARTESIAN_POINT('Ctrl Pts',(24.6213224611228,1.29357720438108,0.));
#255634=CARTESIAN_POINT('Ctrl Pts',(24.6213224611228,1.29357720438108,12.));
#255635=CARTESIAN_POINT('Ctrl Pts',(24.6440210805278,1.28491102661514,0.));
#255636=CARTESIAN_POINT('Ctrl Pts',(24.6440210805278,1.28491102661514,12.));
#255637=CARTESIAN_POINT('Ctrl Pts',(24.666777902156,1.2761592194164,0.));
#255638=CARTESIAN_POINT('Ctrl Pts',(24.666777902156,1.2761592194164,12.));
#255639=CARTESIAN_POINT('Ctrl Pts',(24.6895923066837,1.26732170513497,0.));
#255640=CARTESIAN_POINT('Ctrl Pts',(24.6895923066837,1.26732170513497,12.));
#255641=CARTESIAN_POINT('Ctrl Pts',(24.7124636797895,1.25839840807415,0.));
#255642=CARTESIAN_POINT('Ctrl Pts',(24.7124636797895,1.25839840807415,12.));
#255643=CARTESIAN_POINT('Ctrl Pts',(24.7353914120012,1.24938925444324,0.));
#255644=CARTESIAN_POINT('Ctrl Pts',(24.7353914120012,1.24938925444324,12.));
#255645=CARTESIAN_POINT('Ctrl Pts',(24.7583748985439,1.24029417231988,0.));
#255646=CARTESIAN_POINT('Ctrl Pts',(24.7583748985439,1.24029417231988,12.));
#255647=CARTESIAN_POINT('Ctrl Pts',(24.78141353918,1.23111309161843,0.));
#255648=CARTESIAN_POINT('Ctrl Pts',(24.78141353918,1.23111309161843,12.));
#255649=CARTESIAN_POINT('Ctrl Pts',(24.8045067380536,1.22184594406527,0.));
#255650=CARTESIAN_POINT('Ctrl Pts',(24.8045067380536,1.22184594406527,12.));
#255651=CARTESIAN_POINT('Ctrl Pts',(24.8276539035092,1.21249266318205,0.));
#255652=CARTESIAN_POINT('Ctrl Pts',(24.8276539035092,1.21249266318205,12.));
#255653=CARTESIAN_POINT('Ctrl Pts',(24.8508544481973,1.20305318426016,0.));
#255654=CARTESIAN_POINT('Ctrl Pts',(24.8508544481973,1.20305318426016,12.));
#255655=CARTESIAN_POINT('Ctrl Pts',(24.8741077892074,1.19352744434059,0.));
#255656=CARTESIAN_POINT('Ctrl Pts',(24.8741077892074,1.19352744434059,12.));
#255657=CARTESIAN_POINT('Ctrl Pts',(24.8974133481829,1.18391538220098,0.));
#255658=CARTESIAN_POINT('Ctrl Pts',(24.8974133481829,1.18391538220098,12.));
#255659=CARTESIAN_POINT('Ctrl Pts',(24.9207705514449,1.1742169383504,0.));
#255660=CARTESIAN_POINT('Ctrl Pts',(24.9207705514449,1.1742169383504,12.));
#255661=CARTESIAN_POINT('Ctrl Pts',(24.9441788300932,1.16443205502852,0.));
#255662=CARTESIAN_POINT('Ctrl Pts',(24.9441788300932,1.16443205502852,12.));
#255663=CARTESIAN_POINT('Ctrl Pts',(24.9676376201501,1.15456067621894,0.));
#255664=CARTESIAN_POINT('Ctrl Pts',(24.9676376201501,1.15456067621894,12.));
#255665=CARTESIAN_POINT('Ctrl Pts',(24.9911463621431,1.14460274758206,0.));
#255666=CARTESIAN_POINT('Ctrl Pts',(24.9911463621431,1.14460274758206,12.));
#255667=CARTESIAN_POINT('Ctrl Pts',(25.0147045006193,1.13455821638536,0.));
#255668=CARTESIAN_POINT('Ctrl Pts',(25.0147045006193,1.13455821638536,12.));
#255669=CARTESIAN_POINT('Ctrl Pts',(25.0383114836898,1.12442703144455,0.));
#255670=CARTESIAN_POINT('Ctrl Pts',(25.0383114836898,1.12442703144455,12.));
#255671=CARTESIAN_POINT('Ctrl Pts',(25.0619667625336,1.1142091430689,0.));
#255672=CARTESIAN_POINT('Ctrl Pts',(25.0619667625336,1.1142091430689,12.));
#255673=CARTESIAN_POINT('Ctrl Pts',(25.085669790968,1.10390450301741,0.));
#255674=CARTESIAN_POINT('Ctrl Pts',(25.085669790968,1.10390450301741,12.));
#255675=CARTESIAN_POINT('Ctrl Pts',(25.1094200248448,1.09351306445299,0.));
#255676=CARTESIAN_POINT('Ctrl Pts',(25.1094200248448,1.09351306445299,12.));
#255677=CARTESIAN_POINT('Ctrl Pts',(25.1332169227415,1.08303478197174,0.));
#255678=CARTESIAN_POINT('Ctrl Pts',(25.1332169227415,1.08303478197174,12.));
#255679=CARTESIAN_POINT('Ctrl Pts',(25.1570599469311,1.0724696116546,0.));
#255680=CARTESIAN_POINT('Ctrl Pts',(25.1570599469311,1.0724696116546,12.));
#255681=CARTESIAN_POINT('Ctrl Pts',(25.1809485642191,1.06181751111754,0.));
#255682=CARTESIAN_POINT('Ctrl Pts',(25.1809485642191,1.06181751111754,12.));
#255683=CARTESIAN_POINT('Ctrl Pts',(25.2048822469027,1.05107843957926,0.));
#255684=CARTESIAN_POINT('Ctrl Pts',(25.2048822469027,1.05107843957926,12.));
#255685=CARTESIAN_POINT('Ctrl Pts',(25.2288604735087,1.04025235791515,0.));
#255686=CARTESIAN_POINT('Ctrl Pts',(25.2288604735087,1.04025235791515,12.));
#255687=CARTESIAN_POINT('Ctrl Pts',(25.2528827300427,1.0293392287683,0.));
#255688=CARTESIAN_POINT('Ctrl Pts',(25.2528827300427,1.0293392287683,12.));
#255689=CARTESIAN_POINT('Ctrl Pts',(25.2769485087268,1.01833901642273,0.));
#255690=CARTESIAN_POINT('Ctrl Pts',(25.2769485087268,1.01833901642273,12.));
#255691=CARTESIAN_POINT('Ctrl Pts',(25.3010573055557,1.00725168656934,0.));
#255692=CARTESIAN_POINT('Ctrl Pts',(25.3010573055557,1.00725168656934,12.));
#255693=CARTESIAN_POINT('Ctrl Pts',(25.3252086182976,0.996077206120921,
0.));
#255694=CARTESIAN_POINT('Ctrl Pts',(25.3252086182976,0.996077206120921,
12.));
#255695=CARTESIAN_POINT('Ctrl Pts',(25.3494019441444,0.984815543004091,
0.));
#255696=CARTESIAN_POINT('Ctrl Pts',(25.3494019441444,0.984815543004091,
12.));
#255697=CARTESIAN_POINT('Ctrl Pts',(25.3736367778842,0.97346666600005,0.));
#255698=CARTESIAN_POINT('Ctrl Pts',(25.3736367778842,0.97346666600005,12.));
#255699=CARTESIAN_POINT('Ctrl Pts',(25.3979126089155,0.962030544502806,
0.));
#255700=CARTESIAN_POINT('Ctrl Pts',(25.3979126089155,0.962030544502806,
12.));
#255701=CARTESIAN_POINT('Ctrl Pts',(25.4222289223155,0.950507148596971,
0.));
#255702=CARTESIAN_POINT('Ctrl Pts',(25.4222289223155,0.950507148596971,
12.));
#255703=CARTESIAN_POINT('Ctrl Pts',(25.4465852044835,0.938896449495636,
0.));
#255704=CARTESIAN_POINT('Ctrl Pts',(25.4465852044835,0.938896449495636,
12.));
#255705=CARTESIAN_POINT('Ctrl Pts',(25.4709809474996,0.927198419885607,
0.));
#255706=CARTESIAN_POINT('Ctrl Pts',(25.4709809474996,0.927198419885607,
12.));
#255707=CARTESIAN_POINT('Ctrl Pts',(25.4954156541787,0.915413034335334,
0.));
#255708=CARTESIAN_POINT('Ctrl Pts',(25.4954156541787,0.915413034335334,
12.));
#255709=CARTESIAN_POINT('Ctrl Pts',(25.5198888424195,0.903540269651155,
0.));
#255710=CARTESIAN_POINT('Ctrl Pts',(25.5198888424195,0.903540269651155,
12.));
#255711=CARTESIAN_POINT('Ctrl Pts',(25.5444000508223,0.891580105349469,
0.));
#255712=CARTESIAN_POINT('Ctrl Pts',(25.5444000508223,0.891580105349469,
12.));
#255713=CARTESIAN_POINT('Ctrl Pts',(25.568948840818,0.879532523835094,0.));
#255714=CARTESIAN_POINT('Ctrl Pts',(25.568948840818,0.879532523835094,12.));
#255715=CARTESIAN_POINT('Ctrl Pts',(25.5935347843616,0.867397509339473,
0.));
#255716=CARTESIAN_POINT('Ctrl Pts',(25.5935347843616,0.867397509339473,
12.));
#255717=CARTESIAN_POINT('Ctrl Pts',(25.618157453608,0.855175047037618,0.));
#255718=CARTESIAN_POINT('Ctrl Pts',(25.618157453608,0.855175047037618,12.));
#255719=CARTESIAN_POINT('Ctrl Pts',(25.6428164100078,0.842865122121547,
0.));
#255720=CARTESIAN_POINT('Ctrl Pts',(25.6428164100078,0.842865122121547,
12.));
#255721=CARTESIAN_POINT('Ctrl Pts',(25.6675111931957,0.83046771886437,0.));
#255722=CARTESIAN_POINT('Ctrl Pts',(25.6675111931957,0.83046771886437,12.));
#255723=CARTESIAN_POINT('Ctrl Pts',(25.6922413110172,0.817982819786722,
0.));
#255724=CARTESIAN_POINT('Ctrl Pts',(25.6922413110172,0.817982819786722,
12.));
#255725=CARTESIAN_POINT('Ctrl Pts',(25.7170062262474,0.805410404552597,
0.));
#255726=CARTESIAN_POINT('Ctrl Pts',(25.7170062262474,0.805410404552597,
12.));
#255727=CARTESIAN_POINT('Ctrl Pts',(25.7418053757671,0.792750451613538,
0.));
#255728=CARTESIAN_POINT('Ctrl Pts',(25.7418053757671,0.792750451613538,
12.));
#255729=CARTESIAN_POINT('Ctrl Pts',(25.7666381946871,0.780002940289028,
0.));
#255730=CARTESIAN_POINT('Ctrl Pts',(25.7666381946871,0.780002940289028,
12.));
#255731=CARTESIAN_POINT('Ctrl Pts',(25.7915041383304,0.767167852648643,
0.));
#255732=CARTESIAN_POINT('Ctrl Pts',(25.7915041383304,0.767167852648643,
12.));
#255733=CARTESIAN_POINT('Ctrl Pts',(25.816402705995,0.754245175608291,0.));
#255734=CARTESIAN_POINT('Ctrl Pts',(25.816402705995,0.754245175608291,12.));
#255735=CARTESIAN_POINT('Ctrl Pts',(25.841333461908,0.741234902664698,0.));
#255736=CARTESIAN_POINT('Ctrl Pts',(25.841333461908,0.741234902664698,12.));
#255737=CARTESIAN_POINT('Ctrl Pts',(25.8662960624285,0.728137036485881,
0.));
#255738=CARTESIAN_POINT('Ctrl Pts',(25.8662960624285,0.728137036485881,
12.));
#255739=CARTESIAN_POINT('Ctrl Pts',(25.8912902615141,0.714951588533756,
0.));
#255740=CARTESIAN_POINT('Ctrl Pts',(25.8912902615141,0.714951588533756,
12.));
#255741=CARTESIAN_POINT('Ctrl Pts',(25.9163158909645,0.701678575236605,
0.));
#255742=CARTESIAN_POINT('Ctrl Pts',(25.9163158909645,0.701678575236605,
12.));
#255743=CARTESIAN_POINT('Ctrl Pts',(25.941372847213,0.68831801506568,0.));
#255744=CARTESIAN_POINT('Ctrl Pts',(25.941372847213,0.68831801506568,12.));
#255745=CARTESIAN_POINT('Ctrl Pts',(25.9614434298092,0.677559543215907,
0.));
#255746=CARTESIAN_POINT('Ctrl Pts',(25.9614434298092,0.677559543215907,
12.));
#255747=CARTESIAN_POINT('Ctrl Pts',(25.9765104298171,0.669451306784419,
0.));
#255748=CARTESIAN_POINT('Ctrl Pts',(25.9765104298171,0.669451306784419,
12.));
#255749=CARTESIAN_POINT('Ctrl Pts',(25.9865613464809,0.664028313188916,
0.));
#255750=CARTESIAN_POINT('Ctrl Pts',(25.9865613464809,0.664028313188916,
12.));
#255751=CARTESIAN_POINT('Ctrl Pts',(25.991588367311,0.661312440730894,0.));
#255752=CARTESIAN_POINT('Ctrl Pts',(25.991588367311,0.661312440730894,12.));
#255753=CARTESIAN_POINT('',(25.991588367311,0.661312440730894,0.));
#255754=CARTESIAN_POINT('Origin',(0.,0.,0.));
#255755=CARTESIAN_POINT('',(-7.,-8.57252759403147E-16,0.));
#255756=CARTESIAN_POINT('Origin',(0.,0.,0.));
#259188=UNCERTAINTY_MEASURE_WITH_UNIT(LENGTH_MEASURE(0.01),#259225,
'DISTANCE_ACCURACY_VALUE',
'Maximum model space distance between geometric entities at asserted c
onnectivities');
#259202=UNCERTAINTY_MEASURE_WITH_UNIT(LENGTH_MEASURE(0.01),#259225,
'DISTANCE_ACCURACY_VALUE',
'Maximum model space distance between geometric entities at asserted c
onnectivities');
#259210=(
GEOMETRIC_REPRESENTATION_CONTEXT(3)
GLOBAL_UNCERTAINTY_ASSIGNED_CONTEXT((#259188))
GLOBAL_UNIT_ASSIGNED_CONTEXT((#259225,#259227,#259228))
REPRESENTATION_CONTEXT('','3D')
);
#259224=(
GEOMETRIC_REPRESENTATION_CONTEXT(3)
GLOBAL_UNCERTAINTY_ASSIGNED_CONTEXT((#259202))
GLOBAL_UNIT_ASSIGNED_CONTEXT((#259225,#259227,#259228))
REPRESENTATION_CONTEXT('','3D')
);
#259225=(
LENGTH_UNIT()
NAMED_UNIT(*)
SI_UNIT(.MILLI.,.METRE.)
);
#259227=(
NAMED_UNIT(*)
PLANE_ANGLE_UNIT()
SI_UNIT($,.RADIAN.)
);
#259228=(
NAMED_UNIT(*)
SI_UNIT($,.STERADIAN.)
SOLID_ANGLE_UNIT()
);
#259236=SHAPE_DEFINITION_REPRESENTATION(#259257,#259376);
#259257=PRODUCT_DEFINITION_SHAPE('',$,#259398);
#259376=SHAPE_REPRESENTATION('',(#26659),#259210);
#259390=PRODUCT_DEFINITION_CONTEXT('part definition',#259455,'design');
#259398=PRODUCT_DEFINITION('Planet gear','Planet gear',#259419,#259390);
#259419=PRODUCT_DEFINITION_FORMATION('',$,#259464);
#259455=APPLICATION_CONTEXT(
'Core Data for Automotive Mechanical Design Process');
#259456=PRODUCT_CONTEXT('part definition',#259455,'mechanical');
#259464=PRODUCT('Planet gear','Planet gear',
'{"standard_geometry": "Unshifted20degree involute", "teeth": 24, "mod
ule_mm": 2, "pitch_diameter_mm": 48.0, "root_diameter_mm": 43.0, "tip_
diameter_mm": 52.0, "face_mm": 12, "per_gear_circular_tooth_thinning_m
m": 0.1, "derived_root_fillet_mm": 0.5, "involute_fit_points_per_flank
": 41, "internal": false, "source_stock": "Native reusable Gear blank;
 assembly-specific machining", "manufacturing_scope": "Standard profil
e reference; grade, cutter/root transition validation, tolerances, bac
klash and load rating require production selection."}',(#259456));
#259484=PRESENTATION_STYLE_ASSIGNMENT((#259499));
#259499=SURFACE_STYLE_USAGE(.BOTH.,#259514);
#259514=SURFACE_SIDE_STYLE('',(#259529));
#259529=SURFACE_STYLE_FILL_AREA(#259544);
#259544=FILL_AREA_STYLE('Gear light blue',(#259559));
#259559=FILL_AREA_STYLE_COLOUR('Gear light blue',#259574);
#259574=COLOUR_RGB('Gear light blue',0.662745098039216,0.831372549019608,
0.949019607843137);
ENDSEC;
END-ISO-10303-21;
